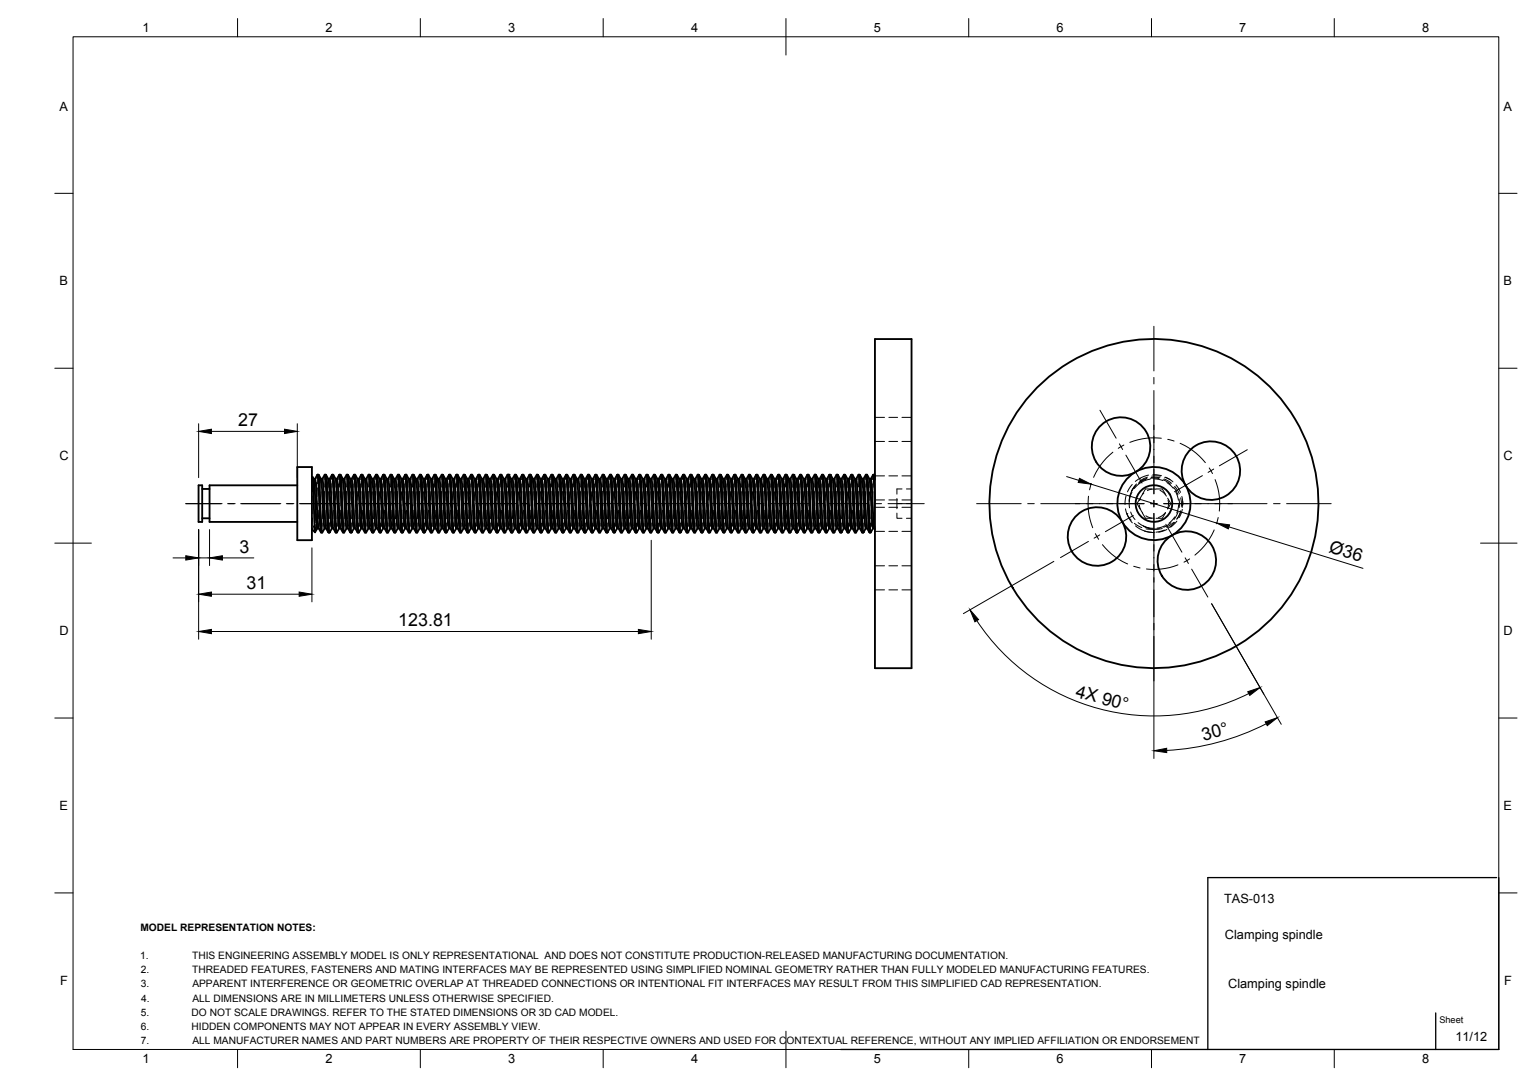
ISO-10303-21;
HEADER;
/* Generated by software containing ST-Developer
 * from STEP Tools, Inc. (www.steptools.com) 
 */

FILE_DESCRIPTION(
/* description */ (
'Independent guided parallel-jaw bracket clamp. Two12mm guide rods, re
placeable bronze sleeves, captured swiveling spindle, replaceable jaw 
pads and modeled M16x2 screw. Native slider/revolute joints linked2mm 
per revolution. Nominal opening0..122 with initial28mm. Base and two i
dentical supports welded. Standard fits, weld details and clamp load r
equire engineering selection.'),
/* implementation_level */ '2;1');

FILE_NAME(
/* name */ 'Clamping spindle.step',
/* time_stamp */ '2026-11-14T09:15:44-08:00',
/* author */ (''),
/* organization */ (''),
/* preprocessor_version */ 'ST-DEVELOPER v20.2',
/* originating_system */ 'Autodesk Translation Framework v15.17.0.0',
/* authorisation */ '');

FILE_SCHEMA (('AUTOMOTIVE_DESIGN { 1 0 10303 214 3 1 1 }'));
ENDSEC;

DATA;
#10=MECHANICAL_DESIGN_GEOMETRIC_PRESENTATION_REPRESENTATION('',(#918),#105806);
#95=B_SPLINE_SURFACE_WITH_KNOTS('',3,3,((#67139,#67140,#67141,#67142,#67143,
#67144,#67145,#67146,#67147,#67148,#67149,#67150,#67151,#67152,#67153,#67154,
#67155,#67156,#67157,#67158,#67159,#67160,#67161,#67162,#67163,#67164,#67165,
#67166,#67167,#67168,#67169,#67170,#67171,#67172,#67173,#67174,#67175,#67176,
#67177,#67178,#67179,#67180,#67181,#67182,#67183,#67184,#67185,#67186,#67187,
#67188,#67189,#67190,#67191,#67192,#67193,#67194,#67195,#67196,#67197,#67198,
#67199,#67200,#67201,#67202,#67203,#67204,#67205,#67206,#67207,#67208,#67209,
#67210,#67211,#67212,#67213,#67214,#67215,#67216,#67217,#67218,#67219,#67220,
#67221,#67222,#67223,#67224,#67225,#67226,#67227,#67228,#67229,#67230,#67231,
#67232,#67233,#67234,#67235,#67236,#67237,#67238,#67239,#67240,#67241,#67242,
#67243,#67244,#67245,#67246,#67247,#67248,#67249,#67250,#67251,#67252,#67253,
#67254,#67255,#67256,#67257,#67258,#67259,#67260,#67261,#67262,#67263,#67264,
#67265,#67266,#67267,#67268,#67269,#67270,#67271,#67272,#67273,#67274,#67275,
#67276,#67277,#67278,#67279,#67280,#67281,#67282,#67283,#67284,#67285,#67286,
#67287,#67288,#67289,#67290,#67291,#67292,#67293,#67294,#67295,#67296,#67297,
#67298,#67299,#67300,#67301,#67302,#67303,#67304,#67305,#67306,#67307,#67308,
#67309,#67310,#67311,#67312,#67313,#67314,#67315,#67316,#67317,#67318,#67319,
#67320,#67321,#67322,#67323,#67324,#67325,#67326,#67327,#67328,#67329,#67330,
#67331,#67332,#67333,#67334,#67335,#67336,#67337,#67338,#67339,#67340,#67341,
#67342,#67343,#67344,#67345,#67346,#67347,#67348,#67349,#67350,#67351,#67352,
#67353,#67354,#67355,#67356,#67357,#67358,#67359,#67360,#67361,#67362,#67363,
#67364,#67365,#67366,#67367,#67368,#67369,#67370,#67371,#67372,#67373,#67374,
#67375,#67376,#67377,#67378,#67379,#67380,#67381,#67382,#67383,#67384,#67385,
#67386,#67387,#67388,#67389,#67390,#67391,#67392,#67393,#67394,#67395,#67396,
#67397,#67398,#67399,#67400,#67401,#67402,#67403,#67404,#67405,#67406,#67407,
#67408,#67409,#67410,#67411,#67412,#67413,#67414,#67415,#67416,#67417,#67418,
#67419,#67420,#67421,#67422,#67423,#67424,#67425,#67426,#67427,#67428,#67429,
#67430,#67431,#67432,#67433,#67434,#67435,#67436,#67437,#67438,#67439,#67440,
#67441,#67442,#67443,#67444,#67445,#67446,#67447,#67448,#67449,#67450,#67451,
#67452,#67453,#67454,#67455,#67456,#67457,#67458,#67459,#67460,#67461,#67462,
#67463,#67464,#67465,#67466,#67467,#67468,#67469,#67470,#67471,#67472,#67473,
#67474,#67475,#67476,#67477,#67478,#67479,#67480,#67481,#67482,#67483,#67484,
#67485,#67486,#67487,#67488,#67489,#67490,#67491,#67492,#67493,#67494,#67495,
#67496,#67497,#67498,#67499,#67500,#67501,#67502,#67503,#67504,#67505,#67506,
#67507,#67508,#67509,#67510,#67511,#67512,#67513,#67514,#67515,#67516,#67517,
#67518,#67519,#67520,#67521,#67522,#67523,#67524,#67525,#67526,#67527,#67528,
#67529,#67530,#67531,#67532,#67533,#67534,#67535,#67536,#67537,#67538,#67539,
#67540,#67541,#67542,#67543,#67544,#67545,#67546,#67547,#67548,#67549,#67550,
#67551,#67552,#67553,#67554,#67555,#67556,#67557,#67558,#67559,#67560,#67561,
#67562,#67563,#67564,#67565,#67566,#67567,#67568,#67569,#67570,#67571,#67572,
#67573,#67574,#67575,#67576,#67577,#67578,#67579,#67580,#67581,#67582,#67583,
#67584,#67585,#67586,#67587,#67588,#67589,#67590,#67591,#67592,#67593,#67594,
#67595,#67596,#67597,#67598,#67599,#67600,#67601,#67602,#67603,#67604,#67605,
#67606,#67607,#67608,#67609,#67610,#67611,#67612,#67613,#67614,#67615,#67616,
#67617,#67618,#67619,#67620,#67621,#67622,#67623,#67624,#67625,#67626,#67627,
#67628,#67629,#67630,#67631,#67632,#67633,#67634,#67635,#67636,#67637,#67638,
#67639,#67640,#67641,#67642,#67643,#67644,#67645,#67646,#67647,#67648,#67649,
#67650,#67651,#67652,#67653,#67654,#67655,#67656,#67657,#67658,#67659,#67660,
#67661,#67662,#67663,#67664,#67665,#67666,#67667,#67668,#67669,#67670,#67671,
#67672,#67673,#67674,#67675,#67676,#67677,#67678,#67679,#67680,#67681,#67682,
#67683,#67684,#67685,#67686,#67687,#67688,#67689,#67690,#67691,#67692,#67693,
#67694,#67695,#67696),(#67697,#67698,#67699,#67700,#67701,#67702,#67703,
#67704,#67705,#67706,#67707,#67708,#67709,#67710,#67711,#67712,#67713,#67714,
#67715,#67716,#67717,#67718,#67719,#67720,#67721,#67722,#67723,#67724,#67725,
#67726,#67727,#67728,#67729,#67730,#67731,#67732,#67733,#67734,#67735,#67736,
#67737,#67738,#67739,#67740,#67741,#67742,#67743,#67744,#67745,#67746,#67747,
#67748,#67749,#67750,#67751,#67752,#67753,#67754,#67755,#67756,#67757,#67758,
#67759,#67760,#67761,#67762,#67763,#67764,#67765,#67766,#67767,#67768,#67769,
#67770,#67771,#67772,#67773,#67774,#67775,#67776,#67777,#67778,#67779,#67780,
#67781,#67782,#67783,#67784,#67785,#67786,#67787,#67788,#67789,#67790,#67791,
#67792,#67793,#67794,#67795,#67796,#67797,#67798,#67799,#67800,#67801,#67802,
#67803,#67804,#67805,#67806,#67807,#67808,#67809,#67810,#67811,#67812,#67813,
#67814,#67815,#67816,#67817,#67818,#67819,#67820,#67821,#67822,#67823,#67824,
#67825,#67826,#67827,#67828,#67829,#67830,#67831,#67832,#67833,#67834,#67835,
#67836,#67837,#67838,#67839,#67840,#67841,#67842,#67843,#67844,#67845,#67846,
#67847,#67848,#67849,#67850,#67851,#67852,#67853,#67854,#67855,#67856,#67857,
#67858,#67859,#67860,#67861,#67862,#67863,#67864,#67865,#67866,#67867,#67868,
#67869,#67870,#67871,#67872,#67873,#67874,#67875,#67876,#67877,#67878,#67879,
#67880,#67881,#67882,#67883,#67884,#67885,#67886,#67887,#67888,#67889,#67890,
#67891,#67892,#67893,#67894,#67895,#67896,#67897,#67898,#67899,#67900,#67901,
#67902,#67903,#67904,#67905,#67906,#67907,#67908,#67909,#67910,#67911,#67912,
#67913,#67914,#67915,#67916,#67917,#67918,#67919,#67920,#67921,#67922,#67923,
#67924,#67925,#67926,#67927,#67928,#67929,#67930,#67931,#67932,#67933,#67934,
#67935,#67936,#67937,#67938,#67939,#67940,#67941,#67942,#67943,#67944,#67945,
#67946,#67947,#67948,#67949,#67950,#67951,#67952,#67953,#67954,#67955,#67956,
#67957,#67958,#67959,#67960,#67961,#67962,#67963,#67964,#67965,#67966,#67967,
#67968,#67969,#67970,#67971,#67972,#67973,#67974,#67975,#67976,#67977,#67978,
#67979,#67980,#67981,#67982,#67983,#67984,#67985,#67986,#67987,#67988,#67989,
#67990,#67991,#67992,#67993,#67994,#67995,#67996,#67997,#67998,#67999,#68000,
#68001,#68002,#68003,#68004,#68005,#68006,#68007,#68008,#68009,#68010,#68011,
#68012,#68013,#68014,#68015,#68016,#68017,#68018,#68019,#68020,#68021,#68022,
#68023,#68024,#68025,#68026,#68027,#68028,#68029,#68030,#68031,#68032,#68033,
#68034,#68035,#68036,#68037,#68038,#68039,#68040,#68041,#68042,#68043,#68044,
#68045,#68046,#68047,#68048,#68049,#68050,#68051,#68052,#68053,#68054,#68055,
#68056,#68057,#68058,#68059,#68060,#68061,#68062,#68063,#68064,#68065,#68066,
#68067,#68068,#68069,#68070,#68071,#68072,#68073,#68074,#68075,#68076,#68077,
#68078,#68079,#68080,#68081,#68082,#68083,#68084,#68085,#68086,#68087,#68088,
#68089,#68090,#68091,#68092,#68093,#68094,#68095,#68096,#68097,#68098,#68099,
#68100,#68101,#68102,#68103,#68104,#68105,#68106,#68107,#68108,#68109,#68110,
#68111,#68112,#68113,#68114,#68115,#68116,#68117,#68118,#68119,#68120,#68121,
#68122,#68123,#68124,#68125,#68126,#68127,#68128,#68129,#68130,#68131,#68132,
#68133,#68134,#68135,#68136,#68137,#68138,#68139,#68140,#68141,#68142,#68143,
#68144,#68145,#68146,#68147,#68148,#68149,#68150,#68151,#68152,#68153,#68154,
#68155,#68156,#68157,#68158,#68159,#68160,#68161,#68162,#68163,#68164,#68165,
#68166,#68167,#68168,#68169,#68170,#68171,#68172,#68173,#68174,#68175,#68176,
#68177,#68178,#68179,#68180,#68181,#68182,#68183,#68184,#68185,#68186,#68187,
#68188,#68189,#68190,#68191,#68192,#68193,#68194,#68195,#68196,#68197,#68198,
#68199,#68200,#68201,#68202,#68203,#68204,#68205,#68206,#68207,#68208,#68209,
#68210,#68211,#68212,#68213,#68214,#68215,#68216,#68217,#68218,#68219,#68220,
#68221,#68222,#68223,#68224,#68225,#68226,#68227,#68228,#68229,#68230,#68231,
#68232,#68233,#68234,#68235,#68236,#68237,#68238,#68239,#68240,#68241,#68242,
#68243,#68244,#68245,#68246,#68247,#68248,#68249,#68250,#68251,#68252,#68253,
#68254),(#68255,#68256,#68257,#68258,#68259,#68260,#68261,#68262,#68263,
#68264,#68265,#68266,#68267,#68268,#68269,#68270,#68271,#68272,#68273,#68274,
#68275,#68276,#68277,#68278,#68279,#68280,#68281,#68282,#68283,#68284,#68285,
#68286,#68287,#68288,#68289,#68290,#68291,#68292,#68293,#68294,#68295,#68296,
#68297,#68298,#68299,#68300,#68301,#68302,#68303,#68304,#68305,#68306,#68307,
#68308,#68309,#68310,#68311,#68312,#68313,#68314,#68315,#68316,#68317,#68318,
#68319,#68320,#68321,#68322,#68323,#68324,#68325,#68326,#68327,#68328,#68329,
#68330,#68331,#68332,#68333,#68334,#68335,#68336,#68337,#68338,#68339,#68340,
#68341,#68342,#68343,#68344,#68345,#68346,#68347,#68348,#68349,#68350,#68351,
#68352,#68353,#68354,#68355,#68356,#68357,#68358,#68359,#68360,#68361,#68362,
#68363,#68364,#68365,#68366,#68367,#68368,#68369,#68370,#68371,#68372,#68373,
#68374,#68375,#68376,#68377,#68378,#68379,#68380,#68381,#68382,#68383,#68384,
#68385,#68386,#68387,#68388,#68389,#68390,#68391,#68392,#68393,#68394,#68395,
#68396,#68397,#68398,#68399,#68400,#68401,#68402,#68403,#68404,#68405,#68406,
#68407,#68408,#68409,#68410,#68411,#68412,#68413,#68414,#68415,#68416,#68417,
#68418,#68419,#68420,#68421,#68422,#68423,#68424,#68425,#68426,#68427,#68428,
#68429,#68430,#68431,#68432,#68433,#68434,#68435,#68436,#68437,#68438,#68439,
#68440,#68441,#68442,#68443,#68444,#68445,#68446,#68447,#68448,#68449,#68450,
#68451,#68452,#68453,#68454,#68455,#68456,#68457,#68458,#68459,#68460,#68461,
#68462,#68463,#68464,#68465,#68466,#68467,#68468,#68469,#68470,#68471,#68472,
#68473,#68474,#68475,#68476,#68477,#68478,#68479,#68480,#68481,#68482,#68483,
#68484,#68485,#68486,#68487,#68488,#68489,#68490,#68491,#68492,#68493,#68494,
#68495,#68496,#68497,#68498,#68499,#68500,#68501,#68502,#68503,#68504,#68505,
#68506,#68507,#68508,#68509,#68510,#68511,#68512,#68513,#68514,#68515,#68516,
#68517,#68518,#68519,#68520,#68521,#68522,#68523,#68524,#68525,#68526,#68527,
#68528,#68529,#68530,#68531,#68532,#68533,#68534,#68535,#68536,#68537,#68538,
#68539,#68540,#68541,#68542,#68543,#68544,#68545,#68546,#68547,#68548,#68549,
#68550,#68551,#68552,#68553,#68554,#68555,#68556,#68557,#68558,#68559,#68560,
#68561,#68562,#68563,#68564,#68565,#68566,#68567,#68568,#68569,#68570,#68571,
#68572,#68573,#68574,#68575,#68576,#68577,#68578,#68579,#68580,#68581,#68582,
#68583,#68584,#68585,#68586,#68587,#68588,#68589,#68590,#68591,#68592,#68593,
#68594,#68595,#68596,#68597,#68598,#68599,#68600,#68601,#68602,#68603,#68604,
#68605,#68606,#68607,#68608,#68609,#68610,#68611,#68612,#68613,#68614,#68615,
#68616,#68617,#68618,#68619,#68620,#68621,#68622,#68623,#68624,#68625,#68626,
#68627,#68628,#68629,#68630,#68631,#68632,#68633,#68634,#68635,#68636,#68637,
#68638,#68639,#68640,#68641,#68642,#68643,#68644,#68645,#68646,#68647,#68648,
#68649,#68650,#68651,#68652,#68653,#68654,#68655,#68656,#68657,#68658,#68659,
#68660,#68661,#68662,#68663,#68664,#68665,#68666,#68667,#68668,#68669,#68670,
#68671,#68672,#68673,#68674,#68675,#68676,#68677,#68678,#68679,#68680,#68681,
#68682,#68683,#68684,#68685,#68686,#68687,#68688,#68689,#68690,#68691,#68692,
#68693,#68694,#68695,#68696,#68697,#68698,#68699,#68700,#68701,#68702,#68703,
#68704,#68705,#68706,#68707,#68708,#68709,#68710,#68711,#68712,#68713,#68714,
#68715,#68716,#68717,#68718,#68719,#68720,#68721,#68722,#68723,#68724,#68725,
#68726,#68727,#68728,#68729,#68730,#68731,#68732,#68733,#68734,#68735,#68736,
#68737,#68738,#68739,#68740,#68741,#68742,#68743,#68744,#68745,#68746,#68747,
#68748,#68749,#68750,#68751,#68752,#68753,#68754,#68755,#68756,#68757,#68758,
#68759,#68760,#68761,#68762,#68763,#68764,#68765,#68766,#68767,#68768,#68769,
#68770,#68771,#68772,#68773,#68774,#68775,#68776,#68777,#68778,#68779,#68780,
#68781,#68782,#68783,#68784,#68785,#68786,#68787,#68788,#68789,#68790,#68791,
#68792,#68793,#68794,#68795,#68796,#68797,#68798,#68799,#68800,#68801,#68802,
#68803,#68804,#68805,#68806,#68807,#68808,#68809,#68810,#68811,#68812),
(#68813,#68814,#68815,#68816,#68817,#68818,#68819,#68820,#68821,#68822,
#68823,#68824,#68825,#68826,#68827,#68828,#68829,#68830,#68831,#68832,#68833,
#68834,#68835,#68836,#68837,#68838,#68839,#68840,#68841,#68842,#68843,#68844,
#68845,#68846,#68847,#68848,#68849,#68850,#68851,#68852,#68853,#68854,#68855,
#68856,#68857,#68858,#68859,#68860,#68861,#68862,#68863,#68864,#68865,#68866,
#68867,#68868,#68869,#68870,#68871,#68872,#68873,#68874,#68875,#68876,#68877,
#68878,#68879,#68880,#68881,#68882,#68883,#68884,#68885,#68886,#68887,#68888,
#68889,#68890,#68891,#68892,#68893,#68894,#68895,#68896,#68897,#68898,#68899,
#68900,#68901,#68902,#68903,#68904,#68905,#68906,#68907,#68908,#68909,#68910,
#68911,#68912,#68913,#68914,#68915,#68916,#68917,#68918,#68919,#68920,#68921,
#68922,#68923,#68924,#68925,#68926,#68927,#68928,#68929,#68930,#68931,#68932,
#68933,#68934,#68935,#68936,#68937,#68938,#68939,#68940,#68941,#68942,#68943,
#68944,#68945,#68946,#68947,#68948,#68949,#68950,#68951,#68952,#68953,#68954,
#68955,#68956,#68957,#68958,#68959,#68960,#68961,#68962,#68963,#68964,#68965,
#68966,#68967,#68968,#68969,#68970,#68971,#68972,#68973,#68974,#68975,#68976,
#68977,#68978,#68979,#68980,#68981,#68982,#68983,#68984,#68985,#68986,#68987,
#68988,#68989,#68990,#68991,#68992,#68993,#68994,#68995,#68996,#68997,#68998,
#68999,#69000,#69001,#69002,#69003,#69004,#69005,#69006,#69007,#69008,#69009,
#69010,#69011,#69012,#69013,#69014,#69015,#69016,#69017,#69018,#69019,#69020,
#69021,#69022,#69023,#69024,#69025,#69026,#69027,#69028,#69029,#69030,#69031,
#69032,#69033,#69034,#69035,#69036,#69037,#69038,#69039,#69040,#69041,#69042,
#69043,#69044,#69045,#69046,#69047,#69048,#69049,#69050,#69051,#69052,#69053,
#69054,#69055,#69056,#69057,#69058,#69059,#69060,#69061,#69062,#69063,#69064,
#69065,#69066,#69067,#69068,#69069,#69070,#69071,#69072,#69073,#69074,#69075,
#69076,#69077,#69078,#69079,#69080,#69081,#69082,#69083,#69084,#69085,#69086,
#69087,#69088,#69089,#69090,#69091,#69092,#69093,#69094,#69095,#69096,#69097,
#69098,#69099,#69100,#69101,#69102,#69103,#69104,#69105,#69106,#69107,#69108,
#69109,#69110,#69111,#69112,#69113,#69114,#69115,#69116,#69117,#69118,#69119,
#69120,#69121,#69122,#69123,#69124,#69125,#69126,#69127,#69128,#69129,#69130,
#69131,#69132,#69133,#69134,#69135,#69136,#69137,#69138,#69139,#69140,#69141,
#69142,#69143,#69144,#69145,#69146,#69147,#69148,#69149,#69150,#69151,#69152,
#69153,#69154,#69155,#69156,#69157,#69158,#69159,#69160,#69161,#69162,#69163,
#69164,#69165,#69166,#69167,#69168,#69169,#69170,#69171,#69172,#69173,#69174,
#69175,#69176,#69177,#69178,#69179,#69180,#69181,#69182,#69183,#69184,#69185,
#69186,#69187,#69188,#69189,#69190,#69191,#69192,#69193,#69194,#69195,#69196,
#69197,#69198,#69199,#69200,#69201,#69202,#69203,#69204,#69205,#69206,#69207,
#69208,#69209,#69210,#69211,#69212,#69213,#69214,#69215,#69216,#69217,#69218,
#69219,#69220,#69221,#69222,#69223,#69224,#69225,#69226,#69227,#69228,#69229,
#69230,#69231,#69232,#69233,#69234,#69235,#69236,#69237,#69238,#69239,#69240,
#69241,#69242,#69243,#69244,#69245,#69246,#69247,#69248,#69249,#69250,#69251,
#69252,#69253,#69254,#69255,#69256,#69257,#69258,#69259,#69260,#69261,#69262,
#69263,#69264,#69265,#69266,#69267,#69268,#69269,#69270,#69271,#69272,#69273,
#69274,#69275,#69276,#69277,#69278,#69279,#69280,#69281,#69282,#69283,#69284,
#69285,#69286,#69287,#69288,#69289,#69290,#69291,#69292,#69293,#69294,#69295,
#69296,#69297,#69298,#69299,#69300,#69301,#69302,#69303,#69304,#69305,#69306,
#69307,#69308,#69309,#69310,#69311,#69312,#69313,#69314,#69315,#69316,#69317,
#69318,#69319,#69320,#69321,#69322,#69323,#69324,#69325,#69326,#69327,#69328,
#69329,#69330,#69331,#69332,#69333,#69334,#69335,#69336,#69337,#69338,#69339,
#69340,#69341,#69342,#69343,#69344,#69345,#69346,#69347,#69348,#69349,#69350,
#69351,#69352,#69353,#69354,#69355,#69356,#69357,#69358,#69359,#69360,#69361,
#69362,#69363,#69364,#69365,#69366,#69367,#69368,#69369,#69370)),
 .UNSPECIFIED.,.F.,.F.,.F.,(4,4),(4,1,1,1,1,1,1,1,1,1,1,1,1,1,1,1,1,1,1,
1,1,1,1,1,1,1,1,1,1,1,1,1,1,1,1,1,1,1,1,1,1,1,1,1,1,1,1,1,1,1,1,1,1,1,1,
1,1,1,1,1,1,1,1,1,1,1,1,1,1,1,1,1,1,1,1,1,1,1,1,1,1,1,1,1,1,1,1,1,1,1,1,
1,1,1,1,1,1,1,1,1,1,1,1,1,1,1,1,1,1,1,1,1,1,1,1,1,1,1,1,1,1,1,1,1,1,1,1,
1,1,1,1,1,1,1,1,1,1,1,1,1,1,1,1,1,1,1,1,1,1,1,1,1,1,1,1,1,1,1,1,1,1,1,1,
1,1,1,1,1,1,1,1,1,1,1,1,1,1,1,1,1,1,1,1,1,1,1,1,1,1,1,1,1,1,1,1,1,1,1,1,
1,1,1,1,1,1,1,1,1,1,1,1,1,1,1,1,1,1,1,1,1,1,1,1,1,1,1,1,1,1,1,1,1,1,1,1,
1,1,1,1,1,1,1,1,1,1,1,1,1,1,1,1,1,1,1,1,1,1,1,1,1,1,1,1,1,1,1,1,1,1,1,1,
1,1,1,1,1,1,1,1,1,1,1,1,1,1,1,1,1,1,1,1,1,1,1,1,1,1,1,1,1,1,1,1,1,1,1,1,
1,1,1,1,1,1,1,1,1,1,1,1,1,1,1,1,1,1,1,1,1,1,1,1,1,1,1,1,1,1,1,1,1,1,1,1,
1,1,1,1,1,1,1,1,1,1,1,1,1,1,1,1,1,1,1,1,1,1,1,1,1,1,1,1,1,1,1,1,1,1,1,1,
1,1,1,1,1,1,1,1,1,1,1,1,1,1,1,1,1,1,1,1,1,1,1,1,1,1,1,1,1,1,1,1,1,1,1,1,
1,1,1,1,1,1,1,1,1,1,1,1,1,1,1,1,1,1,1,1,1,1,1,1,1,1,1,1,1,1,1,1,1,1,1,1,
1,1,1,1,1,1,1,1,1,1,1,1,1,1,1,1,1,1,1,1,1,1,1,1,1,1,1,1,1,1,1,1,1,1,1,1,
1,1,1,1,1,1,1,1,1,1,1,1,1,1,1,1,1,1,1,1,1,1,1,1,1,1,1,1,1,1,1,1,1,1,1,1,
1,1,1,1,1,1,1,1,1,1,1,1,1,1,1,1,1,1,1,1,1,1,1,1,1,1,1,1,1,1,1,1,4),(-0.00312009804042434,
0.132901482941916),(11.6144980695961,12.1142368518449,12.6134408558704,
13.6118488639213,14.6102568719722,15.6086648800232,16.6070728880741,17.605480896125,
18.1046849001504,18.6038889041759,19.6022969122268,20.6007049202777,21.5991129283287,
22.5975209363796,23.5959289444305,24.5943369524814,25.0935409565069,25.5927449605323,
26.5911529685832,27.5895609766342,28.5879689846851,29.586376992736,30.5847850007869,
31.5831930088378,32.0823970128633,32.5816010168887,33.5800090249397,34.5784170329906,
35.5768250410415,36.5752330490924,37.5736410571433,38.5720490651942,39.0712530692197,
39.5704570732452,40.5688650812961,41.567273089347,42.5656810973979,43.5640891054488,
44.5624971134997,45.5609051215507,46.0601091255761,46.5593131296016,47.5577211376525,
48.5561291457034,49.5545371537543,50.5529451618052,51.5513531698562,52.5497611779071,
53.0489651819325,53.548169185958,54.5465771940089,55.5449852020598,56.5433932101108,
57.5418012181617,58.5402092262126,59.5386172342635,60.037821238289,60.5370252423144,
61.5354332503653,62.5338412584163,63.5322492664672,64.5306572745181,65.529065282569,
66.5274732906199,67.0266772946454,67.5258812986708,68.5242893067218,69.5226973147727,
70.5211053228236,71.5195133308745,72.5179213389254,73.5163293469763,74.0155333510018,
74.5147373550273,75.5131453630782,76.5115533711291,77.50996137918,78.5083693872309,
79.5067773952818,80.5051854033328,81.0043894073582,81.5035934113837,82.5020014194346,
83.5004094274855,84.4988174355364,85.4972254435874,86.4956334516383,87.4940414596892,
87.9932454637146,88.4924494677401,89.490857475791,90.4892654838419,91.4876734918928,
92.4860814999438,93.4844895079947,94.4828975160456,94.9821015200711,95.4813055240965,
96.4797135321474,97.4781215401984,98.4765295482493,99.4749375563002,100.473345564351,
101.471753572402,101.970957576427,102.470161580453,103.468569588504,104.466977596555,
105.465385604606,106.463793612657,107.462201620708,108.460609628758,108.959813632784,
109.459017636809,110.45742564486,111.455833652911,112.454241660962,113.452649669013,
114.451057677064,115.449465685115,115.94866968914,116.447873693166,117.446281701217,
118.444689709268,119.443097717319,120.441505725369,121.43991373342,122.438321741471,
122.937525745497,123.436729749522,124.435137757573,125.433545765624,126.431953773675,
127.430361781726,128.428769789777,129.427177797828,129.926381801853,130.425585805879,
131.42399381393,132.42240182198,133.420809830031,134.419217838082,135.417625846133,
136.416033854184,136.91523785821,137.414441862235,138.412849870286,139.411257878337,
140.409665886388,141.408073894439,142.40648190249,143.404889910541,143.904093914566,
144.403297918591,145.401705926642,146.400113934693,147.398521942744,148.396929950795,
149.395337958846,150.393745966897,150.892949970922,151.392153974948,152.390561982999,
153.38896999105,154.387377999101,155.385786007152,156.384194015202,157.382602023253,
157.881806027279,158.381010031304,159.379418039355,160.377826047406,161.376234055457,
162.374642063508,163.373050071559,164.37145807961,164.870662083635,165.369866087661,
166.368274095712,167.366682103763,168.365090111813,169.363498119864,170.361906127915,
171.360314135966,171.859518139992,172.358722144017,173.357130152068,174.355538160119,
175.35394616817,176.352354176221,177.350762184272,178.349170192323,178.848374196348,
179.347578200374,180.345986208424,181.344394216475,182.342802224526,183.341210232577,
184.339618240628,185.338026248679,185.837230252705,186.33643425673,187.334842264781,
188.333250272832,189.331658280883,190.330066288934,191.328474296985,192.326882305035,
192.826086309061,193.325290313086,194.323698321137,195.322106329188,196.320514337239,
197.31892234529,198.317330353341,199.315738361392,199.814942365417,200.314146369443,
201.312554377494,202.310962385545,203.309370393596,204.307778401646,205.306186409697,
206.304594417748,206.803798421774,207.303002425799,208.30141043385,209.299818441901,
210.298226449952,211.296634458003,212.295042466054,213.293450474105,213.79265447813,
214.291858482156,215.290266490207,216.288674498257,217.287082506308,218.285490514359,
219.28389852241,220.282306530461,220.781510534487,221.280714538512,222.279122546563,
223.277530554614,224.275938562665,225.274346570716,226.272754578767,227.271162586818,
227.770366590843,228.269570594868,229.267978602919,230.26638661097,231.264794619021,
232.263202627072,233.261610635123,234.260018643174,234.759222647199,235.258426651225,
236.256834659276,237.255242667327,238.253650675378,239.252058683429,240.250466691479,
241.24887469953,241.748078703556,242.247282707581,243.245690715632,244.244098723683,
245.242506731734,246.240914739785,247.239322747836,248.237730755887,248.736934759912,
249.236138763938,250.234546771989,251.23295478004,252.23136278809,253.229770796141,
254.228178804192,255.226586812243,256.224994820294,257.223402828345,258.221810836396,
258.721014840421,259.220218844447,260.218626852498,261.217034860549,262.2154428686,
263.213850876651,264.212258884701,265.210666892752,265.709870896778,266.209074900803,
267.207482908854,268.205890916905,269.204298924956,270.202706933007,271.201114941058,
272.199522949109,272.698726953134,273.19793095716,274.196338965211,275.194746973262,
276.193154981312,277.191562989363,278.189970997414,279.188379005465,279.687583009491,
280.186787013516,281.185195021567,282.183603029618,283.182011037669,284.18041904572,
285.178827053771,286.177235061822,286.676439065847,287.175643069873,288.174051077923,
289.172459085974,290.170867094025,291.169275102076,292.167683110127,293.166091118178,
293.665295122204,294.164499126229,295.16290713428,296.161315142331,297.159723150382,
298.158131158433,299.156539166484,300.154947174534,300.65415117856,301.153355182585,
302.151763190636,303.150171198687,304.148579206738,305.146987214789,306.14539522284,
307.143803230891,307.643007234916,308.142211238942,309.140619246993,310.139027255044,
311.137435263095,312.135843271145,313.134251279196,314.132659287247,314.631863291273,
315.131067295298,316.129475303349,317.1278833114,318.126291319451,319.124699327502,
320.123107335553,321.121515343604,321.620719347629,322.119923351655,323.118331359706,
324.116739367757,325.115147375807,326.113555383858,327.111963391909,328.11037139996,
328.609575403986,329.108779408011,330.107187416062,331.105595424113,332.104003432164,
333.102411440215,334.100819448266,335.099227456317,335.598431460342,336.097635464367,
337.096043472418,338.094451480469,339.09285948852,340.091267496571,341.089675504622,
342.088083512673,342.587287516698,343.086491520724,344.084899528775,345.083307536826,
346.081715544877,347.080123552928,348.078531560978,349.076939569029,349.576143573055,
350.07534757708,351.073755585131,352.072163593182,353.070571601233,354.068979609284,
355.067387617335,356.065795625386,356.564999629411,357.064203633437,358.062611641488,
359.061019649539,360.059427657589,361.05783566564,362.056243673691,363.054651681742,
363.553855685768,364.053059689793,365.051467697844,366.049875705895,367.048283713946,
368.046691721997,369.045099730048,370.043507738099,370.542711742124,371.04191574615,
372.040323754201,373.038731762251,374.037139770302,375.035547778353,376.033955786404,
377.032363794455,377.531567798481,378.030771802506,379.029179810557,380.027587818608,
381.025995826659,382.02440383471,383.022811842761,384.021219850812,384.520423854837,
385.019627858862,386.018035866913,387.016443874964,388.014851883015,389.013259891066,
390.011667899117,391.010075907168,391.509279911193,392.008483915219,393.00689192327,
394.005299931321,395.003707939372,396.002115947423,397.000523955473,397.998931963524,
398.49813596755,398.997339971575,399.995747979626,400.994155987677,401.992563995728,
402.990972003779,403.98938001183,404.987788019881,405.486992023906,405.986196027932,
406.984604035983,407.983012044034,408.981420052084,409.979828060135,410.978236068186,
411.976644076237,412.475848080263,412.975052084288,413.973460092339,414.97186810039,
415.970276108441,416.968684116492,417.967092124543,418.965500132594,419.464704136619,
419.963908140644,420.962316148695,421.960724156746,422.959132164797,423.957540172848,
424.955948180899,425.95435618895,426.453560192975,426.952764197001,427.951172205052,
428.949580213103,429.947988221154,430.946396229205,431.944804237256,432.943212245306,
433.442416249332,433.941620253357,434.940028261408,435.938436269459,436.93684427751,
437.935252285561,438.933660293612,439.932068301663,440.431272305688,440.930476309714,
441.928884317765,442.927292325816,443.925700333867,444.924108341917,445.922516349968,
446.920924358019,447.420128362045,447.91933236607,448.917740374121,449.916148382172,
450.914556390223,451.912964398274,452.911372406325,453.909780414376,454.408984418401,
454.908188422427,455.906596430478,456.905004438528,457.903412446579,458.90182045463,
459.900228462681,460.898636470732,461.397840474758,461.897044478783,462.895452486834,
463.893860494885,464.892268502936,465.890676510987,466.889084519038,467.887492527089,
468.386696531114,468.885900535139,469.88430854319,470.882716551241,471.881124559292,
472.879532567343,473.877940575394,474.876348583445,475.37555258747,475.874756591496,
476.873164599547,477.871572607598,478.869980615649,479.8683886237,480.86679663175,
481.865204639801,482.364408643827,482.863612647852,483.862020655903,484.860428663954,
485.858836672005,486.857244680056,487.855652688107,488.854060696158,489.353264700183,
489.852468704209,490.85087671226,491.849284720311,492.847692728361,493.846100736412,
494.844508744463,495.343712748489,495.842949180242),.UNSPECIFIED.);
#96=B_SPLINE_SURFACE_WITH_KNOTS('',3,3,((#69480,#69481,#69482,#69483,#69484,
#69485,#69486,#69487,#69488,#69489,#69490,#69491,#69492,#69493,#69494,#69495,
#69496,#69497,#69498,#69499,#69500,#69501,#69502,#69503,#69504,#69505,#69506,
#69507,#69508,#69509,#69510,#69511,#69512,#69513,#69514,#69515,#69516,#69517,
#69518,#69519,#69520,#69521,#69522,#69523,#69524,#69525,#69526,#69527,#69528,
#69529,#69530,#69531,#69532,#69533,#69534,#69535,#69536,#69537,#69538,#69539,
#69540,#69541,#69542,#69543,#69544,#69545,#69546,#69547,#69548,#69549,#69550,
#69551,#69552,#69553,#69554,#69555,#69556,#69557,#69558,#69559,#69560,#69561,
#69562,#69563,#69564,#69565,#69566,#69567,#69568,#69569,#69570,#69571,#69572,
#69573,#69574,#69575,#69576,#69577,#69578,#69579,#69580,#69581,#69582,#69583,
#69584,#69585,#69586,#69587,#69588,#69589,#69590,#69591,#69592,#69593,#69594,
#69595,#69596,#69597,#69598,#69599,#69600,#69601,#69602,#69603,#69604,#69605,
#69606,#69607,#69608,#69609,#69610,#69611,#69612,#69613,#69614,#69615,#69616,
#69617,#69618,#69619,#69620,#69621,#69622,#69623,#69624,#69625,#69626,#69627,
#69628,#69629,#69630,#69631,#69632,#69633,#69634,#69635,#69636,#69637,#69638,
#69639,#69640,#69641,#69642,#69643,#69644,#69645,#69646,#69647,#69648,#69649,
#69650,#69651,#69652,#69653,#69654,#69655,#69656,#69657,#69658,#69659,#69660,
#69661,#69662,#69663,#69664,#69665,#69666,#69667,#69668,#69669,#69670,#69671,
#69672,#69673,#69674,#69675,#69676,#69677,#69678,#69679,#69680,#69681,#69682,
#69683,#69684,#69685,#69686,#69687,#69688,#69689,#69690,#69691,#69692,#69693,
#69694,#69695,#69696,#69697,#69698,#69699,#69700,#69701,#69702,#69703,#69704,
#69705,#69706,#69707,#69708,#69709,#69710,#69711,#69712,#69713,#69714,#69715,
#69716,#69717,#69718,#69719,#69720,#69721,#69722,#69723,#69724,#69725,#69726,
#69727,#69728,#69729,#69730,#69731,#69732,#69733,#69734,#69735,#69736,#69737,
#69738,#69739,#69740,#69741,#69742,#69743,#69744,#69745,#69746,#69747,#69748,
#69749,#69750,#69751,#69752,#69753,#69754,#69755,#69756,#69757,#69758,#69759,
#69760,#69761,#69762,#69763,#69764,#69765,#69766,#69767,#69768,#69769,#69770,
#69771,#69772,#69773,#69774,#69775,#69776,#69777,#69778,#69779,#69780,#69781,
#69782,#69783,#69784,#69785,#69786,#69787,#69788,#69789,#69790,#69791,#69792,
#69793,#69794,#69795,#69796,#69797,#69798,#69799,#69800,#69801,#69802,#69803,
#69804,#69805,#69806,#69807,#69808,#69809,#69810,#69811,#69812,#69813,#69814,
#69815,#69816,#69817,#69818,#69819,#69820,#69821,#69822,#69823,#69824,#69825,
#69826,#69827,#69828,#69829,#69830,#69831,#69832,#69833,#69834,#69835,#69836,
#69837,#69838,#69839,#69840,#69841,#69842,#69843,#69844,#69845,#69846,#69847,
#69848,#69849,#69850,#69851,#69852,#69853,#69854,#69855,#69856,#69857,#69858,
#69859,#69860,#69861,#69862,#69863,#69864,#69865,#69866,#69867,#69868,#69869,
#69870,#69871,#69872,#69873,#69874,#69875,#69876,#69877,#69878,#69879,#69880,
#69881,#69882,#69883,#69884,#69885,#69886,#69887,#69888,#69889,#69890,#69891,
#69892,#69893,#69894,#69895,#69896,#69897,#69898,#69899,#69900,#69901,#69902,
#69903,#69904,#69905,#69906,#69907,#69908,#69909,#69910,#69911,#69912,#69913,
#69914,#69915,#69916,#69917,#69918,#69919,#69920,#69921,#69922,#69923,#69924,
#69925,#69926,#69927,#69928,#69929,#69930,#69931,#69932,#69933,#69934,#69935,
#69936,#69937,#69938,#69939,#69940,#69941,#69942,#69943,#69944,#69945,#69946,
#69947,#69948,#69949,#69950,#69951,#69952,#69953,#69954,#69955,#69956,#69957,
#69958,#69959,#69960,#69961,#69962,#69963,#69964,#69965,#69966,#69967,#69968,
#69969,#69970,#69971,#69972,#69973,#69974,#69975,#69976,#69977,#69978,#69979,
#69980,#69981,#69982,#69983,#69984,#69985,#69986,#69987,#69988,#69989,#69990,
#69991,#69992,#69993,#69994,#69995,#69996,#69997,#69998,#69999,#70000,#70001,
#70002,#70003,#70004,#70005,#70006,#70007,#70008,#70009,#70010,#70011,#70012,
#70013,#70014,#70015,#70016,#70017,#70018,#70019,#70020,#70021,#70022,#70023,
#70024,#70025,#70026,#70027,#70028,#70029,#70030,#70031,#70032,#70033,#70034,
#70035,#70036,#70037,#70038),(#70039,#70040,#70041,#70042,#70043,#70044,
#70045,#70046,#70047,#70048,#70049,#70050,#70051,#70052,#70053,#70054,#70055,
#70056,#70057,#70058,#70059,#70060,#70061,#70062,#70063,#70064,#70065,#70066,
#70067,#70068,#70069,#70070,#70071,#70072,#70073,#70074,#70075,#70076,#70077,
#70078,#70079,#70080,#70081,#70082,#70083,#70084,#70085,#70086,#70087,#70088,
#70089,#70090,#70091,#70092,#70093,#70094,#70095,#70096,#70097,#70098,#70099,
#70100,#70101,#70102,#70103,#70104,#70105,#70106,#70107,#70108,#70109,#70110,
#70111,#70112,#70113,#70114,#70115,#70116,#70117,#70118,#70119,#70120,#70121,
#70122,#70123,#70124,#70125,#70126,#70127,#70128,#70129,#70130,#70131,#70132,
#70133,#70134,#70135,#70136,#70137,#70138,#70139,#70140,#70141,#70142,#70143,
#70144,#70145,#70146,#70147,#70148,#70149,#70150,#70151,#70152,#70153,#70154,
#70155,#70156,#70157,#70158,#70159,#70160,#70161,#70162,#70163,#70164,#70165,
#70166,#70167,#70168,#70169,#70170,#70171,#70172,#70173,#70174,#70175,#70176,
#70177,#70178,#70179,#70180,#70181,#70182,#70183,#70184,#70185,#70186,#70187,
#70188,#70189,#70190,#70191,#70192,#70193,#70194,#70195,#70196,#70197,#70198,
#70199,#70200,#70201,#70202,#70203,#70204,#70205,#70206,#70207,#70208,#70209,
#70210,#70211,#70212,#70213,#70214,#70215,#70216,#70217,#70218,#70219,#70220,
#70221,#70222,#70223,#70224,#70225,#70226,#70227,#70228,#70229,#70230,#70231,
#70232,#70233,#70234,#70235,#70236,#70237,#70238,#70239,#70240,#70241,#70242,
#70243,#70244,#70245,#70246,#70247,#70248,#70249,#70250,#70251,#70252,#70253,
#70254,#70255,#70256,#70257,#70258,#70259,#70260,#70261,#70262,#70263,#70264,
#70265,#70266,#70267,#70268,#70269,#70270,#70271,#70272,#70273,#70274,#70275,
#70276,#70277,#70278,#70279,#70280,#70281,#70282,#70283,#70284,#70285,#70286,
#70287,#70288,#70289,#70290,#70291,#70292,#70293,#70294,#70295,#70296,#70297,
#70298,#70299,#70300,#70301,#70302,#70303,#70304,#70305,#70306,#70307,#70308,
#70309,#70310,#70311,#70312,#70313,#70314,#70315,#70316,#70317,#70318,#70319,
#70320,#70321,#70322,#70323,#70324,#70325,#70326,#70327,#70328,#70329,#70330,
#70331,#70332,#70333,#70334,#70335,#70336,#70337,#70338,#70339,#70340,#70341,
#70342,#70343,#70344,#70345,#70346,#70347,#70348,#70349,#70350,#70351,#70352,
#70353,#70354,#70355,#70356,#70357,#70358,#70359,#70360,#70361,#70362,#70363,
#70364,#70365,#70366,#70367,#70368,#70369,#70370,#70371,#70372,#70373,#70374,
#70375,#70376,#70377,#70378,#70379,#70380,#70381,#70382,#70383,#70384,#70385,
#70386,#70387,#70388,#70389,#70390,#70391,#70392,#70393,#70394,#70395,#70396,
#70397,#70398,#70399,#70400,#70401,#70402,#70403,#70404,#70405,#70406,#70407,
#70408,#70409,#70410,#70411,#70412,#70413,#70414,#70415,#70416,#70417,#70418,
#70419,#70420,#70421,#70422,#70423,#70424,#70425,#70426,#70427,#70428,#70429,
#70430,#70431,#70432,#70433,#70434,#70435,#70436,#70437,#70438,#70439,#70440,
#70441,#70442,#70443,#70444,#70445,#70446,#70447,#70448,#70449,#70450,#70451,
#70452,#70453,#70454,#70455,#70456,#70457,#70458,#70459,#70460,#70461,#70462,
#70463,#70464,#70465,#70466,#70467,#70468,#70469,#70470,#70471,#70472,#70473,
#70474,#70475,#70476,#70477,#70478,#70479,#70480,#70481,#70482,#70483,#70484,
#70485,#70486,#70487,#70488,#70489,#70490,#70491,#70492,#70493,#70494,#70495,
#70496,#70497,#70498,#70499,#70500,#70501,#70502,#70503,#70504,#70505,#70506,
#70507,#70508,#70509,#70510,#70511,#70512,#70513,#70514,#70515,#70516,#70517,
#70518,#70519,#70520,#70521,#70522,#70523,#70524,#70525,#70526,#70527,#70528,
#70529,#70530,#70531,#70532,#70533,#70534,#70535,#70536,#70537,#70538,#70539,
#70540,#70541,#70542,#70543,#70544,#70545,#70546,#70547,#70548,#70549,#70550,
#70551,#70552,#70553,#70554,#70555,#70556,#70557,#70558,#70559,#70560,#70561,
#70562,#70563,#70564,#70565,#70566,#70567,#70568,#70569,#70570,#70571,#70572,
#70573,#70574,#70575,#70576,#70577,#70578,#70579,#70580,#70581,#70582,#70583,
#70584,#70585,#70586,#70587,#70588,#70589,#70590,#70591,#70592,#70593,#70594,
#70595,#70596,#70597),(#70598,#70599,#70600,#70601,#70602,#70603,#70604,
#70605,#70606,#70607,#70608,#70609,#70610,#70611,#70612,#70613,#70614,#70615,
#70616,#70617,#70618,#70619,#70620,#70621,#70622,#70623,#70624,#70625,#70626,
#70627,#70628,#70629,#70630,#70631,#70632,#70633,#70634,#70635,#70636,#70637,
#70638,#70639,#70640,#70641,#70642,#70643,#70644,#70645,#70646,#70647,#70648,
#70649,#70650,#70651,#70652,#70653,#70654,#70655,#70656,#70657,#70658,#70659,
#70660,#70661,#70662,#70663,#70664,#70665,#70666,#70667,#70668,#70669,#70670,
#70671,#70672,#70673,#70674,#70675,#70676,#70677,#70678,#70679,#70680,#70681,
#70682,#70683,#70684,#70685,#70686,#70687,#70688,#70689,#70690,#70691,#70692,
#70693,#70694,#70695,#70696,#70697,#70698,#70699,#70700,#70701,#70702,#70703,
#70704,#70705,#70706,#70707,#70708,#70709,#70710,#70711,#70712,#70713,#70714,
#70715,#70716,#70717,#70718,#70719,#70720,#70721,#70722,#70723,#70724,#70725,
#70726,#70727,#70728,#70729,#70730,#70731,#70732,#70733,#70734,#70735,#70736,
#70737,#70738,#70739,#70740,#70741,#70742,#70743,#70744,#70745,#70746,#70747,
#70748,#70749,#70750,#70751,#70752,#70753,#70754,#70755,#70756,#70757,#70758,
#70759,#70760,#70761,#70762,#70763,#70764,#70765,#70766,#70767,#70768,#70769,
#70770,#70771,#70772,#70773,#70774,#70775,#70776,#70777,#70778,#70779,#70780,
#70781,#70782,#70783,#70784,#70785,#70786,#70787,#70788,#70789,#70790,#70791,
#70792,#70793,#70794,#70795,#70796,#70797,#70798,#70799,#70800,#70801,#70802,
#70803,#70804,#70805,#70806,#70807,#70808,#70809,#70810,#70811,#70812,#70813,
#70814,#70815,#70816,#70817,#70818,#70819,#70820,#70821,#70822,#70823,#70824,
#70825,#70826,#70827,#70828,#70829,#70830,#70831,#70832,#70833,#70834,#70835,
#70836,#70837,#70838,#70839,#70840,#70841,#70842,#70843,#70844,#70845,#70846,
#70847,#70848,#70849,#70850,#70851,#70852,#70853,#70854,#70855,#70856,#70857,
#70858,#70859,#70860,#70861,#70862,#70863,#70864,#70865,#70866,#70867,#70868,
#70869,#70870,#70871,#70872,#70873,#70874,#70875,#70876,#70877,#70878,#70879,
#70880,#70881,#70882,#70883,#70884,#70885,#70886,#70887,#70888,#70889,#70890,
#70891,#70892,#70893,#70894,#70895,#70896,#70897,#70898,#70899,#70900,#70901,
#70902,#70903,#70904,#70905,#70906,#70907,#70908,#70909,#70910,#70911,#70912,
#70913,#70914,#70915,#70916,#70917,#70918,#70919,#70920,#70921,#70922,#70923,
#70924,#70925,#70926,#70927,#70928,#70929,#70930,#70931,#70932,#70933,#70934,
#70935,#70936,#70937,#70938,#70939,#70940,#70941,#70942,#70943,#70944,#70945,
#70946,#70947,#70948,#70949,#70950,#70951,#70952,#70953,#70954,#70955,#70956,
#70957,#70958,#70959,#70960,#70961,#70962,#70963,#70964,#70965,#70966,#70967,
#70968,#70969,#70970,#70971,#70972,#70973,#70974,#70975,#70976,#70977,#70978,
#70979,#70980,#70981,#70982,#70983,#70984,#70985,#70986,#70987,#70988,#70989,
#70990,#70991,#70992,#70993,#70994,#70995,#70996,#70997,#70998,#70999,#71000,
#71001,#71002,#71003,#71004,#71005,#71006,#71007,#71008,#71009,#71010,#71011,
#71012,#71013,#71014,#71015,#71016,#71017,#71018,#71019,#71020,#71021,#71022,
#71023,#71024,#71025,#71026,#71027,#71028,#71029,#71030,#71031,#71032,#71033,
#71034,#71035,#71036,#71037,#71038,#71039,#71040,#71041,#71042,#71043,#71044,
#71045,#71046,#71047,#71048,#71049,#71050,#71051,#71052,#71053,#71054,#71055,
#71056,#71057,#71058,#71059,#71060,#71061,#71062,#71063,#71064,#71065,#71066,
#71067,#71068,#71069,#71070,#71071,#71072,#71073,#71074,#71075,#71076,#71077,
#71078,#71079,#71080,#71081,#71082,#71083,#71084,#71085,#71086,#71087,#71088,
#71089,#71090,#71091,#71092,#71093,#71094,#71095,#71096,#71097,#71098,#71099,
#71100,#71101,#71102,#71103,#71104,#71105,#71106,#71107,#71108,#71109,#71110,
#71111,#71112,#71113,#71114,#71115,#71116,#71117,#71118,#71119,#71120,#71121,
#71122,#71123,#71124,#71125,#71126,#71127,#71128,#71129,#71130,#71131,#71132,
#71133,#71134,#71135,#71136,#71137,#71138,#71139,#71140,#71141,#71142,#71143,
#71144,#71145,#71146,#71147,#71148,#71149,#71150,#71151,#71152,#71153,#71154,
#71155,#71156),(#71157,#71158,#71159,#71160,#71161,#71162,#71163,#71164,
#71165,#71166,#71167,#71168,#71169,#71170,#71171,#71172,#71173,#71174,#71175,
#71176,#71177,#71178,#71179,#71180,#71181,#71182,#71183,#71184,#71185,#71186,
#71187,#71188,#71189,#71190,#71191,#71192,#71193,#71194,#71195,#71196,#71197,
#71198,#71199,#71200,#71201,#71202,#71203,#71204,#71205,#71206,#71207,#71208,
#71209,#71210,#71211,#71212,#71213,#71214,#71215,#71216,#71217,#71218,#71219,
#71220,#71221,#71222,#71223,#71224,#71225,#71226,#71227,#71228,#71229,#71230,
#71231,#71232,#71233,#71234,#71235,#71236,#71237,#71238,#71239,#71240,#71241,
#71242,#71243,#71244,#71245,#71246,#71247,#71248,#71249,#71250,#71251,#71252,
#71253,#71254,#71255,#71256,#71257,#71258,#71259,#71260,#71261,#71262,#71263,
#71264,#71265,#71266,#71267,#71268,#71269,#71270,#71271,#71272,#71273,#71274,
#71275,#71276,#71277,#71278,#71279,#71280,#71281,#71282,#71283,#71284,#71285,
#71286,#71287,#71288,#71289,#71290,#71291,#71292,#71293,#71294,#71295,#71296,
#71297,#71298,#71299,#71300,#71301,#71302,#71303,#71304,#71305,#71306,#71307,
#71308,#71309,#71310,#71311,#71312,#71313,#71314,#71315,#71316,#71317,#71318,
#71319,#71320,#71321,#71322,#71323,#71324,#71325,#71326,#71327,#71328,#71329,
#71330,#71331,#71332,#71333,#71334,#71335,#71336,#71337,#71338,#71339,#71340,
#71341,#71342,#71343,#71344,#71345,#71346,#71347,#71348,#71349,#71350,#71351,
#71352,#71353,#71354,#71355,#71356,#71357,#71358,#71359,#71360,#71361,#71362,
#71363,#71364,#71365,#71366,#71367,#71368,#71369,#71370,#71371,#71372,#71373,
#71374,#71375,#71376,#71377,#71378,#71379,#71380,#71381,#71382,#71383,#71384,
#71385,#71386,#71387,#71388,#71389,#71390,#71391,#71392,#71393,#71394,#71395,
#71396,#71397,#71398,#71399,#71400,#71401,#71402,#71403,#71404,#71405,#71406,
#71407,#71408,#71409,#71410,#71411,#71412,#71413,#71414,#71415,#71416,#71417,
#71418,#71419,#71420,#71421,#71422,#71423,#71424,#71425,#71426,#71427,#71428,
#71429,#71430,#71431,#71432,#71433,#71434,#71435,#71436,#71437,#71438,#71439,
#71440,#71441,#71442,#71443,#71444,#71445,#71446,#71447,#71448,#71449,#71450,
#71451,#71452,#71453,#71454,#71455,#71456,#71457,#71458,#71459,#71460,#71461,
#71462,#71463,#71464,#71465,#71466,#71467,#71468,#71469,#71470,#71471,#71472,
#71473,#71474,#71475,#71476,#71477,#71478,#71479,#71480,#71481,#71482,#71483,
#71484,#71485,#71486,#71487,#71488,#71489,#71490,#71491,#71492,#71493,#71494,
#71495,#71496,#71497,#71498,#71499,#71500,#71501,#71502,#71503,#71504,#71505,
#71506,#71507,#71508,#71509,#71510,#71511,#71512,#71513,#71514,#71515,#71516,
#71517,#71518,#71519,#71520,#71521,#71522,#71523,#71524,#71525,#71526,#71527,
#71528,#71529,#71530,#71531,#71532,#71533,#71534,#71535,#71536,#71537,#71538,
#71539,#71540,#71541,#71542,#71543,#71544,#71545,#71546,#71547,#71548,#71549,
#71550,#71551,#71552,#71553,#71554,#71555,#71556,#71557,#71558,#71559,#71560,
#71561,#71562,#71563,#71564,#71565,#71566,#71567,#71568,#71569,#71570,#71571,
#71572,#71573,#71574,#71575,#71576,#71577,#71578,#71579,#71580,#71581,#71582,
#71583,#71584,#71585,#71586,#71587,#71588,#71589,#71590,#71591,#71592,#71593,
#71594,#71595,#71596,#71597,#71598,#71599,#71600,#71601,#71602,#71603,#71604,
#71605,#71606,#71607,#71608,#71609,#71610,#71611,#71612,#71613,#71614,#71615,
#71616,#71617,#71618,#71619,#71620,#71621,#71622,#71623,#71624,#71625,#71626,
#71627,#71628,#71629,#71630,#71631,#71632,#71633,#71634,#71635,#71636,#71637,
#71638,#71639,#71640,#71641,#71642,#71643,#71644,#71645,#71646,#71647,#71648,
#71649,#71650,#71651,#71652,#71653,#71654,#71655,#71656,#71657,#71658,#71659,
#71660,#71661,#71662,#71663,#71664,#71665,#71666,#71667,#71668,#71669,#71670,
#71671,#71672,#71673,#71674,#71675,#71676,#71677,#71678,#71679,#71680,#71681,
#71682,#71683,#71684,#71685,#71686,#71687,#71688,#71689,#71690,#71691,#71692,
#71693,#71694,#71695,#71696,#71697,#71698,#71699,#71700,#71701,#71702,#71703,
#71704,#71705,#71706,#71707,#71708,#71709,#71710,#71711,#71712,#71713,#71714,
#71715)),.UNSPECIFIED.,.F.,.F.,.F.,(4,4),(4,1,1,1,1,1,1,1,1,1,1,1,1,1,1,
1,1,1,1,1,1,1,1,1,1,1,1,1,1,1,1,1,1,1,1,1,1,1,1,1,1,1,1,1,1,1,1,1,1,1,1,
1,1,1,1,1,1,1,1,1,1,1,1,1,1,1,1,1,1,1,1,1,1,1,1,1,1,1,1,1,1,1,1,1,1,1,1,
1,1,1,1,1,1,1,1,1,1,1,1,1,1,1,1,1,1,1,1,1,1,1,1,1,1,1,1,1,1,1,1,1,1,1,1,
1,1,1,1,1,1,1,1,1,1,1,1,1,1,1,1,1,1,1,1,1,1,1,1,1,1,1,1,1,1,1,1,1,1,1,1,
1,1,1,1,1,1,1,1,1,1,1,1,1,1,1,1,1,1,1,1,1,1,1,1,1,1,1,1,1,1,1,1,1,1,1,1,
1,1,1,1,1,1,1,1,1,1,1,1,1,1,1,1,1,1,1,1,1,1,1,1,1,1,1,1,1,1,1,1,1,1,1,1,
1,1,1,1,1,1,1,1,1,1,1,1,1,1,1,1,1,1,1,1,1,1,1,1,1,1,1,1,1,1,1,1,1,1,1,1,
1,1,1,1,1,1,1,1,1,1,1,1,1,1,1,1,1,1,1,1,1,1,1,1,1,1,1,1,1,1,1,1,1,1,1,1,
1,1,1,1,1,1,1,1,1,1,1,1,1,1,1,1,1,1,1,1,1,1,1,1,1,1,1,1,1,1,1,1,1,1,1,1,
1,1,1,1,1,1,1,1,1,1,1,1,1,1,1,1,1,1,1,1,1,1,1,1,1,1,1,1,1,1,1,1,1,1,1,1,
1,1,1,1,1,1,1,1,1,1,1,1,1,1,1,1,1,1,1,1,1,1,1,1,1,1,1,1,1,1,1,1,1,1,1,1,
1,1,1,1,1,1,1,1,1,1,1,1,1,1,1,1,1,1,1,1,1,1,1,1,1,1,1,1,1,1,1,1,1,1,1,1,
1,1,1,1,1,1,1,1,1,1,1,1,1,1,1,1,1,1,1,1,1,1,1,1,1,1,1,1,1,1,1,1,1,1,1,1,
1,1,1,1,1,1,1,1,1,1,1,1,1,1,1,1,1,1,1,1,1,1,1,1,1,1,1,1,1,1,1,1,1,1,1,1,
1,1,1,1,1,1,1,1,1,1,1,1,1,1,1,1,1,1,1,1,1,1,1,1,1,1,1,1,1,1,1,1,1,1,1,1,
1,4),(-0.00081013426626431,0.132758442671244),(8.30110427451238,8.80100606031193,
9.30088286599662,10.300636477366,11.3003900887353,12.3001437001047,13.2998973114741,
14.2996509228435,14.7995277285281,15.2994045342128,16.2991581455822,17.2989117569516,
18.2986653683209,19.2984189796903,20.2981725910597,21.297926202429,21.7978030081137,
22.2976798137984,23.2974334251678,24.2971870365371,25.2969406479065,26.2966942592759,
27.2964478706452,28.2962014820146,28.7960782876993,29.295955093384,30.2957087047533,
31.2954623161227,32.2952159274921,33.2949695388614,34.2947231502308,35.2944767616002,
35.7943535672848,36.2942303729695,37.2939839843389,38.2937375957083,39.2934912070776,
40.293244818447,41.2929984298164,42.2927520411857,42.7926288468704,43.2925056525551,
44.2922592639245,45.2920128752938,46.2917664866632,47.2915200980326,48.2912737094019,
49.2910273207713,49.790904126456,50.2907809321407,51.29053454351,52.2902881548794,
53.2900417662488,54.2897953776181,55.2895489889875,56.2893026003569,56.7891794060416,
57.2890562117262,58.2888098230956,59.288563434465,60.2883170458343,61.2880706572037,
62.2878242685731,63.2875778799424,63.7874546856271,64.2873314913118,65.2870851026812,
66.2868387140505,67.2865923254199,68.2863459367893,69.2860995481586,70.285853159528,
70.7857299652127,71.2856067708974,72.2853603822667,73.2851139936361,74.2848676050055,
75.2846212163748,76.2843748277442,77.2841284391136,77.7840052447983,78.2838820504829,
79.2836356618523,80.2833892732217,81.283142884591,82.2828964959604,83.2826501073298,
84.2824037186991,84.7822805243838,85.2821573300685,86.2819109414379,87.2816645528073,
88.2814181641766,89.281171775546,90.2809253869154,91.2806789982847,91.7805558039694,
92.2804326096541,93.2801862210235,94.2799398323928,95.2796934437622,96.2794470551316,
97.2792006665009,98.2789542778703,98.778831083555,99.2787078892397,100.278461500609,
101.278215111978,102.277968723348,103.277722334717,104.277475946086,105.277229557456,
105.777106363141,106.276983168825,107.276736780195,108.276490391564,109.276244002933,
110.275997614303,111.275751225672,112.275504837041,112.775381642726,113.275258448411,
114.27501205978,115.27476567115,116.274519282519,117.274272893888,118.274026505258,
119.273780116627,119.773656922312,120.273533727996,121.273287339366,122.273040950735,
123.272794562104,124.272548173474,125.272301784843,126.272055396213,126.771932201897,
127.271809007582,128.271562618951,129.271316230321,130.27106984169,131.270823453059,
132.270577064429,133.270330675798,133.770207481483,134.270084287167,135.269837898537,
136.269591509906,137.269345121276,138.269098732645,139.268852344014,140.268605955384,
140.768482761068,141.268359566753,142.268113178122,143.267866789492,144.267620400861,
145.267374012231,146.2671276236,147.266881234969,147.766758040654,148.266634846339,
149.266388457708,150.266142069077,151.265895680447,152.265649291816,153.265402903185,
154.265156514555,154.76503332024,155.264910125924,156.264663737294,157.264417348663,
158.264170960032,159.263924571402,160.263678182771,161.26343179414,161.763308599825,
162.26318540551,163.262939016879,164.262692628249,165.262446239618,166.262199850987,
167.261953462357,168.261707073726,168.761583879411,169.261460685095,170.261214296465,
171.260967907834,172.260721519203,173.260475130573,174.260228741942,175.259982353312,
175.759859158996,176.259735964681,177.25948957605,178.25924318742,179.258996798789,
180.258750410158,181.258504021528,182.258257632897,182.758134438582,183.258011244266,
184.257764855636,185.257518467005,186.257272078375,187.257025689744,188.256779301113,
189.256532912483,189.756409718167,190.256286523852,191.256040135221,192.255793746591,
193.25554735796,194.25530096933,195.255054580699,196.254808192068,196.754684997753,
197.254561803438,198.254315414807,199.254069026176,200.253822637546,201.253576248915,
202.253329860284,203.253083471654,203.752960277339,204.252837083023,205.252590694393,
206.252344305762,207.252097917131,208.251851528501,209.25160513987,210.251358751239,
210.751235556924,211.251112362609,212.250865973978,213.250619585347,214.250373196717,
215.250126808086,216.249880419456,217.249634030825,217.74951083651,218.249387642194,
219.249141253564,220.248894864933,221.248648476302,222.248402087672,223.248155699041,
224.247909310411,224.747786116095,225.24766292178,226.247416533149,227.247170144519,
228.246923755888,229.246677367257,230.246430978627,231.246184589996,231.746061395681,
232.245938201365,233.245691812735,234.245445424104,235.245199035474,236.244952646843,
237.244706258212,238.244459869582,238.744336675266,239.244213480951,240.24396709232,
241.24372070369,242.243474315059,243.243227926429,244.242981537798,245.242735149167,
245.742611954852,246.242488760537,247.242242371906,248.241995983275,249.241749594645,
250.241503206014,251.241256817383,252.241010428753,253.240764040122,254.240517651492,
255.240271262861,256.24002487423,256.739901679915,257.2397784856,258.239532096969,
259.239285708338,260.239039319708,261.238792931077,262.238546542446,263.238300153816,
263.7381769595,264.238053765185,265.237807376555,266.237560987924,267.237314599293,
268.237068210663,269.236821822032,270.236575433401,270.736452239086,271.236329044771,
272.23608265614,273.23583626751,274.235589878879,275.235343490248,276.235097101618,
277.234850712987,277.734727518672,278.234604324356,279.234357935726,280.234111547095,
281.233865158464,282.233618769834,283.233372381203,284.233125992573,284.733002798257,
285.232879603942,286.232633215311,287.232386826681,288.23214043805,289.231894049419,
290.231647660789,291.231401272158,291.731278077843,292.231154883527,293.230908494897,
294.230662106266,295.230415717636,296.230169329005,297.229922940374,298.229676551744,
298.729553357428,299.229430163113,300.229183774482,301.228937385852,302.228690997221,
303.228444608591,304.22819821996,305.227951831329,305.727828637014,306.227705442699,
307.227459054068,308.227212665437,309.226966276807,310.226719888176,311.226473499545,
312.226227110915,312.7261039166,313.225980722284,314.225734333654,315.225487945023,
316.225241556392,317.224995167762,318.224748779131,319.2245023905,319.724379196185,
320.22425600187,321.224009613239,322.223763224608,323.223516835978,324.223270447347,
325.223024058717,326.222777670086,326.722654475771,327.222531281455,328.222284892825,
329.222038504194,330.221792115563,331.221545726933,332.221299338302,333.221052949672,
333.720929755356,334.220806561041,335.22056017241,336.22031378378,337.220067395149,
338.219821006518,339.219574617888,340.219328229257,340.719205034942,341.219081840626,
342.218835451996,343.218589063365,344.218342674735,345.218096286104,346.217849897473,
347.217603508843,347.717480314527,348.217357120212,349.217110731581,350.216864342951,
351.21661795432,352.216371565689,353.216125177059,354.215878788428,354.715755594113,
355.215632399798,356.215386011167,357.215139622536,358.214893233906,359.214646845275,
360.214400456644,361.214154068014,361.714030873699,362.213907679383,363.213661290753,
364.213414902122,365.213168513491,366.212922124861,367.21267573623,368.212429347599,
368.712306153284,369.212182958969,370.211936570338,371.211690181707,372.211443793077,
373.211197404446,374.210951015816,375.210704627185,375.71058143287,376.210458238554,
377.210211849924,378.209965461293,379.209719072662,380.209472684032,381.209226295401,
382.208979906771,382.708856712455,383.20873351814,384.208487129509,385.208240740879,
386.207994352248,387.207747963617,388.207501574987,389.207255186356,389.707131992041,
390.207008797725,391.206762409095,392.206516020464,393.206269631834,394.206023243203,
395.205776854572,396.205530465942,396.705407271626,397.205284077311,398.20503768868,
399.20479130005,400.204544911419,401.204298522789,402.204052134158,403.203805745527,
403.703682551212,404.203559356897,405.203312968266,406.203066579635,407.202820191005,
408.202573802374,409.202327413743,410.202081025113,410.701957830797,411.201834636482,
412.201588247852,413.201341859221,414.20109547059,415.20084908196,416.200602693329,
417.200356304698,417.700233110383,418.200109916068,419.199863527437,420.199617138806,
421.199370750176,422.199124361545,423.198877972915,424.198631584284,424.698508389969,
425.198385195653,426.198138807023,427.197892418392,428.197646029761,429.197399641131,
430.1971532525,431.19690686387,431.696783669554,432.196660475239,433.196414086608,
434.196167697978,435.195921309347,436.195674920716,437.195428532086,438.195182143455,
438.69505894914,439.194935754824,440.194689366194,441.194442977563,442.194196588933,
443.193950200302,444.193703811671,445.193457423041,445.693334228725,446.19321103441,
447.192964645779,448.192718257149,449.192471868518,450.192225479887,451.191979091257,
452.191732702626,452.691609508311,453.191486313996,454.191239925365,455.190993536734,
456.190747148104,457.190500759473,458.190254370842,459.190007982212,459.689884787896,
460.189761593581,461.189515204951,462.18926881632,463.189022427689,464.188776039059,
465.188529650428,466.188283261797,466.688160067482,467.188036873167,468.187790484536,
469.187544095905,470.187297707275,471.187051318644,472.186804930014,473.186558541383,
473.686435347068,474.186312152752,475.186065764122,476.185819375491,477.18557298686,
478.18532659823,479.185080209599,480.184833820968,480.684710626653,481.184587432338,
482.184341043707,483.184094655077,484.183848266446,485.183601877815,486.183355489185,
487.183109100554,487.682985906239,488.182862711923,489.182616323293,490.182369934662,
491.182123546032,492.181877157401,493.18163076877,493.681507574455,494.18151432674),
 .UNSPECIFIED.);
#105=CONICAL_SURFACE('',#7514,7.5,0.785398163397451);
#107=ELLIPSE('',#7497,6.37218304159764,5.71843041940893);
#108=ELLIPSE('',#7498,6.23535398393752,5.62417080294212);
#109=B_SPLINE_CURVE_WITH_KNOTS('',3,(#8945,#8946,#8947,#8948,#8949,#8950,
#8951,#8952,#8953,#8954,#8955,#8956,#8957,#8958,#8959,#8960,#8961,#8962,
#8963,#8964,#8965,#8966,#8967,#8968,#8969,#8970,#8971,#8972,#8973,#8974,
#8975,#8976,#8977,#8978,#8979,#8980,#8981,#8982,#8983,#8984,#8985,#8986,
#8987,#8988,#8989,#8990,#8991,#8992,#8993,#8994,#8995,#8996,#8997,#8998,
#8999,#9000,#9001,#9002,#9003,#9004,#9005,#9006,#9007,#9008,#9009,#9010,
#9011,#9012,#9013,#9014,#9015,#9016,#9017,#9018,#9019,#9020,#9021,#9022,
#9023,#9024,#9025,#9026,#9027,#9028,#9029,#9030,#9031,#9032,#9033,#9034,
#9035,#9036,#9037,#9038,#9039,#9040,#9041,#9042,#9043,#9044,#9045,#9046,
#9047,#9048,#9049,#9050,#9051,#9052,#9053,#9054,#9055,#9056,#9057,#9058,
#9059,#9060,#9061,#9062,#9063,#9064,#9065,#9066,#9067,#9068,#9069,#9070,
#9071,#9072,#9073,#9074,#9075,#9076,#9077),.UNSPECIFIED.,.F.,.F.,(4,3,3,
3,3,3,3,3,3,3,3,3,3,3,3,3,3,3,3,3,3,3,3,3,3,3,3,3,3,3,3,3,3,3,3,3,3,3,3,
3,3,3,3,3,4),(10.3769047257236,10.4527816077004,10.5285705693428,10.6042884681534,
10.6799520845211,10.7575068350479,10.8331228590851,10.9087383619952,10.9843684364558,
11.0633738495257,11.1391179258011,11.2149124638109,11.2908054681926,11.3003900887353,
11.3780272612758,11.4555770973186,11.5330551296334,11.610476839924,11.6878576694966,
11.7652227836524,11.8425815660687,11.9199479598844,11.9973359098454,12.0748026220138,
12.152309867659,12.2299284461808,12.3001437001047,12.3771329899878,12.4540352583854,
12.5308666134793,12.6076431087672,12.6843807554362,12.761320324941,12.8380442272445,
12.9147794477103,12.9915404486635,13.0686296643661,13.1455244992986,13.2227109053863,
13.2998973114741,13.3773518589841,13.4546868229213,13.531953152234,13.6091519910909,
13.661913603788),.UNSPECIFIED.);
#110=B_SPLINE_CURVE_WITH_KNOTS('',3,(#9080,#9081,#9082,#9083,#9084,#9085,
#9086,#9087,#9088,#9089,#9090,#9091,#9092,#9093,#9094,#9095,#9096,#9097,
#9098,#9099,#9100,#9101,#9102,#9103,#9104,#9105,#9106,#9107,#9108,#9109,
#9110,#9111,#9112,#9113,#9114,#9115,#9116,#9117,#9118,#9119,#9120,#9121,
#9122,#9123,#9124,#9125,#9126,#9127,#9128,#9129,#9130,#9131,#9132,#9133,
#9134,#9135,#9136,#9137,#9138,#9139,#9140,#9141,#9142,#9143,#9144,#9145,
#9146,#9147,#9148,#9149,#9150,#9151,#9152,#9153,#9154,#9155),
 .UNSPECIFIED.,.F.,.F.,(4,3,3,3,3,3,3,3,3,3,3,3,3,3,3,3,3,3,3,3,3,3,3,3,
3,4),(11.6150328478195,11.6974944507364,11.7799553878079,11.8624156864323,
11.9448753740057,12.0273344779219,12.1097930255731,12.1922510443491,12.2747085616382,
12.3613793526067,12.4438461362102,12.5263112474637,12.6087747960201,12.6912368915109,
12.7736976435469,12.8561571617202,12.9386155556056,13.0210729347622,13.1035393166313,
13.1860025148144,13.2684629678307,13.3509211140436,13.4333867103942,13.515846583346,
13.598310680714,13.661441217134),.UNSPECIFIED.);
#111=B_SPLINE_CURVE_WITH_KNOTS('',3,(#9161,#9162,#9163,#9164,#9165,#9166,
#9167,#9168,#9169,#9170,#9171,#9172,#9173,#9174,#9175,#9176,#9177,#9178,
#9179,#9180,#9181,#9182,#9183,#9184,#9185,#9186,#9187,#9188,#9189,#9190,
#9191,#9192,#9193,#9194,#9195,#9196,#9197,#9198,#9199,#9200,#9201,#9202,
#9203,#9204,#9205,#9206,#9207,#9208,#9209,#9210,#9211,#9212,#9213,#9214,
#9215,#9216,#9217,#9218,#9219,#9220,#9221,#9222,#9223,#9224,#9225,#9226,
#9227,#9228,#9229,#9230,#9231,#9232,#9233,#9234,#9235,#9236,#9237,#9238,
#9239,#9240,#9241,#9242,#9243,#9244,#9245,#9246,#9247,#9248,#9249,#9250,
#9251,#9252,#9253,#9254,#9255,#9256,#9257,#9258,#9259,#9260,#9261,#9262,
#9263,#9264,#9265,#9266,#9267,#9268,#9269,#9270,#9271,#9272,#9273,#9274,
#9275,#9276,#9277,#9278,#9279,#9280,#9281,#9282,#9283,#9284,#9285,#9286,
#9287,#9288,#9289,#9290,#9291,#9292,#9293,#9294,#9295,#9296,#9297,#9298,
#9299,#9300,#9301,#9302,#9303,#9304,#9305,#9306,#9307,#9308,#9309,#9310,
#9311,#9312,#9313,#9314,#9315,#9316,#9317),.UNSPECIFIED.,.F.,.F.,(4,3,3,
3,3,3,3,3,3,3,3,3,3,3,3,3,3,3,3,3,3,3,3,3,3,3,3,3,3,3,3,3,3,3,3,3,3,3,3,
3,3,3,3,3,3,3,3,3,3,3,3,3,4),(15.7079632679501,15.7904254739863,15.8728873317261,
15.9553488480197,16.0378100297171,16.1202708836684,16.2027314167227,16.2851916357294,
16.3676515475373,16.450111158995,16.5325704769509,16.6150295082534,16.69748825975,
16.7799467382885,16.8624049507163,16.9448629038807,17.0273206046285,17.1097780598065,
17.1922352762608,17.2782475027625,17.361571847186,17.4440384526314,17.5265042138728,
17.6089691583254,17.6914333134013,17.7738967065101,17.8563593650587,17.9388213164515,
18.0212825880902,18.1037432073744,18.1862032017012,18.2686625984657,18.3511214250608,
18.4335797088775,18.516037477305,18.5984947577303,18.6826279931418,18.7650939912334,
18.8475583675889,18.9300212318511,19.0124826936418,19.0949428625629,19.1774018481984,
19.2598597601156,19.3454556056404,19.4279203422406,19.5103821142425,19.5928413600846,
19.6752985180616,19.7577610363429,19.8402187071978,19.9226774971486,19.9446265243138),
 .UNSPECIFIED.);
#112=B_SPLINE_CURVE_WITH_KNOTS('',3,(#9318,#9319,#9320,#9321,#9322,#9323,
#9324,#9325,#9326,#9327,#9328,#9329,#9330,#9331,#9332,#9333,#9334,#9335,
#9336,#9337,#9338,#9339,#9340,#9341,#9342,#9343,#9344,#9345,#9346,#9347,
#9348,#9349,#9350,#9351,#9352,#9353,#9354,#9355,#9356,#9357,#9358,#9359,
#9360,#9361,#9362,#9363,#9364,#9365,#9366,#9367,#9368,#9369,#9370,#9371,
#9372,#9373,#9374,#9375,#9376,#9377,#9378,#9379,#9380,#9381,#9382,#9383,
#9384,#9385,#9386,#9387,#9388,#9389,#9390,#9391,#9392,#9393,#9394,#9395,
#9396,#9397,#9398,#9399,#9400,#9401,#9402),.UNSPECIFIED.,.F.,.F.,(4,3,3,
3,3,3,3,3,3,3,3,3,3,3,3,3,3,3,3,3,3,3,3,3,3,3,3,3,4),(13.661913603788,13.74163076867,
13.8187547130951,13.8958776827639,13.9730138226308,14.0501772823724,14.1274181186823,
14.2047051682193,14.2820865197271,14.2996509228435,14.3812500628693,14.4627432830108,
14.5469393943902,14.6282018702999,14.7093852717979,14.79047384344,14.7995277285281,
14.8805147931035,14.9615778600741,15.0460345286088,15.1273201750453,15.2086838620509,
15.2901690288209,15.2994045342128,15.3835468826529,15.4674320024452,15.5511589990445,
15.634627823912,15.7079632679501),.UNSPECIFIED.);
#113=B_SPLINE_CURVE_WITH_KNOTS('',3,(#9404,#9405,#9406,#9407,#9408,#9409,
#9410,#9411,#9412,#9413,#9414,#9415,#9416,#9417,#9418,#9419,#9420,#9421,
#9422,#9423,#9424,#9425,#9426,#9427,#9428,#9429,#9430,#9431,#9432,#9433,
#9434,#9435,#9436,#9437,#9438,#9439,#9440,#9441,#9442,#9443,#9444,#9445,
#9446,#9447,#9448,#9449,#9450,#9451,#9452,#9453,#9454,#9455,#9456,#9457,
#9458,#9459,#9460,#9461,#9462,#9463,#9464,#9465,#9466,#9467,#9468,#9469,
#9470,#9471,#9472,#9473,#9474,#9475,#9476,#9477,#9478,#9479),
 .UNSPECIFIED.,.F.,.F.,(4,3,3,3,3,3,3,3,3,3,3,3,3,3,3,3,3,3,3,3,3,3,3,3,
3,4),(13.661441217134,13.7439028162622,13.8263637496976,13.9088240448388,
13.9912837290816,14.0737428298202,14.1562013744464,14.2386593903501,14.3211169049196,
14.4077589589255,14.4902257335027,14.5726908363028,14.6551543769792,14.7376164651628,
14.8200772104646,14.9025367224764,14.9849951107731,15.0674524849134,15.1499188490036,
15.2323820317,15.314842471521,15.3973006068293,15.4797661687128,15.5622260163633,
15.6446900491511,15.7073897690138),.UNSPECIFIED.);
#114=B_SPLINE_CURVE_WITH_KNOTS('',3,(#9480,#9481,#9482,#9483,#9484,#9485,
#9486,#9487,#9488,#9489,#9490,#9491,#9492,#9493,#9494,#9495,#9496,#9497,
#9498,#9499,#9500,#9501,#9502,#9503,#9504,#9505,#9506,#9507,#9508,#9509,
#9510,#9511,#9512,#9513,#9514,#9515,#9516,#9517,#9518,#9519,#9520,#9521,
#9522,#9523,#9524,#9525,#9526,#9527,#9528,#9529,#9530,#9531,#9532,#9533,
#9534,#9535,#9536,#9537,#9538,#9539,#9540,#9541,#9542,#9543,#9544,#9545,
#9546,#9547,#9548,#9549,#9550,#9551,#9552,#9553,#9554,#9555,#9556,#9557,
#9558,#9559,#9560,#9561,#9562,#9563,#9564,#9565,#9566,#9567,#9568,#9569,
#9570,#9571,#9572,#9573,#9574,#9575,#9576,#9577,#9578,#9579,#9580,#9581,
#9582,#9583,#9584,#9585,#9586,#9587,#9588,#9589,#9590,#9591,#9592,#9593,
#9594,#9595,#9596,#9597,#9598,#9599,#9600,#9601,#9602,#9603,#9604,#9605,
#9606,#9607,#9608,#9609,#9610,#9611,#9612,#9613,#9614,#9615,#9616,#9617,
#9618,#9619,#9620,#9621,#9622,#9623,#9624,#9625,#9626,#9627,#9628,#9629,
#9630,#9631,#9632,#9633,#9634,#9635,#9636,#9637,#9638,#9639,#9640,#9641,
#9642,#9643,#9644,#9645,#9646,#9647,#9648,#9649,#9650,#9651),
 .UNSPECIFIED.,.F.,.F.,(4,3,3,3,3,3,3,3,3,3,3,3,3,3,3,3,3,3,3,3,3,3,3,3,
3,3,3,3,3,3,3,3,3,3,3,3,3,3,3,3,3,3,3,3,3,3,3,3,3,3,3,3,3,3,3,3,3,4),(15.7079632952952,
15.7840025321932,15.8599648001924,15.9358667980574,16.011725164846,16.0875668207261,
16.1634020177953,16.2392457593701,16.3151130540793,16.3910644371312,16.4670598741112,
16.5431728456518,16.6070728880741,16.6845222139964,16.7618780204501,16.8391560772364,
16.9163720976792,16.9935417500323,17.0706879712162,17.1478232165181,17.2249616213568,
17.3021173203171,17.3793459856373,17.4566118378682,17.5339848547524,17.605480896125,
17.6870848273324,17.7685832167635,17.8526086376102,17.9338773603292,18.0192811302398,
18.1003738605163,18.1046849001504,18.1856750726475,18.2667409241249,18.3510279191377,
18.432315204022,18.5136802303654,18.5951660787181,18.6038889041759,18.6814065367343,
18.7588426168442,18.8362127393099,18.9135324517233,18.9908172650905,19.0680957040123,
19.1453735563204,19.2226648395218,19.2999835760365,19.3773904489576,19.4548430590586,
19.5324155966512,19.6022969122268,19.6791914072041,19.7559671805278,19.8326746431303,
19.9093157129169,19.9452932995404),.UNSPECIFIED.);
#115=B_SPLINE_CURVE_WITH_KNOTS('',3,(#9657,#9658,#9659,#9660,#9661,#9662,
#9663,#9664,#9665,#9666,#9667,#9668,#9669,#9670,#9671,#9672,#9673,#9674,
#9675,#9676,#9677,#9678,#9679,#9680,#9681,#9682,#9683,#9684,#9685,#9686,
#9687,#9688,#9689,#9690,#9691,#9692,#9693,#9694,#9695,#9696,#9697,#9698,
#9699,#9700,#9701,#9702,#9703,#9704,#9705,#9706,#9707,#9708,#9709,#9710,
#9711,#9712,#9713,#9714,#9715,#9716,#9717,#9718,#9719,#9720,#9721,#9722,
#9723,#9724,#9725,#9726,#9727,#9728,#9729,#9730,#9731,#9732,#9733,#9734,
#9735,#9736,#9737,#9738,#9739,#9740,#9741,#9742,#9743,#9744,#9745,#9746,
#9747,#9748,#9749,#9750,#9751,#9752,#9753,#9754,#9755,#9756,#9757,#9758,
#9759,#9760,#9761,#9762,#9763,#9764,#9765,#9766,#9767,#9768,#9769,#9770,
#9771,#9772,#9773,#9774,#9775,#9776,#9777,#9778,#9779,#9780,#9781,#9782,
#9783,#9784,#9785,#9786,#9787,#9788,#9789,#9790,#9791,#9792,#9793,#9794,
#9795,#9796,#9797,#9798,#9799,#9800,#9801,#9802,#9803,#9804,#9805,#9806,
#9807,#9808,#9809,#9810,#9811,#9812,#9813,#9814,#9815,#9816,#9817,#9818,
#9819,#9820,#9821,#9822),.UNSPECIFIED.,.F.,.F.,(4,3,3,3,3,3,3,3,3,3,3,3,
3,3,3,3,3,3,3,3,3,3,3,3,3,3,3,3,3,3,3,3,3,3,3,3,3,3,3,3,3,3,3,3,3,3,3,3,
3,3,3,3,3,3,3,4),(21.9911485751297,22.0810996357526,22.1714401170014,22.262210689136,
22.2976798137984,22.3751954065669,22.4526295180584,22.5299977443591,22.6073156343901,
22.6845987005346,22.7618755834062,22.8391519603175,22.9164418501864,22.9937592768941,
23.0711652742691,23.1486170734114,23.2261896715283,23.2974334251678,23.374282115361,
23.4510370293504,23.5277144368787,23.6043305452548,23.6809015129049,23.7579372033589,
23.8344796918291,23.9110280983708,23.9875969999661,24.0649945091089,24.1416856601052,
24.2194363483211,24.2971870365371,24.3747045940136,24.4521348195148,24.5294933687083,
24.6067958458031,24.6840578144639,24.7613050472459,24.838546565628,24.9157964232056,
24.9930686756278,25.0704216413305,25.1478160415037,25.2253243771904,25.2969406479065,
25.374461596459,25.4518944782164,25.5292549516708,25.6065586232433,25.6841896108983,
25.7614330861104,25.8386698613634,25.9159139891612,25.9938371229918,26.0711686401118,
26.1493875822976,26.2276065244835),.UNSPECIFIED.);
#116=B_SPLINE_CURVE_WITH_KNOTS('',3,(#9823,#9824,#9825,#9826,#9827,#9828,
#9829,#9830,#9831,#9832,#9833,#9834,#9835,#9836,#9837,#9838,#9839,#9840,
#9841,#9842,#9843,#9844,#9845,#9846,#9847,#9848,#9849,#9850,#9851,#9852,
#9853,#9854,#9855,#9856,#9857,#9858,#9859,#9860,#9861,#9862,#9863,#9864,
#9865,#9866,#9867,#9868,#9869,#9870,#9871,#9872,#9873,#9874,#9875,#9876,
#9877,#9878,#9879,#9880,#9881,#9882,#9883,#9884,#9885,#9886,#9887,#9888,
#9889,#9890,#9891,#9892,#9893,#9894,#9895,#9896,#9897,#9898),
 .UNSPECIFIED.,.F.,.F.,(4,3,3,3,3,3,3,3,3,3,3,3,3,3,3,3,3,3,3,3,3,3,3,3,
3,4),(19.9446265243138,20.0270881281676,20.1095490661382,20.1920093656239,
20.2744690540208,20.3569281587228,20.439386707122,20.5218447266083,20.6043022445699,
20.6909801402299,20.7734469260655,20.8559120394093,20.9383755899145,21.0208376872122,
21.1032984409136,21.1857579606107,21.2682163558785,21.3506737362757,21.4331401225421,
21.5156033245558,21.5980637808363,21.6805219297472,21.7629875346264,21.8454474138409,
21.9279115272047,21.9911485751297),.UNSPECIFIED.);
#117=B_SPLINE_CURVE_WITH_KNOTS('',3,(#9900,#9901,#9902,#9903,#9904,#9905,
#9906,#9907,#9908,#9909,#9910,#9911,#9912,#9913,#9914,#9915,#9916,#9917,
#9918,#9919,#9920,#9921,#9922,#9923,#9924,#9925,#9926,#9927,#9928,#9929,
#9930,#9931,#9932,#9933,#9934,#9935,#9936,#9937,#9938,#9939,#9940,#9941,
#9942,#9943,#9944,#9945,#9946,#9947,#9948,#9949,#9950,#9951,#9952,#9953,
#9954,#9955,#9956,#9957,#9958,#9959,#9960,#9961,#9962,#9963,#9964,#9965,
#9966,#9967,#9968,#9969,#9970,#9971,#9972,#9973,#9974,#9975,#9976,#9977,
#9978,#9979,#9980,#9981),.UNSPECIFIED.,.F.,.F.,(4,3,3,3,3,3,3,3,3,3,3,3,
3,3,3,3,3,3,3,3,3,3,3,3,3,3,3,4),(19.9452932995404,20.0218764286094,20.098449829705,
20.1750215389486,20.2516061131552,20.3282181146041,20.4049138676908,20.4816564455584,
20.5585073870191,20.6007049202777,20.6782317587392,20.7556714715145,20.8330397034221,
20.9103520480074,20.9876240584291,21.0648814996859,21.1421333592579,21.2193936816471,
21.2966765134702,21.3740398998633,21.4514448142151,21.5289629928235,21.5991129283287,
21.6853515317677,21.7712477478555,21.8569207098858,21.9422242479864,21.9911485750449),
 .UNSPECIFIED.);
#118=B_SPLINE_CURVE_WITH_KNOTS('',3,(#9982,#9983,#9984,#9985,#9986,#9987,
#9988,#9989,#9990,#9991,#9992,#9993,#9994,#9995,#9996,#9997,#9998,#9999,
#10000,#10001,#10002,#10003,#10004,#10005,#10006,#10007,#10008,#10009,#10010,
#10011,#10012,#10013,#10014,#10015,#10016,#10017,#10018,#10019,#10020,#10021,
#10022,#10023,#10024,#10025,#10026,#10027,#10028,#10029,#10030,#10031,#10032,
#10033,#10034,#10035,#10036,#10037,#10038,#10039,#10040,#10041,#10042,#10043,
#10044,#10045,#10046,#10047,#10048,#10049,#10050,#10051,#10052,#10053,#10054,
#10055,#10056,#10057,#10058,#10059,#10060,#10061,#10062,#10063,#10064,#10065,
#10066,#10067,#10068,#10069,#10070,#10071,#10072,#10073,#10074,#10075,#10076,
#10077,#10078,#10079,#10080,#10081,#10082,#10083,#10084,#10085,#10086,#10087,
#10088,#10089,#10090,#10091,#10092,#10093,#10094,#10095,#10096,#10097,#10098,
#10099,#10100,#10101,#10102,#10103,#10104,#10105,#10106,#10107,#10108,#10109,
#10110,#10111,#10112,#10113,#10114,#10115,#10116,#10117,#10118,#10119,#10120,
#10121,#10122,#10123,#10124,#10125,#10126,#10127,#10128,#10129,#10130,#10131,
#10132,#10133,#10134,#10135,#10136,#10137,#10138,#10139,#10140,#10141,#10142,
#10143,#10144,#10145,#10146,#10147,#10148,#10149,#10150,#10151,#10152,#10153),
 .UNSPECIFIED.,.F.,.F.,(4,3,3,3,3,3,3,3,3,3,3,3,3,3,3,3,3,3,3,3,3,3,3,3,
3,3,3,3,3,3,3,3,3,3,3,3,3,3,3,3,3,3,3,3,3,3,3,3,3,3,3,3,3,3,3,3,3,4),(21.9911485751295,
22.0695184733941,22.1479066212012,22.2263255018552,22.3047876151167,22.3833550279714,
22.46197914016,22.5407293214231,22.5975209363796,22.6743586591899,22.7511073831277,
22.8277833450473,22.90440272373,22.9809816530099,23.0578500644375,23.1344119450102,
23.2109840282971,23.2875808824072,23.364667897913,23.441396891209,23.5186629178197,
23.5959289444305,23.6735231120596,23.7510248731705,23.8284498505637,23.9058136120981,
23.98313168169,24.0604268738106,24.1377114056863,24.2149992848633,24.2923045181101,
24.3696820492007,24.4470966131919,24.5246167262537,24.5943369524814,24.6758223858517,
24.7572035843824,24.8412879274136,24.922444368254,25.0035242804619,25.0845134135558,
25.0935409565069,25.1745548343586,25.2556443278473,25.3399194860185,25.4212298041297,
25.5026175723088,25.5841255927926,25.5927449605323,25.672078121751,25.7495172508508,
25.8268944839681,25.9042238961777,25.9850204847038,26.0623029562465,26.1395795805683,
26.2168751299167,26.2274102502822),.UNSPECIFIED.);
#119=B_SPLINE_CURVE_WITH_KNOTS('',3,(#10159,#10160,#10161,#10162,#10163,
#10164,#10165,#10166,#10167,#10168,#10169,#10170,#10171,#10172,#10173,#10174,
#10175,#10176,#10177,#10178,#10179,#10180,#10181,#10182,#10183,#10184,#10185,
#10186,#10187,#10188,#10189,#10190,#10191,#10192,#10193,#10194,#10195,#10196,
#10197,#10198,#10199,#10200,#10201,#10202,#10203,#10204,#10205,#10206,#10207,
#10208,#10209,#10210,#10211,#10212,#10213,#10214,#10215,#10216,#10217,#10218,
#10219,#10220,#10221,#10222,#10223,#10224,#10225,#10226,#10227,#10228,#10229,
#10230,#10231,#10232,#10233,#10234,#10235,#10236,#10237,#10238,#10239,#10240,
#10241,#10242,#10243,#10244,#10245,#10246,#10247,#10248,#10249,#10250,#10251,
#10252,#10253,#10254,#10255,#10256,#10257,#10258,#10259,#10260,#10261,#10262,
#10263,#10264,#10265,#10266,#10267,#10268,#10269,#10270,#10271,#10272,#10273,
#10274,#10275,#10276,#10277,#10278,#10279,#10280,#10281,#10282,#10283,#10284,
#10285,#10286,#10287,#10288,#10289,#10290,#10291,#10292,#10293,#10294,#10295,
#10296,#10297,#10298,#10299,#10300,#10301,#10302,#10303,#10304,#10305,#10306,
#10307,#10308,#10309,#10310,#10311,#10312,#10313,#10314,#10315,#10316,#10317,
#10318,#10319,#10320,#10321,#10322,#10323,#10324,#10325,#10326,#10327,#10328,
#10329,#10330),.UNSPECIFIED.,.F.,.F.,(4,3,3,3,3,3,3,3,3,3,3,3,3,3,3,3,3,
3,3,3,3,3,3,3,3,3,3,3,3,3,3,3,3,3,3,3,3,3,3,3,3,3,3,3,3,3,3,3,3,3,3,3,3,
3,3,3,3,4),(28.2743338823092,28.2962014820146,28.3776854389874,28.4590647871843,
28.543318162313,28.6244716418665,28.7055483043996,28.7865337170947,28.7960782876993,
28.8770866933325,28.9581709601934,29.0426169934911,29.1239230857728,29.2053068862678,
29.286811558155,29.295955093384,29.3734708701903,29.4509051691213,29.5282735860479,
29.6055916696782,29.6828749321845,29.7601520149366,29.8374285938519,29.9147186876652,
29.9920363200754,30.0694425247984,30.146894532504,30.2244673392231,30.2957087047533,
30.3725573280629,30.4493121745814,30.5259895141068,30.6026055540021,30.6791764527465,
30.7562121856686,30.8327546044912,30.9093029411695,30.9858717727319,31.0632694085796,
31.1399604896431,31.2177114028829,31.2954623161227,31.3729798679754,31.4504100876332,
31.5277686307702,31.6050711016021,31.6823330637999,31.7595802898336,31.8368218012941,
31.9140716517821,31.9913438969519,32.0686968551811,32.1460912477492,32.2235995756764,
32.2952159274921,32.3727404680712,32.4501637622965,32.5116015420207),
 .UNSPECIFIED.);
#120=B_SPLINE_CURVE_WITH_KNOTS('',3,(#10331,#10332,#10333,#10334,#10335,
#10336,#10337,#10338,#10339,#10340,#10341,#10342,#10343,#10344,#10345,#10346,
#10347,#10348,#10349,#10350,#10351,#10352,#10353,#10354,#10355,#10356,#10357,
#10358,#10359,#10360,#10361,#10362,#10363,#10364,#10365,#10366,#10367,#10368,
#10369,#10370,#10371,#10372,#10373,#10374,#10375,#10376,#10377,#10378,#10379,
#10380,#10381,#10382,#10383,#10384,#10385,#10386,#10387,#10388,#10389,#10390,
#10391,#10392,#10393,#10394,#10395,#10396,#10397,#10398,#10399,#10400,#10401,
#10402,#10403,#10404,#10405,#10406,#10407,#10408,#10409,#10410,#10411,#10412),
 .UNSPECIFIED.,.F.,.F.,(4,3,3,3,3,3,3,3,3,3,3,3,3,3,3,3,3,3,3,3,3,3,3,3,
3,3,3,4),(26.2276065244835,26.2966942592759,26.3735154661939,26.4502474382501,
26.5269064263103,26.6035086227474,26.6800701746596,26.7571173866578,26.8336615714257,
26.9102158616206,26.9867948367697,27.0642080952385,27.1409195856865,27.2186837281658,
27.2964478706452,27.3737810706327,27.4510218443257,27.5281860713245,27.605289574782,
27.6823481331002,27.7593848991671,27.836412147927,27.9134441159848,27.9904950400087,
28.0676179573777,28.1447798002582,28.2220420502019,28.2743338821727),
 .UNSPECIFIED.);
#121=B_SPLINE_CURVE_WITH_KNOTS('',3,(#10414,#10415,#10416,#10417,#10418,
#10419,#10420,#10421,#10422,#10423,#10424,#10425,#10426,#10427,#10428,#10429,
#10430,#10431,#10432,#10433,#10434,#10435,#10436,#10437,#10438,#10439,#10440,
#10441,#10442,#10443,#10444,#10445,#10446,#10447,#10448,#10449,#10450,#10451,
#10452,#10453,#10454,#10455,#10456,#10457,#10458,#10459,#10460,#10461,#10462,
#10463,#10464,#10465,#10466,#10467,#10468,#10469,#10470,#10471,#10472,#10473,
#10474,#10475,#10476,#10477,#10478,#10479,#10480,#10481,#10482,#10483,#10484,
#10485,#10486,#10487,#10488,#10489,#10490,#10491,#10492,#10493,#10494,#10495),
 .UNSPECIFIED.,.F.,.F.,(4,3,3,3,3,3,3,3,3,3,3,3,3,3,3,3,3,3,3,3,3,3,3,3,
3,3,3,4),(26.2274102502822,26.3047485634863,26.3821761878827,26.4596522575986,
26.5372438213464,26.5911529685832,26.6680164211604,26.7447863214985,26.8214789265624,
26.8981104312959,26.9746969820839,27.0515549814027,27.1281133751358,27.2046777808017,
27.2812627650986,27.3583373179825,27.435044209929,27.5123025932816,27.5895609766342,
27.6669870549331,27.7442937112837,27.821530825017,27.8987126059822,27.975853229399,
28.0529751002743,28.130084055375,28.2072164237887,28.2743338823091),
 .UNSPECIFIED.);
#122=B_SPLINE_CURVE_WITH_KNOTS('',3,(#10496,#10497,#10498,#10499,#10500,
#10501,#10502,#10503,#10504,#10505,#10506,#10507,#10508,#10509,#10510,#10511,
#10512,#10513,#10514,#10515,#10516,#10517,#10518,#10519,#10520,#10521,#10522,
#10523,#10524,#10525,#10526,#10527,#10528,#10529,#10530,#10531,#10532,#10533,
#10534,#10535,#10536,#10537,#10538,#10539,#10540,#10541,#10542,#10543,#10544,
#10545,#10546,#10547,#10548,#10549,#10550,#10551,#10552,#10553,#10554,#10555,
#10556,#10557,#10558,#10559,#10560,#10561,#10562,#10563,#10564,#10565,#10566,
#10567,#10568,#10569,#10570,#10571,#10572,#10573,#10574,#10575,#10576,#10577,
#10578,#10579,#10580,#10581,#10582,#10583,#10584,#10585,#10586,#10587,#10588,
#10589,#10590,#10591,#10592,#10593,#10594,#10595,#10596,#10597,#10598,#10599,
#10600,#10601,#10602,#10603,#10604,#10605,#10606,#10607,#10608,#10609,#10610,
#10611,#10612,#10613,#10614,#10615,#10616,#10617,#10618,#10619,#10620,#10621,
#10622,#10623,#10624,#10625,#10626,#10627,#10628,#10629,#10630,#10631,#10632,
#10633,#10634,#10635,#10636,#10637,#10638,#10639,#10640,#10641,#10642,#10643,
#10644,#10645,#10646,#10647,#10648,#10649,#10650,#10651,#10652,#10653,#10654,
#10655,#10656,#10657,#10658,#10659,#10660,#10661,#10662,#10663,#10664),
 .UNSPECIFIED.,.F.,.F.,(4,3,3,3,3,3,3,3,3,3,3,3,3,3,3,3,3,3,3,3,3,3,3,3,
3,3,3,3,3,3,3,3,3,3,3,3,3,3,3,3,3,3,3,3,3,3,3,3,3,3,3,3,3,3,3,3,4),(28.2743338823925,
28.3653751030432,28.4569879802351,28.5492606248583,28.5879689846851,28.6654990819551,
28.7429420901964,28.8203136506885,28.8976293534778,28.9749047482534,29.0521656022372,
29.1294208913882,29.2066846571501,29.283970943089,29.3613377821852,29.4387461535387,
29.5162677639265,29.586376992736,29.6632130347834,29.7399600605163,29.8166343081586,
29.8932519578245,29.9698291446533,30.04669862667,30.1232587394907,30.1998290469636,
30.2764241183324,30.353514338946,30.4302415458469,30.5075132733169,30.5847850007869,
30.6623796722761,30.7398819404659,30.8173074276379,30.8946717011361,30.9719902843659,
31.0492859909964,31.126571037823,31.2038594319365,31.2811651796506,31.3585432218276,
31.4359582957656,31.5134789122165,31.5831930088378,31.6646793075531,31.7460613742313,
31.8301452838893,31.9113025873758,31.9923833559512,32.0733733331285,32.0823970128633,
32.1633981440914,32.2444746546452,32.3256813350582,32.4069598838733,32.4883571744755,
32.5108171892216),.UNSPECIFIED.);
#123=B_SPLINE_CURVE_WITH_KNOTS('',3,(#10670,#10671,#10672,#10673,#10674,
#10675,#10676,#10677,#10678,#10679,#10680,#10681,#10682,#10683,#10684,#10685,
#10686,#10687,#10688,#10689,#10690,#10691,#10692,#10693,#10694,#10695,#10696,
#10697,#10698,#10699,#10700,#10701,#10702,#10703,#10704,#10705,#10706,#10707,
#10708,#10709,#10710,#10711,#10712,#10713,#10714,#10715,#10716,#10717,#10718,
#10719,#10720,#10721,#10722,#10723,#10724,#10725,#10726,#10727,#10728,#10729,
#10730,#10731,#10732,#10733,#10734,#10735,#10736,#10737,#10738,#10739,#10740,
#10741,#10742,#10743,#10744,#10745,#10746,#10747,#10748,#10749,#10750,#10751,
#10752,#10753,#10754,#10755,#10756,#10757,#10758,#10759,#10760,#10761,#10762,
#10763,#10764,#10765,#10766,#10767,#10768,#10769,#10770,#10771,#10772,#10773,
#10774,#10775,#10776,#10777,#10778,#10779,#10780,#10781,#10782,#10783,#10784,
#10785,#10786,#10787,#10788,#10789,#10790,#10791,#10792,#10793,#10794,#10795,
#10796,#10797,#10798,#10799,#10800,#10801,#10802,#10803,#10804,#10805,#10806,
#10807,#10808,#10809,#10810,#10811,#10812,#10813,#10814,#10815,#10816,#10817,
#10818,#10819,#10820,#10821,#10822,#10823,#10824,#10825,#10826),
 .UNSPECIFIED.,.F.,.F.,(4,3,3,3,3,3,3,3,3,3,3,3,3,3,3,3,3,3,3,3,3,3,3,3,
3,3,3,3,3,3,3,3,3,3,3,3,3,3,3,3,3,3,3,3,3,3,3,3,3,3,3,3,4),(34.5575191894888,
34.639981395525,34.7224432532648,34.8049047695584,34.887365951256,34.9698268052072,
35.0522873382615,35.1347475572681,35.217207469076,35.2996670805337,35.3821263984897,
35.4645854297921,35.5470441812887,35.6295026598273,35.7119608722552,35.7944188254196,
35.8768765261672,35.959333981345,36.0417911977997,36.1278034243013,36.2111277687248,
36.2935943741702,36.3760601354117,36.4585250798642,36.5409892349401,36.623452628049,
36.7059152865976,36.7883772379904,36.870838509629,36.9532991289132,37.03575912324,
37.1182185200045,37.2006773465996,37.2831356304163,37.3655933988438,37.4480506792692,
37.5321839146807,37.6146499127723,37.6971142891278,37.77957715339,37.8620386151806,
37.9444987841018,38.0269577697373,38.1094156816546,38.1950115271793,38.2774762637794,
38.3599380357814,38.4423972816235,38.5248544396006,38.6073169578818,38.6897746287368,
38.7722334186875,38.7941824458525),.UNSPECIFIED.);
#124=B_SPLINE_CURVE_WITH_KNOTS('',3,(#10827,#10828,#10829,#10830,#10831,
#10832,#10833,#10834,#10835,#10836,#10837,#10838,#10839,#10840,#10841,#10842,
#10843,#10844,#10845,#10846,#10847,#10848,#10849,#10850,#10851,#10852,#10853,
#10854,#10855,#10856,#10857,#10858,#10859,#10860,#10861,#10862,#10863,#10864,
#10865,#10866,#10867,#10868,#10869,#10870,#10871,#10872,#10873,#10874,#10875,
#10876,#10877,#10878,#10879,#10880,#10881,#10882,#10883,#10884,#10885,#10886,
#10887,#10888,#10889,#10890,#10891,#10892,#10893,#10894,#10895,#10896,#10897,
#10898,#10899,#10900,#10901,#10902,#10903,#10904,#10905),.UNSPECIFIED.,
 .F.,.F.,(4,3,3,3,3,3,3,3,3,3,3,3,3,3,3,3,3,3,3,3,3,3,3,3,3,3,4),(32.5116015420207,
32.5889141847545,32.666183147843,32.7447814467203,32.8220229675921,32.8992702080937,
32.9765372229118,33.0561453018992,33.1335323916167,33.214250965239,33.2949695388614,
33.3717907360345,33.4485226982671,33.5251816764331,33.6017838629126,33.6783454048116,
33.755392622989,33.8319367976511,33.908491077714,33.9850700427109,34.0624833195909,
34.1391947999148,34.2169589750728,34.2947231502308,34.398883755279,34.5003194542774,
34.5575191894888),.UNSPECIFIED.);
#125=B_SPLINE_CURVE_WITH_KNOTS('',3,(#10907,#10908,#10909,#10910,#10911,
#10912,#10913,#10914,#10915,#10916,#10917,#10918,#10919,#10920,#10921,#10922,
#10923,#10924,#10925,#10926,#10927,#10928,#10929,#10930,#10931,#10932,#10933,
#10934,#10935,#10936,#10937,#10938,#10939,#10940,#10941,#10942,#10943,#10944,
#10945,#10946,#10947,#10948,#10949,#10950,#10951,#10952,#10953,#10954,#10955,
#10956,#10957,#10958,#10959,#10960,#10961,#10962,#10963,#10964,#10965,#10966,
#10967,#10968,#10969,#10970,#10971,#10972,#10973,#10974,#10975,#10976,#10977,
#10978,#10979,#10980,#10981,#10982,#10983,#10984,#10985,#10986,#10987,#10988),
 .UNSPECIFIED.,.F.,.F.,(4,3,3,3,3,3,3,3,3,3,3,3,3,3,3,3,3,3,3,3,3,3,3,3,
3,3,3,4),(32.5108171892216,32.5816010168887,32.6591291686339,32.7365760421083,
32.8139572193074,32.8912882352399,32.9685845885241,33.0458748872923,33.1231647934493,
33.2004683138543,33.2777994603781,33.3552189485883,33.4326843053928,33.5102696900783,
33.5800090249397,33.656604099681,33.7331059794936,33.8095311195445,33.8858959089002,
33.9622166853699,34.0385190780695,34.1148140336137,34.1911162890776,34.2674405842712,
34.3438449513389,34.4202916671493,34.4968502747876,34.5575191893733),
 .UNSPECIFIED.);
#126=B_SPLINE_CURVE_WITH_KNOTS('',3,(#10989,#10990,#10991,#10992,#10993,
#10994,#10995,#10996,#10997,#10998,#10999,#11000,#11001,#11002,#11003,#11004,
#11005,#11006,#11007,#11008,#11009,#11010,#11011,#11012,#11013,#11014,#11015,
#11016,#11017,#11018,#11019,#11020,#11021,#11022,#11023,#11024,#11025,#11026,
#11027,#11028,#11029,#11030,#11031,#11032,#11033,#11034,#11035,#11036,#11037,
#11038,#11039,#11040,#11041,#11042,#11043,#11044,#11045,#11046,#11047,#11048,
#11049,#11050,#11051,#11052,#11053,#11054,#11055,#11056,#11057,#11058,#11059,
#11060,#11061,#11062,#11063,#11064,#11065,#11066,#11067,#11068,#11069,#11070,
#11071,#11072,#11073,#11074,#11075,#11076,#11077,#11078,#11079,#11080,#11081,
#11082,#11083,#11084,#11085,#11086,#11087,#11088,#11089,#11090,#11091,#11092,
#11093,#11094,#11095,#11096,#11097,#11098,#11099,#11100,#11101,#11102,#11103,
#11104,#11105,#11106,#11107,#11108,#11109,#11110,#11111,#11112,#11113,#11114,
#11115,#11116,#11117,#11118,#11119,#11120,#11121,#11122,#11123,#11124,#11125,
#11126,#11127,#11128,#11129,#11130,#11131,#11132,#11133,#11134,#11135,#11136,
#11137,#11138,#11139,#11140,#11141,#11142,#11143,#11144,#11145,#11146,#11147,
#11148,#11149,#11150,#11151,#11152,#11153,#11154,#11155,#11156,#11157),
 .UNSPECIFIED.,.F.,.F.,(4,3,3,3,3,3,3,3,3,3,3,3,3,3,3,3,3,3,3,3,3,3,3,3,
3,3,3,3,3,3,3,3,3,3,3,3,3,3,3,3,3,3,3,3,3,3,3,3,3,3,3,3,3,3,3,3,4),(34.5575191894887,
34.5784170329906,34.6559472296781,34.7333903245148,34.810761958805,34.8880777226114,
34.9653531656302,35.0426140482937,35.1198693541842,35.1971331247264,35.2744194034607,
35.3517862165038,35.4291945514629,35.5067161082775,35.5768250410415,35.6543551589462,
35.7317981881018,35.8091697697655,35.886485493962,35.9637609103589,36.0410217862186,
36.1182770973981,36.1955408853225,36.2728271935386,36.3501940549771,36.4276024487411,
36.5051240814463,36.5752330490924,36.6520690812362,36.7288160969845,36.8054903345689,
36.8821079741115,36.9586851507596,37.0355546390576,37.112114741601,37.188685038769,
37.2652800998119,37.3423703391448,37.4190975357463,37.4963692964448,37.5736410571433,
37.6512357266259,37.7287379927851,37.806163477905,37.8835277493315,37.9608463304722,
38.0381420349939,38.1154270797002,38.1927154716837,38.2700212172599,38.3473992572976,
38.4248143290925,38.5023349434136,38.5720490651942,38.6535432663946,38.7349057059727,
38.7946740022541),.UNSPECIFIED.);
#127=B_SPLINE_CURVE_WITH_KNOTS('',3,(#11163,#11164,#11165,#11166,#11167,
#11168,#11169,#11170,#11171,#11172,#11173,#11174,#11175,#11176,#11177,#11178,
#11179,#11180,#11181,#11182,#11183,#11184,#11185,#11186,#11187,#11188,#11189,
#11190,#11191,#11192,#11193,#11194,#11195,#11196,#11197,#11198,#11199,#11200,
#11201,#11202,#11203,#11204,#11205,#11206,#11207,#11208,#11209,#11210,#11211,
#11212,#11213,#11214,#11215,#11216,#11217,#11218,#11219,#11220,#11221,#11222,
#11223,#11224,#11225,#11226,#11227,#11228,#11229,#11230,#11231,#11232,#11233,
#11234,#11235,#11236,#11237,#11238,#11239,#11240,#11241,#11242,#11243,#11244,
#11245,#11246,#11247,#11248,#11249,#11250,#11251,#11252,#11253,#11254,#11255,
#11256,#11257,#11258,#11259,#11260,#11261,#11262,#11263,#11264,#11265,#11266,
#11267,#11268,#11269,#11270,#11271,#11272,#11273,#11274,#11275,#11276,#11277,
#11278,#11279,#11280,#11281,#11282,#11283,#11284,#11285,#11286,#11287,#11288,
#11289,#11290,#11291,#11292,#11293,#11294,#11295,#11296,#11297,#11298,#11299,
#11300,#11301,#11302,#11303,#11304,#11305,#11306,#11307,#11308,#11309,#11310,
#11311,#11312,#11313,#11314,#11315,#11316,#11317,#11318,#11319,#11320,#11321,
#11322,#11323,#11324,#11325,#11326,#11327,#11328,#11329,#11330,#11331,#11332,
#11333,#11334),.UNSPECIFIED.,.F.,.F.,(4,3,3,3,3,3,3,3,3,3,3,3,3,3,3,3,3,
3,3,3,3,3,3,3,3,3,3,3,3,3,3,3,3,3,3,3,3,3,3,3,3,3,3,3,3,3,3,3,3,3,3,3,3,
3,3,3,3,4),(40.8407044966684,40.9226860206192,41.0048355818795,41.0872473425637,
41.169800636749,41.2525762919204,41.2929984298164,41.3705810534312,41.4480710356402,
41.5254840128659,41.6028355663674,41.680141233279,41.7574238263243,41.8346956132684,
41.9119706131257,41.9892628440641,42.0666275164294,42.1440291248622,42.2215369394709,
42.2927520411857,42.3742360141403,42.4556153782796,42.5398687454273,42.6210222405984,
42.7020989185568,42.7830843463464,42.7926288468704,42.8736372427747,42.9547214996063,
43.0391675378435,43.1204736195508,43.2018574093194,43.2833620703483,43.2925056525551,
43.3700214308182,43.4474557312288,43.5248241496561,43.6021422348063,43.6794254988508,
43.7567025831623,43.8339791636502,43.9112692590475,43.9885868930519,44.0659930993764,
44.1434451086899,44.2210179170119,44.2922592639245,44.3691208876133,44.4458862286764,
44.5247399268615,44.6013498667174,44.6779187437654,44.7544611603038,44.8309916999188,
44.9075431458621,44.9841078702885,45.0607207321892,45.0767158141578),
 .UNSPECIFIED.);
#128=B_SPLINE_CURVE_WITH_KNOTS('',3,(#11335,#11336,#11337,#11338,#11339,
#11340,#11341,#11342,#11343,#11344,#11345,#11346,#11347,#11348,#11349,#11350,
#11351,#11352,#11353,#11354,#11355,#11356,#11357,#11358,#11359,#11360,#11361,
#11362,#11363,#11364,#11365,#11366,#11367,#11368,#11369,#11370,#11371,#11372,
#11373,#11374,#11375,#11376,#11377,#11378,#11379,#11380,#11381,#11382,#11383,
#11384,#11385,#11386,#11387,#11388,#11389,#11390,#11391,#11392,#11393,#11394,
#11395,#11396,#11397,#11398,#11399,#11400,#11401,#11402,#11403,#11404,#11405,
#11406,#11407,#11408,#11409,#11410),.UNSPECIFIED.,.F.,.F.,(4,3,3,3,3,3,
3,3,3,3,3,3,3,3,3,3,3,3,3,3,3,3,3,3,3,4),(38.7941824458525,38.8766440497063,
38.9591049876769,39.0415652871625,39.1240249755595,39.2064840802615,39.2889426286607,
39.371400648147,39.4538581661086,39.5405360617686,39.6230028476043,39.7054679609481,
39.7879315114532,39.870393608751,39.9528543624523,40.0353138821495,40.1177722774172,
40.2002296578144,40.2826960440808,40.3651592460946,40.4476197023751,40.5300778512858,
40.6125434561651,40.6950033353796,40.7774674487435,40.8407044966684),
 .UNSPECIFIED.);
#129=B_SPLINE_CURVE_WITH_KNOTS('',3,(#11412,#11413,#11414,#11415,#11416,
#11417,#11418,#11419,#11420,#11421,#11422,#11423,#11424,#11425,#11426,#11427,
#11428,#11429,#11430,#11431,#11432,#11433,#11434,#11435,#11436,#11437,#11438,
#11439,#11440,#11441,#11442,#11443,#11444,#11445,#11446,#11447,#11448,#11449,
#11450,#11451,#11452,#11453,#11454,#11455,#11456,#11457,#11458,#11459,#11460,
#11461,#11462,#11463,#11464,#11465,#11466,#11467,#11468,#11469,#11470,#11471,
#11472,#11473,#11474,#11475,#11476,#11477,#11478,#11479,#11480,#11481,#11482,
#11483,#11484,#11485,#11486,#11487,#11488,#11489,#11490,#11491,#11492,#11493),
 .UNSPECIFIED.,.F.,.F.,(4,3,3,3,3,3,3,3,3,3,3,3,3,3,3,3,3,3,3,3,3,3,3,3,
3,3,3,4),(38.7946740022541,38.8758554047595,38.9569584929794,39.037964427007,
39.0712530692197,39.1522661755758,39.2333548699162,39.3176304207485,39.3989398872088,
39.4803267884912,39.5618339273282,39.5704570732452,39.6479852264478,39.7254321014026,
39.8028132801034,39.8801442975572,39.9574406523807,40.03473095271,40.1120208604414,
40.1893243824326,40.2666555305528,40.3440750203668,40.4215403787817,40.4991257650728,
40.5688650812961,40.6659056003397,40.7613323688028,40.8407044966683),
 .UNSPECIFIED.);
#130=B_SPLINE_CURVE_WITH_KNOTS('',3,(#11494,#11495,#11496,#11497,#11498,
#11499,#11500,#11501,#11502,#11503,#11504,#11505,#11506,#11507,#11508,#11509,
#11510,#11511,#11512,#11513,#11514,#11515,#11516,#11517,#11518,#11519,#11520,
#11521,#11522,#11523,#11524,#11525,#11526,#11527,#11528,#11529,#11530,#11531,
#11532,#11533,#11534,#11535,#11536,#11537,#11538,#11539,#11540,#11541,#11542,
#11543,#11544,#11545,#11546,#11547,#11548,#11549,#11550,#11551,#11552,#11553,
#11554,#11555,#11556,#11557,#11558,#11559,#11560,#11561,#11562,#11563,#11564,
#11565,#11566,#11567,#11568,#11569,#11570,#11571,#11572,#11573,#11574,#11575,
#11576,#11577,#11578,#11579,#11580,#11581,#11582,#11583,#11584,#11585,#11586,
#11587,#11588,#11589,#11590,#11591,#11592,#11593,#11594,#11595,#11596,#11597,
#11598,#11599,#11600,#11601,#11602,#11603,#11604,#11605,#11606,#11607,#11608,
#11609,#11610,#11611,#11612,#11613,#11614,#11615,#11616,#11617,#11618,#11619,
#11620,#11621,#11622,#11623,#11624,#11625,#11626,#11627,#11628,#11629,#11630,
#11631,#11632,#11633,#11634,#11635,#11636,#11637,#11638,#11639,#11640,#11641,
#11642,#11643,#11644,#11645,#11646,#11647,#11648,#11649,#11650),
 .UNSPECIFIED.,.F.,.F.,(4,3,3,3,3,3,3,3,3,3,3,3,3,3,3,3,3,3,3,3,3,3,3,3,
3,3,3,3,3,3,3,3,3,3,3,3,3,3,3,3,3,3,3,3,3,3,3,3,3,3,3,3,4),(40.8407044966683,
40.9231667027045,41.0056285604443,41.088090076738,41.1705512584355,41.2530121123868,
41.3354726454411,41.4179328644477,41.5003927762555,41.5828523877132,41.6653117056691,
41.7477707369714,41.830229488468,41.9126879670064,41.9951461794344,42.0776041325986,
42.1600618333463,42.242519288524,42.3249765049787,42.4109887314803,42.4943130759038,
42.5767796813492,42.6592454425907,42.7417103870432,42.8241745421191,42.906637935228,
42.9891005937767,43.0715625451694,43.1540238168081,43.2364844360922,43.318944430419,
43.4014038271835,43.4838626537786,43.5663209375953,43.6487787060228,43.7312359864481,
43.8153692218596,43.8978352199512,43.9802995963067,44.062762460569,44.1452239223596,
44.2276840912808,44.3101430769163,44.3926009888336,44.4781968343584,44.5606615709585,
44.6431233429604,44.7255825888025,44.8080397467795,44.8905022650607,44.9729599359157,
45.0554187258664,45.0773677530319),.UNSPECIFIED.);
#131=B_SPLINE_CURVE_WITH_KNOTS('',3,(#11656,#11657,#11658,#11659,#11660,
#11661,#11662,#11663,#11664,#11665,#11666,#11667,#11668,#11669,#11670,#11671,
#11672,#11673,#11674,#11675,#11676,#11677,#11678,#11679,#11680,#11681,#11682,
#11683,#11684,#11685,#11686,#11687,#11688,#11689,#11690,#11691,#11692,#11693,
#11694,#11695,#11696,#11697,#11698,#11699,#11700,#11701,#11702,#11703,#11704,
#11705,#11706,#11707,#11708,#11709,#11710,#11711,#11712,#11713,#11714,#11715,
#11716,#11717,#11718,#11719,#11720,#11721,#11722,#11723,#11724,#11725,#11726,
#11727,#11728,#11729,#11730,#11731,#11732,#11733,#11734,#11735,#11736,#11737,
#11738,#11739,#11740,#11741,#11742,#11743,#11744,#11745,#11746,#11747,#11748,
#11749,#11750,#11751,#11752,#11753,#11754,#11755,#11756,#11757,#11758,#11759,
#11760,#11761,#11762,#11763,#11764,#11765,#11766,#11767,#11768,#11769,#11770,
#11771,#11772,#11773,#11774,#11775,#11776,#11777,#11778,#11779,#11780,#11781,
#11782,#11783,#11784,#11785,#11786,#11787,#11788,#11789,#11790,#11791,#11792,
#11793,#11794,#11795,#11796,#11797,#11798,#11799,#11800,#11801,#11802,#11803,
#11804,#11805,#11806,#11807,#11808,#11809,#11810,#11811,#11812,#11813,#11814,
#11815,#11816,#11817,#11818,#11819,#11820,#11821,#11822,#11823,#11824),
 .UNSPECIFIED.,.F.,.F.,(4,3,3,3,3,3,3,3,3,3,3,3,3,3,3,3,3,3,3,3,3,3,3,3,
3,3,3,3,3,3,3,3,3,3,3,3,3,3,3,3,3,3,3,3,3,3,3,3,3,3,3,3,3,3,3,3,4),(47.123889803848,
47.2517194303792,47.2915200980326,47.3683412951874,47.4450732574017,47.5217322355495,
47.5983344220109,47.6748959638918,47.7519431820806,47.8284873567249,47.9050416367702,
47.9816206017498,48.0590338786628,48.1357453589698,48.2135095341858,48.2912737094019,
48.3688563330162,48.4463463152247,48.5237592924499,48.601110845951,48.6784165128622,
48.7556991059071,48.8329708928507,48.9102458927076,48.9875381236454,49.0649027960103,
49.1423044044427,49.2198122190509,49.2910273207713,49.3725112937265,49.4538906578663,
49.5381440250137,49.6192975201854,49.7003741981444,49.7813596259345,49.790904126456,
49.8719125223601,49.9529967791915,50.0374428174288,50.1187488991358,50.2001326889043,
50.2816373499328,50.2907809321407,50.3682967104038,50.4457310108144,50.5230994292416,
50.6004175143919,50.6777007784363,50.7549778627479,50.8322544432357,50.9095445386331,
50.9868621726374,51.0642683789619,51.1417203882753,51.2192931965973,51.29053454351,
51.3611629585881),.UNSPECIFIED.);
#132=B_SPLINE_CURVE_WITH_KNOTS('',3,(#11825,#11826,#11827,#11828,#11829,
#11830,#11831,#11832,#11833,#11834,#11835,#11836,#11837,#11838,#11839,#11840,
#11841,#11842,#11843,#11844,#11845,#11846,#11847,#11848,#11849,#11850,#11851,
#11852,#11853,#11854,#11855,#11856,#11857,#11858,#11859,#11860,#11861,#11862,
#11863,#11864,#11865,#11866,#11867,#11868,#11869,#11870,#11871,#11872,#11873,
#11874,#11875,#11876,#11877,#11878,#11879,#11880,#11881,#11882,#11883,#11884,
#11885,#11886,#11887,#11888,#11889,#11890,#11891,#11892,#11893,#11894,#11895,
#11896,#11897,#11898,#11899,#11900,#11901,#11902,#11903,#11904,#11905,#11906),
 .UNSPECIFIED.,.F.,.F.,(4,3,3,3,3,3,3,3,3,3,3,3,3,3,3,3,3,3,3,3,3,3,3,3,
3,3,3,4),(45.0767158141578,45.1534176377557,45.2302334351738,45.2920128752938,
45.3695304269119,45.4469606463314,45.5243191892268,45.6016216598141,45.6788836217642,
45.7561308475469,45.8333723587542,45.910622208987,45.9878944538999,46.0652474118709,
46.1426418041797,46.2201501318482,46.2917664866632,46.3680381413798,46.4442228719431,
46.5203373350376,46.5963945826144,46.6724205164471,46.7484300824388,46.8244382133086,
46.9004926659308,46.976569510054,47.0527320234986,47.1238898037382),
 .UNSPECIFIED.);
#133=B_SPLINE_CURVE_WITH_KNOTS('',3,(#11908,#11909,#11910,#11911,#11912,
#11913,#11914,#11915,#11916,#11917,#11918,#11919,#11920,#11921,#11922,#11923,
#11924,#11925,#11926,#11927,#11928,#11929,#11930,#11931,#11932,#11933,#11934,
#11935,#11936,#11937,#11938,#11939,#11940,#11941,#11942,#11943,#11944,#11945,
#11946,#11947,#11948,#11949,#11950,#11951,#11952,#11953,#11954,#11955,#11956,
#11957,#11958,#11959,#11960,#11961,#11962,#11963,#11964,#11965,#11966,#11967,
#11968,#11969,#11970,#11971,#11972,#11973,#11974,#11975,#11976,#11977,#11978,
#11979,#11980,#11981,#11982,#11983),.UNSPECIFIED.,.F.,.F.,(4,3,3,3,3,3,
3,3,3,3,3,3,3,3,3,3,3,3,3,3,3,3,3,3,3,4),(45.0773677530319,45.1598293568857,
45.2422902948563,45.3247505943419,45.4072102827389,45.4896693874409,45.5721279358401,
45.6545859553264,45.7370434732879,45.8237213689479,45.9061881547836,45.9886532681274,
46.0711168186325,46.1535789159302,46.2360396696316,46.3184991893287,46.4009575845963,
46.4834149649933,46.5658813512597,46.6483445532735,46.7308050095539,46.8132631584647,
46.895728763344,46.9781886425586,47.0606527559224,47.1238898038478),
 .UNSPECIFIED.);
#134=B_SPLINE_CURVE_WITH_KNOTS('',3,(#11984,#11985,#11986,#11987,#11988,
#11989,#11990,#11991,#11992,#11993,#11994,#11995,#11996,#11997,#11998,#11999,
#12000,#12001,#12002,#12003,#12004,#12005,#12006,#12007,#12008,#12009,#12010,
#12011,#12012,#12013,#12014,#12015,#12016,#12017,#12018,#12019,#12020,#12021,
#12022,#12023,#12024,#12025,#12026,#12027,#12028,#12029,#12030,#12031,#12032,
#12033,#12034,#12035,#12036,#12037,#12038,#12039,#12040,#12041,#12042,#12043,
#12044,#12045,#12046,#12047,#12048,#12049,#12050,#12051,#12052,#12053,#12054,
#12055,#12056,#12057,#12058,#12059,#12060,#12061,#12062,#12063,#12064,#12065,
#12066,#12067,#12068,#12069,#12070,#12071,#12072,#12073,#12074,#12075,#12076,
#12077,#12078,#12079,#12080,#12081,#12082,#12083,#12084,#12085,#12086,#12087,
#12088,#12089,#12090,#12091,#12092,#12093,#12094,#12095,#12096,#12097,#12098,
#12099,#12100,#12101,#12102,#12103,#12104,#12105,#12106,#12107,#12108,#12109,
#12110,#12111,#12112,#12113,#12114,#12115,#12116,#12117,#12118,#12119,#12120,
#12121,#12122,#12123,#12124,#12125,#12126,#12127,#12128,#12129,#12130,#12131,
#12132,#12133,#12134,#12135,#12136,#12137,#12138,#12139,#12140,#12141,#12142,
#12143,#12144,#12145,#12146,#12147,#12148,#12149),.UNSPECIFIED.,.F.,.F.,
(4,3,3,3,3,3,3,3,3,3,3,3,3,3,3,3,3,3,3,3,3,3,3,3,3,3,3,3,3,3,3,3,3,3,3,
3,3,3,3,3,3,3,3,3,3,3,3,3,3,3,3,3,3,3,3,4),(47.1238898038478,47.2087594582049,
47.2959998780668,47.3815228915232,47.4696220145879,47.5577211376525,47.6345845223047,
47.7113543541143,47.7880468901028,47.8646783252696,47.941264806053,48.0181228485093,
48.0946811714726,48.171245506145,48.2478304192723,48.32490510088,48.4016119217489,
48.4788705337262,48.5561291457034,48.6336593421632,48.7111024367686,48.7884740708243,
48.865789834393,48.9430652771715,49.0203261595911,49.0975814652355,49.1748452355298,
49.2521315140141,49.3294983268062,49.4069066615132,49.4844282180761,49.5545371537543,
49.6320672718176,49.7095103011336,49.7868818829591,49.8641976073189,49.9414730238803,
50.0187338999058,50.095989211252,50.1732529993437,50.2505393077278,50.327906169334,
50.4053145632661,50.482836196138,50.5529451618052,50.6297918919989,50.7065473799042,
50.7832278737467,50.8598420747927,50.9364195440692,51.0129748672405,51.0895226140708,
51.166100998141,51.2426961532365,51.3193532626057,51.3596845371041),
 .UNSPECIFIED.);
#135=B_SPLINE_CURVE_WITH_KNOTS('',3,(#12155,#12156,#12157,#12158,#12159,
#12160,#12161,#12162,#12163,#12164,#12165,#12166,#12167,#12168,#12169,#12170,
#12171,#12172,#12173,#12174,#12175,#12176,#12177,#12178,#12179,#12180,#12181,
#12182,#12183,#12184,#12185,#12186,#12187,#12188,#12189,#12190,#12191,#12192,
#12193,#12194,#12195,#12196,#12197,#12198,#12199,#12200,#12201,#12202,#12203,
#12204,#12205,#12206,#12207,#12208,#12209,#12210,#12211,#12212,#12213,#12214,
#12215,#12216,#12217,#12218,#12219,#12220,#12221,#12222,#12223,#12224,#12225,
#12226,#12227,#12228,#12229,#12230,#12231,#12232,#12233,#12234,#12235,#12236,
#12237,#12238,#12239,#12240,#12241,#12242,#12243,#12244,#12245,#12246,#12247,
#12248,#12249,#12250,#12251,#12252,#12253,#12254,#12255,#12256,#12257,#12258,
#12259,#12260,#12261,#12262,#12263,#12264,#12265,#12266,#12267,#12268,#12269,
#12270,#12271,#12272,#12273,#12274,#12275,#12276,#12277,#12278,#12279,#12280,
#12281,#12282,#12283,#12284,#12285,#12286,#12287,#12288,#12289,#12290,#12291,
#12292,#12293,#12294,#12295,#12296,#12297,#12298,#12299,#12300,#12301,#12302,
#12303,#12304,#12305,#12306,#12307,#12308,#12309,#12310,#12311,#12312,#12313,
#12314,#12315,#12316,#12317,#12318,#12319,#12320,#12321,#12322,#12323,#12324,
#12325,#12326),.UNSPECIFIED.,.F.,.F.,(4,3,3,3,3,3,3,3,3,3,3,3,3,3,3,3,3,
3,3,3,3,3,3,3,3,3,3,3,3,3,3,3,3,3,3,3,3,3,3,3,3,3,3,3,3,3,3,3,3,3,3,3,3,
3,3,3,3,4),(53.4070751111438,53.4835343669011,53.5599178969044,53.63624215006,
53.7125235237776,53.7887875517728,53.8650452206851,53.941311322949,54.0176006546155,
54.0939682612546,54.1703794615919,54.2468951712867,54.2897953776181,54.3666165747729,
54.4433485369872,54.5200075151348,54.5966097015961,54.6731712434767,54.7502184616656,
54.8267626363099,54.9033169163554,54.9798958813348,55.057309158248,55.134020638555,
55.2117848137712,55.2895489889875,55.3671316126018,55.4446215948104,55.5220345720357,
55.5993861255369,55.6766917924485,55.7539743854934,55.8312461724371,55.9085211722938,
55.9858134032314,56.0631780755963,56.1405796840288,56.2180874986371,56.2893026003569,
56.3707865733119,56.4521659374517,56.5364193045992,56.6175727997706,56.6986494777297,
56.7796349055199,56.7891794060416,56.8701878019459,56.9512720587777,57.0357180970148,
57.1170241787221,57.1984079684906,57.2799126295192,57.2890562117262,57.36658694434,
57.4440154159151,57.5213849283417,57.5987011855334,57.6440769298056),
 .UNSPECIFIED.);
#136=B_SPLINE_CURVE_WITH_KNOTS('',3,(#12327,#12328,#12329,#12330,#12331,
#12332,#12333,#12334,#12335,#12336,#12337,#12338,#12339,#12340,#12341,#12342,
#12343,#12344,#12345,#12346,#12347,#12348,#12349,#12350,#12351,#12352,#12353,
#12354,#12355,#12356,#12357,#12358,#12359,#12360,#12361,#12362,#12363,#12364,
#12365,#12366,#12367,#12368,#12369,#12370,#12371,#12372,#12373,#12374,#12375,
#12376,#12377,#12378,#12379,#12380,#12381,#12382,#12383,#12384,#12385,#12386,
#12387,#12388,#12389,#12390,#12391,#12392,#12393,#12394,#12395,#12396,#12397,
#12398,#12399,#12400,#12401,#12402,#12403,#12404,#12405),.UNSPECIFIED.,
 .F.,.F.,(4,3,3,3,3,3,3,3,3,3,3,3,3,3,3,3,3,3,3,3,3,3,3,3,3,3,4),(51.3611629585881,
51.437924793484,51.5146078062219,51.5912282087005,51.6678021628812,51.7456129118809,
51.8221554642554,51.8987029014922,51.9752698002357,52.0540243888966,52.1307129766142,
52.2105005657468,52.2902881548794,52.3678057064975,52.445235925917,52.5225944688125,
52.5998969393998,52.6771589013499,52.7544061271325,52.8316476383397,52.9088974885726,
52.9861697334856,53.0635226914566,53.1409170837653,53.2184254114338,53.2900417662488,
53.4070751110276),.UNSPECIFIED.);
#137=B_SPLINE_CURVE_WITH_KNOTS('',3,(#12407,#12408,#12409,#12410,#12411,
#12412,#12413,#12414,#12415,#12416,#12417,#12418,#12419,#12420,#12421,#12422,
#12423,#12424,#12425,#12426,#12427,#12428,#12429,#12430,#12431,#12432,#12433,
#12434,#12435,#12436,#12437,#12438,#12439,#12440,#12441,#12442,#12443,#12444,
#12445,#12446,#12447,#12448,#12449,#12450,#12451,#12452,#12453,#12454,#12455,
#12456,#12457,#12458,#12459,#12460,#12461,#12462,#12463,#12464,#12465,#12466,
#12467,#12468,#12469,#12470,#12471,#12472,#12473,#12474,#12475,#12476,#12477,
#12478,#12479,#12480,#12481,#12482,#12483,#12484,#12485,#12486,#12487,#12488,
#12489,#12490,#12491),.UNSPECIFIED.,.F.,.F.,(4,3,3,3,3,3,3,3,3,3,3,3,3,
3,3,3,3,3,3,3,3,3,3,3,3,3,3,3,4),(51.3596845371041,51.4364397650722,51.5133076851397,
51.5513531698562,51.6289478392903,51.7064501054006,51.7838755904712,51.8612398618481,
51.938558442939,52.0158541474106,52.0931391920665,52.1704275839996,52.2477333295252,
52.3251113695126,52.4025264412572,52.4800470555284,52.5497611779071,52.63124749234,
52.7126295746991,52.7967134765075,52.8778707953606,52.958951579115,53.0399415711485,
53.0489651819325,53.1255961689623,53.202287407139,53.2790111285547,53.3558252447557,
53.4065880026861),.UNSPECIFIED.);
#138=B_SPLINE_CURVE_WITH_KNOTS('',3,(#12492,#12493,#12494,#12495,#12496,
#12497,#12498,#12499,#12500,#12501,#12502,#12503,#12504,#12505,#12506,#12507,
#12508,#12509,#12510,#12511,#12512,#12513,#12514,#12515,#12516,#12517,#12518,
#12519,#12520,#12521,#12522,#12523,#12524,#12525,#12526,#12527,#12528,#12529,
#12530,#12531,#12532,#12533,#12534,#12535,#12536,#12537,#12538,#12539,#12540,
#12541,#12542,#12543,#12544,#12545,#12546,#12547,#12548,#12549,#12550,#12551,
#12552,#12553,#12554,#12555,#12556,#12557,#12558,#12559,#12560,#12561,#12562,
#12563,#12564,#12565,#12566,#12567,#12568,#12569,#12570,#12571,#12572,#12573,
#12574,#12575,#12576,#12577,#12578,#12579,#12580,#12581,#12582,#12583,#12584,
#12585,#12586,#12587,#12588,#12589,#12590,#12591,#12592,#12593,#12594,#12595,
#12596,#12597,#12598,#12599,#12600,#12601,#12602,#12603,#12604,#12605,#12606,
#12607,#12608,#12609,#12610,#12611,#12612,#12613,#12614,#12615,#12616,#12617,
#12618,#12619,#12620,#12621,#12622,#12623,#12624,#12625,#12626,#12627,#12628,
#12629,#12630,#12631,#12632,#12633,#12634,#12635,#12636,#12637,#12638,#12639,
#12640,#12641,#12642,#12643,#12644,#12645,#12646,#12647,#12648),
 .UNSPECIFIED.,.F.,.F.,(4,3,3,3,3,3,3,3,3,3,3,3,3,3,3,3,3,3,3,3,3,3,3,3,
3,3,3,3,3,3,3,3,3,3,3,3,3,3,3,3,3,3,3,3,3,3,3,3,3,3,3,3,4),(53.4070751110274,
53.4895373170636,53.5719991748034,53.6544606910971,53.7369218727946,53.8193827267458,
53.9018432598001,53.9843034788068,54.0667633906146,54.1492230020723,54.2316823200283,
54.3141413513307,54.3966001028272,54.4790585813658,54.5615167937936,54.6439747469578,
54.7264324477054,54.8088899028833,54.8913471193378,54.9773593458395,55.0606836902629,
55.1431502957084,55.2256160569498,55.3080810014024,55.3905451564784,55.4730085495872,
55.5554712081358,55.6379331595286,55.7203944311673,55.8028550504514,55.8853150447782,
55.9677744415428,56.0502332681379,56.1326915519547,56.215149320382,56.2976066008073,
56.3817398362188,56.4642058343104,56.5466702106659,56.6291330749281,56.7115945367188,
56.7940547056399,56.8765136912755,56.9589716031927,57.0445674487175,57.1270321853176,
57.2094939573196,57.2919532031617,57.3744103611388,57.45687287942,57.539330550275,
57.6217893402258,57.6437383673911),.UNSPECIFIED.);
#139=B_SPLINE_CURVE_WITH_KNOTS('',3,(#12654,#12655,#12656,#12657,#12658,
#12659,#12660,#12661,#12662,#12663,#12664,#12665,#12666,#12667,#12668,#12669,
#12670,#12671,#12672,#12673,#12674,#12675,#12676,#12677,#12678,#12679,#12680,
#12681,#12682,#12683,#12684,#12685,#12686,#12687,#12688,#12689,#12690,#12691,
#12692,#12693,#12694,#12695,#12696,#12697,#12698,#12699,#12700,#12701,#12702,
#12703,#12704,#12705,#12706,#12707,#12708,#12709,#12710,#12711,#12712,#12713,
#12714,#12715,#12716,#12717,#12718,#12719,#12720,#12721,#12722,#12723,#12724,
#12725,#12726,#12727,#12728,#12729,#12730,#12731,#12732,#12733,#12734,#12735,
#12736,#12737,#12738,#12739,#12740,#12741,#12742,#12743,#12744,#12745,#12746,
#12747,#12748,#12749,#12750,#12751,#12752,#12753,#12754,#12755,#12756,#12757,
#12758,#12759,#12760,#12761,#12762,#12763,#12764,#12765,#12766,#12767,#12768,
#12769,#12770,#12771,#12772,#12773,#12774,#12775,#12776,#12777,#12778,#12779,
#12780,#12781,#12782,#12783,#12784,#12785,#12786,#12787,#12788,#12789,#12790,
#12791,#12792,#12793,#12794,#12795,#12796,#12797,#12798,#12799,#12800,#12801,
#12802,#12803,#12804,#12805,#12806,#12807,#12808,#12809,#12810),
 .UNSPECIFIED.,.F.,.F.,(4,3,3,3,3,3,3,3,3,3,3,3,3,3,3,3,3,3,3,3,3,3,3,3,
3,3,3,3,3,3,3,3,3,3,3,3,3,3,3,3,3,3,3,3,3,3,3,3,3,3,3,3,4),(59.6902604182072,
59.7727226242434,59.8551844819832,59.9376459982768,60.0201071799743,60.1025680339255,
60.1850285669798,60.2674887859865,60.3499486977942,60.4324083092519,60.514867627208,
60.5973266585102,60.6797854100069,60.7622438885454,60.8447021009733,60.9271600541376,
61.0096177548854,61.0920752100632,61.1745324265176,61.2605446530193,61.3438689974428,
61.4263356028882,61.5088013641297,61.5912663085822,61.6737304636581,61.756193856767,
61.8386565153156,61.9211184667083,62.003579738347,62.0860403576312,62.168500351958,
62.2509597487226,62.3334185753177,62.4158768591345,62.4983346275619,62.5807919079872,
62.6649251433987,62.7473911414903,62.8298555178458,62.912318382108,62.9947798438987,
63.0772400128198,63.1596989984554,63.2421569103726,63.3277527558974,63.4102174924975,
63.4926792644995,63.5751385103415,63.6575956683186,63.7400581865999,63.822515857455,
63.9049746474057,63.9269236745709),.UNSPECIFIED.);
#140=B_SPLINE_CURVE_WITH_KNOTS('',3,(#12811,#12812,#12813,#12814,#12815,
#12816,#12817,#12818,#12819,#12820,#12821,#12822,#12823,#12824,#12825,#12826,
#12827,#12828,#12829,#12830,#12831,#12832,#12833,#12834,#12835,#12836,#12837,
#12838,#12839,#12840,#12841,#12842,#12843,#12844,#12845,#12846,#12847,#12848,
#12849,#12850,#12851,#12852,#12853,#12854,#12855,#12856,#12857,#12858,#12859,
#12860,#12861,#12862,#12863,#12864,#12865,#12866,#12867,#12868,#12869,#12870,
#12871,#12872,#12873,#12874,#12875,#12876,#12877,#12878,#12879,#12880,#12881,
#12882,#12883,#12884,#12885,#12886,#12887,#12888,#12889,#12890,#12891,#12892),
 .UNSPECIFIED.,.F.,.F.,(4,3,3,3,3,3,3,3,3,3,3,3,3,3,3,3,3,3,3,3,3,3,3,3,
3,3,3,4),(57.6440769298056,57.7246685414669,57.8019436746278,57.8792271368914,
57.9565329492142,58.0338751424344,58.1113087178789,58.1887960545296,58.2663905274488,
58.2888098230956,58.3656584462832,58.4424132926799,58.5190906320844,58.5957066718592,
58.6722775704842,58.7493133034818,58.8258557221875,58.90240405875,58.9789728901979,
59.0563705262647,59.1330616072173,59.2108125208412,59.288563434465,59.3753375230801,
59.4617551097612,59.5479378979409,59.6337172903819,59.6902604182072),
 .UNSPECIFIED.);
#141=B_SPLINE_CURVE_WITH_KNOTS('',3,(#12894,#12895,#12896,#12897,#12898,
#12899,#12900,#12901,#12902,#12903,#12904,#12905,#12906,#12907,#12908,#12909,
#12910,#12911,#12912,#12913,#12914,#12915,#12916,#12917,#12918,#12919,#12920,
#12921,#12922,#12923,#12924,#12925,#12926,#12927,#12928,#12929,#12930,#12931,
#12932,#12933,#12934,#12935,#12936,#12937,#12938,#12939,#12940,#12941,#12942,
#12943,#12944,#12945,#12946,#12947,#12948,#12949,#12950,#12951,#12952,#12953,
#12954,#12955,#12956,#12957,#12958,#12959,#12960,#12961,#12962,#12963,#12964,
#12965,#12966,#12967,#12968,#12969),.UNSPECIFIED.,.F.,.F.,(4,3,3,3,3,3,
3,3,3,3,3,3,3,3,3,3,3,3,3,3,3,3,3,3,3,4),(57.6437383673911,57.7261999712449,
57.8086609092155,57.8911212087012,57.973580897098,58.0560400018002,58.1384985501993,
58.2209565696855,58.3034140876471,58.3900919833071,58.4725587691428,58.5550238824865,
58.6374874329917,58.7199495302894,58.8024102839909,58.884869803688,58.9673281989556,
59.0497855793529,59.1322519656194,59.2147151676331,59.2971756239135,59.3796337728243,
59.4620993777036,59.5445592569181,59.627023370282,59.690260418207),
 .UNSPECIFIED.);
#142=B_SPLINE_CURVE_WITH_KNOTS('',3,(#12970,#12971,#12972,#12973,#12974,
#12975,#12976,#12977,#12978,#12979,#12980,#12981,#12982,#12983,#12984,#12985,
#12986,#12987,#12988,#12989,#12990,#12991,#12992,#12993,#12994,#12995,#12996,
#12997,#12998,#12999,#13000,#13001,#13002,#13003,#13004,#13005,#13006,#13007,
#13008,#13009,#13010,#13011,#13012,#13013,#13014,#13015,#13016,#13017,#13018,
#13019,#13020,#13021,#13022,#13023,#13024,#13025,#13026,#13027,#13028,#13029,
#13030,#13031,#13032,#13033,#13034,#13035,#13036,#13037,#13038,#13039,#13040,
#13041,#13042,#13043,#13044,#13045,#13046,#13047,#13048,#13049,#13050,#13051,
#13052,#13053,#13054,#13055,#13056,#13057,#13058,#13059,#13060,#13061,#13062,
#13063,#13064,#13065,#13066,#13067,#13068,#13069,#13070,#13071,#13072,#13073,
#13074,#13075,#13076,#13077,#13078,#13079,#13080,#13081,#13082,#13083,#13084,
#13085,#13086,#13087,#13088,#13089,#13090,#13091,#13092,#13093,#13094,#13095,
#13096,#13097,#13098,#13099,#13100,#13101,#13102,#13103,#13104,#13105,#13106,
#13107,#13108,#13109,#13110,#13111,#13112,#13113,#13114,#13115,#13116,#13117,
#13118,#13119,#13120,#13121,#13122,#13123,#13124,#13125,#13126,#13127,#13128,
#13129,#13130,#13131,#13132,#13133,#13134,#13135,#13136,#13137,#13138),
 .UNSPECIFIED.,.F.,.F.,(4,3,3,3,3,3,3,3,3,3,3,3,3,3,3,3,3,3,3,3,3,3,3,3,
3,3,3,3,3,3,3,3,3,3,3,3,3,3,3,3,3,3,3,3,3,3,3,3,3,3,3,3,3,3,3,3,4),(59.690777377404,
59.7673619185021,59.8438612447857,59.9203113702036,59.9967242576866,60.037821238289,
60.1188343445795,60.1999230388526,60.284198589718,60.3655080561077,60.4468949573183,
60.5284020960833,60.5370252423144,60.6145533955236,60.6920002704849,60.7693814491924,
60.8467124666531,60.9240088214836,61.0012991218198,61.0785890295582,61.1558925515562,
61.2332236996835,61.3106431895045,61.3881085479264,61.4656939342244,61.5354332503653,
61.6122966350176,61.6890664668272,61.7657590028159,61.8423904379825,61.918976918766,
61.9958349612223,62.0723932841857,62.1489576188581,62.2255425319854,62.3026172135931,
62.379324034462,62.4565826464392,62.5338412584163,62.6113714548761,62.6888145494816,
62.7661861835372,62.8435019471059,62.9207773898842,62.9980382723037,63.075293577948,
63.1525573482421,63.2298436267263,63.3072104395184,63.3846187742254,63.4621403307883,
63.5322492664672,63.6097908036147,63.6891614337623,63.7665285349367,63.8469009295709,
63.9272733242051),.UNSPECIFIED.);
#143=B_SPLINE_CURVE_WITH_KNOTS('',3,(#13144,#13145,#13146,#13147,#13148,
#13149,#13150,#13151,#13152,#13153,#13154,#13155,#13156,#13157,#13158,#13159,
#13160,#13161,#13162,#13163,#13164,#13165,#13166,#13167,#13168,#13169,#13170,
#13171,#13172,#13173,#13174,#13175,#13176,#13177,#13178,#13179,#13180,#13181,
#13182,#13183,#13184,#13185,#13186,#13187,#13188,#13189,#13190,#13191,#13192,
#13193,#13194,#13195,#13196,#13197,#13198,#13199,#13200,#13201,#13202,#13203,
#13204,#13205,#13206,#13207,#13208,#13209,#13210,#13211,#13212,#13213,#13214,
#13215,#13216,#13217,#13218,#13219,#13220,#13221,#13222,#13223,#13224,#13225,
#13226,#13227,#13228,#13229,#13230,#13231,#13232,#13233,#13234,#13235,#13236,
#13237,#13238,#13239,#13240,#13241,#13242,#13243,#13244,#13245,#13246,#13247,
#13248,#13249,#13250,#13251,#13252,#13253,#13254,#13255,#13256,#13257,#13258,
#13259,#13260,#13261,#13262,#13263,#13264,#13265,#13266,#13267,#13268,#13269,
#13270,#13271,#13272,#13273,#13274,#13275,#13276,#13277,#13278,#13279,#13280,
#13281,#13282,#13283,#13284,#13285,#13286,#13287,#13288,#13289,#13290,#13291,
#13292,#13293,#13294,#13295,#13296,#13297,#13298,#13299,#13300,#13301,#13302,
#13303,#13304,#13305,#13306,#13307,#13308,#13309),.UNSPECIFIED.,.F.,.F.,
(4,3,3,3,3,3,3,3,3,3,3,3,3,3,3,3,3,3,3,3,3,3,3,3,3,3,3,3,3,3,3,3,3,3,3,
3,3,3,3,3,3,3,3,3,3,3,3,3,3,3,3,3,3,3,3,4),(65.9734457253868,66.0640275444732,
66.1552001016788,66.2470822494204,66.2868387140505,66.3643562656686,66.4417864850882,
66.5191450279837,66.596447498571,66.6737094605213,66.750956686304,66.8281981975113,
66.905448047744,66.9827202926568,67.0600732506278,67.1374676429365,67.214975970605,
67.2865923254199,67.364109694616,67.4415397620673,67.518898183337,67.5962005625517,
67.6734624633146,67.7507096740056,67.8279511982241,67.9052010895703,67.9824734037138,
68.0598264749397,68.1372210046912,68.2147295096535,68.2863459367893,68.3631671339441,
68.4398990961584,68.5165580743062,68.5931602607676,68.6697218026485,68.7467690208373,
68.8233131954816,68.8998674755269,68.9764464405066,69.0538597174196,69.1305711977265,
69.2083353729425,69.2860995481586,69.3636865021404,69.4411799732403,69.518595601332,
69.5959489704174,69.6732543422776,69.7505336933602,69.8278010512468,69.9050704341445,
69.9823887172598,70.0597308627986,70.1371583399476,70.2096877536336),
 .UNSPECIFIED.);
#144=B_SPLINE_CURVE_WITH_KNOTS('',3,(#13310,#13311,#13312,#13313,#13314,
#13315,#13316,#13317,#13318,#13319,#13320,#13321,#13322,#13323,#13324,#13325,
#13326,#13327,#13328,#13329,#13330,#13331,#13332,#13333,#13334,#13335,#13336,
#13337,#13338,#13339,#13340,#13341,#13342,#13343,#13344,#13345,#13346,#13347,
#13348,#13349,#13350,#13351,#13352,#13353,#13354,#13355,#13356,#13357,#13358,
#13359,#13360,#13361,#13362,#13363,#13364,#13365,#13366,#13367,#13368,#13369,
#13370,#13371,#13372,#13373,#13374,#13375,#13376,#13377,#13378,#13379,#13380,
#13381,#13382,#13383,#13384,#13385),.UNSPECIFIED.,.F.,.F.,(4,3,3,3,3,3,
3,3,3,3,3,3,3,3,3,3,3,3,3,3,3,3,3,3,3,4),(63.9269236745709,64.0093852784247,
64.0918462163953,64.1743065158809,64.2567662042778,64.3392253089798,64.421683857379,
64.5041418768653,64.5865993948268,64.6732772904868,64.7557440763225,64.8382091896663,
64.9206727401714,65.0031348374692,65.0855955911706,65.1680551108677,65.2505135061353,
65.3329708865325,65.415437272799,65.4979004748128,65.5803609310932,65.6628190800038,
65.7452846848831,65.8277445640976,65.9102086774615,65.9734457253868),
 .UNSPECIFIED.);
#145=B_SPLINE_CURVE_WITH_KNOTS('',3,(#13387,#13388,#13389,#13390,#13391,
#13392,#13393,#13394,#13395,#13396,#13397,#13398,#13399,#13400,#13401,#13402,
#13403,#13404,#13405,#13406,#13407,#13408,#13409,#13410,#13411,#13412,#13413,
#13414,#13415,#13416,#13417,#13418,#13419,#13420,#13421,#13422,#13423,#13424,
#13425,#13426,#13427,#13428,#13429,#13430,#13431,#13432,#13433,#13434,#13435,
#13436,#13437,#13438,#13439,#13440,#13441,#13442,#13443,#13444,#13445,#13446,
#13447,#13448,#13449,#13450,#13451,#13452,#13453,#13454,#13455,#13456,#13457,
#13458,#13459,#13460,#13461,#13462,#13463,#13464,#13465,#13466,#13467,#13468),
 .UNSPECIFIED.,.F.,.F.,(4,3,3,3,3,3,3,3,3,3,3,3,3,3,3,3,3,3,3,3,3,3,3,3,
3,3,3,4),(63.9272733242051,64.0045329596442,64.0817885003611,64.1590539876398,
64.2363434656992,64.3137140801567,64.3911275495765,64.4686520662923,64.5306572745181,
64.6074933066408,64.6842403223678,64.7609145599314,64.8375321994535,64.9141093760802,
64.9909788643913,65.0675389669138,65.144109264061,65.2207043250835,65.2977945644549,
65.3745217610364,65.4517935218027,65.529065282569,65.6144079592789,65.6995528569604,
65.7843842943116,65.8690119703541,65.9533377016775,65.9734457253866),
 .UNSPECIFIED.);
#146=B_SPLINE_CURVE_WITH_KNOTS('',3,(#13469,#13470,#13471,#13472,#13473,
#13474,#13475,#13476,#13477,#13478,#13479,#13480,#13481,#13482,#13483,#13484,
#13485,#13486,#13487,#13488,#13489,#13490,#13491,#13492,#13493,#13494,#13495,
#13496,#13497,#13498,#13499,#13500,#13501,#13502,#13503,#13504,#13505,#13506,
#13507,#13508,#13509,#13510,#13511,#13512,#13513,#13514,#13515,#13516,#13517,
#13518,#13519,#13520,#13521,#13522,#13523,#13524,#13525,#13526,#13527,#13528,
#13529,#13530,#13531,#13532,#13533,#13534,#13535,#13536,#13537,#13538,#13539,
#13540,#13541,#13542,#13543,#13544,#13545,#13546,#13547,#13548,#13549,#13550,
#13551,#13552,#13553,#13554,#13555,#13556,#13557,#13558,#13559,#13560,#13561,
#13562,#13563,#13564,#13565,#13566,#13567,#13568,#13569,#13570,#13571,#13572,
#13573,#13574,#13575,#13576,#13577,#13578,#13579,#13580,#13581,#13582,#13583,
#13584,#13585,#13586,#13587,#13588,#13589,#13590,#13591,#13592,#13593,#13594,
#13595,#13596,#13597,#13598,#13599,#13600,#13601,#13602,#13603,#13604,#13605,
#13606,#13607,#13608,#13609,#13610,#13611,#13612,#13613,#13614,#13615,#13616,
#13617,#13618,#13619,#13620,#13621,#13622,#13623,#13624,#13625),
 .UNSPECIFIED.,.F.,.F.,(4,3,3,3,3,3,3,3,3,3,3,3,3,3,3,3,3,3,3,3,3,3,3,3,
3,3,3,3,3,3,3,3,3,3,3,3,3,3,3,3,3,3,3,3,3,3,3,3,3,3,3,3,4),(65.9734457253866,
66.0559079314229,66.1383697891626,66.2208313054562,66.3032924871537,66.3857533411049,
66.4682138741592,66.5506740931658,66.6331340049737,66.7155936164313,66.7980529343874,
66.8805119656898,66.9629707171864,67.0454291957249,67.1278874081526,67.2103453613168,
67.2928030620647,67.3752605172425,67.457717733697,67.5437299601987,67.6270543046221,
67.7095209100676,67.7919866713091,67.8744516157616,67.9569157708375,68.0393791639464,
68.121841822495,68.2043037738878,68.2867650455265,68.3692256648107,68.4516856591375,
68.534145055902,68.6166038824972,68.6990621663138,68.7815199347413,68.8639772151668,
68.9481104505782,69.0305764486698,69.1130408250253,69.1955036892875,69.2779651510782,
69.3604253199993,69.4428843056349,69.5253422175521,69.6109380630769,69.693402799677,
69.775864571679,69.8583238175211,69.9407809754981,70.0232434937793,70.1057011646343,
70.188159954585,70.2101089817503),.UNSPECIFIED.);
#147=B_SPLINE_CURVE_WITH_KNOTS('',3,(#13631,#13632,#13633,#13634,#13635,
#13636,#13637,#13638,#13639,#13640,#13641,#13642,#13643,#13644,#13645,#13646,
#13647,#13648,#13649,#13650,#13651,#13652,#13653,#13654,#13655,#13656,#13657,
#13658,#13659,#13660,#13661,#13662,#13663,#13664,#13665,#13666,#13667,#13668,
#13669,#13670,#13671,#13672,#13673,#13674,#13675,#13676,#13677,#13678,#13679,
#13680,#13681,#13682,#13683,#13684,#13685,#13686,#13687,#13688,#13689,#13690,
#13691,#13692,#13693,#13694,#13695,#13696,#13697,#13698,#13699,#13700,#13701,
#13702,#13703,#13704,#13705,#13706,#13707,#13708,#13709,#13710,#13711,#13712,
#13713,#13714,#13715,#13716,#13717,#13718,#13719,#13720,#13721,#13722,#13723,
#13724,#13725,#13726,#13727,#13728,#13729,#13730,#13731,#13732,#13733,#13734,
#13735,#13736,#13737,#13738,#13739,#13740,#13741,#13742,#13743,#13744,#13745,
#13746,#13747,#13748,#13749,#13750,#13751,#13752,#13753,#13754,#13755,#13756,
#13757,#13758,#13759,#13760,#13761,#13762,#13763,#13764,#13765,#13766,#13767,
#13768,#13769,#13770,#13771,#13772,#13773,#13774,#13775,#13776,#13777,#13778,
#13779,#13780,#13781,#13782,#13783,#13784,#13785,#13786,#13787,#13788,#13789,
#13790,#13791,#13792,#13793,#13794,#13795,#13796,#13797,#13798,#13799),
 .UNSPECIFIED.,.F.,.F.,(4,3,3,3,3,3,3,3,3,3,3,3,3,3,3,3,3,3,3,3,3,3,3,3,
3,3,3,3,3,3,3,3,3,3,3,3,3,3,3,3,3,3,3,3,3,3,3,3,3,3,3,3,3,3,3,3,4),(72.2566310325664,
72.2853603822667,72.3622090054542,72.4389638518509,72.5156411912554,72.5922572310304,
72.6688281296554,72.745863862653,72.8224062813587,72.8989546179213,72.975523449369,
73.0529210854358,73.1296121663885,73.2073630800123,73.2851139936361,73.3626315452542,
73.4400617646737,73.5174203075691,73.5947227781564,73.6719847401067,73.7492319658892,
73.8264734770964,73.9037233273291,73.9809955722419,74.0583485302129,74.1357429225217,
74.2132512501902,74.2848676050055,74.3623849742017,74.4398150416529,74.5171734629223,
74.594475842137,74.6717377429,74.7489849535909,74.8262264778095,74.9034763691557,
74.9807486832996,75.0581017545255,75.1354962842769,75.2130047892393,75.2846212163748,
75.3614424135295,75.4381743757438,75.5148333538919,75.5914355403534,75.6679970822344,
75.7450443004231,75.8215884750676,75.8981427551129,75.9747217200926,76.0521349970055,
76.1288464773124,76.2066106525283,76.2843748277442,76.3619669411825,76.4394513885415,
76.4938209771541),.UNSPECIFIED.);
#148=B_SPLINE_CURVE_WITH_KNOTS('',3,(#13800,#13801,#13802,#13803,#13804,
#13805,#13806,#13807,#13808,#13809,#13810,#13811,#13812,#13813,#13814,#13815,
#13816,#13817,#13818,#13819,#13820,#13821,#13822,#13823,#13824,#13825,#13826,
#13827,#13828,#13829,#13830,#13831,#13832,#13833,#13834,#13835,#13836,#13837,
#13838,#13839,#13840,#13841,#13842,#13843,#13844,#13845,#13846,#13847,#13848,
#13849,#13850,#13851,#13852,#13853,#13854,#13855,#13856,#13857,#13858,#13859,
#13860,#13861,#13862,#13863,#13864,#13865,#13866,#13867,#13868,#13869,#13870,
#13871,#13872,#13873,#13874,#13875,#13876,#13877,#13878,#13879,#13880,#13881,
#13882,#13883,#13884),.UNSPECIFIED.,.F.,.F.,(4,3,3,3,3,3,3,3,3,3,3,3,3,
3,3,3,3,3,3,3,3,3,3,3,3,3,3,3,4),(70.2096877536336,70.285853159528,70.3673371324832,
70.4487164966231,70.5329698637705,70.6141233589421,70.6952000369013,70.7761854646915,
70.7857299652127,70.8667383611168,70.9478226179482,71.0322686561855,71.1135747378926,
71.194958527661,71.2764631886896,71.2856067708974,71.3627095955525,71.43973077825,
71.5166863056749,71.5935921150844,71.6704641059723,71.7473312580087,71.8241995322672,
71.9010832966186,71.9779969254215,72.0549985610845,72.132048764585,72.209212210575,
72.2566310324216),.UNSPECIFIED.);
#149=B_SPLINE_CURVE_WITH_KNOTS('',3,(#13886,#13887,#13888,#13889,#13890,
#13891,#13892,#13893,#13894,#13895,#13896,#13897,#13898,#13899,#13900,#13901,
#13902,#13903,#13904,#13905,#13906,#13907,#13908,#13909,#13910,#13911,#13912,
#13913,#13914,#13915,#13916,#13917,#13918,#13919,#13920,#13921,#13922,#13923,
#13924,#13925,#13926,#13927,#13928,#13929,#13930,#13931,#13932,#13933,#13934,
#13935,#13936,#13937,#13938,#13939,#13940,#13941,#13942,#13943,#13944,#13945,
#13946,#13947,#13948,#13949,#13950,#13951,#13952,#13953,#13954,#13955,#13956,
#13957,#13958,#13959,#13960,#13961),.UNSPECIFIED.,.F.,.F.,(4,3,3,3,3,3,
3,3,3,3,3,3,3,3,3,3,3,3,3,3,3,3,3,3,3,4),(70.2101089817503,70.292570585604,
70.3750315235746,70.4574918230603,70.5399515114572,70.6224106161593,70.7048691645584,
70.7873271840447,70.8697847020062,70.9564625976662,71.0389293835019,71.1213944968457,
71.2038580473508,71.2863201446486,71.36878089835,71.4512404180471,71.5336988133147,
71.6161561937119,71.6986225799783,71.781085781992,71.8635462382725,71.9460043871834,
72.0284699920626,72.1109298712771,72.193393984641,72.2566310325662),
 .UNSPECIFIED.);
#150=B_SPLINE_CURVE_WITH_KNOTS('',3,(#13962,#13963,#13964,#13965,#13966,
#13967,#13968,#13969,#13970,#13971,#13972,#13973,#13974,#13975,#13976,#13977,
#13978,#13979,#13980,#13981,#13982,#13983,#13984,#13985,#13986,#13987,#13988,
#13989,#13990,#13991,#13992,#13993,#13994,#13995,#13996,#13997,#13998,#13999,
#14000,#14001,#14002,#14003,#14004,#14005,#14006,#14007,#14008,#14009,#14010,
#14011,#14012,#14013,#14014,#14015,#14016,#14017,#14018,#14019,#14020,#14021,
#14022,#14023,#14024,#14025,#14026,#14027,#14028,#14029,#14030,#14031,#14032,
#14033,#14034,#14035,#14036,#14037,#14038,#14039,#14040,#14041,#14042,#14043,
#14044,#14045,#14046,#14047,#14048,#14049,#14050,#14051,#14052,#14053,#14054,
#14055,#14056,#14057,#14058,#14059,#14060,#14061,#14062,#14063,#14064,#14065,
#14066,#14067,#14068,#14069,#14070,#14071,#14072,#14073,#14074,#14075,#14076,
#14077,#14078,#14079,#14080,#14081,#14082,#14083,#14084,#14085,#14086,#14087,
#14088,#14089,#14090,#14091,#14092,#14093,#14094,#14095,#14096,#14097,#14098,
#14099,#14100,#14101,#14102,#14103,#14104,#14105,#14106,#14107,#14108,#14109,
#14110,#14111,#14112,#14113,#14114,#14115,#14116,#14117,#14118,#14119,#14120,
#14121,#14122,#14123,#14124,#14125,#14126,#14127,#14128,#14129,#14130),
 .UNSPECIFIED.,.F.,.F.,(4,3,3,3,3,3,3,3,3,3,3,3,3,3,3,3,3,3,3,3,3,3,3,3,
3,3,3,3,3,3,3,3,3,3,3,3,3,3,3,3,3,3,3,3,3,3,3,3,3,3,3,3,3,3,3,3,4),(72.2566310325662,
72.3530747522459,72.4514122093326,72.5179213389254,72.5955160083595,72.6730182744698,
72.7504437595404,72.8278080309172,72.9051266120081,72.9824223164796,73.0597073611356,
73.1369957530686,73.2143014985944,73.2916795385818,73.3690946103264,73.4466152245976,
73.5163293469763,73.5978156614092,73.6791977437682,73.7632816455766,73.8444389644296,
73.925519748184,74.0065097402177,74.0155333510018,74.0965464572923,74.1776351515654,
74.2619107024309,74.3432201688204,74.4246070700312,74.5061142087961,74.5147373550273,
74.5922655082364,74.6697123831978,74.7470935619053,74.8244245793659,74.9017209341962,
74.9790112345324,75.0563011422706,75.1336046642688,75.2109358123959,75.2883553022169,
75.3658206606387,75.4434060469367,75.5131453630782,75.5900097845677,75.66678043819,
75.7434735819713,75.8201054116923,75.8966920743709,75.973257994182,76.0498150013944,
76.1263776610667,76.2029605393919,76.2796199398358,76.3563198459075,76.433127667564,
76.4930533832794),.UNSPECIFIED.);
#151=B_SPLINE_CURVE_WITH_KNOTS('',3,(#14136,#14137,#14138,#14139,#14140,
#14141,#14142,#14143,#14144,#14145,#14146,#14147,#14148,#14149,#14150,#14151,
#14152,#14153,#14154,#14155,#14156,#14157,#14158,#14159,#14160,#14161,#14162,
#14163,#14164,#14165,#14166,#14167,#14168,#14169,#14170,#14171,#14172,#14173,
#14174,#14175,#14176,#14177,#14178,#14179,#14180,#14181,#14182,#14183,#14184,
#14185,#14186,#14187,#14188,#14189,#14190,#14191,#14192,#14193,#14194,#14195,
#14196,#14197,#14198,#14199,#14200,#14201,#14202,#14203,#14204,#14205,#14206,
#14207,#14208,#14209,#14210,#14211,#14212,#14213,#14214,#14215,#14216,#14217,
#14218,#14219,#14220,#14221,#14222,#14223,#14224,#14225,#14226,#14227,#14228,
#14229,#14230,#14231,#14232,#14233,#14234,#14235,#14236,#14237,#14238,#14239,
#14240,#14241,#14242,#14243,#14244,#14245,#14246,#14247,#14248,#14249,#14250,
#14251,#14252,#14253,#14254,#14255,#14256,#14257,#14258,#14259,#14260,#14261,
#14262,#14263,#14264,#14265,#14266,#14267,#14268,#14269,#14270,#14271,#14272,
#14273,#14274,#14275,#14276,#14277,#14278,#14279,#14280,#14281,#14282,#14283,
#14284,#14285,#14286,#14287,#14288,#14289,#14290,#14291,#14292),
 .UNSPECIFIED.,.F.,.F.,(4,3,3,3,3,3,3,3,3,3,3,3,3,3,3,3,3,3,3,3,3,3,3,3,
3,3,3,3,3,3,3,3,3,3,3,3,3,3,3,3,3,3,3,3,3,3,3,3,3,3,3,3,4),(78.539816339746,
78.6222785457822,78.7047404035219,78.7872019198156,78.869663101513,78.9521239554642,
79.0345844885185,79.1170447075251,79.1995046193329,79.2819642307906,79.3644235487466,
79.4468825800489,79.5293413315456,79.6117998100843,79.6942580225122,79.7767159756763,
79.8591736764241,79.941631131602,80.0240883480567,80.1101005745584,80.1934249189818,
80.2758915244273,80.3583572856687,80.4408222301212,80.5232863851971,80.605749778306,
80.6882124368546,80.7706743882473,80.853135659886,80.9355962791702,81.0180562734971,
81.1005156702615,81.1829744968567,81.2654327806733,81.3478905491008,81.430347829526,
81.5144810649375,81.5969470630291,81.6794114393846,81.7618743036468,81.8443357654375,
81.9267959343587,82.0092549199942,82.0917128319114,82.1773086774362,82.2597734140363,
82.3422351860383,82.4246944318803,82.5071515898574,82.5896141081386,82.6720717789937,
82.7545305689444,82.7764795961097),.UNSPECIFIED.);
#152=B_SPLINE_CURVE_WITH_KNOTS('',3,(#14293,#14294,#14295,#14296,#14297,
#14298,#14299,#14300,#14301,#14302,#14303,#14304,#14305,#14306,#14307,#14308,
#14309,#14310,#14311,#14312,#14313,#14314,#14315,#14316,#14317,#14318,#14319,
#14320,#14321,#14322,#14323,#14324,#14325,#14326,#14327,#14328,#14329,#14330,
#14331,#14332,#14333,#14334,#14335,#14336,#14337,#14338,#14339,#14340,#14341,
#14342,#14343,#14344,#14345,#14346,#14347,#14348,#14349,#14350,#14351,#14352,
#14353,#14354,#14355,#14356,#14357,#14358,#14359,#14360,#14361,#14362,#14363,
#14364,#14365,#14366,#14367,#14368,#14369,#14370,#14371,#14372,#14373,#14374,
#14375,#14376,#14377),.UNSPECIFIED.,.F.,.F.,(4,3,3,3,3,3,3,3,3,3,3,3,3,
3,3,3,3,3,3,3,3,3,3,3,3,3,3,3,4),(76.4938209771541,76.5711891910363,76.6485068967613,
76.7279595895554,76.80523291,76.8825056629844,76.9597918661467,77.0408760093884,
77.1182683546864,77.1957074620667,77.2732383485027,77.2841284391136,77.3656124120689,
77.4469917762085,77.5312451433559,77.6123986385272,77.6934753164871,77.7744607442775,
77.7840052447983,77.8650136407026,77.9460978975344,78.0305439357715,78.1118500174784,
78.1932338072473,78.2747384682758,78.2838820504829,78.380327679951,78.4755543569099,
78.539816339746),.UNSPECIFIED.);
#153=B_SPLINE_CURVE_WITH_KNOTS('',3,(#14379,#14380,#14381,#14382,#14383,
#14384,#14385,#14386,#14387,#14388,#14389,#14390,#14391,#14392,#14393,#14394,
#14395,#14396,#14397,#14398,#14399,#14400,#14401,#14402,#14403,#14404,#14405,
#14406,#14407,#14408,#14409,#14410,#14411,#14412,#14413,#14414,#14415,#14416,
#14417,#14418,#14419,#14420,#14421,#14422,#14423,#14424,#14425,#14426,#14427,
#14428,#14429,#14430,#14431,#14432,#14433,#14434,#14435,#14436,#14437,#14438,
#14439,#14440,#14441,#14442,#14443,#14444,#14445,#14446,#14447,#14448,#14449,
#14450,#14451,#14452,#14453,#14454,#14455,#14456,#14457,#14458,#14459,#14460,
#14461,#14462,#14463),.UNSPECIFIED.,.F.,.F.,(4,3,3,3,3,3,3,3,3,3,3,3,3,
3,3,3,3,3,3,3,3,3,3,3,3,3,3,3,4),(76.4930533832794,76.5115533711291,76.5890835675889,
76.6665266621943,76.74389829625,76.8212140598187,76.8984895025971,76.9757503850166,
77.053005690661,77.1302694609553,77.2075557394397,77.2849225522317,77.3623308869388,
77.4398524435017,77.50996137918,77.5874914972433,77.6649345265592,77.7423061083848,
77.8196218327448,77.8968972493061,77.9741581253316,78.0514134366779,78.1286772247696,
78.2059635331534,78.2833303947596,78.3607387886916,78.4382604215636,78.5083693872309,
78.5398163397458),.UNSPECIFIED.);
#154=B_SPLINE_CURVE_WITH_KNOTS('',3,(#14464,#14465,#14466,#14467,#14468,
#14469,#14470,#14471,#14472,#14473,#14474,#14475,#14476,#14477,#14478,#14479,
#14480,#14481,#14482,#14483,#14484,#14485,#14486,#14487,#14488,#14489,#14490,
#14491,#14492,#14493,#14494,#14495,#14496,#14497,#14498,#14499,#14500,#14501,
#14502,#14503,#14504,#14505,#14506,#14507,#14508,#14509,#14510,#14511,#14512,
#14513,#14514,#14515,#14516,#14517,#14518,#14519,#14520,#14521,#14522,#14523,
#14524,#14525,#14526,#14527,#14528,#14529,#14530,#14531,#14532,#14533,#14534,
#14535,#14536,#14537,#14538,#14539,#14540,#14541,#14542,#14543,#14544,#14545,
#14546,#14547,#14548,#14549,#14550,#14551,#14552,#14553,#14554,#14555,#14556,
#14557,#14558,#14559,#14560,#14561,#14562,#14563,#14564,#14565,#14566,#14567,
#14568,#14569,#14570,#14571,#14572,#14573,#14574,#14575,#14576,#14577,#14578,
#14579,#14580,#14581,#14582,#14583,#14584,#14585,#14586,#14587,#14588,#14589,
#14590,#14591,#14592,#14593,#14594,#14595,#14596,#14597,#14598,#14599,#14600,
#14601,#14602,#14603,#14604,#14605,#14606,#14607,#14608,#14609,#14610,#14611,
#14612,#14613,#14614,#14615,#14616,#14617,#14618,#14619,#14620,#14621,#14622,
#14623,#14624,#14625,#14626,#14627,#14628,#14629,#14630,#14631,#14632,#14633,
#14634,#14635),.UNSPECIFIED.,.F.,.F.,(4,3,3,3,3,3,3,3,3,3,3,3,3,3,3,3,3,
3,3,3,3,3,3,3,3,3,3,3,3,3,3,3,3,3,3,3,3,3,3,3,3,3,3,3,3,3,3,3,3,3,3,3,3,
3,3,3,3,4),(78.5398163398252,78.6162568128587,78.6926100374869,78.7688925258994,
78.8451207276279,78.9213110445758,78.9974920317676,79.0736713944741,79.1498639412457,
79.2260844876471,79.302392510473,79.3787481973464,79.4552194143481,79.5067773952818,
79.5843720647159,79.6618743308263,79.7392998158967,79.8166640872737,79.8939826683645,
79.9712783728361,80.048563417492,80.125851809425,80.2031575549505,80.2805355949379,
80.3579506666826,80.4354712809538,80.5051854033328,80.5866717177657,80.6680538001247,
80.7521377019331,80.833295020786,80.9143758045396,80.9953657965727,81.0043894073582,
81.0854025136485,81.1664912079208,81.2507667587865,81.3320762251763,81.4134631263875,
81.4949702651519,81.5035934113837,81.5811215645928,81.6585684395543,81.7359496182619,
81.8132806357227,81.8905769905536,81.9678672908898,82.045157198628,82.1224607206263,
82.1997918687533,82.2772113585743,82.3546767169963,82.4322621032943,82.5020014194346,
82.578859309981,82.6556351312199,82.7323238361827,82.7772962578755),
 .UNSPECIFIED.);
#155=B_SPLINE_CURVE_WITH_KNOTS('',3,(#14641,#14642,#14643,#14644,#14645,
#14646,#14647,#14648,#14649,#14650,#14651,#14652,#14653,#14654,#14655,#14656,
#14657,#14658,#14659,#14660,#14661,#14662,#14663,#14664,#14665,#14666,#14667,
#14668,#14669,#14670,#14671,#14672,#14673,#14674,#14675,#14676,#14677,#14678,
#14679,#14680,#14681,#14682,#14683,#14684,#14685,#14686,#14687,#14688,#14689,
#14690,#14691,#14692,#14693,#14694,#14695,#14696,#14697,#14698,#14699,#14700,
#14701,#14702,#14703,#14704,#14705,#14706,#14707,#14708,#14709,#14710,#14711,
#14712,#14713,#14714,#14715,#14716,#14717,#14718,#14719,#14720,#14721,#14722,
#14723,#14724,#14725,#14726,#14727,#14728,#14729,#14730,#14731,#14732,#14733,
#14734,#14735,#14736,#14737,#14738,#14739,#14740,#14741,#14742,#14743,#14744,
#14745,#14746,#14747,#14748,#14749,#14750,#14751,#14752,#14753,#14754,#14755,
#14756,#14757,#14758,#14759,#14760,#14761,#14762,#14763,#14764,#14765,#14766,
#14767,#14768,#14769,#14770,#14771,#14772,#14773,#14774,#14775,#14776,#14777,
#14778,#14779,#14780,#14781,#14782,#14783,#14784,#14785,#14786,#14787,#14788,
#14789,#14790,#14791,#14792,#14793,#14794,#14795,#14796,#14797,#14798,#14799,
#14800,#14801,#14802,#14803,#14804,#14805,#14806),.UNSPECIFIED.,.F.,.F.,
(4,3,3,3,3,3,3,3,3,3,3,3,3,3,3,3,3,3,3,3,3,3,3,3,3,3,3,3,3,3,3,3,3,3,3,
3,3,3,3,3,3,3,3,3,3,3,3,3,3,3,3,3,3,3,3,4),(84.8230016469256,84.9051841266213,
84.9874806104735,85.0699595040246,85.1525329936525,85.2352616759044,85.2821573300685,
85.3596731083316,85.4371074087423,85.5144758271695,85.5917939123196,85.669077176364,
85.7463542606756,85.8236308411634,85.9009209365608,85.9782385705651,86.0556447768896,
86.133096786203,86.2106695945251,86.2819109414379,86.3587595646253,86.4355144110222,
86.5121917504266,86.5888077902016,86.6653786888265,86.7424144218241,86.8189568405298,
86.8955051770924,86.97207400854,87.0494716446069,87.1261627255596,87.2039136391834,
87.2816645528073,87.3591821044254,87.4366123238449,87.5139708667404,87.5912733373275,
87.6685352992777,87.7457825250603,87.8230240362676,87.9002738865004,87.9775461314133,
88.0548990893843,88.132293481693,88.2098018093615,88.2814181641766,88.3589477898889,
88.4363876561042,88.5142386608849,88.5915371477998,88.668798429308,88.7460365802883,
88.8243263588036,88.9015777359387,88.9803867151441,89.0591956943495),
 .UNSPECIFIED.);
#156=B_SPLINE_CURVE_WITH_KNOTS('',3,(#14807,#14808,#14809,#14810,#14811,
#14812,#14813,#14814,#14815,#14816,#14817,#14818,#14819,#14820,#14821,#14822,
#14823,#14824,#14825,#14826,#14827,#14828,#14829,#14830,#14831,#14832,#14833,
#14834,#14835,#14836,#14837,#14838,#14839,#14840,#14841,#14842,#14843,#14844,
#14845,#14846,#14847,#14848,#14849,#14850,#14851,#14852,#14853,#14854,#14855,
#14856,#14857,#14858,#14859,#14860,#14861,#14862,#14863,#14864,#14865,#14866,
#14867,#14868,#14869,#14870,#14871,#14872,#14873,#14874,#14875,#14876,#14877,
#14878,#14879,#14880,#14881,#14882),.UNSPECIFIED.,.F.,.F.,(4,3,3,3,3,3,
3,3,3,3,3,3,3,3,3,3,3,3,3,3,3,3,3,3,3,4),(82.7764795961097,82.8589411999635,
82.941402137934,83.0238624374197,83.1063221258167,83.1887812305187,83.271239778918,
83.3536977984043,83.4361553163657,83.5228332120257,83.6052999978614,83.6877651112052,
83.7702286617103,83.852690759008,83.9351515127094,84.0176110324066,84.1000694276743,
84.1825268080714,84.2649931943378,84.3474563963516,84.4299168526321,84.5123750015429,
84.5948406064222,84.6773004856367,84.7597645990006,84.8230016469256),
 .UNSPECIFIED.);
#157=B_SPLINE_CURVE_WITH_KNOTS('',3,(#14884,#14885,#14886,#14887,#14888,
#14889,#14890,#14891,#14892,#14893,#14894,#14895,#14896,#14897,#14898,#14899,
#14900,#14901,#14902,#14903,#14904,#14905,#14906,#14907,#14908,#14909,#14910,
#14911,#14912,#14913,#14914,#14915,#14916,#14917,#14918,#14919,#14920,#14921,
#14922,#14923,#14924,#14925,#14926,#14927,#14928,#14929,#14930,#14931,#14932,
#14933,#14934,#14935,#14936,#14937,#14938,#14939,#14940,#14941,#14942,#14943,
#14944,#14945,#14946,#14947,#14948,#14949,#14950,#14951,#14952,#14953,#14954,
#14955,#14956,#14957,#14958,#14959,#14960,#14961,#14962,#14963,#14964,#14965),
 .UNSPECIFIED.,.F.,.F.,(4,3,3,3,3,3,3,3,3,3,3,3,3,3,3,3,3,3,3,3,3,3,3,3,
3,3,3,4),(82.7772962578755,82.8538993615407,82.9304669669959,83.0070270870308,
83.0835871435194,83.1601617015671,83.2367653327514,83.3134533235216,83.3901896333783,
83.4670319898012,83.5004094274855,83.5779396239453,83.655382718551,83.732754352607,
83.8100701161757,83.8873455589542,83.9646064413739,84.0418617470183,84.1191255173126,
84.1964117957971,84.2737786085891,84.3511869432957,84.4287084998586,84.4988174355364,
84.5900064650122,84.6808065702415,84.770854205132,84.8230016468377),
 .UNSPECIFIED.);
#158=B_SPLINE_CURVE_WITH_KNOTS('',3,(#14966,#14967,#14968,#14969,#14970,
#14971,#14972,#14973,#14974,#14975,#14976,#14977,#14978,#14979,#14980,#14981,
#14982,#14983,#14984,#14985,#14986,#14987,#14988,#14989,#14990,#14991,#14992,
#14993,#14994,#14995,#14996,#14997,#14998,#14999,#15000,#15001,#15002,#15003,
#15004,#15005,#15006,#15007,#15008,#15009,#15010,#15011,#15012,#15013,#15014,
#15015,#15016,#15017,#15018,#15019,#15020,#15021,#15022,#15023,#15024,#15025,
#15026,#15027,#15028,#15029,#15030,#15031,#15032,#15033,#15034,#15035,#15036,
#15037,#15038,#15039,#15040,#15041,#15042,#15043,#15044,#15045,#15046,#15047,
#15048,#15049,#15050,#15051,#15052,#15053,#15054,#15055,#15056,#15057,#15058,
#15059,#15060,#15061,#15062,#15063,#15064,#15065,#15066,#15067,#15068,#15069,
#15070,#15071,#15072,#15073,#15074,#15075,#15076,#15077,#15078,#15079,#15080,
#15081,#15082,#15083,#15084,#15085,#15086,#15087,#15088,#15089,#15090,#15091,
#15092,#15093,#15094,#15095,#15096,#15097,#15098,#15099,#15100,#15101,#15102,
#15103,#15104,#15105,#15106,#15107,#15108,#15109,#15110,#15111,#15112,#15113,
#15114,#15115,#15116,#15117,#15118,#15119,#15120,#15121,#15122,#15123,#15124,
#15125,#15126,#15127,#15128,#15129,#15130,#15131,#15132,#15133,#15134,#15135,
#15136,#15137),.UNSPECIFIED.,.F.,.F.,(4,3,3,3,3,3,3,3,3,3,3,3,3,3,3,3,3,
3,3,3,3,3,3,3,3,3,3,3,3,3,3,3,3,3,3,3,3,3,3,3,3,3,3,3,3,3,3,3,3,3,3,3,3,
3,3,3,3,4),(84.8230016469254,84.900259979548,84.9775140309716,85.0547691519919,
85.1320393290555,85.2093385544003,85.2867251748822,85.3641589545451,85.4417070272323,
85.4972254435874,85.57406147571,85.6508084914372,85.7274827290005,85.8041003685221,
85.8806775451493,85.9575470334604,86.0341071359831,86.1106774331304,86.1872724941531,
86.2643627335244,86.3410899301058,86.4183616908721,86.4956334516383,86.5732281210723,
86.6507303871827,86.7281558722534,86.8055201436303,86.8828387247205,86.9601344291921,
87.0374194738481,87.1147078657812,87.1920136113069,87.2693916512942,87.3468067230389,
87.4243273373101,87.4940414596892,87.5755277741222,87.6569098564808,87.7409937582893,
87.8221510771424,87.9032318608979,87.9842218529317,87.9932454637146,88.074258570005,
88.1553472642779,88.2396228151435,88.3209322815331,88.4023191827436,88.4838263215085,
88.4924494677401,88.5699718073358,88.6474167446868,88.724798397842,88.8021308455058,
88.8794289255214,88.9567073170796,89.0339881810012,89.0594182937293),
 .UNSPECIFIED.);
#159=B_SPLINE_CURVE_WITH_KNOTS('',3,(#15143,#15144,#15145,#15146,#15147,
#15148,#15149,#15150,#15151,#15152,#15153,#15154,#15155,#15156,#15157,#15158,
#15159,#15160,#15161,#15162,#15163,#15164,#15165,#15166,#15167,#15168,#15169,
#15170,#15171,#15172,#15173,#15174,#15175,#15176,#15177,#15178,#15179,#15180,
#15181,#15182,#15183,#15184,#15185,#15186,#15187,#15188,#15189,#15190,#15191,
#15192,#15193,#15194,#15195,#15196,#15197,#15198,#15199,#15200,#15201,#15202,
#15203,#15204,#15205,#15206,#15207,#15208,#15209,#15210,#15211,#15212,#15213,
#15214,#15215,#15216,#15217,#15218,#15219,#15220,#15221,#15222,#15223,#15224,
#15225,#15226,#15227,#15228,#15229,#15230,#15231,#15232,#15233,#15234,#15235,
#15236,#15237,#15238,#15239,#15240,#15241,#15242,#15243,#15244,#15245,#15246,
#15247,#15248,#15249,#15250,#15251,#15252,#15253,#15254,#15255,#15256,#15257,
#15258,#15259,#15260,#15261,#15262,#15263,#15264,#15265,#15266,#15267,#15268,
#15269,#15270,#15271,#15272,#15273,#15274,#15275,#15276,#15277,#15278,#15279,
#15280,#15281,#15282,#15283,#15284,#15285,#15286,#15287,#15288,#15289,#15290,
#15291,#15292,#15293,#15294,#15295,#15296,#15297,#15298,#15299),
 .UNSPECIFIED.,.F.,.F.,(4,3,3,3,3,3,3,3,3,3,3,3,3,3,3,3,3,3,3,3,3,3,3,3,
3,3,3,3,3,3,3,3,3,3,3,3,3,3,3,3,3,3,3,3,3,3,3,3,3,3,3,3,4),(91.1061869541052,
91.1886491601415,91.2711110178812,91.3535725341748,91.4360337158723,91.5184945698235,
91.6009551028778,91.6834153218843,91.7658752336922,91.8483348451498,91.9307941631057,
92.0132531944081,92.0957119459048,92.1781704244433,92.2606286368711,92.3430865900354,
92.4255442907829,92.508001745961,92.5904589624156,92.6764711889173,92.7597955333408,
92.8422621387863,92.9247279000277,93.0071928444802,93.0896569995562,93.172120392665,
93.2545830512136,93.3370450026064,93.4195062742451,93.5019668935292,93.584426887856,
93.6668862846205,93.7493451112156,93.8318033950323,93.9142611634597,93.996718443885,
94.0808516792965,94.1633176773882,94.2457820537436,94.3282449180059,94.4107063797965,
94.4931665487176,94.5756255343531,94.6580834462704,94.7436792917952,94.8261440283953,
94.9086058003973,94.9910650462394,95.0735222042164,95.1559847224976,95.2384423933526,
95.3209011833033,95.3428502104689),.UNSPECIFIED.);
#160=B_SPLINE_CURVE_WITH_KNOTS('',3,(#15300,#15301,#15302,#15303,#15304,
#15305,#15306,#15307,#15308,#15309,#15310,#15311,#15312,#15313,#15314,#15315,
#15316,#15317,#15318,#15319,#15320,#15321,#15322,#15323,#15324,#15325,#15326,
#15327,#15328,#15329,#15330,#15331,#15332,#15333,#15334,#15335,#15336,#15337,
#15338,#15339,#15340,#15341,#15342,#15343,#15344,#15345,#15346,#15347,#15348,
#15349,#15350,#15351,#15352,#15353,#15354,#15355,#15356,#15357,#15358,#15359,
#15360,#15361,#15362,#15363,#15364,#15365,#15366,#15367,#15368,#15369,#15370,
#15371,#15372,#15373,#15374,#15375,#15376,#15377,#15378,#15379,#15380,#15381),
 .UNSPECIFIED.,.F.,.F.,(4,3,3,3,3,3,3,3,3,3,3,3,3,3,3,3,3,3,3,3,3,3,3,3,
3,3,3,4),(89.0591956943495,89.1365930519662,89.2141031437056,89.281171775546,
89.3579929727008,89.4347249349151,89.5113839130629,89.5879860995243,89.6645476414052,
89.741594859594,89.8181390342383,89.8946933142836,89.9712722792633,90.0486855561763,
90.1253970364832,90.2031612116993,90.2809253869154,90.3576414403888,90.4342648893733,
90.5108121340303,90.5872920412522,90.663734501548,90.7401542288347,90.8165659204488,
90.8930108655814,90.9694722519528,91.0460033091413,91.105416707111),
 .UNSPECIFIED.);
#161=B_SPLINE_CURVE_WITH_KNOTS('',3,(#15383,#15384,#15385,#15386,#15387,
#15388,#15389,#15390,#15391,#15392,#15393,#15394,#15395,#15396,#15397,#15398,
#15399,#15400,#15401,#15402,#15403,#15404,#15405,#15406,#15407,#15408,#15409,
#15410,#15411,#15412,#15413,#15414,#15415,#15416,#15417,#15418,#15419,#15420,
#15421,#15422,#15423,#15424,#15425,#15426,#15427,#15428,#15429,#15430,#15431,
#15432,#15433,#15434,#15435,#15436,#15437,#15438,#15439,#15440,#15441,#15442,
#15443,#15444,#15445,#15446,#15447,#15448,#15449,#15450,#15451,#15452,#15453,
#15454,#15455,#15456,#15457,#15458,#15459,#15460,#15461,#15462,#15463,#15464),
 .UNSPECIFIED.,.F.,.F.,(4,3,3,3,3,3,3,3,3,3,3,3,3,3,3,3,3,3,3,3,3,3,3,3,
3,3,3,4),(89.0594182937293,89.1367293492698,89.2140726386133,89.2915058024444,
89.3689889815936,89.4465849562361,89.490857475791,89.5677208604433,89.6444906922528,
89.7211832282412,89.7978146634082,89.8744011441913,89.9512591866476,90.027817509611,
90.1043818442834,90.1809667574108,90.2580414390186,90.3347482598874,90.4120068718647,
90.4892654838419,90.5677895481334,90.6462209244004,90.7245725981383,90.8028575049273,
90.8810803650547,90.9592661290473,91.0374327518346,91.106186954105),
 .UNSPECIFIED.);
#162=B_SPLINE_CURVE_WITH_KNOTS('',3,(#15465,#15466,#15467,#15468,#15469,
#15470,#15471,#15472,#15473,#15474,#15475,#15476,#15477,#15478,#15479,#15480,
#15481,#15482,#15483,#15484,#15485,#15486,#15487,#15488,#15489,#15490,#15491,
#15492,#15493,#15494,#15495,#15496,#15497,#15498,#15499,#15500,#15501,#15502,
#15503,#15504,#15505,#15506,#15507,#15508,#15509,#15510,#15511,#15512,#15513,
#15514,#15515,#15516,#15517,#15518,#15519,#15520,#15521,#15522,#15523,#15524,
#15525,#15526,#15527,#15528,#15529,#15530,#15531,#15532,#15533,#15534,#15535,
#15536,#15537,#15538,#15539,#15540,#15541,#15542,#15543,#15544,#15545,#15546,
#15547,#15548,#15549,#15550,#15551,#15552,#15553,#15554,#15555,#15556,#15557,
#15558,#15559,#15560,#15561,#15562,#15563,#15564,#15565,#15566,#15567,#15568,
#15569,#15570,#15571,#15572,#15573,#15574,#15575,#15576,#15577,#15578,#15579,
#15580,#15581,#15582,#15583,#15584,#15585,#15586,#15587,#15588,#15589,#15590,
#15591,#15592,#15593,#15594,#15595,#15596,#15597,#15598,#15599,#15600,#15601,
#15602,#15603,#15604,#15605,#15606,#15607,#15608,#15609,#15610,#15611,#15612,
#15613,#15614,#15615,#15616,#15617,#15618,#15619,#15620,#15621,#15622,#15623,
#15624,#15625,#15626,#15627,#15628,#15629,#15630,#15631,#15632,#15633),
 .UNSPECIFIED.,.F.,.F.,(4,3,3,3,3,3,3,3,3,3,3,3,3,3,3,3,3,3,3,3,3,3,3,3,
3,3,3,3,3,3,3,3,3,3,3,3,3,3,3,3,3,3,3,3,3,3,3,3,3,3,3,3,3,3,3,3,4),(91.106186954195,
91.1920170383312,91.2783242322604,91.3648739223735,91.4517397796147,91.4876734918928,
91.5652036099561,91.642646639272,91.7200182210975,91.7973339454571,91.8746093620186,
91.951870238044,92.0291255493902,92.1063893374818,92.1836756458659,92.2610425074721,
92.3384509014041,92.4159725342761,92.4860814999438,92.5629175320664,92.6396645477935,
92.7163387853568,92.7929564248784,92.8695336015055,92.9464030898166,93.0229631923393,
93.0995334894866,93.1761285505091,93.2532187898805,93.329945986462,93.4072177472283,
93.4844895079947,93.5620841774288,93.6395864435391,93.7170119286096,93.7943761999865,
93.8716947810774,93.9489904855489,94.0262755302049,94.1035639221379,94.1808696676636,
94.258247707651,94.3356627793956,94.4131833936668,94.4828975160456,94.5643838304785,
94.6457659128375,94.7298498146459,94.8110071334989,94.8920879172536,94.9730779092874,
94.9821015200711,95.0630915629816,95.1442058159851,95.2253866236002,95.3066844308499,
95.3424746944017),.UNSPECIFIED.);
#163=B_SPLINE_CURVE_WITH_KNOTS('',3,(#15639,#15640,#15641,#15642,#15643,
#15644,#15645,#15646,#15647,#15648,#15649,#15650,#15651,#15652,#15653,#15654,
#15655,#15656,#15657,#15658,#15659,#15660,#15661,#15662,#15663,#15664,#15665,
#15666,#15667,#15668,#15669,#15670,#15671,#15672,#15673,#15674,#15675,#15676,
#15677,#15678,#15679,#15680,#15681,#15682,#15683,#15684,#15685,#15686,#15687,
#15688,#15689,#15690,#15691,#15692,#15693,#15694,#15695,#15696,#15697,#15698,
#15699,#15700,#15701,#15702,#15703,#15704,#15705,#15706,#15707,#15708,#15709,
#15710,#15711,#15712,#15713,#15714,#15715,#15716,#15717,#15718,#15719,#15720,
#15721,#15722,#15723,#15724,#15725,#15726,#15727,#15728,#15729,#15730,#15731,
#15732,#15733,#15734,#15735,#15736,#15737,#15738,#15739,#15740,#15741,#15742,
#15743,#15744,#15745,#15746,#15747,#15748,#15749,#15750,#15751,#15752,#15753,
#15754,#15755,#15756,#15757,#15758,#15759,#15760,#15761,#15762,#15763,#15764,
#15765,#15766,#15767,#15768,#15769,#15770,#15771,#15772,#15773,#15774,#15775,
#15776,#15777,#15778,#15779,#15780,#15781,#15782,#15783,#15784,#15785,#15786,
#15787,#15788,#15789,#15790,#15791,#15792,#15793,#15794,#15795,#15796,#15797,
#15798,#15799,#15800,#15801,#15802,#15803,#15804,#15805,#15806,#15807,#15808,
#15809,#15810),.UNSPECIFIED.,.F.,.F.,(4,3,3,3,3,3,3,3,3,3,3,3,3,3,3,3,3,
3,3,3,3,3,3,3,3,3,3,3,3,3,3,3,3,3,3,3,3,3,3,3,3,3,3,3,3,3,3,3,3,3,3,3,3,
3,3,3,3,4),(97.3898726090998,97.4662065462312,97.5424567142456,97.6186396946541,
97.6947720072897,97.7708759140936,97.846966464458,97.9230585390012,97.9991670176848,
98.0753453720321,98.1515615244939,98.227877771978,98.2789542778703,98.3604382508255,
98.4418176149653,98.5260709821127,98.6072244772844,98.6883011552429,98.7692865830328,
98.778831083555,98.8598394794593,98.9409237362904,99.0253697745277,99.1066758562345,
99.1880596460033,99.2695643070317,99.2787078892397,99.3562236675028,99.4336579679133,
99.5110263863403,99.5883444714906,99.6656277355348,99.7429048198463,99.8201814003342,
99.8974714957315,99.9747891297362,100.052195336061,100.129647345374,100.207220153696,
100.278461500609,100.355310123796,100.432064970194,100.508742309598,100.585358349373,
100.661929247998,100.738964980996,100.815507399701,100.892055736264,100.968624567712,
101.046022203778,101.122713284731,101.200464198355,101.278215111978,101.355749929111,
101.433174288491,101.510534996438,101.587835153039,101.626359673358),
 .UNSPECIFIED.);
#164=B_SPLINE_CURVE_WITH_KNOTS('',3,(#15811,#15812,#15813,#15814,#15815,
#15816,#15817,#15818,#15819,#15820,#15821,#15822,#15823,#15824,#15825,#15826,
#15827,#15828,#15829,#15830,#15831,#15832,#15833,#15834,#15835,#15836,#15837,
#15838,#15839,#15840,#15841,#15842,#15843,#15844,#15845,#15846,#15847,#15848,
#15849,#15850,#15851,#15852,#15853,#15854,#15855,#15856,#15857,#15858,#15859,
#15860,#15861,#15862,#15863,#15864,#15865,#15866,#15867,#15868,#15869,#15870,
#15871,#15872,#15873,#15874,#15875,#15876,#15877,#15878,#15879,#15880,#15881,
#15882,#15883,#15884,#15885,#15886),.UNSPECIFIED.,.F.,.F.,(4,3,3,3,3,3,
3,3,3,3,3,3,3,3,3,3,3,3,3,3,3,3,3,3,3,4),(95.3428502104689,95.4253118143227,
95.5077727522932,95.5902330517789,95.6726927401757,95.7551518448778,95.837610393277,
95.9200684127633,96.0025259307248,96.0892038263848,96.1716706122204,96.2541357255642,
96.3365992760693,96.4190613733671,96.5015221270684,96.5839816467656,96.6664400420332,
96.7488974224304,96.8313638086968,96.9138270107106,96.9962874669912,97.0787456159018,
97.161211220781,97.2436710999955,97.3261352133594,97.3893722612848),
 .UNSPECIFIED.);
#165=B_SPLINE_CURVE_WITH_KNOTS('',3,(#15888,#15889,#15890,#15891,#15892,
#15893,#15894,#15895,#15896,#15897,#15898,#15899,#15900,#15901,#15902,#15903,
#15904,#15905,#15906,#15907,#15908,#15909,#15910,#15911,#15912,#15913,#15914,
#15915,#15916,#15917,#15918,#15919,#15920,#15921,#15922,#15923,#15924,#15925,
#15926,#15927,#15928,#15929,#15930,#15931,#15932,#15933,#15934,#15935,#15936,
#15937,#15938,#15939,#15940,#15941,#15942,#15943,#15944,#15945,#15946,#15947,
#15948,#15949,#15950,#15951,#15952,#15953,#15954,#15955,#15956,#15957,#15958,
#15959,#15960,#15961,#15962,#15963,#15964,#15965,#15966,#15967,#15968,#15969),
 .UNSPECIFIED.,.F.,.F.,(4,3,3,3,3,3,3,3,3,3,3,3,3,3,3,3,3,3,3,3,3,3,3,3,
3,3,3,4),(95.3424746944017,95.423953095677,95.4813055240965,95.5588336773056,
95.636280552267,95.7136617309745,95.7909927484351,95.8682891032655,95.9455794036017,
96.02286931134,96.1001728333381,96.1775039814651,96.2549234712861,96.3323888297079,
96.409974216006,96.4797135321474,96.5556971028836,96.6315883519272,96.7074041199809,
96.7831611674713,96.8588792362736,96.934577022471,97.0102695900154,97.0859719978792,
97.1617397381996,97.2375397227215,97.3134445270289,97.3887660913681),
 .UNSPECIFIED.);
#166=B_SPLINE_CURVE_WITH_KNOTS('',3,(#15970,#15971,#15972,#15973,#15974,
#15975,#15976,#15977,#15978,#15979,#15980,#15981,#15982,#15983,#15984,#15985,
#15986,#15987,#15988,#15989,#15990,#15991,#15992,#15993,#15994,#15995,#15996,
#15997,#15998,#15999,#16000,#16001,#16002,#16003,#16004,#16005,#16006,#16007,
#16008,#16009,#16010,#16011,#16012,#16013,#16014,#16015,#16016,#16017,#16018,
#16019,#16020,#16021,#16022,#16023,#16024,#16025,#16026,#16027,#16028,#16029,
#16030,#16031,#16032,#16033,#16034,#16035,#16036,#16037,#16038,#16039,#16040,
#16041,#16042,#16043,#16044,#16045,#16046,#16047,#16048,#16049,#16050,#16051,
#16052,#16053,#16054,#16055,#16056,#16057,#16058,#16059,#16060,#16061,#16062,
#16063,#16064,#16065,#16066,#16067,#16068,#16069,#16070,#16071,#16072,#16073,
#16074,#16075,#16076,#16077,#16078,#16079,#16080,#16081,#16082,#16083,#16084,
#16085,#16086,#16087,#16088,#16089,#16090,#16091,#16092,#16093,#16094,#16095,
#16096,#16097,#16098,#16099,#16100,#16101,#16102,#16103,#16104,#16105,#16106,
#16107,#16108,#16109,#16110,#16111,#16112,#16113,#16114,#16115,#16116,#16117,
#16118,#16119,#16120,#16121,#16122,#16123,#16124,#16125,#16126),
 .UNSPECIFIED.,.F.,.F.,(4,3,3,3,3,3,3,3,3,3,3,3,3,3,3,3,3,3,3,3,3,3,3,3,
3,3,3,3,3,3,3,3,3,3,3,3,3,3,3,3,3,3,3,3,3,3,3,3,3,3,3,3,4),(97.3893956674183,
97.4718578733547,97.5543197309966,97.6367812471942,97.7192424287977,97.8017032826569,
97.8841638156211,97.9666240345395,98.0490839462611,98.1315435576345,98.2140028755081,
98.29646190673,98.3789206581482,98.46137913661,98.5438373489633,98.6262953020549,
98.7087530027319,98.791210457841,98.8736676742287,98.9596791693356,99.0430028052203,
99.1254694104373,99.2079351714575,99.2904001156961,99.3728642705655,99.455327663475,
99.5377903218316,99.6202522730397,99.702713544501,99.785174163615,99.867634157779,
99.950093554388,100.032552380835,100.115010664511,100.197468432805,100.279925713104,
100.364057575888,100.446523573561,100.528987949525,100.611450813423,100.693912274877,
100.776372443489,100.858831428843,100.941289340506,101.026882612649,101.109347348554,
101.191809119956,101.274268365294,101.356725522863,101.439188039894,101.521645709882,
101.604104497894,101.626035517648),.UNSPECIFIED.);
#167=B_SPLINE_CURVE_WITH_KNOTS('',3,(#16132,#16133,#16134,#16135,#16136,
#16137,#16138,#16139,#16140,#16141,#16142,#16143,#16144,#16145,#16146,#16147,
#16148,#16149,#16150,#16151,#16152,#16153,#16154,#16155,#16156,#16157,#16158,
#16159,#16160,#16161,#16162,#16163,#16164,#16165,#16166,#16167,#16168,#16169,
#16170,#16171,#16172,#16173,#16174,#16175,#16176,#16177,#16178,#16179,#16180,
#16181,#16182,#16183,#16184,#16185,#16186,#16187,#16188,#16189,#16190,#16191,
#16192,#16193,#16194,#16195,#16196,#16197,#16198,#16199,#16200,#16201,#16202,
#16203,#16204,#16205,#16206,#16207,#16208,#16209,#16210,#16211,#16212,#16213,
#16214,#16215,#16216,#16217,#16218,#16219,#16220,#16221,#16222,#16223,#16224,
#16225,#16226,#16227,#16228,#16229,#16230,#16231,#16232,#16233,#16234,#16235,
#16236,#16237,#16238,#16239,#16240,#16241,#16242,#16243,#16244,#16245,#16246,
#16247,#16248,#16249,#16250,#16251,#16252,#16253,#16254,#16255,#16256,#16257,
#16258,#16259,#16260,#16261,#16262,#16263,#16264,#16265,#16266,#16267,#16268,
#16269,#16270,#16271,#16272,#16273,#16274,#16275,#16276,#16277,#16278,#16279,
#16280,#16281,#16282,#16283,#16284,#16285,#16286,#16287,#16288),
 .UNSPECIFIED.,.F.,.F.,(4,3,3,3,3,3,3,3,3,3,3,3,3,3,3,3,3,3,3,3,3,3,3,3,
3,3,3,3,3,3,3,3,3,3,3,3,3,3,3,3,3,3,3,3,3,3,3,3,3,3,3,3,4),(103.672557568464,
103.7550197745,103.83748163224,103.919943148534,104.002404330231,104.084865184182,
104.167325717237,104.249785936243,104.332245848051,104.414705459509,104.497164777465,
104.579623808767,104.662082560264,104.744541038802,104.82699925123,104.909457204394,
104.991914905142,105.07437236032,105.156829576775,105.242841803276,105.3261661477,
105.408632753145,105.491098514387,105.573563458839,105.656027613915,105.738491007024,
105.820953665572,105.903415616965,105.985876888604,106.068337507888,106.150797502215,
106.233256898979,106.315715725575,106.398174009391,106.480631777819,106.563089058244,
106.647222293656,106.729688291747,106.812152668103,106.894615532365,106.977076994156,
107.059537163077,107.141996148712,107.224454060629,107.310049906154,107.392514642754,
107.474976414756,107.557435660598,107.639892818576,107.722355336857,107.804813007712,
107.887271797662,107.909220824828),.UNSPECIFIED.);
#168=B_SPLINE_CURVE_WITH_KNOTS('',3,(#16289,#16290,#16291,#16292,#16293,
#16294,#16295,#16296,#16297,#16298,#16299,#16300,#16301,#16302,#16303,#16304,
#16305,#16306,#16307,#16308,#16309,#16310,#16311,#16312,#16313,#16314,#16315,
#16316,#16317,#16318,#16319,#16320,#16321,#16322,#16323,#16324,#16325,#16326,
#16327,#16328,#16329,#16330,#16331,#16332,#16333,#16334,#16335,#16336,#16337,
#16338,#16339,#16340,#16341,#16342,#16343,#16344,#16345,#16346,#16347,#16348,
#16349,#16350,#16351,#16352,#16353,#16354,#16355,#16356,#16357,#16358,#16359,
#16360,#16361,#16362,#16363,#16364,#16365,#16366,#16367,#16368,#16369,#16370),
 .UNSPECIFIED.,.F.,.F.,(4,3,3,3,3,3,3,3,3,3,3,3,3,3,3,3,3,3,3,3,3,3,3,3,
3,3,3,4),(101.626359673358,101.703607239662,101.780849858977,101.858093771854,
101.935353031952,102.012641698857,102.090013724377,102.167433491956,102.244956987448,
102.277968723348,102.355486092544,102.432916159996,102.510274581265,102.58757696048,
102.664838861243,102.742086071934,102.819327596153,102.896577487499,102.973849801642,
103.051202872868,103.12859740262,103.206105907582,103.277722334717,103.363331372225,
103.448584455864,103.533612860426,103.618273980915,103.672557568464),
 .UNSPECIFIED.);
#169=B_SPLINE_CURVE_WITH_KNOTS('',3,(#16372,#16373,#16374,#16375,#16376,
#16377,#16378,#16379,#16380,#16381,#16382,#16383,#16384,#16385,#16386,#16387,
#16388,#16389,#16390,#16391,#16392,#16393,#16394,#16395,#16396,#16397,#16398,
#16399,#16400,#16401,#16402,#16403,#16404,#16405,#16406,#16407,#16408,#16409,
#16410,#16411,#16412,#16413,#16414,#16415,#16416,#16417,#16418,#16419,#16420,
#16421,#16422,#16423,#16424,#16425,#16426,#16427,#16428,#16429,#16430,#16431,
#16432,#16433,#16434,#16435,#16436,#16437,#16438,#16439,#16440,#16441,#16442,
#16443,#16444,#16445,#16446,#16447),.UNSPECIFIED.,.F.,.F.,(4,3,3,3,3,3,
3,3,3,3,3,3,3,3,3,3,3,3,3,3,3,3,3,3,3,4),(101.626035517648,101.708497121502,
101.790958059472,101.873418358958,101.955878047355,102.038337152057,102.120795700456,
102.203253719943,102.285711237904,102.372389133564,102.4548559194,102.537321032744,
102.619784583249,102.702246680546,102.784707434248,102.867166953945,102.949625349213,
103.03208272961,103.114549115876,103.19701231789,103.279472774171,103.361930923081,
103.444396527961,103.526856407175,103.609320520539,103.672557568464),
 .UNSPECIFIED.);
#170=B_SPLINE_CURVE_WITH_KNOTS('',3,(#16448,#16449,#16450,#16451,#16452,
#16453,#16454,#16455,#16456,#16457,#16458,#16459,#16460,#16461,#16462,#16463,
#16464,#16465,#16466,#16467,#16468,#16469,#16470,#16471,#16472,#16473,#16474,
#16475,#16476,#16477,#16478,#16479,#16480,#16481,#16482,#16483,#16484,#16485,
#16486,#16487,#16488,#16489,#16490,#16491,#16492,#16493,#16494,#16495,#16496,
#16497,#16498,#16499,#16500,#16501,#16502,#16503,#16504,#16505,#16506,#16507,
#16508,#16509,#16510,#16511,#16512,#16513,#16514,#16515,#16516,#16517,#16518,
#16519,#16520,#16521,#16522,#16523,#16524,#16525,#16526,#16527,#16528,#16529,
#16530,#16531,#16532,#16533,#16534,#16535,#16536,#16537,#16538,#16539,#16540,
#16541,#16542,#16543,#16544,#16545,#16546,#16547,#16548,#16549,#16550,#16551,
#16552,#16553,#16554,#16555,#16556,#16557,#16558,#16559,#16560,#16561,#16562,
#16563,#16564,#16565,#16566,#16567,#16568,#16569,#16570,#16571,#16572,#16573,
#16574,#16575,#16576,#16577,#16578,#16579,#16580,#16581,#16582,#16583,#16584,
#16585,#16586,#16587,#16588,#16589,#16590,#16591,#16592,#16593,#16594,#16595,
#16596,#16597,#16598,#16599,#16600,#16601,#16602,#16603,#16604,#16605,#16606,
#16607,#16608,#16609,#16610,#16611,#16612,#16613,#16614,#16615,#16616),
 .UNSPECIFIED.,.F.,.F.,(4,3,3,3,3,3,3,3,3,3,3,3,3,3,3,3,3,3,3,3,3,3,3,3,
3,3,3,3,3,3,3,3,3,3,3,3,3,3,3,3,3,3,3,3,3,3,3,3,3,3,3,3,3,3,3,3,4),(103.673734240473,
103.74932672623,103.824858365227,103.900345978336,103.975815541418,104.051278467764,
104.126749916025,104.202245051749,104.277819299239,104.353438159594,104.429161669901,
104.466977596555,104.544507793015,104.62195088762,104.699322521676,104.776638285245,
104.853913728023,104.931174610443,105.008429916087,105.085693686381,105.162979964866,
105.240346777658,105.317755112365,105.395276668928,105.465385604606,105.542915722669,
105.620358751985,105.697730333811,105.77504605817,105.852321474732,105.929582350757,
106.006837662104,106.084101450195,106.161387758579,106.238754620185,106.316163014118,
106.39368464699,106.463793612657,106.54062964478,106.617376660507,106.69405089807,
106.770668537592,106.847245714218,106.92411520253,107.000675305052,107.0772456022,
107.153840663222,107.230930902593,107.307658099175,107.384929859941,107.462201620708,
107.539802243061,107.617313191671,107.694730000345,107.772092372968,107.849409710893,
107.909426078052),.UNSPECIFIED.);
#171=B_SPLINE_CURVE_WITH_KNOTS('',3,(#16622,#16623,#16624,#16625,#16626,
#16627,#16628,#16629,#16630,#16631,#16632,#16633,#16634,#16635,#16636,#16637,
#16638,#16639,#16640,#16641,#16642,#16643,#16644,#16645,#16646,#16647,#16648,
#16649,#16650,#16651,#16652,#16653,#16654,#16655,#16656,#16657,#16658,#16659,
#16660,#16661,#16662,#16663,#16664,#16665,#16666,#16667,#16668,#16669,#16670,
#16671,#16672,#16673,#16674,#16675,#16676,#16677,#16678,#16679,#16680,#16681,
#16682,#16683,#16684,#16685,#16686,#16687,#16688,#16689,#16690,#16691,#16692,
#16693,#16694,#16695,#16696,#16697,#16698,#16699,#16700,#16701,#16702,#16703,
#16704,#16705,#16706,#16707,#16708,#16709,#16710,#16711,#16712,#16713,#16714,
#16715,#16716,#16717,#16718,#16719,#16720,#16721,#16722,#16723,#16724,#16725,
#16726,#16727,#16728,#16729,#16730,#16731,#16732,#16733,#16734,#16735,#16736,
#16737,#16738,#16739,#16740,#16741,#16742,#16743,#16744,#16745,#16746,#16747,
#16748,#16749,#16750,#16751,#16752,#16753,#16754,#16755,#16756,#16757,#16758,
#16759,#16760,#16761,#16762,#16763,#16764,#16765,#16766,#16767,#16768,#16769,
#16770,#16771,#16772,#16773,#16774,#16775,#16776,#16777,#16778,#16779,#16780,
#16781,#16782,#16783,#16784,#16785,#16786,#16787,#16788,#16789,#16790),
 .UNSPECIFIED.,.F.,.F.,(4,3,3,3,3,3,3,3,3,3,3,3,3,3,3,3,3,3,3,3,3,3,3,3,
3,3,3,3,3,3,3,3,3,3,3,3,3,3,3,3,3,3,3,3,3,3,3,3,3,3,3,3,3,3,3,3,4),(109.955742875644,
110.04775906347,110.140427565771,110.233832795629,110.275997614303,110.352818811458,
110.429550773672,110.50620975182,110.582811938281,110.659373480162,110.736420698351,
110.812964872995,110.88951915304,110.96609811802,111.043511394933,111.12022287524,
111.197987050456,111.275751225672,111.353333849286,111.430823831495,111.50823680872,
111.585588362221,111.662894029132,111.740176622177,111.817448409121,111.894723408977,
111.972015639915,112.04938031228,112.126781920713,112.204289735321,112.275504837041,
112.356988809996,112.438368174136,112.522621541284,112.603775036455,112.684851714414,
112.765837142205,112.775381642726,112.85639003863,112.937474295461,113.021920333699,
113.103226415406,113.184610205174,113.266114866203,113.275258448411,113.352778156027,
113.430215472643,113.507585997295,113.584905281123,113.662193120441,113.739465144431,
113.816735373775,113.894017825487,113.971363883941,114.048742610616,114.126217904742,
114.192169701311),.UNSPECIFIED.);
#172=B_SPLINE_CURVE_WITH_KNOTS('',3,(#16791,#16792,#16793,#16794,#16795,
#16796,#16797,#16798,#16799,#16800,#16801,#16802,#16803,#16804,#16805,#16806,
#16807,#16808,#16809,#16810,#16811,#16812,#16813,#16814,#16815,#16816,#16817,
#16818,#16819,#16820,#16821,#16822,#16823,#16824,#16825,#16826,#16827,#16828,
#16829,#16830,#16831,#16832,#16833,#16834,#16835,#16836,#16837,#16838,#16839,
#16840,#16841,#16842,#16843,#16844,#16845,#16846,#16847,#16848,#16849,#16850,
#16851,#16852,#16853,#16854,#16855,#16856,#16857,#16858,#16859,#16860,#16861,
#16862,#16863,#16864,#16865,#16866),.UNSPECIFIED.,.F.,.F.,(4,3,3,3,3,3,
3,3,3,3,3,3,3,3,3,3,3,3,3,3,3,3,3,3,3,4),(107.909220824828,107.991682428682,
108.074143366652,108.156603666138,108.239063354535,108.321522459237,108.403981007636,
108.486439027122,108.568896545084,108.655574440744,108.73804122658,108.820506339923,
108.902969890429,108.985431987726,109.067892741428,109.150352261125,109.232810656392,
109.315268036789,109.397734423056,109.48019762507,109.56265808135,109.645116230261,
109.72758183514,109.810041714355,109.892505827719,109.955742875644),
 .UNSPECIFIED.);
#173=B_SPLINE_CURVE_WITH_KNOTS('',3,(#16868,#16869,#16870,#16871,#16872,
#16873,#16874,#16875,#16876,#16877,#16878,#16879,#16880,#16881,#16882,#16883,
#16884,#16885,#16886,#16887,#16888,#16889,#16890,#16891,#16892,#16893,#16894,
#16895,#16896,#16897,#16898,#16899,#16900,#16901,#16902,#16903,#16904,#16905,
#16906,#16907,#16908,#16909,#16910,#16911,#16912,#16913,#16914,#16915,#16916,
#16917,#16918,#16919,#16920,#16921,#16922,#16923,#16924,#16925,#16926,#16927,
#16928,#16929,#16930,#16931,#16932,#16933,#16934,#16935,#16936,#16937,#16938,
#16939,#16940,#16941,#16942,#16943,#16944,#16945,#16946,#16947,#16948,#16949,
#16950,#16951,#16952),.UNSPECIFIED.,.F.,.F.,(4,3,3,3,3,3,3,3,3,3,3,3,3,
3,3,3,3,3,3,3,3,3,3,3,3,3,3,3,4),(107.909426078052,107.986712289755,108.063998718063,
108.141299368798,108.221126933788,108.298533931578,108.379571780168,108.460609628758,
108.542095943191,108.623478025549,108.707561927358,108.788719246211,108.869800029965,
108.950790021998,108.959813632784,109.040826739075,109.121915433348,109.206190984213,
109.287500450603,109.368887351815,109.45039449058,109.459017636809,109.53951051673,
109.619892861137,109.703855364764,109.784009846555,109.864090723313,109.944088707341,
109.955742875644),.UNSPECIFIED.);
#174=B_SPLINE_CURVE_WITH_KNOTS('',3,(#16953,#16954,#16955,#16956,#16957,
#16958,#16959,#16960,#16961,#16962,#16963,#16964,#16965,#16966,#16967,#16968,
#16969,#16970,#16971,#16972,#16973,#16974,#16975,#16976,#16977,#16978,#16979,
#16980,#16981,#16982,#16983,#16984,#16985,#16986,#16987,#16988,#16989,#16990,
#16991,#16992,#16993,#16994,#16995,#16996,#16997,#16998,#16999,#17000,#17001,
#17002,#17003,#17004,#17005,#17006,#17007,#17008,#17009,#17010,#17011,#17012,
#17013,#17014,#17015,#17016,#17017,#17018,#17019,#17020,#17021,#17022,#17023,
#17024,#17025,#17026,#17027,#17028,#17029,#17030,#17031,#17032,#17033,#17034,
#17035,#17036,#17037,#17038,#17039,#17040,#17041,#17042,#17043,#17044,#17045,
#17046,#17047,#17048,#17049,#17050,#17051,#17052,#17053,#17054,#17055,#17056,
#17057,#17058,#17059,#17060,#17061,#17062,#17063,#17064,#17065,#17066,#17067,
#17068,#17069,#17070,#17071,#17072,#17073,#17074,#17075,#17076,#17077,#17078,
#17079,#17080,#17081,#17082,#17083,#17084,#17085,#17086,#17087,#17088,#17089,
#17090,#17091,#17092,#17093,#17094,#17095,#17096,#17097,#17098,#17099,#17100,
#17101,#17102,#17103,#17104,#17105,#17106,#17107,#17108,#17109,#17110,#17111,
#17112,#17113,#17114,#17115,#17116,#17117,#17118),.UNSPECIFIED.,.F.,.F.,
(4,3,3,3,3,3,3,3,3,3,3,3,3,3,3,3,3,3,3,3,3,3,3,3,3,3,3,3,3,3,3,3,3,3,3,
3,3,3,3,3,3,3,3,3,3,3,3,3,3,3,3,3,3,3,3,4),(109.955742875756,110.037633904134,
110.119660663075,110.204101908521,110.286477313102,110.371951478981,110.45742564486,
110.534289029512,110.611058861322,110.68775139731,110.764382832477,110.840969313261,
110.917827355717,110.99438567868,111.070950013353,111.14753492648,111.224609608088,
111.301316428957,111.378575040934,111.455833652911,111.533363849371,111.610806943976,
111.688178578032,111.765494341601,111.842769784379,111.920030666799,111.997285972443,
112.074549742738,112.151836021222,112.229202834014,112.306611168721,112.384132725284,
112.454241660962,112.531771779025,112.609214808341,112.686586390167,112.763902114527,
112.841177531088,112.918438407113,112.99569371846,113.072957506551,113.150243814935,
113.227610676542,113.305019070474,113.382540703346,113.452649669013,113.529500559795,
113.606259420334,113.682926572603,113.759541261625,113.836118100225,113.912671675508,
113.989233366542,114.065798318672,114.142407825684,114.191567845393),
 .UNSPECIFIED.);
#175=B_SPLINE_CURVE_WITH_KNOTS('',3,(#17124,#17125,#17126,#17127,#17128,
#17129,#17130,#17131,#17132,#17133,#17134,#17135,#17136,#17137,#17138,#17139,
#17140,#17141,#17142,#17143,#17144,#17145,#17146,#17147,#17148,#17149,#17150,
#17151,#17152,#17153,#17154,#17155,#17156,#17157,#17158,#17159,#17160,#17161,
#17162,#17163,#17164,#17165,#17166,#17167,#17168,#17169,#17170,#17171,#17172,
#17173,#17174,#17175,#17176,#17177,#17178,#17179,#17180,#17181,#17182,#17183,
#17184,#17185,#17186,#17187,#17188,#17189,#17190,#17191,#17192,#17193,#17194,
#17195,#17196,#17197,#17198,#17199,#17200,#17201,#17202,#17203,#17204,#17205,
#17206,#17207,#17208,#17209,#17210,#17211,#17212,#17213,#17214,#17215,#17216,
#17217,#17218,#17219,#17220,#17221,#17222,#17223,#17224,#17225,#17226,#17227,
#17228,#17229,#17230,#17231,#17232,#17233,#17234,#17235,#17236,#17237,#17238,
#17239,#17240,#17241,#17242,#17243,#17244,#17245,#17246,#17247,#17248,#17249,
#17250,#17251,#17252,#17253,#17254,#17255,#17256,#17257,#17258,#17259,#17260,
#17261,#17262,#17263,#17264,#17265,#17266,#17267,#17268,#17269,#17270,#17271,
#17272,#17273,#17274,#17275,#17276,#17277,#17278,#17279,#17280,#17281,#17282,
#17283,#17284,#17285,#17286,#17287,#17288,#17289,#17290,#17291,#17292,#17293,
#17294,#17295),.UNSPECIFIED.,.F.,.F.,(4,3,3,3,3,3,3,3,3,3,3,3,3,3,3,3,3,
3,3,3,3,3,3,3,3,3,3,3,3,3,3,3,3,3,3,3,3,3,3,3,3,3,3,3,3,3,3,3,3,3,3,3,3,
3,3,3,3,4),(116.238928182824,116.274519282519,116.352036651715,116.429466719167,
116.506825140436,116.584127519651,116.661389420414,116.738636631105,116.815878155324,
116.89312804667,116.970400360813,117.047753432039,117.125147961791,117.202656466753,
117.274272893888,117.351094091043,117.427826053257,117.504485031405,117.581087217866,
117.657648759747,117.734695977936,117.81124015258,117.887794432626,117.964373397605,
118.041786674519,118.118498154826,118.196262330042,118.274026505258,118.351609128872,
118.429099111081,118.506512088306,118.583863641807,118.661169308719,118.738451901764,
118.815723688708,118.892998688564,118.970290919503,119.047655591867,119.1250572003,
119.202565014908,119.273780116627,119.355264089582,119.436643453721,119.520896820869,
119.60205031604,119.683126993999,119.764112421789,119.773656922312,119.854665318216,
119.935749575048,120.020195613285,120.101501694992,120.182885484761,120.264390145789,
120.273533727996,120.351058891167,120.428490576211,120.47615534713),
 .UNSPECIFIED.);
#176=B_SPLINE_CURVE_WITH_KNOTS('',3,(#17296,#17297,#17298,#17299,#17300,
#17301,#17302,#17303,#17304,#17305,#17306,#17307,#17308,#17309,#17310,#17311,
#17312,#17313,#17314,#17315,#17316,#17317,#17318,#17319,#17320,#17321,#17322,
#17323,#17324,#17325,#17326,#17327,#17328,#17329,#17330,#17331,#17332,#17333,
#17334,#17335,#17336,#17337,#17338,#17339,#17340,#17341,#17342,#17343,#17344,
#17345,#17346,#17347,#17348,#17349,#17350,#17351,#17352,#17353,#17354,#17355,
#17356,#17357,#17358,#17359,#17360,#17361,#17362,#17363,#17364,#17365,#17366,
#17367,#17368,#17369,#17370,#17371,#17372,#17373,#17374,#17375,#17376,#17377,
#17378,#17379,#17380),.UNSPECIFIED.,.F.,.F.,(4,3,3,3,3,3,3,3,3,3,3,3,3,
3,3,3,3,3,3,3,3,3,3,3,3,3,3,3,4),(114.192169701311,114.269773263717,114.27501205978,
114.351860682967,114.428615529364,114.505292868769,114.581908908544,114.658479807169,
114.735515540166,114.812057958872,114.888606295434,114.965175126882,115.042572762949,
115.119263843902,115.197014757526,115.27476567115,115.351855019129,115.428857167646,
115.50578817035,115.582664026712,115.659500694152,115.736324251519,115.813143990561,
115.889974319783,115.966829651356,116.043764396594,116.120743639361,116.197826713264,
116.238928182687),.UNSPECIFIED.);
#177=B_SPLINE_CURVE_WITH_KNOTS('',3,(#17382,#17383,#17384,#17385,#17386,
#17387,#17388,#17389,#17390,#17391,#17392,#17393,#17394,#17395,#17396,#17397,
#17398,#17399,#17400,#17401,#17402,#17403,#17404,#17405,#17406,#17407,#17408,
#17409,#17410,#17411,#17412,#17413,#17414,#17415,#17416,#17417,#17418,#17419,
#17420,#17421,#17422,#17423,#17424,#17425,#17426,#17427,#17428,#17429,#17430,
#17431,#17432,#17433,#17434,#17435,#17436,#17437,#17438,#17439,#17440,#17441,
#17442,#17443,#17444,#17445,#17446,#17447,#17448,#17449,#17450,#17451,#17452,
#17453,#17454,#17455,#17456,#17457,#17458,#17459,#17460,#17461,#17462,#17463,
#17464,#17465,#17466),.UNSPECIFIED.,.F.,.F.,(4,3,3,3,3,3,3,3,3,3,3,3,3,
3,3,3,3,3,3,3,3,3,3,3,3,3,3,3,4),(114.191567845393,114.268277197137,114.345039195796,
114.42191142385,114.451057677064,114.528652346498,114.606154612608,114.683580097679,
114.760944369056,114.838262950147,114.915558654618,114.992843699274,115.070132091207,
115.147437836733,115.22481587672,115.302230948465,115.379751562736,115.449465685115,
115.530951999548,115.612334081907,115.696417983715,115.777575302568,115.858656086323,
115.939646078357,115.94866968914,116.024039768399,116.099422917702,116.174874532357,
116.238928182733),.UNSPECIFIED.);
#178=B_SPLINE_CURVE_WITH_KNOTS('',3,(#17467,#17468,#17469,#17470,#17471,
#17472,#17473,#17474,#17475,#17476,#17477,#17478,#17479,#17480,#17481,#17482,
#17483,#17484,#17485,#17486,#17487,#17488,#17489,#17490,#17491,#17492,#17493,
#17494,#17495,#17496,#17497,#17498,#17499,#17500,#17501,#17502,#17503,#17504,
#17505,#17506,#17507,#17508,#17509,#17510,#17511,#17512,#17513,#17514,#17515,
#17516,#17517,#17518,#17519,#17520,#17521,#17522,#17523,#17524,#17525,#17526,
#17527,#17528,#17529,#17530,#17531,#17532,#17533,#17534,#17535,#17536,#17537,
#17538,#17539,#17540,#17541,#17542,#17543,#17544,#17545,#17546,#17547,#17548,
#17549,#17550,#17551,#17552,#17553,#17554,#17555,#17556,#17557,#17558,#17559,
#17560,#17561,#17562,#17563,#17564,#17565,#17566,#17567,#17568,#17569,#17570,
#17571,#17572,#17573,#17574,#17575,#17576,#17577,#17578,#17579,#17580,#17581,
#17582,#17583,#17584,#17585,#17586,#17587,#17588,#17589,#17590,#17591,#17592,
#17593,#17594,#17595,#17596,#17597,#17598,#17599,#17600,#17601,#17602,#17603,
#17604,#17605,#17606,#17607,#17608,#17609,#17610,#17611,#17612,#17613,#17614,
#17615,#17616,#17617,#17618,#17619,#17620,#17621,#17622,#17623,#17624,#17625,
#17626,#17627,#17628,#17629,#17630,#17631,#17632),.UNSPECIFIED.,.F.,.F.,
(4,3,3,3,3,3,3,3,3,3,3,3,3,3,3,3,3,3,3,3,3,3,3,3,3,3,3,3,3,3,3,3,3,3,3,
3,3,3,3,3,3,3,3,3,3,3,3,3,3,3,3,3,3,3,3,4),(116.238928182823,116.343400937995,
116.447873693166,116.525401846375,116.602848721337,116.680229900044,116.757560917505,
116.834857272335,116.912147572671,116.98943748041,117.066741002408,117.144072150535,
117.221491640356,117.298956998778,117.376542385076,117.446281701217,117.523145085869,
117.599914917679,117.676607453668,117.753238888834,117.829825369618,117.906683412074,
117.983241735037,118.05980606971,118.136390982837,118.213465664445,118.290172485314,
118.367431097291,118.444689709268,118.522219905728,118.599663000333,118.677034634389,
118.754350397958,118.831625840736,118.908886723155,118.9861420288,119.063405799094,
119.140692077578,119.21805889037,119.295467225077,119.37298878164,119.443097717319,
119.520627835382,119.598070864698,119.675442446524,119.752758170883,119.830033587445,
119.90729446347,119.984549774816,120.061813562908,120.139099871292,120.216466732898,
120.29387512683,120.371396759702,120.441505725369,120.47591264955),
 .UNSPECIFIED.);
#179=B_SPLINE_CURVE_WITH_KNOTS('',3,(#17638,#17639,#17640,#17641,#17642,
#17643,#17644,#17645,#17646,#17647,#17648,#17649,#17650,#17651,#17652,#17653,
#17654,#17655,#17656,#17657,#17658,#17659,#17660,#17661,#17662,#17663,#17664,
#17665,#17666,#17667,#17668,#17669,#17670,#17671,#17672,#17673,#17674,#17675,
#17676,#17677,#17678,#17679,#17680,#17681,#17682,#17683,#17684,#17685,#17686,
#17687,#17688,#17689,#17690,#17691,#17692,#17693,#17694,#17695,#17696,#17697,
#17698,#17699,#17700,#17701,#17702,#17703,#17704,#17705,#17706,#17707,#17708,
#17709,#17710,#17711,#17712,#17713,#17714,#17715,#17716,#17717,#17718,#17719,
#17720,#17721,#17722,#17723,#17724,#17725,#17726,#17727,#17728,#17729,#17730,
#17731,#17732,#17733,#17734,#17735,#17736,#17737,#17738,#17739,#17740,#17741,
#17742,#17743,#17744,#17745,#17746,#17747,#17748,#17749,#17750,#17751,#17752,
#17753,#17754,#17755,#17756,#17757,#17758,#17759,#17760,#17761,#17762,#17763,
#17764,#17765,#17766,#17767,#17768,#17769,#17770,#17771,#17772,#17773,#17774,
#17775,#17776,#17777,#17778,#17779,#17780,#17781,#17782,#17783,#17784,#17785,
#17786,#17787,#17788,#17789,#17790,#17791,#17792,#17793,#17794),
 .UNSPECIFIED.,.F.,.F.,(4,3,3,3,3,3,3,3,3,3,3,3,3,3,3,3,3,3,3,3,3,3,3,3,
3,3,3,3,3,3,3,3,3,3,3,3,3,3,3,3,3,3,3,3,3,3,3,3,3,3,3,3,4),(122.522113490003,
122.604575696039,122.687037553779,122.769499070073,122.85196025177,122.934421105721,
123.016881638776,123.099341857782,123.18180176959,123.264261381048,123.346720699004,
123.429179730306,123.511638481803,123.594096960342,123.67655517277,123.759013125934,
123.841470826682,123.92392828186,124.006385498314,124.092397724816,124.175722069239,
124.258188674685,124.340654435926,124.423119380379,124.505583535455,124.588046928563,
124.670509587112,124.752971538505,124.835432810143,124.917893429428,125.000353423754,
125.082812820519,125.165271647114,125.247729930931,125.330187699358,125.412644979784,
125.496778215195,125.579244213287,125.661708589642,125.744171453904,125.826632915695,
125.909093084616,125.991552070252,126.074009982169,126.159605827694,126.242070564294,
126.324532336296,126.406991582138,126.489448740115,126.571911258396,126.654368929251,
126.736827719202,126.758776746367),.UNSPECIFIED.);
#180=B_SPLINE_CURVE_WITH_KNOTS('',3,(#17795,#17796,#17797,#17798,#17799,
#17800,#17801,#17802,#17803,#17804,#17805,#17806,#17807,#17808,#17809,#17810,
#17811,#17812,#17813,#17814,#17815,#17816,#17817,#17818,#17819,#17820,#17821,
#17822,#17823,#17824,#17825,#17826,#17827,#17828,#17829,#17830,#17831,#17832,
#17833,#17834,#17835,#17836,#17837,#17838,#17839,#17840,#17841,#17842,#17843,
#17844,#17845,#17846,#17847,#17848,#17849,#17850,#17851,#17852,#17853,#17854,
#17855,#17856,#17857,#17858,#17859,#17860,#17861,#17862,#17863,#17864,#17865,
#17866,#17867,#17868,#17869,#17870,#17871,#17872,#17873,#17874,#17875,#17876),
 .UNSPECIFIED.,.F.,.F.,(4,3,3,3,3,3,3,3,3,3,3,3,3,3,3,3,3,3,3,3,3,3,3,3,
3,3,3,4),(120.47615534713,120.553490920204,120.630785720323,120.711098422703,
120.788373593687,120.865657447954,120.942964006615,121.020307300857,121.097742078208,
121.175230936057,121.252826406552,121.273287339366,121.350135962554,121.42689080895,
121.503568148355,121.58018418813,121.656755086755,121.733790819752,121.810333238458,
121.886881575021,121.963450406469,122.040848042535,122.117539123488,122.195290037111,
122.273040950735,122.376675837801,122.477853026382,122.522113490003),
 .UNSPECIFIED.);
#181=B_SPLINE_CURVE_WITH_KNOTS('',3,(#17878,#17879,#17880,#17881,#17882,
#17883,#17884,#17885,#17886,#17887,#17888,#17889,#17890,#17891,#17892,#17893,
#17894,#17895,#17896,#17897,#17898,#17899,#17900,#17901,#17902,#17903,#17904,
#17905,#17906,#17907,#17908,#17909,#17910,#17911,#17912,#17913,#17914,#17915,
#17916,#17917,#17918,#17919,#17920,#17921,#17922,#17923,#17924,#17925,#17926,
#17927,#17928,#17929,#17930,#17931,#17932,#17933,#17934,#17935,#17936,#17937,
#17938,#17939,#17940,#17941,#17942,#17943,#17944,#17945,#17946,#17947,#17948,
#17949,#17950,#17951,#17952,#17953,#17954,#17955,#17956,#17957,#17958,#17959),
 .UNSPECIFIED.,.F.,.F.,(4,3,3,3,3,3,3,3,3,3,3,3,3,3,3,3,3,3,3,3,3,3,3,3,
3,3,3,4),(120.47591264955,120.55270682257,120.629419256148,120.706066160806,
120.782663694973,120.859227977659,120.935788714438,121.012351541726,121.088931025486,
121.165541739534,121.242242394116,121.318993148849,121.395858281635,121.43991373342,
121.517508402854,121.595010668965,121.672436154035,121.749800425412,121.827119006503,
121.904414710975,121.981699755631,122.058988147564,122.136293893089,122.213671933077,
122.291087004821,122.368607619093,122.438321741471,122.522113490003),
 .UNSPECIFIED.);
#182=B_SPLINE_CURVE_WITH_KNOTS('',3,(#17960,#17961,#17962,#17963,#17964,
#17965,#17966,#17967,#17968,#17969,#17970,#17971,#17972,#17973,#17974,#17975,
#17976,#17977,#17978,#17979,#17980,#17981,#17982,#17983,#17984,#17985,#17986,
#17987,#17988,#17989,#17990,#17991,#17992,#17993,#17994,#17995,#17996,#17997,
#17998,#17999,#18000,#18001,#18002,#18003,#18004,#18005,#18006,#18007,#18008,
#18009,#18010,#18011,#18012,#18013,#18014,#18015,#18016,#18017,#18018,#18019,
#18020,#18021,#18022,#18023,#18024,#18025,#18026,#18027,#18028,#18029,#18030,
#18031,#18032,#18033,#18034,#18035,#18036,#18037,#18038,#18039,#18040,#18041,
#18042,#18043,#18044,#18045,#18046,#18047,#18048,#18049,#18050,#18051,#18052,
#18053,#18054,#18055,#18056,#18057,#18058,#18059,#18060,#18061,#18062,#18063,
#18064,#18065,#18066,#18067,#18068,#18069,#18070,#18071,#18072,#18073,#18074,
#18075,#18076,#18077,#18078,#18079,#18080,#18081,#18082,#18083,#18084,#18085,
#18086,#18087,#18088,#18089,#18090,#18091,#18092,#18093,#18094,#18095,#18096,
#18097,#18098,#18099,#18100,#18101,#18102,#18103,#18104,#18105,#18106,#18107,
#18108,#18109,#18110,#18111,#18112,#18113,#18114,#18115,#18116,#18117,#18118,
#18119,#18120,#18121,#18122,#18123,#18124,#18125,#18126,#18127,#18128,#18129,
#18130,#18131),.UNSPECIFIED.,.F.,.F.,(4,3,3,3,3,3,3,3,3,3,3,3,3,3,3,3,3,
3,3,3,3,3,3,3,3,3,3,3,3,3,3,3,3,3,3,3,3,3,3,3,3,3,3,3,3,3,3,3,3,3,3,3,3,
3,3,3,3,4),(122.522113490138,122.600488126397,122.678775016274,122.756968288714,
122.835107118422,122.913196242504,122.937525745497,123.018538851787,123.099627546061,
123.183903096926,123.265212563315,123.346599464526,123.428106603291,123.436729749522,
123.514257902731,123.591704777692,123.6690859564,123.746416973861,123.823713328691,
123.901003629027,123.978293536765,124.055597058764,124.132928206891,124.210347696712,
124.287813055134,124.365398441432,124.435137757573,124.512001142225,124.588770974035,
124.665463510023,124.74209494519,124.818681425974,124.89553946843,124.972097791393,
125.048662126066,125.125247039194,125.202321720801,125.27902854167,125.356287153647,
125.433545765624,125.511075962084,125.588519056689,125.665890690745,125.743206454314,
125.820481897092,125.897742779511,125.974998085156,126.05226185545,126.129548133934,
126.206914946726,126.284323281433,126.361844837996,126.431953773675,126.509503675387,
126.586943713325,126.664320168059,126.741635992966,126.759271559359),
 .UNSPECIFIED.);
#183=B_SPLINE_CURVE_WITH_KNOTS('',3,(#18137,#18138,#18139,#18140,#18141,
#18142,#18143,#18144,#18145,#18146,#18147,#18148,#18149,#18150,#18151,#18152,
#18153,#18154,#18155,#18156,#18157,#18158,#18159,#18160,#18161,#18162,#18163,
#18164,#18165,#18166,#18167,#18168,#18169,#18170,#18171,#18172,#18173,#18174,
#18175,#18176,#18177,#18178,#18179,#18180,#18181,#18182,#18183,#18184,#18185,
#18186,#18187,#18188,#18189,#18190,#18191,#18192,#18193,#18194,#18195,#18196,
#18197,#18198,#18199,#18200,#18201,#18202,#18203,#18204,#18205,#18206,#18207,
#18208,#18209,#18210,#18211,#18212,#18213,#18214,#18215,#18216,#18217,#18218,
#18219,#18220,#18221,#18222,#18223,#18224,#18225,#18226,#18227,#18228,#18229,
#18230,#18231,#18232,#18233,#18234,#18235,#18236,#18237,#18238,#18239,#18240,
#18241,#18242,#18243,#18244,#18245,#18246,#18247,#18248,#18249,#18250,#18251,
#18252,#18253,#18254,#18255,#18256,#18257,#18258,#18259,#18260,#18261,#18262,
#18263,#18264,#18265,#18266,#18267,#18268,#18269,#18270,#18271,#18272,#18273,
#18274,#18275,#18276,#18277,#18278,#18279,#18280,#18281,#18282,#18283,#18284,
#18285,#18286,#18287,#18288,#18289,#18290,#18291,#18292,#18293,#18294,#18295,
#18296,#18297,#18298,#18299,#18300,#18301,#18302),.UNSPECIFIED.,.F.,.F.,
(4,3,3,3,3,3,3,3,3,3,3,3,3,3,3,3,3,3,3,3,3,3,3,3,3,3,3,3,3,3,3,3,3,3,3,
3,3,3,3,3,3,3,3,3,3,3,3,3,3,3,3,3,3,3,3,4),(128.805298797183,128.886590232838,
128.968013348574,129.049656555529,129.131416007228,129.213377057373,129.271316230321,
129.348833781939,129.426264001358,129.503622544254,129.580925014841,129.658186976791,
129.735434202574,129.812675713781,129.889925564013,129.967197808926,130.044550766897,
130.121945159206,130.199453486874,130.27106984169,130.348587210886,130.426017278337,
130.503375699607,130.580678078822,130.657939979585,130.735187190276,130.812428714494,
130.88967860584,130.966950919984,131.04430399121,131.121698520961,131.199207025924,
131.270823453059,131.347644650214,131.424376612428,131.501035590576,131.577637777037,
131.654199318918,131.731246537107,131.807790711751,131.884344991797,131.960923956776,
132.03833723369,132.115048713996,132.192812889213,132.270577064429,132.348173410429,
132.425674585281,132.503077670776,132.580424226377,132.657728326265,132.735004017898,
132.812281275791,132.889556293537,132.966874340892,133.041412044979),
 .UNSPECIFIED.);
#184=B_SPLINE_CURVE_WITH_KNOTS('',3,(#18303,#18304,#18305,#18306,#18307,
#18308,#18309,#18310,#18311,#18312,#18313,#18314,#18315,#18316,#18317,#18318,
#18319,#18320,#18321,#18322,#18323,#18324,#18325,#18326,#18327,#18328,#18329,
#18330,#18331,#18332,#18333,#18334,#18335,#18336,#18337,#18338,#18339,#18340,
#18341,#18342,#18343,#18344,#18345,#18346,#18347,#18348,#18349,#18350,#18351,
#18352,#18353,#18354,#18355,#18356,#18357,#18358,#18359,#18360,#18361,#18362,
#18363,#18364,#18365,#18366,#18367,#18368,#18369,#18370,#18371,#18372,#18373,
#18374,#18375,#18376,#18377,#18378),.UNSPECIFIED.,.F.,.F.,(4,3,3,3,3,3,
3,3,3,3,3,3,3,3,3,3,3,3,3,3,3,3,3,3,3,4),(126.758776746367,126.841238350221,
126.923699288191,127.006159587677,127.088619276074,127.171078380776,127.253536929175,
127.335994948661,127.418452466623,127.505130362283,127.587597148119,127.670062261462,
127.752525811968,127.834987909265,127.917448662967,127.999908182664,128.082366577931,
128.164823958328,128.247290344595,128.329753546609,128.412214002889,128.4946721518,
128.577137756679,128.659597635894,128.742061749258,128.805298797183),
 .UNSPECIFIED.);
#185=B_SPLINE_CURVE_WITH_KNOTS('',3,(#18380,#18381,#18382,#18383,#18384,
#18385,#18386,#18387,#18388,#18389,#18390,#18391,#18392,#18393,#18394,#18395,
#18396,#18397,#18398,#18399,#18400,#18401,#18402,#18403,#18404,#18405,#18406,
#18407,#18408,#18409,#18410,#18411,#18412,#18413,#18414,#18415,#18416,#18417,
#18418,#18419,#18420,#18421,#18422,#18423,#18424,#18425,#18426,#18427,#18428,
#18429,#18430,#18431,#18432,#18433,#18434,#18435,#18436,#18437,#18438,#18439,
#18440,#18441,#18442,#18443,#18444,#18445,#18446,#18447,#18448,#18449,#18450,
#18451,#18452,#18453,#18454,#18455,#18456,#18457,#18458,#18459,#18460,#18461),
 .UNSPECIFIED.,.F.,.F.,(4,3,3,3,3,3,3,3,3,3,3,3,3,3,3,3,3,3,3,3,3,3,3,3,
3,3,3,4),(126.759271559359,126.836539945911,126.913798313184,126.991054323545,
127.06832201822,127.145615442332,127.222990672096,127.300410320789,127.377938467087,
127.430361781726,127.507197813849,127.583944829576,127.660619067139,127.73723670666,
127.813813883287,127.890683371598,127.967243474121,128.043813771268,128.12040883229,
128.197499071661,128.274226268243,128.35149802901,128.428769789777,128.522902041628,
128.612256050619,128.701233126335,128.789600144613,128.805298797183),
 .UNSPECIFIED.);
#186=B_SPLINE_CURVE_WITH_KNOTS('',3,(#18462,#18463,#18464,#18465,#18466,
#18467,#18468,#18469,#18470,#18471,#18472,#18473,#18474,#18475,#18476,#18477,
#18478,#18479,#18480,#18481,#18482,#18483,#18484,#18485,#18486,#18487,#18488,
#18489,#18490,#18491,#18492,#18493,#18494,#18495,#18496,#18497,#18498,#18499,
#18500,#18501,#18502,#18503,#18504,#18505,#18506,#18507,#18508,#18509,#18510,
#18511,#18512,#18513,#18514,#18515,#18516,#18517,#18518,#18519,#18520,#18521,
#18522,#18523,#18524,#18525,#18526,#18527,#18528,#18529,#18530,#18531,#18532,
#18533,#18534,#18535,#18536,#18537,#18538,#18539,#18540,#18541,#18542,#18543,
#18544,#18545,#18546,#18547,#18548,#18549,#18550,#18551,#18552,#18553,#18554,
#18555,#18556,#18557,#18558,#18559,#18560,#18561,#18562,#18563,#18564,#18565,
#18566,#18567,#18568,#18569,#18570,#18571,#18572,#18573,#18574,#18575,#18576,
#18577,#18578,#18579,#18580,#18581,#18582,#18583,#18584,#18585,#18586,#18587,
#18588,#18589,#18590,#18591,#18592,#18593,#18594,#18595,#18596,#18597,#18598,
#18599,#18600,#18601,#18602,#18603,#18604,#18605,#18606,#18607,#18608,#18609,
#18610,#18611,#18612,#18613,#18614,#18615,#18616,#18617,#18618),
 .UNSPECIFIED.,.F.,.F.,(4,3,3,3,3,3,3,3,3,3,3,3,3,3,3,3,3,3,3,3,3,3,3,3,
3,3,3,3,3,3,3,3,3,3,3,3,3,3,3,3,3,3,3,3,3,3,3,3,3,3,3,3,4),(128.805298797183,
128.887761003219,128.970222860959,129.052684377253,129.13514555895,129.217606412901,
129.300066945956,129.382527164962,129.46498707677,129.547446688228,129.629906006184,
129.712365037486,129.794823788983,129.877282267521,129.959740479949,130.042198433113,
130.124656133861,130.207113589039,130.289570805493,130.375583031995,130.458907376419,
130.541373981864,130.623839743105,130.706304687558,130.788768842634,130.871232235743,
130.953694894291,131.036156845684,131.118618117323,131.201078736607,131.283538730934,
131.365998127698,131.448456954294,131.53091523811,131.613373006538,131.695830286963,
131.779963522374,131.862429520466,131.944893896822,132.027356761084,132.109818222874,
132.192278391796,132.274737377431,132.357195289348,132.442791134873,132.525255871473,
132.607717643475,132.690176889317,132.772634047294,132.855096565576,132.93755423643,
133.020013026381,133.041962053546),.UNSPECIFIED.);
#187=B_SPLINE_CURVE_WITH_KNOTS('',3,(#18624,#18625,#18626,#18627,#18628,
#18629,#18630,#18631,#18632,#18633,#18634,#18635,#18636,#18637,#18638,#18639,
#18640,#18641,#18642,#18643,#18644,#18645,#18646,#18647,#18648,#18649,#18650,
#18651,#18652,#18653,#18654,#18655,#18656,#18657,#18658,#18659,#18660,#18661,
#18662,#18663,#18664,#18665,#18666,#18667,#18668,#18669,#18670,#18671,#18672,
#18673,#18674,#18675,#18676,#18677,#18678,#18679,#18680,#18681,#18682,#18683,
#18684,#18685,#18686,#18687,#18688,#18689,#18690,#18691,#18692,#18693,#18694,
#18695,#18696,#18697,#18698,#18699,#18700,#18701,#18702,#18703,#18704,#18705,
#18706,#18707,#18708,#18709,#18710,#18711,#18712,#18713,#18714,#18715,#18716,
#18717,#18718,#18719,#18720,#18721,#18722,#18723,#18724,#18725,#18726,#18727,
#18728,#18729,#18730,#18731,#18732,#18733,#18734,#18735,#18736,#18737,#18738,
#18739,#18740,#18741,#18742,#18743,#18744,#18745,#18746,#18747,#18748,#18749,
#18750,#18751,#18752,#18753,#18754,#18755,#18756,#18757,#18758,#18759,#18760,
#18761,#18762,#18763,#18764,#18765,#18766,#18767,#18768,#18769,#18770,#18771,
#18772,#18773,#18774,#18775,#18776,#18777,#18778,#18779,#18780),
 .UNSPECIFIED.,.F.,.F.,(4,3,3,3,3,3,3,3,3,3,3,3,3,3,3,3,3,3,3,3,3,3,3,3,
3,3,3,3,3,3,3,3,3,3,3,3,3,3,3,3,3,3,3,3,3,3,3,3,3,3,3,3,4),(135.088484104362,
135.170946310398,135.253408168138,135.335869684432,135.418330866129,135.50079172008,
135.583252253135,135.665712472141,135.748172383949,135.830631995407,135.913091313363,
135.995550344665,136.078009096162,136.1604675747,136.242925787128,136.325383740292,
136.40784144104,136.490298896218,136.572756112673,136.658768339175,136.742092683598,
136.824559289043,136.907025050285,136.989489994737,137.071954149813,137.154417542922,
137.236880201471,137.319342152864,137.401803424502,137.484264043786,137.566724038113,
137.649183434878,137.731642261473,137.81410054529,137.896558313717,137.979015594142,
138.063148829554,138.145614827645,138.228079204001,138.310542068263,138.393003530054,
138.475463698975,138.557922684611,138.640380596528,138.725976442053,138.808441178653,
138.890902950655,138.973362196497,139.055819354474,139.138281872755,139.22073954361,
139.303198333561,139.325147360726),.UNSPECIFIED.);
#188=B_SPLINE_CURVE_WITH_KNOTS('',3,(#18781,#18782,#18783,#18784,#18785,
#18786,#18787,#18788,#18789,#18790,#18791,#18792,#18793,#18794,#18795,#18796,
#18797,#18798,#18799,#18800,#18801,#18802,#18803,#18804,#18805,#18806,#18807,
#18808,#18809,#18810,#18811,#18812,#18813,#18814,#18815,#18816,#18817,#18818,
#18819,#18820,#18821,#18822,#18823,#18824,#18825,#18826,#18827,#18828,#18829,
#18830,#18831,#18832,#18833,#18834,#18835,#18836,#18837,#18838,#18839,#18840,
#18841,#18842,#18843,#18844,#18845,#18846,#18847,#18848,#18849,#18850,#18851,
#18852,#18853,#18854,#18855,#18856,#18857,#18858,#18859,#18860,#18861,#18862,
#18863,#18864,#18865),.UNSPECIFIED.,.F.,.F.,(4,3,3,3,3,3,3,3,3,3,3,3,3,
3,3,3,3,3,3,3,3,3,3,3,3,3,3,3,4),(133.041412044979,133.118812100158,133.19631907369,
133.270330675798,133.351814648753,133.433194012892,133.51744738004,133.598600875211,
133.67967755317,133.76066298096,133.770207481483,133.851215877387,133.932300134219,
134.016746172456,134.098052254163,134.179436043931,134.26094070496,134.270084287167,
134.346164168423,134.42216215834,134.498094981456,134.573978218577,134.649834970144,
134.725680252268,134.801529071145,134.877429864499,134.953357532579,135.029372167759,
135.087670040789),.UNSPECIFIED.);
#189=B_SPLINE_CURVE_WITH_KNOTS('',3,(#18867,#18868,#18869,#18870,#18871,
#18872,#18873,#18874,#18875,#18876,#18877,#18878,#18879,#18880,#18881,#18882,
#18883,#18884,#18885,#18886,#18887,#18888,#18889,#18890,#18891,#18892,#18893,
#18894,#18895,#18896,#18897,#18898,#18899,#18900,#18901,#18902,#18903,#18904,
#18905,#18906,#18907,#18908,#18909,#18910,#18911,#18912,#18913,#18914,#18915,
#18916,#18917,#18918,#18919,#18920,#18921,#18922,#18923,#18924,#18925,#18926,
#18927,#18928,#18929,#18930,#18931,#18932,#18933,#18934,#18935,#18936,#18937,
#18938,#18939,#18940,#18941,#18942),.UNSPECIFIED.,.F.,.F.,(4,3,3,3,3,3,
3,3,3,3,3,3,3,3,3,3,3,3,3,3,3,3,3,3,3,4),(133.041962053546,133.1244236574,
133.206884595371,133.289344894856,133.371804583253,133.454263687955,133.536722236354,
133.619180255841,133.701637773802,133.788315669462,133.870782455298,133.953247568642,
134.035711119147,134.118173216444,134.200633970146,134.283093489843,134.365551885111,
134.448009265508,134.530475651774,134.612938853788,134.695399310068,134.777857458979,
134.860323063858,134.942782943073,135.025247056437,135.088484104362),
 .UNSPECIFIED.);
#190=B_SPLINE_CURVE_WITH_KNOTS('',3,(#18943,#18944,#18945,#18946,#18947,
#18948,#18949,#18950,#18951,#18952,#18953,#18954,#18955,#18956,#18957,#18958,
#18959,#18960,#18961,#18962,#18963,#18964,#18965,#18966,#18967,#18968,#18969,
#18970,#18971,#18972,#18973,#18974,#18975,#18976,#18977,#18978,#18979,#18980,
#18981,#18982,#18983,#18984,#18985,#18986,#18987,#18988,#18989,#18990,#18991,
#18992,#18993,#18994,#18995,#18996,#18997,#18998,#18999,#19000,#19001,#19002,
#19003,#19004,#19005,#19006,#19007,#19008,#19009,#19010,#19011,#19012,#19013,
#19014,#19015,#19016,#19017,#19018,#19019,#19020,#19021,#19022,#19023,#19024,
#19025,#19026,#19027,#19028,#19029,#19030,#19031,#19032,#19033,#19034,#19035,
#19036,#19037,#19038,#19039,#19040,#19041,#19042,#19043,#19044,#19045,#19046,
#19047,#19048,#19049,#19050,#19051,#19052,#19053,#19054,#19055,#19056,#19057,
#19058,#19059,#19060,#19061,#19062,#19063,#19064,#19065,#19066,#19067,#19068,
#19069,#19070,#19071,#19072,#19073,#19074,#19075,#19076,#19077,#19078,#19079,
#19080,#19081,#19082,#19083,#19084,#19085,#19086,#19087,#19088,#19089,#19090,
#19091,#19092,#19093,#19094,#19095,#19096,#19097,#19098,#19099,#19100,#19101,
#19102,#19103,#19104,#19105,#19106,#19107,#19108,#19109,#19110,#19111),
 .UNSPECIFIED.,.F.,.F.,(4,3,3,3,3,3,3,3,3,3,3,3,3,3,3,3,3,3,3,3,3,3,3,3,
3,3,3,3,3,3,3,3,3,3,3,3,3,3,3,3,3,3,3,3,3,3,3,3,3,3,3,3,3,3,3,3,4),(135.088484104362,
135.17791010341,135.267858742395,135.358486777205,135.417625846133,135.495220515567,
135.572722781677,135.650148266748,135.727512538125,135.804831119216,135.882126823688,
135.959411868344,136.036700260277,136.114006005803,136.19138404579,136.268799117535,
136.346319731806,136.416033854184,136.497520168617,136.578902250976,136.662986152784,
136.744143471637,136.825224255392,136.906214247426,136.91523785821,136.9962509645,
137.077339658773,137.161615209639,137.242924676028,137.324311577239,137.405818716004,
137.414441862235,137.491970015444,137.569416890405,137.646798069113,137.724129086573,
137.801425441404,137.87871574174,137.956005649478,138.033309171476,138.110640319603,
138.188059809424,138.265525167846,138.343110554144,138.412849870286,138.489718235985,
138.566492041822,138.643187549574,138.719820957949,138.796408239568,138.87297091787,
138.949523565454,139.026080746546,139.102691812507,139.179329837236,139.256058308962,
139.324627500385),.UNSPECIFIED.);
#191=B_SPLINE_CURVE_WITH_KNOTS('',3,(#19117,#19118,#19119,#19120,#19121,
#19122,#19123,#19124,#19125,#19126,#19127,#19128,#19129,#19130,#19131,#19132,
#19133,#19134,#19135,#19136,#19137,#19138,#19139,#19140,#19141,#19142,#19143,
#19144,#19145,#19146,#19147,#19148,#19149,#19150,#19151,#19152,#19153,#19154,
#19155,#19156,#19157,#19158,#19159,#19160,#19161,#19162,#19163,#19164,#19165,
#19166,#19167,#19168,#19169,#19170,#19171,#19172,#19173,#19174,#19175,#19176,
#19177,#19178,#19179,#19180,#19181,#19182,#19183,#19184,#19185,#19186,#19187,
#19188,#19189,#19190,#19191,#19192,#19193,#19194,#19195,#19196,#19197,#19198,
#19199,#19200,#19201,#19202,#19203,#19204,#19205,#19206,#19207,#19208,#19209,
#19210,#19211,#19212,#19213,#19214,#19215,#19216,#19217,#19218,#19219,#19220,
#19221,#19222,#19223,#19224,#19225,#19226,#19227,#19228,#19229,#19230,#19231,
#19232,#19233,#19234,#19235,#19236,#19237,#19238,#19239,#19240,#19241,#19242,
#19243,#19244,#19245,#19246,#19247,#19248,#19249,#19250,#19251,#19252,#19253,
#19254,#19255,#19256,#19257,#19258,#19259,#19260,#19261,#19262,#19263,#19264,
#19265,#19266,#19267,#19268,#19269,#19270,#19271,#19272,#19273,#19274,#19275,
#19276,#19277,#19278,#19279,#19280,#19281,#19282,#19283,#19284,#19285),
 .UNSPECIFIED.,.F.,.F.,(4,3,3,3,3,3,3,3,3,3,3,3,3,3,3,3,3,3,3,3,3,3,3,3,
3,3,3,3,3,3,3,3,3,3,3,3,3,3,3,3,3,3,3,3,3,3,3,3,3,3,3,3,3,3,3,3,4),(141.372263151081,
141.448917194025,141.525499836524,141.602027358791,141.6785159959,141.754993398329,
141.831467912504,141.907954196066,141.984466911852,142.061064659906,142.137708459711,
142.214465870369,142.268113178122,142.344961801309,142.421716647706,142.498393987111,
142.575010026885,142.65158092551,142.728616658508,142.805159077214,142.881707413776,
142.958276245224,143.035673881291,143.112364962244,143.190115875868,143.267866789492,
143.34538434111,143.42281456053,143.500173103425,143.577475574013,143.654737535963,
143.731984761746,143.809226272953,143.886476123186,143.963748368098,144.041101326069,
144.118495718378,144.196004046047,144.267620400861,144.345137770057,144.422567837509,
144.499926258778,144.577228637993,144.654490538756,144.731737749447,144.808979273666,
144.886229165012,144.963501479155,145.040854550381,145.118249080132,145.195757585095,
145.267374012231,145.344213795142,145.42094068026,145.497602569752,145.57420299272,
145.608744731738),.UNSPECIFIED.);
#192=B_SPLINE_CURVE_WITH_KNOTS('',3,(#19286,#19287,#19288,#19289,#19290,
#19291,#19292,#19293,#19294,#19295,#19296,#19297,#19298,#19299,#19300,#19301,
#19302,#19303,#19304,#19305,#19306,#19307,#19308,#19309,#19310,#19311,#19312,
#19313,#19314,#19315,#19316,#19317,#19318,#19319,#19320,#19321,#19322,#19323,
#19324,#19325,#19326,#19327,#19328,#19329,#19330,#19331,#19332,#19333,#19334,
#19335,#19336,#19337,#19338,#19339,#19340,#19341,#19342,#19343,#19344,#19345,
#19346,#19347,#19348,#19349,#19350,#19351,#19352,#19353,#19354,#19355,#19356,
#19357,#19358,#19359,#19360,#19361),.UNSPECIFIED.,.F.,.F.,(4,3,3,3,3,3,
3,3,3,3,3,3,3,3,3,3,3,3,3,3,3,3,3,3,3,4),(139.325147360726,139.40760896458,
139.49006990255,139.572530202036,139.654989890433,139.737448995135,139.819907543534,
139.90236556302,139.984823080982,140.071500976642,140.153967762478,140.236432875821,
140.318896426327,140.401358523624,140.483819277326,140.566278797023,140.64873719229,
140.731194572688,140.813660958954,140.896124160968,140.978584617248,141.061042766159,
141.143508371038,141.225968250253,141.308432363617,141.371669411542),
 .UNSPECIFIED.);
#193=B_SPLINE_CURVE_WITH_KNOTS('',3,(#19363,#19364,#19365,#19366,#19367,
#19368,#19369,#19370,#19371,#19372,#19373,#19374,#19375,#19376,#19377,#19378,
#19379,#19380,#19381,#19382,#19383,#19384,#19385,#19386,#19387,#19388,#19389,
#19390,#19391,#19392,#19393,#19394,#19395,#19396,#19397,#19398,#19399,#19400,
#19401,#19402,#19403,#19404,#19405,#19406,#19407,#19408,#19409,#19410,#19411,
#19412,#19413,#19414,#19415,#19416,#19417,#19418,#19419,#19420,#19421,#19422,
#19423,#19424,#19425,#19426,#19427,#19428,#19429,#19430,#19431,#19432,#19433,
#19434,#19435,#19436,#19437,#19438,#19439,#19440,#19441,#19442,#19443,#19444,
#19445,#19446,#19447),.UNSPECIFIED.,.F.,.F.,(4,3,3,3,3,3,3,3,3,3,3,3,3,
3,3,3,3,3,3,3,3,3,3,3,3,3,3,3,4),(139.324627500385,139.401481316582,139.411257878337,
139.488788074797,139.566231169402,139.643602803458,139.720918567027,139.798194009805,
139.875454892224,139.952710197869,140.029973968163,140.107260246647,140.18462705944,
140.262035394147,140.33955695071,140.409665886388,140.48672274472,140.563692688849,
140.640591798251,140.717436098154,140.794241571758,140.871034465617,140.947823924016,
141.024624379267,141.101450267632,141.178355915937,141.255306485282,141.332360681074,
141.371669411465),.UNSPECIFIED.);
#194=B_SPLINE_CURVE_WITH_KNOTS('',3,(#19448,#19449,#19450,#19451,#19452,
#19453,#19454,#19455,#19456,#19457,#19458,#19459,#19460,#19461,#19462,#19463,
#19464,#19465,#19466,#19467,#19468,#19469,#19470,#19471,#19472,#19473,#19474,
#19475,#19476,#19477,#19478,#19479,#19480,#19481,#19482,#19483,#19484,#19485,
#19486,#19487,#19488,#19489,#19490,#19491,#19492,#19493,#19494,#19495,#19496,
#19497,#19498,#19499,#19500,#19501,#19502,#19503,#19504,#19505,#19506,#19507,
#19508,#19509,#19510,#19511,#19512,#19513,#19514,#19515,#19516,#19517,#19518,
#19519,#19520,#19521,#19522,#19523,#19524,#19525,#19526,#19527,#19528,#19529,
#19530,#19531,#19532,#19533,#19534,#19535,#19536,#19537,#19538,#19539,#19540,
#19541,#19542,#19543,#19544,#19545,#19546,#19547,#19548,#19549,#19550,#19551,
#19552,#19553,#19554,#19555,#19556,#19557,#19558,#19559,#19560,#19561,#19562,
#19563,#19564,#19565,#19566,#19567,#19568,#19569,#19570,#19571,#19572,#19573,
#19574,#19575,#19576,#19577,#19578,#19579,#19580,#19581,#19582,#19583,#19584,
#19585,#19586,#19587,#19588,#19589,#19590,#19591,#19592,#19593,#19594,#19595,
#19596,#19597,#19598,#19599,#19600,#19601,#19602,#19603,#19604,#19605,#19606,
#19607,#19608,#19609,#19610,#19611,#19612,#19613,#19614,#19615,#19616,#19617,
#19618,#19619),.UNSPECIFIED.,.F.,.F.,(4,3,3,3,3,3,3,3,3,3,3,3,3,3,3,3,3,
3,3,3,3,3,3,3,3,3,3,3,3,3,3,3,3,3,3,3,3,3,3,3,3,3,3,3,3,3,3,3,3,3,3,3,3,
3,3,3,3,4),(141.371669411542,141.408073894439,141.484909926562,141.561656942289,
141.638331179852,141.714948819374,141.791525996001,141.868395484312,141.944955586835,
142.021525883982,142.098120945005,142.175211184376,142.251938380958,142.329210141724,
142.40648190249,142.484076571924,142.561578838034,142.639004323105,142.716368594482,
142.793687175573,142.870982880044,142.9482679247,143.025556316633,143.102862062159,
143.180240102146,143.257655173891,143.335175788162,143.404889910541,143.486376224974,
143.567758307333,143.651842209141,143.732999527994,143.814080311748,143.895070303782,
143.904093914566,143.985107020856,144.066195715129,144.150471265995,144.231780732384,
144.313167633595,144.39467477236,144.403297918591,144.4808260718,144.558272946762,
144.635654125469,144.71298514293,144.79028149776,144.867571798096,144.944861705834,
145.022165227832,145.09949637596,145.176915865781,145.254381224202,145.331966610501,
145.401705926642,145.478579288395,145.555343991007,145.609203979305),
 .UNSPECIFIED.);
#195=B_SPLINE_CURVE_WITH_KNOTS('',3,(#19625,#19626,#19627,#19628,#19629,
#19630,#19631,#19632,#19633,#19634,#19635,#19636,#19637,#19638,#19639,#19640,
#19641,#19642,#19643,#19644,#19645,#19646,#19647,#19648,#19649,#19650,#19651,
#19652,#19653,#19654,#19655,#19656,#19657,#19658,#19659,#19660,#19661,#19662,
#19663,#19664,#19665,#19666,#19667,#19668,#19669,#19670,#19671,#19672,#19673,
#19674,#19675,#19676,#19677,#19678,#19679,#19680,#19681,#19682,#19683,#19684,
#19685,#19686,#19687,#19688,#19689,#19690,#19691,#19692,#19693,#19694,#19695,
#19696,#19697,#19698,#19699,#19700,#19701,#19702,#19703,#19704,#19705,#19706,
#19707,#19708,#19709,#19710,#19711,#19712,#19713,#19714,#19715,#19716,#19717,
#19718,#19719,#19720,#19721,#19722,#19723,#19724,#19725,#19726,#19727,#19728,
#19729,#19730,#19731,#19732,#19733,#19734,#19735,#19736,#19737,#19738,#19739,
#19740,#19741,#19742,#19743,#19744,#19745,#19746,#19747,#19748,#19749,#19750,
#19751,#19752,#19753,#19754,#19755,#19756,#19757,#19758,#19759,#19760,#19761,
#19762,#19763,#19764,#19765,#19766,#19767,#19768,#19769,#19770,#19771,#19772,
#19773,#19774,#19775,#19776,#19777,#19778,#19779,#19780,#19781),
 .UNSPECIFIED.,.F.,.F.,(4,3,3,3,3,3,3,3,3,3,3,3,3,3,3,3,3,3,3,3,3,3,3,3,
3,3,3,3,3,3,3,3,3,3,3,3,3,3,3,3,3,3,3,3,3,3,3,3,3,3,3,3,4),(147.654854718721,
147.737316924757,147.819778782497,147.902240298791,147.984701480488,148.067162334439,
148.149622867494,148.2320830865,148.314542998308,148.397002609766,148.479461927722,
148.561920959024,148.644379710521,148.726838189059,148.809296401487,148.891754354652,
148.974212055399,149.056669510577,149.139126727032,149.225138953534,149.308463297957,
149.390929903402,149.473395664644,149.555860609096,149.638324764172,149.720788157281,
149.80325081583,149.885712767223,149.968174038861,150.050634658146,150.133094652472,
150.215554049237,150.298012875832,150.380471159649,150.462928928076,150.545386208501,
150.629519443913,150.711985442004,150.79444981836,150.876912682622,150.959374144413,
151.041834313334,151.124293298969,151.206751210887,151.292347056411,151.374811793012,
151.457273565014,151.539732810856,151.622189968833,151.704652487114,151.787110157969,
151.86956894792,151.891517975085),.UNSPECIFIED.);
#196=B_SPLINE_CURVE_WITH_KNOTS('',3,(#19782,#19783,#19784,#19785,#19786,
#19787,#19788,#19789,#19790,#19791,#19792,#19793,#19794,#19795,#19796,#19797,
#19798,#19799,#19800,#19801,#19802,#19803,#19804,#19805,#19806,#19807,#19808,
#19809,#19810,#19811,#19812,#19813,#19814,#19815,#19816,#19817,#19818,#19819,
#19820,#19821,#19822,#19823,#19824,#19825,#19826,#19827,#19828,#19829,#19830,
#19831,#19832,#19833,#19834,#19835,#19836,#19837,#19838,#19839,#19840,#19841,
#19842,#19843,#19844,#19845,#19846,#19847,#19848,#19849,#19850,#19851,#19852,
#19853,#19854,#19855,#19856,#19857,#19858,#19859,#19860,#19861,#19862,#19863),
 .UNSPECIFIED.,.F.,.F.,(4,3,3,3,3,3,3,3,3,3,3,3,3,3,3,3,3,3,3,3,3,3,3,3,
3,3,3,4),(145.608744731738,145.685293209367,145.761838066389,145.838384935465,
145.914948392851,145.99154302266,146.06822781809,146.144962671921,146.221812557441,
146.2671276236,146.344710247214,146.422200229423,146.499613206648,146.576964760148,
146.654270427059,146.731553020104,146.808824807048,146.886099806905,146.963392037843,
147.040756710208,147.11815831864,147.195666133248,147.266881234969,147.352578401241,
147.438023806837,147.523300561661,147.608298891338,147.654854718721),
 .UNSPECIFIED.);
#197=B_SPLINE_CURVE_WITH_KNOTS('',3,(#19865,#19866,#19867,#19868,#19869,
#19870,#19871,#19872,#19873,#19874,#19875,#19876,#19877,#19878,#19879,#19880,
#19881,#19882,#19883,#19884,#19885,#19886,#19887,#19888,#19889,#19890,#19891,
#19892,#19893,#19894,#19895,#19896,#19897,#19898,#19899,#19900,#19901,#19902,
#19903,#19904,#19905,#19906,#19907,#19908,#19909,#19910,#19911,#19912,#19913,
#19914,#19915,#19916,#19917,#19918,#19919,#19920,#19921,#19922,#19923,#19924,
#19925,#19926,#19927,#19928,#19929,#19930,#19931,#19932,#19933,#19934,#19935,
#19936,#19937,#19938,#19939,#19940,#19941,#19942,#19943,#19944,#19945,#19946),
 .UNSPECIFIED.,.F.,.F.,(4,3,3,3,3,3,3,3,3,3,3,3,3,3,3,3,3,3,3,3,3,3,3,3,
3,3,3,4),(145.609203979305,145.685851916934,145.762450096981,145.842158076695,
145.918717225157,145.995278590263,146.071856737559,146.148466240428,146.225160926237,
146.301905983306,146.378753985428,146.400113934693,146.477644131153,146.555087225758,
146.632458859814,146.709774623383,146.787050066161,146.864310948581,146.941566254225,
147.018830024519,147.096116303004,147.173483115796,147.250891450503,147.328413007066,
147.398521942744,147.497828613867,147.595438794475,147.654854718574),
 .UNSPECIFIED.);
#198=B_SPLINE_CURVE_WITH_KNOTS('',3,(#19947,#19948,#19949,#19950,#19951,
#19952,#19953,#19954,#19955,#19956,#19957,#19958,#19959,#19960,#19961,#19962,
#19963,#19964,#19965,#19966,#19967,#19968,#19969,#19970,#19971,#19972,#19973,
#19974,#19975,#19976,#19977,#19978,#19979,#19980,#19981,#19982,#19983,#19984,
#19985,#19986,#19987,#19988,#19989,#19990,#19991,#19992,#19993,#19994,#19995,
#19996,#19997,#19998,#19999,#20000,#20001,#20002,#20003,#20004,#20005,#20006,
#20007,#20008,#20009,#20010,#20011,#20012,#20013,#20014,#20015,#20016,#20017,
#20018,#20019,#20020,#20021,#20022,#20023,#20024,#20025,#20026,#20027,#20028,
#20029,#20030,#20031,#20032,#20033,#20034,#20035,#20036,#20037,#20038,#20039,
#20040,#20041,#20042,#20043,#20044,#20045,#20046,#20047,#20048,#20049,#20050,
#20051,#20052,#20053,#20054,#20055,#20056,#20057,#20058,#20059,#20060,#20061,
#20062,#20063,#20064,#20065,#20066,#20067,#20068,#20069,#20070,#20071,#20072,
#20073,#20074,#20075,#20076,#20077,#20078,#20079,#20080,#20081,#20082,#20083,
#20084,#20085,#20086,#20087,#20088,#20089,#20090,#20091,#20092,#20093,#20094,
#20095,#20096,#20097,#20098,#20099,#20100,#20101,#20102,#20103,#20104,#20105,
#20106,#20107,#20108,#20109,#20110,#20111,#20112,#20113,#20114,#20115,#20116,
#20117,#20118),.UNSPECIFIED.,.F.,.F.,(4,3,3,3,3,3,3,3,3,3,3,3,3,3,3,3,3,
3,3,3,3,3,3,3,3,3,3,3,3,3,3,3,3,3,3,3,3,3,3,3,3,3,3,3,3,3,3,3,3,3,3,3,3,
3,3,3,3,4),(147.654854718721,147.73146308114,147.808029341825,147.884579267218,
147.961123174402,148.037675664688,148.114251342376,148.190906657983,148.267605147702,
148.34441194142,148.396929950795,148.473765982918,148.550512998645,148.627187236208,
148.70380487573,148.780382052357,148.857251540668,148.933811643191,149.010381940338,
149.08697700136,149.164067240732,149.240794437313,149.31806619808,149.395337958846,
149.47293262828,149.55043489439,149.627860379461,149.705224650838,149.782543231928,
149.8598389364,149.937123981056,150.014412372988,150.091718118514,150.169096158502,
150.246511230246,150.324031844517,150.393745966897,150.47523228133,150.556614363689,
150.640698265497,150.72185558435,150.802936368105,150.883926360138,150.892949970922,
150.973963077213,151.055051771486,151.139327322352,151.220636788742,151.302023689953,
151.383530828717,151.392153974948,151.469682119129,151.547131796174,151.624517128286,
151.701846132548,151.779142456503,151.856423902883,151.891456894454),
 .UNSPECIFIED.);
#199=B_SPLINE_CURVE_WITH_KNOTS('',3,(#20124,#20125,#20126,#20127,#20128,
#20129,#20130,#20131,#20132,#20133,#20134,#20135,#20136,#20137,#20138,#20139,
#20140,#20141,#20142,#20143,#20144,#20145,#20146,#20147,#20148,#20149,#20150,
#20151,#20152,#20153,#20154,#20155,#20156,#20157,#20158,#20159,#20160,#20161,
#20162,#20163,#20164,#20165,#20166,#20167,#20168,#20169,#20170,#20171,#20172,
#20173,#20174,#20175,#20176,#20177,#20178,#20179,#20180,#20181,#20182,#20183,
#20184,#20185,#20186,#20187,#20188,#20189,#20190,#20191,#20192,#20193,#20194,
#20195,#20196,#20197,#20198,#20199,#20200,#20201,#20202,#20203,#20204,#20205,
#20206,#20207,#20208,#20209,#20210,#20211,#20212,#20213,#20214,#20215,#20216,
#20217,#20218,#20219,#20220,#20221,#20222,#20223,#20224,#20225,#20226,#20227,
#20228,#20229,#20230,#20231,#20232,#20233,#20234,#20235,#20236,#20237,#20238,
#20239,#20240,#20241,#20242,#20243,#20244,#20245,#20246,#20247,#20248,#20249,
#20250,#20251,#20252,#20253,#20254,#20255,#20256,#20257,#20258,#20259,#20260,
#20261,#20262,#20263,#20264,#20265,#20266,#20267,#20268,#20269,#20270,#20271,
#20272,#20273,#20274,#20275,#20276,#20277,#20278,#20279,#20280,#20281,#20282,
#20283,#20284,#20285,#20286,#20287,#20288,#20289,#20290,#20291,#20292),
 .UNSPECIFIED.,.F.,.F.,(4,3,3,3,3,3,3,3,3,3,3,3,3,3,3,3,3,3,3,3,3,3,3,3,
3,3,3,3,3,3,3,3,3,3,3,3,3,3,3,3,3,3,3,3,3,3,3,3,3,3,3,3,3,3,3,3,4),(153.938040025901,
154.026398361422,154.115124679214,154.204323905769,154.265156514555,154.34664048751,
154.428019851649,154.512273218797,154.593426713968,154.674503391927,154.755488819716,
154.76503332024,154.846041716144,154.927125972976,155.011572011213,155.09287809292,
155.174261882689,155.255766543717,155.264910125924,155.342425904187,155.419860204598,
155.497228623025,155.574546708175,155.65182997222,155.729107056531,155.806383637019,
155.883673732416,155.960991366421,156.038397572745,156.115849582059,156.193422390381,
156.264663737294,156.341512360481,156.418267206878,156.494944546283,156.571560586058,
156.648131484683,156.72516721768,156.801709636386,156.878257972948,156.954826804396,
157.032224440463,157.108915521415,157.186666435039,157.264417348663,157.341939624551,
157.419373573263,157.496734854269,157.574039074757,157.651302890406,157.728545527247,
157.805781044169,157.883023493393,157.960320239351,158.037645216973,158.115056529675,
158.174289778564),.UNSPECIFIED.);
#200=B_SPLINE_CURVE_WITH_KNOTS('',3,(#20293,#20294,#20295,#20296,#20297,
#20298,#20299,#20300,#20301,#20302,#20303,#20304,#20305,#20306,#20307,#20308,
#20309,#20310,#20311,#20312,#20313,#20314,#20315,#20316,#20317,#20318,#20319,
#20320,#20321,#20322,#20323,#20324,#20325,#20326,#20327,#20328,#20329,#20330,
#20331,#20332,#20333,#20334,#20335,#20336,#20337,#20338,#20339,#20340,#20341,
#20342,#20343,#20344,#20345,#20346,#20347,#20348,#20349,#20350,#20351,#20352,
#20353,#20354,#20355,#20356,#20357,#20358,#20359,#20360,#20361,#20362,#20363,
#20364,#20365,#20366,#20367,#20368),.UNSPECIFIED.,.F.,.F.,(4,3,3,3,3,3,
3,3,3,3,3,3,3,3,3,3,3,3,3,3,3,3,3,3,3,4),(151.891517975085,151.973979578939,
152.056440516909,152.138900816395,152.221360504792,152.303819609494,152.386278157893,
152.46873617738,152.551193695341,152.637871591001,152.720338376837,152.80280349018,
152.885267040686,152.967729137983,153.050189891685,153.132649411382,153.215107806649,
153.297565187046,153.380031573313,153.462494775327,153.544955231607,153.627413380518,
153.709878985397,153.792338864612,153.874802977975,153.938040025901),
 .UNSPECIFIED.);
#201=B_SPLINE_CURVE_WITH_KNOTS('',3,(#20370,#20371,#20372,#20373,#20374,
#20375,#20376,#20377,#20378,#20379,#20380,#20381,#20382,#20383,#20384,#20385,
#20386,#20387,#20388,#20389,#20390,#20391,#20392,#20393,#20394,#20395,#20396,
#20397,#20398,#20399,#20400,#20401,#20402,#20403,#20404,#20405,#20406,#20407,
#20408,#20409,#20410,#20411,#20412,#20413,#20414,#20415,#20416,#20417,#20418,
#20419,#20420,#20421,#20422,#20423,#20424,#20425,#20426,#20427,#20428,#20429,
#20430,#20431,#20432,#20433,#20434,#20435,#20436,#20437,#20438,#20439,#20440,
#20441,#20442,#20443,#20444,#20445,#20446,#20447,#20448,#20449,#20450,#20451),
 .UNSPECIFIED.,.F.,.F.,(4,3,3,3,3,3,3,3,3,3,3,3,3,3,3,3,3,3,3,3,3,3,3,3,
3,3,3,4),(151.891456894454,151.968751236879,152.046065543027,152.123413829604,
152.200852531408,152.27834282066,152.355943247076,152.390561982999,152.467425367651,
152.544195199461,152.620887735449,152.697519170616,152.774105651399,152.850963693856,
152.927522016819,153.004086351492,153.080671264619,153.157745946227,153.234452767096,
153.311711379073,153.38896999105,153.469176480459,153.549273741512,153.629271620513,
153.709148776534,153.788955061789,153.868679826393,153.938040025901),
 .UNSPECIFIED.);
#202=B_SPLINE_CURVE_WITH_KNOTS('',3,(#20452,#20453,#20454,#20455,#20456,
#20457,#20458,#20459,#20460,#20461,#20462,#20463,#20464,#20465,#20466,#20467,
#20468,#20469,#20470,#20471,#20472,#20473,#20474,#20475,#20476,#20477,#20478,
#20479,#20480,#20481,#20482,#20483,#20484,#20485,#20486,#20487,#20488,#20489,
#20490,#20491,#20492,#20493,#20494,#20495,#20496,#20497,#20498,#20499,#20500,
#20501,#20502,#20503,#20504,#20505,#20506,#20507,#20508,#20509,#20510,#20511,
#20512,#20513,#20514,#20515,#20516,#20517,#20518,#20519,#20520,#20521,#20522,
#20523,#20524,#20525,#20526,#20527,#20528,#20529,#20530,#20531,#20532,#20533,
#20534,#20535,#20536,#20537,#20538,#20539,#20540,#20541,#20542,#20543,#20544,
#20545,#20546,#20547,#20548,#20549,#20550,#20551,#20552,#20553,#20554,#20555,
#20556,#20557,#20558,#20559,#20560,#20561,#20562,#20563,#20564,#20565,#20566,
#20567,#20568,#20569,#20570,#20571,#20572,#20573,#20574,#20575,#20576,#20577,
#20578,#20579,#20580,#20581,#20582,#20583,#20584,#20585,#20586,#20587,#20588,
#20589,#20590,#20591,#20592,#20593,#20594,#20595,#20596,#20597,#20598,#20599,
#20600,#20601,#20602,#20603,#20604,#20605,#20606,#20607,#20608,#20609,#20610,
#20611,#20612,#20613,#20614,#20615,#20616,#20617,#20618,#20619,#20620),
 .UNSPECIFIED.,.F.,.F.,(4,3,3,3,3,3,3,3,3,3,3,3,3,3,3,3,3,3,3,3,3,3,3,3,
3,3,3,3,3,3,3,3,3,3,3,3,3,3,3,3,3,3,3,3,3,3,3,3,3,3,3,3,3,3,3,3,4),(153.93804002599,
154.020503748665,154.103125959518,154.185989566382,154.268982219652,154.352171395724,
154.387377999101,154.464908117164,154.54235114648,154.619722728306,154.697038452665,
154.774313869227,154.851574745252,154.928830056598,155.00609384469,155.083380153074,
155.16074701468,155.238155408612,155.315677041484,155.385786007152,155.462622039275,
155.539369055002,155.616043292565,155.692660932086,155.769238108713,155.846107597024,
155.922667699547,155.999237996694,156.075833057717,156.152923297088,156.229650493669,
156.306922254436,156.384194015202,156.461788684636,156.539290950746,156.616716435817,
156.694080707194,156.771399288285,156.848694992756,156.925980037412,157.003268429345,
157.080574174871,157.157952214858,157.235367286603,157.312887900874,157.382602023253,
157.464088337686,157.545470420045,157.629554321854,157.710711640707,157.791792424462,
157.872782416495,157.881806027279,157.962834259542,158.043923776839,158.12512824495,
158.174223456389),.UNSPECIFIED.);
#203=B_SPLINE_CURVE_WITH_KNOTS('',3,(#20626,#20627,#20628,#20629,#20630,
#20631,#20632,#20633,#20634,#20635,#20636,#20637,#20638,#20639,#20640,#20641,
#20642,#20643,#20644,#20645,#20646,#20647,#20648,#20649,#20650,#20651,#20652,
#20653,#20654,#20655,#20656,#20657,#20658,#20659,#20660,#20661,#20662,#20663,
#20664,#20665,#20666,#20667,#20668,#20669,#20670,#20671,#20672,#20673,#20674,
#20675,#20676,#20677,#20678,#20679,#20680,#20681,#20682,#20683,#20684,#20685,
#20686,#20687,#20688,#20689,#20690,#20691,#20692,#20693,#20694,#20695,#20696,
#20697,#20698,#20699,#20700,#20701,#20702,#20703,#20704,#20705,#20706,#20707,
#20708,#20709,#20710,#20711,#20712,#20713,#20714,#20715,#20716,#20717,#20718,
#20719,#20720,#20721,#20722,#20723,#20724,#20725,#20726,#20727,#20728,#20729,
#20730,#20731,#20732,#20733,#20734,#20735,#20736,#20737,#20738,#20739,#20740,
#20741,#20742,#20743,#20744,#20745,#20746,#20747,#20748,#20749,#20750,#20751,
#20752,#20753,#20754,#20755,#20756,#20757,#20758,#20759,#20760,#20761,#20762,
#20763,#20764,#20765,#20766,#20767,#20768,#20769,#20770,#20771,#20772,#20773,
#20774,#20775,#20776,#20777,#20778,#20779,#20780,#20781,#20782),
 .UNSPECIFIED.,.F.,.F.,(4,3,3,3,3,3,3,3,3,3,3,3,3,3,3,3,3,3,3,3,3,3,3,3,
3,3,3,3,3,3,3,3,3,3,3,3,3,3,3,3,3,3,3,3,3,3,3,3,3,3,3,3,4),(160.221293919461,
160.303756125205,160.386217982658,160.46867949867,160.551140680093,160.633601533774,
160.716062066564,160.798522285313,160.880982196868,160.963441808079,161.045901125793,
161.12836015686,161.210818908127,161.293277386441,161.37573559865,161.458193551602,
161.540651252142,161.623108707119,161.705565923378,161.791576006692,161.874898274903,
161.957364879679,162.039830640272,162.122295584098,162.204759738569,162.287223131093,
162.369685789079,162.452147739931,162.53460901105,162.617069629836,162.699529623685,
162.781989019994,162.864447846155,162.946906129559,163.029363897595,163.11182117765,
163.195950390887,163.278416387752,163.360880762961,163.443343626157,163.525805086962,
163.608265254977,163.690724239787,163.773182150959,163.85877045577,163.941235190332,
164.023696960577,164.106156204942,164.188613361723,164.271075876341,164.353533544655,
164.435992328928,164.457888589444),.UNSPECIFIED.);
#204=B_SPLINE_CURVE_WITH_KNOTS('',3,(#20783,#20784,#20785,#20786,#20787,
#20788,#20789,#20790,#20791,#20792,#20793,#20794,#20795,#20796,#20797,#20798,
#20799,#20800,#20801,#20802,#20803,#20804,#20805,#20806,#20807,#20808,#20809,
#20810,#20811,#20812,#20813,#20814,#20815,#20816,#20817,#20818,#20819,#20820,
#20821,#20822,#20823,#20824,#20825,#20826,#20827,#20828,#20829,#20830,#20831,
#20832,#20833,#20834,#20835,#20836,#20837,#20838,#20839,#20840,#20841,#20842,
#20843,#20844,#20845,#20846,#20847,#20848,#20849,#20850,#20851,#20852,#20853,
#20854,#20855,#20856,#20857,#20858,#20859,#20860,#20861,#20862,#20863,#20864,
#20865,#20866,#20867),.UNSPECIFIED.,.F.,.F.,(4,3,3,3,3,3,3,3,3,3,3,3,3,
3,3,3,3,3,3,3,3,3,3,3,3,3,3,3,4),(158.174289778564,158.25182298141,158.264170960032,
158.341688329228,158.419118396679,158.496476817949,158.573779197164,158.651041097927,
158.728288308618,158.805529832837,158.882779724183,158.960052038326,159.037405109552,
159.114799639304,159.192308144266,159.263924571402,159.340232490144,159.416451593538,
159.492598491568,159.568689727161,159.644741792255,159.720782406705,159.796820324337,
159.872870430293,159.948947616582,160.025109268506,160.101317979426,160.177636942526,
160.220785774833),.UNSPECIFIED.);
#205=B_SPLINE_CURVE_WITH_KNOTS('',3,(#20869,#20870,#20871,#20872,#20873,
#20874,#20875,#20876,#20877,#20878,#20879,#20880,#20881,#20882,#20883,#20884,
#20885,#20886,#20887,#20888,#20889,#20890,#20891,#20892,#20893,#20894,#20895,
#20896,#20897,#20898,#20899,#20900,#20901,#20902,#20903,#20904,#20905,#20906,
#20907,#20908,#20909,#20910,#20911,#20912,#20913,#20914,#20915,#20916,#20917,
#20918,#20919,#20920,#20921,#20922,#20923,#20924,#20925,#20926,#20927,#20928,
#20929,#20930,#20931,#20932,#20933,#20934,#20935,#20936,#20937,#20938,#20939,
#20940,#20941,#20942,#20943,#20944,#20945,#20946,#20947,#20948,#20949,#20950),
 .UNSPECIFIED.,.F.,.F.,(4,3,3,3,3,3,3,3,3,3,3,3,3,3,3,3,3,3,3,3,3,3,3,3,
3,3,3,4),(158.174223456389,158.255576040659,158.337061991695,158.381010031304,
158.458538184513,158.535985059474,158.613366238182,158.690697255642,158.767993610473,
158.845283910809,158.922573818547,158.999877340545,159.077208488672,159.154627978493,
159.232093336915,159.309678723213,159.379418039355,159.455165032216,159.530819705694,
159.606399033243,159.683142945243,159.758622758066,159.834082616388,159.909537686717,
159.987240847348,160.062760807305,160.141555568273,160.220350329241),
 .UNSPECIFIED.);
#206=B_SPLINE_CURVE_WITH_KNOTS('',3,(#20951,#20952,#20953,#20954,#20955,
#20956,#20957,#20958,#20959,#20960,#20961,#20962,#20963,#20964,#20965,#20966,
#20967,#20968,#20969,#20970,#20971,#20972,#20973,#20974,#20975,#20976,#20977,
#20978,#20979,#20980,#20981,#20982,#20983,#20984,#20985,#20986,#20987,#20988,
#20989,#20990,#20991,#20992,#20993,#20994,#20995,#20996,#20997,#20998,#20999,
#21000,#21001,#21002,#21003,#21004,#21005,#21006,#21007,#21008,#21009,#21010,
#21011,#21012,#21013,#21014,#21015,#21016,#21017,#21018,#21019,#21020,#21021,
#21022,#21023,#21024,#21025,#21026,#21027,#21028,#21029,#21030,#21031,#21032,
#21033,#21034,#21035,#21036,#21037,#21038,#21039,#21040,#21041,#21042,#21043,
#21044,#21045,#21046,#21047,#21048,#21049,#21050,#21051,#21052,#21053,#21054,
#21055,#21056,#21057,#21058,#21059,#21060,#21061,#21062,#21063,#21064,#21065,
#21066,#21067,#21068,#21069,#21070,#21071,#21072,#21073,#21074,#21075,#21076,
#21077,#21078,#21079,#21080,#21081,#21082,#21083,#21084,#21085,#21086,#21087,
#21088,#21089,#21090,#21091,#21092,#21093,#21094,#21095,#21096,#21097,#21098,
#21099,#21100,#21101,#21102,#21103,#21104,#21105,#21106,#21107),
 .UNSPECIFIED.,.F.,.F.,(4,3,3,3,3,3,3,3,3,3,3,3,3,3,3,3,3,3,3,3,3,3,3,3,
3,3,3,3,3,3,3,3,3,3,3,3,3,3,3,3,3,3,3,3,3,3,3,3,3,3,3,3,4),(160.22122533308,
160.303687539116,160.386149396856,160.46861091315,160.551072094847,160.633532948798,
160.715993481853,160.798453700859,160.880913612667,160.963373224125,161.045832542081,
161.128291573383,161.21075032488,161.293208803418,161.375667015846,161.45812496901,
161.540582669758,161.623040124936,161.70549734139,161.791509567892,161.874833912315,
161.957300517761,162.039766279002,162.122231223455,162.204695378531,162.28715877164,
162.369621430188,162.452083381581,162.53454465322,162.617005272504,162.699465266831,
162.781924663595,162.86438349019,162.946841774007,163.029299542434,163.11175682286,
163.195890058271,163.278356056363,163.360820432718,163.443283296981,163.525744758771,
163.608204927692,163.690663913328,163.773121825245,163.85871767077,163.94118240737,
164.023644179372,164.106103425214,164.188560583191,164.271023101472,164.353480772327,
164.435939562278,164.457888589444),.UNSPECIFIED.);
#207=B_SPLINE_CURVE_WITH_KNOTS('',3,(#21113,#21114,#21115,#21116,#21117,
#21118,#21119,#21120,#21121,#21122,#21123,#21124,#21125,#21126,#21127,#21128,
#21129,#21130,#21131,#21132,#21133,#21134,#21135,#21136,#21137,#21138,#21139,
#21140,#21141,#21142,#21143,#21144,#21145,#21146,#21147,#21148,#21149,#21150,
#21151,#21152,#21153,#21154,#21155,#21156,#21157,#21158,#21159,#21160,#21161,
#21162,#21163,#21164,#21165,#21166,#21167,#21168,#21169,#21170,#21171,#21172,
#21173,#21174,#21175,#21176,#21177,#21178,#21179,#21180,#21181,#21182,#21183,
#21184,#21185,#21186,#21187,#21188,#21189,#21190,#21191,#21192,#21193,#21194,
#21195,#21196,#21197,#21198,#21199,#21200,#21201,#21202,#21203,#21204,#21205,
#21206,#21207,#21208,#21209,#21210,#21211,#21212,#21213,#21214,#21215,#21216,
#21217,#21218,#21219,#21220,#21221,#21222,#21223,#21224,#21225,#21226,#21227,
#21228,#21229,#21230,#21231,#21232,#21233,#21234,#21235,#21236,#21237,#21238,
#21239,#21240,#21241,#21242,#21243,#21244,#21245,#21246,#21247,#21248,#21249,
#21250,#21251,#21252,#21253,#21254,#21255,#21256,#21257,#21258,#21259,#21260,
#21261,#21262,#21263,#21264,#21265,#21266,#21267,#21268,#21269),
 .UNSPECIFIED.,.F.,.F.,(4,3,3,3,3,3,3,3,3,3,3,3,3,3,3,3,3,3,3,3,3,3,3,3,
3,3,3,3,3,3,3,3,3,3,3,3,3,3,3,3,3,3,3,3,3,3,3,3,3,3,3,3,4),(166.50441064026,
166.586872846296,166.669334704036,166.75179622033,166.834257402027,166.916718255978,
166.999178789033,167.081639008039,167.164098919847,167.246558531305,167.329017849261,
167.411476880563,167.49393563206,167.576394110598,167.658852323026,167.741310276191,
167.823767976939,167.906225432117,167.988682648571,168.074694875073,168.158019219496,
168.240485824942,168.322951586183,168.405416530636,168.487880685712,168.570344078821,
168.652806737369,168.735268688762,168.817729960401,168.900190579685,168.982650574012,
169.065109970776,169.147568797371,169.230027081188,169.312484849615,169.394942130041,
169.479075365452,169.561541363544,169.644005739899,169.726468604162,169.808930065952,
169.891390234873,169.973849220509,170.056307132426,170.141902977951,170.224367714551,
170.306829486553,170.389288732395,170.471745890372,170.554208408653,170.636666079508,
170.719124869459,170.741073896624),.UNSPECIFIED.);
#208=B_SPLINE_CURVE_WITH_KNOTS('',3,(#21270,#21271,#21272,#21273,#21274,
#21275,#21276,#21277,#21278,#21279,#21280,#21281,#21282,#21283,#21284,#21285,
#21286,#21287,#21288,#21289,#21290,#21291,#21292,#21293,#21294,#21295,#21296,
#21297,#21298,#21299,#21300,#21301,#21302,#21303,#21304,#21305,#21306,#21307,
#21308,#21309,#21310,#21311,#21312,#21313,#21314,#21315,#21316,#21317,#21318,
#21319,#21320,#21321,#21322,#21323,#21324,#21325,#21326,#21327,#21328,#21329,
#21330,#21331,#21332,#21333,#21334,#21335,#21336,#21337,#21338,#21339,#21340,
#21341,#21342,#21343,#21344,#21345),.UNSPECIFIED.,.F.,.F.,(4,3,3,3,3,3,
3,3,3,3,3,3,3,3,3,3,3,3,3,3,3,3,3,3,3,4),(164.457888589444,164.540350193298,
164.622811131269,164.705271430754,164.787731119151,164.870190223853,164.952648772253,
165.035106791739,165.1175643097,165.204242205355,165.28670899119,165.369174104534,
165.451637655039,165.534099752337,165.616560506038,165.699020025736,165.781478421003,
165.8639358014,165.946402187667,166.028865389681,166.111325845961,166.193783994872,
166.276249599751,166.358709478965,166.441173592329,166.50441064017),
 .UNSPECIFIED.);
#209=B_SPLINE_CURVE_WITH_KNOTS('',3,(#21347,#21348,#21349,#21350,#21351,
#21352,#21353,#21354,#21355,#21356,#21357,#21358,#21359,#21360,#21361,#21362,
#21363,#21364,#21365,#21366,#21367,#21368,#21369,#21370,#21371,#21372,#21373,
#21374,#21375,#21376,#21377,#21378,#21379,#21380,#21381,#21382,#21383,#21384,
#21385,#21386,#21387,#21388,#21389,#21390,#21391,#21392,#21393,#21394,#21395,
#21396,#21397,#21398,#21399,#21400,#21401,#21402,#21403,#21404,#21405,#21406,
#21407,#21408,#21409,#21410,#21411,#21412,#21413,#21414,#21415,#21416,#21417,
#21418,#21419,#21420,#21421,#21422),.UNSPECIFIED.,.F.,.F.,(4,3,3,3,3,3,
3,3,3,3,3,3,3,3,3,3,3,3,3,3,3,3,3,3,3,4),(164.457888589444,164.540350193298,
164.622811131268,164.705271430754,164.787731119151,164.870190223853,164.952648772252,
165.035106791738,165.1175643097,165.20424220536,165.286708991196,165.369174104539,
165.451637655044,165.534099752342,165.616560506044,165.699020025741,165.781478421009,
165.863935801406,165.946402187672,166.028865389686,166.111325845966,166.193783994877,
166.276249599756,166.358709478971,166.441173592335,166.50441064026),
 .UNSPECIFIED.);
#210=B_SPLINE_CURVE_WITH_KNOTS('',3,(#21423,#21424,#21425,#21426,#21427,
#21428,#21429,#21430,#21431,#21432,#21433,#21434,#21435,#21436,#21437,#21438,
#21439,#21440,#21441,#21442,#21443,#21444,#21445,#21446,#21447,#21448,#21449,
#21450,#21451,#21452,#21453,#21454,#21455,#21456,#21457,#21458,#21459,#21460,
#21461,#21462,#21463,#21464,#21465,#21466,#21467,#21468,#21469,#21470,#21471,
#21472,#21473,#21474,#21475,#21476,#21477,#21478,#21479,#21480,#21481,#21482,
#21483,#21484,#21485,#21486,#21487,#21488,#21489,#21490,#21491,#21492,#21493,
#21494,#21495,#21496,#21497,#21498,#21499,#21500,#21501,#21502,#21503,#21504,
#21505,#21506,#21507,#21508,#21509,#21510,#21511,#21512,#21513,#21514,#21515,
#21516,#21517,#21518,#21519,#21520,#21521,#21522,#21523,#21524,#21525,#21526,
#21527,#21528,#21529,#21530,#21531,#21532,#21533,#21534,#21535,#21536,#21537,
#21538,#21539,#21540,#21541,#21542,#21543,#21544,#21545,#21546,#21547,#21548,
#21549,#21550,#21551,#21552,#21553,#21554,#21555,#21556,#21557,#21558,#21559,
#21560,#21561,#21562,#21563,#21564,#21565,#21566,#21567,#21568,#21569,#21570,
#21571,#21572,#21573,#21574,#21575,#21576,#21577,#21578,#21579,#21580,#21581,
#21582,#21583,#21584,#21585,#21586,#21587,#21588,#21589,#21590,#21591),
 .UNSPECIFIED.,.F.,.F.,(4,3,3,3,3,3,3,3,3,3,3,3,3,3,3,3,3,3,3,3,3,3,3,3,
3,3,3,3,3,3,3,3,3,3,3,3,3,3,3,3,3,3,3,3,3,3,3,3,3,3,3,3,3,3,3,3,4),(166.50541292827,
166.581074695536,166.656660402689,166.732186932408,166.811498828828,166.886966429492,
166.962429663997,167.037903691478,167.113403679882,167.188983704042,167.264610390849,
167.34033877611,167.366682103763,167.444212300223,167.521655394828,167.599027028884,
167.676342792453,167.753618235231,167.83087911765,167.908134423295,167.985398193589,
168.062684472073,168.140051284865,168.217459619572,168.294981176135,168.365090111813,
168.442620229876,168.520063259192,168.597434841018,168.674750565378,168.752025981939,
168.829286857964,168.90654216931,168.983805957402,169.061092265786,169.138459127392,
169.215867521324,169.293389154196,169.363498119864,169.440334151987,169.517081167714,
169.593755405277,169.670373044799,169.746950221425,169.823819709737,169.900379812259,
169.976950109407,170.053545170429,170.130635409801,170.207362606382,170.284634367149,
170.361906127915,170.439515156729,170.517006394961,170.594430128243,170.671788667788,
170.74144325617),.UNSPECIFIED.);
#211=B_SPLINE_CURVE_WITH_KNOTS('',3,(#21597,#21598,#21599,#21600,#21601,
#21602,#21603,#21604,#21605,#21606,#21607,#21608,#21609,#21610,#21611,#21612,
#21613,#21614,#21615,#21616,#21617,#21618,#21619,#21620,#21621,#21622,#21623,
#21624,#21625,#21626,#21627,#21628,#21629,#21630,#21631,#21632,#21633,#21634,
#21635,#21636,#21637,#21638,#21639,#21640,#21641,#21642,#21643,#21644,#21645,
#21646,#21647,#21648,#21649,#21650,#21651,#21652,#21653,#21654,#21655,#21656,
#21657,#21658,#21659,#21660,#21661,#21662,#21663,#21664,#21665,#21666,#21667,
#21668,#21669,#21670,#21671,#21672,#21673,#21674,#21675,#21676,#21677,#21678,
#21679,#21680,#21681,#21682,#21683,#21684,#21685,#21686,#21687,#21688,#21689,
#21690,#21691,#21692,#21693,#21694,#21695,#21696,#21697,#21698,#21699,#21700,
#21701,#21702,#21703,#21704,#21705,#21706,#21707,#21708,#21709,#21710,#21711,
#21712,#21713,#21714,#21715,#21716,#21717,#21718,#21719,#21720,#21721,#21722,
#21723,#21724,#21725,#21726,#21727,#21728,#21729,#21730,#21731,#21732,#21733,
#21734,#21735,#21736,#21737,#21738,#21739,#21740,#21741,#21742,#21743,#21744,
#21745,#21746,#21747,#21748,#21749,#21750,#21751,#21752,#21753,#21754,#21755,
#21756,#21757,#21758,#21759,#21760,#21761,#21762,#21763,#21764,#21765),
 .UNSPECIFIED.,.F.,.F.,(4,3,3,3,3,3,3,3,3,3,3,3,3,3,3,3,3,3,3,3,3,3,3,3,
3,3,3,3,3,3,3,3,3,3,3,3,3,3,3,3,3,3,3,3,3,3,3,3,3,3,3,3,3,3,3,3,4),(172.78759594744,
172.86986216778,172.952274762003,173.034920623703,173.117686797904,173.200653382848,
173.260475130573,173.337296327728,173.414028289942,173.49068726809,173.567289454552,
173.643850996432,173.720898214621,173.797442389266,173.873996669311,173.950575634291,
174.027988911204,174.104700391511,174.182464566726,174.260228741942,174.337811365556,
174.415301347765,174.49271432499,174.570065878491,174.647371545402,174.724654138447,
174.801925925391,174.879200925247,174.956493156185,175.03385782855,175.111259436983,
175.188767251591,175.259982353312,175.341466326267,175.422845690407,175.507099057554,
175.588252552726,175.669329230685,175.750314658476,175.759859158996,175.8408675549,
175.921951811731,176.006397849968,176.087703931675,176.169087721443,176.250592382472,
176.259735964681,176.337263655425,176.414707268943,176.492069608677,176.569385657828,
176.646669470485,176.723935079898,176.801217331499,176.87850613038,176.95584990749,
177.023722386416),.UNSPECIFIED.);
#212=B_SPLINE_CURVE_WITH_KNOTS('',3,(#21766,#21767,#21768,#21769,#21770,
#21771,#21772,#21773,#21774,#21775,#21776,#21777,#21778,#21779,#21780,#21781,
#21782,#21783,#21784,#21785,#21786,#21787,#21788,#21789,#21790,#21791,#21792,
#21793,#21794,#21795,#21796,#21797,#21798,#21799,#21800,#21801,#21802,#21803,
#21804,#21805,#21806,#21807,#21808,#21809,#21810,#21811,#21812,#21813,#21814,
#21815,#21816,#21817,#21818,#21819,#21820,#21821,#21822,#21823,#21824,#21825,
#21826,#21827,#21828,#21829,#21830,#21831,#21832,#21833,#21834,#21835,#21836,
#21837,#21838,#21839,#21840,#21841),.UNSPECIFIED.,.F.,.F.,(4,3,3,3,3,3,
3,3,3,3,3,3,3,3,3,3,3,3,3,3,3,3,3,3,3,4),(170.741073896624,170.823535500478,
170.905996438448,170.988456737934,171.070916426331,171.153375531033,171.235834079432,
171.318292098918,171.40074961688,171.48742751254,171.569894298376,171.652359411719,
171.734822962225,171.817285059522,171.899745813224,171.982205332921,172.064663728188,
172.147121108585,172.229587494852,172.312050696865,172.394511153146,172.476969302057,
172.559434906936,172.641894786151,172.724358899514,172.78759594744),
 .UNSPECIFIED.);
#213=B_SPLINE_CURVE_WITH_KNOTS('',3,(#21843,#21844,#21845,#21846,#21847,
#21848,#21849,#21850,#21851,#21852,#21853,#21854,#21855,#21856,#21857,#21858,
#21859,#21860,#21861,#21862,#21863,#21864,#21865,#21866,#21867,#21868,#21869,
#21870,#21871,#21872,#21873,#21874,#21875,#21876,#21877,#21878,#21879,#21880,
#21881,#21882,#21883,#21884,#21885,#21886,#21887,#21888,#21889,#21890,#21891,
#21892,#21893,#21894,#21895,#21896,#21897,#21898,#21899,#21900,#21901,#21902,
#21903,#21904,#21905,#21906,#21907,#21908,#21909,#21910,#21911,#21912,#21913,
#21914,#21915,#21916,#21917,#21918,#21919,#21920,#21921,#21922,#21923,#21924,
#21925,#21926,#21927),.UNSPECIFIED.,.F.,.F.,(4,3,3,3,3,3,3,3,3,3,3,3,3,
3,3,3,3,3,3,3,3,3,3,3,3,3,3,3,4),(170.74144325617,170.818802116145,170.896087588298,
170.973375029628,171.050678446185,171.12808736863,171.205498258243,171.283016619449,
171.360314135966,171.441800450399,171.523182532758,171.607266434566,171.688423753419,
171.769504537174,171.850494529207,171.859518139992,171.940531246283,172.021619940555,
172.105895491421,172.187204957811,172.268591859021,172.350098997786,172.358722144017,
172.44182853159,172.528270385522,172.61101135579,172.693618768605,172.776046178395,
172.787595947318),.UNSPECIFIED.);
#214=B_SPLINE_CURVE_WITH_KNOTS('',3,(#21928,#21929,#21930,#21931,#21932,
#21933,#21934,#21935,#21936,#21937,#21938,#21939,#21940,#21941,#21942,#21943,
#21944,#21945,#21946,#21947,#21948,#21949,#21950,#21951,#21952,#21953,#21954,
#21955,#21956,#21957,#21958,#21959,#21960,#21961,#21962,#21963,#21964,#21965,
#21966,#21967,#21968,#21969,#21970,#21971,#21972,#21973,#21974,#21975,#21976,
#21977,#21978,#21979,#21980,#21981,#21982,#21983,#21984,#21985,#21986,#21987,
#21988,#21989,#21990,#21991,#21992,#21993,#21994,#21995,#21996,#21997,#21998,
#21999,#22000,#22001,#22002,#22003,#22004,#22005,#22006,#22007,#22008,#22009,
#22010,#22011,#22012,#22013,#22014,#22015,#22016,#22017,#22018,#22019,#22020,
#22021,#22022,#22023,#22024,#22025,#22026,#22027,#22028,#22029,#22030,#22031,
#22032,#22033,#22034,#22035,#22036,#22037,#22038,#22039,#22040,#22041,#22042,
#22043,#22044,#22045,#22046,#22047,#22048,#22049,#22050,#22051,#22052,#22053,
#22054,#22055,#22056,#22057,#22058,#22059,#22060,#22061,#22062,#22063,#22064,
#22065,#22066,#22067,#22068,#22069,#22070,#22071,#22072,#22073,#22074,#22075,
#22076,#22077,#22078,#22079,#22080,#22081,#22082,#22083,#22084,#22085,#22086,
#22087,#22088,#22089,#22090,#22091,#22092,#22093),.UNSPECIFIED.,.F.,.F.,
(4,3,3,3,3,3,3,3,3,3,3,3,3,3,3,3,3,3,3,3,3,3,3,3,3,3,3,3,3,3,3,3,3,3,3,
3,3,3,3,3,3,3,3,3,3,3,3,3,3,3,3,3,3,3,3,4),(172.78759594744,172.867358168951,
172.947180515715,173.027072473787,173.109586893358,173.189701149854,173.273415650961,
173.357130152068,173.43399353672,173.51076336853,173.587455904518,173.664087339685,
173.740673820468,173.817531862925,173.894090185888,173.97065452056,174.047239433687,
174.124314115295,174.201020936164,174.278279548142,174.355538160119,174.433068356579,
174.510511451184,174.58788308524,174.665198848809,174.742474291587,174.819735174007,
174.896990479651,174.974254249945,175.05154052843,175.128907341222,175.206315675929,
175.283837232491,175.35394616817,175.431476286233,175.508919315549,175.586290897375,
175.663606621735,175.740882038296,175.818142914321,175.895398225668,175.972662013759,
176.049948322143,176.127315183749,176.204723577681,176.282245210553,176.352354176221,
176.42920941739,176.50594720523,176.582616756367,176.659232722429,176.735809718978,
176.812371831209,176.888923699021,176.965501877551,177.023545810813),
 .UNSPECIFIED.);
#215=B_SPLINE_CURVE_WITH_KNOTS('',3,(#22099,#22100,#22101,#22102,#22103,
#22104,#22105,#22106,#22107,#22108,#22109,#22110,#22111,#22112,#22113,#22114,
#22115,#22116,#22117,#22118,#22119,#22120,#22121,#22122,#22123,#22124,#22125,
#22126,#22127,#22128,#22129,#22130,#22131,#22132,#22133,#22134,#22135,#22136,
#22137,#22138,#22139,#22140,#22141,#22142,#22143,#22144,#22145,#22146,#22147,
#22148,#22149,#22150,#22151,#22152,#22153,#22154,#22155,#22156,#22157,#22158,
#22159,#22160,#22161,#22162,#22163,#22164,#22165,#22166,#22167,#22168,#22169,
#22170,#22171,#22172,#22173,#22174,#22175,#22176,#22177,#22178,#22179,#22180,
#22181,#22182,#22183,#22184,#22185,#22186,#22187,#22188,#22189,#22190,#22191,
#22192,#22193,#22194,#22195,#22196,#22197,#22198,#22199,#22200,#22201,#22202,
#22203,#22204,#22205,#22206,#22207,#22208,#22209,#22210,#22211,#22212,#22213,
#22214,#22215,#22216,#22217,#22218,#22219,#22220,#22221,#22222,#22223,#22224,
#22225,#22226,#22227,#22228,#22229,#22230,#22231,#22232,#22233,#22234,#22235,
#22236,#22237,#22238,#22239,#22240,#22241,#22242,#22243,#22244,#22245,#22246,
#22247,#22248,#22249,#22250,#22251,#22252,#22253,#22254,#22255,#22256,#22257,
#22258,#22259,#22260,#22261,#22262,#22263,#22264,#22265,#22266,#22267),
 .UNSPECIFIED.,.F.,.F.,(4,3,3,3,3,3,3,3,3,3,3,3,3,3,3,3,3,3,3,3,3,3,3,3,
3,3,3,3,3,3,3,3,3,3,3,3,3,3,3,3,3,3,3,3,3,3,3,3,3,3,3,3,3,3,3,3,4),(179.070781254619,
179.183730485173,179.258996798789,179.336514167985,179.413944235437,179.491302656706,
179.568605035921,179.645866936684,179.723114147375,179.800355671594,179.87760556294,
179.954877877083,180.032230948309,180.109625478061,180.187133983023,180.258750410158,
180.335571607313,180.412303569527,180.488962547675,180.565564734136,180.642126276017,
180.719173494206,180.79571766885,180.872271948896,180.948850913875,181.026264190788,
181.102975671095,181.180739846312,181.258504021528,181.336086645142,181.413576627351,
181.490989604576,181.568341158077,181.645646824989,181.722929418034,181.800201204978,
181.877476204834,181.954768435773,182.032133108138,182.10953471657,182.187042531178,
182.258257632897,182.339741605852,182.421120969991,182.505374337139,182.58652783231,
182.667604510269,182.748589938059,182.758134438582,182.839142834486,182.920227091318,
183.004673129555,183.085979211262,183.167363001031,183.24886766206,183.258011244266,
183.307783619138),.UNSPECIFIED.);
#216=B_SPLINE_CURVE_WITH_KNOTS('',3,(#22268,#22269,#22270,#22271,#22272,
#22273,#22274,#22275,#22276,#22277,#22278,#22279,#22280,#22281,#22282,#22283,
#22284,#22285,#22286,#22287,#22288,#22289,#22290,#22291,#22292,#22293,#22294,
#22295,#22296,#22297,#22298,#22299,#22300,#22301,#22302,#22303,#22304,#22305,
#22306,#22307,#22308,#22309,#22310,#22311,#22312,#22313,#22314,#22315,#22316,
#22317,#22318,#22319,#22320,#22321,#22322,#22323,#22324,#22325,#22326,#22327,
#22328,#22329,#22330,#22331,#22332,#22333,#22334,#22335,#22336,#22337,#22338,
#22339,#22340,#22341,#22342,#22343,#22344,#22345,#22346,#22347,#22348,#22349),
 .UNSPECIFIED.,.F.,.F.,(4,3,3,3,3,3,3,3,3,3,3,3,3,3,3,3,3,3,3,3,3,3,3,3,
3,3,3,4),(177.023722386416,177.101168095,177.180328835525,177.25948957605,
177.336338199237,177.413093045634,177.489770385039,177.566386424814,177.642957323439,
177.719993056436,177.796535475142,177.873083811704,177.949652643152,178.027050279219,
178.103741360172,178.181492273796,178.25924318742,178.335709385331,178.412087926232,
178.488395345374,178.564643301564,178.640858774118,178.717056604626,178.793251620891,
178.869486590712,178.945742773932,179.022071940622,179.070781254518),
 .UNSPECIFIED.);
#217=B_SPLINE_CURVE_WITH_KNOTS('',3,(#22351,#22352,#22353,#22354,#22355,
#22356,#22357,#22358,#22359,#22360,#22361,#22362,#22363,#22364,#22365,#22366,
#22367,#22368,#22369,#22370,#22371,#22372,#22373,#22374,#22375,#22376,#22377,
#22378,#22379,#22380,#22381,#22382,#22383,#22384,#22385,#22386,#22387,#22388,
#22389,#22390,#22391,#22392,#22393,#22394,#22395,#22396,#22397,#22398,#22399,
#22400,#22401,#22402,#22403,#22404,#22405,#22406,#22407,#22408,#22409,#22410,
#22411,#22412,#22413,#22414,#22415,#22416,#22417,#22418,#22419,#22420,#22421,
#22422,#22423,#22424,#22425,#22426,#22427,#22428,#22429,#22430,#22431,#22432,
#22433,#22434,#22435),.UNSPECIFIED.,.F.,.F.,(4,3,3,3,3,3,3,3,3,3,3,3,3,
3,3,3,3,3,3,3,3,3,3,3,3,3,3,3,4),(177.023545810813,177.100169179658,177.176883966167,
177.253652922408,177.330529681703,177.350762184272,177.428356853706,177.505859119816,
177.583284604887,177.660648876263,177.737967457355,177.815263161827,177.892548206483,
177.969836598416,178.047142343942,178.124520383929,178.201935455673,178.279456069945,
178.349170192323,178.430656506756,178.512038589115,178.596122490923,178.677279809776,
178.758360593529,178.839350585564,178.848374196348,178.922846731534,178.997365107791,
179.070781254619),.UNSPECIFIED.);
#218=B_SPLINE_CURVE_WITH_KNOTS('',3,(#22436,#22437,#22438,#22439,#22440,
#22441,#22442,#22443,#22444,#22445,#22446,#22447,#22448,#22449,#22450,#22451,
#22452,#22453,#22454,#22455,#22456,#22457,#22458,#22459,#22460,#22461,#22462,
#22463,#22464,#22465,#22466,#22467,#22468,#22469,#22470,#22471,#22472,#22473,
#22474,#22475,#22476,#22477,#22478,#22479,#22480,#22481,#22482,#22483,#22484,
#22485,#22486,#22487,#22488,#22489,#22490,#22491,#22492,#22493,#22494,#22495,
#22496,#22497,#22498,#22499,#22500,#22501,#22502,#22503,#22504,#22505,#22506,
#22507,#22508,#22509,#22510,#22511,#22512,#22513,#22514,#22515,#22516,#22517,
#22518,#22519,#22520,#22521,#22522,#22523,#22524,#22525,#22526,#22527,#22528,
#22529,#22530,#22531,#22532,#22533,#22534,#22535,#22536,#22537,#22538,#22539,
#22540,#22541,#22542,#22543,#22544,#22545,#22546,#22547,#22548,#22549,#22550,
#22551,#22552,#22553,#22554,#22555,#22556,#22557,#22558,#22559,#22560,#22561,
#22562,#22563,#22564,#22565,#22566,#22567,#22568,#22569,#22570,#22571,#22572,
#22573,#22574,#22575,#22576,#22577,#22578,#22579,#22580,#22581,#22582,#22583,
#22584,#22585,#22586,#22587,#22588,#22589,#22590,#22591,#22592,#22593,#22594,
#22595,#22596,#22597,#22598,#22599,#22600,#22601),.UNSPECIFIED.,.F.,.F.,
(4,3,3,3,3,3,3,3,3,3,3,3,3,3,3,3,3,3,3,3,3,3,3,3,3,3,3,3,3,3,3,3,3,3,3,
3,3,3,3,3,3,3,3,3,3,3,3,3,3,3,3,3,3,3,3,4),(179.070781254733,179.163109084924,
179.256222027202,179.347578200374,179.425106353583,179.502553228544,179.579934407252,
179.657265424712,179.734561779543,179.811852079879,179.889141987617,179.966445509615,
180.043776657743,180.121196147563,180.198661505985,180.276246892283,180.345986208424,
180.422849593076,180.499619424886,180.576311960874,180.652943396041,180.729529876824,
180.806387919281,180.882946242244,180.959510576916,181.036095490044,181.113170171652,
181.18987699252,181.267135604498,181.344394216475,181.421924412935,181.49936750754,
181.576739141596,181.654054905165,181.731330347943,181.808591230363,181.885846536007,
181.963110306301,182.040396584786,182.117763397578,182.195171732285,182.272693288848,
182.342802224526,182.420334076243,182.497778465331,182.575151034455,182.652467374736,
182.729743036649,182.807002031298,182.884254933068,182.961515782812,183.038798623121,
183.116154358625,183.193551410602,183.271044226858,183.307393789556),
 .UNSPECIFIED.);
#219=B_SPLINE_CURVE_WITH_KNOTS('',3,(#22607,#22608,#22609,#22610,#22611,
#22612,#22613,#22614,#22615,#22616,#22617,#22618,#22619,#22620,#22621,#22622,
#22623,#22624,#22625,#22626,#22627,#22628,#22629,#22630,#22631,#22632,#22633,
#22634,#22635,#22636,#22637,#22638,#22639,#22640,#22641,#22642,#22643,#22644,
#22645,#22646,#22647,#22648,#22649,#22650,#22651,#22652,#22653,#22654,#22655,
#22656,#22657,#22658,#22659,#22660,#22661,#22662,#22663,#22664,#22665,#22666,
#22667,#22668,#22669,#22670,#22671,#22672,#22673,#22674,#22675,#22676,#22677,
#22678,#22679,#22680,#22681,#22682,#22683,#22684,#22685,#22686,#22687,#22688,
#22689,#22690,#22691,#22692,#22693,#22694,#22695,#22696,#22697,#22698,#22699,
#22700,#22701,#22702,#22703,#22704,#22705,#22706,#22707,#22708,#22709,#22710,
#22711,#22712,#22713,#22714,#22715,#22716,#22717,#22718,#22719,#22720,#22721,
#22722,#22723,#22724,#22725,#22726,#22727,#22728,#22729,#22730,#22731,#22732,
#22733,#22734,#22735,#22736,#22737,#22738,#22739,#22740,#22741,#22742,#22743,
#22744,#22745,#22746,#22747,#22748,#22749,#22750,#22751,#22752,#22753,#22754,
#22755,#22756,#22757,#22758,#22759,#22760,#22761,#22762,#22763,#22764,#22765,
#22766,#22767,#22768,#22769,#22770,#22771,#22772),.UNSPECIFIED.,.F.,.F.,
(4,3,3,3,3,3,3,3,3,3,3,3,3,3,3,3,3,3,3,3,3,3,3,3,3,3,3,3,3,3,3,3,3,3,3,
3,3,3,3,3,3,3,3,3,3,3,3,3,3,3,3,3,3,3,3,4),(185.353966561943,185.430445028092,
185.506843351555,185.583177999209,185.659465382457,185.735729770735,185.811983844163,
185.888242397231,185.964520225521,186.040874639006,186.117269092864,186.193773470763,
186.257272078375,186.334789447571,186.412219515022,186.489577936292,186.566880315507,
186.64414221627,186.721389426961,186.798630951179,186.875880842525,186.953153156669,
187.030506227895,187.107900757646,187.185409262608,187.257025689744,187.333846886899,
187.410578849113,187.487237827261,187.563840013722,187.640401555603,187.717448773792,
187.793992948436,187.870547228482,187.947126193461,188.024539470374,188.101250950681,
188.179015125897,188.256779301113,188.334361924727,188.411851906936,188.489264884161,
188.566616437662,188.643922104574,188.721204697618,188.798476484562,188.875751484419,
188.953043715357,189.030408387722,189.107809996154,189.185317810762,189.256532912483,
189.340169471562,189.421534418449,189.506306783624,189.591079148798),
 .UNSPECIFIED.);
#220=B_SPLINE_CURVE_WITH_KNOTS('',3,(#22773,#22774,#22775,#22776,#22777,
#22778,#22779,#22780,#22781,#22782,#22783,#22784,#22785,#22786,#22787,#22788,
#22789,#22790,#22791,#22792,#22793,#22794,#22795,#22796,#22797,#22798,#22799,
#22800,#22801,#22802,#22803,#22804,#22805,#22806,#22807,#22808,#22809,#22810,
#22811,#22812,#22813,#22814,#22815,#22816,#22817,#22818,#22819,#22820,#22821,
#22822,#22823,#22824,#22825,#22826,#22827,#22828,#22829,#22830,#22831,#22832,
#22833,#22834,#22835,#22836,#22837,#22838,#22839,#22840,#22841,#22842,#22843,
#22844,#22845,#22846,#22847,#22848,#22849,#22850,#22851,#22852,#22853,#22854),
 .UNSPECIFIED.,.F.,.F.,(4,3,3,3,3,3,3,3,3,3,3,3,3,3,3,3,3,3,3,3,3,3,3,3,
3,3,3,4),(183.307783619138,183.385245296581,183.462635514118,183.539969836095,
183.617263786572,183.697326420205,183.774601632708,183.851885846054,183.929193081493,
184.006537370534,184.083973232362,184.161463460977,184.239059834349,184.257764855636,
184.334613478824,184.41136832522,184.488045664625,184.5646617044,184.641232603025,
184.718268336023,184.794810754728,184.871359091291,184.947927922739,185.025325558805,
185.102016639758,185.179767553382,185.257518467005,185.353966561799),
 .UNSPECIFIED.);
#221=B_SPLINE_CURVE_WITH_KNOTS('',3,(#22856,#22857,#22858,#22859,#22860,
#22861,#22862,#22863,#22864,#22865,#22866,#22867,#22868,#22869,#22870,#22871,
#22872,#22873,#22874,#22875,#22876,#22877,#22878,#22879,#22880,#22881,#22882,
#22883,#22884,#22885,#22886,#22887,#22888,#22889,#22890,#22891,#22892,#22893,
#22894,#22895,#22896,#22897,#22898,#22899,#22900,#22901,#22902,#22903,#22904,
#22905,#22906,#22907,#22908,#22909,#22910,#22911,#22912,#22913,#22914,#22915,
#22916,#22917,#22918,#22919,#22920,#22921,#22922,#22923,#22924,#22925,#22926,
#22927,#22928,#22929,#22930,#22931,#22932,#22933,#22934,#22935,#22936,#22937,
#22938,#22939,#22940),.UNSPECIFIED.,.F.,.F.,(4,3,3,3,3,3,3,3,3,3,3,3,3,
3,3,3,3,3,3,3,3,3,3,3,3,3,3,3,4),(183.307393789556,183.341210232577,183.4180462647,
183.494793280427,183.57146751799,183.648085157511,183.724662334139,183.80153182245,
183.878091924972,183.95466222212,184.031257283142,184.108347522514,184.185074719095,
184.262346479862,184.339618240628,184.417212910062,184.494715176172,184.572140661243,
184.64950493262,184.726823513711,184.804119218182,184.881404262838,184.958692654771,
185.035998400297,185.113376440285,185.190791512029,185.2683121263,185.338026248679,
185.353966561707),.UNSPECIFIED.);
#222=B_SPLINE_CURVE_WITH_KNOTS('',3,(#22941,#22942,#22943,#22944,#22945,
#22946,#22947,#22948,#22949,#22950,#22951,#22952,#22953,#22954,#22955,#22956,
#22957,#22958,#22959,#22960,#22961,#22962,#22963,#22964,#22965,#22966,#22967,
#22968,#22969,#22970,#22971,#22972,#22973,#22974,#22975,#22976,#22977,#22978,
#22979,#22980,#22981,#22982,#22983,#22984,#22985,#22986,#22987,#22988,#22989,
#22990,#22991,#22992,#22993,#22994,#22995,#22996,#22997,#22998,#22999,#23000,
#23001,#23002,#23003,#23004,#23005,#23006,#23007,#23008,#23009,#23010,#23011,
#23012,#23013,#23014,#23015,#23016,#23017,#23018,#23019,#23020,#23021,#23022,
#23023,#23024,#23025,#23026,#23027,#23028,#23029,#23030,#23031,#23032,#23033,
#23034,#23035,#23036,#23037,#23038,#23039,#23040,#23041,#23042,#23043,#23044,
#23045,#23046,#23047,#23048,#23049,#23050,#23051,#23052,#23053,#23054,#23055,
#23056,#23057,#23058,#23059,#23060,#23061,#23062,#23063,#23064,#23065,#23066,
#23067,#23068,#23069,#23070,#23071,#23072,#23073,#23074,#23075,#23076,#23077,
#23078,#23079,#23080,#23081,#23082,#23083,#23084,#23085,#23086,#23087,#23088,
#23089,#23090,#23091,#23092,#23093,#23094,#23095,#23096,#23097,#23098,#23099,
#23100,#23101,#23102,#23103,#23104,#23105,#23106,#23107,#23108,#23109),
 .UNSPECIFIED.,.F.,.F.,(4,3,3,3,3,3,3,3,3,3,3,3,3,3,3,3,3,3,3,3,3,3,3,3,
3,3,3,3,3,3,3,3,3,3,3,3,3,3,3,3,3,3,3,3,3,3,3,3,3,3,3,3,3,3,3,3,4),(185.353966561799,
185.434768406434,185.515467769198,185.596036962336,185.676529401149,185.756926595685,
185.837230252705,185.918243358995,185.999332053268,186.083607604134,186.164917070524,
186.246303971735,186.327811110499,186.33643425673,186.413962409939,186.491409284901,
186.568790463608,186.646121481069,186.723417835899,186.800708136235,186.877998043973,
186.955301565971,187.032632714098,187.110052203919,187.187517562341,187.265102948639,
187.334842264781,187.411705649433,187.488475481243,187.565168017232,187.641799452398,
187.718385933182,187.795243975638,187.871802298601,187.948366633274,188.024951546401,
188.102026228009,188.178733048878,188.255991660855,188.333250272832,188.410780469292,
188.488223563897,188.565595197953,188.642910961522,188.7201864043,188.79744728672,
188.874702592364,188.951966362658,189.029252641143,189.106619453935,189.184027788642,
189.261549345205,189.331658280883,189.409186417329,189.486637831798,189.564009604359,
189.59121340711),.UNSPECIFIED.);
#223=B_SPLINE_CURVE_WITH_KNOTS('',3,(#23115,#23116,#23117,#23118,#23119,
#23120,#23121,#23122,#23123,#23124,#23125,#23126,#23127,#23128,#23129,#23130,
#23131,#23132,#23133,#23134,#23135,#23136,#23137,#23138,#23139,#23140,#23141,
#23142,#23143,#23144,#23145,#23146,#23147,#23148,#23149,#23150,#23151,#23152,
#23153,#23154,#23155,#23156,#23157,#23158,#23159,#23160,#23161,#23162,#23163,
#23164,#23165,#23166,#23167,#23168,#23169,#23170,#23171,#23172,#23173,#23174,
#23175,#23176,#23177,#23178,#23179,#23180,#23181,#23182,#23183,#23184,#23185,
#23186,#23187,#23188,#23189,#23190,#23191,#23192,#23193,#23194,#23195,#23196,
#23197,#23198,#23199,#23200,#23201,#23202,#23203,#23204,#23205,#23206,#23207,
#23208,#23209,#23210,#23211,#23212,#23213,#23214,#23215,#23216,#23217,#23218,
#23219,#23220,#23221,#23222,#23223,#23224,#23225,#23226,#23227,#23228,#23229,
#23230,#23231,#23232,#23233,#23234,#23235,#23236,#23237,#23238,#23239,#23240,
#23241,#23242,#23243,#23244,#23245,#23246,#23247,#23248,#23249,#23250,#23251,
#23252,#23253,#23254,#23255,#23256,#23257,#23258,#23259,#23260,#23261,#23262,
#23263,#23264,#23265,#23266,#23267,#23268,#23269,#23270,#23271),
 .UNSPECIFIED.,.F.,.F.,(4,3,3,3,3,3,3,3,3,3,3,3,3,3,3,3,3,3,3,3,3,3,3,3,
3,3,3,3,3,3,3,3,3,3,3,3,3,3,3,3,3,3,3,3,3,3,3,3,3,3,3,3,4),(191.637151868978,
191.719614075014,191.802075932754,191.884537449048,191.966998630745,192.049459484696,
192.131920017751,192.214380236757,192.296840148565,192.379299760023,192.461759077979,
192.544218109281,192.626676860778,192.709135339316,192.791593551744,192.874051504908,
192.956509205656,193.038966660834,193.121423877288,193.20743610379,193.290760448213,
193.373227053659,193.4556928149,193.538157759353,193.620621914429,193.703085307538,
193.785547966086,193.868009917479,193.950471189118,194.032931808402,194.115391802729,
194.197851199493,194.280310026088,194.362768309905,194.445226078333,194.527683358758,
194.611816594169,194.694282592261,194.776746968617,194.859209832879,194.941671294669,
195.024131463591,195.106590449226,195.189048361143,195.274644206668,195.357108943268,
195.43957071527,195.522029961112,195.604487119089,195.686949637371,195.769407308226,
195.851866098176,195.873815125342),.UNSPECIFIED.);
#224=B_SPLINE_CURVE_WITH_KNOTS('',3,(#23272,#23273,#23274,#23275,#23276,
#23277,#23278,#23279,#23280,#23281,#23282,#23283,#23284,#23285,#23286,#23287,
#23288,#23289,#23290,#23291,#23292,#23293,#23294,#23295,#23296,#23297,#23298,
#23299,#23300,#23301,#23302,#23303,#23304,#23305,#23306,#23307,#23308,#23309,
#23310,#23311,#23312,#23313,#23314,#23315,#23316,#23317,#23318,#23319,#23320,
#23321,#23322,#23323,#23324,#23325,#23326,#23327,#23328,#23329,#23330,#23331,
#23332,#23333,#23334,#23335,#23336,#23337,#23338,#23339,#23340,#23341,#23342,
#23343,#23344,#23345,#23346,#23347,#23348,#23349,#23350,#23351,#23352,#23353),
 .UNSPECIFIED.,.F.,.F.,(4,3,3,3,3,3,3,3,3,3,3,3,3,3,3,3,3,3,3,3,3,3,3,3,
3,3,3,4),(189.591079148798,189.673744433483,189.756409718167,189.837418114071,
189.918502370903,190.00294840914,190.084254490847,190.165638280615,190.247142941643,
190.256286523852,190.333802302115,190.411236602526,190.488605020953,190.565923106103,
190.643206370148,190.72048345446,190.797760034947,190.875050130344,190.952367764349,
191.029773970673,191.107225979987,191.184798788309,191.256040135221,191.342802993755,
191.42913778928,191.51519425617,191.600806779982,191.637151868978),
 .UNSPECIFIED.);
#225=B_SPLINE_CURVE_WITH_KNOTS('',3,(#23355,#23356,#23357,#23358,#23359,
#23360,#23361,#23362,#23363,#23364,#23365,#23366,#23367,#23368,#23369,#23370,
#23371,#23372,#23373,#23374,#23375,#23376,#23377,#23378,#23379,#23380,#23381,
#23382,#23383,#23384,#23385,#23386,#23387,#23388,#23389,#23390,#23391,#23392,
#23393,#23394,#23395,#23396,#23397,#23398,#23399,#23400,#23401,#23402,#23403,
#23404,#23405,#23406,#23407,#23408,#23409,#23410,#23411,#23412,#23413,#23414,
#23415,#23416,#23417,#23418,#23419,#23420,#23421,#23422,#23423,#23424,#23425,
#23426,#23427,#23428,#23429,#23430,#23431,#23432,#23433,#23434,#23435,#23436),
 .UNSPECIFIED.,.F.,.F.,(4,3,3,3,3,3,3,3,3,3,3,3,3,3,3,3,3,3,3,3,3,3,3,3,
3,3,3,4),(189.59121340711,189.668513177153,189.745778103156,189.823035420156,
189.900292112866,189.977562222576,190.054859795428,190.132239819409,190.209665821967,
190.287197824615,190.330066288934,190.406902321057,190.483649336784,190.560323574347,
190.636941213869,190.713518390495,190.790387878807,190.866947981329,190.943518278477,
191.020113339499,191.097203578871,191.173930775452,191.251202536219,191.328474296985,
191.425080755061,191.52096575684,191.615472617705,191.637151868978),
 .UNSPECIFIED.);
#226=B_SPLINE_CURVE_WITH_KNOTS('',3,(#23437,#23438,#23439,#23440,#23441,
#23442,#23443,#23444,#23445,#23446,#23447,#23448,#23449,#23450,#23451,#23452,
#23453,#23454,#23455,#23456,#23457,#23458,#23459,#23460,#23461,#23462,#23463,
#23464,#23465,#23466,#23467,#23468,#23469,#23470,#23471,#23472,#23473,#23474,
#23475,#23476,#23477,#23478,#23479,#23480,#23481,#23482,#23483,#23484,#23485,
#23486,#23487,#23488,#23489,#23490,#23491,#23492,#23493,#23494,#23495,#23496,
#23497,#23498,#23499,#23500,#23501,#23502,#23503,#23504,#23505,#23506,#23507,
#23508,#23509,#23510,#23511,#23512,#23513,#23514,#23515,#23516,#23517,#23518,
#23519,#23520,#23521,#23522,#23523,#23524,#23525,#23526,#23527,#23528,#23529,
#23530,#23531,#23532,#23533,#23534,#23535,#23536,#23537,#23538,#23539,#23540,
#23541,#23542,#23543,#23544,#23545,#23546,#23547,#23548,#23549,#23550,#23551,
#23552,#23553,#23554,#23555,#23556,#23557,#23558,#23559,#23560,#23561,#23562,
#23563,#23564,#23565,#23566,#23567,#23568,#23569,#23570,#23571,#23572,#23573,
#23574,#23575,#23576,#23577,#23578,#23579,#23580,#23581,#23582,#23583,#23584,
#23585,#23586,#23587,#23588,#23589,#23590,#23591,#23592,#23593),
 .UNSPECIFIED.,.F.,.F.,(4,3,3,3,3,3,3,3,3,3,3,3,3,3,3,3,3,3,3,3,3,3,3,3,
3,3,3,3,3,3,3,3,3,3,3,3,3,3,3,3,3,3,3,3,3,3,3,3,3,3,3,3,4),(191.637151868978,
191.719614075014,191.802075932754,191.884537449048,191.966998630745,192.049459484696,
192.131920017751,192.214380236757,192.296840148565,192.379299760023,192.461759077979,
192.544218109281,192.626676860778,192.709135339316,192.791593551744,192.874051504908,
192.956509205656,193.038966660834,193.121423877288,193.20743610379,193.290760448214,
193.373227053659,193.4556928149,193.538157759353,193.620621914429,193.703085307538,
193.785547966086,193.868009917479,193.950471189118,194.032931808402,194.115391802729,
194.197851199493,194.280310026089,194.362768309905,194.445226078333,194.527683358758,
194.61181659417,194.694282592261,194.776746968617,194.859209832879,194.94167129467,
195.024131463591,195.106590449226,195.189048361143,195.274644206668,195.357108943268,
195.43957071527,195.522029961112,195.604487119089,195.686949637371,195.769407308226,
195.851866098176,195.873815125342),.UNSPECIFIED.);
#227=B_SPLINE_CURVE_WITH_KNOTS('',3,(#23599,#23600,#23601,#23602,#23603,
#23604,#23605,#23606,#23607,#23608,#23609,#23610,#23611,#23612,#23613,#23614,
#23615,#23616,#23617,#23618,#23619,#23620,#23621,#23622,#23623,#23624,#23625,
#23626,#23627,#23628,#23629,#23630,#23631,#23632,#23633,#23634,#23635,#23636,
#23637,#23638,#23639,#23640,#23641,#23642,#23643,#23644,#23645,#23646,#23647,
#23648,#23649,#23650,#23651,#23652,#23653,#23654,#23655,#23656,#23657,#23658,
#23659,#23660,#23661,#23662,#23663,#23664,#23665,#23666,#23667,#23668,#23669,
#23670,#23671,#23672,#23673,#23674,#23675,#23676,#23677,#23678,#23679,#23680,
#23681,#23682,#23683,#23684,#23685,#23686,#23687,#23688,#23689,#23690,#23691,
#23692,#23693,#23694,#23695,#23696,#23697,#23698,#23699,#23700,#23701,#23702,
#23703,#23704,#23705,#23706,#23707,#23708,#23709,#23710,#23711,#23712,#23713,
#23714,#23715,#23716,#23717,#23718,#23719,#23720,#23721,#23722,#23723,#23724,
#23725,#23726,#23727,#23728,#23729,#23730,#23731,#23732,#23733,#23734,#23735,
#23736,#23737,#23738,#23739,#23740,#23741,#23742,#23743,#23744,#23745,#23746,
#23747,#23748,#23749,#23750,#23751,#23752,#23753,#23754,#23755,#23756,#23757,
#23758,#23759,#23760,#23761,#23762,#23763,#23764),.UNSPECIFIED.,.F.,.F.,
(4,3,3,3,3,3,3,3,3,3,3,3,3,3,3,3,3,3,3,3,3,3,3,3,3,3,3,3,3,3,3,3,3,3,3,
3,3,3,3,3,3,3,3,3,3,3,3,3,3,3,3,3,3,3,3,4),(197.920337176158,198.012592287876,
198.105554173127,198.199343179307,198.254315414807,198.331164037994,198.407918884391,
198.484596223796,198.561212263571,198.637783162196,198.714818895193,198.791361313899,
198.867909650462,198.944478481909,199.021876117976,199.098567198929,199.176318112552,
199.254069026176,199.331586577794,199.409016797214,199.486375340109,199.563677810696,
199.640939772647,199.718186998429,199.795428509637,199.872678359869,199.949950604782,
200.027303562753,200.104697955062,200.182206282731,200.253822637546,200.331340006742,
200.408770074193,200.486128495463,200.563430874678,200.640692775441,200.717939986132,
200.79518151035,200.872431401696,200.94970371584,201.027056787066,201.104451316817,
201.181959821779,201.253576248915,201.330402679678,201.407138747595,201.483800708564,
201.560404758837,201.636968776588,201.713512055413,201.790049175251,201.866594709989,
201.943198542006,202.019832748578,202.096558624748,202.15629239339),
 .UNSPECIFIED.);
#228=B_SPLINE_CURVE_WITH_KNOTS('',3,(#23765,#23766,#23767,#23768,#23769,
#23770,#23771,#23772,#23773,#23774,#23775,#23776,#23777,#23778,#23779,#23780,
#23781,#23782,#23783,#23784,#23785,#23786,#23787,#23788,#23789,#23790,#23791,
#23792,#23793,#23794,#23795,#23796,#23797,#23798,#23799,#23800,#23801,#23802,
#23803,#23804,#23805,#23806,#23807,#23808,#23809,#23810,#23811,#23812,#23813,
#23814,#23815,#23816,#23817,#23818,#23819,#23820,#23821,#23822,#23823,#23824,
#23825,#23826,#23827,#23828,#23829,#23830,#23831,#23832,#23833,#23834,#23835,
#23836,#23837,#23838,#23839,#23840),.UNSPECIFIED.,.F.,.F.,(4,3,3,3,3,3,
3,3,3,3,3,3,3,3,3,3,3,3,3,3,3,3,3,3,3,4),(195.873815125342,195.956276729196,
196.038737667166,196.121197966652,196.203657655049,196.286116759751,196.36857530815,
196.451033327636,196.533490845598,196.620168741258,196.702635527094,196.785100640437,
196.867564190943,196.95002628824,197.032487041942,197.114946561639,197.197404956906,
197.279862337303,197.36232872357,197.444791925584,197.527252381864,197.609710530775,
197.692176135654,197.774636014869,197.857100128233,197.920337176158),
 .UNSPECIFIED.);
#229=B_SPLINE_CURVE_WITH_KNOTS('',3,(#23842,#23843,#23844,#23845,#23846,
#23847,#23848,#23849,#23850,#23851,#23852,#23853,#23854,#23855,#23856,#23857,
#23858,#23859,#23860,#23861,#23862,#23863,#23864,#23865,#23866,#23867,#23868,
#23869,#23870,#23871,#23872,#23873,#23874,#23875,#23876,#23877,#23878,#23879,
#23880,#23881,#23882,#23883,#23884,#23885,#23886,#23887,#23888,#23889,#23890,
#23891,#23892,#23893,#23894,#23895,#23896,#23897,#23898,#23899,#23900,#23901,
#23902,#23903,#23904,#23905,#23906,#23907,#23908,#23909,#23910,#23911,#23912,
#23913,#23914,#23915,#23916,#23917),.UNSPECIFIED.,.F.,.F.,(4,3,3,3,3,3,
3,3,3,3,3,3,3,3,3,3,3,3,3,3,3,3,3,3,3,4),(195.873815125342,195.956276729196,
196.038737667166,196.121197966652,196.203657655049,196.286116759751,196.36857530815,
196.451033327637,196.533490845598,196.620168741258,196.702635527094,196.785100640437,
196.867564190943,196.95002628824,197.032487041942,197.114946561639,197.197404956906,
197.279862337304,197.36232872357,197.444791925584,197.527252381865,197.609710530775,
197.692176135654,197.774636014869,197.857100128233,197.920337176158),
 .UNSPECIFIED.);
#230=B_SPLINE_CURVE_WITH_KNOTS('',3,(#23918,#23919,#23920,#23921,#23922,
#23923,#23924,#23925,#23926,#23927,#23928,#23929,#23930,#23931,#23932,#23933,
#23934,#23935,#23936,#23937,#23938,#23939,#23940,#23941,#23942,#23943,#23944,
#23945,#23946,#23947,#23948,#23949,#23950,#23951,#23952,#23953,#23954,#23955,
#23956,#23957,#23958,#23959,#23960,#23961,#23962,#23963,#23964,#23965,#23966,
#23967,#23968,#23969,#23970,#23971,#23972,#23973,#23974,#23975,#23976,#23977,
#23978,#23979,#23980,#23981,#23982,#23983,#23984,#23985,#23986,#23987,#23988,
#23989,#23990,#23991,#23992,#23993,#23994,#23995,#23996,#23997,#23998,#23999,
#24000,#24001,#24002,#24003,#24004,#24005,#24006,#24007,#24008,#24009,#24010,
#24011,#24012,#24013,#24014,#24015,#24016,#24017,#24018,#24019,#24020,#24021,
#24022,#24023,#24024,#24025,#24026,#24027,#24028,#24029,#24030,#24031,#24032,
#24033,#24034,#24035,#24036,#24037,#24038,#24039,#24040,#24041,#24042,#24043,
#24044,#24045,#24046,#24047,#24048,#24049,#24050,#24051,#24052,#24053,#24054,
#24055,#24056,#24057,#24058,#24059,#24060,#24061,#24062,#24063,#24064,#24065,
#24066,#24067,#24068,#24069,#24070,#24071,#24072,#24073,#24074,#24075,#24076,
#24077,#24078,#24079,#24080,#24081,#24082,#24083,#24084,#24085,#24086),
 .UNSPECIFIED.,.F.,.F.,(4,3,3,3,3,3,3,3,3,3,3,3,3,3,3,3,3,3,3,3,3,3,3,3,
3,3,3,3,3,3,3,3,3,3,3,3,3,3,3,3,3,3,3,3,3,3,3,3,3,3,3,3,3,3,3,3,4),(197.920337176158,
198.004940290032,198.089996506174,198.175284949322,198.260912878968,198.317330353341,
198.394925022775,198.472427288885,198.549852773956,198.627217045333,198.704535626423,
198.781831330895,198.859116375551,198.936404767484,199.013710513009,199.091088552997,
199.168503624741,199.246024239012,199.315738361392,199.397224675825,199.478606758184,
199.562690659992,199.643847978845,199.7249287626,199.805918754634,199.814942365417,
199.895955471707,199.97704416598,200.061319716846,200.142629183236,200.224016084447,
200.305523223211,200.314146369443,200.391674522652,200.469121397614,200.546502576321,
200.623833593782,200.701129948612,200.778420248948,200.855710156687,200.933013678685,
201.010344826812,201.087764316633,201.165229675055,201.242815061353,201.312554377494,
201.389426875665,201.466204023589,201.542902086867,201.619583820612,201.696169755043,
201.77272997862,201.849279064318,201.926048287445,202.002641694228,202.079498825528,
202.156355956828),.UNSPECIFIED.);
#231=B_SPLINE_CURVE_WITH_KNOTS('',3,(#24092,#24093,#24094,#24095,#24096,
#24097,#24098,#24099,#24100,#24101,#24102,#24103,#24104,#24105,#24106,#24107,
#24108,#24109,#24110,#24111,#24112,#24113,#24114,#24115,#24116,#24117,#24118,
#24119,#24120,#24121,#24122,#24123,#24124,#24125,#24126,#24127,#24128,#24129,
#24130,#24131,#24132,#24133,#24134,#24135,#24136,#24137,#24138,#24139,#24140,
#24141,#24142,#24143,#24144,#24145,#24146,#24147,#24148,#24149,#24150,#24151,
#24152,#24153,#24154,#24155,#24156,#24157,#24158,#24159,#24160,#24161,#24162,
#24163,#24164,#24165,#24166,#24167,#24168,#24169,#24170,#24171,#24172,#24173,
#24174,#24175,#24176,#24177,#24178,#24179,#24180,#24181,#24182,#24183,#24184,
#24185,#24186,#24187,#24188,#24189,#24190,#24191,#24192,#24193,#24194,#24195,
#24196,#24197,#24198,#24199,#24200,#24201,#24202,#24203,#24204,#24205,#24206,
#24207,#24208,#24209,#24210,#24211,#24212,#24213,#24214,#24215,#24216,#24217,
#24218,#24219,#24220,#24221,#24222,#24223,#24224,#24225,#24226,#24227,#24228,
#24229,#24230,#24231,#24232,#24233,#24234,#24235,#24236,#24237,#24238,#24239,
#24240,#24241,#24242,#24243,#24244,#24245,#24246,#24247,#24248,#24249,#24250,
#24251,#24252,#24253,#24254,#24255,#24256,#24257,#24258,#24259,#24260),
 .UNSPECIFIED.,.F.,.F.,(4,3,3,3,3,3,3,3,3,3,3,3,3,3,3,3,3,3,3,3,3,3,3,3,
3,3,3,3,3,3,3,3,3,3,3,3,3,3,3,3,3,3,3,3,3,3,3,3,3,3,3,3,3,3,3,3,4),(204.203522483338,
204.252837083023,204.330352861286,204.407787161697,204.485155580124,204.562473665274,
204.639756929319,204.71703401363,204.794310594118,204.871600689515,204.94891832352,
205.026324529844,205.103776539158,205.18134934748,205.252590694393,205.32943931758,
205.406194163977,205.482871503382,205.559487543157,205.636058441782,205.713094174779,
205.789636593485,205.866184930047,205.942753761495,206.020151397562,206.096842478515,
206.174593392138,206.252344305762,206.32986185738,206.4072920768,206.484650619695,
206.561953090282,206.639215052232,206.716462278015,206.793703789222,206.870953639455,
206.948225884368,207.025578842339,207.102973234648,207.180481562316,207.252097917131,
207.329615286327,207.407045353779,207.484403775048,207.561706154263,207.638968055026,
207.716215265717,207.793456789936,207.870706681282,207.947978995425,208.025332066651,
208.102726596403,208.180235101365,208.251851528501,208.328686636382,208.405419630659,
208.44084770076),.UNSPECIFIED.);
#232=B_SPLINE_CURVE_WITH_KNOTS('',3,(#24261,#24262,#24263,#24264,#24265,
#24266,#24267,#24268,#24269,#24270,#24271,#24272,#24273,#24274,#24275,#24276,
#24277,#24278,#24279,#24280,#24281,#24282,#24283,#24284,#24285,#24286,#24287,
#24288,#24289,#24290,#24291,#24292,#24293,#24294,#24295,#24296,#24297,#24298,
#24299,#24300,#24301,#24302,#24303,#24304,#24305,#24306,#24307,#24308,#24309,
#24310,#24311,#24312,#24313,#24314,#24315,#24316,#24317,#24318,#24319,#24320,
#24321,#24322,#24323,#24324,#24325,#24326,#24327,#24328,#24329,#24330,#24331,
#24332,#24333,#24334,#24335,#24336,#24337,#24338,#24339,#24340,#24341,#24342,
#24343,#24344,#24345),.UNSPECIFIED.,.F.,.F.,(4,3,3,3,3,3,3,3,3,3,3,3,3,
3,3,3,3,3,3,3,3,3,3,3,3,3,3,3,4),(202.15629239339,202.233154548504,202.253329860284,
202.330912483898,202.408402466107,202.485815443332,202.563166996833,202.640472663745,
202.717755256789,202.795027043733,202.87230204359,202.949594274528,203.026958946893,
203.104360555325,203.181868369934,203.253083471654,203.334567444609,203.415946808749,
203.500200175897,203.581353671069,203.662430349028,203.743415776818,203.752960277339,
203.832117663368,203.911324253774,203.990640924028,204.070016779426,204.149517729411,
204.203522483196),.UNSPECIFIED.);
#233=B_SPLINE_CURVE_WITH_KNOTS('',3,(#24347,#24348,#24349,#24350,#24351,
#24352,#24353,#24354,#24355,#24356,#24357,#24358,#24359,#24360,#24361,#24362,
#24363,#24364,#24365,#24366,#24367,#24368,#24369,#24370,#24371,#24372,#24373,
#24374,#24375,#24376,#24377,#24378,#24379,#24380,#24381,#24382,#24383,#24384,
#24385,#24386,#24387,#24388,#24389,#24390,#24391,#24392,#24393,#24394,#24395,
#24396,#24397,#24398,#24399,#24400,#24401,#24402,#24403,#24404,#24405,#24406,
#24407,#24408,#24409,#24410,#24411,#24412,#24413,#24414,#24415,#24416,#24417,
#24418,#24419,#24420,#24421,#24422,#24423,#24424,#24425,#24426,#24427,#24428),
 .UNSPECIFIED.,.F.,.F.,(4,3,3,3,3,3,3,3,3,3,3,3,3,3,3,3,3,3,3,3,3,3,3,3,
3,3,3,4),(202.156355956828,202.233659171187,202.310962385545,202.388492582005,
202.46593567661,202.543307310666,202.620623074235,202.697898517013,202.775159399432,
202.852414705077,202.929678475371,203.006964753856,203.084331566648,203.161739901355,
203.239261457917,203.309370393596,203.385852975525,203.462249014357,203.538575024898,
203.614847459918,203.691087020697,203.767310391095,203.843532386166,203.919767818159,
203.996069078579,204.072405451451,204.148839305911,204.203522483193),
 .UNSPECIFIED.);
#234=B_SPLINE_CURVE_WITH_KNOTS('',3,(#24429,#24430,#24431,#24432,#24433,
#24434,#24435,#24436,#24437,#24438,#24439,#24440,#24441,#24442,#24443,#24444,
#24445,#24446,#24447,#24448,#24449,#24450,#24451,#24452,#24453,#24454,#24455,
#24456,#24457,#24458,#24459,#24460,#24461,#24462,#24463,#24464,#24465,#24466,
#24467,#24468,#24469,#24470,#24471,#24472,#24473,#24474,#24475,#24476,#24477,
#24478,#24479,#24480,#24481,#24482,#24483,#24484,#24485,#24486,#24487,#24488,
#24489,#24490,#24491,#24492,#24493,#24494,#24495,#24496,#24497,#24498,#24499,
#24500,#24501,#24502,#24503,#24504,#24505,#24506,#24507,#24508,#24509,#24510,
#24511,#24512,#24513,#24514,#24515,#24516,#24517,#24518,#24519,#24520,#24521,
#24522,#24523,#24524,#24525,#24526,#24527,#24528,#24529,#24530,#24531,#24532,
#24533,#24534,#24535,#24536,#24537,#24538,#24539,#24540,#24541,#24542,#24543,
#24544,#24545,#24546,#24547,#24548,#24549,#24550,#24551,#24552,#24553,#24554,
#24555,#24556,#24557,#24558,#24559,#24560,#24561,#24562,#24563,#24564,#24565,
#24566,#24567,#24568,#24569,#24570,#24571,#24572,#24573,#24574,#24575,#24576,
#24577,#24578,#24579,#24580,#24581,#24582,#24583,#24584,#24585,#24586,#24587,
#24588,#24589,#24590,#24591,#24592,#24593,#24594,#24595,#24596,#24597),
 .UNSPECIFIED.,.F.,.F.,(4,3,3,3,3,3,3,3,3,3,3,3,3,3,3,3,3,3,3,3,3,3,3,3,
3,3,3,3,3,3,3,3,3,3,3,3,3,3,3,3,3,3,3,3,3,3,3,3,3,3,3,3,3,3,3,3,4),(204.203522483337,
204.307778401646,204.384614433769,204.461361449496,204.538035687059,204.614653326581,
204.691230503207,204.768099991519,204.844660094041,204.921230391189,204.997825452211,
205.074915691583,205.151642888164,205.228914648931,205.306186409697,205.383781079131,
205.461283345242,205.538708830312,205.616073101689,205.69339168278,205.770687387251,
205.847972431907,205.92526082384,206.002566569366,206.079944609354,206.157359681098,
206.234880295369,206.304594417748,206.386080732181,206.46746281454,206.551546716348,
206.632704035201,206.713784818956,206.79477481099,206.803798421774,206.884811528064,
206.965900222338,207.050175773203,207.131485239593,207.212872140803,207.294379279568,
207.303002425799,207.380530579008,207.457977453969,207.535358632677,207.612689650137,
207.689986004968,207.767276305304,207.844566213042,207.92186973504,207.999200883167,
208.076620372988,208.15408573141,208.231671117708,208.30141043385,208.378267534226,
208.440996940824),.UNSPECIFIED.);
#235=B_SPLINE_CURVE_WITH_KNOTS('',3,(#24603,#24604,#24605,#24606,#24607,
#24608,#24609,#24610,#24611,#24612,#24613,#24614,#24615,#24616,#24617,#24618,
#24619,#24620,#24621,#24622,#24623,#24624,#24625,#24626,#24627,#24628,#24629,
#24630,#24631,#24632,#24633,#24634,#24635,#24636,#24637,#24638,#24639,#24640,
#24641,#24642,#24643,#24644,#24645,#24646,#24647,#24648,#24649,#24650,#24651,
#24652,#24653,#24654,#24655,#24656,#24657,#24658,#24659,#24660,#24661,#24662,
#24663,#24664,#24665,#24666,#24667,#24668,#24669,#24670,#24671,#24672,#24673,
#24674,#24675,#24676,#24677,#24678,#24679,#24680,#24681,#24682,#24683,#24684,
#24685,#24686,#24687,#24688,#24689,#24690,#24691,#24692,#24693,#24694,#24695,
#24696,#24697,#24698,#24699,#24700,#24701,#24702,#24703,#24704,#24705,#24706,
#24707,#24708,#24709,#24710,#24711,#24712,#24713,#24714,#24715,#24716,#24717,
#24718,#24719,#24720,#24721,#24722,#24723,#24724,#24725,#24726,#24727,#24728,
#24729,#24730,#24731,#24732,#24733,#24734,#24735,#24736,#24737,#24738,#24739,
#24740,#24741,#24742,#24743,#24744,#24745,#24746,#24747,#24748,#24749,#24750,
#24751,#24752,#24753,#24754,#24755,#24756,#24757,#24758,#24759,#24760,#24761,
#24762,#24763,#24764,#24765,#24766,#24767,#24768,#24769,#24770,#24771),
 .UNSPECIFIED.,.F.,.F.,(4,3,3,3,3,3,3,3,3,3,3,3,3,3,3,3,3,3,3,3,3,3,3,3,
3,3,3,3,3,3,3,3,3,3,3,3,3,3,3,3,3,3,3,3,3,3,3,3,3,3,3,3,3,3,3,3,4),(210.486707790621,
210.561737282258,210.636722085166,210.711678368504,210.751235556924,210.832243952828,
210.91332820966,210.997774247897,211.079080329604,211.160464119372,211.2419687804,
211.251112362609,211.328628140872,211.406062441283,211.48343085971,211.56074894486,
211.638032208904,211.715309293216,211.792585873703,211.869875969101,211.947193603105,
212.02459980943,212.102051818743,212.179624627065,212.250865973978,212.327714597165,
212.404469443562,212.481146782966,212.557762822741,212.634333721366,212.711369454364,
212.787911873069,212.864460209632,212.94102904108,213.018426677146,213.095117758099,
213.172868671723,213.250619585347,213.328137136965,213.405567356384,213.48292589928,
213.560228369867,213.637490331817,213.7147375576,213.791979068807,213.86922891904,
213.946501163953,214.023854121924,214.101248514233,214.178756841901,214.250373196717,
214.327893335513,214.405328948147,214.48487533695,214.562173789417,214.642844146388,
214.723514503359),.UNSPECIFIED.);
#236=B_SPLINE_CURVE_WITH_KNOTS('',3,(#24772,#24773,#24774,#24775,#24776,
#24777,#24778,#24779,#24780,#24781,#24782,#24783,#24784,#24785,#24786,#24787,
#24788,#24789,#24790,#24791,#24792,#24793,#24794,#24795,#24796,#24797,#24798,
#24799,#24800,#24801,#24802,#24803,#24804,#24805,#24806,#24807,#24808,#24809,
#24810,#24811,#24812,#24813,#24814,#24815,#24816,#24817,#24818,#24819,#24820,
#24821,#24822,#24823,#24824,#24825,#24826,#24827,#24828,#24829,#24830,#24831,
#24832,#24833,#24834,#24835,#24836,#24837,#24838,#24839,#24840,#24841,#24842,
#24843,#24844,#24845,#24846,#24847,#24848,#24849,#24850,#24851,#24852,#24853),
 .UNSPECIFIED.,.F.,.F.,(4,3,3,3,3,3,3,3,3,3,3,3,3,3,3,3,3,3,3,3,3,3,3,3,
3,3,3,4),(208.44084770076,208.517478417994,208.594059812263,208.670608013932,
208.747152814121,208.823699785788,208.900263505226,208.976858556687,209.053543828347,
209.130279301935,209.207129569358,209.25160513987,209.329187763484,209.406677745693,
209.484090722918,209.561442276419,209.63874794333,209.716030536375,209.793302323319,
209.870577323175,209.947869554113,210.025234226478,210.102635834911,210.180143649519,
210.251358751239,210.349353062697,210.44622784609,210.486707790517),
 .UNSPECIFIED.);
#237=B_SPLINE_CURVE_WITH_KNOTS('',3,(#24855,#24856,#24857,#24858,#24859,
#24860,#24861,#24862,#24863,#24864,#24865,#24866,#24867,#24868,#24869,#24870,
#24871,#24872,#24873,#24874,#24875,#24876,#24877,#24878,#24879,#24880,#24881,
#24882,#24883,#24884,#24885,#24886,#24887,#24888,#24889,#24890,#24891,#24892,
#24893,#24894,#24895,#24896,#24897,#24898,#24899,#24900,#24901,#24902,#24903,
#24904,#24905,#24906,#24907,#24908,#24909,#24910,#24911,#24912,#24913,#24914,
#24915,#24916,#24917,#24918,#24919,#24920,#24921,#24922,#24923,#24924,#24925,
#24926,#24927,#24928,#24929,#24930,#24931,#24932,#24933,#24934,#24935,#24936),
 .UNSPECIFIED.,.F.,.F.,(4,3,3,3,3,3,3,3,3,3,3,3,3,3,3,3,3,3,3,3,3,3,3,3,
3,3,3,4),(208.440996940824,208.517702413484,208.594343824787,208.670937329106,
208.749547468205,208.826106181576,208.902668573492,208.979249209891,209.059391517893,
209.136092755801,209.212846284827,209.289699924151,209.299818441901,209.377348638361,
209.454791732966,209.532163367022,209.609479130591,209.686754573369,209.764015455789,
209.841270761433,209.918534531727,209.995820810212,210.073187623004,210.150595957711,
210.228117514274,210.298226449952,210.4108480197,210.486707790517),
 .UNSPECIFIED.);
#238=B_SPLINE_CURVE_WITH_KNOTS('',3,(#24937,#24938,#24939,#24940,#24941,
#24942,#24943,#24944,#24945,#24946,#24947,#24948,#24949,#24950,#24951,#24952,
#24953,#24954,#24955,#24956,#24957,#24958,#24959,#24960,#24961,#24962,#24963,
#24964,#24965,#24966,#24967,#24968,#24969,#24970,#24971,#24972,#24973,#24974,
#24975,#24976,#24977,#24978,#24979,#24980,#24981,#24982,#24983,#24984,#24985,
#24986,#24987,#24988,#24989,#24990,#24991,#24992,#24993,#24994,#24995,#24996,
#24997,#24998,#24999,#25000,#25001,#25002,#25003,#25004,#25005,#25006,#25007,
#25008,#25009,#25010,#25011,#25012,#25013,#25014,#25015,#25016,#25017,#25018,
#25019,#25020,#25021,#25022,#25023,#25024,#25025,#25026,#25027,#25028,#25029,
#25030,#25031,#25032,#25033,#25034,#25035,#25036,#25037,#25038,#25039,#25040,
#25041,#25042,#25043,#25044,#25045,#25046,#25047,#25048,#25049,#25050,#25051,
#25052,#25053,#25054,#25055,#25056,#25057,#25058,#25059,#25060,#25061,#25062,
#25063,#25064,#25065,#25066,#25067,#25068,#25069,#25070,#25071,#25072,#25073,
#25074,#25075,#25076,#25077,#25078,#25079,#25080,#25081,#25082,#25083,#25084,
#25085,#25086,#25087,#25088,#25089,#25090,#25091,#25092,#25093,#25094,#25095,
#25096,#25097,#25098,#25099,#25100,#25101,#25102,#25103,#25104,#25105,#25106,
#25107,#25108),.UNSPECIFIED.,.F.,.F.,(4,3,3,3,3,3,3,3,3,3,3,3,3,3,3,3,3,
3,3,3,3,3,3,3,3,3,3,3,3,3,3,3,3,3,3,3,3,3,3,3,3,3,3,3,3,3,3,3,3,3,3,3,3,
3,3,3,3,4),(210.486707790615,210.56305843767,210.639348328246,210.715593890765,
210.791820201114,210.868038882577,210.944264751554,211.020512627365,211.09683785511,
211.173205632822,211.249678514956,211.296634458003,211.373470490126,211.450217505853,
211.526891743416,211.603509382938,211.680086559565,211.756956047876,211.833516150399,
211.910086447546,211.986681508569,212.06377174794,212.140498944522,212.217770705288,
212.295042466054,212.372637135488,212.450139401598,212.527564886669,212.604929158045,
212.682247739136,212.759543443608,212.836828488264,212.914116880197,212.991422625723,
213.06880066571,213.146215737455,213.223736351726,213.293450474105,213.374936788538,
213.456318870897,213.540402772705,213.621560091558,213.702640875313,213.783630867346,
213.79265447813,213.873667584421,213.954756278693,214.039031829559,214.120341295949,
214.20172819716,214.283235335925,214.291858482156,214.369393170772,214.446848326865,
214.524224655243,214.601555290006,214.678852783169,214.723504023201),
 .UNSPECIFIED.);
#239=B_SPLINE_CURVE_WITH_KNOTS('',3,(#25114,#25115,#25116,#25117,#25118,
#25119,#25120,#25121,#25122,#25123,#25124,#25125,#25126,#25127,#25128,#25129,
#25130,#25131,#25132,#25133,#25134,#25135,#25136,#25137,#25138,#25139,#25140,
#25141,#25142,#25143,#25144,#25145,#25146,#25147,#25148,#25149,#25150,#25151,
#25152,#25153,#25154,#25155,#25156,#25157,#25158,#25159,#25160,#25161,#25162,
#25163,#25164,#25165,#25166,#25167,#25168,#25169,#25170,#25171,#25172,#25173,
#25174,#25175,#25176,#25177,#25178,#25179,#25180,#25181,#25182,#25183,#25184,
#25185,#25186,#25187,#25188,#25189,#25190,#25191,#25192,#25193,#25194,#25195,
#25196,#25197,#25198,#25199,#25200,#25201,#25202,#25203,#25204,#25205,#25206,
#25207,#25208,#25209,#25210,#25211,#25212,#25213,#25214,#25215,#25216,#25217,
#25218,#25219,#25220,#25221,#25222,#25223,#25224,#25225,#25226,#25227,#25228,
#25229,#25230,#25231,#25232,#25233,#25234,#25235,#25236,#25237,#25238,#25239,
#25240,#25241,#25242,#25243,#25244,#25245,#25246,#25247,#25248,#25249,#25250,
#25251,#25252,#25253,#25254,#25255,#25256,#25257,#25258,#25259,#25260,#25261,
#25262,#25263,#25264,#25265,#25266,#25267,#25268,#25269,#25270,#25271,#25272,
#25273,#25274,#25275,#25276,#25277,#25278,#25279,#25280,#25281,#25282),
 .UNSPECIFIED.,.F.,.F.,(4,3,3,3,3,3,3,3,3,3,3,3,3,3,3,3,3,3,3,3,3,3,3,3,
3,3,3,3,3,3,3,3,3,3,3,3,3,3,3,3,3,3,3,3,3,3,3,3,3,3,3,3,3,3,3,3,4),(216.769893157937,
216.850458882996,216.931110322007,217.011923257324,217.092818695108,217.173879256297,
217.249634030825,217.33111800378,217.412497367919,217.496750735067,217.577904230238,
217.658980908197,217.739966335986,217.74951083651,217.830519232414,217.911603489246,
217.996049527483,218.077355609191,218.158739398959,218.240244059988,218.249387642194,
218.326903420457,218.404337720868,218.481706139295,218.559024224445,218.636307488489,
218.713584572801,218.790861153289,218.868151248686,218.94546888269,219.022875089015,
219.100327098329,219.177899906651,219.249141253564,219.325989876751,219.402744723148,
219.479422062552,219.556038102327,219.632609000952,219.709644733949,219.786187152655,
219.862735489217,219.939304320665,220.016701956732,220.093393037685,220.171143951309,
220.248894864933,220.326425925142,220.403866965942,220.481217794065,220.558516873395,
220.635778303344,220.713016159321,220.790261594575,220.867509085248,220.944801936219,
221.00595800351),.UNSPECIFIED.);
#240=B_SPLINE_CURVE_WITH_KNOTS('',3,(#25283,#25284,#25285,#25286,#25287,
#25288,#25289,#25290,#25291,#25292,#25293,#25294,#25295,#25296,#25297,#25298,
#25299,#25300,#25301,#25302,#25303,#25304,#25305,#25306,#25307,#25308,#25309,
#25310,#25311,#25312,#25313,#25314,#25315,#25316,#25317,#25318,#25319,#25320,
#25321,#25322,#25323,#25324,#25325,#25326,#25327,#25328,#25329,#25330,#25331,
#25332,#25333,#25334,#25335,#25336,#25337,#25338,#25339,#25340,#25341,#25342,
#25343,#25344,#25345,#25346,#25347,#25348,#25349,#25350,#25351,#25352,#25353,
#25354,#25355,#25356,#25357,#25358,#25359,#25360,#25361,#25362,#25363,#25364),
 .UNSPECIFIED.,.F.,.F.,(4,3,3,3,3,3,3,3,3,3,3,3,3,3,3,3,3,3,3,3,3,3,3,3,
3,3,3,4),(214.723514503359,214.800756280101,214.878008065805,214.955283916887,
215.032641176327,215.110041371675,215.187553084504,215.250126808086,215.326948005241,
215.403679967455,215.480338945602,215.556941132064,215.633502673945,215.710549892134,
215.787094066779,215.863648346824,215.940227311803,216.017640588716,216.094352069023,
216.172116244239,216.249880419456,216.331821893514,216.413627368325,216.49530143724,
216.576798267279,216.658187206882,216.739434041545,216.769893097697),
 .UNSPECIFIED.);
#241=B_SPLINE_CURVE_WITH_KNOTS('',3,(#25366,#25367,#25368,#25369,#25370,
#25371,#25372,#25373,#25374,#25375,#25376,#25377,#25378,#25379,#25380,#25381,
#25382,#25383,#25384,#25385,#25386,#25387,#25388,#25389,#25390,#25391,#25392,
#25393,#25394,#25395,#25396,#25397,#25398,#25399,#25400,#25401,#25402,#25403,
#25404,#25405,#25406,#25407,#25408,#25409,#25410,#25411,#25412,#25413,#25414,
#25415,#25416,#25417,#25418,#25419,#25420,#25421,#25422,#25423,#25424,#25425,
#25426,#25427,#25428,#25429,#25430,#25431,#25432,#25433,#25434,#25435,#25436,
#25437,#25438,#25439,#25440,#25441,#25442,#25443,#25444,#25445,#25446,#25447),
 .UNSPECIFIED.,.F.,.F.,(4,3,3,3,3,3,3,3,3,3,3,3,3,3,3,3,3,3,3,3,3,3,3,3,
3,3,3,4),(214.723504023201,214.800792388271,214.878088454244,214.955406229928,
215.032759733642,215.110204171467,215.187701769873,215.265306891419,215.290266490207,
215.367129874859,215.443899706669,215.520592242657,215.597223677824,215.673810158607,
215.750668201063,215.827226524026,215.903790858699,215.980375771825,216.057450453433,
216.134157274302,216.21141588628,216.288674498257,216.371275620547,216.453735688925,
216.535990978226,216.618123682984,216.700074313751,216.769893097696),
 .UNSPECIFIED.);
#242=B_SPLINE_CURVE_WITH_KNOTS('',3,(#25448,#25449,#25450,#25451,#25452,
#25453,#25454,#25455,#25456,#25457,#25458,#25459,#25460,#25461,#25462,#25463,
#25464,#25465,#25466,#25467,#25468,#25469,#25470,#25471,#25472,#25473,#25474,
#25475,#25476,#25477,#25478,#25479,#25480,#25481,#25482,#25483,#25484,#25485,
#25486,#25487,#25488,#25489,#25490,#25491,#25492,#25493,#25494,#25495,#25496,
#25497,#25498,#25499,#25500,#25501,#25502,#25503,#25504,#25505,#25506,#25507,
#25508,#25509,#25510,#25511,#25512,#25513,#25514,#25515,#25516,#25517,#25518,
#25519,#25520,#25521,#25522,#25523,#25524,#25525,#25526,#25527,#25528,#25529,
#25530,#25531,#25532,#25533,#25534,#25535,#25536,#25537,#25538,#25539,#25540,
#25541,#25542,#25543,#25544,#25545,#25546,#25547,#25548,#25549,#25550,#25551,
#25552,#25553,#25554,#25555,#25556,#25557,#25558,#25559,#25560,#25561,#25562,
#25563,#25564,#25565,#25566,#25567,#25568,#25569,#25570,#25571,#25572,#25573,
#25574,#25575,#25576,#25577,#25578,#25579,#25580,#25581,#25582,#25583,#25584,
#25585,#25586,#25587,#25588,#25589,#25590,#25591,#25592,#25593,#25594,#25595,
#25596,#25597,#25598,#25599,#25600,#25601,#25602,#25603,#25604),
 .UNSPECIFIED.,.F.,.F.,(4,3,3,3,3,3,3,3,3,3,3,3,3,3,3,3,3,3,3,3,3,3,3,3,
3,3,3,3,3,3,3,3,3,3,3,3,3,3,3,3,3,3,3,3,3,3,3,3,3,3,3,3,4),(216.769893097696,
216.852355303732,216.934817161472,217.017278677766,217.099739859463,217.182200713414,
217.264661246469,217.347121465475,217.429581377283,217.512040988741,217.594500306697,
217.676959337999,217.759418089496,217.841876568034,217.924334780462,218.006792733627,
218.089250434374,218.171707889552,218.254165106007,218.340177332509,218.423501676932,
218.505968282378,218.588434043619,218.670898988072,218.753363143148,218.835826536257,
218.918289194805,219.000751146198,219.083212417837,219.165673037121,219.248133031448,
219.330592428212,219.413051254807,219.495509538624,219.577967307051,219.660424587477,
219.744557822888,219.82702382098,219.909488197335,219.991951061598,220.074412523388,
220.156872692309,220.239331677945,220.321789589862,220.407385435387,220.489850171987,
220.572311943989,220.654771189831,220.737228347808,220.819690866089,220.902148536944,
220.984607326895,221.00655635406),.UNSPECIFIED.);
#243=B_SPLINE_CURVE_WITH_KNOTS('',3,(#25610,#25611,#25612,#25613,#25614,
#25615,#25616,#25617,#25618,#25619,#25620,#25621,#25622,#25623,#25624,#25625,
#25626,#25627,#25628,#25629,#25630,#25631,#25632,#25633,#25634,#25635,#25636,
#25637,#25638,#25639,#25640,#25641,#25642,#25643,#25644,#25645,#25646,#25647,
#25648,#25649,#25650,#25651,#25652,#25653,#25654,#25655,#25656,#25657,#25658,
#25659,#25660,#25661,#25662,#25663,#25664,#25665,#25666,#25667,#25668,#25669,
#25670,#25671,#25672,#25673,#25674,#25675,#25676,#25677,#25678,#25679,#25680,
#25681,#25682,#25683,#25684,#25685,#25686,#25687,#25688,#25689,#25690,#25691,
#25692,#25693,#25694,#25695,#25696,#25697,#25698,#25699,#25700,#25701,#25702,
#25703,#25704,#25705,#25706,#25707,#25708,#25709,#25710,#25711,#25712,#25713,
#25714,#25715,#25716,#25717,#25718,#25719,#25720,#25721,#25722,#25723,#25724,
#25725,#25726,#25727,#25728,#25729,#25730,#25731,#25732,#25733,#25734,#25735,
#25736,#25737,#25738,#25739,#25740,#25741,#25742,#25743,#25744,#25745,#25746,
#25747,#25748,#25749,#25750,#25751,#25752,#25753,#25754,#25755,#25756,#25757,
#25758,#25759,#25760,#25761,#25762,#25763,#25764,#25765,#25766),
 .UNSPECIFIED.,.F.,.F.,(4,3,3,3,3,3,3,3,3,3,3,3,3,3,3,3,3,3,3,3,3,3,3,3,
3,3,3,3,3,3,3,3,3,3,3,3,3,3,3,3,3,3,3,3,3,3,3,3,3,3,3,3,4),(223.053078404876,
223.135540610912,223.218002468652,223.300463984946,223.382925166643,223.465386020594,
223.547846553649,223.630306772655,223.712766684463,223.795226295921,223.877685613877,
223.960144645179,224.042603396676,224.125061875214,224.207520087642,224.289978040806,
224.372435741554,224.454893196732,224.537350413187,224.623362639688,224.706686984112,
224.789153589557,224.871619350799,224.954084295251,225.036548450327,225.119011843436,
225.201474501985,225.283936453377,225.366397725016,225.4488583443,225.531318338627,
225.613777735392,225.696236561987,225.778694845803,225.861152614231,225.943609894656,
226.027743130068,226.110209128159,226.192673504515,226.275136368777,226.357597830568,
226.440057999489,226.522516985125,226.604974897042,226.690570742567,226.773035479167,
226.855497251169,226.937956497011,227.020413654988,227.102876173269,227.185333844124,
227.267792634075,227.28974166124),.UNSPECIFIED.);
#244=B_SPLINE_CURVE_WITH_KNOTS('',3,(#25767,#25768,#25769,#25770,#25771,
#25772,#25773,#25774,#25775,#25776,#25777,#25778,#25779,#25780,#25781,#25782,
#25783,#25784,#25785,#25786,#25787,#25788,#25789,#25790,#25791,#25792,#25793,
#25794,#25795,#25796,#25797,#25798,#25799,#25800,#25801,#25802,#25803,#25804,
#25805,#25806,#25807,#25808,#25809,#25810,#25811,#25812,#25813,#25814,#25815,
#25816,#25817,#25818,#25819,#25820,#25821,#25822,#25823,#25824,#25825,#25826,
#25827,#25828,#25829,#25830,#25831,#25832,#25833,#25834,#25835,#25836,#25837,
#25838,#25839,#25840,#25841,#25842,#25843,#25844,#25845,#25846,#25847,#25848,
#25849,#25850,#25851),.UNSPECIFIED.,.F.,.F.,(4,3,3,3,3,3,3,3,3,3,3,3,3,
3,3,3,3,3,3,3,3,3,3,3,3,3,3,3,4),(221.00595800351,221.083342689106,221.160778822706,
221.238313030152,221.248648476302,221.326165845499,221.403595912951,221.480954334221,
221.558256713437,221.6355186142,221.712765824892,221.790007349111,221.867257240458,
221.944529554602,222.021882625829,222.099277155581,222.176785660544,222.248402087672,
222.324092888759,222.39969460951,222.475224219875,222.550694126437,222.626131444521,
222.701551365929,222.776969066577,222.852428778147,222.927910739162,223.003468440949,
223.05190658296),.UNSPECIFIED.);
#245=B_SPLINE_CURVE_WITH_KNOTS('',3,(#25853,#25854,#25855,#25856,#25857,
#25858,#25859,#25860,#25861,#25862,#25863,#25864,#25865,#25866,#25867,#25868,
#25869,#25870,#25871,#25872,#25873,#25874,#25875,#25876,#25877,#25878,#25879,
#25880,#25881,#25882,#25883,#25884,#25885,#25886,#25887,#25888,#25889,#25890,
#25891,#25892,#25893,#25894,#25895,#25896,#25897,#25898,#25899,#25900,#25901,
#25902,#25903,#25904,#25905,#25906,#25907,#25908,#25909,#25910,#25911,#25912,
#25913,#25914,#25915,#25916,#25917,#25918,#25919,#25920,#25921,#25922,#25923,
#25924,#25925,#25926,#25927,#25928),.UNSPECIFIED.,.F.,.F.,(4,3,3,3,3,3,
3,3,3,3,3,3,3,3,3,3,3,3,3,3,3,3,3,3,3,4),(221.00655635406,221.089017957914,
221.171478895885,221.25393919537,221.336398883767,221.418857988469,221.501316536869,
221.583774556355,221.666232074316,221.75290996997,221.835376755805,221.917841869149,
222.000305419654,222.082767516952,222.165228270653,222.24768779035,222.330146185618,
222.412603566015,222.495069952282,222.577533154295,222.659993610576,222.742451759487,
222.824917364366,222.90737724358,222.989841356944,223.053078404766),
 .UNSPECIFIED.);
#246=B_SPLINE_CURVE_WITH_KNOTS('',3,(#25929,#25930,#25931,#25932,#25933,
#25934,#25935,#25936,#25937,#25938,#25939,#25940,#25941,#25942,#25943,#25944,
#25945,#25946,#25947,#25948,#25949,#25950,#25951,#25952,#25953,#25954,#25955,
#25956,#25957,#25958,#25959,#25960,#25961,#25962,#25963,#25964,#25965,#25966,
#25967,#25968,#25969,#25970,#25971,#25972,#25973,#25974,#25975,#25976,#25977,
#25978,#25979,#25980,#25981,#25982,#25983,#25984,#25985,#25986,#25987,#25988,
#25989,#25990,#25991,#25992,#25993,#25994,#25995,#25996,#25997,#25998,#25999,
#26000,#26001,#26002,#26003,#26004,#26005,#26006,#26007,#26008,#26009,#26010,
#26011,#26012,#26013,#26014,#26015,#26016,#26017,#26018,#26019,#26020,#26021,
#26022,#26023,#26024,#26025,#26026,#26027,#26028,#26029,#26030,#26031,#26032,
#26033,#26034,#26035,#26036,#26037,#26038,#26039,#26040,#26041,#26042,#26043,
#26044,#26045,#26046,#26047,#26048,#26049,#26050,#26051,#26052,#26053,#26054,
#26055,#26056,#26057,#26058,#26059,#26060,#26061,#26062,#26063,#26064,#26065,
#26066,#26067,#26068,#26069,#26070,#26071,#26072,#26073,#26074,#26075,#26076,
#26077,#26078,#26079,#26080,#26081,#26082,#26083,#26084,#26085),
 .UNSPECIFIED.,.F.,.F.,(4,3,3,3,3,3,3,3,3,3,3,3,3,3,3,3,3,3,3,3,3,3,3,3,
3,3,3,3,3,3,3,3,3,3,3,3,3,3,3,3,3,3,3,3,3,3,3,3,3,3,3,3,4),(223.053078404876,
223.135540610912,223.218002468652,223.300463984946,223.382925166643,223.465386020595,
223.547846553649,223.630306772655,223.712766684463,223.795226295921,223.877685613877,
223.960144645179,224.042603396676,224.125061875214,224.207520087642,224.289978040806,
224.372435741554,224.454893196732,224.537350413186,224.623362639688,224.706686984112,
224.789153589557,224.871619350799,224.954084295251,225.036548450327,225.119011843436,
225.201474501985,225.283936453377,225.366397725016,225.4488583443,225.531318338627,
225.613777735391,225.696236561987,225.778694845803,225.861152614231,225.943609894656,
226.027743130068,226.110209128159,226.192673504515,226.275136368777,226.357597830568,
226.440057999489,226.522516985124,226.604974897041,226.690570742566,226.773035479166,
226.855497251168,226.93795649701,227.020413654987,227.102876173269,227.185333844124,
227.267792634074,227.28974166124),.UNSPECIFIED.);
#247=B_SPLINE_CURVE_WITH_KNOTS('',3,(#26091,#26092,#26093,#26094,#26095,
#26096,#26097,#26098,#26099,#26100,#26101,#26102,#26103,#26104,#26105,#26106,
#26107,#26108,#26109,#26110,#26111,#26112,#26113,#26114,#26115,#26116,#26117,
#26118,#26119,#26120,#26121,#26122,#26123,#26124,#26125,#26126,#26127,#26128,
#26129,#26130,#26131,#26132,#26133,#26134,#26135,#26136,#26137,#26138,#26139,
#26140,#26141,#26142,#26143,#26144,#26145,#26146,#26147,#26148,#26149,#26150,
#26151,#26152,#26153,#26154,#26155,#26156,#26157,#26158,#26159,#26160,#26161,
#26162,#26163,#26164,#26165,#26166,#26167,#26168,#26169,#26170,#26171,#26172,
#26173,#26174,#26175,#26176,#26177,#26178,#26179,#26180,#26181,#26182,#26183,
#26184,#26185,#26186,#26187,#26188,#26189,#26190,#26191,#26192,#26193,#26194,
#26195,#26196,#26197,#26198,#26199,#26200,#26201,#26202,#26203,#26204,#26205,
#26206,#26207,#26208,#26209,#26210,#26211,#26212,#26213,#26214,#26215,#26216,
#26217,#26218,#26219,#26220,#26221,#26222,#26223,#26224,#26225,#26226,#26227,
#26228,#26229,#26230,#26231,#26232,#26233,#26234,#26235,#26236,#26237,#26238,
#26239,#26240,#26241,#26242,#26243,#26244,#26245,#26246,#26247,#26248,#26249,
#26250,#26251,#26252,#26253,#26254,#26255,#26256,#26257,#26258,#26259,#26260,
#26261,#26262),.UNSPECIFIED.,.F.,.F.,(4,3,3,3,3,3,3,3,3,3,3,3,3,3,3,3,3,
3,3,3,3,3,3,3,3,3,3,3,3,3,3,3,3,3,3,3,3,3,3,3,3,3,3,3,3,3,3,3,3,3,3,3,3,
3,3,3,3,4),(229.336901162253,229.412795891483,229.488610273219,229.56436110011,
229.640065098054,229.715860833126,229.791534894963,229.867214836791,229.942915732088,
230.018794543723,230.094620344256,230.170567362008,230.246430978627,230.324013601862,
230.401503583692,230.478916560538,230.55626811366,230.633573780193,230.710856372862,
230.788128159431,230.865403158915,230.942695389483,231.020060061483,231.097461669552,
231.174969483806,231.246184589996,231.327668566192,231.409047933538,231.493301299074,
231.57445479732,231.655531478291,231.736516908996,231.746061395681,231.827069786551,
231.908154038244,231.992600079024,232.073906155435,232.155289939871,232.236794595554,
232.245938201365,232.323453981237,232.400888283264,232.478256703313,232.55557479009,
232.632858055762,232.710135141701,232.787411723814,232.864701820835,232.942019456458,
233.019425664387,233.096877675298,233.174450485193,233.245691812735,233.322562143436,
233.399313507969,233.475996166199,233.552611946368,233.573644710383),
 .UNSPECIFIED.);
#248=B_SPLINE_CURVE_WITH_KNOTS('',3,(#26263,#26264,#26265,#26266,#26267,
#26268,#26269,#26270,#26271,#26272,#26273,#26274,#26275,#26276,#26277,#26278,
#26279,#26280,#26281,#26282,#26283,#26284,#26285,#26286,#26287,#26288,#26289,
#26290,#26291,#26292,#26293,#26294,#26295,#26296,#26297,#26298,#26299,#26300,
#26301,#26302,#26303,#26304,#26305,#26306,#26307,#26308,#26309,#26310,#26311,
#26312,#26313,#26314,#26315,#26316,#26317,#26318,#26319,#26320,#26321,#26322,
#26323,#26324,#26325,#26326,#26327,#26328,#26329,#26330,#26331,#26332,#26333,
#26334,#26335,#26336,#26337,#26338),.UNSPECIFIED.,.F.,.F.,(4,3,3,3,3,3,
3,3,3,3,3,3,3,3,3,3,3,3,3,3,3,3,3,3,3,4),(227.28974166124,227.372203265094,
227.454664203065,227.53712450255,227.619584190947,227.702043295649,227.784501844048,
227.866959863535,227.949417381496,228.036095277156,228.118562062992,228.201027176336,
228.283490726841,228.365952824138,228.44841357784,228.530873097537,228.613331492805,
228.695788873202,228.778255259468,228.860718461482,228.943178917763,229.025637066673,
229.108102671553,229.190562550767,229.273026664131,229.336263712056),
 .UNSPECIFIED.);
#249=B_SPLINE_CURVE_WITH_KNOTS('',3,(#26340,#26341,#26342,#26343,#26344,
#26345,#26346,#26347,#26348,#26349,#26350,#26351,#26352,#26353,#26354,#26355,
#26356,#26357,#26358,#26359,#26360,#26361,#26362,#26363,#26364,#26365,#26366,
#26367,#26368,#26369,#26370,#26371,#26372,#26373,#26374,#26375,#26376,#26377,
#26378,#26379,#26380,#26381,#26382,#26383,#26384,#26385,#26386,#26387,#26388,
#26389,#26390,#26391,#26392,#26393,#26394,#26395,#26396,#26397,#26398,#26399,
#26400,#26401,#26402,#26403,#26404,#26405,#26406,#26407,#26408,#26409,#26410,
#26411,#26412,#26413,#26414,#26415),.UNSPECIFIED.,.F.,.F.,(4,3,3,3,3,3,
3,3,3,3,3,3,3,3,3,3,3,3,3,3,3,3,3,3,3,4),(227.28974166124,227.372203265094,
227.454664203065,227.53712450255,227.619584190947,227.702043295649,227.784501844048,
227.866959863535,227.949417381496,228.036095277156,228.118562062992,228.201027176336,
228.283490726841,228.365952824139,228.44841357784,228.530873097537,228.613331492805,
228.695788873202,228.778255259468,228.860718461482,228.943178917763,229.025637066674,
229.108102671553,229.190562550767,229.273026664131,229.336263712056),
 .UNSPECIFIED.);
#250=B_SPLINE_CURVE_WITH_KNOTS('',3,(#26416,#26417,#26418,#26419,#26420,
#26421,#26422,#26423,#26424,#26425,#26426,#26427,#26428,#26429,#26430,#26431,
#26432,#26433,#26434,#26435,#26436,#26437,#26438,#26439,#26440,#26441,#26442,
#26443,#26444,#26445,#26446,#26447,#26448,#26449,#26450,#26451,#26452,#26453,
#26454,#26455,#26456,#26457,#26458,#26459,#26460,#26461,#26462,#26463,#26464,
#26465,#26466,#26467,#26468,#26469,#26470,#26471,#26472,#26473,#26474,#26475,
#26476,#26477,#26478,#26479,#26480,#26481,#26482,#26483,#26484,#26485,#26486,
#26487,#26488,#26489,#26490,#26491,#26492,#26493,#26494,#26495,#26496,#26497,
#26498,#26499,#26500,#26501,#26502,#26503,#26504,#26505,#26506,#26507,#26508,
#26509,#26510,#26511,#26512,#26513,#26514,#26515,#26516,#26517,#26518,#26519,
#26520,#26521,#26522,#26523,#26524,#26525,#26526,#26527,#26528,#26529,#26530,
#26531,#26532,#26533,#26534,#26535,#26536,#26537,#26538,#26539,#26540,#26541,
#26542,#26543,#26544,#26545,#26546,#26547,#26548,#26549,#26550,#26551,#26552,
#26553,#26554,#26555,#26556,#26557,#26558,#26559,#26560,#26561,#26562,#26563,
#26564,#26565,#26566,#26567,#26568,#26569,#26570,#26571,#26572,#26573,#26574,
#26575,#26576,#26577,#26578,#26579,#26580,#26581,#26582,#26583,#26584),
 .UNSPECIFIED.,.F.,.F.,(4,3,3,3,3,3,3,3,3,3,3,3,3,3,3,3,3,3,3,3,3,3,3,3,
3,3,3,3,3,3,3,3,3,3,3,3,3,3,3,3,3,3,3,3,3,3,3,3,3,3,3,3,3,3,3,3,4),(229.336929791429,
229.413011331548,229.489005470862,229.564928948207,229.640798431607,229.718996954027,
229.794819117296,229.870640824301,229.946477073216,230.022342871793,230.098291275127,
230.174289251926,230.250387401808,230.26638661097,230.343916807397,230.42135990197,
230.498731535993,230.57604729953,230.653322742275,230.730583624662,230.807838930274,
230.885102700535,230.962388978987,231.039755791747,231.117164126422,231.194685682953,
231.264794619021,231.34232473716,231.419767766552,231.497139348453,231.574455072888,
231.651730489525,231.728991365625,231.806246677046,231.883510465212,231.96079677367,
232.038163635349,232.115572029353,232.193093662296,232.263202627072,232.340038659166,
232.416785674865,232.4934599124,232.570077551894,232.646654728493,232.723524216822,
232.800084319319,232.876654616441,232.953249677439,233.03033991686,233.107067113419,
233.184338874271,233.261610635123,233.339561228579,233.417062450996,233.495237729972,
233.573413008948),.UNSPECIFIED.);
#251=B_SPLINE_CURVE_WITH_KNOTS('',3,(#26590,#26591,#26592,#26593,#26594,
#26595,#26596,#26597,#26598,#26599,#26600,#26601,#26602,#26603,#26604,#26605,
#26606,#26607,#26608,#26609,#26610,#26611,#26612,#26613,#26614,#26615,#26616,
#26617,#26618,#26619,#26620,#26621,#26622,#26623,#26624,#26625,#26626,#26627,
#26628,#26629,#26630,#26631,#26632,#26633,#26634,#26635,#26636,#26637,#26638,
#26639,#26640,#26641,#26642,#26643,#26644,#26645,#26646,#26647,#26648,#26649,
#26650,#26651,#26652,#26653,#26654,#26655,#26656,#26657,#26658,#26659,#26660,
#26661,#26662,#26663,#26664,#26665,#26666,#26667,#26668,#26669,#26670,#26671,
#26672,#26673,#26674,#26675,#26676,#26677,#26678,#26679,#26680,#26681,#26682,
#26683,#26684,#26685,#26686,#26687,#26688,#26689,#26690,#26691,#26692,#26693,
#26694,#26695,#26696,#26697,#26698,#26699,#26700,#26701,#26702,#26703,#26704,
#26705,#26706,#26707,#26708,#26709,#26710,#26711,#26712,#26713,#26714,#26715,
#26716,#26717,#26718,#26719,#26720,#26721,#26722,#26723,#26724,#26725,#26726,
#26727,#26728,#26729,#26730,#26731,#26732,#26733,#26734,#26735,#26736,#26737,
#26738,#26739,#26740,#26741,#26742,#26743,#26744,#26745,#26746,#26747,#26748,
#26749,#26750,#26751,#26752,#26753,#26754,#26755,#26756,#26757,#26758),
 .UNSPECIFIED.,.F.,.F.,(4,3,3,3,3,3,3,3,3,3,3,3,3,3,3,3,3,3,3,3,3,3,3,3,
3,3,3,3,3,3,3,3,3,3,3,3,3,3,3,3,3,3,3,3,3,3,3,3,3,3,3,3,3,3,3,3,4),(235.619449019235,
235.697636972686,235.775661087235,235.853706983637,235.931787708974,236.010078943441,
236.08830869253,236.166667592051,236.244952646843,236.321773856025,236.398505830341,
236.475164820654,236.551767019336,236.628328573482,236.705375784073,236.781919971036,
236.858474263409,236.935053240718,237.012466495091,237.089177987635,237.166942122923,
237.244706258212,237.322288813279,237.399778727044,237.477191635997,237.554543121465,
237.631848720652,237.709131246666,237.786402967016,237.863677900776,237.940970066177,
238.018334674233,238.095736218936,238.173243971391,238.244459869582,238.325944237156,
238.407323990691,238.491577161835,238.572731027894,238.653808068408,238.734793845643,
238.744336675266,238.825344565016,238.90642830662,238.990874600203,239.072180154111,
239.153563413515,239.235067544458,239.244213480951,239.321720046175,239.39914970984,
239.476516599848,239.553834805187,239.631122514021,239.708390676439,239.785671978346,
239.855757872884),.UNSPECIFIED.);
#252=B_SPLINE_CURVE_WITH_KNOTS('',3,(#26759,#26760,#26761,#26762,#26763,
#26764,#26765,#26766,#26767,#26768,#26769,#26770,#26771,#26772,#26773,#26774,
#26775,#26776,#26777,#26778,#26779,#26780,#26781,#26782,#26783,#26784,#26785,
#26786,#26787,#26788,#26789,#26790,#26791,#26792,#26793,#26794,#26795,#26796,
#26797,#26798,#26799,#26800,#26801,#26802,#26803,#26804,#26805,#26806,#26807,
#26808,#26809,#26810,#26811,#26812,#26813,#26814,#26815,#26816,#26817,#26818,
#26819,#26820,#26821,#26822,#26823,#26824,#26825,#26826,#26827,#26828,#26829,
#26830,#26831,#26832,#26833,#26834,#26835,#26836,#26837,#26838,#26839,#26840),
 .UNSPECIFIED.,.F.,.F.,(4,3,3,3,3,3,3,3,3,3,3,3,3,3,3,3,3,3,3,3,3,3,3,3,
3,3,3,4),(233.573644710383,233.650206026682,233.726753347748,233.803295926123,
233.879848336966,233.956425159158,234.033084777737,234.10978853501,234.186605455697,
234.245445424104,234.322962968516,234.400393180715,234.477751716383,234.555054179741,
234.63231613447,234.709563353064,234.786804857104,234.864054700197,234.941326938003,
235.018679888958,235.09607427429,235.173582595113,235.245199035474,235.332641113957,
235.419691044101,235.506472933431,235.592824860091,235.619449019142),
 .UNSPECIFIED.);
#253=B_SPLINE_CURVE_WITH_KNOTS('',3,(#26842,#26843,#26844,#26845,#26846,
#26847,#26848,#26849,#26850,#26851,#26852,#26853,#26854,#26855,#26856,#26857,
#26858,#26859,#26860,#26861,#26862,#26863,#26864,#26865,#26866,#26867,#26868,
#26869,#26870,#26871,#26872,#26873,#26874,#26875,#26876,#26877,#26878,#26879,
#26880,#26881,#26882,#26883,#26884,#26885,#26886,#26887,#26888,#26889,#26890,
#26891,#26892,#26893,#26894,#26895,#26896,#26897,#26898,#26899,#26900,#26901,
#26902,#26903,#26904,#26905,#26906,#26907,#26908,#26909,#26910,#26911,#26912,
#26913,#26914,#26915,#26916,#26917,#26918,#26919,#26920,#26921,#26922,#26923,
#26924,#26925,#26926),.UNSPECIFIED.,.F.,.F.,(4,3,3,3,3,3,3,3,3,3,3,3,3,
3,3,3,3,3,3,3,3,3,3,3,3,3,3,3,4),(233.573413008948,233.650730654674,233.728025925574,
233.805310883667,233.882599535934,233.959905888768,234.037284693043,234.114700841062,
234.19222204831,234.260018643174,234.341504960257,234.422887045237,234.506970945728,
234.588128267094,234.66920905331,234.750199047725,234.759222647199,234.840235749427,
234.921324439555,235.005599992472,235.086909454592,235.168296351503,235.249803485959,
235.258426651225,235.348682243228,235.435146195971,235.521372742441,235.607236547391,
235.619449019235),.UNSPECIFIED.);
#254=B_SPLINE_CURVE_WITH_KNOTS('',3,(#26927,#26928,#26929,#26930,#26931,
#26932,#26933,#26934,#26935,#26936,#26937,#26938,#26939,#26940,#26941,#26942,
#26943,#26944,#26945,#26946,#26947,#26948,#26949,#26950,#26951,#26952,#26953,
#26954,#26955,#26956,#26957,#26958,#26959,#26960,#26961,#26962,#26963,#26964,
#26965,#26966,#26967,#26968,#26969,#26970,#26971,#26972,#26973,#26974,#26975,
#26976,#26977,#26978,#26979,#26980,#26981,#26982,#26983,#26984,#26985,#26986,
#26987,#26988,#26989,#26990,#26991,#26992,#26993,#26994,#26995,#26996,#26997,
#26998,#26999,#27000,#27001,#27002,#27003,#27004,#27005,#27006,#27007,#27008,
#27009,#27010,#27011,#27012,#27013,#27014,#27015,#27016,#27017,#27018,#27019,
#27020,#27021,#27022,#27023,#27024,#27025,#27026,#27027,#27028,#27029,#27030,
#27031,#27032,#27033,#27034,#27035,#27036,#27037,#27038,#27039,#27040,#27041,
#27042,#27043,#27044,#27045,#27046,#27047,#27048,#27049,#27050,#27051,#27052,
#27053,#27054,#27055,#27056,#27057,#27058,#27059,#27060,#27061,#27062,#27063,
#27064,#27065,#27066,#27067,#27068,#27069,#27070,#27071,#27072,#27073,#27074,
#27075,#27076,#27077,#27078,#27079,#27080,#27081,#27082,#27083),
 .UNSPECIFIED.,.F.,.F.,(4,3,3,3,3,3,3,3,3,3,3,3,3,3,3,3,3,3,3,3,3,3,3,3,
3,3,3,3,3,3,3,3,3,3,3,3,3,3,3,3,3,3,3,3,3,3,3,3,3,3,3,3,4),(235.619449019235,
235.701911225271,235.784373083011,235.866834599305,235.949295781002,236.031756634953,
236.114217168008,236.196677387014,236.279137298822,236.36159691028,236.444056228236,
236.526515259538,236.608974011035,236.691432489573,236.773890702001,236.856348655165,
236.938806355913,237.021263811091,237.103721027545,237.189733254047,237.273057598471,
237.355524203916,237.437989965157,237.52045490961,237.602919064686,237.685382457795,
237.767845116343,237.850307067736,237.932768339375,238.015228958659,238.097688952986,
238.18014834975,238.262607176345,238.345065460162,238.42752322859,238.509980509015,
238.594113744427,238.676579742518,238.759044118874,238.841506983136,238.923968444927,
239.006428613848,239.088887599483,239.1713455114,239.256941356925,239.339406093525,
239.421867865527,239.50432711137,239.586784269347,239.669246787628,239.751704458483,
239.834163248434,239.856112275599),.UNSPECIFIED.);
#255=B_SPLINE_CURVE_WITH_KNOTS('',3,(#27089,#27090,#27091,#27092,#27093,
#27094,#27095,#27096,#27097,#27098,#27099,#27100,#27101,#27102,#27103,#27104,
#27105,#27106,#27107,#27108,#27109,#27110,#27111,#27112,#27113,#27114,#27115,
#27116,#27117,#27118,#27119,#27120,#27121,#27122,#27123,#27124,#27125,#27126,
#27127,#27128,#27129,#27130,#27131,#27132,#27133,#27134,#27135,#27136,#27137,
#27138,#27139,#27140,#27141,#27142,#27143,#27144,#27145,#27146,#27147,#27148,
#27149,#27150,#27151,#27152,#27153,#27154,#27155,#27156,#27157,#27158,#27159,
#27160,#27161,#27162,#27163,#27164,#27165,#27166,#27167,#27168,#27169,#27170,
#27171,#27172,#27173,#27174,#27175,#27176,#27177,#27178,#27179,#27180,#27181,
#27182,#27183,#27184,#27185,#27186,#27187,#27188,#27189,#27190,#27191,#27192,
#27193,#27194,#27195,#27196,#27197,#27198,#27199,#27200,#27201,#27202,#27203,
#27204,#27205,#27206,#27207,#27208,#27209,#27210,#27211,#27212,#27213,#27214,
#27215,#27216,#27217,#27218,#27219,#27220,#27221,#27222,#27223,#27224,#27225,
#27226,#27227,#27228,#27229,#27230,#27231,#27232,#27233,#27234,#27235,#27236,
#27237,#27238,#27239,#27240,#27241,#27242,#27243,#27244,#27245,#27246,#27247,
#27248,#27249,#27250,#27251,#27252,#27253,#27254),.UNSPECIFIED.,.F.,.F.,
(4,3,3,3,3,3,3,3,3,3,3,3,3,3,3,3,3,3,3,3,3,3,3,3,3,3,3,3,3,3,3,3,3,3,3,
3,3,3,3,3,3,3,3,3,3,3,3,3,3,3,3,3,3,3,3,4),(241.902634326508,241.991481549631,
242.08074815538,242.170566176986,242.243474315059,242.32099144496,242.398421266536,
242.47577943567,242.553081556801,242.630343193839,242.707590133178,242.784831381439,
242.862080992487,242.939353022252,243.016705804237,243.094100041666,243.171608251892,
243.243227926429,243.320052559492,243.396787962553,243.473450383891,243.550056013341,
243.626620995494,243.703666063282,243.780213655939,243.856771342673,243.933353700752,
244.010760660013,244.087475474036,244.165228505917,244.242981537798,244.320557095295,
244.398040041958,244.475446020934,244.552790620198,244.63008938361,244.707365173255,
244.784630219071,244.861898546201,244.93918417898,245.01654240536,245.093937641863,
245.171439269109,245.242735149167,245.324239347918,245.405638509028,245.489881870484,
245.571053821512,245.652148394617,245.733150864216,245.742611954852,245.823593928372,
245.904708754097,245.985890162213,246.067205728831,246.139010671909),
 .UNSPECIFIED.);
#256=B_SPLINE_CURVE_WITH_KNOTS('',3,(#27255,#27256,#27257,#27258,#27259,
#27260,#27261,#27262,#27263,#27264,#27265,#27266,#27267,#27268,#27269,#27270,
#27271,#27272,#27273,#27274,#27275,#27276,#27277,#27278,#27279,#27280,#27281,
#27282,#27283,#27284,#27285,#27286,#27287,#27288,#27289,#27290,#27291,#27292,
#27293,#27294,#27295,#27296,#27297,#27298,#27299,#27300,#27301,#27302,#27303,
#27304,#27305,#27306,#27307,#27308,#27309,#27310,#27311,#27312,#27313,#27314,
#27315,#27316,#27317,#27318,#27319,#27320,#27321,#27322,#27323,#27324,#27325,
#27326,#27327,#27328,#27329,#27330,#27331,#27332,#27333,#27334,#27335,#27336),
 .UNSPECIFIED.,.F.,.F.,(4,3,3,3,3,3,3,3,3,3,3,3,3,3,3,3,3,3,3,3,3,3,3,3,
3,3,3,4),(239.855757872884,239.93307233432,240.01079602382,240.088243427902,
240.166105260111,240.24396709232,240.320816209889,240.397571551698,240.474249387176,
240.550865923322,240.627437318259,240.704472741438,240.78101565417,240.857564483456,
240.934133806003,241.011530530425,241.088222094877,241.165971399284,241.24372070369,
241.3215239023,241.39920307501,241.476809248804,241.554356273541,241.631857962595,
241.709331190126,241.786787502144,241.864252488673,241.902634326415),
 .UNSPECIFIED.);
#257=B_SPLINE_CURVE_WITH_KNOTS('',3,(#27338,#27339,#27340,#27341,#27342,
#27343,#27344,#27345,#27346,#27347,#27348,#27349,#27350,#27351,#27352,#27353,
#27354,#27355,#27356,#27357,#27358,#27359,#27360,#27361,#27362,#27363,#27364,
#27365,#27366,#27367,#27368,#27369,#27370,#27371,#27372,#27373,#27374,#27375,
#27376,#27377,#27378,#27379,#27380,#27381,#27382,#27383,#27384,#27385,#27386,
#27387,#27388,#27389,#27390,#27391,#27392,#27393,#27394,#27395,#27396,#27397,
#27398,#27399,#27400,#27401,#27402,#27403,#27404,#27405,#27406,#27407,#27408,
#27409,#27410,#27411,#27412,#27413),.UNSPECIFIED.,.F.,.F.,(4,3,3,3,3,3,
3,3,3,3,3,3,3,3,3,3,3,3,3,3,3,3,3,3,3,4),(239.856112275599,239.938573879453,
240.021034817424,240.103495116909,240.185954805306,240.268413910008,240.350872458408,
240.433330477894,240.515787995855,240.602465891515,240.684932677351,240.767397790695,
240.8498613412,240.932323438498,241.014784192199,241.097243711896,241.179702107164,
241.262159487561,241.344625873827,241.427089075841,241.509549532122,241.592007681033,
241.674473285912,241.756933165126,241.83939727849,241.902634326415),
 .UNSPECIFIED.);
#258=B_SPLINE_CURVE_WITH_KNOTS('',3,(#27414,#27415,#27416,#27417,#27418,
#27419,#27420,#27421,#27422,#27423,#27424,#27425,#27426,#27427,#27428,#27429,
#27430,#27431,#27432,#27433,#27434,#27435,#27436,#27437,#27438,#27439,#27440,
#27441,#27442,#27443,#27444,#27445,#27446,#27447,#27448,#27449,#27450,#27451,
#27452,#27453,#27454,#27455,#27456,#27457,#27458,#27459,#27460,#27461,#27462,
#27463,#27464,#27465,#27466,#27467,#27468,#27469,#27470,#27471,#27472,#27473,
#27474,#27475,#27476,#27477,#27478,#27479,#27480,#27481,#27482,#27483,#27484,
#27485,#27486,#27487,#27488,#27489,#27490,#27491,#27492,#27493,#27494,#27495,
#27496,#27497,#27498,#27499,#27500,#27501,#27502,#27503,#27504,#27505,#27506,
#27507,#27508,#27509,#27510,#27511,#27512,#27513,#27514,#27515,#27516,#27517,
#27518,#27519,#27520,#27521,#27522,#27523,#27524,#27525,#27526,#27527,#27528,
#27529,#27530,#27531,#27532,#27533,#27534,#27535,#27536,#27537,#27538,#27539,
#27540,#27541,#27542,#27543,#27544,#27545,#27546,#27547,#27548,#27549,#27550,
#27551,#27552,#27553,#27554,#27555,#27556,#27557,#27558,#27559,#27560,#27561,
#27562,#27563,#27564,#27565,#27566,#27567,#27568,#27569,#27570,#27571,#27572,
#27573,#27574,#27575,#27576,#27577,#27578,#27579),.UNSPECIFIED.,.F.,.F.,
(4,3,3,3,3,3,3,3,3,3,3,3,3,3,3,3,3,3,3,3,3,3,3,3,3,3,3,3,3,3,3,3,3,3,3,
3,3,3,3,3,3,3,3,3,3,3,3,3,3,3,3,3,3,3,3,4),(241.902634326415,241.989992668194,
242.077614906619,242.165592798624,242.247282707581,242.324810843968,242.402257701764,
242.479638862983,242.556969862651,242.634266199403,242.711556481288,242.78884637035,
242.866149873463,242.943481002511,243.020900473052,243.098365812055,243.175951178883,
243.245690715632,243.322554508064,243.399324748456,243.476017693521,243.552649537958,
243.629236427911,243.706094214882,243.782652944994,243.859217685687,243.93580300344,
244.012876933501,244.089584152607,244.166841438145,244.244098723683,244.321628306997,
244.399070789021,244.476441811629,244.553756965454,244.63103180076,244.708292081124,
244.785546788089,244.862809963593,244.940095651694,245.017461884113,245.094869643067,
245.172390637053,245.242506731734,245.320041956006,245.397488959025,245.474863386662,
245.552180832619,245.629457522982,245.706713006305,245.78396132947,245.861216532633,
245.938523563794,246.015858858115,246.093274423267,246.138985228352),
 .UNSPECIFIED.);
#259=B_SPLINE_CURVE_WITH_KNOTS('',3,(#27585,#27586,#27587,#27588,#27589,
#27590,#27591,#27592,#27593,#27594,#27595,#27596,#27597,#27598,#27599,#27600,
#27601,#27602,#27603,#27604,#27605,#27606,#27607,#27608,#27609,#27610,#27611,
#27612,#27613,#27614,#27615,#27616,#27617,#27618,#27619,#27620,#27621,#27622,
#27623,#27624,#27625,#27626,#27627,#27628,#27629,#27630,#27631,#27632,#27633,
#27634,#27635,#27636,#27637,#27638,#27639,#27640,#27641,#27642,#27643,#27644,
#27645,#27646,#27647,#27648,#27649,#27650,#27651,#27652,#27653,#27654,#27655,
#27656,#27657,#27658,#27659,#27660,#27661,#27662,#27663,#27664,#27665,#27666,
#27667,#27668,#27669,#27670,#27671,#27672,#27673,#27674,#27675,#27676,#27677,
#27678,#27679,#27680,#27681,#27682,#27683,#27684,#27685,#27686,#27687,#27688,
#27689,#27690,#27691,#27692,#27693,#27694,#27695,#27696,#27697,#27698,#27699,
#27700,#27701,#27702,#27703,#27704,#27705,#27706,#27707,#27708,#27709,#27710,
#27711,#27712,#27713,#27714,#27715,#27716,#27717,#27718,#27719,#27720,#27721,
#27722,#27723,#27724,#27725,#27726,#27727,#27728,#27729,#27730,#27731,#27732,
#27733,#27734,#27735,#27736,#27737,#27738,#27739,#27740,#27741,#27742,#27743,
#27744,#27745,#27746,#27747,#27748,#27749,#27750,#27751,#27752,#27753),
 .UNSPECIFIED.,.F.,.F.,(4,3,3,3,3,3,3,3,3,3,3,3,3,3,3,3,3,3,3,3,3,3,3,3,
3,3,3,3,3,3,3,3,3,3,3,3,3,3,3,3,3,3,3,3,3,3,3,3,3,3,3,3,3,3,3,3,4),(248.185819633594,
248.241995983275,248.319487727223,248.396892528157,248.474226060436,248.551503947157,
248.628741771101,248.705965609896,248.783184193659,248.860411594013,248.937661884912,
249.014993781544,249.092367567984,249.16985625361,249.241749594645,249.3190756192,
249.396313467627,249.47347898075,249.550587946356,249.627656110613,249.704709720991,
249.781757743613,249.858814395049,249.935893894216,250.013055834642,250.090259859986,
250.167580736355,250.241503206014,250.318795771638,250.395999058236,250.473128942955,
250.550201248839,250.627231756401,250.704246300672,250.781254399568,250.858270298374,
250.935308244274,251.012427570257,251.089588337495,251.166865255886,251.241256817383,
251.318543779487,251.395742395434,251.472868538853,251.54993802998,251.626966647179,
251.703980715081,251.780989198166,251.858006341696,251.935046393322,252.012169177978,
252.089334144646,252.16661649259,252.241010428753,252.318356969681,252.395602472991,
252.423061447523),.UNSPECIFIED.);
#260=B_SPLINE_CURVE_WITH_KNOTS('',3,(#27754,#27755,#27756,#27757,#27758,
#27759,#27760,#27761,#27762,#27763,#27764,#27765,#27766,#27767,#27768,#27769,
#27770,#27771,#27772,#27773,#27774,#27775,#27776,#27777,#27778,#27779,#27780,
#27781,#27782,#27783,#27784,#27785,#27786,#27787,#27788,#27789,#27790,#27791,
#27792,#27793,#27794,#27795,#27796,#27797,#27798,#27799,#27800,#27801,#27802,
#27803,#27804,#27805,#27806,#27807,#27808,#27809,#27810,#27811,#27812,#27813,
#27814,#27815,#27816,#27817,#27818,#27819,#27820,#27821,#27822,#27823,#27824,
#27825,#27826,#27827,#27828,#27829,#27830,#27831,#27832,#27833,#27834,#27835,
#27836,#27837,#27838),.UNSPECIFIED.,.F.,.F.,(4,3,3,3,3,3,3,3,3,3,3,3,3,
3,3,3,3,3,3,3,3,3,3,3,3,3,3,3,4),(246.139010671909,246.22049939025,246.242488760537,
246.319972614284,246.39737478087,246.47471088857,246.55199651825,246.629247214064,
246.706491667892,246.783735582781,246.860993005942,246.938277989561,247.015651755802,
247.093071389889,247.17061224538,247.242242371906,247.318525712687,247.394716184162,
247.470830452629,247.54688511173,247.626751926949,247.702745016196,247.778732529846,
247.854729383306,247.930750496942,248.006848406085,248.082991117387,248.159232220467,
248.185819633476),.UNSPECIFIED.);
#261=B_SPLINE_CURVE_WITH_KNOTS('',3,(#27840,#27841,#27842,#27843,#27844,
#27845,#27846,#27847,#27848,#27849,#27850,#27851,#27852,#27853,#27854,#27855,
#27856,#27857,#27858,#27859,#27860,#27861,#27862,#27863,#27864,#27865,#27866,
#27867,#27868,#27869,#27870,#27871,#27872,#27873,#27874,#27875,#27876,#27877,
#27878,#27879,#27880,#27881,#27882,#27883,#27884,#27885,#27886,#27887,#27888,
#27889,#27890,#27891,#27892,#27893,#27894,#27895,#27896,#27897,#27898,#27899,
#27900,#27901,#27902,#27903,#27904,#27905,#27906,#27907,#27908,#27909,#27910,
#27911,#27912,#27913,#27914,#27915,#27916,#27917,#27918,#27919,#27920,#27921,
#27922,#27923,#27924),.UNSPECIFIED.,.F.,.F.,(4,3,3,3,3,3,3,3,3,3,3,3,3,
3,3,3,3,3,3,3,3,3,3,3,3,3,3,3,4),(246.138985228352,246.216525059607,246.240914739785,
246.317753603474,246.394503454466,246.471180528847,246.547801004633,246.624381014889,
246.701248731507,246.777811648328,246.854384750045,246.930982604032,247.008067639983,
247.084797579722,247.162060163779,247.239322747836,247.316388332712,247.393362019337,
247.47025992237,247.547098097972,247.626938289913,247.703711618014,247.780477476615,
247.857250311506,247.934044570009,248.010908994861,248.087815045339,248.164811091715,
248.185819633502),.UNSPECIFIED.);
#262=B_SPLINE_CURVE_WITH_KNOTS('',3,(#27925,#27926,#27927,#27928,#27929,
#27930,#27931,#27932,#27933,#27934,#27935,#27936,#27937,#27938,#27939,#27940,
#27941,#27942,#27943,#27944,#27945,#27946,#27947,#27948,#27949,#27950,#27951,
#27952,#27953,#27954,#27955,#27956,#27957,#27958,#27959,#27960,#27961,#27962,
#27963,#27964,#27965,#27966,#27967,#27968,#27969,#27970,#27971,#27972,#27973,
#27974,#27975,#27976,#27977,#27978,#27979,#27980,#27981,#27982,#27983,#27984,
#27985,#27986,#27987,#27988,#27989,#27990,#27991,#27992,#27993,#27994,#27995,
#27996,#27997,#27998,#27999,#28000,#28001,#28002,#28003,#28004,#28005,#28006,
#28007,#28008,#28009,#28010,#28011,#28012,#28013,#28014,#28015,#28016,#28017,
#28018,#28019,#28020,#28021,#28022,#28023,#28024,#28025,#28026,#28027,#28028,
#28029,#28030,#28031,#28032,#28033,#28034,#28035,#28036,#28037,#28038,#28039,
#28040,#28041,#28042,#28043,#28044,#28045,#28046,#28047,#28048,#28049,#28050,
#28051,#28052,#28053,#28054,#28055,#28056,#28057,#28058,#28059,#28060,#28061,
#28062,#28063,#28064,#28065,#28066,#28067,#28068,#28069,#28070,#28071,#28072,
#28073,#28074,#28075,#28076,#28077,#28078,#28079,#28080,#28081,#28082,#28083,
#28084,#28085,#28086,#28087,#28088,#28089,#28090,#28091,#28092,#28093,#28094,
#28095,#28096),.UNSPECIFIED.,.F.,.F.,(4,3,3,3,3,3,3,3,3,3,3,3,3,3,3,3,3,
3,3,3,3,3,3,3,3,3,3,3,3,3,3,3,3,3,3,3,3,3,3,3,3,3,3,3,3,3,3,3,3,3,3,3,3,
3,3,3,3,4),(248.185819633594,248.237730755887,248.319231491894,248.400627669662,
248.484704442224,248.565874851764,248.646968309605,248.727970345441,248.736934759912,
248.817943698033,248.899028371482,248.983305969596,249.064611849977,249.145995327554,
249.227499291205,249.236138763938,249.313639927106,249.39105963649,249.468413501639,
249.545717084913,249.622985912136,249.700248635407,249.777510938544,249.854786852635,
249.932090413791,250.009482497813,250.08692050769,250.164478904197,250.234546771989,
250.311465957294,250.388291594326,250.465039899041,250.541727026095,250.618369082065,
250.695192294312,250.771805665824,250.848424800283,250.925064228465,251.002036866359,
251.078797104637,251.155875942338,251.23295478004,251.310468016654,251.387894476587,
251.465249812563,251.542549626252,251.619809479155,251.697055364972,251.774296037089,
251.851545548233,251.928817953463,252.006171569364,252.083567057275,252.161076476131,
252.23136278809,252.308745271866,252.386027282496,252.423069114013),
 .UNSPECIFIED.);
#263=B_SPLINE_CURVE_WITH_KNOTS('',3,(#28102,#28103,#28104,#28105,#28106,
#28107,#28108,#28109,#28110,#28111,#28112,#28113,#28114,#28115,#28116,#28117,
#28118,#28119,#28120,#28121,#28122,#28123,#28124,#28125,#28126,#28127,#28128,
#28129,#28130,#28131,#28132,#28133,#28134,#28135,#28136,#28137,#28138,#28139,
#28140,#28141,#28142,#28143,#28144,#28145,#28146,#28147,#28148,#28149,#28150,
#28151,#28152,#28153,#28154,#28155,#28156,#28157,#28158,#28159,#28160,#28161,
#28162,#28163,#28164,#28165,#28166,#28167,#28168,#28169,#28170,#28171,#28172,
#28173,#28174,#28175,#28176,#28177,#28178,#28179,#28180,#28181,#28182,#28183,
#28184,#28185,#28186,#28187,#28188,#28189,#28190,#28191,#28192,#28193,#28194,
#28195,#28196,#28197,#28198,#28199,#28200,#28201,#28202,#28203,#28204,#28205,
#28206,#28207,#28208,#28209,#28210,#28211,#28212,#28213,#28214,#28215,#28216,
#28217,#28218,#28219,#28220,#28221,#28222,#28223,#28224,#28225,#28226,#28227,
#28228,#28229,#28230,#28231,#28232,#28233,#28234,#28235,#28236,#28237,#28238,
#28239,#28240,#28241,#28242,#28243,#28244,#28245,#28246,#28247,#28248,#28249,
#28250,#28251,#28252,#28253,#28254,#28255,#28256,#28257,#28258),
 .UNSPECIFIED.,.F.,.F.,(4,3,3,3,3,3,3,3,3,3,3,3,3,3,3,3,3,3,3,3,3,3,3,3,
3,3,3,3,3,3,3,3,3,3,3,3,3,3,3,3,3,3,3,3,3,3,3,3,3,3,3,3,4),(254.469004940774,
254.55146714681,254.63392900455,254.716390520844,254.798851702541,254.881312556492,
254.963773089547,255.046233308553,255.128693220361,255.211152831819,255.293612149775,
255.376071181077,255.458529932574,255.540988411113,255.623446623541,255.705904576705,
255.788362277453,255.87081973263,255.953276949085,256.039289175586,256.12261352001,
256.205080125455,256.287545886697,256.370010831149,256.452474986225,256.534938379334,
256.617401037883,256.699862989275,256.782324260914,256.864784880198,256.947244874525,
257.02970427129,257.112163097885,257.194621381701,257.277079150129,257.359536430554,
257.443669665966,257.526135664057,257.608600040413,257.691062904675,257.773524366466,
257.855984535387,257.938443521023,258.02090143294,258.106497278465,258.188962015065,
258.271423787067,258.353883032909,258.436340190886,258.518802709167,258.601260380022,
258.683719169973,258.705668197138),.UNSPECIFIED.);
#264=B_SPLINE_CURVE_WITH_KNOTS('',3,(#28259,#28260,#28261,#28262,#28263,
#28264,#28265,#28266,#28267,#28268,#28269,#28270,#28271,#28272,#28273,#28274,
#28275,#28276,#28277,#28278,#28279,#28280,#28281,#28282,#28283,#28284,#28285,
#28286,#28287,#28288,#28289,#28290,#28291,#28292,#28293,#28294,#28295,#28296,
#28297,#28298,#28299,#28300,#28301,#28302,#28303,#28304,#28305,#28306,#28307,
#28308,#28309,#28310,#28311,#28312,#28313,#28314,#28315,#28316,#28317,#28318,
#28319,#28320,#28321,#28322,#28323,#28324,#28325,#28326,#28327,#28328,#28329,
#28330,#28331,#28332,#28333,#28334,#28335,#28336,#28337,#28338,#28339,#28340),
 .UNSPECIFIED.,.F.,.F.,(4,3,3,3,3,3,3,3,3,3,3,3,3,3,3,3,3,3,3,3,3,3,3,3,
3,3,3,4),(252.423061447523,252.500207989694,252.577302788264,252.654361578884,
252.731411716478,252.808460577922,252.885522379586,252.962611342577,253.039783546726,
253.117001743405,253.194328265335,253.240764040122,253.318261963832,253.395671913165,
253.47300956625,253.550290549208,253.62753044714,253.704754798586,253.781972943272,
253.859198952847,253.936446900755,254.013774962946,254.0911440958,254.168626777181,
254.240517651492,254.344578896921,254.445902077886,254.469004940774),
 .UNSPECIFIED.);
#265=B_SPLINE_CURVE_WITH_KNOTS('',3,(#28342,#28343,#28344,#28345,#28346,
#28347,#28348,#28349,#28350,#28351,#28352,#28353,#28354,#28355,#28356,#28357,
#28358,#28359,#28360,#28361,#28362,#28363,#28364,#28365,#28366,#28367,#28368,
#28369,#28370,#28371,#28372,#28373,#28374,#28375,#28376,#28377,#28378,#28379,
#28380,#28381,#28382,#28383,#28384,#28385,#28386,#28387,#28388,#28389,#28390,
#28391,#28392,#28393,#28394,#28395,#28396,#28397,#28398,#28399,#28400,#28401,
#28402,#28403,#28404,#28405,#28406,#28407,#28408,#28409,#28410,#28411,#28412,
#28413,#28414,#28415,#28416,#28417,#28418,#28419,#28420,#28421,#28422,#28423),
 .UNSPECIFIED.,.F.,.F.,(4,3,3,3,3,3,3,3,3,3,3,3,3,3,3,3,3,3,3,3,3,3,3,3,
3,3,3,4),(252.423069114013,252.500249935134,252.57738204784,252.654481140577,
252.731575367837,252.808670952456,252.885782074225,252.962922919092,253.040148347162,
253.117421991369,253.1948013524,253.229770796141,253.306987152008,253.384114373385,
253.46116840088,253.538165120588,253.615120375872,253.69206034023,253.768994302006,
253.845936563417,253.922901428936,253.999948640481,254.077037871748,254.154244171017,
254.228178804192,254.331935348037,254.433147614106,254.469004940774),
 .UNSPECIFIED.);
#266=B_SPLINE_CURVE_WITH_KNOTS('',3,(#28424,#28425,#28426,#28427,#28428,
#28429,#28430,#28431,#28432,#28433,#28434,#28435,#28436,#28437,#28438,#28439,
#28440,#28441,#28442,#28443,#28444,#28445,#28446,#28447,#28448,#28449,#28450,
#28451,#28452,#28453,#28454,#28455,#28456,#28457,#28458,#28459,#28460,#28461,
#28462,#28463,#28464,#28465,#28466,#28467,#28468,#28469,#28470,#28471,#28472,
#28473,#28474,#28475,#28476,#28477,#28478,#28479,#28480,#28481,#28482,#28483,
#28484,#28485,#28486,#28487,#28488,#28489,#28490,#28491,#28492,#28493,#28494,
#28495,#28496,#28497,#28498,#28499,#28500,#28501,#28502,#28503,#28504,#28505,
#28506,#28507,#28508,#28509,#28510,#28511,#28512,#28513,#28514,#28515,#28516,
#28517,#28518,#28519,#28520,#28521,#28522,#28523,#28524,#28525,#28526,#28527,
#28528,#28529,#28530,#28531,#28532,#28533,#28534,#28535,#28536,#28537,#28538,
#28539,#28540,#28541,#28542,#28543,#28544,#28545,#28546,#28547,#28548,#28549,
#28550,#28551,#28552,#28553,#28554,#28555,#28556,#28557,#28558,#28559,#28560,
#28561,#28562,#28563,#28564,#28565,#28566,#28567,#28568,#28569,#28570,#28571,
#28572,#28573,#28574,#28575,#28576,#28577,#28578,#28579,#28580),
 .UNSPECIFIED.,.F.,.F.,(4,3,3,3,3,3,3,3,3,3,3,3,3,3,3,3,3,3,3,3,3,3,3,3,
3,3,3,3,3,3,3,3,3,3,3,3,3,3,3,3,3,3,3,3,3,3,3,3,3,3,3,3,4),(254.469004940774,
254.55146714681,254.63392900455,254.716390520844,254.798851702541,254.881312556492,
254.963773089547,255.046233308553,255.128693220361,255.211152831819,255.293612149775,
255.376071181077,255.458529932574,255.540988411112,255.62344662354,255.705904576704,
255.788362277452,255.87081973263,255.953276949084,256.039289175586,256.122613520009,
256.205080125455,256.287545886696,256.370010831148,256.452474986224,256.534938379333,
256.617401037882,256.699862989275,256.782324260913,256.864784880198,256.947244874524,
257.029704271289,257.112163097884,257.194621381701,257.277079150128,257.359536430553,
257.443669665965,257.526135664057,257.608600040412,257.691062904674,257.773524366465,
257.855984535386,257.938443521022,258.020901432939,258.106497278464,258.188962015064,
258.271423787066,258.353883032908,258.436340190885,258.518802709166,258.601260380021,
258.683719169972,258.705668197138),.UNSPECIFIED.);
#267=B_SPLINE_CURVE_WITH_KNOTS('',3,(#28586,#28587,#28588,#28589,#28590,
#28591,#28592,#28593,#28594,#28595,#28596,#28597,#28598,#28599,#28600,#28601,
#28602,#28603,#28604,#28605,#28606,#28607,#28608,#28609,#28610,#28611,#28612,
#28613,#28614,#28615,#28616,#28617,#28618,#28619,#28620,#28621,#28622,#28623,
#28624,#28625,#28626,#28627,#28628,#28629,#28630,#28631,#28632,#28633,#28634,
#28635,#28636,#28637,#28638,#28639,#28640,#28641,#28642,#28643,#28644,#28645,
#28646,#28647,#28648,#28649,#28650,#28651,#28652,#28653,#28654,#28655,#28656,
#28657,#28658,#28659,#28660,#28661,#28662,#28663,#28664,#28665,#28666,#28667,
#28668,#28669,#28670,#28671,#28672,#28673,#28674,#28675,#28676,#28677,#28678,
#28679,#28680,#28681,#28682,#28683,#28684,#28685,#28686,#28687,#28688,#28689,
#28690,#28691,#28692,#28693,#28694,#28695,#28696,#28697,#28698,#28699,#28700,
#28701,#28702,#28703,#28704,#28705,#28706,#28707,#28708,#28709,#28710,#28711,
#28712,#28713,#28714,#28715,#28716,#28717,#28718,#28719,#28720,#28721,#28722,
#28723,#28724,#28725,#28726,#28727,#28728,#28729,#28730,#28731,#28732,#28733,
#28734,#28735,#28736,#28737,#28738,#28739,#28740,#28741,#28742,#28743,#28744,
#28745,#28746,#28747,#28748,#28749,#28750,#28751,#28752,#28753,#28754),
 .UNSPECIFIED.,.F.,.F.,(4,3,3,3,3,3,3,3,3,3,3,3,3,3,3,3,3,3,3,3,3,3,3,3,
3,3,3,3,3,3,3,3,3,3,3,3,3,3,3,3,3,3,3,3,3,3,3,3,3,3,3,3,3,3,3,3,4),(260.752190247954,
260.833924659858,260.915784801191,260.997857630573,261.080038110251,261.162414601535,
261.238792931077,261.315614602842,261.392347043997,261.469006505033,261.54560917796,
261.622171209519,261.699218126134,261.775762796189,261.852317573389,261.928897036949,
262.006309413323,262.083021391968,262.160783967207,262.238546542446,262.316129158385,
262.393619133169,262.471032103223,262.548383649812,262.625689310076,262.702971896898,
262.780243677878,262.857518672036,262.934810897546,263.012175564937,263.089577168637,
263.167084978965,263.238300153816,263.319783597925,263.401162433877,263.485416065282,
263.566569041431,263.64764520618,263.728630130979,263.7381769595,263.819185708317,
263.900270329473,263.984716188401,264.066022655456,264.147406836517,264.228911894201,
264.238053765185,264.315582157019,264.393026319221,264.470388847433,264.547704869653,
264.624988440364,264.702253593051,264.779533264968,264.856819399072,264.934155284713,
264.988317180418),.UNSPECIFIED.);
#268=B_SPLINE_CURVE_WITH_KNOTS('',3,(#28755,#28756,#28757,#28758,#28759,
#28760,#28761,#28762,#28763,#28764,#28765,#28766,#28767,#28768,#28769,#28770,
#28771,#28772,#28773,#28774,#28775,#28776,#28777,#28778,#28779,#28780,#28781,
#28782,#28783,#28784,#28785,#28786,#28787,#28788,#28789,#28790,#28791,#28792,
#28793,#28794,#28795,#28796,#28797,#28798,#28799,#28800,#28801,#28802,#28803,
#28804,#28805,#28806,#28807,#28808,#28809,#28810,#28811,#28812,#28813,#28814,
#28815,#28816,#28817,#28818,#28819,#28820,#28821,#28822,#28823,#28824,#28825,
#28826,#28827,#28828,#28829,#28830),.UNSPECIFIED.,.F.,.F.,(4,3,3,3,3,3,
3,3,3,3,3,3,3,3,3,3,3,3,3,3,3,3,3,3,3,4),(258.705668197138,258.788129800992,
258.870590738963,258.953051038448,259.035510726845,259.117969831547,259.200428379947,
259.282886399433,259.365343917394,259.452021813054,259.53448859889,259.616953712234,
259.699417262739,259.781879360037,259.864340113738,259.946799633435,260.029258028703,
260.1117154091,260.194181795366,260.27664499738,260.359105453661,260.441563602571,
260.524029207451,260.606489086665,260.688953200029,260.752190247954),
 .UNSPECIFIED.);
#269=B_SPLINE_CURVE_WITH_KNOTS('',3,(#28832,#28833,#28834,#28835,#28836,
#28837,#28838,#28839,#28840,#28841,#28842,#28843,#28844,#28845,#28846,#28847,
#28848,#28849,#28850,#28851,#28852,#28853,#28854,#28855,#28856,#28857,#28858,
#28859,#28860,#28861,#28862,#28863,#28864,#28865,#28866,#28867,#28868,#28869,
#28870,#28871,#28872,#28873,#28874,#28875,#28876,#28877,#28878,#28879,#28880,
#28881,#28882,#28883,#28884,#28885,#28886,#28887,#28888,#28889,#28890,#28891,
#28892,#28893,#28894,#28895,#28896,#28897,#28898,#28899,#28900,#28901,#28902,
#28903,#28904,#28905,#28906,#28907),.UNSPECIFIED.,.F.,.F.,(4,3,3,3,3,3,
3,3,3,3,3,3,3,3,3,3,3,3,3,3,3,3,3,3,3,4),(258.705668197138,258.788129800991,
258.870590738962,258.953051038448,259.035510726845,259.117969831547,259.200428379946,
259.282886399432,259.365343917394,259.452021813054,259.534488598889,259.616953712233,
259.699417262738,259.781879360036,259.864340113737,259.946799633435,260.029258028702,
260.111715409099,260.194181795366,260.276644997379,260.35910545366,260.441563602571,
260.52402920745,260.606489086665,260.688953200028,260.752190247953),
 .UNSPECIFIED.);
#270=B_SPLINE_CURVE_WITH_KNOTS('',3,(#28908,#28909,#28910,#28911,#28912,
#28913,#28914,#28915,#28916,#28917,#28918,#28919,#28920,#28921,#28922,#28923,
#28924,#28925,#28926,#28927,#28928,#28929,#28930,#28931,#28932,#28933,#28934,
#28935,#28936,#28937,#28938,#28939,#28940,#28941,#28942,#28943,#28944,#28945,
#28946,#28947,#28948,#28949,#28950,#28951,#28952,#28953,#28954,#28955,#28956,
#28957,#28958,#28959,#28960,#28961,#28962,#28963,#28964,#28965,#28966,#28967,
#28968,#28969,#28970,#28971,#28972,#28973,#28974,#28975,#28976,#28977,#28978,
#28979,#28980,#28981,#28982,#28983,#28984,#28985,#28986,#28987,#28988,#28989,
#28990,#28991,#28992,#28993,#28994,#28995,#28996,#28997,#28998,#28999,#29000,
#29001,#29002,#29003,#29004,#29005,#29006,#29007,#29008,#29009,#29010,#29011,
#29012,#29013,#29014,#29015,#29016,#29017,#29018,#29019,#29020,#29021,#29022,
#29023,#29024,#29025,#29026,#29027,#29028,#29029,#29030,#29031,#29032,#29033,
#29034,#29035,#29036,#29037,#29038,#29039,#29040,#29041,#29042,#29043,#29044,
#29045,#29046,#29047,#29048,#29049,#29050,#29051,#29052,#29053,#29054,#29055,
#29056,#29057,#29058,#29059,#29060,#29061,#29062,#29063,#29064,#29065,#29066,
#29067,#29068,#29069,#29070,#29071,#29072,#29073),.UNSPECIFIED.,.F.,.F.,
(4,3,3,3,3,3,3,3,3,3,3,3,3,3,3,3,3,3,3,3,3,3,3,3,3,3,3,3,3,3,3,3,3,3,3,
3,3,3,3,3,3,3,3,3,3,3,3,3,3,3,3,3,3,3,3,4),(260.752190247953,260.833508676024,
260.914959009631,260.996629128698,261.07841550255,261.160402427617,261.217034860549,
261.294564756422,261.372007551726,261.449378888063,261.526694355795,261.603969504918,
261.681230098028,261.758485117062,261.835748603716,261.913034601805,261.990401140851,
262.067809205046,262.145330499162,262.2154428686,262.29297242758,262.370414889339,
262.447785895736,262.525101037391,262.60237586456,262.679636142938,262.756890851673,
262.834154032701,262.911439730082,262.988805977652,263.066213754988,263.14373477266,
263.213850876651,263.290687299622,263.367434709828,263.444109345184,263.520727385502,
263.59730496563,263.674174205513,263.750734716384,263.827305423362,263.903900895436,
263.980990392753,264.057718000293,264.134988442497,264.212258884701,264.289866799726,
264.367379857018,264.444995213602,264.522354264186,264.599671172362,264.676959973276,
264.754795657381,264.832085034435,264.910193872066,264.988302709697),
 .UNSPECIFIED.);
#271=B_SPLINE_CURVE_WITH_KNOTS('',3,(#29079,#29080,#29081,#29082,#29083,
#29084,#29085,#29086,#29087,#29088,#29089,#29090,#29091,#29092,#29093,#29094,
#29095,#29096,#29097,#29098,#29099,#29100,#29101,#29102,#29103,#29104,#29105,
#29106,#29107,#29108,#29109,#29110,#29111,#29112,#29113,#29114,#29115,#29116,
#29117,#29118,#29119,#29120,#29121,#29122,#29123,#29124,#29125,#29126,#29127,
#29128,#29129,#29130,#29131,#29132,#29133,#29134,#29135,#29136,#29137,#29138,
#29139,#29140,#29141,#29142,#29143,#29144,#29145,#29146,#29147,#29148,#29149,
#29150,#29151,#29152,#29153,#29154,#29155,#29156,#29157,#29158,#29159,#29160,
#29161,#29162,#29163,#29164,#29165,#29166,#29167,#29168,#29169,#29170,#29171,
#29172,#29173,#29174,#29175,#29176,#29177,#29178,#29179,#29180,#29181,#29182,
#29183,#29184,#29185,#29186,#29187,#29188,#29189,#29190,#29191,#29192,#29193,
#29194,#29195,#29196,#29197,#29198,#29199,#29200,#29201,#29202,#29203,#29204,
#29205,#29206,#29207,#29208,#29209,#29210,#29211,#29212,#29213,#29214,#29215,
#29216,#29217,#29218,#29219,#29220,#29221,#29222,#29223,#29224,#29225,#29226,
#29227,#29228,#29229,#29230,#29231,#29232,#29233,#29234,#29235,#29236,#29237,
#29238,#29239,#29240,#29241,#29242,#29243,#29244,#29245,#29246,#29247),
 .UNSPECIFIED.,.F.,.F.,(4,3,3,3,3,3,3,3,3,3,3,3,3,3,3,3,3,3,3,3,3,3,3,3,
3,3,3,3,3,3,3,3,3,3,3,3,3,3,3,3,3,3,3,3,3,3,3,3,3,3,3,3,3,3,3,3,4),(267.035375555133,
267.144452834569,267.237314599293,267.314831961683,267.392262022246,267.469620436555,
267.546922808741,267.624184702416,267.701431905952,267.778673422974,267.855923307091,
267.933195613976,268.010548677938,268.087943200411,268.16545169814,268.237068210663,
268.313889409591,268.390621373587,268.467280353525,268.543882541783,268.620444085465,
268.697491302536,268.774035478986,268.850589760838,268.927168727623,269.004582001225,
269.081293483321,269.159057652676,269.236821822032,269.31440444721,269.391894430998,
269.469307409814,269.546658964918,269.623964633442,269.701247228109,269.77851901668,
269.855794018169,269.933086250741,270.010450924736,270.087852534799,270.165360351022,
270.236575433401,270.318059401026,270.399438759856,270.483692129663,270.564845619648,
270.64592229249,270.726907715281,270.736452239086,270.817460637931,270.89854489779,
270.982990934535,271.064297019422,271.145680812412,271.227185476696,271.236329044771,
271.272326787262),.UNSPECIFIED.);
#272=B_SPLINE_CURVE_WITH_KNOTS('',3,(#29248,#29249,#29250,#29251,#29252,
#29253,#29254,#29255,#29256,#29257,#29258,#29259,#29260,#29261,#29262,#29263,
#29264,#29265,#29266,#29267,#29268,#29269,#29270,#29271,#29272,#29273,#29274,
#29275,#29276,#29277,#29278,#29279,#29280,#29281,#29282,#29283,#29284,#29285,
#29286,#29287,#29288,#29289,#29290,#29291,#29292,#29293,#29294,#29295,#29296,
#29297,#29298,#29299,#29300,#29301,#29302,#29303,#29304,#29305,#29306,#29307,
#29308,#29309,#29310,#29311,#29312,#29313,#29314,#29315,#29316,#29317,#29318,
#29319,#29320,#29321,#29322,#29323,#29324,#29325,#29326,#29327,#29328,#29329,
#29330,#29331,#29332),.UNSPECIFIED.,.F.,.F.,(4,3,3,3,3,3,3,3,3,3,3,3,3,
3,3,3,3,3,3,3,3,3,3,3,3,3,3,3,4),(264.988317180418,265.065754055233,265.143245580455,
265.220842788067,265.237807376555,265.31465601182,265.391410870359,265.468088221961,
265.544704273979,265.621275184883,265.698310910263,265.774853341281,265.851401690157,
265.92797053391,266.005368147414,266.082059240563,266.159810114243,266.237560987924,
266.314064343492,266.390479740073,266.46682368928,266.543107292491,266.619357978181,
266.695590567042,266.771819865679,266.848086066066,266.924373142649,267.000726718474,
267.035375555007),.UNSPECIFIED.);
#273=B_SPLINE_CURVE_WITH_KNOTS('',3,(#29334,#29335,#29336,#29337,#29338,
#29339,#29340,#29341,#29342,#29343,#29344,#29345,#29346,#29347,#29348,#29349,
#29350,#29351,#29352,#29353,#29354,#29355,#29356,#29357,#29358,#29359,#29360,
#29361,#29362,#29363,#29364,#29365,#29366,#29367,#29368,#29369,#29370,#29371,
#29372,#29373,#29374,#29375,#29376,#29377,#29378,#29379,#29380,#29381,#29382,
#29383,#29384,#29385,#29386,#29387,#29388,#29389,#29390,#29391,#29392,#29393,
#29394,#29395,#29396,#29397,#29398,#29399,#29400,#29401,#29402,#29403,#29404,
#29405,#29406,#29407,#29408,#29409,#29410,#29411,#29412,#29413,#29414,#29415,
#29416,#29417,#29418),.UNSPECIFIED.,.F.,.F.,(4,3,3,3,3,3,3,3,3,3,3,3,3,
3,3,3,3,3,3,3,3,3,3,3,3,3,3,3,4),(264.988302709697,265.065719049362,265.143240355639,
265.210666892752,265.292152799803,265.373534475164,265.457618580567,265.53877549918,
265.619855887071,265.700845490964,265.709870896778,265.790884280144,265.871973260509,
265.956248670583,266.037558439693,266.118945648338,266.200453098809,266.209074900803,
266.285179233415,266.361201935431,266.437159715668,266.513068483997,266.588951011644,
266.664822302395,266.740697350382,266.816626102046,266.892581841232,266.968628479594,
267.034597505135),.UNSPECIFIED.);
#274=B_SPLINE_CURVE_WITH_KNOTS('',3,(#29419,#29420,#29421,#29422,#29423,
#29424,#29425,#29426,#29427,#29428,#29429,#29430,#29431,#29432,#29433,#29434,
#29435,#29436,#29437,#29438,#29439,#29440,#29441,#29442,#29443,#29444,#29445,
#29446,#29447,#29448,#29449,#29450,#29451,#29452,#29453,#29454,#29455,#29456,
#29457,#29458,#29459,#29460,#29461,#29462,#29463,#29464,#29465,#29466,#29467,
#29468,#29469,#29470,#29471,#29472,#29473,#29474,#29475,#29476,#29477,#29478,
#29479,#29480,#29481,#29482,#29483,#29484,#29485,#29486,#29487,#29488,#29489,
#29490,#29491,#29492,#29493,#29494,#29495,#29496,#29497,#29498,#29499,#29500,
#29501,#29502,#29503,#29504,#29505,#29506,#29507,#29508,#29509,#29510,#29511,
#29512,#29513,#29514,#29515,#29516,#29517,#29518,#29519,#29520,#29521,#29522,
#29523,#29524,#29525,#29526,#29527,#29528,#29529,#29530,#29531,#29532,#29533,
#29534,#29535,#29536,#29537,#29538,#29539,#29540,#29541,#29542,#29543,#29544,
#29545,#29546,#29547,#29548,#29549,#29550,#29551,#29552,#29553,#29554,#29555,
#29556,#29557,#29558,#29559,#29560,#29561,#29562,#29563,#29564,#29565,#29566,
#29567,#29568,#29569,#29570,#29571,#29572,#29573,#29574,#29575),
 .UNSPECIFIED.,.F.,.F.,(4,3,3,3,3,3,3,3,3,3,3,3,3,3,3,3,3,3,3,3,3,3,3,3,
3,3,3,3,3,3,3,3,3,3,3,3,3,3,3,3,3,3,3,3,3,3,3,3,3,3,3,3,4),(267.035375555133,
267.117837761169,267.200299618909,267.282761135203,267.3652223169,267.447683170851,
267.530143703906,267.612603922912,267.69506383472,267.777523446178,267.859982764134,
267.942441795436,268.024900546933,268.107359025471,268.189817237899,268.272275191063,
268.354732891811,268.437190346989,268.519647563443,268.605659789945,268.688984134369,
268.771450739814,268.853916501055,268.936381445508,269.018845600584,269.101308993693,
269.183771652241,269.266233603634,269.348694875273,269.431155494557,269.513615488884,
269.596074885648,269.678533712244,269.76099199606,269.843449764488,269.925907044913,
270.010040280324,270.092506278416,270.174970654772,270.257433519034,270.339894980824,
270.422355149746,270.504814135381,270.587272047298,270.672867892823,270.755332629423,
270.837794401425,270.920253647267,271.002710805245,271.085173323526,271.167630994381,
271.250089784331,271.272038811497),.UNSPECIFIED.);
#275=B_SPLINE_CURVE_WITH_KNOTS('',3,(#29581,#29582,#29583,#29584,#29585,
#29586,#29587,#29588,#29589,#29590,#29591,#29592,#29593,#29594,#29595,#29596,
#29597,#29598,#29599,#29600,#29601,#29602,#29603,#29604,#29605,#29606,#29607,
#29608,#29609,#29610,#29611,#29612,#29613,#29614,#29615,#29616,#29617,#29618,
#29619,#29620,#29621,#29622,#29623,#29624,#29625,#29626,#29627,#29628,#29629,
#29630,#29631,#29632,#29633,#29634,#29635,#29636,#29637,#29638,#29639,#29640,
#29641,#29642,#29643,#29644,#29645,#29646,#29647,#29648,#29649,#29650,#29651,
#29652,#29653,#29654,#29655,#29656,#29657,#29658,#29659,#29660,#29661,#29662,
#29663,#29664,#29665,#29666,#29667,#29668,#29669,#29670,#29671,#29672,#29673,
#29674,#29675,#29676,#29677,#29678,#29679,#29680,#29681,#29682,#29683,#29684,
#29685,#29686,#29687,#29688,#29689,#29690,#29691,#29692,#29693,#29694,#29695,
#29696,#29697,#29698,#29699,#29700,#29701,#29702,#29703,#29704,#29705,#29706,
#29707,#29708,#29709,#29710,#29711,#29712,#29713,#29714,#29715,#29716,#29717,
#29718,#29719,#29720,#29721,#29722,#29723,#29724,#29725,#29726,#29727,#29728,
#29729,#29730,#29731,#29732,#29733,#29734,#29735,#29736,#29737,#29738,#29739,
#29740,#29741,#29742,#29743,#29744,#29745,#29746),.UNSPECIFIED.,.F.,.F.,
(4,3,3,3,3,3,3,3,3,3,3,3,3,3,3,3,3,3,3,3,3,3,3,3,3,3,3,3,3,3,3,3,3,3,3,
3,3,3,3,3,3,3,3,3,3,3,3,3,3,3,3,3,3,3,3,4),(273.318560862452,273.395142880457,
273.471642911441,273.548077363806,273.624462590287,273.700853501361,273.777200930976,
273.853550909225,273.929918174114,274.006361413199,274.082842797132,274.15943777032,
274.235589878879,274.313107248038,274.390537315452,274.467895736685,274.545198115862,
274.622460016587,274.69970722724,274.77694875142,274.854198642728,274.931470956833,
275.008824028021,275.086218557734,275.163727062659,275.235343490248,275.312164687398,
275.388896649607,275.465555627749,275.542157814205,275.61871935608,275.695766574272,
275.77231074891,275.84886502895,275.925443993923,276.002857270847,276.079568751148,
276.157332926383,276.235097101618,276.31267972525,276.390169707476,276.467582684719,
276.544934238238,276.622239905168,276.699522498231,276.776794285192,276.854069285067,
276.931361516023,277.008726188406,277.086127796857,277.163635611483,277.234850712987,
277.316315177658,277.397686217241,277.478930272538,277.55569081987),
 .UNSPECIFIED.);
#276=B_SPLINE_CURVE_WITH_KNOTS('',3,(#29747,#29748,#29749,#29750,#29751,
#29752,#29753,#29754,#29755,#29756,#29757,#29758,#29759,#29760,#29761,#29762,
#29763,#29764,#29765,#29766,#29767,#29768,#29769,#29770,#29771,#29772,#29773,
#29774,#29775,#29776,#29777,#29778,#29779,#29780,#29781,#29782,#29783,#29784,
#29785,#29786,#29787,#29788,#29789,#29790,#29791,#29792,#29793,#29794,#29795,
#29796,#29797,#29798,#29799,#29800,#29801,#29802,#29803,#29804,#29805,#29806,
#29807,#29808,#29809,#29810,#29811,#29812,#29813,#29814,#29815,#29816,#29817,
#29818,#29819,#29820,#29821,#29822,#29823,#29824,#29825,#29826,#29827,#29828),
 .UNSPECIFIED.,.F.,.F.,(4,3,3,3,3,3,3,3,3,3,3,3,3,3,3,3,3,3,3,3,3,3,3,3,
3,3,3,4),(271.272326787262,271.349802796202,271.427204574214,271.504547693917,
271.581847685763,271.659120048451,271.736395155182,271.813676265128,271.890977398363,
271.968312583541,272.045738465872,272.123216012992,272.200804181388,272.23608265614,
272.31293127929,272.389686125647,272.466363465012,272.542979504746,272.619550403329,
272.696586136352,272.773128555014,272.849676891532,272.926245722935,273.003643359079,
273.080334439985,273.158085353747,273.23583626751,273.318560862313),
 .UNSPECIFIED.);
#277=B_SPLINE_CURVE_WITH_KNOTS('',3,(#29830,#29831,#29832,#29833,#29834,
#29835,#29836,#29837,#29838,#29839,#29840,#29841,#29842,#29843,#29844,#29845,
#29846,#29847,#29848,#29849,#29850,#29851,#29852,#29853,#29854,#29855,#29856,
#29857,#29858,#29859,#29860,#29861,#29862,#29863,#29864,#29865,#29866,#29867,
#29868,#29869,#29870,#29871,#29872,#29873,#29874,#29875,#29876,#29877,#29878,
#29879,#29880,#29881,#29882,#29883,#29884,#29885,#29886,#29887,#29888,#29889,
#29890,#29891,#29892,#29893,#29894,#29895,#29896,#29897,#29898,#29899,#29900,
#29901,#29902,#29903,#29904,#29905),.UNSPECIFIED.,.F.,.F.,(4,3,3,3,3,3,
3,3,3,3,3,3,3,3,3,3,3,3,3,3,3,3,3,3,3,4),(271.272038811497,271.354500415351,
271.436961353322,271.519421652807,271.601881341204,271.684340445906,271.766798994306,
271.849257013792,271.931714531753,272.018392427413,272.100859213249,272.183324326593,
272.265787877098,272.348249974396,272.430710728097,272.513170247794,272.595628643062,
272.678086023459,272.760552409725,272.843015611739,272.92547606802,273.007934216931,
273.09039982181,273.172859701024,273.255323814388,273.318560862313),
 .UNSPECIFIED.);
#278=B_SPLINE_CURVE_WITH_KNOTS('',3,(#29906,#29907,#29908,#29909,#29910,
#29911,#29912,#29913,#29914,#29915,#29916,#29917,#29918,#29919,#29920,#29921,
#29922,#29923,#29924,#29925,#29926,#29927,#29928,#29929,#29930,#29931,#29932,
#29933,#29934,#29935,#29936,#29937,#29938,#29939,#29940,#29941,#29942,#29943,
#29944,#29945,#29946,#29947,#29948,#29949,#29950,#29951,#29952,#29953,#29954,
#29955,#29956,#29957,#29958,#29959,#29960,#29961,#29962,#29963,#29964,#29965,
#29966,#29967,#29968,#29969,#29970,#29971,#29972,#29973,#29974,#29975,#29976,
#29977,#29978,#29979,#29980,#29981,#29982,#29983,#29984,#29985,#29986,#29987,
#29988,#29989,#29990,#29991,#29992,#29993,#29994,#29995,#29996,#29997,#29998,
#29999,#30000,#30001,#30002,#30003,#30004,#30005,#30006,#30007,#30008,#30009,
#30010,#30011,#30012,#30013,#30014,#30015,#30016,#30017,#30018,#30019,#30020,
#30021,#30022,#30023,#30024,#30025,#30026,#30027,#30028,#30029,#30030,#30031,
#30032,#30033,#30034,#30035,#30036,#30037,#30038,#30039,#30040,#30041,#30042,
#30043,#30044,#30045,#30046,#30047,#30048,#30049,#30050,#30051,#30052,#30053,
#30054,#30055,#30056,#30057,#30058,#30059,#30060,#30061,#30062,#30063,#30064,
#30065,#30066,#30067,#30068,#30069,#30070,#30071,#30072,#30073,#30074),
 .UNSPECIFIED.,.F.,.F.,(4,3,3,3,3,3,3,3,3,3,3,3,3,3,3,3,3,3,3,3,3,3,3,3,
3,3,3,3,3,3,3,3,3,3,3,3,3,3,3,3,3,3,3,3,3,3,3,3,3,3,3,3,3,3,3,3,4),(273.319207559223,
273.395811164144,273.472346602566,273.548830171782,273.62527812616,273.701718887028,
273.778159754071,273.854615409225,273.931100541588,274.007671395534,274.084291096307,
274.161018943372,274.196338965211,274.273202349841,274.349972181628,274.426664717593,
274.503296152736,274.579882633495,274.656740675966,274.733298998903,274.809863333548,
274.886448246649,274.963522928302,275.040229749143,275.117488361202,275.194746973262,
275.272277169792,275.349720264468,275.427091898596,275.504407662237,275.581683105089,
275.658943987583,275.736199293302,275.813463063672,275.890749342232,275.9681161551,
276.045524489883,276.123046046522,276.193154981312,276.270685099344,276.348128128628,
276.425499710421,276.502815434749,276.580090851278,276.657351727271,276.734607038584,
276.811870826643,276.889157134995,276.966523996568,277.043932390467,277.121454023307,
277.191562989363,277.268414568166,277.345153547054,277.421827869475,277.498442284338,
277.555563663649),.UNSPECIFIED.);
#279=B_SPLINE_CURVE_WITH_KNOTS('',3,(#30080,#30081,#30082,#30083,#30084,
#30085,#30086,#30087,#30088,#30089,#30090,#30091,#30092,#30093,#30094,#30095,
#30096,#30097,#30098,#30099,#30100,#30101,#30102,#30103,#30104,#30105,#30106,
#30107,#30108,#30109,#30110,#30111,#30112,#30113,#30114,#30115,#30116,#30117,
#30118,#30119,#30120,#30121,#30122,#30123,#30124,#30125,#30126,#30127,#30128,
#30129,#30130,#30131,#30132,#30133,#30134,#30135,#30136,#30137,#30138,#30139,
#30140,#30141,#30142,#30143,#30144,#30145,#30146,#30147,#30148,#30149,#30150,
#30151,#30152,#30153,#30154,#30155,#30156,#30157,#30158,#30159,#30160,#30161,
#30162,#30163,#30164,#30165,#30166,#30167,#30168,#30169,#30170,#30171,#30172,
#30173,#30174,#30175,#30176,#30177,#30178,#30179,#30180,#30181,#30182,#30183,
#30184,#30185,#30186,#30187,#30188,#30189,#30190,#30191,#30192,#30193,#30194,
#30195,#30196,#30197,#30198,#30199,#30200,#30201,#30202,#30203,#30204,#30205,
#30206,#30207,#30208,#30209,#30210,#30211,#30212,#30213,#30214,#30215,#30216,
#30217,#30218,#30219,#30220,#30221,#30222,#30223,#30224,#30225,#30226,#30227,
#30228,#30229,#30230,#30231,#30232,#30233,#30234,#30235,#30236),
 .UNSPECIFIED.,.F.,.F.,(4,3,3,3,3,3,3,3,3,3,3,3,3,3,3,3,3,3,3,3,3,3,3,3,
3,3,3,3,3,3,3,3,3,3,3,3,3,3,3,3,3,3,3,3,3,3,3,3,3,3,3,3,4),(279.601746169492,
279.684208375528,279.766670233268,279.849131749562,279.931592931259,280.01405378521,
280.096514318265,280.178974537271,280.261434449079,280.343894060537,280.426353378493,
280.508812409795,280.591271161292,280.67372963983,280.756187852258,280.838645805422,
280.92110350617,281.003560961348,281.086018177803,281.172030404304,281.255354748728,
281.337821354173,281.420287115415,281.502752059867,281.585216214943,281.667679608052,
281.750142266601,281.832604217993,281.915065489632,281.997526108916,282.079986103243,
282.162445500008,282.244904326603,282.32736261042,282.409820378847,282.492277659272,
282.576410894684,282.658876892776,282.741341269131,282.823804133393,282.906265595184,
282.988725764105,283.071184749741,283.153642661658,283.239238507183,283.321703243783,
283.404165015785,283.486624261627,283.569081419604,283.651543937885,283.73400160874,
283.816460398691,283.838409425857),.UNSPECIFIED.);
#280=B_SPLINE_CURVE_WITH_KNOTS('',3,(#30237,#30238,#30239,#30240,#30241,
#30242,#30243,#30244,#30245,#30246,#30247,#30248,#30249,#30250,#30251,#30252,
#30253,#30254,#30255,#30256,#30257,#30258,#30259,#30260,#30261,#30262,#30263,
#30264,#30265,#30266,#30267,#30268,#30269,#30270,#30271,#30272,#30273,#30274,
#30275,#30276,#30277,#30278,#30279,#30280,#30281,#30282,#30283,#30284,#30285,
#30286,#30287,#30288,#30289,#30290,#30291,#30292,#30293,#30294,#30295,#30296,
#30297,#30298,#30299,#30300,#30301,#30302,#30303,#30304,#30305,#30306,#30307,
#30308,#30309,#30310,#30311,#30312,#30313,#30314,#30315,#30316,#30317,#30318,
#30319,#30320,#30321),.UNSPECIFIED.,.F.,.F.,(4,3,3,3,3,3,3,3,3,3,3,3,3,
3,3,3,3,3,3,3,3,3,3,3,3,3,3,3,4),(277.55569081987,277.636774286884,277.717764514931,
277.734727518672,277.81573591459,277.896820171437,277.981266209667,278.062572291388,
278.143956081171,278.225460742215,278.234604324356,278.312120102618,278.389554403028,
278.466922821455,278.544240906604,278.621524170649,278.69880125496,278.776077835447,
278.853367930843,278.930685564847,279.008091771171,279.085543780483,279.163116588805,
279.234357935726,279.326204994167,279.413442625825,279.500358458254,279.586782436634,
279.601746169492),.UNSPECIFIED.);
#281=B_SPLINE_CURVE_WITH_KNOTS('',3,(#30323,#30324,#30325,#30326,#30327,
#30328,#30329,#30330,#30331,#30332,#30333,#30334,#30335,#30336,#30337,#30338,
#30339,#30340,#30341,#30342,#30343,#30344,#30345,#30346,#30347,#30348,#30349,
#30350,#30351,#30352,#30353,#30354,#30355,#30356,#30357,#30358,#30359,#30360,
#30361,#30362,#30363,#30364,#30365,#30366,#30367,#30368,#30369,#30370,#30371,
#30372,#30373,#30374,#30375,#30376,#30377,#30378,#30379,#30380,#30381,#30382,
#30383,#30384,#30385,#30386,#30387,#30388,#30389,#30390,#30391,#30392,#30393,
#30394,#30395,#30396,#30397,#30398,#30399,#30400,#30401,#30402,#30403,#30404),
 .UNSPECIFIED.,.F.,.F.,(4,3,3,3,3,3,3,3,3,3,3,3,3,3,3,3,3,3,3,3,3,3,3,3,
3,3,3,4),(277.555563663649,277.63486458037,277.711424395415,277.787991167071,
277.864579462952,277.941203861465,278.017919785118,278.094690191056,278.171567907073,
278.189970997414,278.267565666862,278.345067932986,278.422493418071,278.499857689461,
278.577176270567,278.654471975053,278.731757019723,278.80904541167,278.88635115721,
278.963729197212,279.041144268971,279.118664883257,279.188379005465,279.272860664689,
279.357122338694,279.441244749164,279.525133664988,279.601746169492),
 .UNSPECIFIED.);
#282=B_SPLINE_CURVE_WITH_KNOTS('',3,(#30405,#30406,#30407,#30408,#30409,
#30410,#30411,#30412,#30413,#30414,#30415,#30416,#30417,#30418,#30419,#30420,
#30421,#30422,#30423,#30424,#30425,#30426,#30427,#30428,#30429,#30430,#30431,
#30432,#30433,#30434,#30435,#30436,#30437,#30438,#30439,#30440,#30441,#30442,
#30443,#30444,#30445,#30446,#30447,#30448,#30449,#30450,#30451,#30452,#30453,
#30454,#30455,#30456,#30457,#30458,#30459,#30460,#30461,#30462,#30463,#30464,
#30465,#30466,#30467,#30468,#30469,#30470,#30471,#30472,#30473,#30474,#30475,
#30476,#30477,#30478,#30479,#30480,#30481,#30482,#30483,#30484,#30485,#30486,
#30487,#30488,#30489,#30490,#30491,#30492,#30493,#30494,#30495,#30496,#30497,
#30498,#30499,#30500,#30501,#30502,#30503,#30504,#30505,#30506,#30507,#30508,
#30509,#30510,#30511,#30512,#30513,#30514,#30515,#30516,#30517,#30518,#30519,
#30520,#30521,#30522,#30523,#30524,#30525,#30526,#30527,#30528,#30529,#30530,
#30531,#30532,#30533,#30534,#30535,#30536,#30537,#30538,#30539,#30540,#30541,
#30542,#30543,#30544,#30545,#30546,#30547,#30548,#30549,#30550,#30551,#30552,
#30553,#30554,#30555,#30556,#30557,#30558,#30559,#30560,#30561),
 .UNSPECIFIED.,.F.,.F.,(4,3,3,3,3,3,3,3,3,3,3,3,3,3,3,3,3,3,3,3,3,3,3,3,
3,3,3,3,3,3,3,3,3,3,3,3,3,3,3,3,3,3,3,3,3,3,3,3,3,3,3,3,4),(279.601746169492,
279.684208375528,279.766670233268,279.849131749562,279.931592931259,280.01405378521,
280.096514318265,280.178974537271,280.261434449079,280.343894060537,280.426353378493,
280.508812409795,280.591271161292,280.67372963983,280.756187852258,280.838645805422,
280.92110350617,281.003560961348,281.086018177803,281.172030404304,281.255354748728,
281.337821354173,281.420287115415,281.502752059867,281.585216214943,281.667679608052,
281.750142266601,281.832604217993,281.915065489632,281.997526108916,282.079986103243,
282.162445500008,282.244904326603,282.32736261042,282.409820378847,282.492277659272,
282.576410894684,282.658876892775,282.741341269131,282.823804133393,282.906265595184,
282.988725764105,283.071184749741,283.153642661658,283.239238507183,283.321703243783,
283.404165015785,283.486624261627,283.569081419604,283.651543937885,283.73400160874,
283.816460398691,283.838409425856),.UNSPECIFIED.);
#283=B_SPLINE_CURVE_WITH_KNOTS('',3,(#30567,#30568,#30569,#30570,#30571,
#30572,#30573,#30574,#30575,#30576,#30577,#30578,#30579,#30580,#30581,#30582,
#30583,#30584,#30585,#30586,#30587,#30588,#30589,#30590,#30591,#30592,#30593,
#30594,#30595,#30596,#30597,#30598,#30599,#30600,#30601,#30602,#30603,#30604,
#30605,#30606,#30607,#30608,#30609,#30610,#30611,#30612,#30613,#30614,#30615,
#30616,#30617,#30618,#30619,#30620,#30621,#30622,#30623,#30624,#30625,#30626,
#30627,#30628,#30629,#30630,#30631,#30632,#30633,#30634,#30635,#30636,#30637,
#30638,#30639,#30640,#30641,#30642,#30643,#30644,#30645,#30646,#30647,#30648,
#30649,#30650,#30651,#30652,#30653,#30654,#30655,#30656,#30657,#30658,#30659,
#30660,#30661,#30662,#30663,#30664,#30665,#30666,#30667,#30668,#30669,#30670,
#30671,#30672,#30673,#30674,#30675,#30676,#30677,#30678,#30679,#30680,#30681,
#30682,#30683,#30684,#30685,#30686,#30687,#30688,#30689,#30690,#30691,#30692,
#30693,#30694,#30695,#30696,#30697,#30698,#30699,#30700,#30701,#30702,#30703,
#30704,#30705,#30706,#30707,#30708,#30709,#30710,#30711,#30712,#30713,#30714,
#30715,#30716,#30717,#30718,#30719,#30720,#30721,#30722,#30723,#30724,#30725,
#30726,#30727,#30728,#30729,#30730,#30731,#30732),.UNSPECIFIED.,.F.,.F.,
(4,3,3,3,3,3,3,3,3,3,3,3,3,3,3,3,3,3,3,3,3,3,3,3,3,3,3,3,3,3,3,3,3,3,3,
3,3,3,3,3,3,3,3,3,3,3,3,3,3,3,3,3,3,3,3,4),(285.884931476672,285.975939179837,
286.067542544567,286.159888532299,286.232633215311,286.309481838498,286.386236684895,
286.462914024299,286.539530064074,286.616100962699,286.693136695697,286.769679114403,
286.846227450965,286.922796282413,287.00019391848,287.076884999432,287.154635913057,
287.232386826681,287.309904378299,287.387334597719,287.464693140614,287.541995611201,
287.619257573152,287.696504798934,287.773746310141,287.850996160374,287.928268405287,
288.005621363258,288.083015755567,288.160524083235,288.23214043805,288.309657807246,
288.387087874697,288.464446295967,288.541748675182,288.619010575945,288.696257786636,
288.773499310854,288.8507492022,288.928021516344,289.00537458757,289.082769117321,
289.160277622283,289.231894049419,289.308721255141,289.385457937991,289.462120354592,
289.538724701759,289.615288304219,289.691830941501,289.768367193544,289.844911634042,
289.92151149413,289.998141634467,290.074856761555,290.120845093709),
 .UNSPECIFIED.);
#284=B_SPLINE_CURVE_WITH_KNOTS('',3,(#30733,#30734,#30735,#30736,#30737,
#30738,#30739,#30740,#30741,#30742,#30743,#30744,#30745,#30746,#30747,#30748,
#30749,#30750,#30751,#30752,#30753,#30754,#30755,#30756,#30757,#30758,#30759,
#30760,#30761,#30762,#30763,#30764,#30765,#30766,#30767,#30768,#30769,#30770,
#30771,#30772,#30773,#30774,#30775,#30776,#30777,#30778,#30779,#30780,#30781,
#30782,#30783,#30784,#30785,#30786,#30787,#30788,#30789,#30790,#30791,#30792,
#30793,#30794,#30795,#30796,#30797,#30798,#30799,#30800,#30801,#30802,#30803,
#30804,#30805,#30806,#30807,#30808),.UNSPECIFIED.,.F.,.F.,(4,3,3,3,3,3,
3,3,3,3,3,3,3,3,3,3,3,3,3,3,3,3,3,3,3,4),(283.838409425857,283.92087102971,
284.003331967681,284.085792267167,284.168251955563,284.250711060266,284.333169608665,
284.415627628151,284.498085146113,284.584763041773,284.667229827608,284.749694940952,
284.832158491457,284.914620588755,284.997081342456,285.079540862153,285.161999257421,
285.244456637818,285.326923024085,285.409386226098,285.491846682379,285.57430483129,
285.656770436169,285.739230315383,285.821694428747,285.884931476672),
 .UNSPECIFIED.);
#285=B_SPLINE_CURVE_WITH_KNOTS('',3,(#30810,#30811,#30812,#30813,#30814,
#30815,#30816,#30817,#30818,#30819,#30820,#30821,#30822,#30823,#30824,#30825,
#30826,#30827,#30828,#30829,#30830,#30831,#30832,#30833,#30834,#30835,#30836,
#30837,#30838,#30839,#30840,#30841,#30842,#30843,#30844,#30845,#30846,#30847,
#30848,#30849,#30850,#30851,#30852,#30853,#30854,#30855,#30856,#30857,#30858,
#30859,#30860,#30861,#30862,#30863,#30864,#30865,#30866,#30867,#30868,#30869,
#30870,#30871,#30872,#30873,#30874,#30875,#30876,#30877,#30878,#30879,#30880,
#30881,#30882,#30883,#30884,#30885),.UNSPECIFIED.,.F.,.F.,(4,3,3,3,3,3,
3,3,3,3,3,3,3,3,3,3,3,3,3,3,3,3,3,3,3,4),(283.838409425856,283.92087102971,
284.003331967681,284.085792267167,284.168251955563,284.250711060265,284.333169608665,
284.415627628151,284.498085146112,284.584763041772,284.667229827608,284.749694940952,
284.832158491457,284.914620588755,284.997081342456,285.079540862153,285.161999257421,
285.244456637818,285.326923024085,285.409386226098,285.491846682379,285.574304831289,
285.656770436169,285.739230315383,285.821694428747,285.884931476672),
 .UNSPECIFIED.);
#286=B_SPLINE_CURVE_WITH_KNOTS('',3,(#30886,#30887,#30888,#30889,#30890,
#30891,#30892,#30893,#30894),.UNSPECIFIED.,.F.,.F.,(4,1,1,1,1,1,4),(285.884931476672,
286.177235061822,286.676439065847,287.175643069873,288.174051077923,289.172459085974,
290.121294042707),.UNSPECIFIED.);
#287=B_SPLINE_CURVE_WITH_KNOTS('',3,(#30900,#30901,#30902,#30903,#30904,
#30905,#30906,#30907,#30908,#30909,#30910,#30911,#30912,#30913,#30914,#30915,
#30916,#30917,#30918,#30919,#30920,#30921,#30922,#30923,#30924,#30925,#30926,
#30927,#30928,#30929,#30930,#30931,#30932,#30933,#30934,#30935,#30936,#30937,
#30938,#30939,#30940,#30941,#30942,#30943,#30944,#30945,#30946,#30947,#30948,
#30949,#30950,#30951,#30952,#30953,#30954,#30955,#30956,#30957,#30958,#30959,
#30960,#30961,#30962,#30963,#30964,#30965,#30966,#30967,#30968,#30969,#30970,
#30971,#30972,#30973,#30974,#30975,#30976,#30977,#30978,#30979,#30980,#30981,
#30982,#30983,#30984,#30985,#30986,#30987,#30988,#30989,#30990,#30991,#30992,
#30993,#30994,#30995,#30996,#30997,#30998,#30999,#31000,#31001,#31002,#31003,
#31004,#31005,#31006,#31007,#31008,#31009,#31010,#31011,#31012,#31013,#31014,
#31015,#31016,#31017,#31018,#31019,#31020,#31021,#31022,#31023,#31024,#31025,
#31026,#31027,#31028,#31029,#31030,#31031,#31032,#31033,#31034,#31035,#31036,
#31037,#31038,#31039,#31040,#31041,#31042,#31043,#31044,#31045,#31046,#31047,
#31048,#31049,#31050,#31051,#31052,#31053,#31054,#31055,#31056,#31057,#31058,
#31059,#31060,#31061,#31062,#31063,#31064,#31065,#31066,#31067,#31068),
 .UNSPECIFIED.,.F.,.F.,(4,3,3,3,3,3,3,3,3,3,3,3,3,3,3,3,3,3,3,3,3,3,3,3,
3,3,3,3,3,3,3,3,3,3,3,3,3,3,3,3,3,3,3,3,3,3,3,3,3,3,3,3,3,3,3,3,4),(292.168116783851,
292.231154883527,292.30867066179,292.386104962201,292.463473380628,292.540791465778,
292.618074729823,292.695351814134,292.772628394622,292.849918490019,292.927236124024,
293.004642330348,293.082094339661,293.159667147983,293.230908494897,293.307757118085,
293.384511964481,293.461189303886,293.537805343661,293.614376242286,293.691411975283,
293.767954393989,293.844502730552,293.921071561999,293.998469198066,294.075160279019,
294.152911192642,294.230662106266,294.308179657884,294.385609877304,294.462968420199,
294.540270890786,294.617532852736,294.694780078519,294.772021589726,294.849271439959,
294.926543684872,295.003896642843,295.081291035152,295.15879936282,295.230415717636,
295.307933086832,295.385363154283,295.462721575553,295.540023954768,295.617285855531,
295.694533066222,295.77177459044,295.849024481786,295.92629679593,296.003649867156,
296.081044396907,296.158552901869,296.230169329005,296.307007919613,296.383745713197,
296.405440486054),.UNSPECIFIED.);
#288=B_SPLINE_CURVE_WITH_KNOTS('',3,(#31069,#31070,#31071,#31072,#31073,
#31074,#31075,#31076,#31077,#31078,#31079,#31080,#31081,#31082,#31083,#31084,
#31085,#31086,#31087,#31088,#31089,#31090,#31091,#31092,#31093,#31094,#31095,
#31096,#31097,#31098,#31099,#31100,#31101,#31102,#31103,#31104,#31105,#31106,
#31107,#31108,#31109,#31110,#31111,#31112,#31113,#31114,#31115,#31116,#31117,
#31118,#31119,#31120,#31121,#31122,#31123,#31124,#31125,#31126,#31127,#31128,
#31129,#31130,#31131,#31132,#31133,#31134,#31135,#31136,#31137,#31138,#31139,
#31140,#31141,#31142,#31143,#31144,#31145,#31146,#31147,#31148,#31149,#31150,
#31151,#31152,#31153),.UNSPECIFIED.,.F.,.F.,(4,3,3,3,3,3,3,3,3,3,3,3,3,
3,3,3,3,3,3,3,3,3,3,3,3,3,3,3,4),(290.120845093709,290.197700313849,290.231647660789,
290.309230284403,290.386720266612,290.464133243837,290.541484797339,290.61879046425,
290.696073057295,290.773344844239,290.850619844096,290.927912075034,291.005276747399,
291.082678355831,291.160186170439,291.231401272158,291.312885245113,291.394264609253,
291.4785179764,291.559671471572,291.640748149531,291.721733577321,291.731278077843,
291.809987718527,291.888741433474,291.967597102425,292.046509246341,292.125538329813,
292.16811678375),.UNSPECIFIED.);
#289=B_SPLINE_CURVE_WITH_KNOTS('',3,(#31155,#31156,#31157,#31158,#31159,
#31160),.UNSPECIFIED.,.F.,.F.,(4,1,1,4),(290.121294042707,290.170867094025,
291.169275102076,292.168116783851),.UNSPECIFIED.);
#290=B_SPLINE_CURVE_WITH_KNOTS('',3,(#31161,#31162,#31163,#31164,#31165,
#31166,#31167,#31168,#31169,#31170,#31171,#31172,#31173,#31174,#31175,#31176,
#31177,#31178,#31179,#31180,#31181,#31182,#31183,#31184,#31185,#31186,#31187,
#31188,#31189,#31190,#31191,#31192,#31193,#31194,#31195,#31196,#31197,#31198,
#31199,#31200,#31201,#31202,#31203,#31204,#31205,#31206,#31207,#31208,#31209,
#31210,#31211,#31212,#31213,#31214,#31215,#31216,#31217,#31218,#31219,#31220,
#31221,#31222,#31223,#31224,#31225,#31226,#31227,#31228,#31229,#31230,#31231,
#31232,#31233,#31234,#31235,#31236,#31237,#31238,#31239,#31240,#31241,#31242,
#31243,#31244,#31245,#31246,#31247,#31248,#31249,#31250,#31251,#31252,#31253,
#31254,#31255,#31256,#31257,#31258,#31259,#31260,#31261,#31262,#31263,#31264,
#31265,#31266,#31267,#31268,#31269,#31270,#31271,#31272,#31273,#31274,#31275,
#31276,#31277,#31278,#31279,#31280,#31281,#31282,#31283,#31284,#31285,#31286,
#31287,#31288,#31289,#31290,#31291,#31292,#31293,#31294,#31295,#31296,#31297,
#31298,#31299,#31300,#31301,#31302,#31303,#31304,#31305,#31306,#31307,#31308,
#31309,#31310,#31311,#31312,#31313,#31314,#31315,#31316,#31317,#31318,#31319,
#31320,#31321,#31322,#31323,#31324,#31325,#31326,#31327,#31328,#31329,#31330,
#31331,#31332),.UNSPECIFIED.,.F.,.F.,(4,3,3,3,3,3,3,3,3,3,3,3,3,3,3,3,3,
3,3,3,3,3,3,3,3,3,3,3,3,3,3,3,3,3,3,3,3,3,3,3,3,3,3,3,3,3,3,3,3,3,3,3,3,
3,3,3,3,4),(292.168116807891,292.245704681638,292.32320014403,292.40061882437,
292.477976296989,292.555288092261,292.632577034805,292.709855342602,292.787137029005,
292.864436106611,292.941807486204,293.019215943154,293.09672985486,293.166091118178,
293.247577432611,293.32895951497,293.413043416778,293.494200735631,293.575281519386,
293.65627151142,293.665295122204,293.746308228494,293.827396922767,293.911672473633,
293.992981940022,294.074368841233,294.155875979998,294.164499126229,294.242027279438,
294.319474154399,294.396855333107,294.474186350567,294.551482705398,294.628773005734,
294.706062913472,294.78336643547,294.860697583597,294.938117073418,295.01558243184,
295.093167818138,295.16290713428,295.239770518932,295.316540350742,295.39323288673,
295.469864321897,295.546450802681,295.623308845137,295.6998671681,295.776431502773,
295.8530164159,295.930091097508,296.006797918377,296.084056530354,296.161315142331,
296.238846498326,296.316301020837,296.393676769827,296.405239013614),
 .UNSPECIFIED.);
#291=B_SPLINE_CURVE_WITH_KNOTS('',3,(#31338,#31339,#31340,#31341,#31342,
#31343,#31344,#31345,#31346,#31347,#31348,#31349,#31350,#31351,#31352,#31353,
#31354,#31355,#31356,#31357,#31358,#31359,#31360,#31361,#31362,#31363,#31364,
#31365,#31366,#31367,#31368,#31369,#31370,#31371,#31372,#31373,#31374,#31375,
#31376,#31377,#31378,#31379,#31380,#31381,#31382,#31383,#31384,#31385,#31386,
#31387,#31388,#31389,#31390,#31391,#31392,#31393,#31394,#31395,#31396,#31397,
#31398,#31399,#31400,#31401,#31402,#31403,#31404,#31405,#31406,#31407,#31408,
#31409,#31410,#31411,#31412,#31413,#31414,#31415,#31416,#31417,#31418,#31419,
#31420,#31421,#31422,#31423,#31424,#31425,#31426,#31427,#31428,#31429,#31430,
#31431,#31432,#31433,#31434,#31435,#31436,#31437,#31438,#31439,#31440,#31441,
#31442,#31443,#31444,#31445,#31446,#31447,#31448,#31449,#31450,#31451,#31452,
#31453,#31454,#31455,#31456,#31457,#31458,#31459,#31460,#31461,#31462,#31463,
#31464,#31465,#31466,#31467,#31468,#31469,#31470,#31471,#31472,#31473,#31474,
#31475,#31476,#31477,#31478,#31479,#31480,#31481,#31482,#31483,#31484,#31485,
#31486,#31487,#31488,#31489,#31490,#31491,#31492,#31493,#31494,#31495,#31496,
#31497,#31498,#31499,#31500,#31501,#31502,#31503,#31504,#31505,#31506),
 .UNSPECIFIED.,.F.,.F.,(4,3,3,3,3,3,3,3,3,3,3,3,3,3,3,3,3,3,3,3,3,3,3,3,
3,3,3,3,3,3,3,3,3,3,3,3,3,3,3,3,3,3,3,3,3,3,3,3,3,3,3,3,3,3,3,3,4),(298.451302091176,
298.526537089347,298.601724537959,298.676880845604,298.729553357428,298.810561753332,
298.891646010163,298.976092048401,299.057398130108,299.138781919876,299.220286580905,
299.229430163113,299.306945941376,299.384380241787,299.461748660214,299.539066745364,
299.616350009409,299.693627093721,299.770903674209,299.848193769606,299.925511403611,
300.002917609935,300.080369619249,300.157942427571,300.229183774482,300.306032397669,
300.382787244066,300.459464583471,300.536080623246,300.612651521871,300.689687254868,
300.766229673574,300.842778010136,300.919346841584,300.996744477651,301.073435558604,
301.151186472228,301.228937385852,301.30645493747,301.38388515689,301.461243699785,
301.538546170373,301.615808132323,301.693055358106,301.770296869313,301.847546719545,
301.924818964458,302.002171922429,302.079566314738,302.157074642406,302.228690997221,
302.306212598582,302.383649456979,302.460999992763,302.538300277288,302.615564024868,
302.688147330401),.UNSPECIFIED.);
#292=B_SPLINE_CURVE_WITH_KNOTS('',3,(#31507,#31508,#31509,#31510,#31511,
#31512,#31513,#31514,#31515,#31516,#31517,#31518,#31519,#31520,#31521,#31522,
#31523,#31524,#31525,#31526,#31527,#31528,#31529,#31530,#31531,#31532,#31533,
#31534,#31535,#31536,#31537,#31538,#31539,#31540,#31541,#31542,#31543,#31544,
#31545,#31546,#31547,#31548,#31549,#31550,#31551,#31552,#31553,#31554,#31555,
#31556,#31557,#31558,#31559,#31560,#31561,#31562,#31563,#31564,#31565,#31566,
#31567,#31568,#31569,#31570,#31571,#31572,#31573,#31574,#31575,#31576,#31577,
#31578,#31579,#31580,#31581,#31582,#31583,#31584,#31585,#31586,#31587,#31588),
 .UNSPECIFIED.,.F.,.F.,(4,3,3,3,3,3,3,3,3,3,3,3,3,3,3,3,3,3,3,3,3,3,3,3,
3,3,3,4),(296.405440486054,296.482081738333,296.558670776144,296.635223736031,
296.711769685511,296.788315197546,296.864874847928,296.941463218834,297.018140894284,
297.094866423305,297.171710683336,297.229922940374,297.307505563988,297.384995546197,
297.462408523422,297.539760076923,297.617065743835,297.694348336879,297.771620123823,
297.84889512368,297.926187354618,298.003552026983,298.080953635415,298.158461450023,
298.229676551744,298.329594899379,298.428201754546,298.451302091031),
 .UNSPECIFIED.);
#293=B_SPLINE_CURVE_WITH_KNOTS('',3,(#31590,#31591,#31592,#31593,#31594,
#31595,#31596,#31597,#31598,#31599,#31600,#31601,#31602,#31603,#31604,#31605,
#31606,#31607,#31608,#31609,#31610,#31611,#31612,#31613,#31614,#31615,#31616,
#31617,#31618,#31619,#31620,#31621,#31622,#31623,#31624,#31625,#31626,#31627,
#31628,#31629,#31630,#31631,#31632,#31633,#31634,#31635,#31636,#31637,#31638,
#31639,#31640,#31641,#31642,#31643,#31644,#31645,#31646,#31647,#31648,#31649,
#31650,#31651,#31652,#31653,#31654,#31655,#31656,#31657,#31658,#31659,#31660,
#31661,#31662,#31663,#31664,#31665,#31666,#31667,#31668,#31669,#31670,#31671),
 .UNSPECIFIED.,.F.,.F.,(4,3,3,3,3,3,3,3,3,3,3,3,3,3,3,3,3,3,3,3,3,3,3,3,
3,3,3,4),(296.405239013614,296.4825477514,296.559818493679,296.637077647407,
296.714333326596,296.791599572495,296.868890429628,296.946262650532,297.023678284972,
297.101204017291,297.159723150382,297.237253268445,297.314696297761,297.392067879587,
297.469383603947,297.546659020508,297.623919896534,297.70117520788,297.778438995972,
297.855725304356,297.933092165962,298.010500559894,298.088022192766,298.158131158433,
298.252011547859,298.345286298481,298.437505102726,298.451302091031),
 .UNSPECIFIED.);
#294=B_SPLINE_CURVE_WITH_KNOTS('',3,(#31672,#31673,#31674,#31675,#31676,
#31677,#31678,#31679,#31680,#31681,#31682,#31683,#31684,#31685,#31686,#31687,
#31688,#31689,#31690,#31691,#31692,#31693,#31694,#31695,#31696,#31697,#31698,
#31699,#31700,#31701,#31702,#31703,#31704,#31705,#31706,#31707,#31708,#31709,
#31710,#31711,#31712,#31713,#31714,#31715,#31716,#31717,#31718,#31719,#31720,
#31721,#31722,#31723,#31724,#31725,#31726,#31727,#31728,#31729,#31730,#31731,
#31732,#31733,#31734,#31735,#31736,#31737,#31738,#31739,#31740,#31741,#31742,
#31743,#31744,#31745,#31746,#31747,#31748,#31749,#31750,#31751,#31752,#31753,
#31754,#31755,#31756,#31757,#31758,#31759,#31760,#31761,#31762,#31763,#31764,
#31765,#31766,#31767,#31768,#31769,#31770,#31771,#31772,#31773,#31774,#31775,
#31776,#31777,#31778,#31779,#31780,#31781,#31782,#31783,#31784,#31785,#31786,
#31787,#31788,#31789,#31790,#31791,#31792,#31793,#31794,#31795,#31796,#31797,
#31798,#31799,#31800,#31801,#31802,#31803,#31804,#31805,#31806,#31807,#31808,
#31809,#31810,#31811,#31812,#31813,#31814,#31815,#31816,#31817,#31818,#31819,
#31820,#31821,#31822,#31823,#31824,#31825,#31826,#31827,#31828),
 .UNSPECIFIED.,.F.,.F.,(4,3,3,3,3,3,3,3,3,3,3,3,3,3,3,3,3,3,3,3,3,3,3,3,
3,3,3,3,3,3,3,3,3,3,3,3,3,3,3,3,3,3,3,3,3,3,3,3,3,3,3,3,4),(298.451302091031,
298.533764297067,298.616226154807,298.698687671101,298.781148852798,298.86360970675,
298.946070239804,299.02853045881,299.110990370618,299.193449982076,299.275909300032,
299.358368331334,299.440827082831,299.52328556137,299.605743773797,299.688201726962,
299.770659427709,299.853116882887,299.935574099342,300.021586325843,300.104910670267,
300.187377275712,300.269843036954,300.352307981406,300.434772136482,300.517235529591,
300.59969818814,300.682160139532,300.764621411171,300.847082030455,300.929542024782,
301.012001421547,301.094460248142,301.176918531959,301.259376300386,301.341833580811,
301.425966816223,301.508432814314,301.59089719067,301.673360054932,301.755821516723,
301.838281685644,301.920740671279,302.003198583197,302.088794428721,302.171259165321,
302.253720937323,302.336180183165,302.418637341143,302.501099859424,302.583557530279,
302.66601632023,302.687965347395),.UNSPECIFIED.);
#295=B_SPLINE_CURVE_WITH_KNOTS('',3,(#31834,#31835,#31836,#31837,#31838,
#31839,#31840,#31841,#31842,#31843,#31844,#31845,#31846,#31847,#31848,#31849,
#31850,#31851,#31852,#31853,#31854,#31855,#31856,#31857,#31858,#31859,#31860,
#31861,#31862,#31863,#31864,#31865,#31866,#31867,#31868,#31869,#31870,#31871,
#31872,#31873,#31874,#31875,#31876,#31877,#31878,#31879,#31880,#31881,#31882,
#31883,#31884,#31885,#31886,#31887,#31888,#31889,#31890,#31891,#31892,#31893,
#31894,#31895,#31896,#31897,#31898,#31899,#31900,#31901,#31902,#31903,#31904,
#31905,#31906,#31907,#31908,#31909,#31910,#31911,#31912,#31913,#31914,#31915,
#31916,#31917,#31918,#31919,#31920,#31921,#31922,#31923,#31924,#31925,#31926,
#31927,#31928,#31929,#31930,#31931,#31932,#31933,#31934,#31935,#31936,#31937,
#31938,#31939,#31940,#31941,#31942,#31943,#31944,#31945,#31946,#31947,#31948,
#31949,#31950,#31951,#31952,#31953,#31954,#31955,#31956,#31957,#31958,#31959,
#31960,#31961,#31962,#31963,#31964,#31965,#31966,#31967,#31968,#31969,#31970,
#31971,#31972,#31973,#31974,#31975,#31976,#31977,#31978,#31979,#31980,#31981,
#31982,#31983,#31984,#31985,#31986,#31987,#31988,#31989,#31990,#31991,#31992,
#31993,#31994,#31995,#31996,#31997,#31998,#31999,#32000,#32001,#32002),
 .UNSPECIFIED.,.F.,.F.,(4,3,3,3,3,3,3,3,3,3,3,3,3,3,3,3,3,3,3,3,3,3,3,3,
3,3,3,3,3,3,3,3,3,3,3,3,3,3,3,3,3,3,3,3,3,3,3,3,3,3,3,3,3,3,3,3,4),(304.734487420068,
304.814617174688,304.894819206556,304.978102362749,305.058528818975,305.143240325152,
305.227951831329,305.309435804284,305.390815168424,305.475068535572,305.556222030744,
305.637298708704,305.718284136494,305.727828637014,305.808837032918,305.889921289749,
305.974367327987,306.055673409694,306.137057199462,306.218561860491,306.227705442699,
306.305221220962,306.382655521373,306.4600239398,306.53734202495,306.614625288994,
306.691902373306,306.769178953793,306.84646904919,306.923786683195,307.001192889519,
307.078644898833,307.156217707154,307.227459054068,307.304307677255,307.381062523652,
307.457739863057,307.534355902832,307.610926801457,307.687962534454,307.76450495316,
307.841053289722,307.91762212117,307.995019757237,308.07171083819,308.149461751813,
308.227212665437,308.3047445604,308.382186284033,308.459537513191,308.536836778233,
308.614098178985,308.691335791111,308.768579033392,308.845824246208,308.923110025222,
308.970560612253),.UNSPECIFIED.);
#296=B_SPLINE_CURVE_WITH_KNOTS('',3,(#32003,#32004,#32005,#32006,#32007,
#32008,#32009,#32010,#32011,#32012,#32013,#32014,#32015,#32016,#32017,#32018,
#32019,#32020,#32021,#32022,#32023,#32024,#32025,#32026,#32027,#32028,#32029,
#32030,#32031,#32032,#32033,#32034,#32035,#32036,#32037,#32038,#32039,#32040,
#32041,#32042,#32043,#32044,#32045,#32046,#32047,#32048,#32049,#32050,#32051,
#32052,#32053,#32054,#32055,#32056,#32057,#32058,#32059,#32060,#32061,#32062,
#32063,#32064,#32065,#32066,#32067,#32068,#32069,#32070,#32071,#32072,#32073,
#32074,#32075,#32076,#32077,#32078,#32079,#32080,#32081,#32082,#32083,#32084),
 .UNSPECIFIED.,.F.,.F.,(4,3,3,3,3,3,3,3,3,3,3,3,3,3,3,3,3,3,3,3,3,3,3,3,
3,3,3,4),(302.688147330401,302.765388799308,302.842637787327,302.919908349782,
302.997259325273,303.074650996299,303.152157927652,303.228444608591,303.305265805746,
303.38199776796,303.458656746108,303.53525893257,303.611820474451,303.68886769264,
303.765411867284,303.841966147329,303.918545112309,303.995958389222,304.072669869529,
304.150434044744,304.22819821996,304.310669468899,304.392996678695,304.478369358574,
304.560356137155,304.642222416059,304.723932153712,304.73448739821),
 .UNSPECIFIED.);
#297=B_SPLINE_CURVE_WITH_KNOTS('',3,(#32086,#32087,#32088,#32089,#32090,
#32091,#32092,#32093,#32094,#32095,#32096,#32097,#32098,#32099,#32100,#32101,
#32102,#32103,#32104,#32105,#32106,#32107,#32108,#32109,#32110,#32111,#32112,
#32113,#32114,#32115,#32116,#32117,#32118,#32119,#32120,#32121,#32122,#32123,
#32124,#32125,#32126,#32127,#32128,#32129,#32130,#32131,#32132,#32133,#32134,
#32135,#32136,#32137,#32138,#32139,#32140,#32141,#32142,#32143,#32144,#32145,
#32146,#32147,#32148,#32149,#32150,#32151,#32152,#32153,#32154,#32155,#32156,
#32157,#32158,#32159,#32160,#32161),.UNSPECIFIED.,.F.,.F.,(4,3,3,3,3,3,
3,3,3,3,3,3,3,3,3,3,3,3,3,3,3,3,3,3,3,4),(302.687965347395,302.770426951249,
302.852887889219,302.935348188705,303.017807877102,303.100266981804,303.182725530203,
303.265183549689,303.347641067651,303.434318963311,303.516785749146,303.59925086249,
303.681714412995,303.764176510293,303.846637263994,303.929096783691,304.011555178959,
304.094012559356,304.176478945622,304.258942147636,304.341402603916,304.423860752827,
304.506326357706,304.588786236921,304.671250350285,304.73448739821),
 .UNSPECIFIED.);
#298=B_SPLINE_CURVE_WITH_KNOTS('',3,(#32162,#32163,#32164,#32165,#32166,
#32167,#32168,#32169,#32170,#32171,#32172,#32173,#32174,#32175,#32176,#32177,
#32178,#32179,#32180,#32181,#32182,#32183,#32184,#32185,#32186,#32187,#32188,
#32189,#32190,#32191,#32192,#32193,#32194,#32195,#32196,#32197,#32198,#32199,
#32200,#32201,#32202,#32203,#32204,#32205,#32206,#32207,#32208,#32209,#32210,
#32211,#32212,#32213,#32214,#32215,#32216,#32217,#32218,#32219,#32220,#32221,
#32222,#32223,#32224,#32225,#32226,#32227,#32228,#32229,#32230,#32231,#32232,
#32233,#32234,#32235,#32236,#32237,#32238,#32239,#32240,#32241,#32242,#32243,
#32244,#32245,#32246,#32247,#32248,#32249,#32250,#32251,#32252,#32253,#32254,
#32255,#32256,#32257,#32258,#32259,#32260,#32261,#32262,#32263,#32264,#32265,
#32266,#32267,#32268,#32269,#32270,#32271,#32272,#32273,#32274,#32275,#32276,
#32277,#32278,#32279,#32280,#32281,#32282,#32283,#32284,#32285,#32286,#32287,
#32288,#32289,#32290,#32291,#32292,#32293,#32294,#32295,#32296,#32297,#32298,
#32299,#32300,#32301,#32302,#32303,#32304,#32305,#32306,#32307,#32308,#32309,
#32310,#32311,#32312,#32313,#32314,#32315,#32316,#32317,#32318,#32319,#32320,
#32321,#32322,#32323,#32324,#32325,#32326,#32327,#32328,#32329,#32330),
 .UNSPECIFIED.,.F.,.F.,(4,3,3,3,3,3,3,3,3,3,3,3,3,3,3,3,3,3,3,3,3,3,3,3,
3,3,3,3,3,3,3,3,3,3,3,3,3,3,3,3,3,3,3,3,3,3,3,3,3,3,3,3,3,3,3,3,4),(304.73448739821,
304.819534618296,304.905005814465,304.990685396803,305.076670221159,305.146987214789,
305.223823246912,305.300570262639,305.377244500202,305.453862139724,305.530439316351,
305.607308804662,305.683868907185,305.760439204332,305.837034265354,305.914124504726,
305.990851701307,306.068123462074,306.14539522284,306.222989892274,306.300492158384,
306.377917643455,306.455281914832,306.532600495923,306.609896200394,306.68718124505,
306.764469636983,306.841775382509,306.919153422496,306.996568494241,307.074089108512,
307.143803230891,307.225289545324,307.306671627683,307.390755529491,307.471912848344,
307.552993632099,307.633983624133,307.643007234916,307.724020341206,307.80510903548,
307.889384586345,307.970694052735,308.052080953946,308.13358809271,308.142211238942,
308.219747731918,308.297201075221,308.37458685742,308.451916100716,308.529214275392,
308.606495402004,308.683773488848,308.761089684787,308.838425502775,308.915831968875,
308.970671977892),.UNSPECIFIED.);
#299=B_SPLINE_CURVE_WITH_KNOTS('',3,(#32336,#32337,#32338,#32339,#32340,
#32341,#32342,#32343,#32344,#32345,#32346,#32347,#32348,#32349,#32350,#32351,
#32352,#32353,#32354,#32355,#32356,#32357,#32358,#32359,#32360,#32361,#32362,
#32363,#32364,#32365,#32366,#32367,#32368,#32369,#32370,#32371,#32372,#32373,
#32374,#32375,#32376,#32377,#32378,#32379,#32380,#32381,#32382,#32383,#32384,
#32385,#32386,#32387,#32388,#32389,#32390,#32391,#32392,#32393,#32394,#32395,
#32396,#32397,#32398,#32399,#32400,#32401,#32402,#32403,#32404,#32405,#32406,
#32407,#32408,#32409,#32410,#32411,#32412,#32413,#32414,#32415,#32416,#32417,
#32418,#32419,#32420,#32421,#32422,#32423,#32424,#32425,#32426,#32427,#32428,
#32429,#32430,#32431,#32432,#32433,#32434,#32435,#32436,#32437,#32438,#32439,
#32440,#32441,#32442,#32443,#32444,#32445,#32446,#32447,#32448,#32449,#32450,
#32451,#32452,#32453,#32454,#32455,#32456,#32457,#32458,#32459,#32460,#32461,
#32462,#32463,#32464,#32465,#32466,#32467,#32468,#32469,#32470,#32471,#32472,
#32473,#32474,#32475,#32476,#32477,#32478,#32479,#32480,#32481,#32482,#32483,
#32484,#32485,#32486,#32487,#32488,#32489,#32490,#32491,#32492),
 .UNSPECIFIED.,.F.,.F.,(4,3,3,3,3,3,3,3,3,3,3,3,3,3,3,3,3,3,3,3,3,3,3,3,
3,3,3,3,3,3,3,3,3,3,3,3,3,3,3,3,3,3,3,3,3,3,3,3,3,3,3,3,4),(311.01767270539,
311.100134911426,311.182596769166,311.26505828546,311.347519467157,311.429980321108,
311.512440854162,311.594901073169,311.677360984977,311.759820596435,311.842279914391,
311.924738945693,312.007197697189,312.089656175728,312.172114388156,312.25457234132,
312.337030042068,312.419487497245,312.5019447137,312.587956940202,312.671281284625,
312.753747890071,312.836213651312,312.918678595765,313.001142750841,313.08360614395,
313.166068802498,313.248530753891,313.33099202553,313.413452644814,313.495912639141,
313.578372035905,313.6608308625,313.743289146317,313.825746914745,313.90820419517,
313.992337430581,314.074803428673,314.157267805029,314.239730669291,314.322192131081,
314.404652300003,314.487111285638,314.569569197555,314.65516504308,314.73762977968,
314.820091551682,314.902550797524,314.985007955501,315.067470473783,315.149928144638,
315.232386934588,315.254335961755),.UNSPECIFIED.);
#300=B_SPLINE_CURVE_WITH_KNOTS('',3,(#32493,#32494,#32495,#32496,#32497,
#32498,#32499,#32500,#32501,#32502,#32503,#32504,#32505,#32506,#32507,#32508,
#32509,#32510,#32511,#32512,#32513,#32514,#32515,#32516,#32517,#32518,#32519,
#32520,#32521,#32522,#32523,#32524,#32525,#32526,#32527,#32528,#32529,#32530,
#32531,#32532,#32533,#32534,#32535,#32536,#32537,#32538,#32539,#32540,#32541,
#32542,#32543,#32544,#32545,#32546,#32547,#32548,#32549,#32550,#32551,#32552,
#32553,#32554,#32555,#32556,#32557,#32558,#32559,#32560,#32561,#32562,#32563,
#32564,#32565,#32566,#32567,#32568,#32569,#32570,#32571,#32572,#32573,#32574,
#32575,#32576,#32577),.UNSPECIFIED.,.F.,.F.,(4,3,3,3,3,3,3,3,3,3,3,3,3,
3,3,3,3,3,3,3,3,3,3,3,3,3,3,3,4),(308.970560612253,309.047937498109,309.125363586437,
309.20289114427,309.226966276807,309.304483646003,309.381913713454,309.459272134724,
309.536574513939,309.613836414702,309.691083625393,309.768325149612,309.845575040958,
309.922847355101,310.000200426327,310.077594956079,310.155103461041,310.226719888176,
310.302445972709,310.37808266474,310.453646918017,310.529150574392,310.604621220853,
310.680074035677,310.755524180882,310.831013238727,310.906524250404,310.982104336895,
311.016482328777),.UNSPECIFIED.);
#301=B_SPLINE_CURVE_WITH_KNOTS('',3,(#32579,#32580,#32581,#32582,#32583,
#32584,#32585,#32586,#32587,#32588,#32589,#32590,#32591,#32592,#32593,#32594,
#32595,#32596,#32597,#32598,#32599,#32600,#32601,#32602,#32603,#32604,#32605,
#32606,#32607,#32608,#32609,#32610,#32611,#32612,#32613,#32614,#32615,#32616,
#32617,#32618,#32619,#32620,#32621,#32622,#32623,#32624,#32625,#32626,#32627,
#32628,#32629,#32630,#32631,#32632,#32633,#32634,#32635,#32636,#32637,#32638,
#32639,#32640,#32641,#32642,#32643,#32644,#32645,#32646,#32647,#32648,#32649,
#32650,#32651,#32652,#32653,#32654,#32655,#32656,#32657,#32658,#32659,#32660,
#32661,#32662,#32663),.UNSPECIFIED.,.F.,.F.,(4,3,3,3,3,3,3,3,3,3,3,3,3,
3,3,3,3,3,3,3,3,3,3,3,3,3,3,3,4),(308.970671977892,309.048177449884,309.125787753225,
309.140619246993,309.217482631645,309.294252463455,309.370944999443,309.44757643461,
309.524162915393,309.60102095785,309.677579280813,309.754143615486,309.830728528613,
309.90780321022,309.984510031089,310.061768643067,310.139027255044,310.215551403013,
310.29198879418,310.368355917333,310.444669199715,310.520948512192,310.597211241812,
310.673472180531,310.749746117098,310.826082051884,310.902452802341,310.978912686717,
311.017672705276),.UNSPECIFIED.);
#302=B_SPLINE_CURVE_WITH_KNOTS('',3,(#32664,#32665,#32666,#32667,#32668,
#32669,#32670,#32671,#32672,#32673,#32674,#32675,#32676,#32677,#32678,#32679,
#32680,#32681,#32682,#32683,#32684,#32685,#32686,#32687,#32688,#32689,#32690,
#32691,#32692,#32693,#32694,#32695,#32696,#32697,#32698,#32699,#32700,#32701,
#32702,#32703,#32704,#32705,#32706,#32707,#32708,#32709,#32710,#32711,#32712,
#32713,#32714,#32715,#32716,#32717,#32718,#32719,#32720,#32721,#32722,#32723,
#32724,#32725,#32726,#32727,#32728,#32729,#32730,#32731,#32732,#32733,#32734,
#32735,#32736,#32737,#32738,#32739,#32740,#32741,#32742,#32743,#32744,#32745,
#32746,#32747,#32748,#32749,#32750,#32751,#32752,#32753,#32754,#32755,#32756,
#32757,#32758,#32759,#32760,#32761,#32762,#32763,#32764,#32765,#32766,#32767,
#32768,#32769,#32770,#32771,#32772,#32773,#32774,#32775,#32776,#32777,#32778,
#32779,#32780,#32781,#32782,#32783,#32784,#32785,#32786,#32787,#32788,#32789,
#32790,#32791,#32792,#32793,#32794,#32795,#32796,#32797,#32798,#32799,#32800,
#32801,#32802,#32803,#32804,#32805,#32806,#32807,#32808,#32809,#32810,#32811,
#32812,#32813,#32814,#32815,#32816,#32817,#32818,#32819,#32820,#32821,#32822,
#32823,#32824,#32825,#32826,#32827,#32828,#32829,#32830,#32831,#32832),
 .UNSPECIFIED.,.F.,.F.,(4,3,3,3,3,3,3,3,3,3,3,3,3,3,3,3,3,3,3,3,3,3,3,3,
3,3,3,3,3,3,3,3,3,3,3,3,3,3,3,3,3,3,3,3,3,3,3,3,3,3,3,3,3,3,3,3,4),(311.01767270539,
311.137435263095,311.214965381158,311.292408410474,311.3697799923,311.44709571666,
311.524371133221,311.601632009246,311.678887320593,311.756151108684,311.833437417069,
311.910804278675,311.988212672607,312.065734305479,312.135843271145,312.212679303268,
312.289426318995,312.366100556558,312.442718196079,312.519295372706,312.596164861018,
312.67272496354,312.749295260688,312.82589032171,312.902980561082,312.979707757663,
313.056979518429,313.134251279196,313.21184594863,313.289348214741,313.366773699811,
313.444137971188,313.521456552279,313.598752256751,313.676037301407,313.75332569334,
313.830631438866,313.908009478853,313.985424550598,314.062945164869,314.132659287247,
314.21414560168,314.295527684039,314.379611585847,314.460768904701,314.541849688455,
314.622839680489,314.631863291273,314.712876397564,314.793965091837,314.878240642702,
314.959550109092,315.040937010302,315.122444149067,315.131067295298,315.20859582047,
315.254853130802),.UNSPECIFIED.);
#303=B_SPLINE_CURVE_WITH_KNOTS('',3,(#32838,#32839,#32840,#32841,#32842,
#32843,#32844,#32845,#32846,#32847,#32848,#32849,#32850,#32851,#32852,#32853,
#32854,#32855,#32856,#32857,#32858,#32859,#32860,#32861,#32862,#32863,#32864,
#32865,#32866,#32867,#32868,#32869,#32870,#32871,#32872,#32873,#32874,#32875,
#32876,#32877,#32878,#32879,#32880,#32881,#32882,#32883,#32884,#32885,#32886,
#32887,#32888,#32889,#32890,#32891,#32892,#32893,#32894,#32895,#32896,#32897,
#32898,#32899,#32900,#32901,#32902,#32903,#32904,#32905,#32906,#32907,#32908,
#32909,#32910,#32911,#32912,#32913,#32914,#32915,#32916,#32917,#32918,#32919,
#32920,#32921,#32922,#32923,#32924,#32925,#32926,#32927,#32928,#32929,#32930,
#32931,#32932,#32933,#32934,#32935,#32936,#32937,#32938,#32939,#32940,#32941,
#32942,#32943,#32944,#32945,#32946,#32947,#32948,#32949,#32950,#32951,#32952,
#32953,#32954,#32955,#32956,#32957,#32958,#32959,#32960,#32961,#32962,#32963,
#32964,#32965,#32966,#32967,#32968,#32969,#32970,#32971,#32972,#32973,#32974,
#32975,#32976,#32977,#32978,#32979,#32980,#32981,#32982,#32983,#32984,#32985,
#32986,#32987,#32988,#32989,#32990,#32991,#32992,#32993,#32994,#32995,#32996,
#32997,#32998,#32999,#33000,#33001,#33002,#33003,#33004,#33005,#33006,#33007,
#33008,#33009),.UNSPECIFIED.,.F.,.F.,(4,3,3,3,3,3,3,3,3,3,3,3,3,3,3,3,3,
3,3,3,3,3,3,3,3,3,3,3,3,3,3,3,3,3,3,3,3,3,3,3,3,3,3,3,3,3,3,3,3,3,3,3,3,
3,3,3,3,4),(317.301428870433,317.377425349235,317.453339462372,317.52918796026,
317.604987526603,317.682457683169,317.758222508873,317.833991512175,317.909779722749,
317.988521986845,318.064434773949,318.140401796158,318.216471684351,318.224748779131,
318.302331402745,318.379821384954,318.457234362179,318.53458591568,318.611891582591,
318.689174175636,318.76644596258,318.843720962437,318.921013193375,318.998377865739,
319.075779474172,319.15328728878,319.2245023905,319.305986363455,319.387365727595,
319.471619094743,319.552772589915,319.633849267873,319.714834695664,319.724379196185,
319.805387592089,319.886471848921,319.970917887158,320.052223968865,320.133607758634,
320.215112419662,320.22425600187,320.301771780133,320.379206080543,320.456574498971,
320.533892584121,320.611175848165,320.688452932477,320.765729512964,320.843019608362,
320.920337242366,320.99774344869,321.075195458004,321.152768266326,321.224009613239,
321.302574934875,321.379326931844,321.458798915814,321.538270899783),
 .UNSPECIFIED.);
#304=B_SPLINE_CURVE_WITH_KNOTS('',3,(#33010,#33011,#33012,#33013,#33014,
#33015,#33016,#33017,#33018,#33019,#33020,#33021,#33022,#33023,#33024,#33025,
#33026,#33027,#33028,#33029,#33030,#33031,#33032,#33033,#33034,#33035,#33036,
#33037,#33038,#33039,#33040,#33041,#33042,#33043,#33044,#33045,#33046,#33047,
#33048,#33049,#33050,#33051,#33052,#33053,#33054,#33055,#33056,#33057,#33058,
#33059,#33060,#33061,#33062,#33063,#33064,#33065,#33066,#33067,#33068,#33069,
#33070,#33071,#33072,#33073,#33074,#33075,#33076,#33077,#33078,#33079,#33080,
#33081,#33082,#33083,#33084,#33085),.UNSPECIFIED.,.F.,.F.,(4,3,3,3,3,3,
3,3,3,3,3,3,3,3,3,3,3,3,3,3,3,3,3,3,3,4),(315.254335961755,315.336797565608,
315.419258503579,315.501718803065,315.584178491462,315.666637596164,315.749096144563,
315.831554164049,315.914011682011,316.000689577671,316.083156363506,316.16562147685,
316.248085027355,316.330547124653,316.413007878354,316.495467398051,316.577925793319,
316.660383173716,316.742849559983,316.825312761996,316.907773218277,316.990231367188,
317.072696972067,317.155156851281,317.237620964645,317.30085801257),
 .UNSPECIFIED.);
#305=B_SPLINE_CURVE_WITH_KNOTS('',3,(#33087,#33088,#33089,#33090,#33091,
#33092,#33093,#33094,#33095,#33096,#33097,#33098,#33099,#33100,#33101,#33102,
#33103,#33104,#33105,#33106,#33107,#33108,#33109,#33110,#33111,#33112,#33113,
#33114,#33115,#33116,#33117,#33118,#33119,#33120,#33121,#33122,#33123,#33124,
#33125,#33126,#33127,#33128,#33129,#33130,#33131,#33132,#33133,#33134,#33135,
#33136,#33137,#33138,#33139,#33140,#33141,#33142,#33143,#33144,#33145,#33146,
#33147,#33148,#33149,#33150,#33151,#33152,#33153,#33154,#33155,#33156,#33157,
#33158,#33159,#33160,#33161,#33162,#33163,#33164,#33165,#33166,#33167,#33168),
 .UNSPECIFIED.,.F.,.F.,(4,3,3,3,3,3,3,3,3,3,3,3,3,3,3,3,3,3,3,3,3,3,3,3,
3,3,3,4),(315.254853130802,315.332258903035,315.409608261007,315.486916716749,
315.567236540074,315.644524969973,315.721821920583,315.799141401053,315.876497430504,
315.953944630171,316.031445729455,316.109053139725,316.129475303349,316.206338688001,
316.283108519811,316.3598010558,316.436432490966,316.51301897175,316.589877014206,
316.66643533717,316.742999671842,316.819584584969,316.896659266577,316.973366087446,
317.050624699423,317.1278833114,317.252579983701,317.300858012569),
 .UNSPECIFIED.);
#306=B_SPLINE_CURVE_WITH_KNOTS('',3,(#33169,#33170,#33171,#33172,#33173,
#33174,#33175,#33176,#33177,#33178,#33179,#33180,#33181,#33182,#33183,#33184,
#33185,#33186,#33187,#33188,#33189,#33190,#33191,#33192,#33193,#33194,#33195,
#33196,#33197,#33198,#33199,#33200,#33201,#33202,#33203,#33204,#33205,#33206,
#33207,#33208,#33209,#33210,#33211,#33212,#33213,#33214,#33215,#33216,#33217,
#33218,#33219,#33220,#33221,#33222,#33223,#33224,#33225,#33226,#33227,#33228,
#33229,#33230,#33231,#33232,#33233,#33234,#33235,#33236,#33237,#33238,#33239,
#33240,#33241,#33242,#33243,#33244,#33245,#33246,#33247,#33248,#33249,#33250,
#33251,#33252,#33253,#33254,#33255,#33256,#33257,#33258,#33259,#33260,#33261,
#33262,#33263,#33264,#33265,#33266,#33267,#33268,#33269,#33270,#33271,#33272,
#33273,#33274,#33275,#33276,#33277,#33278,#33279,#33280,#33281,#33282,#33283,
#33284,#33285,#33286,#33287,#33288,#33289,#33290,#33291,#33292,#33293,#33294,
#33295,#33296,#33297,#33298,#33299,#33300,#33301,#33302,#33303,#33304,#33305,
#33306,#33307,#33308,#33309,#33310,#33311,#33312,#33313,#33314,#33315,#33316,
#33317,#33318,#33319,#33320,#33321,#33322,#33323,#33324,#33325,#33326,#33327,
#33328,#33329,#33330,#33331,#33332,#33333,#33334),.UNSPECIFIED.,.F.,.F.,
(4,3,3,3,3,3,3,3,3,3,3,3,3,3,3,3,3,3,3,3,3,3,3,3,3,3,3,3,3,3,3,3,3,3,3,
3,3,3,3,3,3,3,3,3,3,3,3,3,3,3,3,3,3,3,3,4),(317.300858012671,317.377039648526,
317.453155161215,317.529221117743,317.605261090874,317.681288920083,317.757319530207,
317.833367846566,317.909490964028,317.985652971468,318.06192404716,318.126291319451,
318.203821437514,318.281264466831,318.358636048656,318.435951773016,318.513227189577,
318.590488065603,318.667743376949,318.745007165041,318.822293473425,318.899660335031,
318.977068728963,319.054590361835,319.124699327502,319.201535359625,319.278282375352,
319.354956612915,319.431574252437,319.508151429064,319.585020917376,319.661581019898,
319.738151317046,319.814746378068,319.891836617439,319.968563814021,320.045835574787,
320.123107335553,320.200702004987,320.278204271098,320.355629756168,320.432994027545,
320.510312608635,320.587608313107,320.664893357763,320.742181749696,320.819487495222,
320.896865535209,320.974280606954,321.051801221225,321.121515343604,321.203013892014,
321.28671011981,321.367969374234,321.452884088717,321.537798803201),
 .UNSPECIFIED.);
#307=B_SPLINE_CURVE_WITH_KNOTS('',3,(#33340,#33341,#33342,#33343,#33344,
#33345,#33346,#33347,#33348,#33349,#33350,#33351,#33352,#33353,#33354,#33355,
#33356,#33357,#33358,#33359,#33360,#33361,#33362,#33363,#33364,#33365,#33366,
#33367,#33368,#33369,#33370,#33371,#33372,#33373,#33374,#33375,#33376,#33377,
#33378,#33379,#33380,#33381,#33382,#33383,#33384,#33385,#33386,#33387,#33388,
#33389,#33390,#33391,#33392,#33393,#33394,#33395,#33396,#33397,#33398,#33399,
#33400,#33401,#33402,#33403,#33404,#33405,#33406,#33407,#33408,#33409,#33410,
#33411,#33412,#33413,#33414,#33415,#33416,#33417,#33418,#33419,#33420,#33421,
#33422,#33423,#33424,#33425,#33426,#33427,#33428,#33429,#33430,#33431,#33432,
#33433,#33434,#33435,#33436,#33437,#33438,#33439,#33440,#33441,#33442,#33443,
#33444,#33445,#33446,#33447,#33448,#33449,#33450,#33451,#33452,#33453,#33454,
#33455,#33456,#33457,#33458,#33459,#33460,#33461,#33462,#33463,#33464,#33465,
#33466,#33467,#33468,#33469,#33470,#33471,#33472,#33473,#33474,#33475,#33476,
#33477,#33478,#33479,#33480,#33481,#33482,#33483,#33484,#33485,#33486,#33487,
#33488,#33489,#33490,#33491,#33492,#33493,#33494,#33495,#33496,#33497,#33498,
#33499,#33500,#33501,#33502,#33503,#33504,#33505,#33506,#33507,#33508,#33509,
#33510,#33511),.UNSPECIFIED.,.F.,.F.,(4,3,3,3,3,3,3,3,3,3,3,3,3,3,3,3,3,
3,3,3,3,3,3,3,3,3,3,3,3,3,3,3,3,3,3,3,3,3,3,3,3,3,3,3,3,3,3,3,3,3,3,3,3,
3,3,3,3,4),(323.584043319749,323.663946710699,323.741728431509,323.819526019224,
323.897352847792,323.978832247681,324.056801261427,324.134828908685,324.212963354016,
324.223270447347,324.300091644502,324.376823606716,324.453482584864,324.530084771325,
324.606646313206,324.683693531395,324.76023770604,324.836791986085,324.913370951065,
324.990784227978,325.067495708285,325.145259883501,325.223024058717,325.300606682331,
325.37809666454,325.455509641765,325.532861195267,325.610166862178,325.687449455223,
325.764721242167,325.841996242024,325.919288472962,325.996653145327,326.074054753759,
326.151562568367,326.222777670086,326.304261643041,326.385641007181,326.469894374328,
326.5510478695,326.632124547458,326.713109975248,326.722654475771,326.803662871675,
326.884747128507,326.969193166744,327.050499248452,327.13188303822,327.213387699248,
327.222531281455,327.300038871417,327.377469344525,327.454836829461,327.532155415822,
327.609442145055,327.686709244247,327.763985749949,327.820383538779),
 .UNSPECIFIED.);
#308=B_SPLINE_CURVE_WITH_KNOTS('',3,(#33512,#33513,#33514,#33515,#33516,
#33517,#33518,#33519,#33520,#33521,#33522,#33523,#33524,#33525,#33526,#33527,
#33528,#33529,#33530,#33531,#33532,#33533,#33534,#33535,#33536,#33537,#33538,
#33539,#33540,#33541,#33542,#33543,#33544,#33545,#33546,#33547,#33548,#33549,
#33550,#33551,#33552,#33553,#33554,#33555,#33556,#33557,#33558,#33559,#33560,
#33561,#33562,#33563,#33564,#33565,#33566,#33567,#33568,#33569,#33570,#33571,
#33572,#33573,#33574,#33575,#33576,#33577,#33578,#33579,#33580,#33581,#33582,
#33583,#33584,#33585,#33586,#33587,#33588,#33589,#33590),.UNSPECIFIED.,
 .F.,.F.,(4,3,3,3,3,3,3,3,3,3,3,3,3,3,3,3,3,3,3,3,3,3,3,3,3,3,4),(321.538270899783,
321.614838307952,321.691388010917,321.767930365409,321.844479946831,321.921051332763,
321.997704444672,322.074399352265,322.151211241319,322.223763224608,322.301280776226,
322.378710995646,322.456069538541,322.533372009128,322.610633971078,322.68788119686,
322.765122708068,322.8423725583,322.919644803214,322.996997761185,323.074392153494,
323.151900481162,323.223516835978,323.313648456897,323.401631282329,323.492837300992,
323.584043319654),.UNSPECIFIED.);
#309=B_SPLINE_CURVE_WITH_KNOTS('',3,(#33592,#33593,#33594,#33595,#33596,
#33597,#33598,#33599,#33600,#33601,#33602,#33603,#33604,#33605,#33606,#33607,
#33608,#33609,#33610,#33611,#33612,#33613,#33614,#33615,#33616,#33617,#33618,
#33619,#33620,#33621,#33622,#33623,#33624,#33625,#33626,#33627,#33628,#33629,
#33630,#33631,#33632,#33633,#33634,#33635,#33636,#33637,#33638,#33639,#33640,
#33641,#33642,#33643,#33644,#33645,#33646,#33647,#33648,#33649,#33650,#33651,
#33652,#33653,#33654,#33655,#33656,#33657,#33658,#33659,#33660,#33661,#33662,
#33663,#33664,#33665,#33666,#33667,#33668,#33669,#33670,#33671,#33672,#33673),
 .UNSPECIFIED.,.F.,.F.,(4,3,3,3,3,3,3,3,3,3,3,3,3,3,3,3,3,3,3,3,3,3,3,3,
3,3,3,4),(321.537798803201,321.620719347629,321.701732453919,321.782821148193,
321.867096699058,321.948406165448,322.029793066659,322.111300205424,322.119923351655,
322.197451504864,322.274898379826,322.352279558533,322.429610575994,322.506906930824,
322.584197231161,322.661487138899,322.738790660897,322.816121809025,322.893541298846,
322.971006657268,323.048592043566,323.118331359706,323.200496339367,323.28250033732,
323.364275949166,323.44591614499,323.527362179731,323.584043319749),
 .UNSPECIFIED.);
#310=B_SPLINE_CURVE_WITH_KNOTS('',3,(#33674,#33675,#33676,#33677,#33678,
#33679,#33680,#33681,#33682,#33683,#33684,#33685,#33686,#33687,#33688,#33689,
#33690,#33691,#33692,#33693,#33694,#33695,#33696,#33697,#33698,#33699,#33700,
#33701,#33702,#33703,#33704,#33705,#33706,#33707,#33708,#33709,#33710,#33711,
#33712,#33713,#33714,#33715,#33716,#33717,#33718,#33719,#33720,#33721,#33722,
#33723,#33724,#33725,#33726,#33727,#33728,#33729,#33730,#33731,#33732,#33733,
#33734,#33735,#33736,#33737,#33738,#33739,#33740,#33741,#33742,#33743,#33744,
#33745,#33746,#33747,#33748,#33749,#33750,#33751,#33752,#33753,#33754,#33755,
#33756,#33757,#33758,#33759,#33760,#33761,#33762,#33763,#33764,#33765,#33766,
#33767,#33768,#33769,#33770,#33771,#33772,#33773,#33774,#33775,#33776,#33777,
#33778,#33779,#33780,#33781,#33782,#33783,#33784,#33785,#33786,#33787,#33788,
#33789,#33790,#33791,#33792,#33793,#33794,#33795,#33796,#33797,#33798,#33799,
#33800,#33801,#33802,#33803,#33804,#33805,#33806,#33807,#33808,#33809,#33810,
#33811,#33812,#33813,#33814,#33815,#33816,#33817,#33818,#33819,#33820,#33821,
#33822,#33823,#33824,#33825,#33826,#33827,#33828,#33829,#33830),
 .UNSPECIFIED.,.F.,.F.,(4,3,3,3,3,3,3,3,3,3,3,3,3,3,3,3,3,3,3,3,3,3,3,3,
3,3,3,3,3,3,3,3,3,3,3,3,3,3,3,3,3,3,3,3,3,3,3,3,3,3,3,3,4),(323.584043319749,
323.666505525785,323.748967383525,323.831428899819,323.913890081516,323.996350935467,
324.078811468522,324.161271687528,324.243731599336,324.326191210794,324.40865052875,
324.491109560052,324.573568311549,324.656026790088,324.738485002515,324.82094295568,
324.903400656427,324.985858111605,325.06831532806,325.154327554562,325.237651898985,
325.320118504431,325.402584265672,325.485049210125,325.567513365201,325.649976758309,
325.732439416858,325.814901368251,325.89736263989,325.979823259174,326.062283253501,
326.144742650265,326.22720147686,326.309659760677,326.392117529104,326.47457480953,
326.558708044941,326.641174043033,326.723638419388,326.80610128365,326.888562745441,
326.971022914362,327.053481899998,327.135939811915,327.22153565744,327.30400039404,
327.386462166042,327.468921411884,327.551378569861,327.633841088142,327.716298758997,
327.798757548948,327.820706576114),.UNSPECIFIED.);
#311=B_SPLINE_CURVE_WITH_KNOTS('',3,(#33836,#33837,#33838,#33839,#33840,
#33841,#33842,#33843,#33844,#33845,#33846,#33847,#33848,#33849,#33850,#33851,
#33852,#33853,#33854,#33855,#33856,#33857,#33858,#33859,#33860,#33861,#33862,
#33863,#33864,#33865,#33866,#33867,#33868,#33869,#33870,#33871,#33872,#33873,
#33874,#33875,#33876,#33877,#33878,#33879,#33880,#33881,#33882,#33883,#33884,
#33885,#33886,#33887,#33888,#33889,#33890,#33891,#33892,#33893,#33894,#33895,
#33896,#33897,#33898,#33899,#33900,#33901,#33902,#33903,#33904,#33905,#33906,
#33907,#33908,#33909,#33910,#33911,#33912,#33913,#33914,#33915,#33916,#33917,
#33918,#33919,#33920,#33921,#33922,#33923,#33924,#33925,#33926,#33927,#33928,
#33929,#33930,#33931,#33932,#33933,#33934,#33935,#33936,#33937,#33938,#33939,
#33940,#33941,#33942,#33943,#33944,#33945,#33946,#33947,#33948,#33949,#33950,
#33951,#33952,#33953,#33954,#33955,#33956,#33957,#33958,#33959,#33960,#33961,
#33962,#33963,#33964,#33965,#33966,#33967,#33968,#33969,#33970,#33971,#33972,
#33973,#33974,#33975,#33976,#33977,#33978,#33979,#33980,#33981,#33982,#33983,
#33984,#33985,#33986,#33987,#33988,#33989,#33990,#33991,#33992,#33993,#33994,
#33995,#33996,#33997,#33998,#33999,#34000,#34001),.UNSPECIFIED.,.F.,.F.,
(4,3,3,3,3,3,3,3,3,3,3,3,3,3,3,3,3,3,3,3,3,3,3,3,3,3,3,3,3,3,3,3,3,3,3,
3,3,3,3,3,3,3,3,3,3,3,3,3,3,3,3,3,3,3,3,4),(329.867228627023,329.955869499158,
330.044072983203,330.132932549383,330.221792115563,330.299309484759,330.37673955221,
330.45409797348,330.531400352695,330.608662253457,330.685909464148,330.763150988367,
330.840400879713,330.917673193857,330.995026265082,331.072420794834,331.149929299796,
331.221545726933,331.298366924088,331.375098886302,331.45175786445,331.528360050912,
331.604921592793,331.681968810981,331.758512985626,331.835067265671,331.911646230651,
331.989059507564,332.065770987871,332.143535163086,332.221299338302,332.298881961916,
332.376371944125,332.45378492135,332.531136474851,332.608442141762,332.685724734807,
332.762996521751,332.840271521607,332.917563752545,332.99492842491,333.072330033342,
333.149837847951,333.221052949672,333.302536922627,333.383916286767,333.468169653915,
333.549323149086,333.630399827046,333.711385254836,333.720929755356,333.801918491159,
333.883036778197,333.964221658522,334.045533951161,334.10356649952),
 .UNSPECIFIED.);
#312=B_SPLINE_CURVE_WITH_KNOTS('',3,(#34002,#34003,#34004,#34005,#34006,
#34007,#34008,#34009,#34010,#34011,#34012,#34013,#34014,#34015,#34016,#34017,
#34018,#34019,#34020,#34021,#34022,#34023,#34024,#34025,#34026,#34027,#34028,
#34029,#34030,#34031,#34032,#34033,#34034,#34035,#34036,#34037,#34038,#34039,
#34040,#34041,#34042,#34043,#34044,#34045,#34046,#34047,#34048,#34049,#34050,
#34051,#34052,#34053,#34054,#34055,#34056,#34057,#34058,#34059,#34060,#34061,
#34062,#34063,#34064,#34065,#34066,#34067,#34068,#34069,#34070,#34071,#34072,
#34073,#34074,#34075,#34076,#34077,#34078,#34079,#34080,#34081,#34082,#34083,
#34084,#34085,#34086),.UNSPECIFIED.,.F.,.F.,(4,3,3,3,3,3,3,3,3,3,3,3,3,
3,3,3,3,3,3,3,3,3,3,3,3,3,3,3,4),(327.820383538779,327.897692338465,327.978840477055,
328.056281233109,328.13377762746,328.211378106877,328.222284892825,328.299133516012,
328.375888362409,328.452565701814,328.529181741589,328.605752640213,328.682788373211,
328.759330791917,328.835879128479,328.912447959927,328.989845595994,329.066536676947,
329.14428759057,329.222038504194,329.302687269536,329.380591352408,329.458420870289,
329.536189422896,329.613910572277,329.691598450072,329.769267328952,329.846937730223,
329.867228626929),.UNSPECIFIED.);
#313=B_SPLINE_CURVE_WITH_KNOTS('',3,(#34088,#34089,#34090,#34091,#34092,
#34093,#34094,#34095,#34096,#34097,#34098,#34099,#34100,#34101,#34102,#34103,
#34104,#34105,#34106,#34107,#34108,#34109,#34110,#34111,#34112,#34113,#34114,
#34115,#34116,#34117,#34118,#34119,#34120,#34121,#34122,#34123,#34124,#34125,
#34126,#34127,#34128,#34129,#34130,#34131,#34132,#34133,#34134,#34135,#34136,
#34137,#34138,#34139,#34140,#34141,#34142,#34143,#34144,#34145,#34146,#34147,
#34148,#34149,#34150,#34151,#34152,#34153,#34154,#34155,#34156,#34157,#34158,
#34159,#34160,#34161,#34162,#34163),.UNSPECIFIED.,.F.,.F.,(4,3,3,3,3,3,
3,3,3,3,3,3,3,3,3,3,3,3,3,3,3,3,3,3,3,4),(327.820706576114,327.903168179967,
327.985629117938,328.068089417424,328.15054910582,328.233008210523,328.315466758922,
328.397924778408,328.48038229637,328.56706019203,328.649526977865,328.731992091209,
328.814455641714,328.896917739012,328.979378492713,329.06183801241,329.144296407678,
329.226753788075,329.309220174342,329.391683376355,329.474143832636,329.556601981547,
329.639067586426,329.72152746564,329.803991579004,329.867228626929),
 .UNSPECIFIED.);
#314=B_SPLINE_CURVE_WITH_KNOTS('',3,(#34164,#34165,#34166,#34167,#34168,
#34169,#34170,#34171,#34172,#34173,#34174,#34175,#34176,#34177,#34178,#34179,
#34180,#34181,#34182,#34183,#34184,#34185,#34186,#34187,#34188,#34189,#34190,
#34191,#34192,#34193,#34194,#34195,#34196,#34197,#34198,#34199,#34200,#34201,
#34202,#34203,#34204,#34205,#34206,#34207,#34208,#34209,#34210,#34211,#34212,
#34213,#34214,#34215,#34216,#34217,#34218,#34219,#34220,#34221,#34222,#34223,
#34224,#34225,#34226,#34227,#34228,#34229,#34230,#34231,#34232,#34233,#34234,
#34235,#34236,#34237,#34238,#34239,#34240,#34241,#34242,#34243,#34244,#34245,
#34246,#34247,#34248,#34249,#34250,#34251,#34252,#34253,#34254,#34255,#34256,
#34257,#34258,#34259,#34260,#34261,#34262,#34263,#34264,#34265,#34266,#34267,
#34268,#34269,#34270,#34271,#34272,#34273,#34274,#34275,#34276,#34277,#34278,
#34279,#34280,#34281,#34282,#34283,#34284,#34285,#34286,#34287,#34288,#34289,
#34290,#34291,#34292,#34293,#34294,#34295,#34296,#34297,#34298,#34299,#34300,
#34301,#34302,#34303,#34304,#34305,#34306,#34307,#34308,#34309,#34310,#34311,
#34312,#34313,#34314,#34315,#34316,#34317,#34318,#34319,#34320,#34321,#34322,
#34323,#34324,#34325,#34326,#34327,#34328,#34329,#34330,#34331,#34332),
 .UNSPECIFIED.,.F.,.F.,(4,3,3,3,3,3,3,3,3,3,3,3,3,3,3,3,3,3,3,3,3,3,3,3,
3,3,3,3,3,3,3,3,3,3,3,3,3,3,3,3,3,3,3,3,3,3,3,3,3,3,3,3,3,3,3,3,4),(329.867228626929,
329.972215293944,330.081178832984,330.107187416062,330.184050800714,330.260820632524,
330.337513168512,330.414144603679,330.490731084463,330.567589126919,330.644147449882,
330.720711784555,330.797296697682,330.87437137929,330.951078200159,331.028336812136,
331.105595424113,331.183125620573,331.260568715178,331.337940349234,331.415256112803,
331.492531555581,331.569792438001,331.647047743645,331.724311513939,331.801597792424,
331.878964605216,331.956372939923,332.033894496486,332.104003432164,332.181533550227,
332.258976579543,332.336348161369,332.413663885729,332.49093930229,332.568200178315,
332.645455489662,332.722719277753,332.800005586137,332.877372447744,332.954780841676,
333.032302474548,333.102411440215,333.179247472338,333.255994488065,333.332668725628,
333.40928636515,333.485863541777,333.562733030088,333.639293132611,333.715863429758,
333.79245849078,333.869548730152,333.946275926733,334.0235476875,334.100819448266,
334.103694651294),.UNSPECIFIED.);
#315=B_SPLINE_CURVE_WITH_KNOTS('',3,(#34338,#34339,#34340,#34341,#34342,
#34343,#34344,#34345,#34346,#34347,#34348,#34349,#34350,#34351,#34352,#34353,
#34354,#34355,#34356,#34357,#34358,#34359,#34360,#34361,#34362,#34363,#34364,
#34365,#34366,#34367,#34368,#34369,#34370,#34371,#34372,#34373,#34374,#34375,
#34376,#34377,#34378,#34379,#34380,#34381,#34382,#34383,#34384,#34385,#34386,
#34387,#34388,#34389,#34390,#34391,#34392,#34393,#34394,#34395,#34396,#34397,
#34398,#34399,#34400,#34401,#34402,#34403,#34404,#34405,#34406,#34407,#34408,
#34409,#34410,#34411,#34412,#34413,#34414,#34415,#34416,#34417,#34418,#34419,
#34420,#34421,#34422,#34423,#34424,#34425,#34426,#34427,#34428,#34429,#34430,
#34431,#34432,#34433,#34434,#34435,#34436,#34437,#34438,#34439,#34440,#34441,
#34442,#34443,#34444,#34445,#34446,#34447,#34448,#34449,#34450,#34451,#34452,
#34453,#34454,#34455,#34456,#34457,#34458,#34459,#34460,#34461,#34462,#34463,
#34464,#34465,#34466,#34467,#34468,#34469,#34470,#34471,#34472,#34473,#34474,
#34475,#34476,#34477,#34478,#34479,#34480,#34481,#34482,#34483,#34484,#34485,
#34486,#34487,#34488,#34489,#34490,#34491,#34492,#34493,#34494),
 .UNSPECIFIED.,.F.,.F.,(4,3,3,3,3,3,3,3,3,3,3,3,3,3,3,3,3,3,3,3,3,3,3,3,
3,3,3,3,3,3,3,3,3,3,3,3,3,3,3,3,3,3,3,3,3,3,3,3,3,3,3,3,4),(336.150413934108,
336.232876140144,336.315337997884,336.397799514178,336.480260695875,336.562721549826,
336.645182082881,336.727642301887,336.810102213695,336.892561825153,336.975021143109,
337.057480174411,337.139938925907,337.222397404446,337.304855616874,337.387313570038,
337.469771270786,337.552228725964,337.634685942418,337.72069816892,337.804022513344,
337.886489118789,337.96895488003,338.051419824483,338.133883979559,338.216347372668,
338.298810031216,338.381271982609,338.463733254248,338.546193873532,338.628653867859,
338.711113264623,338.793572091218,338.876030375035,338.958488143463,339.040945423888,
339.125078659299,339.207544657391,339.290009033747,339.372471898009,339.454933359799,
339.537393528721,339.619852514356,339.702310426273,339.787906271798,339.870371008398,
339.9528327804,340.035292026242,340.11774918422,340.200211702501,340.282669373356,
340.365128163307,340.387077190473),.UNSPECIFIED.);
#316=B_SPLINE_CURVE_WITH_KNOTS('',3,(#34495,#34496,#34497,#34498,#34499,
#34500,#34501,#34502,#34503,#34504,#34505,#34506,#34507,#34508,#34509,#34510,
#34511,#34512,#34513,#34514,#34515,#34516,#34517,#34518,#34519,#34520,#34521,
#34522,#34523,#34524,#34525,#34526,#34527,#34528,#34529,#34530,#34531,#34532,
#34533,#34534,#34535,#34536,#34537,#34538,#34539,#34540,#34541,#34542,#34543,
#34544,#34545,#34546,#34547,#34548,#34549,#34550,#34551,#34552,#34553,#34554,
#34555,#34556,#34557,#34558,#34559,#34560,#34561,#34562,#34563,#34564,#34565,
#34566,#34567,#34568,#34569,#34570,#34571,#34572,#34573,#34574,#34575,#34576,
#34577,#34578,#34579),.UNSPECIFIED.,.F.,.F.,(4,3,3,3,3,3,3,3,3,3,3,3,3,
3,3,3,3,3,3,3,3,3,3,3,3,3,3,3,4),(334.10356649952,334.185054976864,334.220806561041,
334.298322339304,334.375756639715,334.453125058142,334.530443143292,334.607726407336,
334.685003491648,334.762280072136,334.839570167533,334.916887801538,334.994294007862,
335.071746017176,335.149318825498,335.22056017241,335.29665931971,335.372665757179,
335.44859625978,335.5244675252,335.602643271341,335.678454145347,335.754259719948,
335.830074999942,335.90591499605,335.981830549012,336.057791521109,336.133846841639,
336.149873494327),.UNSPECIFIED.);
#317=B_SPLINE_CURVE_WITH_KNOTS('',3,(#34581,#34582,#34583,#34584,#34585,
#34586,#34587,#34588,#34589,#34590,#34591,#34592,#34593,#34594,#34595,#34596,
#34597,#34598,#34599,#34600,#34601,#34602,#34603,#34604,#34605,#34606,#34607,
#34608,#34609,#34610,#34611,#34612,#34613,#34614,#34615,#34616,#34617,#34618,
#34619,#34620,#34621,#34622,#34623,#34624,#34625,#34626,#34627,#34628,#34629,
#34630,#34631,#34632,#34633,#34634,#34635,#34636,#34637,#34638,#34639,#34640,
#34641,#34642,#34643,#34644,#34645,#34646,#34647,#34648,#34649,#34650,#34651,
#34652,#34653,#34654,#34655,#34656,#34657,#34658,#34659,#34660,#34661,#34662,
#34663,#34664,#34665),.UNSPECIFIED.,.F.,.F.,(4,3,3,3,3,3,3,3,3,3,3,3,3,
3,3,3,3,3,3,3,3,3,3,3,3,3,3,3,4),(334.103694651294,334.181285619702,334.258784764403,
334.33620770544,334.413570008341,334.490887195091,334.568182255047,334.645467173949,
334.722755958722,334.800062615803,334.87744180169,334.954858485744,335.032379990469,
335.099227456317,335.18071377075,335.262095853109,335.346179754917,335.42733707377,
335.508417857525,335.589407849559,335.598431460342,335.679444566632,335.760533260905,
335.84480881177,335.92611827816,336.00750517937,336.089012318135,336.097635464367,
336.150413934108),.UNSPECIFIED.);
#318=B_SPLINE_CURVE_WITH_KNOTS('',3,(#34666,#34667,#34668,#34669,#34670,
#34671,#34672,#34673,#34674,#34675,#34676,#34677,#34678,#34679,#34680,#34681,
#34682,#34683,#34684,#34685,#34686,#34687,#34688,#34689,#34690,#34691,#34692,
#34693,#34694,#34695,#34696,#34697,#34698,#34699,#34700,#34701,#34702,#34703,
#34704,#34705,#34706,#34707,#34708,#34709,#34710,#34711,#34712,#34713,#34714,
#34715,#34716,#34717,#34718,#34719,#34720,#34721,#34722,#34723,#34724,#34725,
#34726,#34727,#34728,#34729,#34730,#34731,#34732,#34733,#34734,#34735,#34736,
#34737,#34738,#34739,#34740,#34741,#34742,#34743,#34744,#34745,#34746,#34747,
#34748,#34749,#34750,#34751,#34752,#34753,#34754,#34755,#34756,#34757,#34758,
#34759,#34760,#34761,#34762,#34763,#34764,#34765,#34766,#34767,#34768,#34769,
#34770,#34771,#34772,#34773,#34774,#34775,#34776,#34777,#34778,#34779,#34780,
#34781,#34782,#34783,#34784,#34785,#34786,#34787,#34788,#34789,#34790,#34791,
#34792,#34793,#34794,#34795,#34796,#34797,#34798,#34799,#34800,#34801,#34802,
#34803,#34804,#34805,#34806,#34807,#34808,#34809,#34810,#34811,#34812,#34813,
#34814,#34815,#34816,#34817,#34818,#34819,#34820,#34821,#34822,#34823,#34824,
#34825,#34826,#34827,#34828,#34829,#34830,#34831,#34832,#34833,#34834),
 .UNSPECIFIED.,.F.,.F.,(4,3,3,3,3,3,3,3,3,3,3,3,3,3,3,3,3,3,3,3,3,3,3,3,
3,3,3,3,3,3,3,3,3,3,3,3,3,3,3,3,3,3,3,3,3,3,3,3,3,3,3,3,3,3,3,3,4),(336.150413934201,
336.227400235554,336.304308354968,336.381154357483,336.457954260505,336.537715411994,
336.61448474228,336.69125925539,336.768053400328,336.844881635197,336.921798512557,
336.998767926114,337.075842526394,337.096043472418,337.17290685707,337.24967668888,
337.326369224869,337.403000660035,337.479587140819,337.556445183275,337.633003506238,
337.709567840911,337.786152754038,337.863227435646,337.939934256515,338.017192868492,
338.094451480469,338.171981676929,338.249424771534,338.32679640559,338.404112169159,
338.481387611937,338.558648494356,338.635903800001,338.713167570295,338.790453848779,
338.867820661571,338.945228996279,339.022750552842,339.09285948852,339.170389606583,
339.247832635899,339.325204217725,339.402519942085,339.479795358647,339.557056234672,
339.634311546018,339.71157533411,339.788861642495,339.866228504101,339.943636898033,
340.021158530905,340.091267496571,340.168094604426,340.244843419813,340.321511037319,
340.387601338952),.UNSPECIFIED.);
#319=B_SPLINE_CURVE_WITH_KNOTS('',3,(#34840,#34841,#34842,#34843,#34844,
#34845,#34846,#34847,#34848,#34849,#34850,#34851,#34852,#34853,#34854,#34855,
#34856,#34857,#34858,#34859,#34860,#34861,#34862,#34863,#34864,#34865,#34866,
#34867,#34868,#34869,#34870,#34871,#34872,#34873,#34874,#34875,#34876,#34877,
#34878,#34879,#34880,#34881,#34882,#34883,#34884,#34885,#34886,#34887,#34888,
#34889,#34890,#34891,#34892,#34893,#34894,#34895,#34896,#34897,#34898,#34899,
#34900,#34901,#34902,#34903,#34904,#34905,#34906,#34907,#34908,#34909,#34910,
#34911,#34912,#34913,#34914,#34915,#34916,#34917,#34918,#34919,#34920,#34921,
#34922,#34923,#34924,#34925,#34926,#34927,#34928,#34929,#34930,#34931,#34932,
#34933,#34934,#34935,#34936,#34937,#34938,#34939,#34940,#34941,#34942,#34943,
#34944,#34945,#34946,#34947,#34948,#34949,#34950,#34951,#34952,#34953,#34954,
#34955,#34956,#34957,#34958,#34959,#34960,#34961,#34962,#34963,#34964,#34965,
#34966,#34967,#34968,#34969,#34970,#34971,#34972,#34973,#34974,#34975,#34976,
#34977,#34978,#34979,#34980,#34981,#34982,#34983,#34984,#34985,#34986,#34987,
#34988,#34989,#34990,#34991,#34992,#34993,#34994,#34995,#34996,#34997,#34998,
#34999,#35000,#35001,#35002,#35003,#35004,#35005,#35006,#35007,#35008),
 .UNSPECIFIED.,.F.,.F.,(4,3,3,3,3,3,3,3,3,3,3,3,3,3,3,3,3,3,3,3,3,3,3,3,
3,3,3,3,3,3,3,3,3,3,3,3,3,3,3,3,3,3,3,3,3,3,3,3,3,3,3,3,3,3,3,3,4),(342.434795335461,
342.510391140104,342.585928653286,342.665011204546,342.740491920252,342.815969007295,
342.891457617893,342.966972913604,343.042568927301,343.118212230254,343.193957241268,
343.218589063365,343.296106614983,343.373536834403,343.450895377298,343.528197847885,
343.605459809836,343.682707035618,343.759948546825,343.837198397058,343.914470641971,
343.991823599942,344.069217992251,344.146726319919,344.218342674735,344.295860043931,
344.373290111383,344.450648532652,344.527950911867,344.60521281263,344.682460023321,
344.75970154754,344.836951438886,344.914223753029,344.991576824255,345.068971354007,
345.146479858969,345.218096286104,345.294917483259,345.371649445473,345.448308423621,
345.524910610082,345.601472151963,345.678519370152,345.755063544796,345.831617824842,
345.908196789821,345.985610066734,346.062321547041,346.140085722257,346.217849897473,
346.295437931297,346.372936137223,346.450339998853,346.527689274207,346.604993913737,
346.67045654415),.UNSPECIFIED.);
#320=B_SPLINE_CURVE_WITH_KNOTS('',3,(#35009,#35010,#35011,#35012,#35013,
#35014,#35015,#35016,#35017,#35018,#35019,#35020,#35021,#35022,#35023,#35024,
#35025,#35026,#35027,#35028,#35029,#35030,#35031,#35032,#35033,#35034,#35035,
#35036,#35037,#35038,#35039,#35040,#35041,#35042,#35043,#35044,#35045,#35046,
#35047,#35048,#35049,#35050,#35051,#35052,#35053,#35054,#35055,#35056,#35057,
#35058,#35059,#35060,#35061,#35062,#35063,#35064,#35065,#35066,#35067,#35068,
#35069,#35070,#35071,#35072,#35073,#35074,#35075,#35076,#35077,#35078,#35079,
#35080,#35081,#35082,#35083,#35084),.UNSPECIFIED.,.F.,.F.,(4,3,3,3,3,3,
3,3,3,3,3,3,3,3,3,3,3,3,3,3,3,3,3,3,3,4),(340.387077190473,340.469538794326,
340.551999732297,340.634460031783,340.71691972018,340.799378824882,340.881837373281,
340.964295392767,341.046752910729,341.133430806389,341.215897592224,341.298362705568,
341.380826256073,341.463288353371,341.545749107072,341.628208626769,341.710667022037,
341.793124402434,341.8755907887,341.958053990714,342.040514446995,342.122972595905,
342.205438200785,342.287898079999,342.370362193363,342.433599241288),
 .UNSPECIFIED.);
#321=B_SPLINE_CURVE_WITH_KNOTS('',3,(#35086,#35087,#35088,#35089,#35090,
#35091,#35092,#35093,#35094,#35095,#35096,#35097,#35098,#35099,#35100,#35101,
#35102,#35103,#35104,#35105,#35106,#35107,#35108,#35109,#35110,#35111,#35112,
#35113,#35114,#35115,#35116,#35117,#35118,#35119,#35120,#35121,#35122,#35123,
#35124,#35125,#35126,#35127,#35128,#35129,#35130,#35131,#35132,#35133,#35134,
#35135,#35136,#35137,#35138,#35139,#35140,#35141,#35142,#35143,#35144,#35145,
#35146,#35147,#35148,#35149,#35150,#35151,#35152,#35153,#35154,#35155,#35156,
#35157,#35158,#35159,#35160,#35161,#35162,#35163,#35164),.UNSPECIFIED.,
 .F.,.F.,(4,3,3,3,3,3,3,3,3,3,3,3,3,3,3,3,3,3,3,3,3,3,3,3,3,3,4),(340.387601338952,
340.464183127824,340.542369674924,340.618929532378,340.69549783046,340.77208913748,
340.851485729266,340.92820838647,341.008941945546,341.089675504622,341.167270174056,
341.244772440167,341.322197925238,341.399562196615,341.476880777705,341.554176482177,
341.631461526833,341.708749918765,341.786055664291,341.863433704278,341.940848776023,
342.018369390294,342.088083512673,342.176003795807,342.263719859844,342.351021027598,
342.433599241288),.UNSPECIFIED.);
#322=B_SPLINE_CURVE_WITH_KNOTS('',3,(#35165,#35166,#35167,#35168,#35169,
#35170,#35171,#35172,#35173,#35174,#35175,#35176,#35177,#35178,#35179,#35180,
#35181,#35182,#35183,#35184,#35185,#35186,#35187,#35188,#35189,#35190,#35191,
#35192,#35193,#35194,#35195,#35196,#35197,#35198,#35199,#35200,#35201,#35202,
#35203,#35204,#35205,#35206,#35207,#35208,#35209,#35210,#35211,#35212,#35213,
#35214,#35215,#35216,#35217,#35218,#35219,#35220,#35221,#35222,#35223,#35224,
#35225,#35226,#35227,#35228,#35229,#35230,#35231,#35232,#35233,#35234,#35235,
#35236,#35237,#35238,#35239,#35240,#35241,#35242,#35243,#35244,#35245,#35246,
#35247,#35248,#35249,#35250,#35251,#35252,#35253,#35254,#35255,#35256,#35257,
#35258,#35259,#35260,#35261,#35262,#35263,#35264,#35265,#35266,#35267,#35268,
#35269,#35270,#35271,#35272,#35273,#35274,#35275,#35276,#35277,#35278,#35279,
#35280,#35281,#35282,#35283,#35284,#35285,#35286,#35287,#35288,#35289,#35290,
#35291,#35292,#35293,#35294,#35295,#35296,#35297,#35298,#35299,#35300,#35301,
#35302,#35303,#35304,#35305,#35306,#35307,#35308,#35309,#35310,#35311,#35312,
#35313,#35314,#35315,#35316,#35317,#35318,#35319,#35320,#35321),
 .UNSPECIFIED.,.F.,.F.,(4,3,3,3,3,3,3,3,3,3,3,3,3,3,3,3,3,3,3,3,3,3,3,3,
3,3,3,3,3,3,3,3,3,3,3,3,3,3,3,3,3,3,3,3,3,3,3,3,3,3,3,3,4),(342.433599241288,
342.516061447324,342.598523305064,342.680984821358,342.763446003055,342.845906857006,
342.928367390061,343.010827609067,343.093287520875,343.175747132333,343.258206450289,
343.340665481591,343.423124233088,343.505582711626,343.588040924054,343.670498877219,
343.752956577966,343.835414033144,343.917871249599,344.0038834761,344.087207820524,
344.169674425969,344.252140187211,344.334605131663,344.417069286739,344.499532679848,
344.581995338397,344.664457289789,344.746918561428,344.829379180712,344.911839175039,
344.994298571804,345.076757398399,345.159215682215,345.241673450643,345.324130731068,
345.40826396648,345.490729964571,345.573194340927,345.655657205189,345.73811866698,
345.820578835901,345.903037821536,345.985495733454,346.071091578978,346.153556315578,
346.23601808758,346.318477333422,346.4009344914,346.483397009681,346.565854680536,
346.648313470487,346.670262497652),.UNSPECIFIED.);
#323=B_SPLINE_CURVE_WITH_KNOTS('',3,(#35327,#35328,#35329,#35330,#35331,
#35332,#35333,#35334,#35335,#35336,#35337,#35338,#35339,#35340,#35341,#35342,
#35343,#35344,#35345,#35346,#35347,#35348,#35349,#35350,#35351,#35352,#35353,
#35354,#35355,#35356,#35357,#35358,#35359,#35360,#35361,#35362,#35363,#35364,
#35365,#35366,#35367,#35368,#35369,#35370,#35371,#35372,#35373,#35374,#35375,
#35376,#35377,#35378,#35379,#35380,#35381,#35382,#35383,#35384,#35385,#35386,
#35387,#35388,#35389,#35390,#35391,#35392,#35393,#35394,#35395,#35396,#35397,
#35398,#35399,#35400,#35401,#35402,#35403,#35404,#35405,#35406,#35407,#35408,
#35409,#35410,#35411,#35412,#35413,#35414,#35415,#35416,#35417,#35418,#35419,
#35420,#35421,#35422,#35423,#35424,#35425,#35426,#35427,#35428,#35429,#35430,
#35431,#35432,#35433,#35434,#35435,#35436,#35437,#35438,#35439,#35440,#35441,
#35442,#35443,#35444,#35445,#35446,#35447,#35448,#35449,#35450,#35451,#35452,
#35453,#35454,#35455,#35456,#35457,#35458,#35459,#35460,#35461,#35462,#35463,
#35464,#35465,#35466,#35467,#35468,#35469,#35470,#35471,#35472,#35473,#35474,
#35475,#35476,#35477,#35478,#35479,#35480,#35481,#35482,#35483,#35484,#35485,
#35486,#35487,#35488,#35489,#35490,#35491,#35492),.UNSPECIFIED.,.F.,.F.,
(4,3,3,3,3,3,3,3,3,3,3,3,3,3,3,3,3,3,3,3,3,3,3,3,3,3,3,3,3,3,3,3,3,3,3,
3,3,3,3,3,3,3,3,3,3,3,3,3,3,3,3,3,3,3,3,4),(348.71678454858,348.798749648545,
348.880854154498,348.964918298769,349.047377608491,349.132244170036,349.217110731581,
349.293959354768,349.370714201165,349.44739154057,349.524007580345,349.60057847897,
349.677614211967,349.754156630673,349.830704967236,349.907273798684,349.98467143475,
350.061362515703,350.139113429327,350.216864342951,350.294381894569,350.371812113989,
350.449170656884,350.526473127471,350.603735089421,350.680982315204,350.758223826411,
350.835473676644,350.912745921557,350.990098879528,351.067493271836,351.145001599505,
351.21661795432,351.294135323516,351.371565390967,351.448923812237,351.526226191452,
351.603488092215,351.680735302906,351.757976827124,351.83522671847,351.912499032614,
351.98985210384,352.067246633591,352.144755138553,352.216371565689,352.293207911534,
352.369951958647,352.446603917339,352.523203174201,352.599764352909,352.676302051195,
352.752847255585,352.829395570524,352.905987356481,352.952608162855),
 .UNSPECIFIED.);
#324=B_SPLINE_CURVE_WITH_KNOTS('',3,(#35493,#35494,#35495,#35496,#35497,
#35498,#35499,#35500,#35501,#35502,#35503,#35504,#35505,#35506,#35507,#35508,
#35509,#35510,#35511,#35512,#35513,#35514,#35515,#35516,#35517,#35518,#35519,
#35520,#35521,#35522,#35523,#35524,#35525,#35526,#35527,#35528,#35529,#35530,
#35531,#35532,#35533,#35534,#35535,#35536,#35537,#35538,#35539,#35540,#35541,
#35542,#35543,#35544,#35545,#35546,#35547,#35548,#35549,#35550,#35551,#35552,
#35553,#35554,#35555,#35556,#35557,#35558,#35559,#35560,#35561,#35562,#35563,
#35564,#35565,#35566,#35567,#35568,#35569,#35570,#35571,#35572,#35573,#35574,
#35575,#35576,#35577),.UNSPECIFIED.,.F.,.F.,(4,3,3,3,3,3,3,3,3,3,3,3,3,
3,3,3,3,3,3,3,3,3,3,3,3,3,3,3,4),(346.67045654415,346.747729075593,346.825002676091,
346.902291363443,346.981119399793,347.058515331763,347.138059420303,347.217603508843,
347.299087481798,347.380466845939,347.464720213086,347.545873708258,347.626950386218,
347.707935814007,347.717480314527,347.798488710431,347.879572967262,347.964019005499,
348.045325087206,348.126708876974,348.208213538003,348.217357120212,348.297778607236,
348.378089974019,348.458300350398,348.538389101135,348.618404721531,348.698337586771,
348.716784548467),.UNSPECIFIED.);
#325=B_SPLINE_CURVE_WITH_KNOTS('',3,(#35579,#35580,#35581,#35582,#35583,
#35584,#35585,#35586,#35587,#35588,#35589,#35590,#35591,#35592,#35593,#35594,
#35595,#35596,#35597,#35598,#35599,#35600,#35601,#35602,#35603,#35604,#35605,
#35606,#35607,#35608,#35609,#35610,#35611,#35612,#35613,#35614,#35615,#35616,
#35617,#35618,#35619,#35620,#35621,#35622,#35623,#35624,#35625,#35626,#35627,
#35628,#35629,#35630,#35631,#35632,#35633,#35634,#35635,#35636,#35637,#35638,
#35639,#35640,#35641,#35642,#35643,#35644,#35645,#35646,#35647,#35648,#35649,
#35650,#35651,#35652,#35653,#35654),.UNSPECIFIED.,.F.,.F.,(4,3,3,3,3,3,
3,3,3,3,3,3,3,3,3,3,3,3,3,3,3,3,3,3,3,4),(346.670262497652,346.752724101506,
346.835185039476,346.917645338962,347.000105027359,347.082564132061,347.16502268046,
347.247480699946,347.329938217908,347.416616113568,347.499082899404,347.581548012747,
347.664011563253,347.74647366055,347.828934414252,347.911393933949,347.993852329216,
348.076309709614,348.15877609588,348.241239297894,348.323699754174,348.406157903085,
348.488623507964,348.571083387179,348.653547500543,348.716784548467),
 .UNSPECIFIED.);
#326=B_SPLINE_CURVE_WITH_KNOTS('',3,(#35655,#35656,#35657,#35658,#35659,
#35660,#35661,#35662,#35663,#35664,#35665,#35666,#35667,#35668,#35669,#35670,
#35671,#35672,#35673,#35674,#35675,#35676,#35677,#35678,#35679,#35680,#35681,
#35682,#35683,#35684,#35685,#35686,#35687,#35688,#35689,#35690,#35691,#35692,
#35693,#35694,#35695,#35696,#35697,#35698,#35699,#35700,#35701,#35702,#35703,
#35704,#35705,#35706,#35707,#35708,#35709,#35710,#35711,#35712,#35713,#35714,
#35715,#35716,#35717,#35718,#35719,#35720,#35721,#35722,#35723,#35724,#35725,
#35726,#35727,#35728,#35729,#35730,#35731,#35732,#35733,#35734,#35735,#35736,
#35737,#35738,#35739,#35740,#35741,#35742,#35743,#35744,#35745,#35746,#35747,
#35748,#35749,#35750,#35751,#35752,#35753,#35754,#35755,#35756,#35757,#35758,
#35759,#35760,#35761,#35762,#35763,#35764,#35765,#35766,#35767,#35768,#35769,
#35770,#35771,#35772,#35773,#35774,#35775,#35776,#35777,#35778,#35779,#35780,
#35781,#35782,#35783,#35784,#35785,#35786,#35787,#35788,#35789,#35790,#35791,
#35792,#35793,#35794,#35795,#35796,#35797,#35798,#35799,#35800,#35801,#35802,
#35803,#35804,#35805,#35806,#35807,#35808,#35809,#35810,#35811,#35812,#35813,
#35814,#35815,#35816,#35817,#35818,#35819,#35820,#35821,#35822,#35823,#35824,
#35825,#35826),.UNSPECIFIED.,.F.,.F.,(4,3,3,3,3,3,3,3,3,3,3,3,3,3,3,3,3,
3,3,3,3,3,3,3,3,3,3,3,3,3,3,3,3,3,3,3,3,3,3,3,3,3,3,3,3,3,3,3,3,3,3,3,3,
3,3,3,3,4),(348.716784548467,348.806823303607,348.893179792152,348.979765980959,
349.06662943043,349.076939569029,349.158425883462,349.239807965821,349.323891867629,
349.405049186482,349.486129970237,349.56711996227,349.576143573055,349.657156679345,
349.738245373618,349.822520924484,349.903830390873,349.985217292084,350.066724430849,
350.07534757708,350.152875730289,350.23032260525,350.307703783958,350.385034801418,
350.462331156249,350.539621456585,350.616911364323,350.694214886321,350.771546034448,
350.848965524269,350.926430882691,351.004016268989,351.073755585131,351.150618969783,
351.227388801593,351.304081337581,351.380712772748,351.457299253532,351.534157295988,
351.610715618951,351.687279953624,351.763864866751,351.840939548359,351.917646369228,
351.994904981205,352.072163593182,352.149700020288,352.227148045033,352.304523313686,
352.385577908728,352.462853150381,352.540107610983,352.617355336625,352.694610366867,
352.771914614152,352.84924762751,352.92665352286,352.952960074025),
 .UNSPECIFIED.);
#327=B_SPLINE_CURVE_WITH_KNOTS('',3,(#35832,#35833,#35834,#35835,#35836,
#35837,#35838,#35839,#35840,#35841,#35842,#35843,#35844,#35845,#35846,#35847,
#35848,#35849,#35850,#35851,#35852,#35853,#35854,#35855,#35856,#35857,#35858,
#35859,#35860,#35861,#35862,#35863,#35864,#35865,#35866,#35867,#35868,#35869,
#35870,#35871,#35872,#35873,#35874,#35875,#35876,#35877,#35878,#35879,#35880,
#35881,#35882,#35883,#35884,#35885,#35886,#35887,#35888,#35889,#35890,#35891,
#35892,#35893,#35894,#35895,#35896,#35897,#35898,#35899,#35900,#35901,#35902,
#35903,#35904,#35905,#35906,#35907,#35908,#35909,#35910,#35911,#35912,#35913,
#35914,#35915,#35916,#35917,#35918,#35919,#35920,#35921,#35922,#35923,#35924,
#35925,#35926,#35927,#35928,#35929,#35930,#35931,#35932,#35933,#35934,#35935,
#35936,#35937,#35938,#35939,#35940,#35941,#35942,#35943,#35944,#35945,#35946,
#35947,#35948,#35949,#35950,#35951,#35952,#35953,#35954,#35955,#35956,#35957,
#35958,#35959,#35960,#35961,#35962,#35963,#35964,#35965,#35966,#35967,#35968,
#35969,#35970,#35971,#35972,#35973,#35974,#35975,#35976,#35977,#35978,#35979,
#35980,#35981,#35982,#35983,#35984,#35985,#35986,#35987,#35988,#35989,#35990,
#35991,#35992,#35993,#35994,#35995,#35996,#35997,#35998,#35999,#36000),
 .UNSPECIFIED.,.F.,.F.,(4,3,3,3,3,3,3,3,3,3,3,3,3,3,3,3,3,3,3,3,3,3,3,3,
3,3,3,3,3,3,3,3,3,3,3,3,3,3,3,3,3,3,3,3,3,3,3,3,3,3,3,3,3,3,3,3,4),(354.999969855647,
355.099329048981,355.20011625081,355.215632399798,355.293148178061,355.370582478472,
355.447950896899,355.525268982049,355.602552246093,355.679829330405,355.757105910892,
355.83439600629,355.911713640294,355.989119846618,356.066571855932,356.144144664254,
356.215386011167,356.292234634354,356.368989480751,356.445666820156,356.522282859931,
356.598853758556,356.675889491553,356.752431910259,356.828980246821,356.905549078269,
356.982946714336,357.059637795289,357.137388708912,357.215139622536,357.292657174154,
357.370087393574,357.447445936469,357.524748407056,357.602010369007,357.679257594789,
357.756499105997,357.833748956229,357.911021201142,357.988374159113,358.065768551422,
358.143276879091,358.214893233906,358.292410603102,358.369840670553,358.447199091823,
358.524501471038,358.601763371801,358.679010582492,358.75625210671,358.833501998056,
358.9107743122,358.988127383426,359.065521913177,359.14303041814,359.214646845275,
359.236895376301),.UNSPECIFIED.);
#328=B_SPLINE_CURVE_WITH_KNOTS('',3,(#36001,#36002,#36003,#36004,#36005,
#36006,#36007,#36008,#36009,#36010,#36011,#36012,#36013,#36014,#36015,#36016,
#36017,#36018,#36019,#36020,#36021,#36022,#36023,#36024,#36025,#36026,#36027,
#36028,#36029,#36030,#36031,#36032,#36033,#36034,#36035,#36036,#36037,#36038,
#36039,#36040,#36041,#36042,#36043,#36044,#36045,#36046,#36047,#36048,#36049,
#36050,#36051,#36052,#36053,#36054,#36055,#36056,#36057,#36058,#36059,#36060,
#36061,#36062,#36063,#36064,#36065,#36066,#36067,#36068,#36069,#36070,#36071,
#36072,#36073,#36074,#36075,#36076,#36077,#36078,#36079,#36080,#36081,#36082,
#36083,#36084,#36085),.UNSPECIFIED.,.F.,.F.,(4,3,3,3,3,3,3,3,3,3,3,3,3,
3,3,3,3,3,3,3,3,3,3,3,3,3,3,3,4),(352.952608162855,353.029299967087,353.106043896697,
353.182899467382,353.216125177059,353.293707800673,353.371197782882,353.448610760107,
353.525962313608,353.60326798052,353.680550573564,353.757822360508,353.835097360365,
353.912389591303,353.989754263668,354.0671558721,354.144663686709,354.215878788428,
354.297362761383,354.378742125522,354.46299549267,354.544148987842,354.6252256658,
354.70621109359,354.715755594113,354.791007671957,354.866272417376,354.941602667642,
354.999969855565),.UNSPECIFIED.);
#329=B_SPLINE_CURVE_WITH_KNOTS('',3,(#36087,#36088,#36089,#36090,#36091,
#36092,#36093,#36094,#36095,#36096,#36097,#36098,#36099,#36100,#36101,#36102,
#36103,#36104,#36105,#36106,#36107,#36108,#36109,#36110,#36111,#36112,#36113,
#36114,#36115,#36116,#36117,#36118,#36119,#36120,#36121,#36122,#36123,#36124,
#36125,#36126,#36127,#36128,#36129,#36130,#36131,#36132,#36133,#36134,#36135,
#36136,#36137,#36138,#36139,#36140,#36141,#36142,#36143,#36144,#36145,#36146,
#36147,#36148,#36149,#36150,#36151,#36152,#36153,#36154,#36155,#36156,#36157,
#36158,#36159,#36160,#36161,#36162,#36163,#36164,#36165,#36166,#36167,#36168,
#36169,#36170,#36171),.UNSPECIFIED.,.F.,.F.,(4,3,3,3,3,3,3,3,3,3,3,3,3,
3,3,3,3,3,3,3,3,3,3,3,3,3,3,3,4),(352.952960074025,353.03049316836,353.070571601233,
353.148101719296,353.225544748612,353.302916330438,353.380232054798,353.457507471359,
353.534768347385,353.612023658731,353.689287446823,353.766573755207,353.843940616813,
353.921349010745,353.998870643617,354.068979609284,354.145073751402,354.2210795021,
354.297013600867,354.372892715455,354.451194742664,354.52702406611,354.602852026218,
354.678693617442,354.754563843074,354.830515470671,354.906515871729,354.982615653516,
354.999308933125),.UNSPECIFIED.);
#330=B_SPLINE_CURVE_WITH_KNOTS('',3,(#36172,#36173,#36174,#36175,#36176,
#36177,#36178,#36179,#36180,#36181,#36182,#36183,#36184,#36185,#36186,#36187,
#36188,#36189,#36190,#36191,#36192,#36193,#36194,#36195,#36196,#36197,#36198,
#36199,#36200,#36201,#36202,#36203,#36204,#36205,#36206,#36207,#36208,#36209,
#36210,#36211,#36212,#36213,#36214,#36215,#36216,#36217,#36218,#36219,#36220,
#36221,#36222,#36223,#36224,#36225,#36226,#36227,#36228,#36229,#36230,#36231,
#36232,#36233,#36234,#36235,#36236,#36237,#36238,#36239,#36240,#36241,#36242,
#36243,#36244,#36245,#36246,#36247,#36248,#36249,#36250,#36251,#36252,#36253,
#36254,#36255,#36256,#36257,#36258,#36259,#36260,#36261,#36262,#36263,#36264,
#36265,#36266,#36267,#36268,#36269,#36270,#36271,#36272,#36273,#36274,#36275,
#36276,#36277,#36278,#36279,#36280,#36281,#36282,#36283,#36284,#36285,#36286,
#36287,#36288,#36289,#36290,#36291,#36292,#36293,#36294,#36295,#36296,#36297,
#36298,#36299,#36300,#36301,#36302,#36303,#36304,#36305,#36306,#36307,#36308,
#36309,#36310,#36311,#36312,#36313,#36314,#36315,#36316,#36317,#36318,#36319,
#36320,#36321,#36322,#36323,#36324,#36325,#36326,#36327,#36328),
 .UNSPECIFIED.,.F.,.F.,(4,3,3,3,3,3,3,3,3,3,3,3,3,3,3,3,3,3,3,3,3,3,3,3,
3,3,3,3,3,3,3,3,3,3,3,3,3,3,3,3,3,3,3,3,3,3,3,3,3,3,3,3,4),(354.999969855647,
355.082432061683,355.164893919423,355.247355435717,355.329816617414,355.412277471365,
355.49473800442,355.577198223426,355.659658135234,355.742117746692,355.824577064648,
355.90703609595,355.989494847447,356.071953325985,356.154411538413,356.236869491577,
356.319327192325,356.401784647503,356.484241863957,356.570254090459,356.653578434882,
356.736045040328,356.818510801569,356.900975746022,356.983439901098,357.065903294207,
357.148365952755,357.230827904148,357.313289175787,357.395749795071,357.478209789398,
357.560669186162,357.643128012757,357.725586296574,357.808044065001,357.890501345427,
357.974634580838,358.05710057893,358.139564955285,358.222027819548,358.304489281338,
358.386949450259,358.469408435895,358.551866347812,358.637462193337,358.719926929937,
358.802388701939,358.884847947781,358.967305105758,359.049767624039,359.132225294894,
359.214684084845,359.236633112011),.UNSPECIFIED.);
#331=B_SPLINE_CURVE_WITH_KNOTS('',3,(#36334,#36335,#36336,#36337,#36338,
#36339,#36340,#36341,#36342,#36343,#36344,#36345,#36346,#36347,#36348,#36349,
#36350,#36351,#36352,#36353,#36354,#36355,#36356,#36357,#36358,#36359,#36360,
#36361,#36362,#36363,#36364,#36365,#36366,#36367,#36368,#36369,#36370,#36371,
#36372,#36373,#36374,#36375,#36376,#36377,#36378,#36379,#36380,#36381,#36382,
#36383,#36384,#36385,#36386,#36387,#36388,#36389,#36390,#36391,#36392,#36393,
#36394,#36395,#36396,#36397,#36398,#36399,#36400,#36401,#36402,#36403,#36404,
#36405,#36406,#36407,#36408,#36409,#36410,#36411,#36412,#36413,#36414,#36415,
#36416,#36417,#36418,#36419,#36420,#36421,#36422,#36423,#36424,#36425,#36426,
#36427,#36428,#36429,#36430,#36431,#36432,#36433,#36434,#36435,#36436,#36437,
#36438,#36439,#36440,#36441,#36442,#36443,#36444,#36445,#36446,#36447,#36448,
#36449,#36450,#36451,#36452,#36453,#36454,#36455,#36456,#36457,#36458,#36459,
#36460,#36461,#36462,#36463,#36464,#36465,#36466,#36467,#36468,#36469,#36470,
#36471,#36472,#36473,#36474,#36475,#36476,#36477,#36478,#36479,#36480,#36481,
#36482,#36483,#36484,#36485,#36486,#36487,#36488,#36489,#36490,#36491,#36492,
#36493,#36494,#36495,#36496,#36497,#36498,#36499,#36500,#36501,#36502),
 .UNSPECIFIED.,.F.,.F.,(4,3,3,3,3,3,3,3,3,3,3,3,3,3,3,3,3,3,3,3,3,3,3,3,
3,3,3,3,3,3,3,3,3,3,3,3,3,3,3,3,3,3,3,3,3,3,3,3,3,3,3,3,3,3,3,3,4),(361.283155162939,
361.361992357148,361.440737819558,361.519381858553,361.597966756718,361.676494051824,
361.714030873699,361.795039269603,361.876123526435,361.960569564672,362.041875646379,
362.123259436148,362.204764097177,362.213907679383,362.291423457646,362.368857758057,
362.446226176484,362.523544261634,362.600827525678,362.678104609989,362.755381190477,
362.832671285875,362.909988919879,362.987395126203,363.064847135517,363.142419943839,
363.213661290753,363.29050991394,363.367264760337,363.443942099742,363.520558139517,
363.597129038141,363.674164771139,363.750707189845,363.827255526407,363.903824357855,
363.981221993922,364.057913074875,364.135663988498,364.213414902122,364.29093245374,
364.36836267316,364.445721216055,364.523023686642,364.600285648592,364.677532874375,
364.754774385583,364.832024235815,364.909296480728,364.986649438699,365.064043831008,
365.141552158676,365.213168513491,365.290675335511,365.368105554801,365.445456107835,
365.520350523813),.UNSPECIFIED.);
#332=B_SPLINE_CURVE_WITH_KNOTS('',3,(#36503,#36504,#36505,#36506,#36507,
#36508,#36509,#36510,#36511,#36512,#36513,#36514,#36515,#36516,#36517,#36518,
#36519,#36520,#36521,#36522,#36523,#36524,#36525,#36526,#36527,#36528,#36529,
#36530,#36531,#36532,#36533,#36534,#36535,#36536,#36537,#36538,#36539,#36540,
#36541,#36542,#36543,#36544,#36545,#36546,#36547,#36548,#36549,#36550,#36551,
#36552,#36553,#36554,#36555,#36556,#36557,#36558,#36559,#36560,#36561,#36562,
#36563,#36564,#36565,#36566,#36567,#36568,#36569,#36570,#36571,#36572,#36573,
#36574,#36575,#36576,#36577,#36578,#36579,#36580,#36581,#36582,#36583,#36584),
 .UNSPECIFIED.,.F.,.F.,(4,3,3,3,3,3,3,3,3,3,3,3,3,3,3,3,3,3,3,3,3,3,3,3,
3,3,3,4),(359.236895376301,359.313689066245,359.390398232431,359.467039107372,
359.543627869032,359.620180653732,359.696726555118,359.773272110338,359.849831895196,
359.926420491938,360.003098426069,360.079824295919,360.156668757418,360.214400456644,
360.291983080258,360.369473062467,360.446886039692,360.524237593193,360.601543260104,
360.678825853149,360.756097640093,360.83337263995,360.910664870888,360.988029543253,
361.065431151685,361.142938966293,361.214154068014,361.283155162827),
 .UNSPECIFIED.);
#333=B_SPLINE_CURVE_WITH_KNOTS('',3,(#36586,#36587,#36588,#36589,#36590,
#36591,#36592,#36593,#36594,#36595,#36596,#36597,#36598,#36599,#36600,#36601,
#36602,#36603,#36604,#36605,#36606,#36607,#36608,#36609,#36610,#36611,#36612,
#36613,#36614,#36615,#36616,#36617,#36618,#36619,#36620,#36621,#36622,#36623,
#36624,#36625,#36626,#36627,#36628,#36629,#36630,#36631,#36632,#36633,#36634,
#36635,#36636,#36637,#36638,#36639,#36640,#36641,#36642,#36643,#36644,#36645,
#36646,#36647,#36648,#36649,#36650,#36651,#36652,#36653,#36654,#36655,#36656,
#36657,#36658,#36659,#36660,#36661),.UNSPECIFIED.,.F.,.F.,(4,3,3,3,3,3,
3,3,3,3,3,3,3,3,3,3,3,3,3,3,3,3,3,3,3,4),(359.236633112011,359.319094715865,
359.401555653835,359.484015953321,359.566475641718,359.64893474642,359.731393294819,
359.813851314306,359.896308832267,359.982986727927,360.065453513763,360.147918627107,
360.230382177612,360.31284427491,360.395305028611,360.477764548308,360.560222943576,
360.642680323973,360.725146710239,360.807609912253,360.890070368533,360.972528517444,
361.054994122323,361.137454001538,361.219918114902,361.283155162826),
 .UNSPECIFIED.);
#334=B_SPLINE_CURVE_WITH_KNOTS('',3,(#36662,#36663,#36664,#36665,#36666,
#36667,#36668,#36669,#36670,#36671,#36672,#36673,#36674,#36675,#36676,#36677,
#36678,#36679,#36680,#36681,#36682,#36683,#36684,#36685,#36686,#36687,#36688,
#36689,#36690,#36691,#36692,#36693,#36694,#36695,#36696,#36697,#36698,#36699,
#36700,#36701,#36702,#36703,#36704,#36705,#36706,#36707,#36708,#36709,#36710,
#36711,#36712,#36713,#36714,#36715,#36716,#36717,#36718,#36719,#36720,#36721,
#36722,#36723,#36724,#36725,#36726,#36727,#36728,#36729,#36730,#36731,#36732,
#36733,#36734,#36735,#36736,#36737,#36738,#36739,#36740,#36741,#36742,#36743,
#36744,#36745,#36746,#36747,#36748,#36749,#36750,#36751,#36752,#36753,#36754,
#36755,#36756,#36757,#36758,#36759,#36760,#36761,#36762,#36763,#36764,#36765,
#36766,#36767,#36768,#36769,#36770,#36771,#36772,#36773,#36774,#36775,#36776,
#36777,#36778,#36779,#36780,#36781,#36782,#36783,#36784,#36785,#36786,#36787,
#36788,#36789,#36790,#36791,#36792,#36793,#36794,#36795,#36796,#36797,#36798,
#36799,#36800,#36801,#36802,#36803,#36804,#36805,#36806,#36807,#36808,#36809,
#36810,#36811,#36812,#36813,#36814,#36815,#36816,#36817,#36818),
 .UNSPECIFIED.,.F.,.F.,(4,3,3,3,3,3,3,3,3,3,3,3,3,3,3,3,3,3,3,3,3,3,3,3,
3,3,3,3,3,3,3,3,3,3,3,3,3,3,3,3,3,3,3,3,3,3,3,3,3,3,3,3,4),(361.283155162924,
361.365617368961,361.4480792267,361.530540742994,361.613001924692,361.695462778643,
361.777923311697,361.860383530704,361.942843442512,362.025303053969,362.107762371925,
362.190221403228,362.272680154724,362.355138633263,362.437596845691,362.520054798855,
362.602512499603,362.68496995478,362.767427171235,362.853439397734,362.936763742154,
363.0192303476,363.101696108841,363.184161053294,363.266625208369,363.349088601478,
363.431551260027,363.51401321142,363.596474483059,363.678935102343,363.76139509667,
363.843854493434,363.926313320029,364.008771603846,364.091229372273,364.173686652699,
364.257819888105,364.340285886196,364.422750262552,364.505213126814,364.587674588605,
364.670134757526,364.752593743161,364.835051655079,364.920647500593,365.003112237193,
365.085574009195,365.168033255037,365.250490413014,365.332952931295,365.41541060215,
365.497869392101,365.519818419191),.UNSPECIFIED.);
#335=B_SPLINE_CURVE_WITH_KNOTS('',3,(#36824,#36825,#36826,#36827,#36828,
#36829,#36830,#36831,#36832,#36833,#36834,#36835,#36836,#36837,#36838,#36839,
#36840,#36841,#36842,#36843,#36844,#36845,#36846,#36847,#36848,#36849,#36850,
#36851,#36852,#36853,#36854,#36855,#36856,#36857,#36858,#36859,#36860,#36861,
#36862,#36863,#36864,#36865,#36866,#36867,#36868,#36869,#36870,#36871,#36872,
#36873,#36874,#36875,#36876,#36877,#36878,#36879,#36880,#36881,#36882,#36883,
#36884,#36885,#36886,#36887,#36888,#36889,#36890,#36891,#36892,#36893,#36894,
#36895,#36896,#36897,#36898,#36899,#36900,#36901,#36902,#36903,#36904,#36905,
#36906,#36907,#36908,#36909,#36910,#36911,#36912,#36913,#36914,#36915,#36916,
#36917,#36918,#36919,#36920,#36921,#36922,#36923,#36924,#36925,#36926,#36927,
#36928,#36929,#36930,#36931,#36932,#36933,#36934,#36935,#36936,#36937,#36938,
#36939,#36940,#36941,#36942,#36943,#36944,#36945,#36946,#36947,#36948,#36949,
#36950,#36951,#36952,#36953,#36954,#36955,#36956,#36957,#36958,#36959,#36960,
#36961,#36962,#36963,#36964,#36965,#36966,#36967,#36968,#36969,#36970,#36971,
#36972,#36973,#36974,#36975,#36976,#36977,#36978,#36979,#36980),
 .UNSPECIFIED.,.F.,.F.,(4,3,3,3,3,3,3,3,3,3,3,3,3,3,3,3,3,3,3,3,3,3,3,3,
3,3,3,3,3,3,3,3,3,3,3,3,3,3,3,3,3,3,3,3,3,3,3,3,3,3,3,3,4),(367.566340470006,
367.648802676042,367.731264533782,367.813726050076,367.896187231773,367.978648085724,
368.061108618779,368.143568837785,368.226028749593,368.308488361051,368.390947679007,
368.473406710309,368.555865461806,368.638323940344,368.720782152772,368.803240105936,
368.885697806684,368.968155261862,369.050612478316,369.136624704818,369.219949049241,
369.302415654687,369.384881415928,369.467346360381,369.549810515457,369.632273908566,
369.714736567114,369.797198518507,369.879659790146,369.96212040943,370.044580403757,
370.127039800521,370.209498627116,370.291956910933,370.37441467936,370.456871959786,
370.541005195197,370.623471193289,370.705935569645,370.788398433907,370.870859895697,
370.953320064619,371.035779050254,371.118236962171,371.203832807696,371.286297544296,
371.368759316298,371.451218562141,371.533675720118,371.616138238399,371.698595909254,
371.781054699205,371.803003726371),.UNSPECIFIED.);
#336=B_SPLINE_CURVE_WITH_KNOTS('',3,(#36981,#36982,#36983,#36984,#36985,
#36986,#36987,#36988,#36989,#36990,#36991,#36992,#36993,#36994,#36995,#36996,
#36997,#36998,#36999,#37000,#37001,#37002,#37003,#37004,#37005,#37006,#37007,
#37008,#37009,#37010,#37011,#37012,#37013,#37014,#37015,#37016,#37017,#37018,
#37019,#37020,#37021,#37022,#37023,#37024,#37025,#37026,#37027,#37028,#37029,
#37030,#37031,#37032,#37033,#37034,#37035,#37036,#37037,#37038,#37039,#37040,
#37041,#37042,#37043,#37044,#37045,#37046,#37047,#37048,#37049,#37050,#37051,
#37052,#37053,#37054,#37055,#37056,#37057,#37058,#37059),.UNSPECIFIED.,
 .F.,.F.,(4,3,3,3,3,3,3,3,3,3,3,3,3,3,3,3,3,3,3,3,3,3,3,3,3,3,4),(365.520350523813,
365.59761345909,365.674861075843,365.752102564901,365.829351979924,365.9066233764,
365.983975351626,366.061368388441,366.138876067688,366.212922124861,366.289743322016,
366.36647528423,366.443134262378,366.519736448839,366.59629799072,366.673345208909,
366.749889383553,366.826443663599,366.903022628578,366.980435905491,367.057147385798,
367.134911561014,367.21267573623,367.304424888357,367.395763544426,367.486235917466,
367.566340470006),.UNSPECIFIED.);
#337=B_SPLINE_CURVE_WITH_KNOTS('',3,(#37061,#37062,#37063,#37064,#37065,
#37066,#37067,#37068,#37069,#37070,#37071,#37072,#37073,#37074,#37075,#37076,
#37077,#37078,#37079,#37080,#37081,#37082,#37083,#37084,#37085,#37086,#37087,
#37088,#37089,#37090,#37091,#37092,#37093,#37094,#37095,#37096,#37097,#37098,
#37099,#37100,#37101,#37102,#37103,#37104,#37105,#37106,#37107,#37108,#37109,
#37110,#37111,#37112,#37113,#37114,#37115,#37116,#37117,#37118,#37119,#37120,
#37121,#37122,#37123,#37124,#37125,#37126,#37127,#37128,#37129,#37130,#37131,
#37132,#37133,#37134,#37135,#37136),.UNSPECIFIED.,.F.,.F.,(4,3,3,3,3,3,
3,3,3,3,3,3,3,3,3,3,3,3,3,3,3,3,3,3,3,4),(365.519818419191,365.602280023045,
365.684740961015,365.767201260501,365.849660948898,365.9321200536,366.014578601999,
366.097036621485,366.179494139447,366.266172035107,366.348638820942,366.431103934286,
366.513567484791,366.596029582089,366.67849033579,366.760949855487,366.843408250755,
366.925865631152,367.008332017419,367.090795219433,367.173255675713,367.255713824624,
367.338179429503,367.420639308717,367.503103422081,367.566340470006),
 .UNSPECIFIED.);
#338=B_SPLINE_CURVE_WITH_KNOTS('',3,(#37137,#37138,#37139,#37140,#37141,
#37142,#37143,#37144,#37145,#37146,#37147,#37148,#37149,#37150,#37151,#37152,
#37153,#37154,#37155,#37156,#37157,#37158,#37159,#37160,#37161,#37162,#37163,
#37164,#37165,#37166,#37167,#37168,#37169,#37170,#37171,#37172,#37173,#37174,
#37175,#37176,#37177,#37178,#37179,#37180,#37181,#37182,#37183,#37184,#37185,
#37186,#37187,#37188,#37189,#37190,#37191,#37192,#37193,#37194,#37195,#37196,
#37197,#37198,#37199,#37200,#37201,#37202,#37203,#37204,#37205,#37206,#37207,
#37208,#37209,#37210,#37211,#37212,#37213,#37214,#37215,#37216,#37217,#37218,
#37219,#37220,#37221,#37222,#37223,#37224,#37225,#37226,#37227,#37228,#37229,
#37230,#37231,#37232,#37233,#37234,#37235,#37236,#37237,#37238,#37239,#37240,
#37241,#37242,#37243,#37244,#37245,#37246,#37247,#37248,#37249,#37250,#37251,
#37252,#37253,#37254,#37255,#37256,#37257,#37258,#37259,#37260,#37261,#37262,
#37263,#37264,#37265,#37266,#37267,#37268,#37269,#37270,#37271,#37272,#37273,
#37274,#37275,#37276,#37277,#37278,#37279,#37280,#37281,#37282,#37283,#37284,
#37285,#37286,#37287,#37288,#37289,#37290,#37291,#37292,#37293,#37294,#37295,
#37296,#37297,#37298,#37299,#37300,#37301,#37302,#37303,#37304,#37305),
 .UNSPECIFIED.,.F.,.F.,(4,3,3,3,3,3,3,3,3,3,3,3,3,3,3,3,3,3,3,3,3,3,3,3,
3,3,3,3,3,3,3,3,3,3,3,3,3,3,3,3,3,3,3,3,3,3,3,3,3,3,3,3,3,3,3,3,4),(367.566340470006,
367.648290370595,367.73037350154,367.812676296979,367.895091244229,367.977702695954,
368.046691721997,368.12352775412,368.200274769847,368.27694900741,368.353566646932,
368.430143823559,368.50701331187,368.583573414393,368.66014371154,368.736738772563,
368.813829011934,368.890556208516,368.967827969282,369.045099730048,369.122694399482,
369.200196665592,369.277622150663,369.35498642204,369.432305003131,369.509600707602,
369.586885752258,369.664174144191,369.741479889717,369.818857929704,369.896273001449,
369.97379361572,370.043507738099,370.124994052532,370.206376134891,370.290460036699,
370.371617355552,370.452698139307,370.533688131341,370.542711742124,370.623724848415,
370.704813542688,370.789089093553,370.870398559943,370.951785461154,371.033292599919,
371.04191574615,371.11945589795,371.196912152052,371.274287332535,371.351616341408,
371.428913220703,371.506191991676,371.583487044263,371.660788730736,371.738144147497,
371.802470582125),.UNSPECIFIED.);
#339=B_SPLINE_CURVE_WITH_KNOTS('',3,(#37311,#37312,#37313,#37314,#37315,
#37316,#37317,#37318,#37319,#37320,#37321,#37322,#37323,#37324,#37325,#37326,
#37327,#37328,#37329,#37330,#37331,#37332,#37333,#37334,#37335,#37336,#37337,
#37338,#37339,#37340,#37341,#37342,#37343,#37344,#37345,#37346,#37347,#37348,
#37349,#37350,#37351,#37352,#37353,#37354,#37355,#37356,#37357,#37358,#37359,
#37360,#37361,#37362,#37363,#37364,#37365,#37366,#37367,#37368,#37369,#37370,
#37371,#37372,#37373,#37374,#37375,#37376,#37377,#37378,#37379,#37380,#37381,
#37382,#37383,#37384,#37385,#37386,#37387,#37388,#37389,#37390,#37391,#37392,
#37393,#37394,#37395,#37396,#37397,#37398,#37399,#37400,#37401,#37402,#37403,
#37404,#37405,#37406,#37407,#37408,#37409,#37410,#37411,#37412,#37413,#37414,
#37415,#37416,#37417,#37418,#37419,#37420,#37421,#37422,#37423,#37424,#37425,
#37426,#37427,#37428,#37429,#37430,#37431,#37432,#37433,#37434,#37435,#37436,
#37437,#37438,#37439,#37440,#37441,#37442,#37443,#37444,#37445,#37446,#37447,
#37448,#37449,#37450,#37451,#37452,#37453,#37454,#37455,#37456,#37457,#37458,
#37459,#37460,#37461,#37462,#37463,#37464,#37465,#37466,#37467,#37468,#37469,
#37470,#37471,#37472,#37473,#37474,#37475,#37476,#37477,#37478,#37479),
 .UNSPECIFIED.,.F.,.F.,(4,3,3,3,3,3,3,3,3,3,3,3,3,3,3,3,3,3,3,3,3,3,3,3,
3,3,3,3,3,3,3,3,3,3,3,3,3,3,3,3,3,3,3,3,3,3,3,3,3,3,3,3,3,3,3,3,4),(373.849525777186,
373.939882086844,374.027315055066,374.119133035441,374.210951015816,374.28853363943,
374.366023621639,374.443436598864,374.520788152365,374.598093819277,374.675376412322,
374.752648199266,374.829923199122,374.907215430061,374.984580102425,375.061981710858,
375.139489525466,375.210704627185,375.29218860014,375.373567964279,375.457821331427,
375.538974826598,375.620051504557,375.701036932347,375.71058143287,375.791589828774,
375.872674085606,375.957120123843,376.03842620555,376.119809995319,376.201314656348,
376.210458238554,376.287974016817,376.365408317228,376.442776735655,376.520094820805,
376.59737808485,376.674655169161,376.751931749649,376.829221845046,376.906539479051,
376.983945685375,377.061397694688,377.13897050301,377.210211849924,377.287067742821,
377.363828411422,377.440510132449,377.521143703061,377.597712851444,377.674257387839,
377.750791894756,377.827330946169,377.903916893023,377.980530118534,378.057216121923,
378.085578697343),.UNSPECIFIED.);
#340=B_SPLINE_CURVE_WITH_KNOTS('',3,(#37480,#37481,#37482,#37483,#37484,
#37485,#37486,#37487,#37488,#37489,#37490,#37491,#37492,#37493,#37494,#37495,
#37496,#37497,#37498,#37499,#37500,#37501,#37502,#37503,#37504,#37505,#37506,
#37507,#37508,#37509,#37510,#37511,#37512,#37513,#37514,#37515,#37516,#37517,
#37518,#37519,#37520,#37521,#37522,#37523,#37524,#37525,#37526,#37527,#37528,
#37529,#37530,#37531,#37532,#37533,#37534,#37535,#37536,#37537,#37538,#37539,
#37540,#37541,#37542,#37543,#37544,#37545,#37546,#37547,#37548,#37549,#37550,
#37551,#37552,#37553,#37554,#37555),.UNSPECIFIED.,.F.,.F.,(4,3,3,3,3,3,
3,3,3,3,3,3,3,3,3,3,3,3,3,3,3,3,3,3,3,4),(371.803003726371,371.885465330225,
371.967926268195,372.050386567681,372.132846256078,372.21530536078,372.297763909179,
372.380221928665,372.462679446627,372.549357342287,372.631824128122,372.714289241466,
372.796752791971,372.879214889269,372.96167564297,373.044135162667,373.126593557935,
373.209050938332,373.291517324598,373.373980526612,373.456440982893,373.538899131804,
373.621364736683,373.703824615897,373.786288729261,373.849525777186),
 .UNSPECIFIED.);
#341=B_SPLINE_CURVE_WITH_KNOTS('',3,(#37557,#37558,#37559,#37560,#37561,
#37562,#37563,#37564,#37565,#37566,#37567,#37568,#37569,#37570,#37571,#37572,
#37573,#37574,#37575,#37576,#37577,#37578,#37579,#37580,#37581,#37582,#37583,
#37584,#37585,#37586,#37587,#37588,#37589,#37590,#37591,#37592,#37593,#37594,
#37595,#37596,#37597,#37598,#37599,#37600,#37601,#37602,#37603,#37604,#37605,
#37606,#37607,#37608,#37609,#37610,#37611,#37612,#37613,#37614,#37615,#37616,
#37617,#37618,#37619,#37620,#37621,#37622,#37623,#37624,#37625,#37626,#37627,
#37628,#37629,#37630,#37631,#37632,#37633,#37634,#37635,#37636,#37637,#37638),
 .UNSPECIFIED.,.F.,.F.,(4,3,3,3,3,3,3,3,3,3,3,3,3,3,3,3,3,3,3,3,3,3,3,3,
3,3,3,4),(371.802470582125,371.879927317619,371.96012553591,372.040323754201,
372.117187138853,372.193956970663,372.270649506651,372.347280941818,372.423867422602,
372.500725465058,372.577283788021,372.653848122693,372.730433035821,372.807507717428,
372.884214538297,372.961473150274,373.038731762251,373.115212093748,373.191604985852,
373.267926963156,373.344189739056,373.420420198739,373.496633175304,373.572843488199,
373.649093809448,373.725365467059,373.801709882622,373.849525777084),
 .UNSPECIFIED.);
#342=B_SPLINE_CURVE_WITH_KNOTS('',3,(#37639,#37640,#37641,#37642,#37643,
#37644,#37645,#37646,#37647,#37648,#37649,#37650,#37651,#37652,#37653,#37654,
#37655,#37656,#37657,#37658,#37659,#37660,#37661,#37662,#37663,#37664,#37665,
#37666,#37667,#37668,#37669,#37670,#37671,#37672,#37673,#37674,#37675,#37676,
#37677,#37678,#37679,#37680,#37681,#37682,#37683,#37684,#37685,#37686,#37687,
#37688,#37689,#37690,#37691,#37692,#37693,#37694,#37695,#37696,#37697,#37698,
#37699,#37700,#37701,#37702,#37703,#37704,#37705,#37706,#37707,#37708,#37709,
#37710,#37711,#37712,#37713,#37714,#37715,#37716,#37717,#37718,#37719,#37720,
#37721,#37722,#37723,#37724,#37725,#37726,#37727,#37728,#37729,#37730,#37731,
#37732,#37733,#37734,#37735,#37736,#37737,#37738,#37739,#37740,#37741,#37742,
#37743,#37744,#37745,#37746,#37747,#37748,#37749,#37750,#37751,#37752,#37753,
#37754,#37755,#37756,#37757,#37758,#37759,#37760,#37761,#37762,#37763,#37764,
#37765,#37766,#37767,#37768,#37769,#37770,#37771,#37772,#37773,#37774,#37775,
#37776,#37777,#37778,#37779,#37780,#37781,#37782,#37783,#37784,#37785,#37786,
#37787,#37788,#37789,#37790,#37791,#37792,#37793,#37794,#37795,#37796,#37797,
#37798,#37799,#37800,#37801,#37802,#37803,#37804,#37805,#37806,#37807),
 .UNSPECIFIED.,.F.,.F.,(4,3,3,3,3,3,3,3,3,3,3,3,3,3,3,3,3,3,3,3,3,3,3,3,
3,3,3,3,3,3,3,3,3,3,3,3,3,3,3,3,3,3,3,3,3,3,3,3,3,3,3,3,3,3,3,3,4),(373.849525777185,
373.962412552688,374.037139770302,374.114669888365,374.192112917681,374.269484499507,
374.346800223867,374.424075640428,374.501336516453,374.5785918278,374.655855615891,
374.733141924275,374.810508785882,374.887917179814,374.965438812686,375.035547778353,
375.112383810476,375.189130826203,375.265805063766,375.342422703287,375.418999879914,
375.495869368226,375.572429470748,375.648999767896,375.725594828918,375.80268506829,
375.879412264871,375.956684025638,376.033955786404,376.111550455838,376.189052721949,
376.266478207019,376.343842478396,376.421161059487,376.498456763959,376.575741808615,
376.653030200548,376.730335946073,376.807713986061,376.885129057805,376.962649672077,
377.032363794455,377.113850108888,377.195232191247,377.279316093056,377.360473411909,
377.441554195663,377.522544187697,377.531567798481,377.612580904771,377.693669599045,
377.77794514991,377.8592546163,377.94064151751,378.022148656275,378.030771802506,
378.086546493803),.UNSPECIFIED.);
#343=B_SPLINE_CURVE_WITH_KNOTS('',3,(#37813,#37814,#37815,#37816,#37817,
#37818,#37819,#37820,#37821,#37822,#37823,#37824,#37825,#37826,#37827,#37828,
#37829,#37830,#37831,#37832,#37833,#37834,#37835,#37836,#37837,#37838,#37839,
#37840,#37841,#37842,#37843,#37844,#37845,#37846,#37847,#37848,#37849,#37850,
#37851,#37852,#37853,#37854,#37855,#37856,#37857,#37858,#37859,#37860,#37861,
#37862,#37863,#37864,#37865,#37866,#37867,#37868,#37869,#37870,#37871,#37872,
#37873,#37874,#37875,#37876,#37877,#37878,#37879,#37880,#37881,#37882,#37883,
#37884,#37885,#37886,#37887,#37888,#37889,#37890,#37891,#37892,#37893,#37894,
#37895,#37896,#37897,#37898,#37899,#37900,#37901,#37902,#37903,#37904,#37905,
#37906,#37907,#37908,#37909,#37910,#37911,#37912,#37913,#37914,#37915,#37916,
#37917,#37918,#37919,#37920,#37921,#37922,#37923,#37924,#37925,#37926,#37927,
#37928,#37929,#37930,#37931,#37932,#37933,#37934,#37935,#37936,#37937,#37938,
#37939,#37940,#37941,#37942,#37943,#37944,#37945,#37946,#37947,#37948,#37949,
#37950,#37951,#37952,#37953,#37954,#37955,#37956,#37957,#37958,#37959,#37960,
#37961,#37962,#37963,#37964,#37965,#37966,#37967,#37968,#37969,#37970,#37971,
#37972,#37973,#37974,#37975,#37976,#37977,#37978,#37979,#37980,#37981,#37982,
#37983,#37984),.UNSPECIFIED.,.F.,.F.,(4,3,3,3,3,3,3,3,3,3,3,3,3,3,3,3,3,
3,3,3,3,3,3,3,3,3,3,3,3,3,3,3,3,3,3,3,3,3,3,3,3,3,3,3,3,3,3,3,3,3,3,3,3,
3,3,3,3,4),(380.132711084365,380.209472684032,380.286293881187,380.363025843401,
380.439684821549,380.516287008011,380.592848549892,380.66989576808,380.746439942725,
380.82299422277,380.89957318775,380.976986464663,381.05369794497,381.131462120185,
381.209226295401,381.286808919015,381.364298901224,381.441711878449,381.51906343195,
381.596369098861,381.673651691906,381.750923478849,381.828198478706,381.905490709644,
381.982855382009,382.060256990441,382.137764805049,382.208979906771,382.290463879726,
382.371843243866,382.456096611013,382.537250106185,382.618326784144,382.699312211935,
382.708856712455,382.789865108359,382.87094936519,382.955395403427,383.036701485134,
383.118085274902,383.199589935931,383.20873351814,383.286249296403,383.363683596814,
383.441052015241,383.518370100391,383.595653364436,383.672930448747,383.750207029235,
383.827497124633,383.904814758637,383.982220964962,384.059672974275,384.137245782597,
384.208487129509,384.289356128012,384.366119952296,384.370225126515),
 .UNSPECIFIED.);
#344=B_SPLINE_CURVE_WITH_KNOTS('',3,(#37985,#37986,#37987,#37988,#37989,
#37990,#37991,#37992,#37993,#37994,#37995,#37996,#37997,#37998,#37999,#38000,
#38001,#38002,#38003,#38004,#38005,#38006,#38007,#38008,#38009,#38010,#38011,
#38012,#38013,#38014,#38015,#38016,#38017,#38018,#38019,#38020,#38021,#38022,
#38023,#38024,#38025,#38026,#38027,#38028,#38029,#38030,#38031,#38032,#38033,
#38034,#38035,#38036,#38037,#38038,#38039,#38040,#38041,#38042,#38043,#38044,
#38045,#38046,#38047,#38048,#38049,#38050,#38051,#38052,#38053,#38054,#38055,
#38056,#38057,#38058,#38059,#38060,#38061,#38062,#38063,#38064,#38065,#38066),
 .UNSPECIFIED.,.F.,.F.,(4,3,3,3,3,3,3,3,3,3,3,3,3,3,3,3,3,3,3,3,3,3,3,3,
3,3,3,4),(378.085578697343,378.162400136614,378.209965461293,378.287483012911,
378.364913232331,378.442271775226,378.519574245813,378.596836207763,378.674083433546,
378.751324944753,378.828574794986,378.905847039899,378.98319999787,379.060594390178,
379.138102717847,379.209719072662,379.286373742231,379.362941556512,379.43943891038,
379.515882139391,379.592985757496,379.669379149644,379.745770602541,379.822174824489,
379.899808889424,379.976317652966,380.054514368598,380.132711084231),
 .UNSPECIFIED.);
#345=B_SPLINE_CURVE_WITH_KNOTS('',3,(#38068,#38069,#38070,#38071,#38072,
#38073,#38074,#38075,#38076,#38077,#38078,#38079,#38080,#38081,#38082,#38083,
#38084,#38085,#38086,#38087,#38088,#38089,#38090,#38091,#38092,#38093,#38094,
#38095,#38096,#38097,#38098,#38099,#38100,#38101,#38102,#38103,#38104,#38105,
#38106,#38107,#38108,#38109,#38110,#38111,#38112,#38113,#38114,#38115,#38116,
#38117,#38118,#38119,#38120,#38121,#38122,#38123,#38124,#38125,#38126,#38127,
#38128,#38129,#38130,#38131,#38132,#38133,#38134,#38135,#38136,#38137,#38138,
#38139,#38140,#38141,#38142,#38143,#38144,#38145,#38146,#38147,#38148,#38149),
 .UNSPECIFIED.,.F.,.F.,(4,3,3,3,3,3,3,3,3,3,3,3,3,3,3,3,3,3,3,3,3,3,3,3,
3,3,3,4),(378.086546493803,378.164014608403,378.241412658057,378.318756189873,
378.396060711637,378.475200599002,378.552489271051,378.629787960677,378.707110677723,
378.787627960932,378.865082320076,378.942592443613,379.020205864669,379.029179810557,
379.106043195209,379.182813027019,379.259505563008,379.336136998175,379.412723478958,
379.489581521414,379.566139844378,379.64270417905,379.719289092178,379.796363773785,
379.873070594654,379.950329206631,380.027587818608,380.132711084365),
 .UNSPECIFIED.);
#346=B_SPLINE_CURVE_WITH_KNOTS('',3,(#38150,#38151,#38152,#38153,#38154,
#38155,#38156,#38157,#38158,#38159,#38160,#38161,#38162,#38163,#38164,#38165,
#38166,#38167,#38168,#38169,#38170,#38171,#38172,#38173,#38174,#38175,#38176,
#38177,#38178,#38179,#38180,#38181,#38182,#38183,#38184,#38185,#38186,#38187,
#38188,#38189,#38190,#38191,#38192,#38193,#38194,#38195,#38196,#38197,#38198,
#38199,#38200,#38201,#38202,#38203,#38204,#38205,#38206,#38207,#38208,#38209,
#38210,#38211,#38212,#38213,#38214,#38215,#38216,#38217,#38218,#38219,#38220,
#38221,#38222,#38223,#38224,#38225,#38226,#38227,#38228,#38229,#38230,#38231,
#38232,#38233,#38234,#38235,#38236,#38237,#38238,#38239,#38240,#38241,#38242,
#38243,#38244,#38245,#38246,#38247,#38248,#38249,#38250,#38251,#38252,#38253,
#38254,#38255,#38256,#38257,#38258,#38259,#38260,#38261,#38262,#38263,#38264,
#38265,#38266,#38267,#38268,#38269,#38270,#38271,#38272,#38273,#38274,#38275,
#38276,#38277,#38278,#38279,#38280,#38281,#38282,#38283,#38284,#38285,#38286,
#38287,#38288,#38289,#38290,#38291,#38292,#38293,#38294,#38295,#38296,#38297,
#38298,#38299,#38300,#38301,#38302,#38303,#38304,#38305,#38306,#38307,#38308,
#38309,#38310,#38311,#38312,#38313,#38314,#38315,#38316,#38317,#38318),
 .UNSPECIFIED.,.F.,.F.,(4,3,3,3,3,3,3,3,3,3,3,3,3,3,3,3,3,3,3,3,3,3,3,3,
3,3,3,3,3,3,3,3,3,3,3,3,3,3,3,3,3,3,3,3,3,3,3,3,3,3,3,3,3,3,3,3,4),(380.132711084509,
380.209146011696,380.285502285353,380.361796391818,380.438044762713,380.51427208158,
380.590490501068,380.666714837056,380.74295990752,380.819281847043,380.895645188911,
380.972115510485,381.025995826659,381.103525944722,381.180968974038,381.258340555864,
381.335656280224,381.412931696785,381.49019257281,381.567447884157,381.644711672248,
381.721997980632,381.799364842238,381.87677323617,381.954294869042,382.02440383471,
382.101239866833,382.17798688256,382.254661120123,382.331278759644,382.407855936271,
382.484725424582,382.561285527105,382.637855824252,382.714450885275,382.791541124646,
382.868268321228,382.945540081994,383.022811842761,383.100406512195,383.177908778305,
383.255334263376,383.332698534753,383.410017115843,383.487312820315,383.564597864971,
383.641886256904,383.71919200243,383.796570042417,383.873985114162,383.951505728433,
384.021219850812,384.102728867264,384.184095183531,384.265374191124,384.346544891823,
384.369798917099),.UNSPECIFIED.);
#347=B_SPLINE_CURVE_WITH_KNOTS('',3,(#38324,#38325,#38326,#38327,#38328,
#38329,#38330,#38331,#38332,#38333,#38334,#38335,#38336,#38337,#38338,#38339,
#38340,#38341,#38342,#38343,#38344,#38345,#38346,#38347,#38348,#38349,#38350,
#38351,#38352,#38353,#38354,#38355,#38356,#38357,#38358,#38359,#38360,#38361,
#38362,#38363,#38364,#38365,#38366,#38367,#38368,#38369,#38370,#38371,#38372,
#38373,#38374,#38375,#38376,#38377,#38378,#38379,#38380,#38381,#38382,#38383,
#38384,#38385,#38386,#38387,#38388,#38389,#38390,#38391,#38392,#38393,#38394,
#38395,#38396,#38397,#38398,#38399,#38400,#38401,#38402,#38403,#38404,#38405,
#38406,#38407,#38408,#38409,#38410,#38411,#38412,#38413,#38414,#38415,#38416,
#38417,#38418,#38419,#38420,#38421,#38422,#38423,#38424,#38425,#38426,#38427,
#38428,#38429,#38430,#38431,#38432,#38433,#38434,#38435,#38436,#38437,#38438,
#38439,#38440,#38441,#38442,#38443,#38444,#38445,#38446,#38447,#38448,#38449,
#38450,#38451,#38452,#38453,#38454,#38455,#38456,#38457,#38458,#38459,#38460,
#38461,#38462,#38463,#38464,#38465,#38466,#38467,#38468,#38469,#38470,#38471,
#38472,#38473,#38474,#38475,#38476,#38477,#38478,#38479,#38480,#38481,#38482,
#38483,#38484,#38485,#38486,#38487,#38488,#38489,#38490,#38491,#38492,#38493,
#38494,#38495),.UNSPECIFIED.,.F.,.F.,(4,3,3,3,3,3,3,3,3,3,3,3,3,3,3,3,3,
3,3,3,3,3,3,3,3,3,3,3,3,3,3,3,3,3,3,3,3,3,3,3,3,3,3,3,3,3,3,3,3,3,3,3,3,
3,3,3,3,4),(386.415896391638,386.492266579159,386.568580662424,386.648476575073,
386.724737129527,386.800994886678,386.877264638518,386.953561182954,387.029937546182,
387.106360703212,387.182883946858,387.207747963617,387.284569160772,387.361301122986,
387.437960101134,387.514562287595,387.591123829476,387.668171047665,387.744715222309,
387.821269502354,387.897848467334,387.975261744247,388.051973224554,388.129737399771,
388.207501574987,388.285084198601,388.36257418081,388.439987158035,388.517338711537,
388.594644378448,388.671926971493,388.749198758437,388.826473758294,388.903765989233,
388.981130661597,389.05853227003,389.136040084638,389.207255186356,389.288739159311,
389.370118523451,389.454371890598,389.53552538577,389.616602063728,389.697587491518,
389.707131992041,389.788140387945,389.869224644777,389.953670683014,390.034976764721,
390.116360554489,390.197865215518,390.207008797725,390.284529776728,390.361971240382,
390.439334128285,390.516651255725,390.593936971202,390.65265496374),
 .UNSPECIFIED.);
#348=B_SPLINE_CURVE_WITH_KNOTS('',3,(#38496,#38497,#38498,#38499,#38500,
#38501,#38502,#38503,#38504,#38505,#38506,#38507,#38508,#38509,#38510,#38511,
#38512,#38513,#38514,#38515,#38516,#38517,#38518,#38519,#38520,#38521,#38522,
#38523,#38524,#38525,#38526,#38527,#38528,#38529,#38530,#38531,#38532,#38533,
#38534,#38535,#38536,#38537,#38538,#38539,#38540,#38541,#38542,#38543,#38544,
#38545,#38546,#38547,#38548,#38549,#38550,#38551,#38552,#38553,#38554,#38555,
#38556,#38557,#38558,#38559,#38560,#38561,#38562,#38563,#38564,#38565,#38566,
#38567,#38568,#38569,#38570,#38571,#38572,#38573,#38574),.UNSPECIFIED.,
 .F.,.F.,(4,3,3,3,3,3,3,3,3,3,3,3,3,3,3,3,3,3,3,3,3,3,3,3,3,3,4),(384.370225126515,
384.446895198235,384.52350568592,384.600072743613,384.676622302571,384.753164657178,
384.829714382817,384.906286057132,384.982939517875,385.059634903868,385.13644705767,
385.208240740879,385.285758292497,385.363188511917,385.440547054812,385.5178495254,
385.59511148735,385.672358713133,385.74960022434,385.826850074573,385.904122319486,
385.981475277457,386.058869669766,386.136377997434,386.207994352248,386.315585392158,
386.415896391545),.UNSPECIFIED.);
#349=B_SPLINE_CURVE_WITH_KNOTS('',3,(#38576,#38577,#38578,#38579,#38580,
#38581,#38582,#38583,#38584,#38585,#38586,#38587,#38588,#38589,#38590,#38591,
#38592,#38593,#38594,#38595,#38596,#38597,#38598,#38599,#38600,#38601,#38602,
#38603,#38604,#38605,#38606,#38607,#38608,#38609,#38610,#38611,#38612,#38613,
#38614,#38615,#38616,#38617,#38618,#38619,#38620,#38621,#38622,#38623,#38624,
#38625,#38626,#38627,#38628,#38629,#38630,#38631,#38632,#38633,#38634,#38635,
#38636,#38637,#38638,#38639,#38640,#38641,#38642,#38643,#38644,#38645,#38646,
#38647,#38648,#38649,#38650,#38651,#38652,#38653,#38654,#38655,#38656,#38657),
 .UNSPECIFIED.,.F.,.F.,(4,3,3,3,3,3,3,3,3,3,3,3,3,3,3,3,3,3,3,3,3,3,3,3,
3,3,3,4),(384.369798917099,384.450830355207,384.520423854837,384.601436961128,
384.6825256554,384.766801206265,384.848110672655,384.929497573866,385.011004712631,
385.019627858862,385.097156012071,385.174602887032,385.251984065739,385.3293150832,
385.40661143803,385.483901738366,385.561191646104,385.638495168102,385.71582631623,
385.793245806051,385.870711164473,385.948296550771,386.018035866913,386.103676425215,
386.188941402707,386.273971573959,386.358616605109,386.415896391545),
 .UNSPECIFIED.);
#350=B_SPLINE_CURVE_WITH_KNOTS('',3,(#38658,#38659,#38660,#38661,#38662,
#38663,#38664,#38665,#38666,#38667,#38668,#38669,#38670,#38671,#38672,#38673,
#38674,#38675,#38676,#38677,#38678,#38679,#38680,#38681,#38682,#38683,#38684,
#38685,#38686,#38687,#38688,#38689,#38690,#38691,#38692,#38693,#38694,#38695,
#38696,#38697,#38698,#38699,#38700,#38701,#38702,#38703,#38704,#38705,#38706,
#38707,#38708,#38709,#38710,#38711,#38712,#38713,#38714,#38715,#38716,#38717,
#38718,#38719,#38720,#38721,#38722,#38723,#38724,#38725,#38726,#38727,#38728,
#38729,#38730,#38731,#38732,#38733,#38734,#38735,#38736,#38737,#38738,#38739,
#38740,#38741,#38742,#38743,#38744,#38745,#38746,#38747,#38748,#38749,#38750,
#38751,#38752,#38753,#38754,#38755,#38756,#38757,#38758,#38759,#38760,#38761,
#38762,#38763,#38764,#38765,#38766,#38767,#38768,#38769,#38770,#38771,#38772,
#38773,#38774,#38775,#38776,#38777,#38778,#38779,#38780,#38781,#38782,#38783,
#38784,#38785,#38786,#38787,#38788,#38789,#38790,#38791,#38792,#38793,#38794,
#38795,#38796,#38797,#38798,#38799,#38800,#38801,#38802,#38803,#38804,#38805,
#38806,#38807,#38808,#38809,#38810,#38811,#38812,#38813,#38814),
 .UNSPECIFIED.,.F.,.F.,(4,3,3,3,3,3,3,3,3,3,3,3,3,3,3,3,3,3,3,3,3,3,3,3,
3,3,3,3,3,3,3,3,3,3,3,3,3,3,3,3,3,3,3,3,3,3,3,3,3,3,3,3,4),(386.415896391545,
386.498358597581,386.580820455321,386.663281971615,386.745743153312,386.828204007263,
386.910664540318,386.993124759324,387.075584671132,387.15804428259,387.240503600546,
387.322962631848,387.405421383345,387.487879861883,387.570338074311,387.652796027475,
387.735253728223,387.817711183401,387.900168399856,387.986180626357,388.069504970781,
388.151971576226,388.234437337468,388.31690228192,388.399366436996,388.481829830105,
388.564292488654,388.646754440046,388.729215711685,388.811676330969,388.894136325296,
388.976595722061,389.059054548656,389.141512832472,389.2239706009,389.306427881325,
389.390561116737,389.473027114828,389.555491491184,389.637954355446,389.720415817236,
389.802875986158,389.885334971793,389.96779288371,390.053388729235,390.135853465835,
390.218315237837,390.300774483679,390.383231641656,390.465694159938,390.548151830793,
390.630610620743,390.652559647909),.UNSPECIFIED.);
#351=B_SPLINE_CURVE_WITH_KNOTS('',3,(#38820,#38821,#38822,#38823,#38824,
#38825,#38826,#38827,#38828,#38829,#38830,#38831,#38832,#38833,#38834,#38835,
#38836,#38837,#38838,#38839,#38840,#38841,#38842,#38843,#38844,#38845,#38846,
#38847,#38848,#38849,#38850,#38851,#38852,#38853,#38854,#38855,#38856,#38857,
#38858,#38859,#38860,#38861,#38862,#38863,#38864,#38865,#38866,#38867,#38868,
#38869,#38870,#38871,#38872,#38873,#38874,#38875,#38876,#38877,#38878,#38879,
#38880,#38881,#38882,#38883,#38884,#38885,#38886,#38887,#38888,#38889,#38890,
#38891,#38892,#38893,#38894,#38895,#38896,#38897,#38898,#38899,#38900,#38901,
#38902,#38903,#38904,#38905,#38906,#38907,#38908,#38909,#38910,#38911,#38912,
#38913,#38914,#38915,#38916,#38917,#38918,#38919,#38920,#38921,#38922,#38923,
#38924,#38925,#38926,#38927,#38928,#38929,#38930,#38931,#38932,#38933,#38934,
#38935,#38936,#38937,#38938,#38939,#38940,#38941,#38942,#38943,#38944,#38945,
#38946,#38947,#38948,#38949,#38950,#38951,#38952,#38953,#38954,#38955,#38956,
#38957,#38958,#38959,#38960,#38961,#38962,#38963,#38964,#38965,#38966,#38967,
#38968,#38969,#38970,#38971,#38972,#38973,#38974,#38975,#38976),
 .UNSPECIFIED.,.F.,.F.,(4,3,3,3,3,3,3,3,3,3,3,3,3,3,3,3,3,3,3,3,3,3,3,3,
3,3,3,3,3,3,3,3,3,3,3,3,3,3,3,3,3,3,3,3,3,3,3,3,3,3,3,3,4),(392.699081698725,
392.781543904761,392.864005762501,392.946467278795,393.028928460492,393.111389314443,
393.193849847498,393.276310066504,393.358769978312,393.44122958977,393.523688907726,
393.606147939028,393.688606690525,393.771065169063,393.853523381491,393.935981334655,
394.018439035403,394.100896490581,394.183353707035,394.269365933537,394.35269027796,
394.435156883406,394.517622644647,394.6000875891,394.682551744176,394.765015137285,
394.847477795833,394.929939747226,395.012401018865,395.094861638149,395.177321632476,
395.25978102924,395.342239855835,395.424698139652,395.507155908079,395.589613188505,
395.673746423916,395.756212422008,395.838676798363,395.921139662626,396.003601124416,
396.086061293337,396.168520278973,396.25097819089,396.336574036415,396.419038773015,
396.501500545017,396.583959790859,396.666416948836,396.748879467117,396.831337137972,
396.913795927923,396.935744955089),.UNSPECIFIED.);
#352=B_SPLINE_CURVE_WITH_KNOTS('',3,(#38977,#38978,#38979,#38980,#38981,
#38982,#38983,#38984,#38985,#38986,#38987,#38988,#38989,#38990,#38991,#38992,
#38993,#38994,#38995,#38996,#38997,#38998,#38999,#39000,#39001,#39002,#39003,
#39004,#39005,#39006,#39007,#39008,#39009,#39010,#39011,#39012,#39013,#39014,
#39015,#39016,#39017,#39018,#39019,#39020,#39021,#39022,#39023,#39024,#39025,
#39026,#39027,#39028,#39029,#39030,#39031,#39032,#39033,#39034,#39035,#39036,
#39037,#39038,#39039,#39040,#39041,#39042,#39043,#39044,#39045,#39046,#39047,
#39048,#39049,#39050,#39051,#39052,#39053,#39054,#39055,#39056,#39057,#39058),
 .UNSPECIFIED.,.F.,.F.,(4,3,3,3,3,3,3,3,3,3,3,3,3,3,3,3,3,3,3,3,3,3,3,3,
3,3,3,4),(390.65265496374,390.729930386465,390.807215958564,390.884525701835,
390.96508487865,391.042526763526,391.120024575373,391.197626008844,391.206762409095,
391.283611032282,391.360365878679,391.437043218083,391.513659257858,391.590230156482,
391.66726588948,391.743808308186,391.820356644748,391.896925476196,391.974323112263,
392.051014193216,392.12876510684,392.206516020464,392.288683850341,392.370716624168,
392.452807892807,392.534533417735,392.61680755823,392.699081698725),
 .UNSPECIFIED.);
#353=B_SPLINE_CURVE_WITH_KNOTS('',3,(#39060,#39061,#39062,#39063,#39064,
#39065,#39066,#39067,#39068,#39069,#39070,#39071,#39072,#39073,#39074,#39075,
#39076,#39077,#39078,#39079,#39080,#39081,#39082,#39083,#39084,#39085,#39086,
#39087,#39088,#39089,#39090,#39091,#39092,#39093,#39094,#39095,#39096,#39097,
#39098,#39099,#39100,#39101,#39102,#39103,#39104,#39105,#39106,#39107,#39108,
#39109,#39110,#39111,#39112,#39113,#39114,#39115,#39116,#39117,#39118,#39119,
#39120,#39121,#39122,#39123,#39124,#39125,#39126,#39127,#39128,#39129,#39130,
#39131,#39132,#39133,#39134,#39135),.UNSPECIFIED.,.F.,.F.,(4,3,3,3,3,3,
3,3,3,3,3,3,3,3,3,3,3,3,3,3,3,3,3,3,3,4),(390.652559647909,390.735021251763,
390.817482189734,390.899942489219,390.982402177616,391.064861282318,391.147319830717,
391.229777850204,391.312235368165,391.398913263825,391.481380049661,391.563845163004,
391.64630871351,391.728770810807,391.811231564509,391.893691084206,391.976149479473,
392.058606859871,392.141073246137,392.223536448151,392.305996904431,392.388455053342,
392.470920658221,392.553380537436,392.6358446508,392.699081698724),
 .UNSPECIFIED.);
#354=B_SPLINE_CURVE_WITH_KNOTS('',3,(#39136,#39137,#39138,#39139,#39140,
#39141,#39142,#39143,#39144,#39145,#39146,#39147,#39148,#39149,#39150,#39151,
#39152,#39153,#39154,#39155,#39156,#39157,#39158,#39159,#39160,#39161,#39162,
#39163,#39164,#39165,#39166,#39167,#39168,#39169,#39170,#39171,#39172,#39173,
#39174,#39175,#39176,#39177,#39178,#39179,#39180,#39181,#39182,#39183,#39184,
#39185,#39186,#39187,#39188,#39189,#39190,#39191,#39192,#39193,#39194,#39195,
#39196,#39197,#39198,#39199,#39200,#39201,#39202,#39203,#39204,#39205,#39206,
#39207,#39208,#39209,#39210,#39211,#39212,#39213,#39214,#39215,#39216,#39217,
#39218,#39219,#39220,#39221,#39222,#39223,#39224,#39225,#39226,#39227,#39228,
#39229,#39230,#39231,#39232,#39233,#39234,#39235,#39236,#39237,#39238,#39239,
#39240,#39241,#39242,#39243,#39244,#39245,#39246,#39247,#39248,#39249,#39250,
#39251,#39252,#39253,#39254,#39255,#39256,#39257,#39258,#39259,#39260,#39261,
#39262,#39263,#39264,#39265,#39266,#39267,#39268,#39269,#39270,#39271,#39272,
#39273,#39274,#39275,#39276,#39277,#39278,#39279,#39280,#39281,#39282,#39283,
#39284,#39285,#39286,#39287,#39288,#39289,#39290,#39291,#39292,#39293,#39294,
#39295,#39296,#39297,#39298,#39299,#39300,#39301,#39302,#39303,#39304),
 .UNSPECIFIED.,.F.,.F.,(4,3,3,3,3,3,3,3,3,3,3,3,3,3,3,3,3,3,3,3,3,3,3,3,
3,3,3,3,3,3,3,3,3,3,3,3,3,3,3,3,3,3,3,3,3,3,3,3,3,3,3,3,3,3,3,3,4),(392.699081698724,
392.793961387981,392.889826204111,392.986708190667,393.00689192327,393.083755307922,
393.160525139732,393.237217675721,393.313849110887,393.390435591671,393.467293634127,
393.54385195709,393.620416291763,393.69700120489,393.774075886498,393.850782707367,
393.928041319344,394.005299931321,394.082830127781,394.160273222386,394.237644856442,
394.314960620011,394.392236062789,394.469496945209,394.546752250853,394.624016021147,
394.701302299632,394.778669112424,394.856077447131,394.933599003694,395.003707939372,
395.081238057435,395.158681086751,395.236052668577,395.313368392936,395.390643809498,
395.467904685523,395.545159996869,395.622423784961,395.699710093345,395.777076954951,
395.854485348883,395.932006981755,396.002115947423,396.078955451781,396.155705180829,
396.232381376134,396.30900022039,396.387270367678,396.463830766461,396.540385985712,
396.616950589475,396.69650329178,396.773165637115,396.849872557563,396.926668187919,
396.935161398696),.UNSPECIFIED.);
#355=B_SPLINE_CURVE_WITH_KNOTS('',3,(#39310,#39311,#39312,#39313,#39314,
#39315,#39316,#39317,#39318,#39319,#39320,#39321,#39322,#39323,#39324,#39325,
#39326,#39327,#39328,#39329,#39330,#39331,#39332,#39333,#39334,#39335,#39336,
#39337,#39338,#39339,#39340,#39341,#39342,#39343,#39344,#39345,#39346,#39347,
#39348,#39349,#39350,#39351,#39352,#39353,#39354,#39355,#39356,#39357,#39358,
#39359,#39360,#39361,#39362,#39363,#39364,#39365,#39366,#39367,#39368,#39369,
#39370,#39371,#39372,#39373,#39374,#39375,#39376,#39377,#39378,#39379,#39380,
#39381,#39382,#39383,#39384,#39385,#39386,#39387,#39388,#39389,#39390,#39391,
#39392,#39393,#39394,#39395,#39396,#39397,#39398,#39399,#39400,#39401,#39402,
#39403,#39404,#39405,#39406,#39407,#39408,#39409,#39410,#39411,#39412,#39413,
#39414,#39415,#39416,#39417,#39418,#39419,#39420,#39421,#39422,#39423,#39424,
#39425,#39426,#39427,#39428,#39429,#39430,#39431,#39432,#39433,#39434,#39435,
#39436,#39437,#39438,#39439,#39440,#39441,#39442,#39443,#39444,#39445,#39446,
#39447,#39448,#39449,#39450,#39451,#39452,#39453,#39454,#39455,#39456,#39457,
#39458,#39459,#39460,#39461,#39462,#39463,#39464,#39465,#39466),
 .UNSPECIFIED.,.F.,.F.,(4,3,3,3,3,3,3,3,3,3,3,3,3,3,3,3,3,3,3,3,3,3,3,3,
3,3,3,3,3,3,3,3,3,3,3,3,3,3,3,3,3,3,3,3,3,3,3,3,3,3,3,3,4),(398.982267005904,
399.06472921194,399.14719106968,399.229652585974,399.312113767671,399.394574621622,
399.477035154677,399.559495373683,399.641955285491,399.724414896949,399.806874214905,
399.889333246207,399.971791997704,400.054250476242,400.13670868867,400.219166641834,
400.301624342582,400.38408179776,400.466539014214,400.552551240716,400.63587558514,
400.718342190585,400.800807951827,400.883272896279,400.965737051355,401.048200444464,
401.130663103012,401.213125054405,401.295586326044,401.378046945328,401.460506939655,
401.542966336419,401.625425163015,401.707883446831,401.790341215259,401.872798495684,
401.956931731096,402.039397729187,402.121862105543,402.204324969805,402.286786431596,
402.369246600517,402.451705586152,402.53416349807,402.619759343595,402.702224080195,
402.784685852197,402.867145098039,402.949602256016,403.032064774297,403.114522445152,
403.196981235103,403.218930262269),.UNSPECIFIED.);
#356=B_SPLINE_CURVE_WITH_KNOTS('',3,(#39467,#39468,#39469,#39470,#39471,
#39472,#39473,#39474,#39475,#39476,#39477,#39478,#39479,#39480,#39481,#39482,
#39483,#39484,#39485,#39486,#39487,#39488,#39489,#39490,#39491,#39492,#39493,
#39494,#39495,#39496,#39497,#39498,#39499,#39500,#39501,#39502,#39503,#39504,
#39505,#39506,#39507,#39508,#39509,#39510,#39511,#39512,#39513,#39514,#39515,
#39516,#39517,#39518,#39519,#39520,#39521,#39522,#39523,#39524,#39525,#39526,
#39527,#39528,#39529,#39530,#39531,#39532,#39533,#39534,#39535,#39536,#39537,
#39538,#39539,#39540,#39541,#39542),.UNSPECIFIED.,.F.,.F.,(4,3,3,3,3,3,
3,3,3,3,3,3,3,3,3,3,3,3,3,3,3,3,3,3,3,4),(396.935744955089,397.018206558943,
397.100667496913,397.183127796399,397.265587484796,397.348046589498,397.430505137897,
397.512963157383,397.595420675345,397.682098570996,397.764565356832,397.847030470175,
397.929494020681,398.011956117978,398.09441687168,398.176876391377,398.259334786644,
398.341792167041,398.424258553308,398.506721755322,398.589182211602,398.671640360513,
398.754105965392,398.836565844606,398.91902995797,398.982267005763),
 .UNSPECIFIED.);
#357=B_SPLINE_CURVE_WITH_KNOTS('',3,(#39544,#39545,#39546,#39547,#39548,
#39549,#39550,#39551,#39552,#39553,#39554,#39555,#39556,#39557,#39558,#39559,
#39560,#39561,#39562,#39563,#39564,#39565,#39566,#39567,#39568,#39569,#39570,
#39571,#39572,#39573,#39574,#39575,#39576,#39577,#39578,#39579,#39580,#39581,
#39582,#39583,#39584,#39585,#39586,#39587,#39588,#39589,#39590,#39591,#39592,
#39593,#39594,#39595,#39596,#39597,#39598,#39599,#39600,#39601,#39602,#39603,
#39604,#39605,#39606,#39607,#39608,#39609,#39610,#39611,#39612,#39613,#39614,
#39615,#39616,#39617,#39618,#39619,#39620,#39621,#39622,#39623,#39624,#39625),
 .UNSPECIFIED.,.F.,.F.,(4,3,3,3,3,3,3,3,3,3,3,3,3,3,3,3,3,3,3,3,3,3,3,3,
3,3,3,4),(396.935161398696,397.000523955473,397.078118624907,397.155620891017,
397.233046376088,397.310410647465,397.387729228556,397.465024933027,397.542309977683,
397.619598369616,397.696904115142,397.774282155129,397.851697226874,397.929217841145,
397.998931963524,398.080418277957,398.161800360316,398.245884262125,398.327041580978,
398.408122364732,398.489112356766,398.49813596755,398.57854070701,398.659011250048,
398.739825189012,398.820496803775,398.901381904839,398.982267005904),
 .UNSPECIFIED.);
#358=B_SPLINE_CURVE_WITH_KNOTS('',3,(#39626,#39627,#39628,#39629,#39630,
#39631,#39632,#39633,#39634,#39635,#39636,#39637,#39638,#39639,#39640,#39641,
#39642,#39643,#39644,#39645,#39646,#39647,#39648,#39649,#39650,#39651,#39652,
#39653,#39654,#39655,#39656,#39657,#39658,#39659,#39660,#39661,#39662,#39663,
#39664,#39665,#39666,#39667,#39668,#39669,#39670,#39671,#39672,#39673,#39674,
#39675,#39676,#39677,#39678,#39679,#39680,#39681,#39682,#39683,#39684,#39685,
#39686,#39687,#39688,#39689,#39690,#39691,#39692,#39693,#39694,#39695,#39696,
#39697,#39698,#39699,#39700,#39701,#39702,#39703,#39704,#39705,#39706,#39707,
#39708,#39709,#39710,#39711,#39712,#39713,#39714,#39715,#39716,#39717,#39718,
#39719,#39720,#39721,#39722,#39723,#39724,#39725,#39726,#39727,#39728,#39729,
#39730,#39731,#39732,#39733,#39734,#39735,#39736,#39737,#39738,#39739,#39740,
#39741,#39742,#39743,#39744,#39745,#39746,#39747,#39748,#39749,#39750,#39751,
#39752,#39753,#39754,#39755,#39756,#39757,#39758,#39759,#39760,#39761,#39762,
#39763,#39764,#39765,#39766,#39767,#39768,#39769,#39770,#39771,#39772,#39773,
#39774,#39775,#39776,#39777,#39778,#39779,#39780,#39781,#39782,#39783,#39784,
#39785,#39786,#39787,#39788,#39789,#39790,#39791,#39792,#39793,#39794),
 .UNSPECIFIED.,.F.,.F.,(4,3,3,3,3,3,3,3,3,3,3,3,3,3,3,3,3,3,3,3,3,3,3,3,
3,3,3,3,3,3,3,3,3,3,3,3,3,3,3,3,3,3,3,3,3,3,3,3,3,3,3,3,3,3,3,3,4),(398.982267006007,
398.997339971575,399.074868124784,399.152314999745,399.229696178453,399.307027195914,
399.384323550744,399.46161385108,399.538903758818,399.616207280817,399.693538428944,
399.770957918765,399.848423277186,399.926008663485,399.995747979626,400.072611364278,
400.149381196088,400.226073732077,400.302705167243,400.379291648027,400.456149690483,
400.532708013447,400.609272348119,400.685857261246,400.762931942854,400.839638763723,
400.9168973757,400.994155987677,401.071686184137,401.149129278742,401.226500912798,
401.303816676367,401.381092119145,401.458353001565,401.535608307209,401.612872077503,
401.690158355987,401.767525168779,401.844933503486,401.922455060049,401.992563995728,
402.070094113791,402.147537143107,402.224908724933,402.302224449293,402.379499865854,
402.45676074188,402.534016053226,402.611279841318,402.688566149701,402.765933011308,
402.84334140524,402.920863038112,402.990972003779,403.067812533307,403.144549620671,
403.219566237065),.UNSPECIFIED.);
#359=B_SPLINE_CURVE_WITH_KNOTS('',3,(#39800,#39801,#39802,#39803,#39804,
#39805,#39806,#39807,#39808,#39809,#39810,#39811,#39812,#39813,#39814,#39815,
#39816,#39817,#39818,#39819,#39820,#39821,#39822,#39823,#39824,#39825,#39826,
#39827,#39828,#39829,#39830,#39831,#39832,#39833,#39834,#39835,#39836,#39837,
#39838,#39839,#39840,#39841,#39842,#39843,#39844,#39845,#39846,#39847,#39848,
#39849,#39850,#39851,#39852,#39853,#39854,#39855,#39856,#39857,#39858,#39859,
#39860,#39861,#39862,#39863,#39864,#39865,#39866,#39867,#39868,#39869,#39870,
#39871,#39872,#39873,#39874,#39875,#39876,#39877,#39878,#39879,#39880,#39881,
#39882,#39883,#39884,#39885,#39886,#39887,#39888,#39889,#39890,#39891,#39892,
#39893,#39894,#39895,#39896,#39897,#39898,#39899,#39900,#39901,#39902,#39903,
#39904,#39905,#39906,#39907,#39908,#39909,#39910,#39911,#39912,#39913,#39914,
#39915,#39916,#39917,#39918,#39919,#39920,#39921,#39922,#39923,#39924,#39925,
#39926,#39927,#39928,#39929,#39930,#39931,#39932,#39933,#39934,#39935,#39936,
#39937,#39938,#39939,#39940,#39941,#39942,#39943,#39944,#39945,#39946,#39947,
#39948,#39949,#39950,#39951,#39952,#39953,#39954,#39955,#39956,#39957,#39958,
#39959,#39960,#39961,#39962,#39963,#39964,#39965,#39966,#39967,#39968),
 .UNSPECIFIED.,.F.,.F.,(4,3,3,3,3,3,3,3,3,3,3,3,3,3,3,3,3,3,3,3,3,3,3,3,
3,3,3,3,3,3,3,3,3,3,3,3,3,3,3,3,3,3,3,3,3,3,3,3,3,3,3,3,3,3,3,3,4),(405.266047532152,
405.342168931996,405.418201910201,405.494163189336,405.570069420944,405.649194065781,
405.72505049336,405.800905647069,405.876774507432,405.952672063747,406.028652258912,
406.104681216099,406.180812293953,406.203066579635,406.280584131253,406.358014350673,
406.435372893568,406.512675364155,406.589937326106,406.667184551888,406.744426063095,
406.821675913328,406.898948158241,406.976301116212,407.053695508521,407.131203836189,
407.202820191005,407.280337560201,407.357767627653,407.435126048922,407.512428428137,
407.5896903289,407.666937539591,407.744179063809,407.821428955156,407.898701269299,
407.976054340525,408.053448870277,408.130957375239,408.202573802374,408.279394999529,
408.356126961743,408.432785939891,408.509388126352,408.585949668233,408.662996886422,
408.739541061066,408.816095341111,408.892674306091,408.970087583004,409.046799063311,
409.124563238527,409.202327413743,409.279899717308,409.357391118293,409.434795562625,
409.502619229227),.UNSPECIFIED.);
#360=B_SPLINE_CURVE_WITH_KNOTS('',3,(#39969,#39970,#39971,#39972,#39973,
#39974,#39975,#39976,#39977,#39978,#39979,#39980,#39981,#39982,#39983,#39984,
#39985,#39986,#39987,#39988,#39989,#39990,#39991,#39992,#39993,#39994,#39995,
#39996,#39997,#39998,#39999,#40000,#40001,#40002,#40003,#40004,#40005,#40006,
#40007,#40008,#40009,#40010,#40011,#40012,#40013,#40014,#40015,#40016,#40017,
#40018,#40019,#40020,#40021,#40022,#40023,#40024,#40025,#40026,#40027,#40028,
#40029,#40030,#40031,#40032,#40033,#40034,#40035,#40036,#40037,#40038,#40039,
#40040,#40041,#40042,#40043,#40044),.UNSPECIFIED.,.F.,.F.,(4,3,3,3,3,3,
3,3,3,3,3,3,3,3,3,3,3,3,3,3,3,3,3,3,3,4),(403.218930262269,403.301391865812,
403.383852803484,403.466313102684,403.548772790808,403.631231895249,403.7136904434,
403.796148462651,403.878605980389,403.965281519416,404.047748304511,404.130213417161,
404.21267696702,404.295139063719,404.377599816867,404.460059336059,404.542517730868,
404.624975110854,404.707441495662,404.789904696405,404.872365151602,404.954823299618,
405.037288901668,405.119748778805,405.202212886862,405.26541460481),
 .UNSPECIFIED.);
#361=B_SPLINE_CURVE_WITH_KNOTS('',3,(#40046,#40047,#40048,#40049,#40050,
#40051,#40052,#40053,#40054,#40055,#40056,#40057,#40058,#40059,#40060,#40061,
#40062,#40063,#40064,#40065,#40066,#40067,#40068,#40069,#40070,#40071,#40072,
#40073,#40074,#40075,#40076,#40077,#40078,#40079,#40080,#40081,#40082,#40083,
#40084,#40085,#40086,#40087,#40088,#40089,#40090,#40091,#40092,#40093,#40094,
#40095,#40096,#40097,#40098,#40099,#40100,#40101,#40102,#40103,#40104,#40105,
#40106,#40107,#40108,#40109,#40110,#40111,#40112,#40113,#40114,#40115,#40116,
#40117,#40118,#40119,#40120,#40121,#40122,#40123,#40124),.UNSPECIFIED.,
 .F.,.F.,(4,3,3,3,3,3,3,3,3,3,3,3,3,3,3,3,3,3,3,3,3,3,3,3,3,3,4),(403.219566237065,
403.29618493328,403.372762816884,403.449839966252,403.526400016109,403.602969984034,
403.67956443912,403.757018332297,403.833744806059,403.911562408944,403.98938001183,
404.066974681264,404.144476947374,404.221902432444,404.299266703822,404.376585284913,
404.453880989385,404.531166034041,404.608454425974,404.6857601715,404.763138211487,
404.840553283232,404.918073897503,404.987788019881,405.080944670191,405.173367791108,
405.265452312954),.UNSPECIFIED.);
#362=B_SPLINE_CURVE_WITH_KNOTS('',3,(#40125,#40126,#40127,#40128,#40129,
#40130,#40131,#40132,#40133,#40134,#40135,#40136,#40137,#40138,#40139,#40140,
#40141,#40142,#40143,#40144,#40145,#40146,#40147,#40148,#40149,#40150,#40151,
#40152,#40153,#40154,#40155,#40156,#40157,#40158,#40159,#40160,#40161,#40162,
#40163,#40164,#40165,#40166,#40167,#40168,#40169,#40170,#40171,#40172,#40173,
#40174,#40175,#40176,#40177,#40178,#40179,#40180,#40181,#40182,#40183,#40184,
#40185,#40186,#40187,#40188,#40189,#40190,#40191,#40192,#40193,#40194,#40195,
#40196,#40197,#40198,#40199,#40200,#40201,#40202,#40203,#40204,#40205,#40206,
#40207,#40208,#40209,#40210,#40211,#40212,#40213,#40214,#40215,#40216,#40217,
#40218,#40219,#40220,#40221,#40222,#40223,#40224,#40225,#40226,#40227,#40228,
#40229,#40230,#40231,#40232,#40233,#40234,#40235,#40236,#40237,#40238,#40239,
#40240,#40241,#40242,#40243,#40244,#40245,#40246,#40247,#40248,#40249,#40250,
#40251,#40252,#40253,#40254,#40255,#40256,#40257,#40258,#40259,#40260,#40261,
#40262,#40263,#40264,#40265,#40266,#40267,#40268,#40269,#40270,#40271,#40272,
#40273,#40274,#40275,#40276,#40277,#40278,#40279,#40280,#40281,#40282,#40283,
#40284,#40285,#40286,#40287,#40288,#40289,#40290,#40291,#40292,#40293),
 .UNSPECIFIED.,.F.,.F.,(4,3,3,3,3,3,3,3,3,3,3,3,3,3,3,3,3,3,3,3,3,3,3,3,
3,3,3,3,3,3,3,3,3,3,3,3,3,3,3,3,3,3,3,3,3,3,3,3,3,3,3,3,3,3,3,3,4),(405.265452313083,
405.339961026927,405.414439462604,405.486992023906,405.568005130196,405.649093824469,
405.733369375335,405.814678841724,405.896065742935,405.977572881699,405.986196027932,
406.063724181141,406.141171056103,406.21855223481,406.295883252271,406.373179607101,
406.450469907437,406.527759815175,406.605063337174,406.682394485301,406.759813975122,
406.837279333544,406.914864719842,406.984604035983,407.061467420635,407.138237252445,
407.214929788433,407.2915612236,407.368147704383,407.44500574684,407.521564069803,
407.598128404475,407.674713317602,407.75178799921,407.828494820079,407.905753432056,
407.983012044034,408.060542240494,408.137985335099,408.215356969155,408.292672732723,
408.369948175502,408.447209057922,408.524464363566,408.60172813386,408.679014412345,
408.756381225137,408.833789559843,408.911311116406,408.981420052084,409.058948032863,
409.136392455252,409.21376749302,409.291079443884,409.368354321232,409.445611213136,
409.50212192641),.UNSPECIFIED.);
#363=B_SPLINE_CURVE_WITH_KNOTS('',3,(#40299,#40300,#40301,#40302,#40303,
#40304,#40305,#40306,#40307,#40308,#40309,#40310,#40311,#40312,#40313,#40314,
#40315,#40316,#40317,#40318,#40319,#40320,#40321,#40322,#40323,#40324,#40325,
#40326,#40327,#40328,#40329,#40330,#40331,#40332,#40333,#40334,#40335,#40336,
#40337,#40338,#40339,#40340,#40341,#40342,#40343,#40344,#40345,#40346,#40347,
#40348,#40349,#40350,#40351,#40352,#40353,#40354,#40355,#40356,#40357,#40358,
#40359,#40360,#40361,#40362,#40363,#40364,#40365,#40366,#40367,#40368,#40369,
#40370,#40371,#40372,#40373,#40374,#40375,#40376,#40377,#40378,#40379,#40380,
#40381,#40382,#40383,#40384,#40385,#40386,#40387,#40388,#40389,#40390,#40391,
#40392,#40393,#40394,#40395,#40396,#40397,#40398,#40399,#40400,#40401,#40402,
#40403,#40404,#40405,#40406,#40407,#40408,#40409,#40410,#40411,#40412,#40413,
#40414,#40415,#40416,#40417,#40418,#40419,#40420,#40421,#40422,#40423,#40424,
#40425,#40426,#40427,#40428,#40429,#40430,#40431,#40432,#40433,#40434,#40435,
#40436,#40437,#40438,#40439,#40440,#40441,#40442,#40443,#40444,#40445,#40446,
#40447,#40448,#40449,#40450,#40451,#40452,#40453,#40454,#40455),
 .UNSPECIFIED.,.F.,.F.,(4,3,3,3,3,3,3,3,3,3,3,3,3,3,3,3,3,3,3,3,3,3,3,3,
3,3,3,3,3,3,3,3,3,3,3,3,3,3,3,3,3,3,3,3,3,3,3,3,3,3,3,3,4),(411.548637620263,
411.631099826299,411.713561684039,411.796023200333,411.87848438203,411.960945235981,
412.043405769036,412.125865988042,412.20832589985,412.290785511308,412.373244829264,
412.455703860566,412.538162612063,412.620621090601,412.703079303029,412.785537256194,
412.867994956942,412.950452412119,413.032909628574,413.118921855076,413.202246199499,
413.284712804945,413.367178566186,413.449643510639,413.532107665714,413.614571058823,
413.697033717372,413.779495668765,413.861956940403,413.944417559688,414.026877554014,
414.109336950779,414.191795777374,414.274254061191,414.356711829618,414.439169110044,
414.523302345455,414.605768343547,414.688232719902,414.770695584164,414.853157045955,
414.935617214876,415.018076200512,415.100534112429,415.186129957954,415.268594694554,
415.351056466556,415.433515712398,415.515972870375,415.598435388656,415.680893059511,
415.763351849462,415.785300876628),.UNSPECIFIED.);
#364=B_SPLINE_CURVE_WITH_KNOTS('',3,(#40456,#40457,#40458,#40459,#40460,
#40461,#40462,#40463,#40464,#40465,#40466,#40467,#40468,#40469,#40470,#40471,
#40472,#40473,#40474,#40475,#40476,#40477,#40478,#40479,#40480,#40481,#40482,
#40483,#40484,#40485,#40486,#40487,#40488,#40489,#40490,#40491,#40492,#40493,
#40494,#40495,#40496,#40497,#40498,#40499,#40500,#40501,#40502,#40503,#40504,
#40505,#40506,#40507,#40508,#40509,#40510,#40511,#40512,#40513,#40514,#40515,
#40516,#40517,#40518,#40519,#40520,#40521,#40522,#40523,#40524,#40525,#40526,
#40527,#40528,#40529,#40530,#40531,#40532,#40533,#40534,#40535,#40536,#40537),
 .UNSPECIFIED.,.F.,.F.,(4,3,3,3,3,3,3,3,3,3,3,3,3,3,3,3,3,3,3,3,3,3,3,3,
3,3,3,4),(409.502619229227,409.579929720954,409.657698633974,409.734970961888,
409.812244860335,409.889534347183,409.967671016666,410.045068067043,410.123574546078,
410.202081025113,410.283564998068,410.364944362208,410.449197729356,410.530351224527,
410.611427902487,410.692413330278,410.701957830797,410.782966226701,410.864050483532,
410.948496521769,411.029802603476,411.111186393244,411.192691054272,411.201834636482,
411.289530195866,411.376982381924,411.463959432209,411.548637620263),
 .UNSPECIFIED.);
#365=B_SPLINE_CURVE_WITH_KNOTS('',3,(#40539,#40540,#40541,#40542,#40543,
#40544,#40545,#40546,#40547,#40548,#40549,#40550,#40551,#40552,#40553,#40554,
#40555,#40556,#40557,#40558,#40559,#40560,#40561,#40562,#40563,#40564,#40565,
#40566,#40567,#40568,#40569,#40570,#40571,#40572,#40573,#40574,#40575,#40576,
#40577,#40578,#40579,#40580,#40581,#40582,#40583,#40584,#40585,#40586,#40587,
#40588,#40589,#40590,#40591,#40592,#40593,#40594,#40595,#40596,#40597,#40598,
#40599,#40600,#40601,#40602,#40603,#40604,#40605,#40606,#40607,#40608,#40609,
#40610,#40611,#40612,#40613,#40614,#40615,#40616,#40617,#40618,#40619,#40620),
 .UNSPECIFIED.,.F.,.F.,(4,3,3,3,3,3,3,3,3,3,3,3,3,3,3,3,3,3,3,3,3,3,3,3,
3,3,3,4),(409.50212192641,409.579382058547,409.656660938385,409.737452718823,
409.814850708878,409.89230004659,409.969847131038,409.979828060135,410.056664092258,
410.133411107985,410.210085345548,410.28670298507,410.363280161696,410.440149650008,
410.51670975253,410.593280049678,410.6698751107,410.746965350071,410.823692546653,
410.900964307419,410.978236068186,411.058503823145,411.13865788409,411.218708071292,
411.301190458535,411.381034500472,411.464836060367,411.548637620263),
 .UNSPECIFIED.);
#366=B_SPLINE_CURVE_WITH_KNOTS('',3,(#40621,#40622,#40623,#40624,#40625,
#40626,#40627,#40628,#40629,#40630,#40631,#40632,#40633,#40634,#40635,#40636,
#40637,#40638,#40639,#40640,#40641,#40642,#40643,#40644,#40645,#40646,#40647,
#40648,#40649,#40650,#40651,#40652,#40653,#40654,#40655,#40656,#40657,#40658,
#40659,#40660,#40661,#40662,#40663,#40664,#40665,#40666,#40667,#40668,#40669,
#40670,#40671,#40672,#40673,#40674,#40675,#40676,#40677,#40678,#40679,#40680,
#40681,#40682,#40683,#40684,#40685,#40686,#40687,#40688,#40689,#40690,#40691,
#40692,#40693,#40694,#40695,#40696,#40697,#40698,#40699,#40700,#40701,#40702,
#40703,#40704,#40705,#40706,#40707,#40708,#40709,#40710,#40711,#40712,#40713,
#40714,#40715,#40716,#40717,#40718,#40719,#40720,#40721,#40722,#40723,#40724,
#40725,#40726,#40727,#40728,#40729,#40730,#40731,#40732,#40733,#40734,#40735,
#40736,#40737,#40738,#40739,#40740,#40741,#40742,#40743,#40744,#40745,#40746,
#40747,#40748,#40749,#40750,#40751,#40752,#40753,#40754,#40755,#40756,#40757,
#40758,#40759,#40760,#40761,#40762,#40763,#40764,#40765,#40766,#40767,#40768,
#40769,#40770,#40771,#40772,#40773,#40774,#40775,#40776,#40777,#40778,#40779,
#40780,#40781,#40782,#40783,#40784,#40785,#40786,#40787,#40788,#40789,#40790,
#40791,#40792),.UNSPECIFIED.,.F.,.F.,(4,3,3,3,3,3,3,3,3,3,3,3,3,3,3,3,3,
3,3,3,3,3,3,3,3,3,3,3,3,3,3,3,3,3,3,3,3,3,3,3,3,3,3,3,3,3,3,3,3,3,3,3,3,
3,3,3,3,4),(411.548637620392,411.631116923562,411.717498711731,411.800360156989,
411.883345085508,411.966503474013,411.976644076237,412.05813039067,412.139512473029,
412.223596374837,412.30475369369,412.385834477445,412.466824469478,412.475848080263,
412.556861186553,412.637949880827,412.722225431692,412.803534898082,412.884921799293,
412.966428938058,412.975052084288,413.052580237497,413.130027112458,413.207408291166,
413.284739308626,413.362035663457,413.439325963793,413.516615871531,413.593919393529,
413.671250541656,413.748670031477,413.826135389899,413.903720776197,413.973460092339,
414.050323476991,414.127093308801,414.203785844789,414.280417279956,414.35700376074,
414.433861803196,414.510420126159,414.586984460832,414.663569373959,414.740644055567,
414.817350876436,414.894609488413,414.97186810039,415.04940838302,415.126859511665,
415.20423713556,415.281549096136,415.358824470978,415.436077322192,415.513321696487,
415.590593756579,415.667880944835,415.745225934373,415.784711144052),
 .UNSPECIFIED.);
#367=B_SPLINE_CURVE_WITH_KNOTS('',3,(#40798,#40799,#40800,#40801,#40802,
#40803,#40804,#40805,#40806,#40807,#40808,#40809,#40810,#40811,#40812,#40813,
#40814,#40815,#40816,#40817,#40818,#40819,#40820,#40821,#40822,#40823,#40824,
#40825,#40826,#40827,#40828,#40829,#40830,#40831,#40832,#40833,#40834,#40835,
#40836,#40837,#40838,#40839,#40840,#40841,#40842,#40843,#40844,#40845,#40846,
#40847,#40848,#40849,#40850,#40851,#40852,#40853,#40854,#40855,#40856,#40857,
#40858,#40859,#40860,#40861,#40862,#40863,#40864,#40865,#40866,#40867,#40868,
#40869,#40870,#40871,#40872,#40873,#40874,#40875,#40876,#40877,#40878,#40879,
#40880,#40881,#40882,#40883,#40884,#40885,#40886,#40887,#40888,#40889,#40890,
#40891,#40892,#40893,#40894,#40895,#40896,#40897,#40898,#40899,#40900,#40901,
#40902,#40903,#40904,#40905,#40906,#40907,#40908,#40909,#40910,#40911,#40912,
#40913,#40914,#40915,#40916,#40917,#40918,#40919,#40920,#40921,#40922,#40923,
#40924,#40925,#40926,#40927,#40928,#40929,#40930,#40931,#40932,#40933,#40934,
#40935,#40936,#40937,#40938,#40939,#40940,#40941,#40942,#40943,#40944,#40945,
#40946,#40947,#40948,#40949,#40950,#40951,#40952,#40953,#40954,#40955,#40956,
#40957,#40958,#40959,#40960,#40961,#40962,#40963,#40964,#40965,#40966),
 .UNSPECIFIED.,.F.,.F.,(4,3,3,3,3,3,3,3,3,3,3,3,3,3,3,3,3,3,3,3,3,3,3,3,
3,3,3,3,3,3,3,3,3,3,3,3,3,3,3,3,3,3,3,3,3,3,3,3,3,3,3,3,3,3,3,3,4),(417.831822927443,
417.917729261325,418.004018421998,418.090499078249,418.17721376897,418.200109916068,
418.277625694331,418.355059994742,418.432428413169,418.509746498319,418.587029762363,
418.664306846675,418.741583427162,418.81887352256,418.896191156564,418.973597362888,
419.051049372202,419.128622180524,419.199863527437,419.276712150624,419.353466997021,
419.430144336426,419.506760376201,419.583331274826,419.660367007823,419.736909426529,
419.813457763091,419.890026594539,419.967424230606,420.044115311559,420.121866225182,
420.199617138806,420.277134690424,420.354564909844,420.431923452739,420.509225923326,
420.586487885276,420.663735111059,420.740976622266,420.818226472499,420.895498717412,
420.972851675383,421.050246067692,421.12775439536,421.199370750176,421.276895112083,
421.354330721744,421.431693240297,421.511244244508,421.58850615986,421.665746689699,
421.742979892556,421.824260237913,421.901548057031,421.978864899425,422.05624938853,
422.068101273987),.UNSPECIFIED.);
#368=B_SPLINE_CURVE_WITH_KNOTS('',3,(#40967,#40968,#40969,#40970,#40971,
#40972,#40973,#40974,#40975,#40976,#40977,#40978,#40979,#40980,#40981,#40982,
#40983,#40984,#40985,#40986,#40987,#40988,#40989,#40990,#40991,#40992,#40993,
#40994,#40995,#40996,#40997,#40998,#40999,#41000,#41001,#41002,#41003,#41004,
#41005,#41006,#41007,#41008,#41009,#41010,#41011,#41012,#41013,#41014,#41015,
#41016,#41017,#41018,#41019,#41020,#41021,#41022,#41023,#41024,#41025,#41026,
#41027,#41028,#41029,#41030,#41031,#41032,#41033,#41034,#41035,#41036,#41037,
#41038,#41039,#41040,#41041,#41042),.UNSPECIFIED.,.F.,.F.,(4,3,3,3,3,3,
3,3,3,3,3,3,3,3,3,3,3,3,3,3,3,3,3,3,3,4),(415.785300876628,415.867762480482,
415.950223418452,416.032683717938,416.115143406335,416.197602511037,416.280061059436,
416.362519078922,416.444976596884,416.531654492544,416.614121278379,416.696586391723,
416.779049942228,416.861512039526,416.943972793228,417.026432312925,417.108890708192,
417.191348088589,417.273814474856,417.35627767687,417.43873813315,417.521196282061,
417.60366188694,417.686121766155,417.768585879518,417.831822927443),
 .UNSPECIFIED.);
#369=B_SPLINE_CURVE_WITH_KNOTS('',3,(#41044,#41045,#41046,#41047,#41048,
#41049,#41050,#41051,#41052,#41053,#41054,#41055,#41056,#41057,#41058,#41059,
#41060,#41061,#41062,#41063,#41064,#41065,#41066,#41067,#41068,#41069,#41070,
#41071,#41072,#41073,#41074,#41075,#41076,#41077,#41078,#41079,#41080,#41081,
#41082,#41083,#41084,#41085,#41086,#41087,#41088,#41089,#41090,#41091,#41092,
#41093,#41094,#41095,#41096,#41097,#41098,#41099,#41100,#41101,#41102,#41103,
#41104,#41105,#41106,#41107,#41108,#41109,#41110,#41111,#41112,#41113,#41114,
#41115,#41116,#41117,#41118,#41119,#41120,#41121,#41122,#41123,#41124,#41125,
#41126,#41127,#41128),.UNSPECIFIED.,.F.,.F.,(4,3,3,3,3,3,3,3,3,3,3,3,3,
3,3,3,3,3,3,3,3,3,3,3,3,3,3,3,4),(415.784711144052,415.862145526228,415.939682750499,
415.970276108441,416.047806226504,416.12524925582,416.202620837646,416.279936562006,
416.357211978567,416.434472854593,416.511728165939,416.588991954031,416.666278262415,
416.743645124021,416.821053517953,416.898575150825,416.968684116492,417.044412302149,
417.120052278303,417.19562098838,417.275021363452,417.350500604425,417.425964305112,
417.501427624748,417.576905721553,417.652447414651,417.728026121681,417.803692848326,
417.830823988957),.UNSPECIFIED.);
#370=B_SPLINE_CURVE_WITH_KNOTS('',3,(#41129,#41130,#41131,#41132,#41133,
#41134,#41135,#41136,#41137,#41138,#41139,#41140,#41141,#41142,#41143,#41144,
#41145,#41146,#41147,#41148,#41149,#41150,#41151,#41152,#41153,#41154,#41155,
#41156,#41157,#41158,#41159,#41160,#41161,#41162,#41163,#41164,#41165,#41166,
#41167,#41168,#41169,#41170,#41171,#41172,#41173,#41174,#41175,#41176,#41177,
#41178,#41179,#41180,#41181,#41182,#41183,#41184,#41185,#41186,#41187,#41188,
#41189,#41190,#41191,#41192,#41193,#41194,#41195,#41196,#41197,#41198,#41199,
#41200,#41201,#41202,#41203,#41204,#41205,#41206,#41207,#41208,#41209,#41210,
#41211,#41212,#41213,#41214,#41215,#41216,#41217,#41218,#41219,#41220,#41221,
#41222,#41223,#41224,#41225,#41226,#41227,#41228,#41229,#41230,#41231,#41232,
#41233,#41234,#41235,#41236,#41237,#41238,#41239,#41240,#41241,#41242,#41243,
#41244,#41245,#41246,#41247,#41248,#41249,#41250,#41251,#41252,#41253,#41254,
#41255,#41256,#41257,#41258,#41259,#41260,#41261,#41262,#41263,#41264,#41265,
#41266,#41267,#41268,#41269,#41270,#41271,#41272,#41273,#41274,#41275,#41276,
#41277,#41278,#41279,#41280,#41281,#41282,#41283,#41284,#41285),
 .UNSPECIFIED.,.F.,.F.,(4,3,3,3,3,3,3,3,3,3,3,3,3,3,3,3,3,3,3,3,3,3,3,3,
3,3,3,3,3,3,3,3,3,3,3,3,3,3,3,3,3,3,3,3,3,3,3,3,3,3,3,3,4),(417.831822927443,
417.914285133479,417.996746991219,418.079208507513,418.16166968921,418.244130543161,
418.326591076216,418.409051295222,418.49151120703,418.573970818488,418.656430136444,
418.738889167746,418.821347919243,418.903806397781,418.986264610209,419.068722563373,
419.151180264121,419.233637719299,419.316094935754,419.402107162255,419.485431506679,
419.567898112124,419.650363873366,419.732828817818,419.815292972894,419.897756366003,
419.980219024552,420.062680975944,420.145142247583,420.227602866867,420.310062861194,
420.392522257958,420.474981084554,420.55743936837,420.639897136798,420.722354417223,
420.806487652635,420.888953650726,420.971418027082,421.053880891344,421.136342353135,
421.218802522056,421.301261507691,421.383719419608,421.469315265133,421.551780001734,
421.634241773735,421.716701019578,421.799158177554,421.881620695836,421.964078366691,
422.046537156641,422.068486183807),.UNSPECIFIED.);
#371=B_SPLINE_CURVE_WITH_KNOTS('',3,(#41291,#41292,#41293,#41294,#41295,
#41296,#41297,#41298,#41299,#41300,#41301,#41302,#41303,#41304,#41305,#41306,
#41307,#41308,#41309,#41310,#41311,#41312,#41313,#41314,#41315,#41316,#41317,
#41318,#41319,#41320,#41321,#41322,#41323,#41324,#41325,#41326,#41327,#41328,
#41329,#41330,#41331,#41332,#41333,#41334,#41335,#41336,#41337,#41338,#41339,
#41340,#41341,#41342,#41343,#41344,#41345,#41346,#41347,#41348,#41349,#41350,
#41351,#41352,#41353,#41354,#41355,#41356,#41357,#41358,#41359,#41360,#41361,
#41362,#41363,#41364,#41365,#41366,#41367,#41368,#41369,#41370,#41371,#41372,
#41373,#41374,#41375,#41376,#41377,#41378,#41379,#41380,#41381,#41382,#41383,
#41384,#41385,#41386,#41387,#41388,#41389,#41390,#41391,#41392,#41393,#41394,
#41395,#41396,#41397,#41398,#41399,#41400,#41401,#41402,#41403,#41404,#41405,
#41406,#41407,#41408,#41409,#41410,#41411,#41412,#41413,#41414,#41415,#41416,
#41417,#41418,#41419,#41420,#41421,#41422,#41423,#41424,#41425,#41426,#41427,
#41428,#41429,#41430,#41431,#41432,#41433,#41434,#41435,#41436,#41437,#41438,
#41439,#41440,#41441,#41442,#41443,#41444,#41445,#41446,#41447),
 .UNSPECIFIED.,.F.,.F.,(4,3,3,3,3,3,3,3,3,3,3,3,3,3,3,3,3,3,3,3,3,3,3,3,
3,3,3,3,3,3,3,3,3,3,3,3,3,3,3,3,3,3,3,3,3,3,3,3,3,3,3,3,4),(424.115008234622,
424.197470440658,424.279932298398,424.362393814692,424.444854996389,424.52731585034,
424.609776383395,424.692236602401,424.774696514209,424.857156125667,424.939615443623,
425.022074474925,425.104533226422,425.18699170496,425.269449917388,425.351907870552,
425.4343655713,425.516823026478,425.599280242933,425.685292469434,425.768616813858,
425.851083419303,425.933549180545,426.016014124997,426.098478280073,426.180941673182,
426.263404331731,426.345866283123,426.428327554762,426.510788174046,426.593248168373,
426.675707565138,426.758166391733,426.840624675549,426.923082443977,427.005539724402,
427.089672959814,427.172138957905,427.254603334261,427.337066198523,427.419527660314,
427.501987829235,427.584446814871,427.666904726788,427.752500572313,427.834965308913,
427.917427080915,427.999886326757,428.082343484734,428.164806003015,428.24726367387,
428.329722463821,428.351671490987),.UNSPECIFIED.);
#372=B_SPLINE_CURVE_WITH_KNOTS('',3,(#41448,#41449,#41450,#41451,#41452,
#41453,#41454,#41455,#41456,#41457,#41458,#41459,#41460,#41461,#41462,#41463,
#41464,#41465,#41466,#41467,#41468,#41469,#41470,#41471,#41472,#41473,#41474,
#41475,#41476,#41477,#41478,#41479,#41480,#41481,#41482,#41483,#41484,#41485,
#41486,#41487,#41488,#41489,#41490,#41491,#41492,#41493,#41494,#41495,#41496,
#41497,#41498,#41499,#41500,#41501,#41502,#41503,#41504,#41505,#41506,#41507,
#41508,#41509,#41510,#41511,#41512,#41513,#41514,#41515,#41516,#41517,#41518,
#41519,#41520,#41521,#41522,#41523,#41524,#41525,#41526,#41527,#41528,#41529),
 .UNSPECIFIED.,.F.,.F.,(4,3,3,3,3,3,3,3,3,3,3,3,3,3,3,3,3,3,3,3,3,3,3,3,
3,3,3,4),(422.068101273987,422.145616415958,422.199124361545,422.2759455587,
422.352677520914,422.429336499062,422.505938685523,422.582500227404,422.659547445593,
422.736091620237,422.812645900282,422.889224865262,422.966638142175,423.043349622482,
423.121113797699,423.198877972915,423.275729950139,423.352489963892,423.429174304041,
423.505799199108,423.582382255955,423.658943276863,423.735496866981,423.812057624682,
423.888677214912,423.965326054594,424.042071142312,424.114488541238),
 .UNSPECIFIED.);
#373=B_SPLINE_CURVE_WITH_KNOTS('',3,(#41531,#41532,#41533,#41534,#41535,
#41536,#41537,#41538,#41539,#41540,#41541,#41542,#41543,#41544,#41545,#41546,
#41547,#41548,#41549,#41550,#41551,#41552,#41553,#41554,#41555,#41556,#41557,
#41558,#41559,#41560,#41561,#41562,#41563,#41564,#41565,#41566,#41567,#41568,
#41569,#41570,#41571,#41572,#41573,#41574,#41575,#41576,#41577,#41578,#41579,
#41580,#41581,#41582,#41583,#41584,#41585,#41586,#41587,#41588,#41589,#41590,
#41591,#41592,#41593,#41594,#41595,#41596,#41597,#41598,#41599,#41600,#41601,
#41602,#41603,#41604,#41605,#41606),.UNSPECIFIED.,.F.,.F.,(4,3,3,3,3,3,
3,3,3,3,3,3,3,3,3,3,3,3,3,3,3,3,3,3,3,4),(422.068486183807,422.150947787661,
422.233408725631,422.315869025117,422.398328713514,422.480787818216,422.563246366615,
422.645704386102,422.728161904063,422.814839799723,422.897306585559,422.979771698902,
423.062235249407,423.144697346705,423.227158100407,423.309617620104,423.392076015371,
423.474533395768,423.556999782035,423.639462984048,423.721923440329,423.80438158924,
423.886847194119,423.969307073333,424.051771186697,424.115008234622),
 .UNSPECIFIED.);
#374=B_SPLINE_CURVE_WITH_KNOTS('',3,(#41607,#41608,#41609,#41610,#41611,
#41612,#41613,#41614,#41615,#41616,#41617,#41618,#41619,#41620,#41621,#41622,
#41623,#41624,#41625,#41626,#41627,#41628,#41629,#41630,#41631,#41632,#41633,
#41634,#41635,#41636,#41637,#41638,#41639,#41640,#41641,#41642,#41643,#41644,
#41645,#41646,#41647,#41648,#41649,#41650,#41651,#41652,#41653,#41654,#41655,
#41656,#41657,#41658,#41659,#41660,#41661,#41662,#41663,#41664,#41665,#41666,
#41667,#41668,#41669,#41670,#41671,#41672,#41673,#41674,#41675,#41676,#41677,
#41678,#41679,#41680,#41681,#41682,#41683,#41684,#41685,#41686,#41687,#41688,
#41689,#41690,#41691,#41692,#41693,#41694,#41695,#41696,#41697,#41698,#41699,
#41700,#41701,#41702,#41703,#41704,#41705,#41706,#41707,#41708,#41709,#41710,
#41711,#41712,#41713,#41714,#41715,#41716,#41717,#41718,#41719,#41720,#41721,
#41722,#41723,#41724,#41725,#41726,#41727,#41728,#41729,#41730,#41731,#41732,
#41733,#41734,#41735,#41736,#41737,#41738,#41739,#41740,#41741,#41742,#41743,
#41744,#41745,#41746,#41747,#41748,#41749,#41750,#41751,#41752,#41753,#41754,
#41755,#41756,#41757,#41758,#41759,#41760,#41761,#41762,#41763,#41764,#41765,
#41766,#41767,#41768,#41769,#41770,#41771,#41772,#41773,#41774,#41775,#41776,
#41777,#41778),.UNSPECIFIED.,.F.,.F.,(4,3,3,3,3,3,3,3,3,3,3,3,3,3,3,3,3,
3,3,3,3,3,3,3,3,3,3,3,3,3,3,3,3,3,3,3,3,3,3,3,3,3,3,3,3,3,3,3,3,3,3,3,3,
3,3,3,3,4),(424.115885367393,424.191504095843,424.267055281936,424.342555776663,
424.419229827192,424.494691854454,424.570156747353,424.64563967224,424.723216799404,
424.798820852266,424.877384516583,424.955948180899,425.033542850333,425.111045116443,
425.188470601514,425.265834872891,425.343153453981,425.420449158453,425.497734203109,
425.575022595042,425.652328340568,425.729706380555,425.8071214523,425.884642066571,
425.95435618895,426.035842503383,426.117224585742,426.20130848755,426.282465806403,
426.363546590159,426.444536582192,426.453560192975,426.534573299266,426.615661993539,
426.699937544405,426.781247010794,426.862633912005,426.94414105077,426.952764197001,
427.03029235021,427.107739225172,427.185120403879,427.26245142134,427.339747776171,
427.417038076507,427.494327984246,427.571631506244,427.648962654371,427.726382144192,
427.803847502614,427.881432888912,427.951172205052,428.028047342388,428.104830802628,
428.181519055578,428.258152428406,428.334738399456,428.352171190823),
 .UNSPECIFIED.);
#375=B_SPLINE_CURVE_WITH_KNOTS('',3,(#41784,#41785,#41786,#41787,#41788,
#41789,#41790,#41791,#41792,#41793,#41794,#41795,#41796,#41797,#41798,#41799,
#41800,#41801,#41802,#41803,#41804,#41805,#41806,#41807,#41808,#41809,#41810,
#41811,#41812,#41813,#41814,#41815,#41816,#41817,#41818,#41819,#41820,#41821,
#41822,#41823,#41824,#41825,#41826,#41827,#41828,#41829,#41830,#41831,#41832,
#41833,#41834,#41835,#41836,#41837,#41838,#41839,#41840,#41841,#41842,#41843,
#41844,#41845,#41846,#41847,#41848,#41849,#41850,#41851,#41852,#41853,#41854,
#41855,#41856,#41857,#41858,#41859,#41860,#41861,#41862,#41863,#41864,#41865,
#41866,#41867,#41868,#41869,#41870,#41871,#41872,#41873,#41874,#41875,#41876,
#41877,#41878,#41879,#41880,#41881,#41882,#41883,#41884,#41885,#41886,#41887,
#41888,#41889,#41890,#41891,#41892,#41893,#41894,#41895,#41896,#41897,#41898,
#41899,#41900,#41901,#41902,#41903,#41904,#41905,#41906,#41907,#41908,#41909,
#41910,#41911,#41912,#41913,#41914,#41915,#41916,#41917,#41918,#41919,#41920,
#41921,#41922,#41923,#41924,#41925,#41926,#41927,#41928,#41929,#41930,#41931,
#41932,#41933,#41934,#41935,#41936,#41937,#41938,#41939,#41940,#41941,#41942,
#41943,#41944,#41945,#41946,#41947,#41948,#41949,#41950,#41951,#41952,#41953,
#41954,#41955),.UNSPECIFIED.,.F.,.F.,(4,3,3,3,3,3,3,3,3,3,3,3,3,3,3,3,3,
3,3,3,3,3,3,3,3,3,3,3,3,3,3,3,3,3,3,3,3,3,3,3,3,3,3,3,3,3,3,3,3,3,3,3,3,
3,3,3,3,4),(430.399063857647,430.47506981317,430.551009478196,430.626899514323,
430.702762601598,430.778613508728,430.854467241634,430.930338807012,431.006280296983,
431.082261107464,431.158338427554,431.19690686387,431.278390836825,431.359770200965,
431.444023568112,431.525177063284,431.606253741244,431.687239169034,431.696783669554,
431.777792065458,431.858876322289,431.943322360527,432.024628442234,432.106012232002,
432.18751689303,432.196660475239,432.274176253502,432.351610553913,432.42897897234,
432.50629705749,432.583580321534,432.660857405846,432.738133986334,432.815424081731,
432.892741715736,432.97014792206,433.047599931373,433.125172739696,433.196414086608,
433.273262709795,433.350017556192,433.426694895597,433.503310935372,433.579881833997,
433.656917566995,433.7334599857,433.810008322263,433.886577153711,433.963974789777,
434.04066587073,434.118416784354,434.196167697978,434.273691750868,434.351130704965,
434.428482608017,434.5057841065,434.583046149192,434.634961198303),
 .UNSPECIFIED.);
#376=B_SPLINE_CURVE_WITH_KNOTS('',3,(#41956,#41957,#41958,#41959,#41960,
#41961,#41962,#41963,#41964,#41965,#41966,#41967,#41968,#41969,#41970,#41971,
#41972,#41973,#41974,#41975,#41976,#41977,#41978,#41979,#41980,#41981,#41982,
#41983,#41984,#41985,#41986,#41987,#41988,#41989,#41990,#41991,#41992,#41993,
#41994,#41995,#41996,#41997,#41998,#41999,#42000,#42001,#42002,#42003,#42004,
#42005,#42006,#42007,#42008,#42009,#42010,#42011,#42012,#42013,#42014,#42015,
#42016,#42017,#42018,#42019,#42020,#42021,#42022,#42023,#42024,#42025,#42026,
#42027,#42028,#42029,#42030,#42031),.UNSPECIFIED.,.F.,.F.,(4,3,3,3,3,3,
3,3,3,3,3,3,3,3,3,3,3,3,3,3,3,3,3,3,3,4),(428.351671490987,428.434133094841,
428.516594032811,428.599054332297,428.681514020694,428.763973125396,428.846431673795,
428.928889693281,429.011347211243,429.098025106903,429.180491892739,429.262957006082,
429.345420556587,429.427882653885,429.510343407587,429.592802927284,429.675261322551,
429.757718702948,429.840185089215,429.922648291229,430.005108747509,430.08756689642,
430.170032501299,430.252492380514,430.334956493877,430.398193541802),
 .UNSPECIFIED.);
#377=B_SPLINE_CURVE_WITH_KNOTS('',3,(#42033,#42034,#42035,#42036,#42037,
#42038,#42039,#42040,#42041,#42042,#42043,#42044,#42045,#42046,#42047,#42048,
#42049,#42050,#42051,#42052,#42053,#42054,#42055,#42056,#42057,#42058,#42059,
#42060,#42061,#42062,#42063,#42064,#42065,#42066,#42067,#42068,#42069,#42070,
#42071,#42072,#42073,#42074,#42075,#42076,#42077,#42078,#42079,#42080,#42081,
#42082,#42083,#42084,#42085,#42086,#42087,#42088,#42089,#42090,#42091,#42092,
#42093,#42094,#42095,#42096,#42097,#42098,#42099,#42100,#42101,#42102,#42103,
#42104,#42105,#42106,#42107,#42108,#42109,#42110,#42111,#42112,#42113,#42114),
 .UNSPECIFIED.,.F.,.F.,(4,3,3,3,3,3,3,3,3,3,3,3,3,3,3,3,3,3,3,3,3,3,3,3,
3,3,3,4),(428.352171190823,428.428734883338,428.505293287412,428.581860967938,
428.658452493169,428.735126353376,428.811843832614,428.888674740058,428.949580213103,
429.027110409563,429.104553504168,429.181925138224,429.259240901792,429.336516344571,
429.41377722699,429.491032532635,429.568296302929,429.645582581413,429.722949394205,
429.800357728912,429.877879285475,429.947988221154,430.031143785834,430.114144129527,
430.196918607618,430.27955349429,430.361988636971,430.398193541718),
 .UNSPECIFIED.);
#378=B_SPLINE_CURVE_WITH_KNOTS('',3,(#42115,#42116,#42117,#42118,#42119,
#42120,#42121,#42122,#42123,#42124,#42125,#42126,#42127,#42128,#42129,#42130,
#42131,#42132,#42133,#42134,#42135,#42136,#42137,#42138,#42139,#42140,#42141,
#42142,#42143,#42144,#42145,#42146,#42147,#42148,#42149,#42150,#42151,#42152,
#42153,#42154,#42155,#42156,#42157,#42158,#42159,#42160,#42161,#42162,#42163,
#42164,#42165,#42166,#42167,#42168,#42169,#42170,#42171,#42172,#42173,#42174,
#42175,#42176,#42177,#42178,#42179,#42180,#42181,#42182,#42183,#42184,#42185,
#42186,#42187,#42188,#42189,#42190,#42191,#42192,#42193,#42194,#42195,#42196,
#42197,#42198,#42199,#42200,#42201,#42202,#42203,#42204,#42205,#42206,#42207,
#42208,#42209,#42210,#42211,#42212,#42213,#42214,#42215,#42216,#42217,#42218,
#42219,#42220,#42221,#42222,#42223,#42224,#42225,#42226,#42227,#42228,#42229,
#42230,#42231,#42232,#42233,#42234,#42235,#42236,#42237,#42238,#42239,#42240,
#42241,#42242,#42243,#42244,#42245,#42246,#42247,#42248,#42249,#42250,#42251,
#42252,#42253,#42254,#42255,#42256,#42257,#42258,#42259,#42260,#42261,#42262,
#42263,#42264,#42265,#42266,#42267,#42268,#42269,#42270,#42271,#42272,#42273,
#42274,#42275,#42276,#42277,#42278,#42279,#42280,#42281,#42282,#42283),
 .UNSPECIFIED.,.F.,.F.,(4,3,3,3,3,3,3,3,3,3,3,3,3,3,3,3,3,3,3,3,3,3,3,3,
3,3,3,3,3,3,3,3,3,3,3,3,3,3,3,3,3,3,3,3,3,3,3,3,3,3,3,3,3,3,3,3,4),(430.398193541802,
430.477934676748,430.557733637174,430.637599956251,430.717603913083,430.797679697289,
430.877905131397,430.946396229205,431.023232261328,431.099979277055,431.176653514618,
431.253271154139,431.329848330766,431.406717819077,431.4832779216,431.559848218747,
431.636443279769,431.713533519141,431.790260715722,431.867532476489,431.944804237256,
432.02239890669,432.0999011728,432.177326657871,432.254690929248,432.332009510339,
432.40930521481,432.486590259466,432.563878651399,432.641184396925,432.718562436912,
432.795977508657,432.873498122928,432.943212245306,433.024698559739,433.106080642097,
433.190164543906,433.271321862759,433.352402646513,433.433392638546,433.442416249332,
433.523429355622,433.604518049896,433.688793600761,433.770103067151,433.851489968362,
433.932997107127,433.941620253357,434.019164244903,434.096602312649,434.17397907238,
434.251308597381,434.328604931425,434.405895237983,434.483179196186,434.560499114131,
434.634363295085),.UNSPECIFIED.);
#379=B_SPLINE_CURVE_WITH_KNOTS('',3,(#42289,#42290,#42291,#42292,#42293,
#42294,#42295,#42296,#42297,#42298,#42299,#42300,#42301,#42302,#42303,#42304,
#42305,#42306,#42307,#42308,#42309,#42310,#42311,#42312,#42313,#42314,#42315,
#42316,#42317,#42318,#42319,#42320,#42321,#42322,#42323,#42324,#42325,#42326,
#42327,#42328,#42329,#42330,#42331,#42332,#42333,#42334,#42335,#42336,#42337,
#42338,#42339,#42340,#42341,#42342,#42343,#42344,#42345,#42346,#42347,#42348,
#42349,#42350,#42351,#42352,#42353,#42354,#42355,#42356,#42357,#42358,#42359,
#42360,#42361,#42362,#42363,#42364,#42365,#42366,#42367,#42368,#42369,#42370,
#42371,#42372,#42373,#42374,#42375,#42376,#42377,#42378,#42379,#42380,#42381,
#42382,#42383,#42384,#42385,#42386,#42387,#42388,#42389,#42390,#42391,#42392,
#42393,#42394,#42395,#42396,#42397,#42398,#42399,#42400,#42401,#42402,#42403,
#42404,#42405,#42406,#42407,#42408,#42409,#42410,#42411,#42412,#42413,#42414,
#42415,#42416,#42417,#42418,#42419,#42420,#42421,#42422,#42423,#42424,#42425,
#42426,#42427,#42428,#42429,#42430,#42431,#42432,#42433,#42434,#42435,#42436,
#42437,#42438,#42439,#42440,#42441,#42442,#42443,#42444,#42445),
 .UNSPECIFIED.,.F.,.F.,(4,3,3,3,3,3,3,3,3,3,3,3,3,3,3,3,3,3,3,3,3,3,3,3,
3,3,3,3,3,3,3,3,3,3,3,3,3,3,3,3,3,3,3,3,3,3,3,3,3,3,3,3,4),(436.681385966666,
436.763848172672,436.846310030382,436.928771546646,437.011232728315,437.093693582238,
437.176154115265,437.258614334245,437.341074246026,437.423533857458,437.50599317539,
437.588452206667,437.67091095814,437.753369436655,437.835827649061,437.918285602203,
438.000743302929,438.083200758086,438.16565797452,438.251669978609,438.334994107569,
438.417460712945,438.499926474119,438.582391418507,438.66485557352,438.747318966568,
438.829781625058,438.912243576395,438.99470484798,439.077165467212,439.159625461489,
439.242084858207,439.324543684757,439.407001968531,439.489459736917,439.571917017304,
439.656049835307,439.738515833271,439.820980209508,439.903443073659,439.985904535348,
440.068364704175,440.150823689725,440.233281601565,440.318876664537,440.401341400926,
440.483803172746,440.566262418435,440.648719576287,440.731182094189,440.81363976478,
440.896098554141,440.918042105346),.UNSPECIFIED.);
#380=B_SPLINE_CURVE_WITH_KNOTS('',3,(#42446,#42447,#42448,#42449,#42450,
#42451,#42452,#42453,#42454,#42455,#42456,#42457,#42458,#42459,#42460,#42461,
#42462,#42463,#42464,#42465,#42466,#42467,#42468,#42469,#42470,#42471,#42472,
#42473,#42474,#42475,#42476,#42477,#42478,#42479,#42480,#42481,#42482,#42483,
#42484,#42485,#42486,#42487,#42488,#42489,#42490,#42491,#42492,#42493,#42494,
#42495,#42496,#42497,#42498,#42499,#42500,#42501,#42502,#42503,#42504,#42505,
#42506,#42507,#42508,#42509,#42510,#42511,#42512,#42513,#42514,#42515,#42516,
#42517,#42518,#42519,#42520,#42521,#42522,#42523,#42524,#42525,#42526,#42527),
 .UNSPECIFIED.,.F.,.F.,(4,3,3,3,3,3,3,3,3,3,3,3,3,3,3,3,3,3,3,3,3,3,3,3,
3,3,3,4),(434.634961198303,434.71220303447,434.789448602289,434.866711955887,
434.944007156678,435.021386553096,435.098815887312,435.176345568828,435.195921309347,
435.273438678543,435.350868745995,435.428227167264,435.505529546479,435.582791447241,
435.660038657932,435.737280182151,435.814530073497,435.89180238764,435.969155458866,
436.046549988618,436.12405849358,436.195674920716,436.276868002695,436.357923541258,
436.438790770997,436.519548903297,436.600434123478,436.681319343659),
 .UNSPECIFIED.);
#381=B_SPLINE_CURVE_WITH_KNOTS('',3,(#42529,#42530,#42531,#42532,#42533,
#42534,#42535,#42536,#42537,#42538,#42539,#42540,#42541,#42542,#42543,#42544,
#42545,#42546,#42547,#42548,#42549,#42550,#42551,#42552,#42553,#42554,#42555,
#42556,#42557,#42558,#42559,#42560,#42561,#42562,#42563,#42564,#42565,#42566,
#42567,#42568,#42569,#42570,#42571,#42572,#42573,#42574,#42575,#42576,#42577,
#42578,#42579,#42580,#42581,#42582,#42583,#42584,#42585,#42586,#42587,#42588,
#42589,#42590,#42591,#42592,#42593,#42594,#42595,#42596,#42597,#42598,#42599,
#42600,#42601,#42602,#42603,#42604,#42605,#42606,#42607,#42608,#42609,#42610),
 .UNSPECIFIED.,.F.,.F.,(4,3,3,3,3,3,3,3,3,3,3,3,3,3,3,3,3,3,3,3,3,3,3,3,
3,3,3,4),(434.634363295085,434.711781031404,434.789244072866,434.866828149655,
434.940028261408,435.01689164606,435.09366147787,435.170354013859,435.246985449026,
435.32357192981,435.400429972266,435.476988295229,435.553552629902,435.630137543029,
435.707212224636,435.783919045505,435.861177657482,435.938436269459,436.015252140749,
436.091978335191,436.168616513899,436.245204529027,436.321757030141,436.398288642394,
436.474832648956,436.551381985816,436.627980740001,436.681378848981),
 .UNSPECIFIED.);
#382=B_SPLINE_CURVE_WITH_KNOTS('',3,(#42611,#42612,#42613,#42614,#42615,
#42616,#42617,#42618,#42619,#42620,#42621,#42622,#42623,#42624,#42625,#42626,
#42627,#42628,#42629,#42630,#42631,#42632,#42633,#42634,#42635,#42636,#42637,
#42638,#42639,#42640,#42641,#42642,#42643,#42644,#42645,#42646,#42647,#42648,
#42649,#42650,#42651,#42652,#42653,#42654,#42655,#42656,#42657,#42658,#42659,
#42660,#42661,#42662,#42663,#42664,#42665,#42666,#42667,#42668,#42669,#42670,
#42671,#42672,#42673,#42674,#42675,#42676,#42677,#42678,#42679,#42680,#42681,
#42682,#42683,#42684,#42685,#42686,#42687,#42688,#42689,#42690,#42691,#42692,
#42693,#42694,#42695,#42696,#42697,#42698,#42699,#42700,#42701,#42702,#42703,
#42704,#42705,#42706,#42707,#42708,#42709,#42710,#42711,#42712,#42713,#42714,
#42715,#42716,#42717,#42718,#42719,#42720,#42721,#42722,#42723,#42724,#42725,
#42726,#42727,#42728,#42729,#42730,#42731,#42732,#42733,#42734,#42735,#42736,
#42737,#42738,#42739,#42740,#42741,#42742,#42743,#42744,#42745,#42746,#42747,
#42748,#42749,#42750,#42751,#42752,#42753,#42754,#42755,#42756,#42757,#42758,
#42759,#42760,#42761,#42762,#42763,#42764,#42765,#42766,#42767,#42768,#42769,
#42770,#42771,#42772,#42773,#42774,#42775,#42776),.UNSPECIFIED.,.F.,.F.,
(4,3,3,3,3,3,3,3,3,3,3,3,3,3,3,3,3,3,3,3,3,3,3,3,3,3,3,3,3,3,3,3,3,3,3,
3,3,3,3,3,3,3,3,3,3,3,3,3,3,3,3,3,3,3,3,4),(436.681378849124,436.778854694112,
436.87810332322,436.93684427751,437.014374395573,437.091817424889,437.169189006715,
437.246504731075,437.323780147636,437.401041023662,437.478296335008,437.5555601231,
437.632846431484,437.71021329309,437.787621687022,437.865143319894,437.935252285561,
438.012088317684,438.088835333411,438.165509570974,438.242127210496,438.318704387123,
438.395573875434,438.472133977957,438.548704275104,438.625299336126,438.702389575498,
438.779116772079,438.856388532846,438.933660293612,439.011254963046,439.088757229156,
439.166182714227,439.243546985604,439.320865566695,439.398161271166,439.475446315822,
439.552734707755,439.630040453281,439.707418493268,439.784833565012,439.862354179284,
439.932068301663,440.013554616096,440.094936698455,440.179020600263,440.260177919116,
440.341258702871,440.422248694905,440.431272305688,440.512283283703,440.593369813142,
440.674600105717,440.755901737176,440.837349893263,440.918106228972),
 .UNSPECIFIED.);
#383=B_SPLINE_CURVE_WITH_KNOTS('',3,(#42782,#42783,#42784,#42785,#42786,
#42787,#42788,#42789,#42790,#42791,#42792,#42793,#42794,#42795,#42796,#42797,
#42798,#42799,#42800,#42801,#42802,#42803,#42804,#42805,#42806,#42807,#42808,
#42809,#42810,#42811,#42812,#42813,#42814,#42815,#42816,#42817,#42818,#42819,
#42820,#42821,#42822,#42823,#42824,#42825,#42826,#42827,#42828,#42829,#42830,
#42831,#42832,#42833,#42834,#42835,#42836,#42837,#42838,#42839,#42840,#42841,
#42842,#42843,#42844,#42845,#42846,#42847,#42848,#42849,#42850,#42851,#42852,
#42853,#42854,#42855,#42856,#42857,#42858,#42859,#42860,#42861,#42862,#42863,
#42864,#42865,#42866,#42867,#42868,#42869,#42870,#42871,#42872,#42873,#42874,
#42875,#42876,#42877,#42878,#42879,#42880,#42881,#42882,#42883,#42884,#42885,
#42886,#42887,#42888,#42889,#42890,#42891,#42892,#42893,#42894,#42895,#42896,
#42897,#42898,#42899,#42900,#42901,#42902,#42903,#42904,#42905,#42906,#42907,
#42908,#42909,#42910,#42911,#42912,#42913,#42914,#42915,#42916,#42917,#42918,
#42919,#42920,#42921,#42922,#42923,#42924,#42925,#42926,#42927,#42928,#42929,
#42930,#42931,#42932,#42933,#42934,#42935,#42936,#42937,#42938,#42939,#42940,
#42941,#42942,#42943,#42944,#42945,#42946,#42947,#42948,#42949,#42950,#42951,
#42952,#42953),.UNSPECIFIED.,.F.,.F.,(4,3,3,3,3,3,3,3,3,3,3,3,3,3,3,3,3,
3,3,3,3,3,3,3,3,3,3,3,3,3,3,3,3,3,3,3,3,3,3,3,3,3,3,3,3,3,3,3,3,3,3,3,3,
3,3,3,3,4),(442.964564156161,443.069008632475,443.176903439814,443.193950200302,
443.270771397457,443.347503359671,443.424162337819,443.500764524281,443.577326066162,
443.65437328435,443.730917458995,443.80747173904,443.88405070402,443.961463980933,
444.03817546124,444.115939636455,444.193703811671,444.271286435285,444.348776417494,
444.426189394719,444.50354094822,444.580846615131,444.658129208176,444.73540099512,
444.812675994976,444.889968225914,444.967332898279,445.044734506712,445.12224232132,
445.193457423041,445.274941395996,445.356320760136,445.440574127284,445.521727622455,
445.602804300415,445.683789728205,445.693334228725,445.774342624629,445.85542688146,
445.939872919697,446.021179001404,446.102562791172,446.184067452201,446.19321103441,
446.270726812673,446.348161113084,446.425529531511,446.502847616661,446.580130880706,
446.657407965018,446.734684545506,446.811974640903,446.889292274908,446.966698481232,
447.044150490546,447.121723298868,447.192964645779,447.201503895611),
 .UNSPECIFIED.);
#384=B_SPLINE_CURVE_WITH_KNOTS('',3,(#42954,#42955,#42956,#42957,#42958,
#42959,#42960,#42961,#42962,#42963,#42964,#42965,#42966,#42967,#42968,#42969,
#42970,#42971,#42972,#42973,#42974,#42975,#42976,#42977,#42978,#42979,#42980,
#42981,#42982,#42983,#42984,#42985,#42986,#42987,#42988,#42989,#42990,#42991,
#42992,#42993,#42994,#42995,#42996,#42997,#42998,#42999,#43000,#43001,#43002,
#43003,#43004,#43005,#43006,#43007,#43008,#43009,#43010,#43011,#43012,#43013,
#43014,#43015,#43016,#43017,#43018,#43019,#43020,#43021,#43022,#43023,#43024,
#43025,#43026,#43027,#43028,#43029),.UNSPECIFIED.,.F.,.F.,(4,3,3,3,3,3,
3,3,3,3,3,3,3,3,3,3,3,3,3,3,3,3,3,3,3,4),(440.918042105346,441.0005037092,
441.08296464717,441.165424946656,441.247884635053,441.330343739755,441.412802288154,
441.49526030764,441.577717825602,441.664395721262,441.746862507097,441.829327620441,
441.911791170946,441.994253268244,442.076714021946,442.159173541643,442.24163193691,
442.324089317308,442.406555703574,442.489018905588,442.571479361868,442.653937510779,
442.736403115658,442.818862994873,442.901327108237,442.964564156161),
 .UNSPECIFIED.);
#385=B_SPLINE_CURVE_WITH_KNOTS('',3,(#43031,#43032,#43033,#43034,#43035,
#43036,#43037,#43038,#43039,#43040,#43041,#43042,#43043,#43044,#43045,#43046,
#43047,#43048,#43049,#43050,#43051,#43052,#43053,#43054,#43055,#43056,#43057,
#43058,#43059,#43060,#43061,#43062,#43063,#43064,#43065,#43066,#43067,#43068,
#43069,#43070,#43071,#43072,#43073,#43074,#43075,#43076,#43077,#43078,#43079,
#43080,#43081,#43082,#43083,#43084,#43085,#43086,#43087,#43088,#43089,#43090,
#43091,#43092,#43093,#43094,#43095,#43096,#43097,#43098,#43099,#43100,#43101,
#43102,#43103,#43104,#43105,#43106,#43107,#43108,#43109,#43110,#43111,#43112,
#43113,#43114,#43115),.UNSPECIFIED.,.F.,.F.,(4,3,3,3,3,3,3,3,3,3,3,3,3,
3,3,3,3,3,3,3,3,3,3,3,3,3,3,3,4),(440.918106228972,440.930476309714,441.008004462923,
441.085451337885,441.162832516592,441.240163534053,441.317459888883,441.394750189219,
441.472040096958,441.549343618956,441.626674767083,441.704094256904,441.781559615326,
441.859145001624,441.928884317765,442.005747702417,442.082517534227,442.159210070215,
442.235841505382,442.312427986166,442.389286028622,442.465844351585,442.542408686258,
442.618993599385,442.696068280993,442.772775101861,442.850033713839,442.927292325816,
442.964564156161),.UNSPECIFIED.);
#386=B_SPLINE_CURVE_WITH_KNOTS('',3,(#43116,#43117,#43118,#43119,#43120,
#43121,#43122,#43123,#43124,#43125,#43126,#43127,#43128,#43129,#43130,#43131,
#43132,#43133,#43134,#43135,#43136,#43137,#43138,#43139,#43140,#43141,#43142,
#43143,#43144,#43145,#43146,#43147,#43148,#43149,#43150,#43151,#43152,#43153,
#43154,#43155,#43156,#43157,#43158,#43159,#43160,#43161,#43162,#43163,#43164,
#43165,#43166,#43167,#43168,#43169,#43170,#43171,#43172,#43173,#43174,#43175,
#43176,#43177,#43178,#43179,#43180,#43181,#43182,#43183,#43184,#43185,#43186,
#43187,#43188,#43189,#43190,#43191,#43192,#43193,#43194,#43195,#43196,#43197,
#43198,#43199,#43200,#43201,#43202,#43203,#43204,#43205,#43206,#43207,#43208,
#43209,#43210,#43211,#43212,#43213,#43214,#43215,#43216,#43217,#43218,#43219,
#43220,#43221,#43222,#43223,#43224,#43225,#43226,#43227,#43228,#43229,#43230,
#43231,#43232,#43233,#43234,#43235,#43236,#43237,#43238,#43239,#43240,#43241,
#43242,#43243,#43244,#43245,#43246,#43247,#43248,#43249,#43250,#43251,#43252,
#43253,#43254,#43255,#43256,#43257,#43258,#43259,#43260,#43261,#43262,#43263,
#43264,#43265,#43266,#43267,#43268,#43269,#43270,#43271,#43272,#43273,#43274,
#43275,#43276,#43277,#43278,#43279,#43280,#43281,#43282,#43283,#43284),
 .UNSPECIFIED.,.F.,.F.,(4,3,3,3,3,3,3,3,3,3,3,3,3,3,3,3,3,3,3,3,3,3,3,3,
3,3,3,3,3,3,3,3,3,3,3,3,3,3,3,3,3,3,3,3,3,3,3,3,3,3,3,3,3,3,3,3,4),(442.964564156239,
443.041606665765,443.118563047945,443.195449387586,443.272281715771,443.349076022084,
443.425858940481,443.50263918525,443.579431196097,443.656249417148,443.733148432809,
443.810093056011,443.887141978737,443.925700333867,444.00323045193,444.080673481246,
444.158045063072,444.235360787431,444.312636203992,444.389897080018,444.467152391364,
444.544416179456,444.62170248784,444.699069349446,444.776477743378,444.85399937625,
444.924108341917,445.00094437404,445.077691389767,445.15436562733,445.230983266851,
445.307560443478,445.384429931789,445.460990034312,445.537560331459,445.614155392481,
445.691245631853,445.767972828434,445.845244589201,445.922516349968,446.000111019402,
446.077613285513,446.155038770583,446.23240304196,446.309721623051,446.387017327523,
446.464302372179,446.541590764112,446.618896509638,446.696274549625,446.77368962137,
446.851210235641,446.920924358019,447.002401893102,447.083786687234,447.16505270286,
447.201722713917),.UNSPECIFIED.);
#387=B_SPLINE_CURVE_WITH_KNOTS('',3,(#43290,#43291,#43292,#43293,#43294,
#43295,#43296,#43297,#43298,#43299,#43300,#43301,#43302,#43303,#43304,#43305,
#43306,#43307,#43308,#43309,#43310,#43311,#43312,#43313,#43314,#43315,#43316,
#43317,#43318,#43319,#43320,#43321,#43322,#43323,#43324,#43325,#43326,#43327,
#43328,#43329,#43330,#43331,#43332,#43333,#43334,#43335,#43336,#43337,#43338,
#43339,#43340,#43341,#43342,#43343,#43344,#43345,#43346,#43347,#43348,#43349,
#43350,#43351,#43352,#43353,#43354,#43355,#43356,#43357,#43358,#43359,#43360,
#43361,#43362,#43363,#43364,#43365,#43366,#43367,#43368,#43369,#43370,#43371,
#43372,#43373,#43374,#43375,#43376,#43377,#43378,#43379,#43380,#43381,#43382,
#43383,#43384,#43385,#43386,#43387,#43388,#43389,#43390,#43391,#43392,#43393,
#43394,#43395,#43396,#43397,#43398,#43399,#43400,#43401,#43402,#43403,#43404,
#43405,#43406,#43407,#43408,#43409,#43410,#43411,#43412,#43413,#43414,#43415,
#43416,#43417,#43418,#43419,#43420,#43421,#43422,#43423,#43424,#43425,#43426,
#43427,#43428,#43429,#43430,#43431,#43432,#43433,#43434,#43435,#43436,#43437,
#43438,#43439,#43440,#43441,#43442,#43443,#43444,#43445,#43446,#43447,#43448,
#43449,#43450,#43451,#43452,#43453,#43454,#43455,#43456,#43457,#43458,#43459,
#43460,#43461),.UNSPECIFIED.,.F.,.F.,(4,3,3,3,3,3,3,3,3,3,3,3,3,3,3,3,3,
3,3,3,3,3,3,3,3,3,3,3,3,3,3,3,3,3,3,3,3,3,3,3,3,3,3,3,3,3,3,3,3,3,3,3,3,
3,3,3,3,4),(449.247749463436,449.324633812506,449.401433890599,449.478165896341,
449.554845974575,449.634518412739,449.711153848794,449.787789394436,449.864439596091,
449.941119006604,450.017880231656,450.09468995308,450.171599527214,450.192225479887,
450.269046677042,450.345778639256,450.422437617404,450.499039803865,450.575601345746,
450.652648563934,450.729192738579,450.805747018624,450.882325983604,450.959739260517,
451.036450740824,451.11421491604,451.191979091257,451.269561714871,451.34705169708,
451.424464674305,451.501816227806,451.579121894718,451.656404487763,451.733676274706,
451.810951274563,451.888243505501,451.965608177866,452.043009786299,452.120517600907,
452.191732702626,452.273216675581,452.354596039721,452.438849406868,452.52000290204,
452.601079579999,452.682065007789,452.691609508311,452.772617904215,452.853702161046,
452.938148199284,453.019454280991,453.100838070759,453.182342731788,453.191486313996,
453.268994750771,453.346431169528,453.423794734071,453.484880270082),
 .UNSPECIFIED.);
#388=B_SPLINE_CURVE_WITH_KNOTS('',3,(#43462,#43463,#43464,#43465,#43466,
#43467,#43468,#43469,#43470,#43471,#43472,#43473,#43474,#43475,#43476,#43477,
#43478,#43479,#43480,#43481,#43482,#43483,#43484,#43485,#43486,#43487,#43488,
#43489,#43490,#43491,#43492,#43493,#43494,#43495,#43496,#43497,#43498,#43499,
#43500,#43501,#43502,#43503,#43504,#43505,#43506,#43507,#43508,#43509,#43510,
#43511,#43512,#43513,#43514,#43515,#43516,#43517,#43518,#43519,#43520,#43521,
#43522,#43523,#43524,#43525,#43526,#43527,#43528,#43529,#43530,#43531,#43532,
#43533,#43534,#43535,#43536,#43537,#43538,#43539,#43540,#43541,#43542,#43543),
 .UNSPECIFIED.,.F.,.F.,(4,3,3,3,3,3,3,3,3,3,3,3,3,3,3,3,3,3,3,3,3,3,3,3,
3,3,3,4),(447.201503895611,447.278341299462,447.355086736831,447.431756469874,
447.508366699878,447.584933580683,447.661483067255,447.738025422464,447.814575221681,
447.891147042584,447.967800680472,448.044496309227,448.121308597704,448.192718257149,
448.270235808767,448.347666028187,448.425024571082,448.502327041669,448.579589003619,
448.656836229402,448.734077740609,448.811327590842,448.888599835755,448.965952793727,
449.043347186035,449.120855513704,449.192471868518,449.247749463341),
 .UNSPECIFIED.);
#389=B_SPLINE_CURVE_WITH_KNOTS('',3,(#43545,#43546,#43547,#43548,#43549,
#43550,#43551,#43552,#43553,#43554,#43555,#43556,#43557,#43558,#43559,#43560,
#43561,#43562,#43563,#43564,#43565,#43566,#43567,#43568,#43569,#43570,#43571,
#43572,#43573,#43574,#43575,#43576,#43577,#43578,#43579,#43580,#43581,#43582,
#43583,#43584,#43585,#43586,#43587,#43588,#43589,#43590,#43591,#43592,#43593,
#43594,#43595,#43596,#43597,#43598,#43599,#43600,#43601,#43602,#43603,#43604,
#43605,#43606,#43607,#43608,#43609,#43610,#43611,#43612,#43613,#43614,#43615,
#43616,#43617,#43618,#43619,#43620,#43621,#43622,#43623,#43624,#43625,#43626),
 .UNSPECIFIED.,.F.,.F.,(4,3,3,3,3,3,3,3,3,3,3,3,3,3,3,3,3,3,3,3,3,3,3,3,
3,3,3,4),(447.201722713917,447.282847402085,447.363869242774,447.420128362045,
447.501141468335,447.582230162609,447.666505713474,447.747815179864,447.829202081075,
447.91070921984,447.91933236607,447.996860519279,448.07430739424,448.151688572948,
448.229019590409,448.306315945239,448.383606245575,448.460896153313,448.538199675311,
448.615530823439,448.69295031326,448.770415671682,448.84800105798,448.917740374121,
449.008245292473,449.098328326512,449.187621314979,449.24774946334),
 .UNSPECIFIED.);
#390=B_SPLINE_CURVE_WITH_KNOTS('',3,(#43627,#43628,#43629,#43630,#43631,
#43632,#43633,#43634,#43635,#43636,#43637,#43638,#43639,#43640,#43641,#43642,
#43643,#43644,#43645,#43646,#43647,#43648,#43649,#43650,#43651,#43652,#43653,
#43654,#43655,#43656,#43657,#43658,#43659,#43660,#43661,#43662,#43663,#43664,
#43665,#43666,#43667,#43668,#43669,#43670,#43671,#43672,#43673,#43674,#43675,
#43676,#43677,#43678,#43679,#43680,#43681,#43682,#43683,#43684,#43685,#43686,
#43687,#43688,#43689,#43690,#43691,#43692,#43693,#43694,#43695,#43696,#43697,
#43698,#43699,#43700,#43701,#43702,#43703,#43704,#43705,#43706,#43707,#43708,
#43709,#43710,#43711,#43712,#43713,#43714,#43715,#43716,#43717,#43718,#43719,
#43720,#43721,#43722,#43723,#43724,#43725,#43726,#43727,#43728,#43729,#43730,
#43731,#43732,#43733,#43734,#43735,#43736,#43737,#43738,#43739,#43740,#43741,
#43742,#43743,#43744,#43745,#43746,#43747,#43748,#43749,#43750,#43751,#43752,
#43753,#43754,#43755,#43756,#43757,#43758,#43759,#43760,#43761,#43762,#43763,
#43764,#43765,#43766,#43767,#43768,#43769,#43770,#43771,#43772,#43773,#43774,
#43775,#43776,#43777,#43778,#43779,#43780,#43781,#43782,#43783),
 .UNSPECIFIED.,.F.,.F.,(4,3,3,3,3,3,3,3,3,3,3,3,3,3,3,3,3,3,3,3,3,3,3,3,
3,3,3,3,3,3,3,3,3,3,3,3,3,3,3,3,3,3,3,3,3,3,3,3,3,3,3,3,4),(449.24774946334,
449.330211669376,449.412673527116,449.49513504341,449.577596225107,449.660057079059,
449.742517612113,449.824977831119,449.907437742927,449.989897354385,450.072356672341,
450.154815703643,450.23727445514,450.319732933678,450.402191146106,450.484649099271,
450.567106800018,450.649564255196,450.732021471651,450.818033698152,450.901358042576,
450.983824648021,451.066290409263,451.148755353715,451.231219508791,451.3136829019,
451.396145560449,451.478607511841,451.56106878348,451.643529402764,451.725989397091,
451.808448793856,451.890907620451,451.973365904268,452.055823672695,452.13828095312,
452.222414188532,452.304880186624,452.387344562979,452.469807427241,452.552268889032,
452.634729057953,452.717188043589,452.799645955506,452.885241801031,452.967706537631,
453.050168309633,453.132627555475,453.215084713452,453.297547231733,453.380004902588,
453.462463692539,453.484412719705),.UNSPECIFIED.);
#391=B_SPLINE_CURVE_WITH_KNOTS('',3,(#43789,#43790,#43791,#43792,#43793,
#43794,#43795,#43796,#43797,#43798,#43799,#43800,#43801,#43802,#43803,#43804,
#43805,#43806,#43807,#43808,#43809,#43810,#43811,#43812,#43813,#43814,#43815,
#43816,#43817,#43818,#43819,#43820,#43821,#43822,#43823,#43824,#43825,#43826,
#43827,#43828,#43829,#43830,#43831,#43832,#43833,#43834,#43835,#43836,#43837,
#43838,#43839,#43840,#43841,#43842,#43843,#43844,#43845,#43846,#43847,#43848,
#43849,#43850,#43851,#43852,#43853,#43854,#43855,#43856,#43857,#43858,#43859,
#43860,#43861,#43862,#43863,#43864,#43865,#43866,#43867,#43868,#43869,#43870,
#43871,#43872,#43873,#43874,#43875,#43876,#43877,#43878,#43879,#43880,#43881,
#43882,#43883,#43884,#43885,#43886,#43887,#43888,#43889,#43890,#43891,#43892,
#43893,#43894,#43895,#43896,#43897,#43898,#43899,#43900,#43901,#43902,#43903,
#43904,#43905,#43906,#43907,#43908,#43909,#43910,#43911,#43912,#43913,#43914,
#43915,#43916,#43917,#43918,#43919,#43920,#43921,#43922,#43923,#43924,#43925,
#43926,#43927,#43928,#43929,#43930,#43931,#43932,#43933,#43934,#43935,#43936,
#43937,#43938,#43939,#43940,#43941,#43942,#43943,#43944,#43945),
 .UNSPECIFIED.,.F.,.F.,(4,3,3,3,3,3,3,3,3,3,3,3,3,3,3,3,3,3,3,3,3,3,3,3,
3,3,3,3,3,3,3,3,3,3,3,3,3,3,3,3,3,3,3,3,3,3,3,3,3,3,3,3,4),(455.53093477052,
455.613396976556,455.695858834296,455.77832035059,455.860781532287,455.943242386238,
456.025702919293,456.108163138299,456.190623050107,456.273082661565,456.355541979521,
456.438001010823,456.52045976232,456.602918240858,456.685376453286,456.767834406451,
456.850292107198,456.932749562376,457.015206778831,457.101219005332,457.184543349756,
457.267009955201,457.349475716443,457.431940660895,457.514404815971,457.59686820908,
457.679330867629,457.761792819021,457.84425409066,457.926714709944,458.009174704271,
458.091634101036,458.174092927631,458.256551211448,458.339008979875,458.4214662603,
458.505599495712,458.588065493804,458.670529870159,458.752992734421,458.835454196212,
458.917914365133,459.000373350769,459.082831262686,459.168427108211,459.250891844811,
459.333353616813,459.415812862655,459.498270020632,459.580732538913,459.663190209768,
459.745648999719,459.767598026885),.UNSPECIFIED.);
#392=B_SPLINE_CURVE_WITH_KNOTS('',3,(#43946,#43947,#43948,#43949,#43950,
#43951,#43952,#43953,#43954,#43955,#43956,#43957,#43958,#43959,#43960,#43961,
#43962,#43963,#43964,#43965,#43966,#43967,#43968,#43969,#43970,#43971,#43972,
#43973,#43974,#43975,#43976,#43977,#43978,#43979,#43980,#43981,#43982,#43983,
#43984,#43985,#43986,#43987,#43988,#43989,#43990,#43991,#43992,#43993,#43994,
#43995,#43996,#43997,#43998,#43999,#44000,#44001,#44002,#44003,#44004,#44005,
#44006,#44007,#44008,#44009,#44010,#44011,#44012,#44013,#44014,#44015,#44016,
#44017,#44018,#44019,#44020,#44021,#44022,#44023,#44024),.UNSPECIFIED.,
 .F.,.F.,(4,3,3,3,3,3,3,3,3,3,3,3,3,3,3,3,3,3,3,3,3,3,3,3,3,3,4),(453.484880270082,
453.5621695649,453.640803359958,453.718078947669,453.795365350718,453.872676591241,
453.952317424772,454.029761082876,454.110500504121,454.191239925365,454.268088548552,
454.344843394949,454.421520734353,454.498136774128,454.574707672753,454.65174340575,
454.728285824456,454.804834161018,454.881402992466,454.958800628533,455.035491709486,
455.11324262311,455.190993536734,455.282364191347,455.373352208432,455.463557419382,
455.53093477052),.UNSPECIFIED.);
#393=B_SPLINE_CURVE_WITH_KNOTS('',3,(#44026,#44027,#44028,#44029,#44030,
#44031,#44032,#44033,#44034,#44035,#44036,#44037,#44038,#44039,#44040,#44041,
#44042,#44043,#44044,#44045,#44046,#44047,#44048,#44049,#44050,#44051,#44052,
#44053,#44054,#44055,#44056,#44057,#44058,#44059,#44060,#44061,#44062,#44063,
#44064,#44065,#44066,#44067,#44068,#44069,#44070,#44071,#44072,#44073,#44074,
#44075,#44076,#44077,#44078,#44079,#44080,#44081,#44082,#44083,#44084,#44085,
#44086,#44087,#44088,#44089,#44090,#44091,#44092,#44093,#44094,#44095,#44096,
#44097,#44098,#44099,#44100,#44101),.UNSPECIFIED.,.F.,.F.,(4,3,3,3,3,3,
3,3,3,3,3,3,3,3,3,3,3,3,3,3,3,3,3,3,3,4),(453.484412719705,453.566874323559,
453.649335261529,453.731795561015,453.814255249412,453.896714354114,453.979172902513,
454.061630921999,454.144088439961,454.230766335621,454.313233121457,454.3956982348,
454.478161785305,454.560623882603,454.643084636305,454.725544156002,454.808002551269,
454.890459931666,454.972926317933,455.055389519947,455.137849976227,455.220308125138,
455.302773730017,455.385233609232,455.467697722596,455.53093477052),
 .UNSPECIFIED.);
#394=B_SPLINE_CURVE_WITH_KNOTS('',3,(#44102,#44103,#44104,#44105,#44106,
#44107,#44108,#44109,#44110,#44111,#44112,#44113,#44114,#44115,#44116,#44117,
#44118,#44119,#44120,#44121,#44122,#44123,#44124,#44125,#44126,#44127,#44128,
#44129,#44130,#44131,#44132,#44133,#44134,#44135,#44136,#44137,#44138,#44139,
#44140,#44141,#44142,#44143,#44144,#44145,#44146,#44147,#44148,#44149,#44150,
#44151,#44152,#44153,#44154,#44155,#44156,#44157,#44158,#44159,#44160,#44161,
#44162,#44163,#44164,#44165,#44166,#44167,#44168,#44169,#44170,#44171,#44172,
#44173,#44174,#44175,#44176,#44177,#44178,#44179,#44180,#44181,#44182,#44183,
#44184,#44185,#44186,#44187,#44188,#44189,#44190,#44191,#44192,#44193,#44194,
#44195,#44196,#44197,#44198,#44199,#44200,#44201,#44202,#44203,#44204,#44205,
#44206,#44207,#44208,#44209,#44210,#44211,#44212,#44213,#44214,#44215,#44216,
#44217,#44218,#44219,#44220,#44221,#44222,#44223,#44224,#44225,#44226,#44227,
#44228,#44229,#44230,#44231,#44232,#44233,#44234,#44235,#44236,#44237,#44238,
#44239,#44240,#44241,#44242,#44243,#44244,#44245,#44246,#44247,#44248,#44249,
#44250,#44251,#44252,#44253,#44254,#44255,#44256,#44257,#44258,#44259,#44260,
#44261,#44262,#44263,#44264,#44265,#44266,#44267,#44268,#44269,#44270),
 .UNSPECIFIED.,.F.,.F.,(4,3,3,3,3,3,3,3,3,3,3,3,3,3,3,3,3,3,3,3,3,3,3,3,
3,3,3,3,3,3,3,3,3,3,3,3,3,3,3,3,3,3,3,3,3,3,3,3,3,3,3,3,3,3,3,3,4),(455.53093477052,
455.619328038375,455.708463066107,455.797969399037,455.887897298536,455.906596430478,
455.98345981513,456.06022964694,456.136922182928,456.213553618095,456.290140098879,
456.366998141335,456.443556464298,456.520120798971,456.596705712098,456.673780393705,
456.750487214574,456.827745826551,456.905004438528,456.982534634988,457.059977729593,
457.137349363649,457.214665127217,457.291940569996,457.369201452415,457.44645675806,
457.523720528354,457.601006806838,457.67837361963,457.755781954337,457.8333035109,
457.903412446579,457.980942564642,458.058385593958,458.135757175784,458.213072900144,
458.290348316705,458.367609192731,458.444864504077,458.522128292169,458.599414600553,
458.676781462159,458.754189856091,458.831711488963,458.90182045463,458.978663768531,
459.055416516633,459.132094944059,459.211432932134,459.288010571749,459.364567540298,
459.441118406981,459.517677734815,459.594288165648,459.670929289699,459.747644296304,
459.766798848659),.UNSPECIFIED.);
#395=B_SPLINE_CURVE_WITH_KNOTS('',3,(#44276,#44277,#44278,#44279,#44280,
#44281,#44282,#44283,#44284,#44285,#44286,#44287,#44288,#44289,#44290,#44291,
#44292,#44293,#44294,#44295,#44296,#44297,#44298,#44299,#44300,#44301,#44302,
#44303,#44304,#44305,#44306,#44307,#44308,#44309,#44310,#44311,#44312,#44313,
#44314,#44315,#44316,#44317,#44318,#44319,#44320,#44321,#44322,#44323,#44324,
#44325,#44326,#44327,#44328,#44329,#44330,#44331,#44332,#44333,#44334,#44335,
#44336,#44337,#44338,#44339,#44340,#44341,#44342,#44343,#44344,#44345,#44346,
#44347,#44348,#44349,#44350,#44351,#44352,#44353,#44354,#44355,#44356,#44357,
#44358,#44359,#44360,#44361,#44362,#44363,#44364,#44365,#44366,#44367,#44368,
#44369,#44370,#44371,#44372,#44373,#44374,#44375,#44376,#44377,#44378,#44379,
#44380,#44381,#44382,#44383,#44384,#44385,#44386,#44387,#44388,#44389,#44390,
#44391,#44392,#44393,#44394,#44395,#44396,#44397,#44398,#44399,#44400,#44401,
#44402,#44403,#44404,#44405,#44406,#44407,#44408,#44409,#44410,#44411,#44412,
#44413,#44414,#44415,#44416,#44417,#44418,#44419,#44420,#44421,#44422,#44423,
#44424,#44425,#44426,#44427,#44428,#44429,#44430,#44431,#44432,#44433,#44434,
#44435,#44436,#44437,#44438,#44439,#44440,#44441),.UNSPECIFIED.,.F.,.F.,
(4,3,3,3,3,3,3,3,3,3,3,3,3,3,3,3,3,3,3,3,3,3,3,3,3,3,3,3,3,3,3,3,3,3,3,
3,3,3,3,3,3,3,3,3,3,3,3,3,3,3,3,3,3,3,3,4),(461.8141200777,461.899839896198,
461.986073399186,462.072573444055,462.159420638358,462.18926881632,462.266786367938,
462.344216587357,462.421575130251,462.498877600838,462.576139562788,462.65338678857,
462.730628299776,462.807878150009,462.885150394921,462.962503352891,463.0398977452,
463.117406072867,463.189022427689,463.266539796888,463.343969864341,463.421328285613,
463.498630664831,463.575892565596,463.653139776289,463.73038130051,463.807631191859,
463.884903506005,463.962256577233,464.039651106987,464.117159611951,464.188776039059,
464.265597236211,464.342329198423,464.418988176569,464.495590363028,464.572151904906,
464.649199123096,464.725743297738,464.802297577781,464.878876542759,464.956289819676,
465.033001299981,465.110765475204,465.188529650428,465.266120294956,465.343616772867,
465.421034726906,465.499685965902,465.576989793296,465.654266870418,465.731531224882,
465.81120957838,465.888513538795,465.969379088835,466.050244638876),
 .UNSPECIFIED.);
#396=B_SPLINE_CURVE_WITH_KNOTS('',3,(#44442,#44443,#44444,#44445,#44446,
#44447,#44448,#44449,#44450,#44451,#44452,#44453,#44454,#44455,#44456,#44457,
#44458,#44459,#44460,#44461,#44462,#44463,#44464,#44465,#44466,#44467,#44468,
#44469,#44470,#44471,#44472,#44473,#44474,#44475,#44476,#44477,#44478,#44479,
#44480,#44481,#44482,#44483,#44484,#44485,#44486,#44487,#44488,#44489,#44490,
#44491,#44492,#44493,#44494,#44495,#44496,#44497,#44498,#44499,#44500,#44501,
#44502,#44503,#44504,#44505,#44506,#44507,#44508,#44509,#44510,#44511,#44512,
#44513,#44514,#44515,#44516,#44517),.UNSPECIFIED.,.F.,.F.,(4,3,3,3,3,3,
3,3,3,3,3,3,3,3,3,3,3,3,3,3,3,3,3,3,3,4),(459.767598026885,459.850059630739,
459.932520568709,460.014980868195,460.097440556592,460.179899661294,460.262358209693,
460.34481622918,460.427273747141,460.513951642801,460.596418428637,460.67888354198,
460.761347092486,460.843809189783,460.926269943485,461.008729463182,461.09118785845,
461.173645238847,461.256111625113,461.338574827127,461.421035283408,461.503493432319,
461.585959037198,461.668418916412,461.750883029776,461.8141200777),
 .UNSPECIFIED.);
#397=B_SPLINE_CURVE_WITH_KNOTS('',3,(#44519,#44520,#44521,#44522,#44523,
#44524,#44525,#44526,#44527,#44528,#44529,#44530,#44531,#44532,#44533,#44534,
#44535,#44536,#44537,#44538,#44539,#44540,#44541,#44542,#44543,#44544,#44545,
#44546,#44547,#44548,#44549,#44550,#44551,#44552,#44553,#44554,#44555,#44556,
#44557,#44558,#44559,#44560,#44561,#44562,#44563,#44564,#44565,#44566,#44567,
#44568,#44569,#44570,#44571,#44572,#44573,#44574,#44575,#44576,#44577,#44578,
#44579,#44580,#44581,#44582,#44583,#44584,#44585,#44586,#44587,#44588,#44589,
#44590,#44591,#44592,#44593,#44594,#44595,#44596,#44597,#44598,#44599,#44600,
#44601,#44602,#44603),.UNSPECIFIED.,.F.,.F.,(4,3,3,3,3,3,3,3,3,3,3,3,3,
3,3,3,3,3,3,3,3,3,3,3,3,3,3,3,4),(459.766798848659,459.843658493391,459.900228462681,
459.977823132115,460.055325398226,460.132750883296,460.210115154673,460.287433735764,
460.364729440236,460.442014484892,460.519302876825,460.596608622351,460.673986662338,
460.751401734083,460.828922348354,460.898636470732,460.980122785165,461.061504867524,
461.145588769333,461.226746088186,461.307826871941,461.388816863975,461.397840474758,
461.475955296957,461.554107861435,461.632351562766,461.710648170262,461.789049728251,
461.814120077565),.UNSPECIFIED.);
#398=B_SPLINE_CURVE_WITH_KNOTS('',3,(#44604,#44605,#44606,#44607,#44608,
#44609,#44610,#44611,#44612,#44613,#44614,#44615,#44616,#44617,#44618,#44619,
#44620,#44621,#44622,#44623,#44624,#44625,#44626,#44627,#44628,#44629,#44630,
#44631,#44632,#44633,#44634,#44635,#44636,#44637,#44638,#44639,#44640,#44641,
#44642,#44643,#44644,#44645,#44646,#44647,#44648,#44649,#44650,#44651,#44652,
#44653,#44654,#44655,#44656,#44657,#44658,#44659,#44660,#44661,#44662,#44663,
#44664,#44665,#44666,#44667,#44668,#44669,#44670,#44671,#44672,#44673,#44674,
#44675,#44676,#44677,#44678,#44679,#44680,#44681,#44682,#44683,#44684,#44685,
#44686,#44687,#44688,#44689,#44690,#44691,#44692,#44693,#44694,#44695,#44696,
#44697,#44698,#44699,#44700,#44701,#44702,#44703,#44704,#44705,#44706,#44707,
#44708,#44709,#44710,#44711,#44712,#44713,#44714,#44715,#44716,#44717,#44718,
#44719,#44720,#44721,#44722,#44723,#44724,#44725,#44726,#44727,#44728,#44729,
#44730,#44731,#44732,#44733,#44734,#44735,#44736,#44737,#44738,#44739,#44740,
#44741,#44742,#44743,#44744,#44745,#44746,#44747,#44748,#44749,#44750,#44751,
#44752,#44753,#44754,#44755,#44756,#44757,#44758,#44759,#44760,#44761,#44762,
#44763,#44764,#44765,#44766,#44767,#44768,#44769),.UNSPECIFIED.,.F.,.F.,
(4,3,3,3,3,3,3,3,3,3,3,3,3,3,3,3,3,3,3,3,3,3,3,3,3,3,3,3,3,3,3,3,3,3,3,
3,3,3,3,3,3,3,3,3,3,3,3,3,3,3,3,3,3,3,3,4),(461.814120077699,461.897044478783,
461.974572631993,462.052019506954,462.129400685662,462.206731703123,462.284028057954,
462.361318358291,462.438608266029,462.515911788028,462.593242936156,462.670662425977,
462.748127784399,462.825713170698,462.895452486834,462.972315871486,463.049085703295,
463.125778239283,463.20240967445,463.278996155233,463.35585419769,463.432412520653,
463.508976855325,463.585561768452,463.66263645006,463.739343270929,463.816601882907,
463.893860494885,463.971390691344,464.048833785949,464.126205420004,464.203521183572,
464.28079662635,464.358057508769,464.435312814412,464.512576584706,464.58986286319,
464.667229675981,464.744638010688,464.82215956725,464.892268502936,464.969798621002,
465.04724165032,465.124613232148,465.20192895651,465.279204373074,465.356465249102,
465.43372056045,465.510984348545,465.588270656931,465.665637518539,465.743045912474,
465.820567545348,465.890676510987,465.97105445669,466.051432402393),
 .UNSPECIFIED.);
#399=B_SPLINE_CURVE_WITH_KNOTS('',3,(#44775,#44776,#44777,#44778,#44779,
#44780,#44781,#44782,#44783,#44784,#44785,#44786,#44787,#44788,#44789,#44790,
#44791,#44792,#44793,#44794,#44795,#44796,#44797,#44798,#44799,#44800,#44801,
#44802,#44803,#44804,#44805,#44806,#44807,#44808,#44809,#44810,#44811,#44812,
#44813,#44814,#44815,#44816,#44817,#44818,#44819,#44820,#44821,#44822,#44823,
#44824,#44825,#44826,#44827,#44828,#44829,#44830,#44831,#44832,#44833,#44834,
#44835,#44836,#44837,#44838,#44839,#44840,#44841,#44842,#44843,#44844,#44845,
#44846,#44847,#44848,#44849,#44850,#44851,#44852,#44853,#44854,#44855,#44856,
#44857,#44858,#44859,#44860,#44861,#44862,#44863,#44864,#44865,#44866,#44867,
#44868,#44869,#44870,#44871,#44872,#44873,#44874,#44875,#44876,#44877,#44878,
#44879,#44880,#44881,#44882,#44883,#44884,#44885,#44886,#44887,#44888,#44889,
#44890,#44891,#44892,#44893,#44894,#44895,#44896,#44897,#44898,#44899,#44900,
#44901,#44902,#44903,#44904,#44905,#44906,#44907,#44908,#44909,#44910,#44911,
#44912,#44913,#44914,#44915,#44916,#44917,#44918,#44919,#44920,#44921,#44922,
#44923,#44924,#44925,#44926,#44927,#44928,#44929,#44930,#44931),
 .UNSPECIFIED.,.F.,.F.,(4,3,3,3,3,3,3,3,3,3,3,3,3,3,3,3,3,3,3,3,3,3,3,3,
3,3,3,3,3,3,3,3,3,3,3,3,3,3,3,3,3,3,3,3,3,3,3,3,3,3,3,3,4),(468.097305384879,
468.179767590915,468.262229448655,468.344690964949,468.427152146646,468.509613000597,
468.592073533652,468.674533752658,468.756993664466,468.839453275924,468.92191259388,
469.004371625182,469.086830376679,469.169288855217,469.251747067645,469.33420502081,
469.416662721557,469.499120176735,469.58157739319,469.667589619691,469.750913964115,
469.83338056956,469.915846330802,469.998311275254,470.08077543033,470.163238823439,
470.245701481988,470.328163433381,470.410624705019,470.493085324303,470.57554531863,
470.658004715395,470.74046354199,470.822921825806,470.905379594234,470.987836874659,
471.071970110071,471.154436108162,471.236900484518,471.31936334878,471.401824810571,
471.484284979492,471.566743965127,471.649201877045,471.73479772257,471.81726245917,
471.899724231172,471.982183477014,472.064640634991,472.147103153272,472.229560824127,
472.312019614078,472.333968641244),.UNSPECIFIED.);
#400=B_SPLINE_CURVE_WITH_KNOTS('',3,(#44932,#44933,#44934,#44935,#44936,
#44937,#44938,#44939,#44940,#44941,#44942,#44943,#44944,#44945,#44946,#44947,
#44948,#44949,#44950,#44951,#44952,#44953,#44954,#44955,#44956,#44957,#44958,
#44959,#44960,#44961,#44962,#44963,#44964,#44965,#44966,#44967,#44968,#44969,
#44970,#44971,#44972,#44973,#44974,#44975,#44976,#44977,#44978,#44979,#44980,
#44981,#44982,#44983,#44984,#44985,#44986,#44987,#44988,#44989,#44990,#44991,
#44992,#44993,#44994,#44995,#44996,#44997,#44998,#44999,#45000,#45001,#45002,
#45003,#45004,#45005,#45006,#45007,#45008,#45009,#45010,#45011,#45012,#45013,
#45014,#45015,#45016),.UNSPECIFIED.,.F.,.F.,(4,3,3,3,3,3,3,3,3,3,3,3,3,
3,3,3,3,3,3,3,3,3,3,3,3,3,3,3,4),(466.050244638876,466.127755854532,466.188283261797,
466.269767234823,466.351146599033,466.435399966145,466.516553461384,466.59763013941,
466.678615567264,466.688160067482,466.769168463268,466.850252719979,466.934698758276,
467.016004839858,467.0973886295,467.178893290403,467.188036873167,467.264497215168,
467.340875943928,467.417189540611,467.493454429304,467.569694421594,467.645922807574,
467.722154389377,467.798403969437,467.874729422595,467.951093785583,468.027569488965,
468.096918372593),.UNSPECIFIED.);
#401=B_SPLINE_CURVE_WITH_KNOTS('',3,(#45018,#45019,#45020,#45021,#45022,
#45023,#45024,#45025,#45026,#45027,#45028,#45029,#45030,#45031,#45032,#45033,
#45034,#45035,#45036,#45037,#45038,#45039,#45040,#45041,#45042,#45043,#45044,
#45045,#45046,#45047,#45048,#45049,#45050,#45051,#45052,#45053,#45054,#45055,
#45056,#45057,#45058,#45059,#45060,#45061,#45062,#45063,#45064,#45065,#45066,
#45067,#45068,#45069,#45070,#45071,#45072,#45073,#45074,#45075,#45076,#45077,
#45078,#45079,#45080,#45081,#45082,#45083,#45084,#45085,#45086,#45087,#45088,
#45089,#45090,#45091,#45092,#45093,#45094,#45095,#45096),.UNSPECIFIED.,
 .F.,.F.,(4,3,3,3,3,3,3,3,3,3,3,3,3,3,3,3,3,3,3,3,3,3,3,3,3,3,4),(466.051432402393,
466.128100662332,466.204713834782,466.281288051319,466.357851539603,466.434411961159,
466.510983881253,466.587581869918,466.664267937965,466.740999464938,466.817853223278,
466.889084519038,466.966679188465,467.044181454569,467.121606939632,467.198971211002,
467.276289792086,467.353585496551,467.4308705412,467.508158933126,467.585464678645,
467.662842718626,467.740257790364,467.817778404628,467.887492527089,467.992398955984,
468.097305384879),.UNSPECIFIED.);
#402=B_SPLINE_CURVE_WITH_KNOTS('',3,(#45097,#45098,#45099,#45100,#45101,
#45102,#45103,#45104,#45105,#45106,#45107,#45108,#45109,#45110,#45111,#45112,
#45113,#45114,#45115,#45116,#45117,#45118,#45119,#45120,#45121,#45122,#45123,
#45124,#45125,#45126,#45127,#45128,#45129,#45130,#45131,#45132,#45133,#45134,
#45135,#45136,#45137,#45138,#45139,#45140,#45141,#45142,#45143,#45144,#45145,
#45146,#45147,#45148,#45149,#45150,#45151,#45152,#45153,#45154,#45155,#45156,
#45157,#45158,#45159,#45160,#45161,#45162,#45163,#45164,#45165,#45166,#45167,
#45168,#45169,#45170,#45171,#45172,#45173,#45174,#45175,#45176,#45177,#45178,
#45179,#45180,#45181,#45182,#45183,#45184,#45185,#45186,#45187,#45188,#45189,
#45190,#45191,#45192,#45193,#45194,#45195,#45196,#45197,#45198,#45199,#45200,
#45201,#45202,#45203,#45204,#45205,#45206,#45207,#45208,#45209,#45210,#45211,
#45212,#45213,#45214,#45215,#45216,#45217,#45218,#45219,#45220,#45221,#45222,
#45223,#45224,#45225,#45226,#45227,#45228,#45229,#45230,#45231,#45232,#45233,
#45234,#45235,#45236,#45237,#45238,#45239,#45240,#45241,#45242,#45243,#45244,
#45245,#45246,#45247,#45248,#45249,#45250,#45251,#45252,#45253,#45254,#45255,
#45256,#45257,#45258,#45259,#45260,#45261,#45262,#45263,#45264,#45265),
 .UNSPECIFIED.,.F.,.F.,(4,3,3,3,3,3,3,3,3,3,3,3,3,3,3,3,3,3,3,3,3,3,3,3,
3,3,3,3,3,3,3,3,3,3,3,3,3,3,3,3,3,3,3,3,3,3,3,3,3,3,3,3,3,3,3,3,4),(468.097305384968,
468.172742017472,468.248128780957,468.323482174757,468.386696531114,468.467709637285,
468.548798331437,468.633073882363,468.714383348627,468.795770249711,468.877277388349,
468.885900535139,468.963428688398,469.040875563409,469.118256742166,469.195587759677,
469.272884114558,469.350174414944,469.427464322733,469.504767844781,469.582098992958,
469.659518482829,469.7369838413,469.814569227647,469.88430854319,469.961171927862,
470.037941759691,470.1146342957,470.191265730887,470.267852211691,470.344710254135,
470.421268577119,470.497832911812,470.574417824961,470.651492506531,470.728199327421,
470.805457939331,470.882716551241,470.960246747535,471.037689841973,471.115061475862,
471.192377239264,471.269652681875,471.346913564128,471.424168869606,471.501432639735,
471.578718918054,471.656085730683,471.733494065228,471.811015621632,471.881124559292,
471.958659520324,472.036109852615,472.113473924364,472.19078786829,472.268064511653,
472.334165849073),.UNSPECIFIED.);
#403=B_SPLINE_CURVE_WITH_KNOTS('',3,(#45271,#45272,#45273,#45274,#45275,
#45276,#45277,#45278,#45279,#45280,#45281,#45282,#45283,#45284,#45285,#45286,
#45287,#45288,#45289,#45290,#45291,#45292,#45293,#45294,#45295,#45296,#45297,
#45298,#45299,#45300,#45301,#45302,#45303,#45304,#45305,#45306,#45307,#45308,
#45309,#45310,#45311,#45312,#45313,#45314,#45315,#45316,#45317,#45318,#45319,
#45320,#45321,#45322,#45323,#45324,#45325,#45326,#45327,#45328,#45329,#45330,
#45331,#45332,#45333,#45334,#45335,#45336,#45337,#45338,#45339,#45340,#45341,
#45342,#45343,#45344,#45345,#45346,#45347,#45348,#45349,#45350,#45351,#45352,
#45353,#45354,#45355,#45356,#45357,#45358,#45359,#45360,#45361,#45362,#45363,
#45364,#45365,#45366,#45367,#45368,#45369,#45370,#45371,#45372,#45373,#45374,
#45375,#45376,#45377,#45378,#45379,#45380,#45381,#45382,#45383,#45384,#45385,
#45386,#45387,#45388,#45389,#45390,#45391,#45392,#45393,#45394,#45395,#45396,
#45397,#45398,#45399,#45400,#45401,#45402,#45403,#45404,#45405,#45406,#45407,
#45408,#45409,#45410,#45411,#45412,#45413,#45414,#45415,#45416,#45417,#45418,
#45419,#45420,#45421,#45422,#45423,#45424,#45425,#45426,#45427,#45428,#45429,
#45430,#45431,#45432,#45433,#45434,#45435,#45436,#45437,#45438,#45439),
 .UNSPECIFIED.,.F.,.F.,(4,3,3,3,3,3,3,3,3,3,3,3,3,3,3,3,3,3,3,3,3,3,3,3,
3,3,3,3,3,3,3,3,3,3,3,3,3,3,3,3,3,3,3,3,3,3,3,3,3,3,3,3,3,3,3,3,4),(474.381281477029,
474.45785620268,474.534379006077,474.610866110696,474.687346011724,474.763825899523,
474.840320428267,474.91684425907,474.993454306524,475.070112975877,475.146881411406,
475.186065764122,475.262914397353,475.339669253825,475.416346603329,475.49296265322,
475.569533561969,475.646569288659,475.723111717468,475.799660064117,475.876228905626,
475.953626523092,476.030317613975,476.108068494733,476.185819375491,476.263336904457,
476.34076710121,476.418125621448,476.495428069405,476.572690008776,476.64993721213,
476.727178701002,476.804428529013,476.881700751837,476.959053688043,477.036448058732,
477.113956365229,477.18557298686,477.263090364072,477.340520439403,477.417878868409,
477.495181255212,477.57244316341,477.649690381279,477.726931912518,477.804181810723,
477.881454131557,477.958807209175,478.036201745166,478.113710256049,478.18532659823,
478.26215530598,478.338896867184,478.415549744414,478.492151381125,478.568713263294,
478.61726357937),.UNSPECIFIED.);
#404=B_SPLINE_CURVE_WITH_KNOTS('',3,(#45440,#45441,#45442,#45443,#45444,
#45445,#45446,#45447,#45448,#45449,#45450,#45451,#45452,#45453,#45454,#45455,
#45456,#45457,#45458,#45459,#45460,#45461,#45462,#45463,#45464,#45465,#45466,
#45467,#45468,#45469,#45470,#45471,#45472,#45473,#45474,#45475,#45476,#45477,
#45478,#45479,#45480,#45481,#45482,#45483,#45484,#45485,#45486,#45487,#45488,
#45489,#45490,#45491,#45492,#45493,#45494,#45495,#45496,#45497,#45498,#45499,
#45500,#45501,#45502,#45503,#45504,#45505,#45506,#45507,#45508,#45509,#45510,
#45511,#45512,#45513,#45514,#45515),.UNSPECIFIED.,.F.,.F.,(4,3,3,3,3,3,
3,3,3,3,3,3,3,3,3,3,3,3,3,3,3,3,3,3,3,4),(472.333968641244,472.416430245098,
472.498891183068,472.581351482554,472.663811170951,472.746270275653,472.828728824052,
472.911186843538,472.9936443615,473.080322256826,473.162789042661,473.245254156005,
473.32771770651,473.410179803808,473.492640557509,473.575100077206,473.657558472473,
473.74001585287,473.822482239137,473.90494544115,473.987405897431,474.069864046341,
474.15232965122,474.234789530434,474.317253643797,474.380490686714),
 .UNSPECIFIED.);
#405=B_SPLINE_CURVE_WITH_KNOTS('',3,(#45517,#45518,#45519,#45520,#45521,
#45522,#45523,#45524,#45525,#45526,#45527,#45528,#45529,#45530,#45531,#45532,
#45533,#45534,#45535,#45536,#45537,#45538,#45539,#45540,#45541,#45542,#45543,
#45544,#45545,#45546,#45547,#45548,#45549,#45550,#45551,#45552,#45553,#45554,
#45555,#45556,#45557,#45558,#45559,#45560,#45561,#45562,#45563,#45564,#45565,
#45566,#45567,#45568,#45569,#45570,#45571,#45572,#45573,#45574,#45575,#45576,
#45577,#45578,#45579,#45580,#45581,#45582,#45583,#45584,#45585,#45586,#45587,
#45588,#45589,#45590,#45591,#45592,#45593,#45594,#45595),.UNSPECIFIED.,
 .F.,.F.,(4,3,3,3,3,3,3,3,3,3,3,3,3,3,3,3,3,3,3,3,3,3,3,3,3,3,4),(472.334165849073,
472.411421096754,472.488682793709,472.565964982701,472.644356878861,472.721759112864,
472.800645840103,472.879532567343,472.956368599592,473.033115615447,473.10978985314,
473.186407492793,473.262984669552,473.339854157782,473.416414260441,473.492984557726,
473.569579618888,473.646669858014,473.723397054735,473.800668815065,473.877940575394,
473.960532450875,474.042978969928,474.127356900436,474.209459716935,474.294975204449,
474.380490691962),.UNSPECIFIED.);
#406=B_SPLINE_CURVE_WITH_KNOTS('',3,(#45596,#45597,#45598,#45599,#45600,
#45601,#45602,#45603,#45604,#45605,#45606,#45607,#45608,#45609,#45610,#45611,
#45612,#45613,#45614,#45615,#45616,#45617,#45618,#45619,#45620,#45621,#45622,
#45623,#45624,#45625,#45626,#45627,#45628,#45629,#45630,#45631,#45632,#45633,
#45634,#45635,#45636,#45637,#45638,#45639,#45640,#45641,#45642,#45643,#45644,
#45645,#45646,#45647,#45648,#45649,#45650,#45651,#45652,#45653,#45654,#45655,
#45656,#45657,#45658,#45659,#45660,#45661,#45662,#45663,#45664,#45665,#45666,
#45667,#45668,#45669,#45670,#45671,#45672,#45673,#45674,#45675,#45676,#45677,
#45678,#45679,#45680,#45681,#45682,#45683,#45684,#45685,#45686,#45687,#45688,
#45689,#45690,#45691,#45692,#45693,#45694,#45695,#45696,#45697,#45698,#45699,
#45700,#45701,#45702,#45703,#45704,#45705,#45706,#45707,#45708,#45709,#45710,
#45711,#45712,#45713,#45714,#45715,#45716,#45717,#45718,#45719,#45720,#45721,
#45722,#45723,#45724,#45725,#45726,#45727,#45728,#45729,#45730,#45731,#45732,
#45733,#45734,#45735,#45736,#45737,#45738,#45739,#45740,#45741,#45742,#45743,
#45744,#45745,#45746,#45747,#45748,#45749,#45750,#45751,#45752,#45753,#45754,
#45755,#45756,#45757,#45758,#45759,#45760,#45761,#45762,#45763,#45764,#45765,
#45766,#45767),.UNSPECIFIED.,.F.,.F.,(4,3,3,3,3,3,3,3,3,3,3,3,3,3,3,3,3,
3,3,3,3,3,3,3,3,3,3,3,3,3,3,3,3,3,3,3,3,3,3,3,3,3,3,3,3,3,3,3,3,3,3,3,3,
3,3,3,3,4),(474.380490692059,474.460535231213,474.540649030064,474.624573918409,
474.704907259135,474.785320660555,474.865863059083,474.876348583445,474.957834908585,
475.03921700152,475.123300898008,475.204458226965,475.285539020607,475.366529022188,
475.37555258747,475.456565678807,475.53765435784,475.621929916254,475.703239366989,
475.784626252454,475.866133375462,475.874756591496,475.952284746877,476.029731624016,
476.107112804903,476.184443824544,476.261740181554,476.33903048406,476.416320393962,
476.493623918116,476.570955068389,476.648374560329,476.725839920858,476.803425309224,
476.873164599547,476.950027994422,477.026797836485,477.10349038275,477.18012182821,
477.256708319294,477.333566355332,477.410124688572,477.486689033502,477.563273956862,
477.640348619546,477.71705545051,477.794314029054,477.871572607598,477.949116904188,
478.02657129614,478.103935562688,478.181248091713,478.258522970496,478.335774262294,
478.413031632214,478.49029111365,478.567591847394,478.616565862282),
 .UNSPECIFIED.);
#407=B_SPLINE_CURVE_WITH_KNOTS('',3,(#45773,#45774,#45775,#45776,#45777,
#45778,#45779,#45780,#45781,#45782,#45783,#45784,#45785,#45786,#45787,#45788,
#45789,#45790,#45791,#45792,#45793,#45794,#45795,#45796,#45797,#45798,#45799,
#45800,#45801,#45802,#45803,#45804,#45805,#45806,#45807,#45808,#45809,#45810,
#45811,#45812,#45813,#45814,#45815,#45816,#45817,#45818,#45819,#45820,#45821,
#45822,#45823,#45824,#45825,#45826,#45827,#45828,#45829,#45830,#45831,#45832,
#45833,#45834,#45835,#45836,#45837,#45838,#45839,#45840,#45841,#45842,#45843,
#45844,#45845,#45846,#45847,#45848,#45849,#45850,#45851,#45852,#45853,#45854,
#45855,#45856,#45857,#45858,#45859,#45860,#45861,#45862,#45863,#45864,#45865,
#45866,#45867,#45868,#45869,#45870,#45871,#45872,#45873,#45874,#45875,#45876,
#45877,#45878,#45879,#45880,#45881,#45882,#45883,#45884,#45885,#45886,#45887,
#45888,#45889,#45890,#45891,#45892,#45893,#45894,#45895,#45896,#45897,#45898,
#45899,#45900,#45901,#45902,#45903,#45904,#45905,#45906,#45907,#45908,#45909,
#45910,#45911,#45912,#45913,#45914,#45915,#45916,#45917,#45918,#45919,#45920,
#45921,#45922,#45923,#45924,#45925,#45926,#45927,#45928,#45929,#45930,#45931,
#45932,#45933,#45934,#45935,#45936,#45937,#45938,#45939,#45940,#45941,#45942,
#45943,#45944),.UNSPECIFIED.,.F.,.F.,(4,3,3,3,3,3,3,3,3,3,3,3,3,3,3,3,3,
3,3,3,3,3,3,3,3,3,3,3,3,3,3,3,3,3,3,3,3,3,3,3,3,3,3,3,3,3,3,3,3,3,3,3,3,
3,3,3,3,4),(480.663675999238,480.684710626653,480.765718118816,480.846801459616,
480.931247952797,481.012553105523,481.09393596496,481.175439700502,481.184587432338,
481.262102728308,481.339536542789,481.416904472146,481.494222065579,481.571504835749,
481.648781424568,481.726057508624,481.803347107084,481.880664244083,481.958069955971,
482.035521471495,482.11309379188,482.184341043707,482.261191456613,482.33794809446,
482.414627225727,482.491245056489,482.567817743952,482.644852357843,482.721396552421,
482.797946658388,482.874517251629,482.951911602491,483.028604413594,483.106349534335,
483.184094655077,483.261610631392,483.339039282175,483.416396264486,483.493697183922,
483.57095760554,483.648203312351,483.725443317765,483.802691676646,483.879962445922,
483.957313960686,484.03470692534,484.112213865109,484.183848266446,484.261378360035,
484.341194605466,484.418541443881,484.495836336518,484.573093386162,484.650326671363,
484.727562409331,484.8048003573,484.882070368431,484.899908323481),
 .UNSPECIFIED.);
#408=B_SPLINE_CURVE_WITH_KNOTS('',3,(#45945,#45946,#45947,#45948,#45949,
#45950,#45951,#45952,#45953,#45954,#45955,#45956,#45957,#45958,#45959,#45960,
#45961,#45962,#45963,#45964,#45965,#45966,#45967,#45968,#45969,#45970,#45971,
#45972,#45973,#45974,#45975,#45976,#45977,#45978,#45979,#45980,#45981,#45982,
#45983,#45984,#45985,#45986,#45987,#45988,#45989,#45990,#45991,#45992,#45993,
#45994,#45995,#45996,#45997,#45998,#45999,#46000,#46001,#46002,#46003,#46004,
#46005,#46006,#46007,#46008,#46009,#46010,#46011,#46012,#46013,#46014,#46015,
#46016,#46017,#46018,#46019,#46020,#46021,#46022,#46023,#46024,#46025,#46026),
 .UNSPECIFIED.,.F.,.F.,(4,3,3,3,3,3,3,3,3,3,3,3,3,3,3,3,3,3,3,3,3,3,3,3,
3,3,3,4),(478.61726357937,478.693807784374,478.770356670326,478.846924814219,
478.923526802521,479.000219846047,479.07696535096,479.153821951485,479.185080209599,
479.262662623704,479.340152397017,479.417565166163,479.494916512606,479.572221973682,
479.64950436344,479.726775948689,479.804050748628,479.881342781611,479.958707260156,
480.036108676756,480.113616304678,480.184833820968,480.266932938396,480.348920644616,
480.430754232682,480.512494601567,480.594104446945,480.663675999104),
 .UNSPECIFIED.);
#409=B_SPLINE_CURVE_WITH_KNOTS('',3,(#46028,#46029,#46030,#46031,#46032,
#46033,#46034,#46035,#46036,#46037,#46038,#46039,#46040,#46041,#46042,#46043,
#46044,#46045,#46046,#46047,#46048,#46049,#46050,#46051,#46052,#46053,#46054,
#46055,#46056,#46057,#46058,#46059,#46060,#46061,#46062,#46063,#46064,#46065,
#46066,#46067,#46068,#46069,#46070,#46071,#46072,#46073,#46074,#46075,#46076,
#46077,#46078,#46079,#46080,#46081,#46082,#46083,#46084,#46085,#46086,#46087,
#46088,#46089,#46090,#46091,#46092,#46093,#46094,#46095,#46096,#46097,#46098,
#46099,#46100,#46101,#46102,#46103,#46104,#46105,#46106,#46107,#46108,#46109,
#46110,#46111,#46112),.UNSPECIFIED.,.F.,.F.,(4,3,3,3,3,3,3,3,3,3,3,3,3,
3,3,3,3,3,3,3,3,3,3,3,3,3,3,3,4),(478.616565862282,478.693957480818,478.771398631114,
478.848940229736,478.869980615649,478.947510740726,479.024953776917,479.102325365474,
479.179641096418,479.256916519409,479.334177401614,479.411432718986,479.488696512945,
479.565982827034,479.643349694059,479.720758093262,479.798279731107,479.8683886237,
479.944116203083,480.019754722875,480.095321134249,480.170827543791,480.246301274037,
480.321757502312,480.397211390023,480.472705398315,480.548221608717,480.623809108532,
480.662500463276),.UNSPECIFIED.);
#410=B_SPLINE_CURVE_WITH_KNOTS('',3,(#46113,#46114,#46115,#46116,#46117,
#46118,#46119,#46120,#46121,#46122,#46123,#46124,#46125,#46126,#46127,#46128,
#46129,#46130,#46131,#46132,#46133,#46134,#46135,#46136,#46137,#46138,#46139,
#46140,#46141,#46142,#46143,#46144,#46145,#46146,#46147,#46148,#46149,#46150,
#46151,#46152,#46153,#46154,#46155,#46156,#46157,#46158,#46159,#46160,#46161,
#46162,#46163,#46164,#46165,#46166,#46167,#46168,#46169,#46170,#46171,#46172,
#46173,#46174,#46175,#46176,#46177,#46178,#46179,#46180,#46181,#46182,#46183,
#46184,#46185,#46186,#46187,#46188,#46189,#46190,#46191,#46192,#46193,#46194,
#46195,#46196,#46197,#46198,#46199,#46200,#46201,#46202,#46203,#46204,#46205,
#46206,#46207,#46208,#46209,#46210,#46211,#46212,#46213,#46214,#46215,#46216,
#46217,#46218,#46219,#46220,#46221,#46222,#46223,#46224,#46225,#46226,#46227,
#46228,#46229,#46230,#46231,#46232,#46233,#46234,#46235,#46236,#46237,#46238,
#46239,#46240,#46241,#46242,#46243,#46244,#46245,#46246,#46247,#46248,#46249,
#46250,#46251,#46252,#46253,#46254,#46255,#46256,#46257,#46258,#46259,#46260,
#46261,#46262,#46263,#46264,#46265,#46266,#46267,#46268,#46269),
 .UNSPECIFIED.,.F.,.F.,(4,3,3,3,3,3,3,3,3,3,3,3,3,3,3,3,3,3,3,3,3,3,3,3,
3,3,3,3,3,3,3,3,3,3,3,3,3,3,3,3,3,3,3,3,3,3,3,3,3,3,3,3,4),(480.663675999238,
480.746138205274,480.828600063014,480.911061579308,480.993522761005,481.075983614956,
481.158444148011,481.240904367017,481.323364278825,481.405823890283,481.488283208239,
481.570742239541,481.653200991038,481.735659469576,481.818117682004,481.900575635168,
481.983033335916,482.065490791094,482.147948007548,482.23396023405,482.317284578474,
482.399751183919,482.482216945161,482.564681889613,482.647146044689,482.729609437798,
482.812072096347,482.894534047739,482.976995319378,483.059455938662,483.141915932989,
483.224375329753,483.306834156349,483.389292440165,483.471750208593,483.554207489018,
483.63834072443,483.720806722521,483.803271098877,483.885733963139,483.96819542493,
484.050655593851,484.133114579486,484.215572491404,484.301168336929,484.383633073529,
484.466094845531,484.548554091373,484.63101124935,484.713473767631,484.795931438486,
484.878390228437,484.900339255603),.UNSPECIFIED.);
#411=B_SPLINE_CURVE_WITH_KNOTS('',3,(#46275,#46276,#46277,#46278,#46279,
#46280,#46281,#46282,#46283,#46284,#46285,#46286,#46287,#46288,#46289,#46290,
#46291,#46292,#46293,#46294,#46295,#46296,#46297,#46298,#46299,#46300,#46301,
#46302,#46303,#46304,#46305,#46306,#46307,#46308,#46309,#46310,#46311,#46312,
#46313,#46314,#46315,#46316,#46317,#46318,#46319,#46320,#46321,#46322,#46323,
#46324,#46325,#46326,#46327,#46328,#46329,#46330,#46331,#46332,#46333,#46334,
#46335,#46336,#46337,#46338,#46339,#46340,#46341,#46342,#46343,#46344,#46345,
#46346,#46347,#46348,#46349,#46350,#46351,#46352,#46353,#46354,#46355,#46356,
#46357,#46358,#46359,#46360,#46361,#46362,#46363,#46364,#46365,#46366,#46367,
#46368,#46369,#46370,#46371,#46372,#46373,#46374,#46375,#46376,#46377,#46378,
#46379,#46380,#46381,#46382,#46383,#46384,#46385,#46386,#46387,#46388,#46389,
#46390,#46391,#46392,#46393,#46394,#46395,#46396,#46397,#46398,#46399,#46400,
#46401,#46402,#46403,#46404,#46405,#46406,#46407,#46408,#46409,#46410,#46411,
#46412,#46413,#46414,#46415,#46416,#46417,#46418,#46419,#46420,#46421,#46422,
#46423,#46424,#46425,#46426,#46427,#46428,#46429,#46430,#46431,#46432,#46433,
#46434,#46435,#46436,#46437,#46438,#46439,#46440,#46441,#46442,#46443,#46444,
#46445,#46446),.UNSPECIFIED.,.F.,.F.,(4,3,3,3,3,3,3,3,3,3,3,3,3,3,3,3,3,
3,3,3,3,3,3,3,3,3,3,3,3,3,3,3,3,3,3,3,3,3,3,3,3,3,3,3,3,3,3,3,3,3,3,3,3,
3,3,3,3,4),(486.946861306558,487.044487898057,487.143729854774,487.183109100554,
487.264573506176,487.345932819536,487.430196091212,487.511328644414,487.59238417966,
487.673348279245,487.682985906239,487.764098416933,487.845289914188,487.929683113621,
488.011102046416,488.092600239478,488.174220613748,488.182862711923,488.26023174493,
488.337518441393,488.414738542001,488.491907739137,488.569041687839,488.646169300824,
488.723296324374,488.800436904579,488.877605192613,488.954863121079,489.032167203152,
489.109594111933,489.182616323293,489.259647825886,489.336585302471,489.413444889173,
489.490242661691,489.566994648111,489.64391655893,489.720637692983,489.797363683864,
489.874108990205,489.951174226319,490.028037590024,490.105203762343,490.182369934662,
490.259996871395,490.337538182827,490.415009395564,490.492425986359,490.569803392715,
490.64716767186,490.724527198585,490.801895915988,490.879287769664,490.956760855184,
491.034275833432,491.111904375155,491.182123546032,491.183619892445),
 .UNSPECIFIED.);
#412=B_SPLINE_CURVE_WITH_KNOTS('',3,(#46447,#46448,#46449,#46450,#46451,
#46452,#46453,#46454,#46455,#46456,#46457,#46458,#46459,#46460,#46461,#46462,
#46463,#46464,#46465,#46466,#46467,#46468,#46469,#46470,#46471,#46472,#46473,
#46474,#46475,#46476,#46477,#46478,#46479,#46480,#46481,#46482,#46483,#46484,
#46485,#46486,#46487,#46488,#46489,#46490,#46491,#46492,#46493,#46494,#46495,
#46496,#46497,#46498,#46499,#46500,#46501,#46502,#46503,#46504,#46505,#46506,
#46507,#46508,#46509,#46510,#46511,#46512,#46513,#46514,#46515,#46516,#46517,
#46518,#46519,#46520,#46521,#46522,#46523,#46524,#46525,#46526,#46527,#46528),
 .UNSPECIFIED.,.F.,.F.,(4,3,3,3,3,3,3,3,3,3,3,3,3,3,3,3,3,3,3,3,3,3,3,3,
3,3,3,4),(484.899908323481,484.977267642619,485.054671733857,485.132184395316,
485.183601877815,485.260435582513,485.337180053993,485.41385153389,485.490466205502,
485.567040206957,485.644079617235,485.720636132414,485.797202697583,485.873793884144,
485.951184285404,486.027907737698,486.105631613442,486.183355489185,486.26034438458,
486.337238710065,486.414037400464,486.490781268223,486.567484870917,486.644162739328,
486.720847671068,486.797533478452,486.874268418715,486.946861306418),
 .UNSPECIFIED.);
#413=B_SPLINE_CURVE_WITH_KNOTS('',3,(#46530,#46531,#46532,#46533,#46534,
#46535,#46536,#46537,#46538,#46539,#46540,#46541,#46542,#46543,#46544,#46545,
#46546,#46547,#46548,#46549,#46550,#46551,#46552,#46553,#46554,#46555,#46556,
#46557,#46558,#46559,#46560,#46561,#46562,#46563,#46564,#46565,#46566,#46567,
#46568,#46569,#46570,#46571,#46572,#46573,#46574,#46575,#46576,#46577,#46578,
#46579,#46580,#46581,#46582,#46583,#46584,#46585,#46586,#46587,#46588,#46589,
#46590,#46591,#46592,#46593,#46594,#46595,#46596,#46597,#46598,#46599,#46600,
#46601,#46602,#46603,#46604,#46605),.UNSPECIFIED.,.F.,.F.,(4,3,3,3,3,3,
3,3,3,3,3,3,3,3,3,3,3,3,3,3,3,3,3,3,3,4),(484.900339255603,484.982800859457,
485.065261797427,485.147722096913,485.23018178531,485.312640890012,485.395099438411,
485.477557457898,485.560014975859,485.646692871519,485.729159657355,485.811624770699,
485.894088321204,485.976550418501,486.059011172203,486.1414706919,486.223929087168,
486.306386467565,486.388852853831,486.471316055845,486.553776512125,486.636234661036,
486.718700265915,486.80116014513,486.883624258494,486.946861306418),
 .UNSPECIFIED.);
#414=B_SPLINE_CURVE_WITH_KNOTS('',3,(#46606,#46607,#46608,#46609,#46610,
#46611,#46612,#46613,#46614,#46615,#46616,#46617,#46618,#46619,#46620,#46621,
#46622,#46623,#46624,#46625,#46626,#46627,#46628,#46629,#46630,#46631,#46632,
#46633,#46634,#46635,#46636,#46637,#46638,#46639,#46640,#46641,#46642,#46643,
#46644,#46645,#46646,#46647,#46648,#46649,#46650,#46651,#46652,#46653,#46654,
#46655,#46656,#46657,#46658,#46659,#46660,#46661,#46662,#46663,#46664,#46665,
#46666,#46667,#46668,#46669,#46670,#46671,#46672,#46673,#46674,#46675,#46676,
#46677,#46678,#46679,#46680,#46681,#46682,#46683,#46684,#46685,#46686,#46687,
#46688,#46689,#46690,#46691,#46692,#46693,#46694,#46695,#46696,#46697,#46698,
#46699,#46700,#46701,#46702,#46703,#46704,#46705,#46706,#46707,#46708,#46709,
#46710,#46711,#46712,#46713,#46714,#46715,#46716,#46717,#46718,#46719,#46720,
#46721,#46722,#46723,#46724,#46725,#46726,#46727,#46728,#46729,#46730,#46731,
#46732,#46733,#46734,#46735,#46736,#46737,#46738,#46739,#46740,#46741,#46742,
#46743,#46744,#46745,#46746,#46747,#46748,#46749,#46750,#46751,#46752,#46753,
#46754,#46755,#46756,#46757,#46758,#46759,#46760,#46761,#46762,#46763,#46764,
#46765,#46766,#46767,#46768,#46769,#46770,#46771,#46772,#46773,#46774),
 .UNSPECIFIED.,.F.,.F.,(4,3,3,3,3,3,3,3,3,3,3,3,3,3,3,3,3,3,3,3,3,3,3,3,
3,3,3,3,3,3,3,3,3,3,3,3,3,3,3,3,3,3,3,3,3,3,3,3,3,3,3,3,3,3,3,3,4),(486.947493603795,
487.023416751433,487.099259735571,487.175039333094,487.25077225503,487.326484557484,
487.402187752868,487.477896898353,487.553627054983,487.629439912187,487.705294636798,
487.781269679046,487.855652688107,487.933234538829,488.010724097938,488.088136999181,
488.1654888214,488.242795099555,488.320078763446,488.39735192979,488.474628616324,
488.551922840107,488.629289707096,488.70669378104,488.784203794078,488.854060696158,
488.935525654771,489.016885920646,489.10098061553,489.182115309453,489.263173304526,
489.344140380854,489.353264700183,489.434384302318,489.51558265585,489.599804167939,
489.681228944152,489.76684882418,489.852468704209,489.929849868594,490.00714889331,
490.084381506189,490.161563386952,490.238710178132,490.315850761355,490.392990868986,
490.470144636184,490.547326203241,490.624597185865,490.701914393361,490.779353655883,
490.85087671226,490.927942593232,491.004889365967,491.08176741454,491.158578222174,
491.184226656328),.UNSPECIFIED.);
#415=B_SPLINE_CURVE_WITH_KNOTS('',3,(#46777,#46778,#46779,#46780,#46781,
#46782,#46783,#46784,#46785,#46786,#46787,#46788,#46789,#46790,#46791,#46792,
#46793,#46794,#46795,#46796,#46797,#46798,#46799,#46800,#46801,#46802,#46803,
#46804,#46805,#46806,#46807,#46808,#46809,#46810,#46811,#46812,#46813,#46814,
#46815,#46816,#46817,#46818,#46819,#46820,#46821,#46822,#46823,#46824,#46825,
#46826,#46827,#46828,#46829,#46830,#46831,#46832,#46833,#46834,#46835,#46836,
#46837,#46838,#46839,#46840,#46841,#46842,#46843,#46844,#46845,#46846,#46847,
#46848,#46849,#46850,#46851,#46852,#46853,#46854,#46855,#46856,#46857,#46858),
 .UNSPECIFIED.,.F.,.F.,(4,3,3,3,3,3,3,3,3,3,3,3,3,3,3,3,3,3,3,3,3,3,3,3,
3,3,3,4),(491.184226656328,491.260981276608,491.337721764863,491.414457587017,
491.491203190154,491.567973024665,491.644823201061,491.721717208307,491.798719032839,
491.849284720311,491.926926082042,492.004482049841,492.081968133548,492.159399793344,
492.236792450328,492.314172138313,492.391547200536,492.468931565718,492.546339165133,
492.623827783714,492.701358365424,492.779001757603,492.847692728361,492.93409170758,
493.020099915774,493.10585418754,493.191201426576,493.230046613597),
 .UNSPECIFIED.);
#416=B_SPLINE_CURVE_WITH_KNOTS('',3,(#46860,#46861,#46862,#46863,#46864,
#46865,#46866,#46867,#46868,#46869,#46870,#46871,#46872,#46873,#46874,#46875,
#46876,#46877,#46878,#46879,#46880,#46881,#46882,#46883,#46884,#46885,#46886,
#46887,#46888,#46889,#46890,#46891,#46892,#46893,#46894,#46895,#46896,#46897,
#46898,#46899,#46900,#46901,#46902,#46903,#46904,#46905,#46906,#46907,#46908,
#46909,#46910,#46911,#46912,#46913,#46914,#46915,#46916,#46917,#46918,#46919,
#46920,#46921,#46922,#46923,#46924,#46925,#46926,#46927,#46928,#46929,#46930,
#46931,#46932,#46933,#46934,#46935,#46936,#46937,#46938,#46939,#46940,#46941),
 .UNSPECIFIED.,.F.,.F.,(4,3,3,3,3,3,3,3,3,3,3,3,3,3,3,3,3,3,3,3,3,3,3,3,
3,3,3,4),(493.230046613597,493.312509443594,493.394971559946,493.477432990057,
493.559893761326,493.64235390115,493.724813436927,493.807272396048,493.889730805905,
493.972188693888,494.054646087385,494.139999550714,494.222465923618,494.304930650447,
494.38739384085,494.469855604453,494.552316050861,494.634775289664,494.717233430432,
494.799690582719,494.882156161897,494.964618662462,495.047078522896,495.129536181529,
495.212000247102,495.294459009407,495.376920343153,495.420301500648),
 .UNSPECIFIED.);
#417=B_SPLINE_CURVE_WITH_KNOTS('',3,(#46945,#46946,#46947,#46948,#46949,
#46950,#46951,#46952,#46953,#46954,#46955,#46956,#46957,#46958,#46959,#46960,
#46961,#46962,#46963,#46964,#46965,#46966,#46967,#46968,#46969,#46970,#46971,
#46972,#46973,#46974,#46975,#46976,#46977,#46978,#46979,#46980,#46981),
 .UNSPECIFIED.,.F.,.F.,(4,3,3,3,3,3,3,3,3,3,3,3,4),(493.230046613687,493.306330725309,
493.382561304179,493.458756735131,493.534929937347,493.611114993347,493.681507574455,
493.771594988047,493.861949931434,493.952493420372,494.043038074755,494.133417017897,
494.18138438014),.UNSPECIFIED.);
#418=B_SPLINE_CURVE_WITH_KNOTS('',3,(#46982,#46983,#46984,#46985,#46986,
#46987,#46988,#46989,#46990,#46991,#46992,#46993,#46994,#46995,#46996,#46997,
#46998,#46999,#47000,#47001,#47002,#47003,#47004,#47005,#47006,#47007,#47008,
#47009,#47010,#47011,#47012,#47013,#47014,#47015,#47016,#47017,#47018,#47019,
#47020,#47021,#47022,#47023,#47024,#47025,#47026,#47027,#47028,#47029,#47030,
#47031,#47032,#47033,#47034,#47035,#47036,#47037,#47038,#47039,#47040,#47041,
#47042,#47043,#47044,#47045,#47046,#47047,#47048,#47049,#47050,#47051,#47052,
#47053,#47054,#47055,#47056,#47057,#47058,#47059,#47060,#47061,#47062,#47063),
 .UNSPECIFIED.,.F.,.F.,(4,3,3,3,3,3,3,3,3,3,3,3,3,3,3,3,3,3,3,3,3,3,3,3,
3,3,3,4),(491.183619892445,491.260274943168,491.336841384986,491.413335588533,
491.489773864164,491.566172475915,491.6431355611,491.719519875166,491.795915578857,
491.872337359501,491.949722308976,492.026280748062,492.104078952732,492.181877157401,
492.260273681847,492.338574297521,492.41679371464,492.494946586276,492.573047518285,
492.65111327471,492.729160503911,492.80720237782,492.885252062782,492.963355326503,
493.0414860081,493.119700448305,493.18163076877,493.230046613597),
 .UNSPECIFIED.);
#419=B_SPLINE_CURVE_WITH_KNOTS('',3,(#47067,#47068,#47069,#47070,#47071,
#47072,#47073,#47074),.UNSPECIFIED.,.F.,.F.,(4,2,2,4),(-4.092356615175,
-3.25801350823578,-2.42309659634093,-2.07498647268394),.UNSPECIFIED.);
#420=B_SPLINE_CURVE_WITH_KNOTS('',3,(#47078,#47079,#47080,#47081,#47082,
#47083,#47084,#47085,#47086,#47087,#47088,#47089,#47090,#47091,#47092,#47093,
#47094,#47095,#47096,#47097,#47098,#47099,#47100,#47101,#47102,#47103,#47104,
#47105,#47106,#47107,#47108,#47109,#47110,#47111,#47112,#47113,#47114,#47115,
#47116,#47117,#47118,#47119,#47120),.UNSPECIFIED.,.F.,.F.,(4,3,3,3,3,3,
3,3,3,3,3,3,3,3,4),(1.45814303507282E-15,0.0869025370684598,0.173949593837137,
0.261014425040484,0.347993527889018,0.434679052537863,0.499876805684693,
0.574356627358125,0.64882817249345,0.723303820461166,0.797823564118164,
0.87236646746495,0.946980958560742,0.999753611369385,1.12364870614456),
 .UNSPECIFIED.);
#421=B_SPLINE_CURVE_WITH_KNOTS('',3,(#47122,#47123,#47124,#47125,#47126,
#47127,#47128,#47129,#47130,#47131,#47132,#47133,#47134,#47135,#47136,#47137,
#47138,#47139,#47140,#47141,#47142,#47143,#47144,#47145,#47146,#47147,#47148,
#47149,#47150,#47151,#47152,#47153,#47154,#47155,#47156,#47157,#47158,#47159,
#47160,#47161,#47162,#47163,#47164,#47165,#47166,#47167,#47168,#47169,#47170,
#47171,#47172,#47173,#47174,#47175,#47176,#47177,#47178,#47179,#47180,#47181,
#47182,#47183,#47184,#47185,#47186,#47187,#47188,#47189,#47190,#47191,#47192,
#47193,#47194,#47195,#47196,#47197,#47198,#47199,#47200,#47201,#47202,#47203,
#47204,#47205,#47206,#47207,#47208,#47209,#47210,#47211,#47212,#47213,#47214,
#47215,#47216,#47217,#47218,#47219,#47220,#47221,#47222,#47223,#47224,#47225,
#47226,#47227,#47228,#47229,#47230,#47231,#47232,#47233,#47234,#47235,#47236,
#47237,#47238,#47239,#47240,#47241,#47242,#47243,#47244,#47245,#47246,#47247,
#47248,#47249,#47250,#47251,#47252,#47253,#47254,#47255,#47256,#47257,#47258,
#47259,#47260,#47261,#47262,#47263,#47264,#47265,#47266,#47267,#47268,#47269,
#47270,#47271,#47272,#47273,#47274,#47275,#47276,#47277,#47278,#47279,#47280,
#47281,#47282,#47283,#47284,#47285,#47286,#47287,#47288,#47289,#47290,#47291,
#47292,#47293,#47294,#47295,#47296,#47297,#47298,#47299,#47300,#47301,#47302,
#47303,#47304,#47305,#47306,#47307,#47308,#47309,#47310,#47311,#47312,#47313,
#47314,#47315,#47316,#47317,#47318,#47319,#47320,#47321,#47322,#47323,#47324,
#47325,#47326,#47327,#47328,#47329,#47330,#47331,#47332,#47333,#47334,#47335,
#47336,#47337,#47338,#47339,#47340,#47341,#47342,#47343,#47344,#47345,#47346,
#47347,#47348,#47349,#47350,#47351,#47352,#47353,#47354,#47355,#47356,#47357,
#47358,#47359,#47360,#47361,#47362,#47363,#47364,#47365,#47366,#47367,#47368,
#47369,#47370,#47371,#47372,#47373,#47374,#47375,#47376,#47377,#47378,#47379,
#47380,#47381,#47382,#47383),.UNSPECIFIED.,.F.,.F.,(4,3,3,3,3,3,3,3,3,3,
3,3,3,3,3,3,3,3,3,3,3,3,3,3,3,3,3,3,3,3,3,3,3,3,3,3,3,3,3,3,3,3,3,3,3,3,
3,3,3,3,3,3,3,3,3,3,3,3,3,3,3,3,3,3,3,3,3,3,3,3,3,3,3,3,3,3,3,3,3,3,3,3,
3,3,3,3,3,4),(1.12364870625865,1.19799676400753,1.27229201830982,1.3465483781602,
1.42077972594984,1.49501440487335,1.5692543466832,1.64351211019356,1.71780026139656,
1.7921745179453,1.86659479891783,1.94112608036292,1.99950722273875,2.07326886306519,
2.14694154485294,2.22053985865856,2.29407833719155,2.36757146738224,2.44103370143537,
2.51449117423725,2.5879495180571,2.6614217918124,2.73492106084282,2.80849966885792,
2.88212232271905,2.9558467552384,2.99926083410811,3.07392477490812,3.1485076667527,
3.22302332634866,3.29748552634202,3.37190800412445,3.44630447027535,3.52070089524939,
3.59510114765806,3.66951762969037,3.74396274972424,3.81848536363884,3.89305240626076,
3.96771417016438,3.99901444547747,4.07305531525637,4.14701541720727,4.22090907995211,
4.2947505848787,4.36855417637488,4.44233407140981,4.51611917832578,4.5899113847781,
4.66372355262109,4.73756855269211,4.81150023318393,4.8854806822806,4.95956736916572,
4.99876805684683,5.07323997833421,5.14762491351672,5.22193690173382,5.29618993338574,
5.37039795939829,5.44457490016529,5.51874487792235,5.59291439456977,5.66709603139468,
5.7413023738179,5.81558137441948,5.88990170993551,5.96431394950146,5.99852166821619,
6.07699584702591,6.1553719672994,6.23365495938674,6.31181720086211,6.38990543199449,
6.46790051375185,6.49839847390087,6.57628401760595,6.65423975186325,6.73227087791391,
6.81043242117976,6.88866516313746,6.96701851048475,6.99827527958555,7.07919527083627,
7.16110495645824,7.24163505948288,7.32423453640351,7.40683401332414),
 .UNSPECIFIED.);
#422=B_SPLINE_CURVE_WITH_KNOTS('',3,(#47385,#47386,#47387,#47388,#47389,
#47390,#47391,#47392,#47393,#47394,#47395,#47396,#47397,#47398,#47399,#47400,
#47401,#47402),.UNSPECIFIED.,.F.,.F.,(4,2,2,2,2,2,2,2,4),(7.40683401332414,
8.241750925219,9.07666783711385,9.91158474900871,10.7465016609036,11.5814185727984,
12.4163354846933,13.2512523965881,13.6900193205037),.UNSPECIFIED.);
#423=B_SPLINE_CURVE_WITH_KNOTS('',3,(#47404,#47405,#47406,#47407,#47408,
#47409,#47410,#47411,#47412,#47413,#47414,#47415,#47416,#47417,#47418,#47419,
#47420,#47421,#47422,#47423,#47424,#47425,#47426,#47427,#47428,#47429,#47430,
#47431,#47432,#47433,#47434,#47435,#47436,#47437,#47438,#47439,#47440,#47441,
#47442,#47443,#47444,#47445,#47446,#47447,#47448,#47449,#47450,#47451,#47452,
#47453,#47454,#47455,#47456,#47457,#47458,#47459,#47460,#47461,#47462,#47463,
#47464,#47465,#47466,#47467,#47468,#47469,#47470,#47471,#47472,#47473,#47474,
#47475,#47476,#47477,#47478,#47479,#47480,#47481,#47482,#47483,#47484,#47485,
#47486,#47487,#47488,#47489,#47490,#47491,#47492,#47493,#47494,#47495,#47496,
#47497,#47498,#47499,#47500,#47501,#47502,#47503,#47504,#47505,#47506,#47507,
#47508,#47509,#47510,#47511,#47512,#47513,#47514,#47515,#47516,#47517,#47518,
#47519,#47520,#47521,#47522,#47523,#47524,#47525,#47526,#47527,#47528,#47529,
#47530,#47531,#47532,#47533,#47534,#47535,#47536,#47537,#47538,#47539,#47540,
#47541,#47542,#47543,#47544,#47545,#47546,#47547,#47548,#47549,#47550,#47551,
#47552,#47553,#47554,#47555,#47556,#47557,#47558,#47559,#47560,#47561,#47562,
#47563,#47564,#47565,#47566,#47567,#47568,#47569,#47570,#47571,#47572,#47573,
#47574,#47575,#47576,#47577,#47578,#47579,#47580,#47581,#47582,#47583,#47584,
#47585,#47586,#47587,#47588,#47589,#47590,#47591,#47592,#47593,#47594,#47595,
#47596,#47597,#47598,#47599,#47600,#47601,#47602,#47603,#47604,#47605,#47606,
#47607,#47608,#47609,#47610,#47611,#47612,#47613,#47614,#47615,#47616,#47617,
#47618,#47619,#47620,#47621,#47622,#47623,#47624,#47625,#47626,#47627,#47628,
#47629,#47630,#47631,#47632,#47633,#47634,#47635,#47636,#47637,#47638,#47639,
#47640,#47641,#47642,#47643,#47644,#47645,#47646,#47647,#47648,#47649,#47650,
#47651,#47652,#47653,#47654,#47655,#47656,#47657,#47658,#47659,#47660,#47661,
#47662,#47663,#47664,#47665,#47666,#47667,#47668),.UNSPECIFIED.,.F.,.F.,
(4,3,3,3,3,3,3,3,3,3,3,3,3,3,3,3,3,3,3,3,3,3,3,3,3,3,3,3,3,3,3,3,3,3,3,
3,3,3,3,3,3,3,3,3,3,3,3,3,3,3,3,3,3,3,3,3,3,3,3,3,3,3,3,3,3,3,3,3,3,3,3,
3,3,3,3,3,3,3,3,3,3,3,3,3,3,3,3,3,4),(13.6900193205037,13.7765255706091,
13.8633932766764,13.9506752568707,13.9965505591712,14.0710975762786,14.1455689584512,
14.2199785786351,14.2943402690552,14.3686678299873,14.4429750381826,14.5172909187391,
14.591616066856,14.6659629543546,14.7403440621851,14.8148113990801,14.8893280793008,
14.963947418968,14.9963041705405,15.0702098251051,15.1440284619494,15.2177745535932,
15.291462518635,15.3651067329712,15.4387215401563,15.5123334218691,15.5859473338826,
15.6595762406573,15.7332331132438,15.8069700911002,15.880751806945,15.9546350665569,
15.9960577819099,16.0706066884839,16.1450745481074,16.2194752868081,16.2938227862065,
16.3681308925289,16.4424134252073,16.5166969310457,16.5909849118941,16.6652898684778,
16.739624308151,16.8140380543639,16.8884971160856,16.9630531267513,16.9958113932792,
17.070360098545,17.144827784559,17.2192283772757,17.293575758261,17.3678837737038,
17.442166243016,17.516449726734,17.5907377111628,17.6650426970596,17.7393771918239,
17.8137910318318,17.8882502095728,17.9628063694821,17.9955650046486,18.0694442284512,
18.1432406348715,18.2169686795501,18.2906427675944,18.3642772645184,18.4378865063978,
18.5114990681443,18.5851175300349,18.658754858199,18.7324240275983,18.8061791702291,
18.8799823888292,18.9538922452339,18.9953186160179,19.0696902346647,19.143976089157,
19.2181903048216,19.2923469582718,19.3664600870775,19.4422813918206,19.516359529082,
19.5904390461399,19.6645326051933,19.7416570851506,19.8158504501171,19.8900876218651,
19.9644090480309,19.9730305250225),.UNSPECIFIED.);
#424=B_SPLINE_CURVE_WITH_KNOTS('',3,(#47670,#47671,#47672,#47673,#47674,
#47675,#47676,#47677,#47678,#47679,#47680,#47681,#47682,#47683,#47684,#47685,
#47686,#47687),.UNSPECIFIED.,.F.,.F.,(4,2,2,2,2,2,2,2,4),(19.973267472803,
20.8081215395782,21.643038451473,22.4779553633679,23.3128722752627,24.1477891871576,
24.9827060990525,25.8176230109473,26.2563899348629),.UNSPECIFIED.);
#425=B_SPLINE_CURVE_WITH_KNOTS('',3,(#47689,#47690,#47691,#47692,#47693,
#47694,#47695,#47696,#47697,#47698,#47699,#47700,#47701,#47702,#47703,#47704,
#47705,#47706),.UNSPECIFIED.,.F.,.F.,(4,2,2,2,2,2,2,2,4),(26.2563899348629,
27.0913068467578,27.9262237586526,28.7611406705475,29.5960575824423,30.4309744943372,
31.265891406232,32.1008083181269,32.5395752420425),.UNSPECIFIED.);
#426=B_SPLINE_CURVE_WITH_KNOTS('',3,(#47708,#47709,#47710,#47711,#47712,
#47713,#47714,#47715,#47716,#47717,#47718),.UNSPECIFIED.,.F.,.F.,(4,1,1,
1,1,1,1,1,4),(32.5395752420425,32.9918691751891,33.9916227865585,34.4914995922432,
34.9913763979279,35.9911300092972,36.9908836206666,37.990637232036,38.8223131615157),
 .UNSPECIFIED.);
#427=B_SPLINE_CURVE_WITH_KNOTS('',3,(#47720,#47721,#47722,#47723,#47724,
#47725,#47726,#47727,#47728,#47729,#47730,#47731,#47732,#47733,#47734,#47735,
#47736,#47737),.UNSPECIFIED.,.F.,.F.,(4,2,2,2,2,2,2,2,4),(38.8230221691357,
39.6576774611169,40.4925943730118,41.3275112849067,42.1624281968015,42.9973451086964,
43.8322620205912,44.6671789324861,45.105699052741),.UNSPECIFIED.);
#428=B_SPLINE_CURVE_WITH_KNOTS('',3,(#47739,#47740,#47741,#47742,#47743,
#47744,#47745,#47746,#47747,#47748,#47749),.UNSPECIFIED.,.F.,.F.,(4,1,1,
1,1,1,1,1,4),(45.1063437169403,45.9886661229909,46.9884197343603,47.9881733457296,
48.4880501514143,48.987926957099,49.9876805684683,50.9874341798377,51.3891311635813),
 .UNSPECIFIED.);
#429=B_SPLINE_CURVE_WITH_KNOTS('',3,(#47751,#47752,#47753,#47754,#47755,
#47756,#47757,#47758,#47759,#47760,#47761,#47762,#47763,#47764,#47765,#47766,
#47767,#47768),.UNSPECIFIED.,.F.,.F.,(4,2,2,2,2,2,2,2,4),(51.3891311635813,
52.2240480754761,53.058964987371,53.8938818992658,54.7287988111607,55.5637157230555,
56.3986326349504,57.2335495468452,57.6723164707609),.UNSPECIFIED.);
#430=B_SPLINE_CURVE_WITH_KNOTS('',3,(#47770,#47771,#47772,#47773,#47774,
#47775,#47776,#47777,#47778,#47779,#47780,#47781,#47782,#47783,#47784,#47785,
#47786,#47787),.UNSPECIFIED.,.F.,.F.,(4,2,2,2,2,2,2,2,4),(57.6723164707609,
58.5072333826557,59.3421502945506,60.1770672064454,61.0119841183403,61.8469010302351,
62.68181794213,63.5167348540249,63.9555017779405),.UNSPECIFIED.);
#431=B_SPLINE_CURVE_WITH_KNOTS('',3,(#47789,#47790,#47791,#47792,#47793,
#47794,#47795,#47796,#47797,#47798,#47799,#47800,#47801,#47802,#47803,#47804,
#47805,#47806),.UNSPECIFIED.,.F.,.F.,(4,2,2,2,2,2,2,2,4),(63.9555017779405,
64.7904186898353,65.6253356017302,66.4602525136251,67.29516942552,68.1300863374149,
68.9650032493097,69.7999201612046,70.23868708512),.UNSPECIFIED.);
#432=B_SPLINE_CURVE_WITH_KNOTS('',3,(#47808,#47809,#47810,#47811,#47812,
#47813,#47814,#47815,#47816,#47817,#47818,#47819,#47820,#47821,#47822,#47823,
#47824,#47825),.UNSPECIFIED.,.F.,.F.,(4,2,2,2,2,2,2,2,4),(70.23868708512,
71.0736039970149,71.9085209089098,72.7434378208046,73.5783547326995,74.4132716445944,
75.2481885564892,76.0831054683841,76.5218723922996),.UNSPECIFIED.);
#433=B_SPLINE_CURVE_WITH_KNOTS('',3,(#47827,#47828,#47829,#47830,#47831,
#47832,#47833,#47834,#47835,#47836),.UNSPECIFIED.,.F.,.F.,(4,1,1,1,1,1,
1,4),(76.5218723922996,76.9810280754412,77.9807816868106,78.98053529818,
79.9802889095494,80.9800425209187,81.9797961322881,82.8044636853364),
 .UNSPECIFIED.);
#434=B_SPLINE_CURVE_WITH_KNOTS('',3,(#47838,#47839,#47840,#47841,#47842,
#47843,#47844,#47845,#47846,#47847,#47848,#47849,#47850,#47851,#47852,#47853,
#47854,#47855),.UNSPECIFIED.,.F.,.F.,(4,2,2,2,2,2,2,2,4),(82.8052344214521,
83.6399746113741,84.474891523269,85.3098084351638,86.1447253470587,86.9796422589535,
87.8145591708484,88.6494760827433,89.088071555534),.UNSPECIFIED.);
#435=B_SPLINE_CURVE_WITH_KNOTS('',3,(#47857,#47858,#47859,#47860,#47861,
#47862,#47863,#47864,#47865,#47866,#47867,#47868,#47869,#47870,#47871,#47872,
#47873,#47874,#47875,#47876,#47877,#47878,#47879,#47880,#47881,#47882,#47883,
#47884,#47885,#47886,#47887,#47888,#47889,#47890,#47891,#47892,#47893,#47894,
#47895,#47896,#47897,#47898,#47899,#47900,#47901,#47902,#47903,#47904,#47905,
#47906,#47907,#47908,#47909,#47910,#47911,#47912,#47913,#47914,#47915,#47916,
#47917,#47918,#47919,#47920,#47921,#47922,#47923,#47924,#47925,#47926,#47927,
#47928,#47929,#47930,#47931,#47932,#47933,#47934,#47935,#47936,#47937,#47938,
#47939,#47940,#47941,#47942,#47943,#47944,#47945,#47946,#47947,#47948,#47949,
#47950,#47951,#47952,#47953,#47954,#47955,#47956,#47957,#47958,#47959,#47960,
#47961,#47962,#47963,#47964,#47965,#47966,#47967,#47968,#47969,#47970,#47971,
#47972,#47973,#47974,#47975,#47976,#47977,#47978,#47979,#47980,#47981,#47982,
#47983,#47984,#47985,#47986,#47987,#47988,#47989,#47990,#47991,#47992,#47993,
#47994,#47995,#47996,#47997,#47998,#47999,#48000,#48001,#48002,#48003,#48004,
#48005,#48006,#48007,#48008,#48009,#48010,#48011,#48012,#48013,#48014,#48015,
#48016,#48017,#48018,#48019,#48020,#48021,#48022,#48023,#48024,#48025,#48026,
#48027,#48028,#48029,#48030,#48031,#48032,#48033,#48034,#48035,#48036,#48037,
#48038,#48039,#48040,#48041,#48042,#48043,#48044,#48045,#48046,#48047,#48048,
#48049,#48050,#48051,#48052,#48053,#48054,#48055,#48056,#48057,#48058,#48059,
#48060,#48061,#48062,#48063,#48064,#48065,#48066,#48067,#48068,#48069,#48070,
#48071,#48072,#48073,#48074,#48075,#48076,#48077,#48078,#48079,#48080,#48081,
#48082,#48083,#48084,#48085,#48086,#48087,#48088,#48089,#48090,#48091,#48092,
#48093,#48094,#48095,#48096,#48097,#48098,#48099,#48100,#48101,#48102,#48103,
#48104,#48105,#48106,#48107,#48108,#48109,#48110,#48111,#48112,#48113,#48114,
#48115,#48116,#48117,#48118),.UNSPECIFIED.,.F.,.F.,(4,3,3,3,3,3,3,3,3,3,
3,3,3,3,3,3,3,3,3,3,3,3,3,3,3,3,3,3,3,3,3,3,3,3,3,3,3,3,3,3,3,3,3,3,3,3,
3,3,3,3,3,3,3,3,3,3,3,3,3,3,3,3,3,3,3,3,3,3,3,3,3,3,3,3,3,3,3,3,3,3,3,3,
3,3,3,3,3,4),(89.0885712435139,89.1619820578451,89.2353150691934,89.3085850276093,
89.3818066297448,89.456308928932,89.5294867054481,89.6026631980976,89.6758516412752,
89.7513449867672,89.8246300636465,89.9012275434448,89.977825023243,90.0561884454774,
90.1344550144504,90.2126300235391,90.2906873249174,90.3686726422253,90.4465682640788,
90.4777018289277,90.5556078870461,90.63358400619,90.7116353212181,90.7898165900036,
90.8680687618362,90.9464409348866,90.9775786346124,91.0521258301107,91.1265973938455,
91.2010071985689,91.2753690763153,91.3496968271721,91.4240042277022,91.4983203035823,
91.5726456488703,91.6469927352241,91.7213740434306,91.7958415820151,91.8703584649683,
91.9449780072942,91.9773322459818,92.0512378361067,92.1250564079675,92.1988024341337,
92.2724903332518,92.3461344812655,92.4197492217753,92.4933610364573,92.5669748812107,
92.6406037205372,92.7142605255286,92.7879974358707,92.8617790841371,92.93566227663,
92.9770858573511,93.0516347582909,93.1261026120739,93.2005033447333,93.2748508378962,
93.3491589377945,93.4234414638657,93.4977249628424,93.5720129366706,93.6463178860809,
93.7206523184315,93.7950660571295,93.8695251112157,93.9440811141211,93.9768394687205,
94.0513881942245,94.1258559007383,94.2002565141958,94.2746039161441,94.3489119527517,
94.4231944434118,94.4974779486874,94.5717659548025,94.6460709624977,94.7204054791555,
94.7948193410972,94.8692785408261,94.9438347226313,94.9765930800899,95.0589235913551,
95.1409198345418,95.2227089608825,95.3041468250003,95.3714283138384),
 .UNSPECIFIED.);
#436=B_SPLINE_CURVE_WITH_KNOTS('',3,(#48120,#48121,#48122,#48123,#48124,
#48125,#48126,#48127,#48128,#48129,#48130,#48131,#48132,#48133,#48134,#48135,
#48136,#48137),.UNSPECIFIED.,.F.,.F.,(4,2,2,2,2,2,2,2,4),(95.3714283138384,
96.2063452257333,97.0412621376282,97.876179049523,98.7110959614179,99.5460128733127,
100.380929785208,101.215846697102,101.654613621018),.UNSPECIFIED.);
#437=B_SPLINE_CURVE_WITH_KNOTS('',3,(#48139,#48140,#48141,#48142,#48143,
#48144,#48145,#48146,#48147,#48148,#48149,#48150,#48151,#48152,#48153,#48154,
#48155,#48156,#48157,#48158,#48159,#48160,#48161,#48162,#48163,#48164,#48165,
#48166,#48167,#48168,#48169,#48170,#48171,#48172,#48173,#48174,#48175,#48176,
#48177,#48178,#48179,#48180,#48181,#48182,#48183,#48184,#48185,#48186,#48187,
#48188,#48189,#48190,#48191,#48192,#48193,#48194,#48195,#48196,#48197,#48198,
#48199,#48200,#48201,#48202,#48203,#48204,#48205,#48206,#48207,#48208,#48209,
#48210,#48211,#48212,#48213,#48214,#48215,#48216,#48217,#48218,#48219,#48220,
#48221,#48222,#48223,#48224,#48225,#48226,#48227,#48228,#48229,#48230,#48231,
#48232,#48233,#48234,#48235,#48236,#48237,#48238,#48239,#48240,#48241,#48242,
#48243,#48244,#48245,#48246,#48247,#48248,#48249,#48250,#48251,#48252,#48253,
#48254,#48255,#48256,#48257,#48258,#48259,#48260,#48261,#48262,#48263,#48264,
#48265,#48266,#48267,#48268,#48269,#48270,#48271,#48272,#48273,#48274,#48275,
#48276,#48277,#48278,#48279,#48280,#48281,#48282,#48283,#48284,#48285,#48286,
#48287,#48288,#48289,#48290,#48291,#48292,#48293,#48294,#48295,#48296,#48297,
#48298,#48299,#48300,#48301,#48302,#48303,#48304,#48305,#48306,#48307,#48308,
#48309,#48310,#48311,#48312,#48313,#48314,#48315,#48316,#48317,#48318,#48319,
#48320,#48321,#48322,#48323,#48324,#48325,#48326,#48327,#48328,#48329,#48330,
#48331,#48332,#48333,#48334,#48335,#48336,#48337,#48338,#48339,#48340,#48341,
#48342,#48343,#48344,#48345,#48346,#48347,#48348,#48349,#48350,#48351,#48352,
#48353,#48354,#48355,#48356,#48357,#48358,#48359,#48360,#48361,#48362,#48363,
#48364,#48365,#48366,#48367,#48368,#48369,#48370,#48371,#48372,#48373,#48374,
#48375,#48376,#48377,#48378,#48379,#48380,#48381,#48382,#48383,#48384,#48385,
#48386,#48387,#48388,#48389,#48390,#48391,#48392,#48393,#48394,#48395,#48396,
#48397,#48398,#48399,#48400),.UNSPECIFIED.,.F.,.F.,(4,3,3,3,3,3,3,3,3,3,
3,3,3,3,3,3,3,3,3,3,3,3,3,3,3,3,3,3,3,3,3,3,3,3,3,3,3,3,3,3,3,3,3,3,3,3,
3,3,3,3,3,3,3,3,3,3,3,3,3,3,3,3,3,3,3,3,3,3,3,3,3,3,3,3,3,3,3,3,3,3,3,3,
3,3,3,3,3,4),(101.654613621018,101.743105911189,101.832203522192,101.922010479699,
101.974868359675,102.048747574089,102.122543971047,102.196272006199,102.269946084656,
102.343580571941,102.417189804136,102.490802356154,102.564420808288,102.638058126672,
102.711727286275,102.785482419128,102.859285627944,102.933195474639,102.974621971045,
103.049233451952,103.123758975888,103.198212451839,103.272607741207,103.346958666929,
103.42127902215,103.495592766087,103.569906252374,103.644231949046,103.718582328249,
103.793004671757,103.867468148569,103.942022108588,103.974375582414,104.052739004648,
104.131005573621,104.209180582708,104.287237884086,104.365223201394,104.443118823247,
104.474252388099,104.552158446218,104.630134565364,104.708185880393,104.786367149179,
104.864619321013,104.942991494064,104.974129193784,105.048676389282,105.123147953016,
105.19755775774,105.271919635486,105.346247386342,105.420554786872,105.494870862752,
105.56919620804,105.643543294394,105.7179246026,105.792392141185,105.866909024138,
105.941528566463,105.973882805153,106.047788395278,106.121606967139,106.195352993305,
106.269040892423,106.342685040436,106.416299780946,106.489911595628,106.563525440381,
106.637154279708,106.710811084699,106.784547995041,106.858329643307,106.9322128358,
106.973636416522,107.047773512522,107.121829677063,107.195819190245,107.269756285376,
107.343655159005,107.417923130154,107.491800560376,107.565684533812,107.639587867914,
107.714140632985,107.788154539542,107.86297673387,107.937798928198),
 .UNSPECIFIED.);
#438=B_SPLINE_CURVE_WITH_KNOTS('',3,(#48402,#48403,#48404,#48405,#48406,
#48407,#48408,#48409,#48410,#48411,#48412,#48413,#48414),.UNSPECIFIED.,
 .F.,.F.,(4,2,1,1,1,1,1,1,1,4),(107.937798928198,107.973390027892,108.973143639261,
109.97289725063,110.972650862,111.472527667684,111.972404473369,112.972158084738,
113.971911696108,114.220984235377),.UNSPECIFIED.);
#439=B_SPLINE_CURVE_WITH_KNOTS('',3,(#48416,#48417,#48418,#48419,#48420,
#48421,#48422,#48423,#48424,#48425,#48426,#48427,#48428,#48429,#48430,#48431,
#48432,#48433),.UNSPECIFIED.,.F.,.F.,(4,2,2,2,2,2,2,2,4),(114.220984235377,
115.055901147272,115.890818059167,116.725734971062,117.560651882957,118.395568794852,
119.230485706746,120.065402618641,120.504169542557),.UNSPECIFIED.);
#440=B_SPLINE_CURVE_WITH_KNOTS('',3,(#48435,#48436,#48437,#48438,#48439,
#48440,#48441,#48442,#48443,#48444,#48445,#48446,#48447,#48448,#48449,#48450,
#48451,#48452),.UNSPECIFIED.,.F.,.F.,(4,2,2,2,2,2,2,2,4),(120.504169542557,
121.339086454452,122.174003366346,123.008920278241,123.843837190136,124.678754102031,
125.513671013926,126.348587925821,126.787354849736),.UNSPECIFIED.);
#441=B_SPLINE_CURVE_WITH_KNOTS('',3,(#48454,#48455,#48456,#48457,#48458,
#48459,#48460,#48461,#48462,#48463,#48464,#48465,#48466,#48467,#48468,#48469,
#48470,#48471),.UNSPECIFIED.,.F.,.F.,(4,2,2,2,2,2,2,2,4),(126.787354849736,
127.622271761631,128.457188673526,129.292105585421,130.127022497316,130.961939409211,
131.796856321106,132.631773233001,133.070254297904),.UNSPECIFIED.);
#442=B_SPLINE_CURVE_WITH_KNOTS('',3,(#48473,#48474,#48475,#48476,#48477,
#48478,#48479,#48480,#48481,#48482,#48483,#48484,#48485,#48486,#48487,#48488,
#48489,#48490,#48491,#48492,#48493,#48494,#48495,#48496,#48497,#48498,#48499,
#48500,#48501,#48502,#48503,#48504,#48505,#48506,#48507,#48508,#48509,#48510,
#48511,#48512,#48513,#48514,#48515,#48516,#48517,#48518,#48519,#48520,#48521,
#48522,#48523,#48524,#48525,#48526,#48527,#48528,#48529,#48530,#48531,#48532,
#48533,#48534,#48535,#48536,#48537,#48538,#48539,#48540,#48541,#48542,#48543,
#48544,#48545,#48546,#48547,#48548,#48549,#48550,#48551,#48552,#48553,#48554,
#48555,#48556,#48557,#48558,#48559,#48560,#48561,#48562,#48563,#48564,#48565,
#48566,#48567,#48568,#48569,#48570,#48571,#48572,#48573,#48574,#48575,#48576,
#48577,#48578,#48579,#48580,#48581,#48582,#48583,#48584,#48585,#48586,#48587,
#48588,#48589,#48590,#48591,#48592,#48593,#48594,#48595,#48596,#48597,#48598,
#48599,#48600,#48601,#48602,#48603,#48604,#48605,#48606,#48607,#48608,#48609,
#48610,#48611,#48612,#48613,#48614,#48615,#48616,#48617,#48618,#48619,#48620,
#48621,#48622,#48623,#48624,#48625,#48626,#48627,#48628,#48629,#48630,#48631,
#48632,#48633,#48634,#48635,#48636,#48637,#48638,#48639,#48640,#48641,#48642,
#48643,#48644,#48645,#48646,#48647,#48648,#48649,#48650,#48651,#48652,#48653,
#48654,#48655,#48656,#48657,#48658,#48659,#48660,#48661,#48662,#48663,#48664,
#48665,#48666,#48667,#48668,#48669,#48670,#48671,#48672,#48673,#48674,#48675,
#48676,#48677,#48678,#48679,#48680,#48681,#48682,#48683,#48684,#48685,#48686,
#48687,#48688,#48689,#48690,#48691,#48692,#48693,#48694,#48695,#48696,#48697,
#48698,#48699,#48700,#48701,#48702,#48703,#48704,#48705,#48706,#48707,#48708,
#48709,#48710,#48711,#48712,#48713,#48714,#48715,#48716,#48717,#48718,#48719,
#48720,#48721,#48722,#48723,#48724,#48725,#48726,#48727,#48728,#48729,#48730,
#48731,#48732,#48733,#48734,#48735,#48736,#48737),.UNSPECIFIED.,.F.,.F.,
(4,3,3,3,3,3,3,3,3,3,3,3,3,3,3,3,3,3,3,3,3,3,3,3,3,3,3,3,3,3,3,3,3,3,3,
3,3,3,3,3,3,3,3,3,3,3,3,3,3,3,3,3,3,3,3,3,3,3,3,3,3,3,3,3,3,3,3,3,3,3,3,
3,3,3,3,3,3,3,3,3,3,3,3,3,3,3,3,3,4),(133.070847371309,133.144566118881,
133.218218486221,133.291818954969,133.365381967648,133.440582212129,133.51412749122,
133.587681041332,133.661255902816,133.737687907986,133.811382350179,133.885127816936,
133.958967914573,133.966983923495,134.04088951362,134.114708085481,134.188454111648,
134.262142010766,134.33578615878,134.40940089929,134.483012713973,134.556626558726,
134.630255398053,134.703912203045,134.777649113387,134.851430761653,134.925313954147,
134.966737534865,135.041286435805,135.115754289588,135.190155022248,135.264502515411,
135.338810615309,135.413093141381,135.487376640357,135.561664614186,135.635969563595,
135.710303995946,135.784717734645,135.859176788731,135.933732791636,135.966491146234,
136.041039871738,136.115507578251,136.189908191709,136.264255593657,136.338563630264,
136.412846120925,136.4871296262,136.561417632315,136.63572264001,136.710057156668,
136.784471018609,136.858930218338,136.933486400143,136.966244757603,137.040123972016,
137.113920368974,137.187648404125,137.261322482583,137.334956969868,137.408566202062,
137.48217875408,137.555797206213,137.629434524597,137.703103684199,137.776858817052,
137.850662025868,137.924571872562,137.965998368973,138.04060984988,138.115135373816,
138.189588849767,138.263984139136,138.338335064857,138.412655420078,138.486969164016,
138.561282650302,138.635608346975,138.709958726178,138.784381069686,138.858844546498,
138.933398506517,138.965751980342,139.048167245346,139.130346340956,139.212370217371,
139.294128390232,139.353725464096),.UNSPECIFIED.);
#443=B_SPLINE_CURVE_WITH_KNOTS('',3,(#48739,#48740,#48741,#48742,#48743,
#48744,#48745,#48746,#48747,#48748,#48749,#48750,#48751,#48752,#48753,#48754,
#48755,#48756),.UNSPECIFIED.,.F.,.F.,(4,2,2,2,2,2,2,2,4),(139.353725464096,
140.18864237599,141.023559287885,141.85847619978,142.693393111675,143.52831002357,
144.363226935464,145.198143847359,145.636910771275),.UNSPECIFIED.);
#444=B_SPLINE_CURVE_WITH_KNOTS('',3,(#48758,#48759,#48760,#48761,#48762,
#48763,#48764,#48765,#48766,#48767,#48768),.UNSPECIFIED.,.F.,.F.,(4,1,1,
1,1,1,1,1,4),(145.636910771275,145.964027259928,146.463904065612,146.963780871297,
147.963534482666,148.963288094036,149.963041705405,150.962795316774,151.919720738554),
 .UNSPECIFIED.);
#445=B_SPLINE_CURVE_WITH_KNOTS('',3,(#48770,#48771,#48772,#48773,#48774,
#48775,#48776,#48777,#48778,#48779,#48780,#48781,#48782,#48783,#48784,#48785,
#48786,#48787),.UNSPECIFIED.,.F.,.F.,(4,2,2,2,2,2,2,2,4),(151.920234954538,
152.75501299035,153.589929902244,154.424846814139,155.259763726034,156.094680637929,
156.929597549824,157.764514461719,158.203281385634),.UNSPECIFIED.);
#446=B_SPLINE_CURVE_WITH_KNOTS('',3,(#48789,#48790,#48791,#48792,#48793,
#48794,#48795,#48796,#48797,#48798,#48799,#48800,#48801,#48802,#48803,#48804,
#48805,#48806),.UNSPECIFIED.,.F.,.F.,(4,2,2,2,2,2,2,2,4),(158.203281385634,
159.038198297529,159.873115209424,160.708032121319,161.542949033214,162.377865945108,
163.212782857003,164.047699768898,164.486466692814),.UNSPECIFIED.);
#447=B_SPLINE_CURVE_WITH_KNOTS('',3,(#48808,#48809,#48810,#48811,#48812,
#48813,#48814,#48815,#48816,#48817,#48818),.UNSPECIFIED.,.F.,.F.,(4,1,1,
1,1,1,1,1,4),(164.486466692814,164.959345875946,165.959099487315,166.958853098684,
167.458729904369,167.958606710054,168.958360321423,169.958113932792,170.769651999993),
 .UNSPECIFIED.);
#448=B_SPLINE_CURVE_WITH_KNOTS('',3,(#48820,#48821,#48822,#48823,#48824,
#48825,#48826,#48827,#48828,#48829,#48830,#48831),.UNSPECIFIED.,.F.,.F.,
(4,1,1,1,1,1,1,1,1,4),(170.769651999993,170.957867544162,171.957621155531,
172.957374766901,173.95712837827,174.457005183955,174.956881989639,175.956635601009,
176.956389212378,177.052837307173),.UNSPECIFIED.);
#449=B_SPLINE_CURVE_WITH_KNOTS('',3,(#48833,#48834,#48835,#48836,#48837,
#48838,#48839,#48840,#48841,#48842,#48843,#48844,#48845,#48846,#48847,#48848,
#48849,#48850,#48851,#48852,#48853,#48854,#48855,#48856,#48857,#48858,#48859,
#48860,#48861,#48862,#48863,#48864,#48865,#48866,#48867,#48868,#48869,#48870,
#48871,#48872,#48873,#48874,#48875,#48876,#48877,#48878,#48879,#48880,#48881,
#48882,#48883,#48884,#48885,#48886,#48887,#48888,#48889,#48890,#48891,#48892,
#48893,#48894,#48895,#48896,#48897,#48898,#48899,#48900,#48901,#48902,#48903,
#48904,#48905,#48906,#48907,#48908,#48909,#48910,#48911,#48912,#48913,#48914,
#48915,#48916,#48917,#48918,#48919,#48920,#48921,#48922,#48923,#48924,#48925,
#48926,#48927,#48928,#48929,#48930,#48931,#48932,#48933,#48934,#48935,#48936,
#48937,#48938,#48939,#48940,#48941,#48942,#48943,#48944,#48945,#48946,#48947,
#48948,#48949,#48950,#48951,#48952,#48953,#48954,#48955,#48956,#48957,#48958,
#48959,#48960,#48961,#48962,#48963,#48964,#48965,#48966,#48967,#48968,#48969,
#48970,#48971,#48972,#48973,#48974,#48975,#48976,#48977,#48978,#48979,#48980,
#48981,#48982,#48983,#48984,#48985,#48986,#48987,#48988,#48989,#48990,#48991,
#48992,#48993,#48994,#48995,#48996,#48997,#48998,#48999,#49000,#49001,#49002,
#49003,#49004,#49005,#49006,#49007,#49008,#49009,#49010,#49011,#49012,#49013,
#49014,#49015,#49016,#49017,#49018,#49019,#49020,#49021,#49022,#49023,#49024,
#49025,#49026,#49027,#49028,#49029,#49030,#49031,#49032,#49033,#49034,#49035,
#49036,#49037,#49038,#49039,#49040,#49041,#49042,#49043,#49044,#49045,#49046,
#49047,#49048,#49049,#49050,#49051,#49052,#49053,#49054,#49055,#49056,#49057,
#49058,#49059,#49060,#49061,#49062,#49063,#49064,#49065,#49066,#49067,#49068,
#49069,#49070,#49071,#49072,#49073,#49074,#49075,#49076,#49077,#49078,#49079,
#49080,#49081,#49082,#49083,#49084,#49085,#49086,#49087,#49088,#49089,#49090,
#49091,#49092,#49093,#49094,#49095,#49096,#49097),.UNSPECIFIED.,.F.,.F.,
(4,3,3,3,3,3,3,3,3,3,3,3,3,3,3,3,3,3,3,3,3,3,3,3,3,3,3,3,3,3,3,3,3,3,3,
3,3,3,3,3,3,3,3,3,3,3,3,3,3,3,3,3,3,3,3,3,3,3,3,3,3,3,3,3,3,3,3,3,3,3,3,
3,3,3,3,3,3,3,3,3,3,3,3,3,3,3,3,3,4),(177.052837307173,177.126386915977,
177.199862112356,177.273277544079,177.346647810911,177.422834687515,177.496169099228,
177.569505281043,177.642856392112,177.716235599099,177.789691194626,177.863192111524,
177.936785246187,177.956142823747,178.030691549251,178.105159255765,178.179559869223,
178.253907271172,178.32821530778,178.40249779844,178.476781303716,178.551069309832,
178.625374317527,178.699708834184,178.774122696126,178.848581895855,178.923138077661,
178.955896435117,179.02977564953,179.103572046488,179.177300081639,179.250974160096,
179.324608647381,179.398217879575,179.471830431593,179.545448883726,179.61908620211,
179.692755361712,179.766510494565,179.840313703381,179.914223550075,179.955650046486,
180.030261527392,180.104787051329,180.17924052728,180.253635816648,180.32798674237,
180.402307097591,180.476620841528,180.550934327815,180.625260024487,180.699610403689,
180.774032747197,180.848496224009,180.923050184028,180.955403657855,181.03376708009,
181.112033649062,181.190208658151,181.268265959529,181.346251276837,181.424146898691,
181.45528046354,181.533186521659,181.611162640805,181.689213955835,181.767395224621,
181.845647396454,181.924019569505,181.955157269225,182.029704464723,182.104176028457,
182.17858583318,182.252947710927,182.327275461783,182.401582862314,182.475898938194,
182.550224283482,182.624571369835,182.698952678042,182.773420216626,182.847937099579,
182.922556641905,182.954910880594,183.038351025582,183.121389391934,183.204171436094,
183.286528896845,183.336022614352),.UNSPECIFIED.);
#450=B_SPLINE_CURVE_WITH_KNOTS('',3,(#49099,#49100,#49101,#49102,#49103,
#49104,#49105,#49106,#49107,#49108,#49109,#49110,#49111,#49112,#49113,#49114,
#49115,#49116),.UNSPECIFIED.,.F.,.F.,(4,2,2,2,2,2,2,2,4),(183.336022614352,
184.170939526247,185.005856438142,185.840773350037,186.675690261932,187.510607173827,
188.345524085721,189.180440997616,189.619207921532),.UNSPECIFIED.);
#451=B_SPLINE_CURVE_WITH_KNOTS('',3,(#49118,#49119,#49120,#49121,#49122,
#49123,#49124,#49125,#49126,#49127,#49128,#49129,#49130,#49131,#49132,#49133,
#49134,#49135,#49136,#49137,#49138,#49139,#49140,#49141,#49142,#49143,#49144,
#49145,#49146,#49147,#49148,#49149,#49150,#49151,#49152,#49153,#49154,#49155,
#49156,#49157,#49158,#49159,#49160,#49161,#49162,#49163,#49164,#49165,#49166,
#49167,#49168,#49169,#49170,#49171,#49172,#49173,#49174,#49175,#49176,#49177,
#49178,#49179,#49180,#49181,#49182,#49183,#49184,#49185,#49186,#49187,#49188,
#49189,#49190,#49191,#49192,#49193,#49194,#49195,#49196,#49197,#49198,#49199,
#49200,#49201,#49202,#49203,#49204,#49205,#49206,#49207,#49208,#49209,#49210,
#49211,#49212,#49213,#49214,#49215,#49216,#49217,#49218,#49219,#49220,#49221,
#49222,#49223,#49224,#49225,#49226,#49227,#49228,#49229,#49230,#49231,#49232,
#49233,#49234,#49235,#49236,#49237,#49238,#49239,#49240,#49241,#49242,#49243,
#49244,#49245,#49246,#49247,#49248,#49249,#49250,#49251,#49252,#49253,#49254,
#49255,#49256,#49257,#49258,#49259,#49260,#49261,#49262,#49263,#49264,#49265,
#49266,#49267,#49268,#49269,#49270,#49271,#49272,#49273,#49274,#49275,#49276,
#49277,#49278,#49279,#49280,#49281,#49282,#49283,#49284,#49285,#49286,#49287,
#49288,#49289,#49290,#49291,#49292,#49293,#49294,#49295,#49296,#49297,#49298,
#49299,#49300,#49301,#49302,#49303,#49304,#49305,#49306,#49307,#49308,#49309,
#49310,#49311,#49312,#49313,#49314,#49315,#49316,#49317,#49318,#49319,#49320,
#49321,#49322,#49323,#49324,#49325,#49326,#49327,#49328,#49329,#49330,#49331,
#49332,#49333,#49334,#49335,#49336,#49337,#49338,#49339,#49340,#49341,#49342,
#49343,#49344,#49345,#49346,#49347,#49348,#49349,#49350,#49351,#49352,#49353,
#49354,#49355,#49356,#49357,#49358,#49359,#49360,#49361,#49362,#49363,#49364,
#49365,#49366,#49367,#49368,#49369,#49370,#49371,#49372,#49373,#49374,#49375,
#49376,#49377,#49378,#49379),.UNSPECIFIED.,.F.,.F.,(4,3,3,3,3,3,3,3,3,3,
3,3,3,3,3,3,3,3,3,3,3,3,3,3,3,3,3,3,3,3,3,3,3,3,3,3,3,3,3,3,3,3,3,3,3,3,
3,3,3,3,3,3,3,3,3,3,3,3,3,3,3,3,3,3,3,3,3,3,3,3,3,3,3,3,3,3,3,3,3,3,3,3,
3,3,3,3,3,4),(189.619207921532,189.707929985649,189.797307795922,189.887481770886,
189.95318616018,190.027091750305,190.100910322165,190.174656348331,190.248344247449,
190.321988395462,190.395603135972,190.469214950654,190.542828795407,190.616457634733,
190.690114439724,190.763851350066,190.837632998332,190.911516190825,190.952939771549,
191.027488672489,191.101956526272,191.176357258931,191.250704752094,191.325012851992,
191.399295378063,191.47357887704,191.547866850868,191.622171800277,191.696506232628,
191.770919971326,191.845379025412,191.919935028318,191.952693382918,192.027242108422,
192.101709814936,192.176110428394,192.250457830343,192.324765866951,192.399048357611,
192.473331862887,192.547619869003,192.621924876698,192.696259393356,192.770673255297,
192.845132455027,192.919688636832,192.952446994288,193.026326208701,193.100122605659,
193.17385064081,193.247524719267,193.321159206551,193.394768438745,193.468380990763,
193.541999442896,193.61563676128,193.689305920882,193.763061053734,193.83686426255,
193.910774109244,193.952200605657,194.026812086564,194.1013376105,194.175791086452,
194.25018637582,194.324537301542,194.398857656763,194.473171400701,194.547484886987,
194.62181058366,194.696160962863,194.770583306371,194.845046783183,194.919600743203,
194.951954217027,195.030317639261,195.108584208233,195.186759217321,195.264816518699,
195.342801836007,195.42069745786,195.451831022711,195.527956948324,195.604128185549,
195.680403324837,195.756732301348,195.833183010997,195.902314075429),
 .UNSPECIFIED.);
#452=B_SPLINE_CURVE_WITH_KNOTS('',3,(#49381,#49382,#49383,#49384,#49385,
#49386,#49387,#49388,#49389,#49390,#49391,#49392,#49393,#49394,#49395,#49396,
#49397,#49398),.UNSPECIFIED.,.F.,.F.,(4,2,2,2,2,2,2,2,4),(195.902435354633,
196.737310140606,197.572227052501,198.407143964396,199.242060876291,200.076977788186,
200.911894700081,201.746811611976,202.185578535891),.UNSPECIFIED.);
#453=B_SPLINE_CURVE_WITH_KNOTS('',3,(#49400,#49401,#49402,#49403,#49404,
#49405,#49406,#49407,#49408,#49409,#49410,#49411,#49412,#49413,#49414,#49415,
#49416,#49417),.UNSPECIFIED.,.F.,.F.,(4,2,2,2,2,2,2,2,4),(202.185578535891,
203.020495447786,203.855412359681,204.690329271576,205.525246183471,206.360163095366,
207.19508000726,208.029996919155,208.468725328098),.UNSPECIFIED.);
#454=B_SPLINE_CURVE_WITH_KNOTS('',3,(#49419,#49420,#49421,#49422,#49423,
#49424,#49425,#49426,#49427,#49428,#49429,#49430,#49431,#49432,#49433,#49434,
#49435,#49436,#49437,#49438,#49439,#49440,#49441,#49442,#49443,#49444,#49445,
#49446,#49447,#49448,#49449,#49450,#49451,#49452,#49453,#49454,#49455,#49456,
#49457,#49458,#49459,#49460,#49461,#49462,#49463,#49464,#49465,#49466,#49467,
#49468,#49469,#49470,#49471,#49472,#49473,#49474,#49475,#49476,#49477,#49478,
#49479,#49480,#49481,#49482,#49483,#49484,#49485,#49486,#49487,#49488,#49489,
#49490,#49491,#49492,#49493,#49494,#49495,#49496,#49497,#49498,#49499,#49500,
#49501,#49502,#49503,#49504,#49505,#49506,#49507,#49508,#49509,#49510,#49511,
#49512,#49513,#49514,#49515,#49516,#49517,#49518,#49519,#49520,#49521,#49522,
#49523,#49524,#49525,#49526,#49527,#49528,#49529,#49530,#49531,#49532,#49533,
#49534,#49535,#49536,#49537,#49538,#49539,#49540,#49541,#49542,#49543,#49544,
#49545,#49546,#49547,#49548,#49549,#49550,#49551,#49552,#49553,#49554,#49555,
#49556,#49557,#49558,#49559,#49560,#49561,#49562,#49563,#49564,#49565,#49566,
#49567,#49568,#49569,#49570,#49571,#49572,#49573,#49574,#49575,#49576,#49577,
#49578,#49579,#49580,#49581,#49582,#49583,#49584,#49585,#49586,#49587,#49588,
#49589,#49590,#49591,#49592,#49593,#49594,#49595,#49596,#49597,#49598,#49599,
#49600,#49601,#49602,#49603,#49604,#49605,#49606,#49607,#49608,#49609,#49610,
#49611,#49612,#49613,#49614,#49615,#49616,#49617,#49618,#49619,#49620,#49621,
#49622,#49623,#49624,#49625,#49626,#49627,#49628,#49629,#49630,#49631,#49632,
#49633,#49634,#49635,#49636,#49637,#49638,#49639,#49640,#49641,#49642,#49643,
#49644,#49645,#49646,#49647,#49648,#49649,#49650,#49651,#49652,#49653,#49654,
#49655,#49656,#49657,#49658,#49659,#49660,#49661,#49662,#49663,#49664,#49665,
#49666,#49667,#49668,#49669,#49670,#49671,#49672,#49673,#49674,#49675,#49676,
#49677,#49678,#49679,#49680,#49681,#49682,#49683),.UNSPECIFIED.,.F.,.F.,
(4,3,3,3,3,3,3,3,3,3,3,3,3,3,3,3,3,3,3,3,3,3,3,3,3,3,3,3,3,3,3,3,3,3,3,
3,3,3,3,3,3,3,3,3,3,3,3,3,3,3,3,3,3,3,3,3,3,3,3,3,3,3,3,3,3,3,3,3,3,3,3,
3,3,3,3,3,3,3,3,3,3,3,3,3,3,3,3,3,4),(208.468825252627,208.546305652904,
208.623865211108,208.70502510238,208.78281664577,208.860690344446,208.938691508124,
208.948504776198,209.026868198431,209.105134767403,209.18330977649,209.261367077867,
209.339352395175,209.417248017027,209.448381581882,209.526287640001,209.604263759147,
209.682315074175,209.760496342961,209.838748514795,209.917120687846,209.948258387567,
210.022805583065,210.0972771468,210.171686951523,210.246048829269,210.320376580125,
210.394683980656,210.469000056536,210.543325401824,210.617672488177,210.692053796385,
210.766521334969,210.841038217922,210.915657760248,210.948011998936,211.021917589061,
211.095736160922,211.169482187088,211.243170086206,211.316814234219,211.390428974729,
211.464040789411,211.537654634165,211.611283473491,211.684940278482,211.758677188824,
211.83245883709,211.906342029583,211.947765610306,212.022314511246,212.096782365029,
212.171183097688,212.245530590852,212.31983869075,212.39412121682,212.468404715797,
212.542692689625,212.616997639035,212.691332071385,212.765745810084,212.84020486417,
212.914760867076,212.947519221675,213.02206794718,213.096535653694,213.170936267153,
213.245283669102,213.319591705711,213.393874196372,213.468157701649,213.542445707765,
213.61675071546,213.691085232118,213.76549909406,213.83995829379,213.914514475596,
213.947272833045,214.020064922963,214.092774329337,214.165416148347,214.238628258955,
214.311180237154,214.383713826874,214.45624252789,214.52996015422,214.602544126439,
214.676828579826,214.751113033212),.UNSPECIFIED.);
#455=B_SPLINE_CURVE_WITH_KNOTS('',3,(#49685,#49686,#49687,#49688,#49689,
#49690,#49691,#49692,#49693,#49694,#49695,#49696,#49697,#49698,#49699,#49700,
#49701,#49702),.UNSPECIFIED.,.F.,.F.,(4,2,2,2,2,2,2,2,4),(214.752284980915,
215.586866062145,216.42178297404,217.256699885935,218.091616797829,218.926533709724,
219.761450621619,220.596367533514,221.03492900151),.UNSPECIFIED.);
#456=B_SPLINE_CURVE_WITH_KNOTS('',3,(#49704,#49705,#49706,#49707,#49708,
#49709,#49710,#49711,#49712,#49713,#49714),.UNSPECIFIED.,.F.,.F.,(4,1,1,
1,1,1,1,1,4),(221.035575607579,221.945301723999,222.945055335369,223.444932141054,
223.944808946738,224.944562558108,225.944316169477,226.944069780846,227.31831244083),
 .UNSPECIFIED.);
#457=B_SPLINE_CURVE_WITH_KNOTS('',3,(#49716,#49717,#49718,#49719,#49720,
#49721,#49722,#49723,#49724,#49725,#49726,#49727,#49728,#49729,#49730,#49731,
#49732,#49733,#49734,#49735,#49736,#49737,#49738,#49739,#49740,#49741,#49742,
#49743,#49744,#49745,#49746,#49747,#49748,#49749,#49750,#49751,#49752,#49753,
#49754,#49755,#49756,#49757,#49758,#49759,#49760,#49761,#49762,#49763,#49764,
#49765,#49766,#49767,#49768,#49769,#49770,#49771,#49772,#49773,#49774,#49775,
#49776,#49777,#49778,#49779,#49780,#49781,#49782,#49783,#49784,#49785,#49786,
#49787,#49788,#49789,#49790,#49791,#49792,#49793,#49794,#49795,#49796,#49797,
#49798,#49799,#49800,#49801,#49802,#49803,#49804,#49805,#49806,#49807,#49808,
#49809,#49810,#49811,#49812,#49813,#49814,#49815,#49816,#49817,#49818,#49819,
#49820,#49821,#49822,#49823,#49824,#49825,#49826,#49827,#49828,#49829,#49830,
#49831,#49832,#49833,#49834,#49835,#49836,#49837,#49838,#49839,#49840,#49841,
#49842,#49843,#49844,#49845,#49846,#49847,#49848,#49849,#49850,#49851,#49852,
#49853,#49854,#49855,#49856,#49857,#49858,#49859,#49860,#49861,#49862,#49863,
#49864,#49865,#49866,#49867,#49868,#49869,#49870,#49871,#49872,#49873,#49874,
#49875,#49876,#49877,#49878,#49879,#49880,#49881,#49882,#49883,#49884,#49885,
#49886,#49887,#49888,#49889,#49890,#49891,#49892,#49893,#49894,#49895,#49896,
#49897,#49898,#49899,#49900,#49901,#49902,#49903,#49904,#49905,#49906,#49907,
#49908,#49909,#49910,#49911,#49912,#49913,#49914,#49915,#49916,#49917,#49918,
#49919,#49920,#49921,#49922,#49923,#49924,#49925,#49926,#49927,#49928,#49929,
#49930,#49931,#49932,#49933,#49934,#49935,#49936,#49937,#49938,#49939,#49940,
#49941,#49942,#49943,#49944,#49945,#49946,#49947,#49948,#49949,#49950,#49951,
#49952,#49953,#49954,#49955,#49956,#49957,#49958,#49959,#49960,#49961,#49962,
#49963,#49964,#49965,#49966,#49967,#49968,#49969,#49970,#49971,#49972,#49973,
#49974,#49975,#49976,#49977,#49978,#49979,#49980),.UNSPECIFIED.,.F.,.F.,
(4,3,3,3,3,3,3,3,3,3,3,3,3,3,3,3,3,3,3,3,3,3,3,3,3,3,3,3,3,3,3,3,3,3,3,
3,3,3,3,3,3,3,3,3,3,3,3,3,3,3,3,3,3,3,3,3,3,3,3,3,3,3,3,3,3,3,3,3,3,3,3,
3,3,3,3,3,3,3,3,3,3,3,3,3,3,3,3,3,4),(227.318319764609,227.39650771806,
227.471543782346,227.546599761227,227.621687259185,227.696817895653,227.77204346651,
227.847324610728,227.922710233808,227.943823392216,228.017702618196,228.091499026789,
228.165227073635,228.238901163838,228.312535662911,228.386144906928,228.459757470789,
228.533375934779,228.607013265027,228.680682436492,228.754437581151,228.828240801762,
228.902150660132,228.943577003585,229.018188418569,229.092713876678,229.167167286956,
229.241562510868,229.315913371408,229.390233661785,229.464547341577,229.538860764164,
229.613186397638,229.687536714199,229.761958996198,229.836422412068,229.91097631249,
229.943330614954,230.021694416695,230.099961360367,230.178136738113,230.256194396734,
230.334180063789,230.412076022717,230.443207420639,230.521112991988,230.599088615937,
230.677139428993,230.755320190006,230.833571851398,230.911943514346,230.943084226324,
231.017631417776,231.09210297716,231.166512777232,231.240874650033,231.315202395656,
231.389509790671,231.463825860633,231.538151199751,231.612498279687,231.686879581235,
231.761347112827,231.835863988587,231.91048352347,231.942837837693,232.016743903266,
232.090562951536,232.164309454742,232.237997831207,232.311642456557,232.385257674078,
232.45886996407,232.532484283145,232.606113595521,232.679770872006,232.753508249349,
232.827290362845,232.90117401393,232.942591449063,233.017415057715,233.09212234723,
233.166761385776,233.24134449427,233.315883961881,233.390394708471,233.464887403442,
233.539388711099,233.601505071789),.UNSPECIFIED.);
#458=B_SPLINE_CURVE_WITH_KNOTS('',3,(#49982,#49983,#49984,#49985,#49986,
#49987,#49988,#49989,#49990,#49991,#49992),.UNSPECIFIED.,.F.,.F.,(4,1,1,
1,1,1,1,1,4),(233.60151247774,233.942345060432,234.942098671801,235.941852283171,
236.94160589454,237.441482700225,237.941359505909,238.941113117279,239.884394119578),
 .UNSPECIFIED.);
#459=B_SPLINE_CURVE_WITH_KNOTS('',3,(#49994,#49995,#49996,#49997,#49998,
#49999,#50000,#50001,#50002,#50003,#50004,#50005,#50006,#50007,#50008,#50009,
#50010,#50011),.UNSPECIFIED.,.F.,.F.,(4,2,2,2,2,2,2,2,4),(239.884829668747,
240.719607290863,241.554524202758,242.389441114653,243.224358026548,244.059274938443,
244.894191850337,245.729108762232,246.167875686148),.UNSPECIFIED.);
#460=B_SPLINE_CURVE_WITH_KNOTS('',3,(#50013,#50014,#50015,#50016,#50017,
#50018,#50019,#50020,#50021,#50022,#50023,#50024,#50025,#50026,#50027,#50028,
#50029,#50030),.UNSPECIFIED.,.F.,.F.,(4,2,2,2,2,2,2,2,4),(246.167875686148,
247.002792598043,247.837709509938,248.672626421833,249.507543333728,250.342460245622,
251.177377157517,252.012294069412,252.451060993328),.UNSPECIFIED.);
#461=B_SPLINE_CURVE_WITH_KNOTS('',3,(#50032,#50033,#50034,#50035,#50036,
#50037,#50038,#50039,#50040,#50041,#50042),.UNSPECIFIED.,.F.,.F.,(4,1,1,
1,1,1,1,1,4),(252.451060993328,252.93766367645,253.937417287819,254.937170899189,
255.437047704873,255.936924510558,256.936678121927,257.936431733297,258.734246300507),
 .UNSPECIFIED.);
#462=B_SPLINE_CURVE_WITH_KNOTS('',3,(#50044,#50045,#50046,#50047,#50048,
#50049,#50050,#50051,#50052,#50053,#50054,#50055),.UNSPECIFIED.,.F.,.F.,
(4,1,1,1,1,1,1,1,1,4),(258.734246300507,258.936185344666,259.935938956035,
260.935692567405,261.935446178774,262.435322984459,262.935199790143,263.934953401513,
264.934707012882,265.017431607687),.UNSPECIFIED.);
#463=B_SPLINE_CURVE_WITH_KNOTS('',3,(#50057,#50058,#50059,#50060,#50061,
#50062,#50063,#50064,#50065,#50066,#50067,#50068,#50069,#50070,#50071,#50072,
#50073,#50074,#50075,#50076,#50077,#50078,#50079,#50080,#50081,#50082,#50083,
#50084,#50085,#50086,#50087,#50088,#50089,#50090,#50091,#50092,#50093,#50094,
#50095,#50096,#50097,#50098,#50099,#50100,#50101,#50102,#50103,#50104,#50105,
#50106,#50107,#50108,#50109,#50110,#50111,#50112,#50113,#50114,#50115,#50116,
#50117,#50118,#50119,#50120,#50121,#50122,#50123,#50124,#50125,#50126,#50127,
#50128,#50129,#50130,#50131,#50132,#50133,#50134,#50135,#50136,#50137,#50138,
#50139,#50140,#50141,#50142,#50143,#50144,#50145,#50146,#50147,#50148,#50149,
#50150,#50151,#50152,#50153,#50154,#50155,#50156,#50157,#50158,#50159,#50160,
#50161,#50162,#50163,#50164,#50165,#50166,#50167,#50168,#50169,#50170,#50171,
#50172,#50173,#50174,#50175,#50176,#50177,#50178,#50179,#50180,#50181,#50182,
#50183,#50184,#50185,#50186,#50187,#50188,#50189,#50190,#50191,#50192,#50193,
#50194,#50195,#50196,#50197,#50198,#50199,#50200,#50201,#50202,#50203,#50204,
#50205,#50206,#50207,#50208,#50209,#50210,#50211,#50212,#50213,#50214,#50215,
#50216,#50217,#50218,#50219,#50220,#50221,#50222,#50223,#50224,#50225,#50226,
#50227,#50228,#50229,#50230,#50231,#50232,#50233,#50234,#50235,#50236,#50237,
#50238,#50239,#50240,#50241,#50242,#50243,#50244,#50245,#50246,#50247,#50248,
#50249,#50250,#50251,#50252,#50253,#50254,#50255,#50256,#50257,#50258,#50259,
#50260,#50261,#50262,#50263,#50264,#50265,#50266,#50267,#50268,#50269,#50270,
#50271,#50272,#50273,#50274,#50275,#50276,#50277,#50278,#50279,#50280,#50281,
#50282,#50283,#50284,#50285,#50286,#50287,#50288,#50289,#50290,#50291,#50292,
#50293,#50294,#50295,#50296,#50297,#50298,#50299,#50300,#50301,#50302,#50303,
#50304,#50305,#50306,#50307,#50308,#50309,#50310,#50311,#50312,#50313,#50314,
#50315,#50316,#50317,#50318,#50319,#50320,#50321),.UNSPECIFIED.,.F.,.F.,
(4,3,3,3,3,3,3,3,3,3,3,3,3,3,3,3,3,3,3,3,3,3,3,3,3,3,3,3,3,3,3,3,3,3,3,
3,3,3,3,3,3,3,3,3,3,3,3,3,3,3,3,3,3,3,3,3,3,3,3,3,3,3,3,3,3,3,3,3,3,3,3,
3,3,3,3,3,3,3,3,3,3,3,3,3,3,3,3,3,4),(265.017431607687,265.091080802675,
265.164653880563,265.238165437093,265.311630019861,265.385062139806,265.458486881744,
265.531911102537,265.605347910285,265.678810418899,265.752348714647,265.825930080803,
265.899607635631,265.934460624252,266.009009349721,266.083477056199,266.15787766962,
266.232225071532,266.306533108104,266.380815598728,266.455099103966,266.529387110045,
266.603692117703,266.678026634324,266.752440496229,266.826899695921,266.90145587769,
266.934214235621,267.008093450029,267.081889846982,267.155617882127,267.229291960579,
267.302926447858,267.376535680046,267.450148232058,267.523766684185,267.597404002563,
267.671073162159,267.744828295005,267.818631503815,267.892541350503,267.93396784699,
268.008579327914,268.083104851867,268.157558327836,268.231953617221,268.306304542961,
268.380624898199,268.454938642154,268.529252128458,268.603577825149,268.677928204369,
268.752350547895,268.826814024724,268.901367984761,268.93372145836,269.012084880565,
269.090351449508,269.168526458566,269.246583759916,269.324569077196,269.402464699021,
269.433598264044,269.511504322176,269.589480441333,269.667531756376,269.745713025176,
269.823965197022,269.902337370087,269.933475069729,270.008022265226,270.08249382896,
270.156903633683,270.23126551143,270.305593262286,270.379900662817,270.454216738696,
270.528542083984,270.602889170337,270.677270478544,270.751738017127,270.82625490008,
270.900874442405,270.933228681098,271.017597248774,271.101519179819,271.185146260055,
271.268299188405,271.300616914866),.UNSPECIFIED.);
#464=B_SPLINE_CURVE_WITH_KNOTS('',3,(#50323,#50324,#50325,#50326,#50327,
#50328,#50329,#50330,#50331,#50332,#50333,#50334,#50335,#50336,#50337,#50338,
#50339,#50340),.UNSPECIFIED.,.F.,.F.,(4,2,2,2,2,2,2,2,4),(271.300616914866,
272.135533826761,272.970450738656,273.805367650551,274.640284562446,275.47520147434,
276.310118386235,277.14503529813,277.583802222046),.UNSPECIFIED.);
#465=B_SPLINE_CURVE_WITH_KNOTS('',3,(#50342,#50343,#50344,#50345,#50346,
#50347,#50348,#50349,#50350,#50351,#50352,#50353,#50354,#50355,#50356,#50357,
#50358,#50359,#50360,#50361,#50362,#50363,#50364,#50365,#50366,#50367,#50368,
#50369,#50370,#50371,#50372,#50373,#50374,#50375,#50376,#50377,#50378,#50379,
#50380,#50381,#50382,#50383,#50384,#50385,#50386,#50387,#50388,#50389,#50390,
#50391,#50392,#50393,#50394,#50395,#50396,#50397,#50398,#50399,#50400,#50401,
#50402,#50403,#50404,#50405,#50406,#50407,#50408,#50409,#50410,#50411,#50412,
#50413,#50414,#50415,#50416,#50417,#50418,#50419,#50420,#50421,#50422,#50423,
#50424,#50425,#50426,#50427,#50428,#50429,#50430,#50431,#50432,#50433,#50434,
#50435,#50436,#50437,#50438,#50439,#50440,#50441,#50442,#50443,#50444,#50445,
#50446,#50447,#50448,#50449,#50450,#50451,#50452,#50453,#50454,#50455,#50456,
#50457,#50458,#50459,#50460,#50461,#50462,#50463,#50464,#50465,#50466,#50467,
#50468,#50469,#50470,#50471,#50472,#50473,#50474,#50475,#50476,#50477,#50478,
#50479,#50480,#50481,#50482,#50483,#50484,#50485,#50486,#50487,#50488,#50489,
#50490,#50491,#50492,#50493,#50494,#50495,#50496,#50497,#50498,#50499,#50500,
#50501,#50502,#50503,#50504,#50505,#50506,#50507,#50508,#50509,#50510,#50511,
#50512,#50513,#50514,#50515,#50516,#50517,#50518,#50519,#50520,#50521,#50522,
#50523,#50524,#50525,#50526,#50527,#50528,#50529,#50530,#50531,#50532,#50533,
#50534,#50535,#50536,#50537,#50538,#50539,#50540,#50541,#50542,#50543,#50544,
#50545,#50546,#50547,#50548,#50549,#50550,#50551,#50552,#50553,#50554,#50555,
#50556,#50557,#50558,#50559,#50560,#50561,#50562,#50563,#50564,#50565,#50566,
#50567,#50568,#50569,#50570,#50571,#50572,#50573,#50574,#50575,#50576,#50577,
#50578,#50579,#50580,#50581,#50582,#50583,#50584,#50585,#50586,#50587,#50588,
#50589,#50590,#50591,#50592,#50593,#50594,#50595,#50596,#50597,#50598,#50599,
#50600,#50601,#50602,#50603),.UNSPECIFIED.,.F.,.F.,(4,3,3,3,3,3,3,3,3,3,
3,3,3,3,3,3,3,3,3,3,3,3,3,3,3,3,3,3,3,3,3,3,3,3,3,3,3,3,3,3,3,3,3,3,3,3,
3,3,3,3,3,3,3,3,3,3,3,3,3,3,3,3,3,3,3,3,3,3,3,3,3,3,3,3,3,3,3,3,3,3,3,3,
3,3,3,3,3,4),(277.583802222046,277.671324648983,277.759399580832,277.848188702518,
277.931503960684,278.005409550809,278.07922812267,278.152974148836,278.226662047954,
278.300306195967,278.373920936477,278.447532751159,278.521146595912,278.594775435239,
278.66843224023,278.742169150572,278.815950798838,278.889833991331,278.931257572053,
279.005806472993,279.080274326776,279.154675059436,279.229022552599,279.303330652497,
279.377613178569,279.451896677546,279.526184651374,279.600489600784,279.674824033135,
279.749237771833,279.82369682592,279.898252828826,279.931011183423,280.005559908927,
280.080027615441,280.154428228898,280.228775630846,280.303083667454,280.377366158114,
280.45164966339,280.525937669505,280.6002426772,280.674577193858,280.748991055799,
280.823450255528,280.898006437333,280.930764794792,281.004644009205,281.078440406163,
281.152168441314,281.225842519772,281.299477007056,281.37308623925,281.446698791268,
281.520317243401,281.593954561785,281.667623721387,281.74137885424,281.815182063056,
281.88909190975,281.930518406162,282.005129887069,282.079655411005,282.154108886956,
282.228504176325,282.302855102047,282.377175457268,282.451489201205,282.525802687492,
282.600128384164,282.674478763367,282.748901106875,282.823364583687,282.897918543707,
282.930272017531,283.008635439765,283.086902008738,283.165077017826,283.243134319204,
283.321119636513,283.399015258366,283.430148823216,283.505844145459,283.581580018405,
283.657412021233,283.73329529232,283.80929223256,283.866858317111),
 .UNSPECIFIED.);
#466=B_SPLINE_CURVE_WITH_KNOTS('',3,(#50605,#50606,#50607,#50608,#50609,
#50610,#50611,#50612,#50613,#50614,#50615,#50616,#50617,#50618,#50619,#50620,
#50621,#50622),.UNSPECIFIED.,.F.,.F.,(4,2,2,2,2,2,2,2,4),(283.86704461747,
284.70190444112,285.536821353015,286.37173826491,287.206655176805,288.0415720887,
288.876489000595,289.71140591249,290.150065821723),.UNSPECIFIED.);
#467=B_SPLINE_CURVE_WITH_KNOTS('',3,(#50624,#50625,#50626,#50627,#50628,
#50629,#50630,#50631,#50632,#50633,#50634),.UNSPECIFIED.,.F.,.F.,(4,1,1,
1,1,1,1,1,4),(290.150710098352,290.428424102801,290.928300908486,291.928054519855,
292.927808131225,293.927561742594,294.927315353963,295.927068965333,296.433358143585),
 .UNSPECIFIED.);
#468=B_SPLINE_CURVE_WITH_KNOTS('',3,(#50636,#50637,#50638,#50639,#50640,
#50641,#50642,#50643,#50644,#50645,#50646,#50647,#50648,#50649,#50650,#50651,
#50652,#50653,#50654,#50655,#50656,#50657,#50658,#50659,#50660,#50661,#50662,
#50663,#50664,#50665,#50666,#50667,#50668,#50669,#50670,#50671,#50672,#50673,
#50674,#50675,#50676,#50677,#50678,#50679,#50680,#50681,#50682,#50683,#50684,
#50685,#50686,#50687,#50688,#50689,#50690,#50691,#50692,#50693,#50694,#50695,
#50696,#50697,#50698,#50699,#50700,#50701,#50702,#50703,#50704,#50705,#50706,
#50707,#50708,#50709,#50710,#50711,#50712,#50713,#50714,#50715,#50716,#50717,
#50718,#50719,#50720,#50721,#50722,#50723,#50724,#50725,#50726,#50727,#50728,
#50729,#50730,#50731,#50732,#50733,#50734,#50735,#50736,#50737,#50738,#50739,
#50740,#50741,#50742,#50743,#50744,#50745,#50746,#50747,#50748,#50749,#50750,
#50751,#50752,#50753,#50754,#50755,#50756,#50757,#50758,#50759,#50760,#50761,
#50762,#50763,#50764,#50765,#50766,#50767,#50768,#50769,#50770,#50771,#50772,
#50773,#50774,#50775,#50776,#50777,#50778,#50779,#50780,#50781,#50782,#50783,
#50784,#50785,#50786,#50787,#50788,#50789,#50790,#50791,#50792,#50793,#50794,
#50795,#50796,#50797,#50798,#50799,#50800,#50801,#50802,#50803,#50804,#50805,
#50806,#50807,#50808,#50809,#50810,#50811,#50812,#50813,#50814,#50815,#50816,
#50817,#50818,#50819,#50820,#50821,#50822,#50823,#50824,#50825,#50826,#50827,
#50828,#50829,#50830,#50831,#50832,#50833,#50834,#50835,#50836,#50837,#50838,
#50839,#50840,#50841,#50842,#50843,#50844,#50845,#50846,#50847,#50848,#50849,
#50850,#50851,#50852,#50853,#50854,#50855,#50856,#50857,#50858,#50859,#50860,
#50861,#50862,#50863,#50864,#50865,#50866,#50867,#50868,#50869,#50870,#50871,
#50872,#50873,#50874,#50875,#50876),.UNSPECIFIED.,.F.,.F.,(4,3,3,3,3,3,
3,3,3,3,3,3,3,3,3,3,3,3,3,3,3,3,3,3,3,3,3,3,3,3,3,3,3,3,3,3,3,3,3,3,3,3,
3,3,3,3,3,3,3,3,3,3,3,3,3,3,3,3,3,3,3,3,3,3,3,3,3,3,3,3,3,3,3,3,3,3,3,3,
3,3,4),(296.433358143585,296.434193060497,296.523956293231,296.614011153268,
296.704010814826,296.793789611572,296.883272238627,296.926528890094,297.01529525035,
297.099635862482,297.167580580846,297.235456726032,297.268275055479,297.382618098477,
297.42642079471,297.541622636865,297.656981219889,297.77192883493,297.885910137167,
297.926022241522,298.037858647557,298.103191967374,298.182740066896,298.263144315382,
298.344595510271,298.394132693929,298.497551064862,298.604682910693,298.708091670656,
298.810098624463,298.908937059926,298.926078448187,298.938108879269,299.030135983696,
299.125844824944,299.222631746954,299.319787584731,299.355567335217,299.444448596844,
299.532532628507,299.619446836151,299.704089682706,299.773025791164,299.874821328605,
299.926497576467,300.029786969446,300.133648052168,300.238063752412,300.342340556559,
300.445603442629,300.517740448889,300.579586297339,300.607942703059,300.691865816354,
300.775475710615,300.858356472804,300.925694146258,301.00908707239,301.092604811342,
301.175646167532,301.189824156169,301.261772092477,301.334262910277,301.407337213651,
301.442859614954,301.526505427215,301.610283810116,301.69393111864,301.777377253097,
301.860593466713,301.925033158613,302.009335075365,302.093636992117,302.176114359061,
302.260572822167,302.277776526849,302.367060174878,302.45682417766,302.545782218094,
302.632284231065,302.716543450764),.UNSPECIFIED.);
#469=B_SPLINE_CURVE_WITH_KNOTS('',3,(#50878,#50879,#50880,#50881,#50882,
#50883,#50884,#50885,#50886,#50887,#50888,#50889,#50890,#50891,#50892,#50893,
#50894,#50895),.UNSPECIFIED.,.F.,.F.,(4,2,2,2,2,2,2,2,4),(302.716543450764,
303.551460362659,304.386377274554,305.221294186449,306.056211098343,306.891128010238,
307.726044922133,308.560961834028,308.999527974429),.UNSPECIFIED.);
#470=B_SPLINE_CURVE_WITH_KNOTS('',3,(#50897,#50898,#50899,#50900,#50901,
#50902,#50903,#50904,#50905,#50906,#50907),.UNSPECIFIED.,.F.,.F.,(4,1,1,
1,1,1,1,1,4),(309.000107393854,309.923619524504,310.923373135873,311.423249941558,
311.923126747242,312.922880358612,313.922633969981,314.922387581351,315.282906571436),
 .UNSPECIFIED.);
#471=B_SPLINE_CURVE_WITH_KNOTS('',3,(#50909,#50910,#50911,#50912,#50913,
#50914,#50915,#50916,#50917,#50918,#50919,#50920,#50921,#50922,#50923,#50924,
#50925,#50926,#50927,#50928,#50929,#50930,#50931,#50932,#50933,#50934,#50935,
#50936,#50937,#50938,#50939,#50940,#50941,#50942,#50943,#50944,#50945,#50946,
#50947,#50948,#50949,#50950,#50951,#50952,#50953,#50954,#50955,#50956,#50957,
#50958,#50959,#50960,#50961,#50962,#50963,#50964,#50965,#50966,#50967,#50968,
#50969,#50970,#50971,#50972,#50973,#50974,#50975,#50976,#50977,#50978,#50979,
#50980,#50981,#50982,#50983,#50984,#50985,#50986,#50987,#50988,#50989,#50990,
#50991,#50992,#50993,#50994,#50995,#50996,#50997,#50998,#50999,#51000,#51001,
#51002,#51003,#51004,#51005,#51006,#51007,#51008,#51009,#51010,#51011,#51012,
#51013,#51014,#51015,#51016,#51017,#51018,#51019,#51020,#51021,#51022,#51023,
#51024,#51025,#51026,#51027,#51028,#51029,#51030,#51031,#51032,#51033,#51034,
#51035,#51036,#51037,#51038,#51039,#51040,#51041,#51042,#51043,#51044,#51045,
#51046,#51047,#51048,#51049,#51050,#51051,#51052,#51053,#51054,#51055,#51056,
#51057,#51058,#51059,#51060,#51061,#51062,#51063,#51064,#51065,#51066,#51067,
#51068,#51069,#51070,#51071,#51072,#51073,#51074,#51075,#51076,#51077,#51078,
#51079,#51080,#51081,#51082,#51083,#51084,#51085,#51086,#51087,#51088,#51089,
#51090,#51091,#51092,#51093,#51094,#51095,#51096,#51097,#51098,#51099,#51100,
#51101,#51102,#51103,#51104,#51105,#51106,#51107,#51108,#51109,#51110,#51111,
#51112,#51113,#51114,#51115,#51116,#51117,#51118,#51119,#51120,#51121,#51122,
#51123,#51124,#51125,#51126,#51127,#51128,#51129,#51130,#51131,#51132,#51133,
#51134,#51135,#51136,#51137,#51138,#51139,#51140,#51141,#51142,#51143,#51144,
#51145,#51146,#51147,#51148,#51149,#51150,#51151,#51152,#51153,#51154,#51155,
#51156,#51157,#51158,#51159,#51160,#51161,#51162,#51163,#51164,#51165,#51166,
#51167,#51168,#51169,#51170,#51171,#51172,#51173),.UNSPECIFIED.,.F.,.F.,
(4,3,3,3,3,3,3,3,3,3,3,3,3,3,3,3,3,3,3,3,3,3,3,3,3,3,3,3,3,3,3,3,3,3,3,
3,3,3,3,3,3,3,3,3,3,3,3,3,3,3,3,3,3,3,3,3,3,3,3,3,3,3,3,3,3,3,3,3,3,3,3,
3,3,3,3,3,3,3,3,3,3,3,3,3,3,3,3,3,4),(315.282914065123,315.357699868323,
315.432502268467,315.507318293193,315.582159837218,315.657038806598,315.73200888131,
315.807030003138,315.882158767803,315.92214119272,315.996020407133,316.069816804091,
316.143544839241,316.217218917699,316.290853404983,316.364462637177,316.438075189195,
316.511693641327,316.585330959711,316.659000119313,316.732755252165,316.806558460981,
316.880468307675,316.921894804089,316.996506284996,317.071031808932,317.145485284884,
317.219880574253,317.294231499975,317.368551855196,317.442865599134,317.517179085421,
317.591504782093,317.665855161296,317.740277504804,317.814740981616,317.889294941636,
317.921648415459,318.000011837693,318.078278406666,318.156453415754,318.234510717131,
318.31249603444,318.390391656292,318.421525221143,318.499431279262,318.577407398407,
318.655458713436,318.733639982222,318.811892154054,318.890264327105,318.921402026828,
318.995949222326,319.070420786061,319.144830590784,319.21919246853,319.293520219386,
319.367827619918,319.442143695798,319.516469041086,319.590816127439,319.665197435647,
319.739664974231,319.814181857185,319.88880139951,319.921155638197,319.995061228322,
320.068879800183,320.142625826349,320.216313725467,320.289957873481,320.363572613991,
320.437184428674,320.510798273427,320.584427112754,320.658083917746,320.731820828088,
320.805602476354,320.879485668847,320.920909249567,320.995954235749,321.070880525398,
321.145736706182,321.220534877864,321.295287107226,321.370005534557,321.44470364888,
321.51940290023,321.566099372303),.UNSPECIFIED.);
#472=B_SPLINE_CURVE_WITH_KNOTS('',3,(#51175,#51176,#51177,#51178,#51179,
#51180,#51181,#51182,#51183,#51184,#51185),.UNSPECIFIED.,.F.,.F.,(4,1,1,
1,1,1,1,1,4),(321.566106881173,321.920662860936,322.920416472305,323.920170083675,
324.919923695044,325.419800500729,325.919677306414,326.919430917783,327.848964379533),
 .UNSPECIFIED.);
#473=B_SPLINE_CURVE_WITH_KNOTS('',3,(#51187,#51188,#51189,#51190,#51191,
#51192,#51193,#51194,#51195,#51196,#51197,#51198,#51199,#51200,#51201,#51202,
#51203,#51204),.UNSPECIFIED.,.F.,.F.,(4,2,2,2,2,2,2,2,4),(327.849512828964,
328.684201591377,329.519118503272,330.354035415167,331.188952327061,332.023869238956,
332.858786150851,333.693703062746,334.132469986662),.UNSPECIFIED.);
#474=B_SPLINE_CURVE_WITH_KNOTS('',3,(#51206,#51207,#51208,#51209,#51210,
#51211,#51212,#51213,#51214,#51215,#51216,#51217,#51218,#51219,#51220,#51221,
#51222,#51223),.UNSPECIFIED.,.F.,.F.,(4,2,2,2,2,2,2,2,4),(334.132469986662,
334.967386898557,335.802303810452,336.637220722347,337.472137634242,338.307054546136,
339.141971458031,339.976888369926,340.415655293842),.UNSPECIFIED.);
#475=B_SPLINE_CURVE_WITH_KNOTS('',3,(#51225,#51226,#51227,#51228,#51229,
#51230,#51231,#51232,#51233,#51234,#51235,#51236,#51237,#51238,#51239,#51240,
#51241,#51242,#51243,#51244,#51245,#51246,#51247,#51248,#51249,#51250,#51251,
#51252,#51253,#51254,#51255,#51256,#51257,#51258,#51259,#51260,#51261,#51262,
#51263,#51264,#51265,#51266,#51267,#51268,#51269,#51270,#51271,#51272,#51273,
#51274,#51275,#51276,#51277,#51278,#51279,#51280,#51281,#51282,#51283,#51284,
#51285,#51286,#51287,#51288,#51289,#51290,#51291,#51292,#51293,#51294,#51295,
#51296,#51297,#51298,#51299,#51300,#51301,#51302,#51303,#51304,#51305,#51306,
#51307,#51308,#51309,#51310,#51311,#51312,#51313,#51314,#51315,#51316,#51317,
#51318,#51319,#51320,#51321,#51322,#51323,#51324,#51325,#51326,#51327,#51328,
#51329,#51330,#51331,#51332,#51333,#51334,#51335,#51336,#51337,#51338,#51339,
#51340,#51341,#51342,#51343,#51344,#51345,#51346,#51347,#51348,#51349,#51350,
#51351,#51352,#51353,#51354,#51355,#51356,#51357,#51358,#51359,#51360,#51361,
#51362,#51363,#51364,#51365,#51366,#51367,#51368,#51369,#51370,#51371,#51372,
#51373,#51374,#51375,#51376,#51377,#51378,#51379,#51380,#51381,#51382,#51383,
#51384,#51385,#51386,#51387,#51388,#51389,#51390,#51391,#51392,#51393,#51394,
#51395,#51396,#51397,#51398,#51399,#51400,#51401,#51402,#51403,#51404,#51405,
#51406,#51407,#51408,#51409,#51410,#51411,#51412,#51413,#51414,#51415,#51416,
#51417,#51418,#51419,#51420,#51421,#51422,#51423,#51424,#51425,#51426,#51427,
#51428,#51429,#51430,#51431,#51432,#51433,#51434,#51435,#51436,#51437,#51438,
#51439,#51440,#51441,#51442,#51443,#51444,#51445,#51446,#51447,#51448,#51449,
#51450,#51451,#51452,#51453,#51454,#51455,#51456,#51457,#51458,#51459,#51460,
#51461,#51462,#51463,#51464,#51465,#51466,#51467,#51468,#51469,#51470,#51471,
#51472,#51473,#51474,#51475,#51476,#51477,#51478,#51479,#51480,#51481,#51482,
#51483,#51484,#51485,#51486,#51487,#51488,#51489),.UNSPECIFIED.,.F.,.F.,
(4,3,3,3,3,3,3,3,3,3,3,3,3,3,3,3,3,3,3,3,3,3,3,3,3,3,3,3,3,3,3,3,3,3,3,
3,3,3,3,3,3,3,3,3,3,3,3,3,3,3,3,3,3,3,3,3,3,3,3,3,3,3,3,3,3,3,3,3,3,3,3,
3,3,3,3,3,3,3,3,3,3,3,3,3,3,3,3,3,4),(340.415655293842,340.494481417605,
340.573436456946,340.65252149617,340.731807374889,340.81120335182,340.890766323486,
340.915981476954,340.989887067079,341.063705638941,341.137451665107,341.211139564226,
341.284783712239,341.35839845275,341.432010267432,341.505624112186,341.579252951513,
341.652909756505,341.726646666847,341.800428315114,341.874311507607,341.915735088324,
341.990283989264,342.064751843047,342.139152575706,342.213500068869,342.287808168767,
342.362090694839,342.436374193815,342.510662167644,342.584967117054,342.659301549404,
342.733715288102,342.808174342189,342.882730345094,342.915488699693,342.990037425197,
343.06450513171,343.138905745168,343.213253147116,343.287561183724,343.361843674384,
343.436127179659,343.510415185774,343.584720193469,343.659054710126,343.733468572068,
343.807927771797,343.882483953602,343.915242311062,343.989121525475,344.062917922434,
344.136645957585,344.210320036042,344.283954523327,344.357563755521,344.431176307539,
344.504794759672,344.578432078057,344.652101237659,344.725856370512,344.799659579328,
344.873569426022,344.914995922432,344.989607403339,345.064132927275,345.138586403226,
345.212981692595,345.287332618317,345.361652973537,345.435966717475,345.510280203761,
345.584605900434,345.658956279637,345.733378623144,345.807842099956,345.882396059976,
345.914749533801,345.993112956036,346.071379525009,346.149554534097,346.227611835475,
346.305597152784,346.383492774638,346.414626339486,346.486996405416,346.559377940755,
346.631822367735,346.698290813016),.UNSPECIFIED.);
#476=B_SPLINE_CURVE_WITH_KNOTS('',3,(#51491,#51492,#51493,#51494,#51495,
#51496,#51497,#51498,#51499,#51500,#51501,#51502,#51503,#51504,#51505,#51506,
#51507,#51508),.UNSPECIFIED.,.F.,.F.,(4,2,2,2,2,2,2,2,4),(346.698927745726,
347.533757512916,348.368674424811,349.203591336705,350.0385082486,350.873425160495,
351.70834207239,352.543258984284,352.981965591049),.UNSPECIFIED.);
#477=B_SPLINE_CURVE_WITH_KNOTS('',3,(#51510,#51511,#51512,#51513,#51514,
#51515,#51516,#51517,#51518,#51519,#51520,#51521,#51522,#51523,#51524,#51525,
#51526,#51527,#51528,#51529,#51530,#51531,#51532,#51533,#51534,#51535,#51536,
#51537,#51538,#51539,#51540,#51541,#51542,#51543,#51544,#51545,#51546,#51547,
#51548,#51549,#51550,#51551,#51552,#51553,#51554,#51555,#51556,#51557,#51558,
#51559,#51560,#51561,#51562,#51563,#51564,#51565,#51566,#51567,#51568,#51569,
#51570,#51571,#51572,#51573,#51574,#51575,#51576,#51577,#51578,#51579,#51580,
#51581,#51582,#51583,#51584,#51585,#51586,#51587,#51588,#51589,#51590,#51591,
#51592,#51593,#51594,#51595,#51596,#51597,#51598,#51599,#51600,#51601,#51602,
#51603,#51604,#51605,#51606,#51607,#51608,#51609,#51610,#51611,#51612,#51613,
#51614,#51615,#51616,#51617,#51618,#51619,#51620,#51621,#51622,#51623,#51624,
#51625,#51626,#51627,#51628,#51629,#51630,#51631,#51632,#51633,#51634,#51635,
#51636,#51637,#51638,#51639,#51640,#51641,#51642,#51643,#51644,#51645,#51646,
#51647,#51648,#51649,#51650,#51651,#51652,#51653,#51654,#51655,#51656,#51657,
#51658,#51659,#51660,#51661,#51662,#51663,#51664,#51665,#51666,#51667,#51668,
#51669,#51670,#51671,#51672,#51673,#51674,#51675,#51676,#51677,#51678,#51679,
#51680,#51681,#51682,#51683,#51684,#51685,#51686,#51687,#51688,#51689,#51690,
#51691,#51692,#51693,#51694,#51695,#51696,#51697,#51698,#51699,#51700,#51701,
#51702,#51703,#51704,#51705,#51706,#51707,#51708,#51709,#51710,#51711,#51712,
#51713,#51714,#51715,#51716,#51717,#51718,#51719,#51720,#51721,#51722,#51723,
#51724,#51725,#51726,#51727,#51728,#51729,#51730,#51731,#51732,#51733,#51734,
#51735,#51736,#51737,#51738,#51739,#51740,#51741,#51742,#51743,#51744,#51745,
#51746,#51747,#51748,#51749,#51750,#51751,#51752,#51753,#51754,#51755,#51756,
#51757,#51758,#51759,#51760,#51761,#51762,#51763,#51764,#51765,#51766,#51767,
#51768,#51769,#51770,#51771),.UNSPECIFIED.,.F.,.F.,(4,3,3,3,3,3,3,3,3,3,
3,3,3,3,3,3,3,3,3,3,3,3,3,3,3,3,3,3,3,3,3,3,3,3,3,3,3,3,3,3,3,3,3,3,3,3,
3,3,3,3,3,3,3,3,3,3,3,3,3,3,3,3,3,3,3,3,3,3,3,3,3,3,3,3,3,3,3,3,3,3,3,3,
3,3,3,3,3,4),(352.982179302569,353.057997125252,353.133729911659,353.209366840018,
353.284948102799,353.360473781065,353.412901619071,353.490807677191,353.568783796336,
353.646835111366,353.725016380152,353.803268551986,353.881640725038,353.912778424756,
353.987325620254,354.061797183988,354.136206988712,354.210568866458,354.284896617314,
354.359204017844,354.433520093724,354.507845439012,354.582192525365,354.656573833573,
354.731041372157,354.80555825511,354.880177797435,354.912532036125,354.98643762625,
355.060256198111,355.134002224277,355.207690123395,355.281334271409,355.354949011919,
355.428560826601,355.502174671355,355.575803510682,355.649460315673,355.723197226015,
355.796978874282,355.870862066775,355.912285647495,355.986834548435,356.061302402218,
356.135703134878,356.210050628041,356.284358727939,356.358641254011,356.432924752988,
356.507212726816,356.581517676226,356.655852108576,356.730265847275,356.804724901361,
356.879280904267,356.912039258864,356.986587984368,357.061055690881,357.135456304339,
357.209803706287,357.284111742895,357.358394233555,357.43267773883,357.506965744945,
357.58127075264,357.655605269297,357.730019131239,357.804478330968,357.879034512773,
357.911792870233,357.985672084646,358.059468481605,358.133196516756,358.206870595213,
358.280505082497,358.354114314692,358.427726866709,358.501345318843,358.574982637227,
358.64865179683,358.722406929682,358.796210138499,358.870119985193,358.911546481603,
358.999962665047,359.087819325262,359.176515270321,359.26521121538),
 .UNSPECIFIED.);
#478=B_SPLINE_CURVE_WITH_KNOTS('',3,(#51773,#51774,#51775,#51776,#51777,
#51778,#51779,#51780,#51781,#51782,#51783,#51784,#51785,#51786,#51787,#51788,
#51789,#51790),.UNSPECIFIED.,.F.,.F.,(4,2,2,2,2,2,2,2,4),(359.26521121538,
360.100128127275,360.93504503917,361.769961951065,362.60487886296,363.439795774855,
364.27471268675,365.109629598645,365.54839652256),.UNSPECIFIED.);
#479=B_SPLINE_CURVE_WITH_KNOTS('',3,(#51792,#51793,#51794,#51795,#51796,
#51797,#51798,#51799,#51800,#51801,#51802,#51803,#51804,#51805,#51806,#51807,
#51808,#51809,#51810,#51811,#51812,#51813,#51814,#51815,#51816,#51817,#51818,
#51819,#51820,#51821,#51822,#51823,#51824,#51825,#51826,#51827,#51828,#51829,
#51830,#51831,#51832,#51833,#51834,#51835,#51836,#51837,#51838,#51839,#51840,
#51841,#51842,#51843,#51844,#51845,#51846,#51847,#51848,#51849,#51850,#51851,
#51852,#51853,#51854,#51855,#51856,#51857,#51858,#51859,#51860,#51861,#51862,
#51863,#51864,#51865,#51866,#51867,#51868,#51869,#51870,#51871,#51872,#51873,
#51874,#51875,#51876,#51877,#51878,#51879,#51880,#51881,#51882,#51883,#51884,
#51885,#51886,#51887,#51888,#51889,#51890,#51891,#51892,#51893,#51894,#51895,
#51896,#51897,#51898,#51899,#51900,#51901,#51902,#51903,#51904,#51905,#51906,
#51907,#51908,#51909,#51910,#51911,#51912,#51913,#51914,#51915,#51916,#51917,
#51918,#51919,#51920,#51921,#51922,#51923,#51924,#51925,#51926,#51927,#51928,
#51929,#51930,#51931,#51932,#51933,#51934,#51935,#51936,#51937,#51938,#51939,
#51940,#51941,#51942,#51943,#51944,#51945,#51946,#51947,#51948,#51949,#51950,
#51951,#51952,#51953,#51954,#51955,#51956,#51957,#51958,#51959,#51960,#51961,
#51962,#51963,#51964,#51965,#51966,#51967,#51968,#51969,#51970,#51971,#51972,
#51973,#51974,#51975,#51976,#51977,#51978,#51979,#51980,#51981,#51982,#51983,
#51984,#51985,#51986,#51987,#51988,#51989,#51990,#51991,#51992,#51993,#51994,
#51995,#51996,#51997,#51998,#51999,#52000,#52001,#52002,#52003,#52004,#52005,
#52006,#52007,#52008,#52009,#52010,#52011,#52012,#52013,#52014,#52015,#52016,
#52017,#52018,#52019,#52020,#52021,#52022,#52023,#52024,#52025,#52026,#52027,
#52028,#52029,#52030,#52031,#52032,#52033,#52034,#52035,#52036,#52037,#52038,
#52039,#52040,#52041,#52042,#52043,#52044,#52045,#52046,#52047,#52048,#52049,
#52050,#52051,#52052,#52053,#52054,#52055,#52056),.UNSPECIFIED.,.F.,.F.,
(4,3,3,3,3,3,3,3,3,3,3,3,3,3,3,3,3,3,3,3,3,3,3,3,3,3,3,3,3,3,3,3,3,3,3,
3,3,3,3,3,3,3,3,3,3,3,3,3,3,3,3,3,3,3,3,3,3,3,3,3,3,3,3,3,3,3,3,3,3,3,3,
3,3,3,3,3,3,3,3,3,3,3,3,3,3,3,3,3,4),(365.54839652256,365.631859157807,
365.715917223977,365.800285132278,365.885043684889,365.909821761188,365.984433242095,
366.058958766032,366.133412241984,366.207807531353,366.282158457075,366.356478812296,
366.430792556234,366.505106042521,366.579431739194,366.653782118398,366.728204461906,
366.802667938719,366.877221898739,366.909575372558,366.987938794792,367.066205363764,
367.144380372852,367.222437674229,367.300422991537,367.37831861339,367.409452178242,
367.487358236361,367.565334355506,367.643385670535,367.72156693932,367.799819111153,
367.878191284204,367.909328983927,367.983876179425,368.05834774316,368.132757547883,
368.207119425629,368.281447176486,368.355754577016,368.430070652896,368.504395998184,
368.578743084538,368.653124392745,368.727591931329,368.802108814283,368.876728356608,
368.909082595296,368.982988185421,369.056806757282,369.130552783448,369.204240682566,
369.27788483058,369.35149957109,369.425111385772,369.498725230526,369.572354069853,
369.646010874844,369.719747785186,369.793529433453,369.867412625946,369.908836206666,
369.983385107606,370.057852961389,370.132253694048,370.206601187211,370.28090928711,
370.355191813181,370.429475312158,370.503763285986,370.578068235396,370.652402667747,
370.726816406445,370.801275460532,370.875831463437,370.908589818035,370.982308882286,
371.055947327308,371.129519736888,371.203040643532,371.276524540064,371.349994411399,
371.423459498714,371.496932884262,371.570427653428,371.643992705792,371.717597033695,
371.791294373935,371.831581829739),.UNSPECIFIED.);
#480=B_SPLINE_CURVE_WITH_KNOTS('',3,(#52058,#52059,#52060,#52061,#52062,
#52063,#52064,#52065,#52066,#52067,#52068,#52069,#52070),.UNSPECIFIED.,
 .F.,.F.,(4,2,1,1,1,1,1,1,1,4),(371.831581829739,371.908343429405,372.908097040774,
373.907850652143,374.407727457828,374.907604263513,375.907357874882,376.907111486251,
377.906865097621,378.114767136919),.UNSPECIFIED.);
#481=B_SPLINE_CURVE_WITH_KNOTS('',3,(#52072,#52073,#52074,#52075,#52076,
#52077,#52078,#52079,#52080,#52081,#52082),.UNSPECIFIED.,.F.,.F.,(4,1,1,
1,1,1,1,1,4),(378.114767136919,378.90661870899,379.906372320359,380.906125931729,
381.406002737414,381.905879543098,382.905633154468,383.905386765837,384.397952444099),
 .UNSPECIFIED.);
#482=B_SPLINE_CURVE_WITH_KNOTS('',3,(#52084,#52085,#52086,#52087,#52088,
#52089,#52090,#52091,#52092,#52093,#52094,#52095,#52096,#52097,#52098,#52099,
#52100,#52101),.UNSPECIFIED.,.F.,.F.,(4,2,2,2,2,2,2,2,4),(384.397952444099,
385.232869355993,386.067786267888,386.902703179783,387.737620091678,388.572537003573,
389.407453915467,390.242370827362,390.681137751278),.UNSPECIFIED.);
#483=B_SPLINE_CURVE_WITH_KNOTS('',3,(#52103,#52104,#52105,#52106,#52107,
#52108,#52109,#52110,#52111,#52112,#52113,#52114,#52115,#52116,#52117,#52118,
#52119,#52120),.UNSPECIFIED.,.F.,.F.,(4,2,2,2,2,2,2,2,4),(390.681137751278,
391.516054663173,392.350971575068,393.185888486963,394.020805398858,394.855722310753,
395.690639222648,396.525556134543,396.964110947501),.UNSPECIFIED.);
#484=B_SPLINE_CURVE_WITH_KNOTS('',3,(#52122,#52123,#52124,#52125,#52126,
#52127,#52128,#52129,#52130,#52131,#52132),.UNSPECIFIED.,.F.,.F.,(4,1,1,
1,1,1,1,1,4),(396.964751450397,397.901937325008,398.901690936378,399.901444547747,
400.901198159116,401.900951770486,402.40082857617,402.900705381855,403.247508365637),
 .UNSPECIFIED.);
#485=B_SPLINE_CURVE_WITH_KNOTS('',3,(#52134,#52135,#52136,#52137,#52138,
#52139,#52140,#52141,#52142,#52143,#52144,#52145,#52146,#52147,#52148,#52149,
#52150,#52151),.UNSPECIFIED.,.F.,.F.,(4,2,2,2,2,2,2,2,4),(403.247508365637,
404.082425277532,404.917342189427,405.752259101322,406.587176013217,407.422092925111,
408.257009837006,409.091926748901,409.530693672817),.UNSPECIFIED.);
#486=B_SPLINE_CURVE_WITH_KNOTS('',3,(#52153,#52154,#52155,#52156,#52157,
#52158,#52159,#52160,#52161,#52162,#52163,#52164,#52165,#52166,#52167,#52168,
#52169,#52170,#52171,#52172,#52173,#52174,#52175,#52176,#52177,#52178,#52179,
#52180,#52181,#52182,#52183,#52184,#52185,#52186,#52187,#52188,#52189,#52190,
#52191,#52192,#52193,#52194,#52195,#52196,#52197,#52198,#52199,#52200,#52201,
#52202,#52203,#52204,#52205,#52206,#52207,#52208,#52209,#52210,#52211,#52212,
#52213,#52214,#52215,#52216,#52217,#52218,#52219,#52220,#52221,#52222,#52223,
#52224,#52225,#52226,#52227,#52228,#52229,#52230,#52231,#52232,#52233,#52234,
#52235,#52236,#52237,#52238,#52239,#52240,#52241,#52242,#52243,#52244,#52245,
#52246,#52247,#52248,#52249,#52250,#52251,#52252,#52253,#52254,#52255,#52256,
#52257,#52258,#52259,#52260,#52261,#52262,#52263,#52264,#52265,#52266,#52267,
#52268,#52269,#52270,#52271,#52272,#52273,#52274,#52275,#52276,#52277,#52278,
#52279,#52280,#52281,#52282,#52283,#52284,#52285,#52286,#52287,#52288,#52289,
#52290,#52291,#52292,#52293,#52294,#52295,#52296,#52297,#52298,#52299,#52300,
#52301,#52302,#52303,#52304,#52305,#52306,#52307,#52308,#52309,#52310,#52311,
#52312,#52313,#52314,#52315,#52316,#52317,#52318,#52319,#52320,#52321,#52322,
#52323,#52324,#52325,#52326,#52327,#52328,#52329,#52330,#52331,#52332,#52333,
#52334,#52335,#52336,#52337,#52338,#52339,#52340,#52341,#52342,#52343,#52344,
#52345,#52346,#52347,#52348,#52349,#52350,#52351,#52352,#52353,#52354,#52355,
#52356,#52357,#52358,#52359,#52360,#52361,#52362,#52363,#52364,#52365,#52366,
#52367,#52368,#52369,#52370,#52371,#52372,#52373,#52374,#52375,#52376,#52377,
#52378,#52379,#52380,#52381,#52382,#52383,#52384,#52385,#52386,#52387,#52388,
#52389,#52390,#52391,#52392,#52393,#52394,#52395,#52396,#52397,#52398,#52399,
#52400,#52401,#52402,#52403,#52404,#52405,#52406,#52407,#52408,#52409,#52410,
#52411,#52412,#52413,#52414,#52415,#52416,#52417),.UNSPECIFIED.,.F.,.F.,
(4,3,3,3,3,3,3,3,3,3,3,3,3,3,3,3,3,3,3,3,3,3,3,3,3,3,3,3,3,3,3,3,3,3,3,
3,3,3,3,3,3,3,3,3,3,3,3,3,3,3,3,3,3,3,3,3,3,3,3,3,3,3,3,3,3,3,3,3,3,3,3,
3,3,3,3,3,3,3,3,3,3,3,3,3,3,3,3,3,4),(409.530693672817,409.613310095046,
409.696287231429,409.779442667476,409.862825827951,409.898980661441,409.973527856939,
410.047999420673,410.122409225397,410.196771103143,410.271098853999,410.34540625453,
410.419722330409,410.494047675697,410.568394762051,410.642776070258,410.717243608842,
410.791760491795,410.86638003412,410.89873427281,410.972639862935,411.046458434796,
411.120204460962,411.19389236008,411.267536508093,411.341151248603,411.414763063285,
411.488376908039,411.562005747365,411.635662552356,411.709399462699,411.783181110965,
411.857064303458,411.898487884179,411.973036785119,412.047504638902,412.121905371562,
412.196252864725,412.270560964623,412.344843490695,412.419126989672,412.4934149635,
412.56771991291,412.642054345261,412.71646808396,412.790927138046,412.865483140952,
412.898241495549,412.972790221053,413.047257927567,413.121658541024,413.196005942973,
413.270313979581,413.344596470241,413.418879975516,413.493167981632,413.567472989327,
413.641807505984,413.716221367926,413.790680567655,413.86523674946,413.897995106918,
413.971874321331,414.045670718289,414.11939875344,414.193072831897,414.266707319181,
414.340316551375,414.413929103393,414.487547555526,414.561184873909,414.634854033511,
414.708609166364,414.78241237518,414.856322221874,414.897748718287,414.971657525898,
415.045480993506,415.119233611503,415.192929817296,415.266584006522,415.340215986607,
415.413838250846,415.487463784416,415.56110557239,415.634807941336,415.708545074942,
415.782363994766,415.813507283438),.UNSPECIFIED.);
#487=B_SPLINE_CURVE_WITH_KNOTS('',3,(#52419,#52420,#52421,#52422,#52423,
#52424,#52425,#52426,#52427,#52428,#52429,#52430,#52431,#52432,#52433,#52434,
#52435,#52436),.UNSPECIFIED.,.F.,.F.,(4,2,2,2,2,2,2,2,4),(415.814026695158,
416.648795891891,417.483712803786,418.318629715681,419.153546627576,419.988463539471,
420.823380451366,421.658297363261,422.097064287176),.UNSPECIFIED.);
#488=B_SPLINE_CURVE_WITH_KNOTS('',3,(#52438,#52439,#52440,#52441,#52442,
#52443,#52444,#52445,#52446,#52447,#52448,#52449,#52450,#52451,#52452,#52453,
#52454,#52455),.UNSPECIFIED.,.F.,.F.,(4,2,2,2,2,2,2,2,4),(422.097064287176,
422.931981199071,423.766898110966,424.601815022861,425.436731934755,426.27164884665,
427.106565758545,427.94148267044,428.380249594356),.UNSPECIFIED.);
#489=B_SPLINE_CURVE_WITH_KNOTS('',3,(#52457,#52458,#52459,#52460,#52461,
#52462,#52463,#52464,#52465,#52466,#52467,#52468,#52469,#52470,#52471,#52472,
#52473,#52474),.UNSPECIFIED.,.F.,.F.,(4,2,2,2,2,2,2,2,4),(428.380249594356,
429.21516650625,430.050083418145,430.88500033004,431.719917241935,432.55483415383,
433.389751065724,434.224667977619,434.663434901535),.UNSPECIFIED.);
#490=B_SPLINE_CURVE_WITH_KNOTS('',3,(#52476,#52477,#52478,#52479,#52480,
#52481,#52482,#52483,#52484,#52485,#52486,#52487),.UNSPECIFIED.,.F.,.F.,
(4,1,1,1,1,1,1,1,1,4),(434.663434901535,434.892820945675,435.892574557044,
436.892328168413,437.392204974098,437.892081779783,438.891835391152,439.891589002521,
440.891342613891,440.946620208715),.UNSPECIFIED.);
#491=B_SPLINE_CURVE_WITH_KNOTS('',3,(#52489,#52490,#52491,#52492,#52493,
#52494,#52495,#52496,#52497,#52498,#52499,#52500,#52501,#52502,#52503,#52504,
#52505,#52506,#52507,#52508,#52509,#52510,#52511,#52512,#52513,#52514,#52515,
#52516,#52517,#52518,#52519,#52520,#52521,#52522,#52523,#52524,#52525,#52526,
#52527,#52528,#52529,#52530,#52531,#52532,#52533,#52534,#52535,#52536,#52537,
#52538,#52539,#52540,#52541,#52542,#52543,#52544,#52545,#52546,#52547,#52548,
#52549,#52550,#52551,#52552,#52553,#52554,#52555,#52556,#52557,#52558,#52559,
#52560,#52561,#52562,#52563,#52564,#52565,#52566,#52567,#52568,#52569,#52570,
#52571,#52572,#52573,#52574,#52575,#52576,#52577,#52578,#52579,#52580,#52581,
#52582,#52583,#52584,#52585,#52586,#52587,#52588,#52589,#52590,#52591,#52592,
#52593,#52594,#52595,#52596,#52597,#52598,#52599,#52600,#52601,#52602,#52603,
#52604,#52605,#52606,#52607,#52608,#52609,#52610,#52611,#52612,#52613,#52614,
#52615,#52616,#52617,#52618,#52619,#52620,#52621,#52622,#52623,#52624,#52625,
#52626,#52627,#52628,#52629,#52630,#52631,#52632,#52633,#52634,#52635,#52636,
#52637,#52638,#52639,#52640,#52641,#52642,#52643,#52644,#52645,#52646,#52647,
#52648,#52649,#52650,#52651,#52652,#52653,#52654,#52655,#52656,#52657,#52658,
#52659,#52660,#52661,#52662,#52663,#52664,#52665,#52666,#52667,#52668,#52669,
#52670,#52671,#52672,#52673,#52674,#52675,#52676,#52677,#52678,#52679,#52680,
#52681,#52682,#52683,#52684,#52685,#52686,#52687,#52688,#52689,#52690,#52691,
#52692,#52693,#52694,#52695,#52696,#52697,#52698,#52699,#52700,#52701,#52702,
#52703,#52704,#52705,#52706,#52707,#52708,#52709,#52710,#52711,#52712,#52713,
#52714,#52715,#52716,#52717,#52718,#52719,#52720,#52721,#52722,#52723,#52724,
#52725,#52726,#52727,#52728,#52729,#52730,#52731,#52732,#52733,#52734,#52735,
#52736,#52737,#52738,#52739,#52740,#52741,#52742,#52743,#52744,#52745,#52746,
#52747,#52748,#52749,#52750),.UNSPECIFIED.,.F.,.F.,(4,3,3,3,3,3,3,3,3,3,
3,3,3,3,3,3,3,3,3,3,3,3,3,3,3,3,3,3,3,3,3,3,3,3,3,3,3,3,3,3,3,3,3,3,3,3,
3,3,3,3,3,3,3,3,3,3,3,3,3,3,3,3,3,3,3,3,3,3,3,3,3,3,3,3,3,3,3,3,3,3,3,3,
3,3,3,3,3,4),(440.946620208715,441.020560156546,441.09442187872,441.168219784299,
441.241968235874,441.315681560049,441.389384092514,441.463083360364,441.536792301702,
441.61052385813,441.684330832929,441.758177779877,441.832127614359,441.89109622526,
441.964975439673,442.038771836632,442.112499871783,442.18617395024,442.259808437525,
442.333417669719,442.407030221737,442.48064867387,442.554285992254,442.627955151857,
442.701710284709,442.775513493525,442.84942334022,442.89084983663,442.965461317537,
443.039986841473,443.114440317424,443.188835606793,443.263186532514,443.337506887736,
443.411820631673,443.486134117959,443.560459814632,443.634810193835,443.709232537343,
443.783696014155,443.858249974174,443.890603447999,443.968966870234,444.047233439207,
444.125408448295,444.203465749673,444.281451066982,444.359346688836,444.390480253684,
444.468386311802,444.546362430945,444.624413745972,444.702595014756,444.780847186587,
444.859219359637,444.890357059368,444.964904254867,445.039375818601,445.113785623325,
445.188147501072,445.262475251928,445.336782652459,445.41109872834,445.485424073628,
445.559771159982,445.634152468189,445.708620006774,445.783136889728,445.857756432054,
445.890110670738,445.964016260863,446.037834832724,446.11158085889,446.185268758008,
446.258912906021,446.332527646531,446.406139461213,446.479753305967,446.553382145294,
446.627038950284,446.700775860626,446.774557508893,446.848440701386,446.889864282107,
446.977735760725,447.065254939028,447.152031804136,447.229805515894),
 .UNSPECIFIED.);
#492=B_SPLINE_CURVE_WITH_KNOTS('',3,(#52752,#52753,#52754,#52755,#52756,
#52757,#52758,#52759,#52760,#52761,#52762,#52763,#52764,#52765,#52766,#52767,
#52768,#52769),.UNSPECIFIED.,.F.,.F.,(4,2,2,2,2,2,2,2,4),(447.229805515894,
448.064722427789,448.899639339684,449.734556251579,450.569473163474,451.404390075369,
452.239306987263,453.074223899158,453.512990823074),.UNSPECIFIED.);
#493=B_SPLINE_CURVE_WITH_KNOTS('',3,(#52771,#52772,#52773,#52774,#52775,
#52776,#52777,#52778,#52779,#52780,#52781),.UNSPECIFIED.,.F.,.F.,(4,1,1,
1,1,1,1,1,4),(453.512990823074,453.888139561693,454.887893173062,455.887646784431,
456.887400395801,457.88715400717,458.387030812855,458.886907618539,459.795912565867),
 .UNSPECIFIED.);
#494=B_SPLINE_CURVE_WITH_KNOTS('',3,(#52783,#52784,#52785,#52786,#52787,
#52788,#52789,#52790,#52791,#52792,#52793,#52794,#52795,#52796,#52797,#52798,
#52799,#52800),.UNSPECIFIED.,.F.,.F.,(4,2,2,2,2,2,2,2,4),(459.796309024329,
460.631093042148,461.466009954043,462.300926865938,463.135843777833,463.970760689728,
464.805677601623,465.640594513517,466.079185816377),.UNSPECIFIED.);
#495=B_SPLINE_CURVE_WITH_KNOTS('',3,(#52802,#52803,#52804,#52805,#52806,
#52807,#52808,#52809,#52810,#52811,#52812,#52813,#52814,#52815,#52816,#52817,
#52818,#52819,#52820,#52821,#52822,#52823,#52824,#52825,#52826,#52827,#52828,
#52829,#52830,#52831,#52832,#52833,#52834,#52835,#52836,#52837,#52838,#52839,
#52840,#52841,#52842,#52843,#52844,#52845,#52846,#52847,#52848,#52849,#52850,
#52851,#52852,#52853,#52854,#52855,#52856,#52857,#52858,#52859,#52860,#52861,
#52862,#52863,#52864,#52865,#52866,#52867,#52868,#52869,#52870,#52871,#52872,
#52873,#52874,#52875,#52876,#52877,#52878,#52879,#52880,#52881,#52882,#52883,
#52884,#52885,#52886,#52887,#52888,#52889,#52890,#52891,#52892,#52893,#52894,
#52895,#52896,#52897,#52898,#52899,#52900,#52901,#52902,#52903,#52904,#52905,
#52906,#52907,#52908,#52909,#52910,#52911,#52912,#52913,#52914,#52915,#52916,
#52917,#52918,#52919,#52920,#52921,#52922,#52923,#52924,#52925,#52926,#52927,
#52928,#52929,#52930,#52931,#52932,#52933,#52934,#52935,#52936,#52937,#52938,
#52939,#52940,#52941,#52942,#52943,#52944,#52945,#52946,#52947,#52948,#52949,
#52950,#52951,#52952,#52953,#52954,#52955,#52956,#52957,#52958,#52959,#52960,
#52961,#52962,#52963,#52964,#52965,#52966,#52967,#52968,#52969,#52970,#52971,
#52972,#52973,#52974,#52975,#52976,#52977,#52978,#52979,#52980,#52981,#52982,
#52983,#52984,#52985,#52986,#52987,#52988,#52989,#52990,#52991,#52992,#52993,
#52994,#52995,#52996,#52997,#52998,#52999,#53000,#53001,#53002,#53003,#53004,
#53005,#53006,#53007,#53008,#53009,#53010,#53011,#53012,#53013,#53014,#53015,
#53016,#53017,#53018,#53019,#53020,#53021,#53022,#53023,#53024,#53025,#53026,
#53027,#53028,#53029,#53030,#53031,#53032,#53033,#53034,#53035,#53036,#53037,
#53038,#53039,#53040,#53041,#53042,#53043,#53044,#53045,#53046,#53047,#53048,
#53049,#53050,#53051,#53052,#53053,#53054,#53055,#53056,#53057,#53058,#53059,
#53060,#53061,#53062,#53063),.UNSPECIFIED.,.F.,.F.,(4,3,3,3,3,3,3,3,3,3,
3,3,3,3,3,3,3,3,3,3,3,3,3,3,3,3,3,3,3,3,3,3,3,3,3,3,3,3,3,3,3,3,3,3,3,3,
3,3,3,3,3,3,3,3,3,3,3,3,3,3,3,3,3,3,3,3,3,3,3,3,3,3,3,3,3,3,3,3,3,3,3,3,
3,3,3,3,3,4),(466.079976970098,466.153619284154,466.227213255373,466.300773314523,
466.374325227318,466.447875280061,466.521436506691,466.595021945881,466.668687639501,
466.742394771962,466.816212680748,466.884936509494,466.958842109278,467.032660690828,
467.106406726706,467.180094635551,467.253738793301,467.32735354355,467.400965367951,
467.474579222412,467.548208071428,467.621864886085,467.695601806015,467.76938346384,
467.843266665768,467.884690120864,467.959239000019,468.033706832004,468.108107542872,
468.182455014268,468.256763092443,468.331045596854,468.405329074328,468.479617026755,
468.55392195488,468.628256366081,468.702670083932,468.777129117314,468.851685099901,
468.884443732233,468.958992465446,469.033460179542,469.107860800451,469.182208209713,
469.256516253494,469.33079875118,469.405082263242,469.479370275996,469.553675290175,
469.628009813158,469.702423681156,469.776882886798,469.851439074247,469.884197343602,
469.958076624804,470.031873088724,470.105601190962,470.179275336584,470.252909891066,
470.326519190445,470.400131809449,470.473750328456,470.547387713562,470.621056939692,
470.694812138466,470.768615412974,470.842525324438,470.883950954972,470.958562234393,
471.033087557408,471.107540833182,471.181935923298,471.256286650874,471.330606809237,
471.404920358837,471.479233652386,471.553559158087,471.62790934825,471.70233150652,
471.776794800021,471.851348581114,471.883704566341,471.96265957517,472.041511482441,
472.121770297984,472.200388734976,472.281467739794,472.362546744612),
 .UNSPECIFIED.);
#496=B_SPLINE_CURVE_WITH_KNOTS('',3,(#53065,#53066,#53067,#53068,#53069,
#53070,#53071,#53072,#53073,#53074,#53075,#53076,#53077,#53078,#53079,#53080,
#53081,#53082),.UNSPECIFIED.,.F.,.F.,(4,2,2,2,2,2,2,2,4),(472.362546744612,
473.197463656507,474.032380568402,474.867297480297,475.702214392192,476.537131304087,
477.372048215982,478.206965127877,478.645732051792),.UNSPECIFIED.);
#497=B_SPLINE_CURVE_WITH_KNOTS('',3,(#53084,#53085,#53086,#53087,#53088,
#53089,#53090,#53091),.UNSPECIFIED.,.F.,.F.,(4,1,1,1,1,4),(478.645732051792,
478.881979845927,479.381856651612,479.881733457296,480.881487068666,480.943277745408),
 .UNSPECIFIED.);
#498=B_SPLINE_CURVE_WITH_KNOTS('',3,(#53095,#53096,#53097,#53098,#53099,
#53100),.UNSPECIFIED.,.F.,.F.,(4,2,4),(-483.018264218093,-482.185091679657,
-481.615013765778),.UNSPECIFIED.);
#499=B_SPLINE_CURVE_WITH_KNOTS('',3,(#53102,#53103,#53104,#53105,#53106,
#53107,#53108,#53109,#53110,#53111,#53112),.UNSPECIFIED.,.F.,.F.,(4,1,1,
1,1,1,1,1,4),(-481.615013765778,-481.232659880542,-480.234251872491,-479.23584386444,
-478.237435856389,-477.738231852364,-477.239027848338,-476.240619840287,
-475.332179850449),.UNSPECIFIED.);
#500=B_SPLINE_CURVE_WITH_KNOTS('',3,(#53114,#53115,#53116,#53117,#53118,
#53119,#53120,#53121,#53122,#53123,#53124,#53125,#53126,#53127,#53128,#53129,
#53130,#53131,#53132,#53133,#53134,#53135,#53136,#53137,#53138,#53139,#53140,
#53141,#53142,#53143,#53144,#53145,#53146,#53147,#53148,#53149,#53150,#53151,
#53152,#53153,#53154,#53155,#53156,#53157,#53158,#53159,#53160,#53161,#53162,
#53163,#53164,#53165,#53166,#53167,#53168,#53169,#53170,#53171,#53172,#53173,
#53174,#53175,#53176,#53177,#53178,#53179,#53180,#53181,#53182,#53183,#53184,
#53185,#53186,#53187,#53188,#53189,#53190,#53191,#53192,#53193,#53194,#53195,
#53196,#53197,#53198,#53199,#53200,#53201,#53202,#53203,#53204,#53205,#53206,
#53207,#53208,#53209,#53210,#53211,#53212,#53213,#53214,#53215,#53216,#53217,
#53218,#53219,#53220,#53221,#53222,#53223,#53224,#53225,#53226,#53227,#53228,
#53229,#53230,#53231,#53232,#53233,#53234,#53235,#53236,#53237,#53238,#53239,
#53240,#53241,#53242,#53243,#53244,#53245,#53246,#53247,#53248,#53249,#53250,
#53251,#53252,#53253,#53254,#53255,#53256,#53257,#53258,#53259,#53260,#53261,
#53262,#53263,#53264,#53265,#53266,#53267,#53268,#53269,#53270,#53271,#53272,
#53273,#53274,#53275,#53276,#53277,#53278,#53279,#53280,#53281,#53282,#53283,
#53284,#53285,#53286,#53287,#53288,#53289,#53290,#53291,#53292,#53293,#53294,
#53295,#53296,#53297,#53298,#53299,#53300,#53301,#53302,#53303,#53304,#53305,
#53306,#53307,#53308,#53309,#53310,#53311,#53312,#53313,#53314,#53315,#53316,
#53317,#53318,#53319,#53320,#53321,#53322,#53323,#53324,#53325,#53326,#53327,
#53328,#53329,#53330,#53331,#53332,#53333,#53334,#53335,#53336,#53337,#53338,
#53339,#53340,#53341,#53342,#53343,#53344,#53345,#53346,#53347,#53348,#53349,
#53350,#53351,#53352,#53353,#53354,#53355,#53356,#53357,#53358,#53359,#53360,
#53361,#53362,#53363,#53364,#53365,#53366,#53367,#53368,#53369,#53370,#53371,
#53372,#53373,#53374,#53375,#53376,#53377,#53378,#53379,#53380,#53381,#53382,
#53383,#53384,#53385,#53386,#53387,#53388,#53389,#53390,#53391,#53392,#53393,
#53394,#53395,#53396,#53397,#53398,#53399,#53400,#53401,#53402,#53403,#53404,
#53405,#53406,#53407,#53408,#53409,#53410,#53411,#53412,#53413,#53414,#53415,
#53416,#53417,#53418,#53419,#53420,#53421,#53422,#53423,#53424,#53425,#53426,
#53427,#53428,#53429,#53430,#53431,#53432,#53433,#53434,#53435,#53436,#53437,
#53438,#53439,#53440,#53441,#53442,#53443,#53444,#53445,#53446,#53447,#53448,
#53449,#53450,#53451,#53452,#53453,#53454,#53455,#53456,#53457,#53458,#53459,
#53460,#53461,#53462,#53463,#53464,#53465,#53466,#53467,#53468,#53469,#53470,
#53471,#53472,#53473,#53474,#53475,#53476,#53477,#53478,#53479,#53480,#53481,
#53482,#53483,#53484,#53485,#53486,#53487,#53488,#53489,#53490,#53491,#53492,
#53493,#53494,#53495,#53496,#53497,#53498,#53499,#53500,#53501,#53502,#53503,
#53504,#53505,#53506,#53507,#53508,#53509,#53510,#53511,#53512,#53513,#53514,
#53515,#53516,#53517,#53518,#53519,#53520,#53521,#53522,#53523,#53524,#53525,
#53526,#53527,#53528,#53529,#53530,#53531,#53532,#53533,#53534,#53535,#53536,
#53537,#53538,#53539,#53540,#53541,#53542,#53543,#53544,#53545,#53546,#53547,
#53548,#53549,#53550,#53551,#53552,#53553,#53554,#53555,#53556,#53557,#53558,
#53559,#53560,#53561,#53562,#53563,#53564,#53565,#53566,#53567,#53568,#53569,
#53570,#53571,#53572,#53573,#53574,#53575,#53576,#53577,#53578,#53579,#53580,
#53581,#53582,#53583,#53584,#53585,#53586,#53587,#53588,#53589,#53590,#53591,
#53592,#53593,#53594,#53595,#53596,#53597,#53598,#53599,#53600,#53601,#53602,
#53603,#53604,#53605,#53606,#53607,#53608,#53609,#53610,#53611,#53612,#53613,
#53614,#53615,#53616,#53617,#53618,#53619,#53620,#53621,#53622,#53623,#53624,
#53625,#53626,#53627,#53628,#53629,#53630,#53631,#53632,#53633,#53634,#53635,
#53636,#53637,#53638,#53639,#53640,#53641,#53642,#53643,#53644,#53645,#53646,
#53647,#53648,#53649,#53650,#53651,#53652,#53653,#53654,#53655,#53656,#53657,
#53658,#53659,#53660,#53661,#53662,#53663,#53664,#53665,#53666,#53667,#53668,
#53669,#53670,#53671,#53672,#53673,#53674,#53675,#53676,#53677,#53678,#53679,
#53680,#53681,#53682,#53683,#53684,#53685,#53686,#53687,#53688,#53689,#53690,
#53691,#53692,#53693,#53694,#53695,#53696,#53697,#53698,#53699,#53700,#53701),
 .UNSPECIFIED.,.F.,.F.,(4,2,2,2,2,2,2,2,2,2,2,2,2,2,2,2,2,2,2,2,2,2,2,2,
2,2,2,2,2,2,2,2,2,2,2,2,2,2,2,2,2,2,2,2,2,2,2,2,2,2,2,2,2,2,2,2,2,2,2,2,
2,2,2,2,2,2,2,2,2,2,2,2,2,2,2,2,2,2,2,2,2,2,2,2,2,2,2,2,2,2,2,2,2,2,2,2,
2,2,2,2,2,2,2,2,2,2,2,2,2,2,2,2,2,2,2,2,2,2,2,2,2,2,2,2,2,2,2,2,2,2,2,2,
2,2,2,2,2,2,2,2,2,2,2,2,2,2,2,2,2,2,2,2,2,2,2,2,2,2,2,2,2,2,2,2,2,2,2,2,
2,2,2,2,2,2,2,2,2,2,2,2,2,2,2,2,2,2,2,2,2,2,2,2,2,2,2,2,2,2,2,2,2,2,2,2,
2,2,2,2,2,2,2,2,2,2,2,2,2,2,2,2,2,2,2,2,2,2,2,2,2,2,2,2,2,2,2,2,2,2,2,2,
2,2,2,2,2,2,2,2,2,2,2,2,2,2,2,2,2,2,2,2,2,2,2,2,2,2,2,2,2,2,2,2,2,2,2,2,
2,2,2,2,2,2,2,2,2,2,2,2,2,2,2,2,2,4),(0.00198539612204261,0.0695281946069639,
0.0716483733971968,0.072969179381184,0.073972076551303,0.0749290983747497,
0.0758740341322982,0.0771441643805482,0.0802753384618654,0.11032324343002,
0.120039710884885,0.130454021338825,0.144461220265735,0.151158722935033,
0.363084719465787,0.454778594390875,0.4681349076702,0.471634360179192,0.473707948100735,
0.475542044892056,0.477833097855689,0.481371568867902,0.497446719655115,
0.778439388533868,0.818672492655279,0.846116047052023,0.855305827777556,
0.859172379250651,0.862094882651062,0.863455907775944,0.864442270617736,
0.865420353844057,0.866764935167273,0.869447100869893,0.892145023370465,
0.979737381538867,1.02398715311802,1.03736197047494,1.05265555968575,1.07043577687286,
1.09161394131366,1.16332718260169,1.21958320072858,1.24587362438719,1.25017773952524,
1.25242763347541,1.25408374066612,1.25587302246596,1.25844960236438,1.26565341123742,
1.27742634412946,1.53673525408729,1.60905511442089,1.63591159939473,1.64467059680943,
1.64838242997261,1.65120040753821,1.65252329121769,1.65348787930181,1.65443968533278,
1.65573652623811,1.65901300331603,1.69843339768578,1.80866273025028,1.98900072378921,
2.03584381354957,2.0446062523711,2.04753298908035,2.04942970210845,2.05122099999774,
2.05358346656273,2.05885699648111,2.10270998483147,2.10509827111799,2.11192125691502,
2.11943545989609,2.34943040262198,2.40685031023406,2.43822380802002,2.44179511876934,
2.44450865366691,2.44578773027049,2.44672257302339,2.44764719220153,2.448923625156,
2.45217539313844,2.49144714050303,2.49424509901302,2.69754764137921,2.71034855786606,
2.72487718823149,2.74179232383359,2.76235660355928,2.84197157690997,2.85423034514522,
2.85755998382333,2.85955673968097,2.86133782859566,2.86358260911417,2.86708760972244,
2.88361159567327,3.14610693198268,3.24739137343347,3.25348739652724,3.25559392926881,
3.25695616155746,3.25824599273288,3.25995271061636,3.26353756875168,3.29018256405163,
3.52810358341072,3.61108786406358,3.62601961855358,3.63080097964562,3.63385139291882,
3.63669002827845,3.64034460711267,3.64635727342268,3.67986555768184,3.88593006169828,
3.94648914665783,3.98693520425236,4.00606493204843,4.00913108619559,4.01072660008559,
4.01189780375313,4.01316011289113,4.01534920240838,4.02148880933641,4.10792534506172,
4.20914719257935,4.31736439579036,4.39842706092587,4.40403001113769,4.40649034009506,
4.40830260895753,4.40997659948598,4.41224826432733,4.41783899261654,4.47485505578666,
4.71800008987412,4.76459046956295,4.81166444119114,4.81855000693929,4.82038732051357,
4.82148241188958,4.82246306437885,4.82371014250117,4.82567954488016,4.8353260630709,
4.98259538975935,5.10994957207873,5.20750417298474,5.21401904105974,5.21643320229296,
5.21813631222369,5.219733861687,5.22193708240645,5.22626596375408,5.25648111595309,
5.3540931619433,5.58989094793188,5.61034088149828,5.61313429810774,5.61443501878184,
5.61545205917001,5.61655956749361,5.61833332045687,5.62416489431458,5.65922682939266,
5.72853199034163,5.78272325039861,5.85882676933152,5.99948411178665,6.00914421916709,
6.01237850579145,6.01419255739285,6.01584468599475,6.01804934296407,6.02213798290247,
6.04391039708453,6.08630957800502,6.13820806342962,6.2634291805327,6.37690477397915,
6.39908779934626,6.40201091950928,6.40338441389774,6.40443156985208,6.40555650373806,
6.40733606605516,6.41300200500401,6.44610734723482,6.51553803595748,6.57704285236464,
6.77430879573317,6.78735855004827,6.79092640313139,6.7930099515496,6.7946604386636,
6.79679336749758,6.80055352716823,6.81708426617341,6.87994192662831,6.93964084240221,
7.17595472550011,7.18930243288312,7.19154848261905,7.19288600902966,7.19390881611454,
7.1950001212912,7.19670600001893,7.20216479228494,7.23418971920697,7.28146810419425,
7.38223505699067,7.47687857406694,7.57869661925009,7.58545388975532,7.58812413296717,
7.58994973998226,7.59155375447143,7.59391316563354,7.59902973940588,7.67476473723677,
7.73426722392563,7.96953266292123,7.98287575677924,7.98507410654613,7.98637641689806,
7.98736832063171,7.98842611346783,7.99009391712742,7.99536731034472,8.02579760533239,
8.09520995465294,8.11571820202984,8.1683012150998,8.18949908798207,8.19744449917702,
8.20499631216658,8.21219193535937,8.29811088745238,8.38991537990947,8.39624932650762,
8.398646408409,8.40035392433461,8.40211252131302,8.4043908237084,8.4068895062419,
8.41098896619806,8.41916679068341,8.50146564518136,8.72278377822303,8.78961082403335,
8.79435638219568,8.79612479563324,8.79737560745655,8.79855126751737,8.80017644872472,
8.80338218776118,8.82624982003937,8.9350949730659,9.09991899962067,9.16097684959328,
9.16316410454399,9.16567212020523,9.16851195537729,9.17233875453396,9.17519046310607,
9.17815568852672,9.18253804083694,9.19443827821552,9.25204240797907,9.30482368907358,
9.528984484792,9.5466216554642,9.54952934708034,9.55125436302401,9.55257011153632,
9.55397084876998,9.55614764342539,9.56277813722868,9.59792562535676,9.64403532935967,
9.93113648162764,9.94273763261307,9.94626463558691,9.94851673288571,9.95021775518271,
9.95188223387109,9.9538123127537,9.95655547365957,9.96456728672837),
 .UNSPECIFIED.);
#501=B_SPLINE_CURVE_WITH_KNOTS('',3,(#53703,#53704,#53705,#53706,#53707,
#53708,#53709,#53710,#53711,#53712,#53713,#53714,#53715,#53716,#53717,#53718,
#53719,#53720,#53721,#53722,#53723,#53724,#53725,#53726,#53727,#53728,#53729,
#53730,#53731,#53732,#53733,#53734,#53735,#53736,#53737,#53738,#53739,#53740,
#53741,#53742,#53743,#53744,#53745,#53746,#53747,#53748,#53749,#53750,#53751,
#53752,#53753,#53754,#53755,#53756,#53757,#53758,#53759,#53760,#53761,#53762,
#53763,#53764,#53765,#53766,#53767,#53768,#53769,#53770,#53771,#53772,#53773,
#53774,#53775,#53776,#53777,#53778,#53779,#53780,#53781,#53782,#53783,#53784,
#53785,#53786,#53787,#53788,#53789,#53790,#53791,#53792,#53793,#53794,#53795,
#53796,#53797,#53798,#53799,#53800,#53801,#53802,#53803,#53804,#53805,#53806,
#53807,#53808,#53809,#53810,#53811,#53812,#53813,#53814,#53815,#53816,#53817,
#53818,#53819,#53820,#53821,#53822,#53823,#53824,#53825,#53826,#53827,#53828,
#53829,#53830,#53831,#53832,#53833,#53834,#53835,#53836,#53837,#53838,#53839,
#53840,#53841,#53842,#53843,#53844,#53845,#53846,#53847,#53848,#53849,#53850,
#53851,#53852,#53853,#53854,#53855,#53856,#53857,#53858,#53859,#53860,#53861,
#53862,#53863,#53864,#53865,#53866,#53867,#53868,#53869,#53870,#53871,#53872,
#53873,#53874,#53875,#53876,#53877,#53878,#53879,#53880,#53881,#53882,#53883,
#53884,#53885,#53886,#53887,#53888,#53889,#53890,#53891,#53892,#53893,#53894,
#53895,#53896,#53897,#53898,#53899,#53900,#53901,#53902,#53903,#53904,#53905,
#53906,#53907,#53908,#53909,#53910,#53911,#53912,#53913,#53914,#53915,#53916,
#53917,#53918,#53919,#53920,#53921,#53922,#53923,#53924,#53925,#53926,#53927,
#53928,#53929,#53930,#53931,#53932,#53933,#53934,#53935,#53936,#53937,#53938,
#53939,#53940,#53941,#53942,#53943,#53944,#53945,#53946,#53947,#53948,#53949,
#53950,#53951,#53952,#53953,#53954,#53955,#53956,#53957,#53958,#53959,#53960,
#53961,#53962,#53963,#53964,#53965,#53966,#53967),.UNSPECIFIED.,.F.,.F.,
(4,3,3,3,3,3,3,3,3,3,3,3,3,3,3,3,3,3,3,3,3,3,3,3,3,3,3,3,3,3,3,3,3,3,3,
3,3,3,3,3,3,3,3,3,3,3,3,3,3,3,3,3,3,3,3,3,3,3,3,3,3,3,3,3,3,3,3,3,3,3,3,
3,3,3,3,3,3,3,3,3,3,3,3,3,3,3,3,3,4),(-462.765457844239,-462.686733707007,
-462.607885241033,-462.528910893298,-462.449739943357,-462.37046153861,
-462.291017515773,-462.262907727575,-462.188987941163,-462.115154965673,
-462.041394339911,-461.96769165625,-461.894032549482,-461.82040268652,-461.746775610712,
-461.673146381543,-461.599502043651,-461.525829635064,-461.452077307501,
-461.378280156542,-461.304382129771,-461.264499719524,-461.189938657776,
-461.115458429897,-461.041045122637,-460.966684866971,-460.892363829109,
-460.818068201927,-460.743771465991,-460.669470136212,-460.595151722648,
-460.52080372868,-460.446376612285,-460.371904105249,-460.297335279547,
-460.266091711473,-460.191530725491,-460.11705056126,-460.042637305573,
-459.968277089437,-459.89395607909,-459.819660467428,-459.74536372908,-459.671062385706,
-459.596743947358,-459.522395917408,-459.447968748305,-459.373496178922,
-459.298927276623,-459.267683703422,-459.193790222148,-459.119979355985,
-459.046236660541,-458.972547741626,-458.89889824438,-458.825273843175,
-458.751645996229,-458.678012130141,-458.604359287906,-458.530674503678,
-458.456903950761,-458.383085240126,-458.30916058924,-458.269275695371,
-458.194652629911,-458.120115300983,-458.045649812182,-457.971242314493,
-457.896878997203,-457.822546079253,-457.74821961661,-457.673893284606,
-457.599554625761,-457.525191178434,-457.450755921203,-457.376279447764,
-457.301713075574,-457.27086768732,-457.1925020134,-457.114232844084,-457.036054897808,
-456.957994125735,-456.880005063599,-456.802105210717,-456.771663683295,
-456.699193493567,-456.626711514643,-456.55416419583,-456.482828943308),
 .UNSPECIFIED.);
#502=B_SPLINE_CURVE_WITH_KNOTS('',3,(#53969,#53970,#53971,#53972,#53973,
#53974,#53975,#53976,#53977,#53978,#53979,#53980,#53981,#53982,#53983,#53984,
#53985,#53986),.UNSPECIFIED.,.F.,.F.,(4,2,2,2,2,2,2,2,4),(-456.482201859304,
-455.647355625165,-454.81243871327,-453.977521801375,-453.14260488948,-452.307687977585,
-451.472771065691,-450.637854153796,-450.199157428511),.UNSPECIFIED.);
#503=B_SPLINE_CURVE_WITH_KNOTS('',3,(#53988,#53989,#53990,#53991,#53992,
#53993,#53994,#53995,#53996,#53997,#53998,#53999,#54000,#54001,#54002,#54003,
#54004,#54005,#54006,#54007,#54008,#54009,#54010,#54011,#54012,#54013,#54014,
#54015,#54016,#54017,#54018,#54019,#54020,#54021,#54022,#54023,#54024,#54025,
#54026,#54027,#54028,#54029,#54030,#54031,#54032,#54033,#54034,#54035,#54036,
#54037,#54038,#54039,#54040,#54041,#54042,#54043,#54044,#54045,#54046,#54047,
#54048,#54049,#54050,#54051,#54052,#54053,#54054,#54055,#54056,#54057,#54058,
#54059,#54060,#54061,#54062,#54063,#54064,#54065,#54066,#54067,#54068,#54069,
#54070,#54071,#54072,#54073,#54074,#54075,#54076,#54077,#54078,#54079,#54080,
#54081,#54082,#54083,#54084,#54085,#54086,#54087,#54088,#54089,#54090,#54091,
#54092,#54093,#54094,#54095,#54096,#54097,#54098,#54099,#54100,#54101,#54102,
#54103,#54104,#54105,#54106,#54107,#54108,#54109,#54110,#54111,#54112,#54113,
#54114,#54115,#54116,#54117,#54118,#54119,#54120,#54121,#54122,#54123,#54124,
#54125,#54126,#54127,#54128,#54129,#54130,#54131,#54132,#54133,#54134,#54135,
#54136,#54137,#54138,#54139,#54140,#54141,#54142,#54143,#54144,#54145,#54146,
#54147,#54148,#54149,#54150,#54151,#54152,#54153,#54154,#54155,#54156,#54157,
#54158,#54159,#54160,#54161,#54162,#54163,#54164,#54165,#54166,#54167,#54168,
#54169,#54170,#54171,#54172,#54173,#54174,#54175,#54176,#54177,#54178,#54179,
#54180,#54181,#54182,#54183,#54184,#54185,#54186,#54187,#54188,#54189,#54190,
#54191,#54192,#54193,#54194,#54195,#54196,#54197,#54198,#54199,#54200,#54201,
#54202,#54203,#54204,#54205,#54206,#54207,#54208,#54209,#54210,#54211,#54212,
#54213,#54214,#54215,#54216,#54217,#54218,#54219,#54220,#54221,#54222,#54223,
#54224,#54225,#54226,#54227,#54228,#54229,#54230,#54231,#54232,#54233,#54234,
#54235,#54236,#54237,#54238,#54239,#54240,#54241,#54242,#54243,#54244,#54245,
#54246,#54247,#54248,#54249,#54250,#54251,#54252),.UNSPECIFIED.,.F.,.F.,
(4,3,3,3,3,3,3,3,3,3,3,3,3,3,3,3,3,3,3,3,3,3,3,3,3,3,3,3,3,3,3,3,3,3,3,
3,3,3,3,3,3,3,3,3,3,3,3,3,3,3,3,3,3,3,3,3,3,3,3,3,3,3,3,3,3,3,3,3,3,3,3,
3,3,3,3,3,3,3,3,3,3,3,3,3,3,3,3,3,4),(-450.198883421911,-450.123484883473,
-450.048167901281,-449.972939821452,-449.897763337677,-449.822635356839,
-449.782807626938,-449.704897038825,-449.626916641923,-449.548861312063,
-449.470676596309,-449.392421216702,-449.314046526066,-449.283603622913,
-449.209044526386,-449.134560876773,-449.060138813668,-448.985764517231,
-448.911424199439,-448.837104095692,-448.762775226533,-448.688436993342,
-448.614076934992,-448.53968258119,-448.465202227618,-448.390672474616,
-448.316040743774,-448.285195614862,-448.211275828585,-448.137442853229,
-448.063682227601,-447.989979544073,-447.916320437438,-447.842690574608,
-447.769063498931,-447.695434269892,-447.621789932128,-447.548117523668,
-447.474365196231,-447.400568045397,-447.326670018748,-447.286787606811,
-447.212226545283,-447.137746317625,-447.063333010591,-446.988972755153,
-446.914651717522,-446.840356090572,-446.766059354873,-446.691758025332,
-446.617439612008,-446.543091618281,-446.468664502128,-446.394191995335,
-446.319623169876,-446.28837959876,-446.213818612626,-446.13933844824,-446.064925192397,
-445.990564976105,-445.9162439656,-445.841948353779,-445.767651615271,-445.693350271735,
-445.619031833226,-445.544683803114,-445.47025663385,-445.395784064305,
-445.321215161845,-445.289971590709,-445.216078109455,-445.142267243313,
-445.06852454789,-444.994835628994,-444.921186131768,-444.847561730584,
-444.773933883658,-444.70030001759,-444.626647175374,-444.552962391166,
-444.479191838268,-444.405373127653,-444.331448476786,-444.291563582658,
-444.205052052495,-444.119026734658,-444.033348198667,-443.94826036848,
-443.915901922701),.UNSPECIFIED.);
#504=B_SPLINE_CURVE_WITH_KNOTS('',3,(#54254,#54255,#54256,#54257,#54258,
#54259,#54260,#54261,#54262,#54263,#54264,#54265,#54266,#54267,#54268,#54269,
#54270,#54271),.UNSPECIFIED.,.F.,.F.,(4,2,2,2,2,2,2,2,4),(-443.915901922701,
-443.080985010806,-442.246068098911,-441.411151187016,-440.576234275121,
-439.741317363226,-438.906400451331,-438.071483539437,-437.632716615521),
 .UNSPECIFIED.);
#505=B_SPLINE_CURVE_WITH_KNOTS('',3,(#54273,#54274,#54275,#54276,#54277,
#54278,#54279,#54280,#54281,#54282,#54283),.UNSPECIFIED.,.F.,.F.,(4,1,1,
1,1,1,1,1,4),(-437.632716615521,-437.302707526302,-436.304299518251,-435.805095514225,
-435.3058915102,-434.307483502149,-433.309075494098,-432.310667486047,-431.349536372118),
 .UNSPECIFIED.);
#506=B_SPLINE_CURVE_WITH_KNOTS('',3,(#54285,#54286,#54287,#54288,#54289,
#54290,#54291,#54292,#54293,#54294,#54295,#54296,#54297,#54298,#54299,#54300,
#54301,#54302,#54303,#54304,#54305,#54306,#54307,#54308,#54309,#54310,#54311,
#54312,#54313,#54314,#54315,#54316,#54317,#54318,#54319,#54320,#54321,#54322,
#54323,#54324,#54325,#54326,#54327,#54328,#54329,#54330,#54331,#54332,#54333,
#54334,#54335,#54336,#54337,#54338,#54339,#54340,#54341,#54342,#54343,#54344,
#54345,#54346,#54347,#54348,#54349,#54350,#54351,#54352,#54353,#54354,#54355,
#54356,#54357,#54358,#54359,#54360,#54361,#54362,#54363,#54364,#54365,#54366,
#54367,#54368,#54369,#54370,#54371,#54372,#54373,#54374,#54375,#54376,#54377,
#54378,#54379,#54380,#54381,#54382,#54383,#54384,#54385,#54386,#54387,#54388,
#54389,#54390,#54391,#54392,#54393,#54394,#54395,#54396,#54397,#54398,#54399,
#54400,#54401,#54402,#54403,#54404,#54405,#54406,#54407,#54408,#54409,#54410,
#54411,#54412,#54413,#54414,#54415,#54416,#54417,#54418,#54419,#54420,#54421,
#54422,#54423,#54424,#54425,#54426,#54427,#54428,#54429,#54430,#54431,#54432,
#54433,#54434,#54435,#54436,#54437,#54438,#54439,#54440,#54441,#54442,#54443,
#54444,#54445,#54446,#54447,#54448,#54449,#54450,#54451,#54452,#54453,#54454,
#54455,#54456,#54457,#54458,#54459,#54460,#54461,#54462,#54463,#54464,#54465,
#54466,#54467,#54468,#54469,#54470,#54471,#54472,#54473,#54474,#54475,#54476,
#54477,#54478,#54479,#54480,#54481,#54482,#54483,#54484,#54485,#54486,#54487,
#54488,#54489,#54490,#54491,#54492,#54493,#54494,#54495,#54496,#54497,#54498,
#54499,#54500,#54501,#54502,#54503,#54504,#54505,#54506,#54507,#54508,#54509,
#54510,#54511,#54512,#54513,#54514,#54515,#54516,#54517,#54518,#54519,#54520,
#54521,#54522,#54523,#54524,#54525,#54526,#54527,#54528,#54529,#54530,#54531,
#54532,#54533,#54534,#54535,#54536,#54537,#54538,#54539,#54540,#54541,#54542,
#54543,#54544,#54545,#54546,#54547,#54548,#54549),.UNSPECIFIED.,.F.,.F.,
(4,3,3,3,3,3,3,3,3,3,3,3,3,3,3,3,3,3,3,3,3,3,3,3,3,3,3,3,3,3,3,3,3,3,3,
3,3,3,3,3,3,3,3,3,3,3,3,3,3,3,3,3,3,3,3,3,3,3,3,3,3,3,3,3,3,3,3,3,3,3,3,
3,3,3,3,3,3,3,3,3,3,3,3,3,3,3,3,3,4),(-431.349531308342,-431.312259477996,
-431.238365996742,-431.1645551306,-431.090812435177,-431.017123516282,-430.943474019055,
-430.869849617871,-430.796221770945,-430.722587904877,-430.648935062662,
-430.575250278454,-430.501479725556,-430.427661014941,-430.353736364073,
-430.313851469945,-430.239228404531,-430.16469107565,-430.090225586897,
-430.015818089256,-429.941454772013,-429.867121854112,-429.792795391517,
-429.718469059562,-429.644130400765,-429.569766953487,-429.495331696304,
-429.420855222913,-429.346288850772,-429.315443461894,-429.237077787853,
-429.158808618415,-429.080630672019,-429.002569899829,-428.924580837576,
-428.846680984581,-428.816239457869,-428.738328869755,-428.660348472851,
-428.58229314299,-428.504108427234,-428.425853047627,-428.347478356989,
-428.317035453843,-428.242476357316,-428.167992707704,-428.093570644599,
-428.019196348161,-427.944856030371,-427.870535926624,-427.796207057465,
-427.721868824275,-427.647508765924,-427.573114412122,-427.498634058549,
-427.424104305548,-427.349472574706,-427.318627445792,-427.244707659515,
-427.170874684159,-427.097114058531,-427.023411375003,-426.949752268368,
-426.876122405539,-426.802495329862,-426.728866100823,-426.65522176306,
-426.5815493546,-426.507797027163,-426.433999876329,-426.36010184968,-426.320219437742,
-426.245658376214,-426.171178148556,-426.096764841523,-426.022404586084,
-425.948083548453,-425.873787921505,-425.799491185805,-425.725189856265,
-425.65087144294,-425.576523449214,-425.50209633306,-425.427623826267,-425.353055000808,
-425.321811429691,-425.226177157113,-425.132161910787,-425.066346090687),
 .UNSPECIFIED.);
#507=B_SPLINE_CURVE_WITH_KNOTS('',3,(#54551,#54552,#54553,#54554,#54555,
#54556,#54557,#54558,#54559,#54560,#54561),.UNSPECIFIED.,.F.,.F.,(4,1,1,
1,1,1,1,1,4),(-425.066346001162,-424.32340342164,-423.324995413589,-422.326587405538,
-421.827383401512,-421.328179397487,-420.329771389436,-419.331363381385,
-418.783351185904),.UNSPECIFIED.);
#508=B_SPLINE_CURVE_WITH_KNOTS('',3,(#54563,#54564,#54565,#54566,#54567,
#54568,#54569,#54570,#54571,#54572,#54573,#54574,#54575,#54576,#54577,#54578,
#54579,#54580,#54581,#54582,#54583,#54584,#54585,#54586,#54587,#54588,#54589,
#54590,#54591,#54592,#54593,#54594,#54595,#54596,#54597,#54598,#54599,#54600,
#54601,#54602,#54603,#54604,#54605,#54606,#54607,#54608,#54609,#54610,#54611,
#54612,#54613,#54614,#54615,#54616,#54617,#54618,#54619,#54620,#54621,#54622,
#54623,#54624,#54625,#54626,#54627,#54628,#54629,#54630,#54631,#54632,#54633,
#54634,#54635,#54636,#54637,#54638,#54639,#54640,#54641,#54642,#54643,#54644,
#54645,#54646,#54647,#54648,#54649,#54650,#54651,#54652,#54653,#54654,#54655,
#54656,#54657,#54658,#54659,#54660,#54661,#54662,#54663,#54664,#54665,#54666,
#54667,#54668,#54669,#54670,#54671,#54672,#54673,#54674,#54675,#54676,#54677,
#54678,#54679,#54680,#54681,#54682,#54683,#54684,#54685,#54686,#54687,#54688,
#54689,#54690,#54691,#54692,#54693,#54694,#54695,#54696,#54697,#54698,#54699,
#54700,#54701,#54702,#54703,#54704,#54705,#54706,#54707,#54708,#54709,#54710,
#54711,#54712,#54713,#54714,#54715,#54716,#54717,#54718,#54719,#54720,#54721,
#54722,#54723,#54724,#54725,#54726,#54727,#54728,#54729,#54730,#54731,#54732,
#54733,#54734,#54735,#54736,#54737,#54738,#54739,#54740,#54741,#54742,#54743,
#54744,#54745,#54746,#54747,#54748,#54749,#54750,#54751,#54752,#54753,#54754,
#54755,#54756,#54757,#54758,#54759,#54760,#54761,#54762,#54763,#54764,#54765,
#54766,#54767,#54768,#54769,#54770,#54771,#54772,#54773,#54774,#54775,#54776,
#54777,#54778,#54779,#54780,#54781,#54782,#54783,#54784,#54785,#54786,#54787,
#54788,#54789,#54790,#54791,#54792,#54793,#54794,#54795,#54796,#54797,#54798,
#54799,#54800,#54801,#54802,#54803,#54804,#54805,#54806,#54807,#54808,#54809,
#54810,#54811,#54812,#54813,#54814,#54815,#54816,#54817,#54818,#54819,#54820,
#54821,#54822,#54823,#54824,#54825,#54826,#54827,#54828,#54829,#54830,#54831,
#54832,#54833,#54834,#54835,#54836,#54837,#54838,#54839,#54840,#54841,#54842,
#54843,#54844,#54845,#54846,#54847,#54848,#54849,#54850,#54851,#54852,#54853,
#54854,#54855,#54856,#54857,#54858,#54859,#54860,#54861,#54862,#54863,#54864,
#54865,#54866,#54867,#54868,#54869,#54870,#54871,#54872,#54873,#54874,#54875,
#54876,#54877,#54878,#54879,#54880,#54881,#54882,#54883,#54884,#54885,#54886,
#54887,#54888,#54889,#54890,#54891,#54892,#54893,#54894,#54895,#54896,#54897,
#54898,#54899,#54900,#54901,#54902,#54903,#54904,#54905,#54906,#54907,#54908,
#54909,#54910,#54911,#54912,#54913,#54914,#54915,#54916,#54917,#54918,#54919,
#54920,#54921,#54922,#54923,#54924,#54925,#54926,#54927,#54928,#54929,#54930,
#54931,#54932,#54933,#54934,#54935,#54936,#54937,#54938,#54939,#54940,#54941,
#54942,#54943,#54944,#54945,#54946,#54947,#54948,#54949,#54950,#54951,#54952,
#54953,#54954,#54955,#54956,#54957,#54958,#54959,#54960,#54961,#54962,#54963,
#54964,#54965,#54966,#54967,#54968,#54969,#54970,#54971,#54972,#54973,#54974,
#54975,#54976,#54977,#54978,#54979,#54980,#54981,#54982,#54983,#54984,#54985,
#54986,#54987,#54988,#54989,#54990,#54991,#54992,#54993,#54994,#54995,#54996,
#54997,#54998,#54999,#55000,#55001,#55002,#55003,#55004,#55005,#55006,#55007,
#55008,#55009,#55010,#55011,#55012,#55013,#55014,#55015,#55016,#55017,#55018,
#55019,#55020,#55021,#55022,#55023,#55024,#55025,#55026,#55027,#55028,#55029,
#55030,#55031,#55032,#55033,#55034,#55035,#55036,#55037,#55038,#55039,#55040,
#55041,#55042,#55043,#55044,#55045,#55046,#55047,#55048,#55049,#55050,#55051,
#55052,#55053,#55054,#55055,#55056,#55057,#55058,#55059,#55060,#55061,#55062,
#55063,#55064,#55065,#55066,#55067,#55068,#55069,#55070,#55071,#55072,#55073,
#55074,#55075,#55076,#55077,#55078,#55079,#55080,#55081,#55082,#55083,#55084,
#55085,#55086,#55087,#55088,#55089,#55090,#55091,#55092,#55093,#55094,#55095,
#55096,#55097,#55098,#55099,#55100,#55101,#55102,#55103,#55104,#55105,#55106,
#55107,#55108,#55109,#55110,#55111,#55112,#55113,#55114,#55115,#55116,#55117,
#55118,#55119,#55120,#55121,#55122,#55123,#55124,#55125,#55126,#55127,#55128,
#55129,#55130,#55131,#55132,#55133,#55134,#55135,#55136,#55137,#55138,#55139,
#55140,#55141,#55142,#55143,#55144,#55145,#55146,#55147,#55148,#55149,#55150,
#55151,#55152,#55153,#55154),.UNSPECIFIED.,.F.,.F.,(4,2,2,2,2,2,2,2,2,2,
2,2,2,2,2,2,2,2,2,2,2,2,2,2,2,2,2,2,2,2,2,2,2,2,2,2,2,2,2,2,2,2,2,2,2,2,
2,2,2,2,2,2,2,2,2,2,2,2,2,2,2,2,2,2,2,2,2,2,2,2,2,2,2,2,2,2,2,2,2,2,2,2,
2,2,2,2,2,2,2,2,2,2,2,2,2,2,2,2,2,2,2,2,2,2,2,2,2,2,2,2,2,2,2,2,2,2,2,2,
2,2,2,2,2,2,2,2,2,2,2,2,2,2,2,2,2,2,2,2,2,2,2,2,2,2,2,2,2,2,2,2,2,2,2,2,
2,2,2,2,2,2,2,2,2,2,2,2,2,2,2,2,2,2,2,2,2,2,2,2,2,2,2,2,2,2,2,2,2,2,2,2,
2,2,2,2,2,2,2,2,2,2,2,2,2,2,2,2,2,2,2,2,2,2,2,2,2,2,2,2,2,2,2,2,2,2,2,2,
2,2,2,2,2,2,2,2,2,2,2,2,2,2,2,2,2,2,2,2,2,2,2,2,2,2,2,2,2,2,2,2,2,2,2,2,
2,2,2,2,2,2,2,2,2,2,2,2,2,2,2,2,2,2,2,2,2,2,2,2,2,2,2,2,2,2,2,2,2,4),(0.0021107734850337,
0.313958519844044,0.35040009996185,0.356414794478,0.358234174092905,0.359367833469475,
0.360411547344041,0.361764528000124,0.364011936012669,0.376799783573237,
0.610136391080713,0.709427024510122,0.730459732642549,0.738807201515291,
0.74300297259584,0.745566374542952,0.747906260804457,0.749718256613466,
0.751482239056741,0.754467720453203,0.76242615398281,0.881084939228714,
0.943057554476376,1.05754177401902,1.10690754537228,1.13994018172288,1.14555813163525,
1.14730694929582,1.14840860341799,1.14942692467963,1.15073853363265,1.15292213128534,
1.16584495672315,1.41761405142509,1.47114434912135,1.50807569858058,1.52754146018385,
1.53534526331003,1.53929710978713,1.54172707645712,1.54395167436626,1.54568969179015,
1.54739382466881,1.54981364562728,1.55636884984881,1.65947926616869,1.71676694856147,
1.80926600952225,1.88350406002921,1.93135050162504,1.93830418565468,1.94015507138977,
1.94125709112926,1.94223511845872,1.94347238781967,1.94589446340493,1.95961792695883,
2.18939210654088,2.28466327834053,2.32641266982843,2.34055748272365,2.34671893492178,
2.35005225632904,2.35292677757035,2.35480362396226,2.35660681880789,2.35897650316781,
2.36298023110404,2.38744458822538,2.56296029065471,2.68577795450005,2.73572196891867,
2.74681664312659,2.74942953153049,2.75092662239325,2.75209028838396,2.75361256664475,
2.75626691324694,2.76663282861866,2.89765207232179,3.01540506199868,3.10413029830975,
3.11969968012748,3.12455575079131,3.12762226235055,3.13039514591027,3.13353090684597,
3.13992000122609,3.15489959781632,3.2387503322446,3.29730431605276,3.49307247223651,
3.5010405471248,3.5033702255634,3.50480406808172,3.5061071054925,3.5077551964859,
3.51040369774838,3.52370596033994,3.74780677769619,3.83375470821287,3.87399720222095,
3.89471535369585,3.8986551141331,3.90078571943595,3.90254130743241,3.90461426504689,
3.90819267942106,3.92175629212439,3.92611242701271,4.18472193881074,4.24569611785408,
4.30426635552552,4.31192408655437,4.31382892776188,4.31493854565035,4.31591604467966,
4.31713831127566,4.31902890203739,4.32764366944064,4.46092035292842,4.5860030993019,
4.64114574747391,4.68308640231368,4.70472185691645,4.70868771916486,4.71081361127814,
4.7124012303178,4.71413897389492,4.71722239298175,4.7263317306843,4.86088035479531,
4.9808557402363,5.07974238317828,5.10279583585837,5.10568588946089,5.10700354057489,
5.10802247424256,5.10912074299932,5.11085560287205,5.1163583990433,5.14832171989804,
5.19498872041594,5.34843151741666,5.4914573274337,5.50056617173629,5.50425602016166,
5.50639445823782,5.50820609593985,5.51040548387486,5.51447478919789,5.53593545284701,
5.57764565809867,5.69335417614501,5.73932978047868,5.79106841834415,5.79704213794616,
5.88710299665648,5.89293648269095,5.89480768164182,5.89583814499682,5.8968610469622,
5.89814341094205,5.90064554655125,5.917417671647,5.95724678085269,6.06865881566324,
6.26562322194229,6.27899833269172,6.28262774946748,6.28475201514421,6.28658169613875,
6.2888049579093,6.29298606283135,6.31661398042449,6.35908644372054,6.40676331601866,
6.48890429532695,6.57109364956328,6.67422177707237,6.68114943143726,6.68310097960942,
6.68414326941422,6.68504850002454,6.68616573584713,6.68806108720513,6.69035183626345,
6.69495640776353,6.74309228077589,6.85939758094755,7.06047579780178,7.07440238761392,
7.0779972087994,7.08006372959954,7.08164562436041,7.08368390545715,7.0872493771952,
7.10250905509153,7.27521357952129,7.40685581788151,7.42664699329201,7.43609456650022,
7.47177256101591,7.4749550738992,7.47622244352291,7.47714701563913,7.47813968857575,
7.47946069698554,7.48209105780349,7.48571292366267,7.51791370995304,7.58070347329138,
7.651120675881,7.72935355111975,7.87443180766461,7.88470691150223,7.88795956147616,
7.88974043937623,7.89133709218482,7.8934315626451,7.89720497949486,7.91513257216186,
7.94858233456759,8.01250701867857,8.04518093084793,8.06746826838991,8.07666828331565,
8.08514756286795,8.24409158714607,8.24937568939075,8.25298852654768,8.28038015810245,
8.28397846039894,8.28566266907478,8.28697065857906,8.28835756373514,8.29048447282631,
8.29300654727658,8.29775442611662,8.30899987232049,8.34497437531431,8.42743360480842,
8.60517709048041,8.65052731091322,8.65787307928605,8.66147492406709,8.6642970083782,
8.66739991386669,8.67242037805708,8.68946802306027,8.75152402116829,8.78755807143131,
8.81316434163601,8.83336111729128,8.85006462654123,8.8875679004826,8.98576628035345,
9.03282087370896,9.03698430486048,9.03865553493356,9.03987964687302,9.0411147379669,
9.04280756699977,9.04628535077753,9.05082977772171,9.06118002366665,9.08542244214113,
9.13110559744123,9.41322450409757,9.42992203620607,9.43343800885111,9.43568510058897,
9.43746498511733,9.43945720287359,9.4427717990269,9.45489497949568,9.53299488055051,
9.74268265674979,9.74993515641069,9.79522814704126,9.80157339631034,9.80832310078216,
9.81131441410182,9.81453324129582,9.8172532933142,9.81983574340087,9.82307430044125,
9.84510581793936,9.84793592067282,9.84922249928725,9.85020888203762,9.85127375306111,
9.85236422937948,9.85394563582332,9.85670926869068,9.95650252222412),
 .UNSPECIFIED.);
#509=B_SPLINE_CURVE_WITH_KNOTS('',3,(#55156,#55157,#55158,#55159,#55160,
#55161,#55162,#55163,#55164,#55165,#55166,#55167,#55168,#55169,#55170,#55171,
#55172,#55173,#55174,#55175,#55176,#55177,#55178,#55179,#55180,#55181,#55182,
#55183,#55184,#55185,#55186,#55187,#55188,#55189,#55190,#55191,#55192,#55193,
#55194,#55195,#55196,#55197,#55198,#55199,#55200,#55201,#55202,#55203,#55204,
#55205,#55206,#55207,#55208,#55209,#55210,#55211,#55212,#55213,#55214,#55215,
#55216,#55217,#55218,#55219,#55220,#55221,#55222,#55223,#55224,#55225,#55226,
#55227,#55228,#55229,#55230,#55231,#55232,#55233,#55234,#55235,#55236,#55237,
#55238,#55239,#55240,#55241,#55242,#55243,#55244,#55245,#55246,#55247,#55248,
#55249,#55250,#55251,#55252,#55253,#55254,#55255,#55256,#55257,#55258,#55259,
#55260,#55261,#55262,#55263,#55264,#55265,#55266,#55267,#55268,#55269,#55270,
#55271,#55272,#55273,#55274,#55275,#55276,#55277,#55278,#55279,#55280,#55281,
#55282,#55283,#55284,#55285,#55286,#55287,#55288,#55289,#55290,#55291,#55292,
#55293,#55294,#55295,#55296,#55297,#55298,#55299,#55300,#55301,#55302,#55303,
#55304,#55305,#55306,#55307,#55308,#55309,#55310,#55311,#55312,#55313,#55314,
#55315,#55316,#55317,#55318,#55319,#55320,#55321,#55322,#55323,#55324,#55325,
#55326,#55327,#55328,#55329,#55330,#55331,#55332,#55333,#55334,#55335,#55336,
#55337,#55338,#55339,#55340,#55341,#55342,#55343,#55344,#55345,#55346,#55347,
#55348,#55349,#55350,#55351,#55352,#55353,#55354,#55355,#55356,#55357,#55358,
#55359,#55360,#55361,#55362,#55363,#55364,#55365,#55366,#55367,#55368,#55369,
#55370,#55371,#55372,#55373,#55374,#55375,#55376,#55377,#55378,#55379,#55380,
#55381,#55382,#55383,#55384,#55385,#55386,#55387,#55388,#55389,#55390,#55391,
#55392,#55393,#55394,#55395,#55396,#55397,#55398,#55399,#55400,#55401,#55402,
#55403,#55404,#55405,#55406,#55407,#55408,#55409,#55410,#55411,#55412,#55413,
#55414,#55415,#55416,#55417,#55418,#55419,#55420),.UNSPECIFIED.,.F.,.F.,
(4,3,3,3,3,3,3,3,3,3,3,3,3,3,3,3,3,3,3,3,3,3,3,3,3,3,3,3,3,3,3,3,3,3,3,
3,3,3,3,3,3,3,3,3,3,3,3,3,3,3,3,3,3,3,3,3,3,3,3,3,3,3,3,3,3,3,3,3,3,3,3,
3,3,3,3,3,3,3,3,3,3,3,3,3,3,3,3,3,4),(-406.216115345406,-406.143347772459,
-406.070651068475,-405.998010215403,-405.925410253742,-405.8528277308,-405.780252578522,
-405.707671314702,-405.635070452466,-405.5623959866,-405.489683307801,-405.41686606389,
-405.353651268672,-405.279090207144,-405.204609979486,-405.130196672452,
-405.055836417014,-404.981515379383,-404.907219752434,-404.832923016735,
-404.758621687194,-404.684303273869,-404.609955280143,-404.53552816399,
-404.461055657197,-404.386486831737,-404.355243260621,-404.280682274487,
-404.206202110101,-404.131788854258,-404.057428637965,-403.983107627461,
-403.908812015639,-403.834515277131,-403.760213933595,-403.685895495086,
-403.611547464975,-403.53712029571,-403.462647726165,-403.388078823705,
-403.35683525257,-403.282941771316,-403.209130905174,-403.135388209751,
-403.061699290857,-402.988049793631,-402.914425392447,-402.840797545522,
-402.767163679453,-402.693510837238,-402.61982605303,-402.546055500133,
-402.472236789517,-402.39831213865,-402.35842724452,-402.283804179106,-402.209266850226,
-402.134801361473,-402.060393863831,-401.986030546589,-401.911697628688,
-401.837371166093,-401.763044834138,-401.688706175342,-401.614342728064,
-401.539907470881,-401.46543099749,-401.390864625349,-401.360019236469,
-401.281653562426,-401.203384392987,-401.12520644659,-401.047145674397,
-400.969156612141,-400.891256759144,-400.860815232443,-400.78290464433,
-400.704924247428,-400.626868917569,-400.548684201815,-400.470428822209,
-400.392054131574,-400.361611228418,-400.281649493689,-400.201825534484,
-400.122201686956,-400.042702288608,-399.963379286285,-399.933604772444),
 .UNSPECIFIED.);
#510=B_SPLINE_CURVE_WITH_KNOTS('',3,(#55422,#55423,#55424,#55425,#55426,
#55427,#55428,#55429,#55430,#55431,#55432,#55433,#55434,#55435,#55436,#55437,
#55438,#55439,#55440,#55441,#55442,#55443,#55444,#55445,#55446,#55447,#55448,
#55449,#55450,#55451,#55452,#55453,#55454,#55455,#55456,#55457,#55458,#55459,
#55460,#55461,#55462,#55463,#55464,#55465,#55466,#55467,#55468,#55469,#55470,
#55471,#55472,#55473,#55474,#55475,#55476,#55477,#55478,#55479,#55480,#55481,
#55482,#55483,#55484,#55485,#55486,#55487,#55488,#55489,#55490,#55491,#55492,
#55493,#55494,#55495,#55496,#55497,#55498,#55499,#55500,#55501,#55502,#55503,
#55504,#55505,#55506,#55507,#55508,#55509,#55510,#55511,#55512,#55513,#55514,
#55515,#55516,#55517,#55518,#55519,#55520,#55521,#55522,#55523,#55524,#55525,
#55526,#55527,#55528,#55529,#55530,#55531,#55532,#55533,#55534,#55535,#55536,
#55537,#55538,#55539,#55540,#55541,#55542,#55543,#55544,#55545,#55546,#55547,
#55548,#55549,#55550,#55551,#55552,#55553,#55554,#55555,#55556,#55557,#55558,
#55559,#55560,#55561,#55562,#55563,#55564,#55565,#55566,#55567,#55568,#55569,
#55570,#55571,#55572,#55573,#55574,#55575,#55576,#55577,#55578,#55579,#55580,
#55581,#55582,#55583,#55584,#55585,#55586,#55587,#55588,#55589,#55590,#55591,
#55592,#55593,#55594,#55595,#55596,#55597,#55598,#55599,#55600,#55601,#55602,
#55603,#55604,#55605,#55606,#55607,#55608,#55609,#55610,#55611,#55612,#55613,
#55614,#55615,#55616,#55617,#55618,#55619,#55620,#55621,#55622,#55623,#55624,
#55625,#55626,#55627,#55628,#55629,#55630,#55631,#55632,#55633,#55634,#55635,
#55636,#55637,#55638,#55639,#55640,#55641,#55642,#55643,#55644,#55645,#55646,
#55647,#55648,#55649,#55650,#55651,#55652,#55653),.UNSPECIFIED.,.F.,.F.,
(4,3,3,3,3,3,3,3,3,3,3,3,3,3,3,3,3,3,3,3,3,3,3,3,3,3,3,3,3,3,3,3,3,3,3,
3,3,3,3,3,3,3,3,3,3,3,3,3,3,3,3,3,3,3,3,3,3,3,3,3,3,3,3,3,3,3,3,3,3,3,3,
3,3,3,3,3,3,4),(-399.933604772444,-399.840724028374,-399.747275322167,-399.651442442894,
-399.558193843029,-399.461068824051,-399.363943805073,-399.272254036915,
-399.189836347056,-399.144188462362,-399.098687860549,-398.993531946425,
-398.88744788438,-398.78060582744,-398.673880337361,-398.568532952472,-398.466721211401,
-398.36490947033,-398.263770948654,-398.169261401944,-398.070080276303,
-397.968351387849,-397.865062762489,-397.76182249299,-397.661460916396,
-397.563608224494,-397.469619049145,-397.428854036759,-397.366376810785,
-397.269810333766,-397.1728740931,-397.075644374962,-397.011395580811,-396.923204173434,
-396.834237371584,-396.745961779209,-396.659945332695,-396.593937124864,
-396.499407545471,-396.40630905662,-396.368017440488,-396.274530703769,
-396.180063933608,-396.085912867677,-396.012055671754,-395.936942422972,
-395.861310605271,-395.78560057235,-395.759020212969,-395.681056354592,
-395.603177911801,-395.525486571131,-395.447574940006,-395.369663308881,
-395.292190873668,-395.215031932995,-395.17713875986,-395.106168378275,
-395.034791684364,-394.962843271554,-394.924103301075,-394.829321125232,
-394.734159677891,-394.638919242863,-394.543896244866,-394.449330934484,
-394.371456442117,-394.27823634382,-394.225892546488,-394.167925634083,
-394.110000407008,-394.08918638918,-393.995395485879,-393.900068996454,
-393.871945671379,-393.776560664005,-393.682731182159,-393.650419465264),
 .UNSPECIFIED.);
#511=B_SPLINE_CURVE_WITH_KNOTS('',3,(#55655,#55656,#55657,#55658,#55659,
#55660,#55661,#55662,#55663,#55664,#55665,#55666,#55667,#55668,#55669,#55670,
#55671,#55672,#55673,#55674,#55675,#55676,#55677,#55678,#55679,#55680,#55681,
#55682,#55683,#55684,#55685,#55686,#55687,#55688,#55689,#55690,#55691,#55692,
#55693,#55694,#55695,#55696,#55697,#55698,#55699,#55700,#55701,#55702,#55703,
#55704,#55705,#55706,#55707,#55708,#55709,#55710,#55711,#55712,#55713,#55714,
#55715,#55716,#55717,#55718,#55719,#55720,#55721,#55722,#55723,#55724,#55725,
#55726,#55727,#55728,#55729,#55730,#55731,#55732,#55733,#55734,#55735,#55736,
#55737,#55738,#55739,#55740,#55741,#55742,#55743,#55744,#55745,#55746,#55747,
#55748,#55749,#55750,#55751,#55752,#55753,#55754,#55755,#55756,#55757,#55758,
#55759,#55760,#55761,#55762,#55763,#55764,#55765,#55766,#55767,#55768,#55769,
#55770,#55771,#55772,#55773,#55774,#55775,#55776,#55777,#55778,#55779,#55780,
#55781,#55782,#55783,#55784,#55785,#55786,#55787,#55788,#55789,#55790,#55791,
#55792,#55793,#55794,#55795,#55796,#55797,#55798,#55799,#55800,#55801,#55802,
#55803,#55804,#55805,#55806,#55807,#55808,#55809,#55810,#55811,#55812,#55813,
#55814,#55815,#55816,#55817,#55818,#55819,#55820,#55821,#55822,#55823,#55824,
#55825,#55826,#55827,#55828,#55829,#55830,#55831,#55832,#55833,#55834,#55835,
#55836,#55837,#55838,#55839,#55840,#55841,#55842,#55843,#55844,#55845,#55846,
#55847,#55848,#55849,#55850,#55851,#55852,#55853,#55854,#55855,#55856,#55857,
#55858,#55859,#55860,#55861,#55862,#55863,#55864,#55865,#55866,#55867,#55868,
#55869,#55870,#55871,#55872,#55873,#55874,#55875,#55876,#55877,#55878,#55879,
#55880,#55881,#55882,#55883,#55884,#55885,#55886,#55887,#55888,#55889,#55890,
#55891,#55892,#55893,#55894,#55895,#55896,#55897,#55898,#55899,#55900,#55901,
#55902,#55903,#55904,#55905,#55906,#55907,#55908,#55909,#55910,#55911,#55912,
#55913,#55914,#55915,#55916,#55917,#55918,#55919,#55920,#55921,#55922,#55923,
#55924,#55925,#55926,#55927,#55928,#55929,#55930,#55931,#55932,#55933,#55934,
#55935,#55936,#55937,#55938,#55939,#55940,#55941,#55942,#55943,#55944,#55945,
#55946,#55947,#55948,#55949,#55950,#55951,#55952,#55953,#55954,#55955,#55956,
#55957,#55958,#55959,#55960,#55961,#55962,#55963,#55964,#55965,#55966,#55967,
#55968,#55969,#55970,#55971,#55972,#55973,#55974,#55975,#55976,#55977,#55978,
#55979,#55980,#55981,#55982,#55983,#55984,#55985,#55986,#55987,#55988,#55989,
#55990,#55991,#55992,#55993,#55994,#55995,#55996,#55997,#55998,#55999,#56000,
#56001,#56002,#56003,#56004,#56005,#56006,#56007,#56008,#56009,#56010,#56011,
#56012,#56013,#56014,#56015,#56016,#56017,#56018,#56019,#56020,#56021,#56022,
#56023,#56024,#56025,#56026,#56027,#56028,#56029,#56030,#56031,#56032,#56033,
#56034,#56035,#56036,#56037,#56038,#56039,#56040,#56041,#56042,#56043,#56044,
#56045,#56046,#56047,#56048,#56049,#56050,#56051,#56052,#56053,#56054,#56055,
#56056,#56057,#56058,#56059,#56060,#56061,#56062,#56063,#56064,#56065,#56066,
#56067,#56068,#56069,#56070,#56071,#56072,#56073,#56074,#56075,#56076,#56077,
#56078,#56079,#56080,#56081,#56082,#56083,#56084,#56085,#56086,#56087,#56088,
#56089,#56090,#56091,#56092,#56093,#56094,#56095,#56096,#56097,#56098,#56099,
#56100,#56101,#56102,#56103,#56104,#56105,#56106,#56107,#56108,#56109,#56110,
#56111,#56112,#56113,#56114,#56115,#56116,#56117,#56118,#56119,#56120,#56121,
#56122,#56123,#56124,#56125,#56126,#56127,#56128,#56129,#56130,#56131,#56132,
#56133,#56134,#56135,#56136,#56137,#56138,#56139,#56140,#56141,#56142,#56143,
#56144,#56145,#56146,#56147,#56148,#56149,#56150,#56151,#56152,#56153,#56154,
#56155,#56156,#56157,#56158,#56159,#56160,#56161,#56162,#56163,#56164,#56165,
#56166,#56167,#56168,#56169,#56170,#56171,#56172,#56173,#56174,#56175,#56176,
#56177,#56178,#56179,#56180,#56181,#56182,#56183,#56184,#56185,#56186,#56187,
#56188,#56189,#56190,#56191,#56192,#56193,#56194,#56195,#56196,#56197,#56198,
#56199,#56200,#56201,#56202,#56203,#56204,#56205,#56206,#56207,#56208,#56209,
#56210,#56211,#56212,#56213,#56214,#56215,#56216,#56217,#56218,#56219,#56220,
#56221,#56222,#56223,#56224,#56225,#56226,#56227,#56228,#56229,#56230,#56231,
#56232,#56233,#56234,#56235,#56236,#56237,#56238,#56239,#56240,#56241,#56242,
#56243,#56244),.UNSPECIFIED.,.F.,.F.,(4,2,2,2,2,2,2,2,2,2,2,2,2,2,2,2,2,
2,2,2,2,2,2,2,2,2,2,2,2,2,2,2,2,2,2,2,2,2,2,2,2,2,2,2,2,2,2,2,2,2,2,2,2,
2,2,2,2,2,2,2,2,2,2,2,2,2,2,2,2,2,2,2,2,2,2,2,2,2,2,2,2,2,2,2,2,2,2,2,2,
2,2,2,2,2,2,2,2,2,2,2,2,2,2,2,2,2,2,2,2,2,2,2,2,2,2,2,2,2,2,2,2,2,2,2,2,
2,2,2,2,2,2,2,2,2,2,2,2,2,2,2,2,2,2,2,2,2,2,2,2,2,2,2,2,2,2,2,2,2,2,2,2,
2,2,2,2,2,2,2,2,2,2,2,2,2,2,2,2,2,2,2,2,2,2,2,2,2,2,2,2,2,2,2,2,2,2,2,2,
2,2,2,2,2,2,2,2,2,2,2,2,2,2,2,2,2,2,2,2,2,2,2,2,2,2,2,2,2,2,2,2,2,2,2,2,
2,2,2,2,2,2,2,2,2,2,2,2,2,2,2,2,2,2,2,2,2,2,2,2,2,2,2,2,2,2,2,2,2,2,2,2,
2,2,2,2,2,2,2,2,2,2,2,2,2,2,2,2,2,2,2,2,2,2,2,2,2,4),(0.00126251356552906,
0.186225059591935,0.193990259317628,0.19760417431679,0.200513629682513,
0.202075751102413,0.203357019082192,0.204863069230799,0.207445693352058,
0.217043998252016,0.363438211244255,0.385024522634687,0.412253677348794,
0.463411052219837,0.589938340080337,0.595362951279272,0.597790581231296,
0.599596968016022,0.601278560374348,0.60358068419683,0.609349117916951,
0.673470367871833,0.815646411707306,0.850951794127492,0.883100220265274,
0.963169023255109,1.00316234601866,1.00941479613643,1.0111898642275,1.01227087534843,
1.01325421597341,1.01452547891397,1.01657474515715,1.02739808771365,1.19545040087695,
1.28545896032165,1.30012866446307,1.31921566201163,1.39961935540532,1.40518634575801,
1.40762792674758,1.40942523852921,1.41108462242251,1.41333526615407,1.41886827989882,
1.47516475895015,1.59923116554963,1.69608774112018,1.77531724775118,1.79240853360536,
1.80162765909149,1.80366953286933,1.80483324203958,1.80573882835393,1.8069250295385,
1.80899669625365,1.81777797401388,1.82144251627647,1.82694939923977,1.82768564840291,
1.8281272919608,1.82846786651528,1.82879097821014,1.82916813151138,1.97959339451667,
2.10481190919764,2.16856630786246,2.19695407305411,2.20134383698661,2.20361162585582,
2.20542782710451,2.20724670270543,2.21050818559859,2.22037974297078,2.37069746840366,
2.46801654513442,2.56231872042902,2.58041103267246,2.59013680425805,2.59228294034795,
2.59348923116391,2.59441703281646,2.59563059322422,2.59775137647423,2.60607319936642,
2.73929801363221,2.88638187638445,2.94784061656243,2.97551697690295,2.97987835971894,
2.98214016573425,2.98397267867294,2.98579897459387,2.98909752837871,2.99924785939877,
3.14531770463246,3.29548641033746,3.34214176984737,3.37410469665941,3.37960816752188,
3.38134334966396,3.38244184976096,3.38346101705703,3.38477899723267,3.38766988365334,
3.41073407474417,3.44353826910841,3.46033621650893,3.48689805699996,3.59984625278181,
3.69377985621534,3.74649184098769,3.77147094980812,3.77559627682108,3.77775641769902,
3.77934798960353,3.78106900517781,3.78406762974939,3.79257334228811,3.92214011435952,
4.08876382243618,4.16885607214697,4.17282109331017,4.17431925568893,4.17534357396199,
4.17634200162114,4.17755046195423,4.18060513669474,4.20944701402957,4.21008013036782,
4.21131496566917,4.21263018757763,4.21590635348096,4.22406982146714,4.23191199517075,
4.25921489352442,4.39448143441191,4.49878153598755,4.57899386313192,4.58466603679844,
4.58713836939801,4.58895236935687,4.59062299209048,4.59288254643806,4.59840607784595,
4.6531828280249,4.69205436451527,4.69627726121,4.72394140779277,4.90593207451306,
4.97864316905341,4.98239412207399,4.98410750791603,4.98542041403811,4.98682383866322,
4.98901660506026,4.99578648733437,5.0349271777167,5.09219180809043,5.33876318346483,
5.35359507428902,5.35854968084249,5.36132921066024,5.36411125609756,5.36756599164354,
5.37419198588687,5.41588391906643,5.51032462913216,5.60195616938288,5.65110888612536,
5.68822270573462,5.73191871970059,5.73600781058292,5.7376663761029,5.738887422315,
5.74020824652171,5.74199993481398,5.74607375590731,5.82727778891642,6.02621304286717,
6.03337671366783,6.06454240512269,6.12570791758827,6.1313948625272,6.13368270076109,
6.13536037415255,6.1371687624287,6.13961002527876,6.14498962286527,6.1521777570633,
6.21763669954722,6.2537116853726,6.37703636536662,6.52067717600832,6.54385969572138,
6.54644599819678,6.54772689175005,6.54865235206963,6.54964535379951,6.55098124091396,
6.55397118779999,6.62022197992257,6.72685954668408,6.87584332601442,6.88227289479219,
6.93579800087975,6.94125595077556,6.94349319513139,6.94514899073363,6.9469485092749,
6.94935474901434,6.9547594861787,6.96201258104655,7.02903448389256,7.14691191469804,
7.27480465632261,7.33517892825819,7.33883721822377,7.34019468783558,7.34116201489244,
7.34207784751574,7.34335428844533,7.3459096666313,7.36561724102622,7.45243821239467,
7.62550618070714,7.67417071886145,7.73084580485863,7.73654600221541,7.73887723907269,
7.74060068810342,7.74247190382012,7.74497089728739,7.75057061015039,7.7908098537416,
7.85992648875509,7.93703573742161,7.99171721680425,8.10653411768252,8.12498075648566,
8.12778318624607,8.1291263341347,8.13016503574707,8.13131385358631,8.13320261284503,
8.13987331763765,8.18297928745175,8.29028902764492,8.39675307603804,8.45614085496303,
8.47734992691092,8.51028366880833,8.51526937847719,8.51763204860301,8.51947969075598,
8.52149221508219,8.52355508731986,8.5300520652502,8.58940030098077,8.6778791210809,
8.90114226955788,8.91417096930859,8.91639817338624,8.9177296525736,8.91875087812554,
8.91984346061239,8.9215576849172,8.9270960936443,8.95988641600577,9.02854047039999,
9.10066765360362,9.13741325629974,9.18282148614484,9.23334694231122,9.23651186310549,
9.30452298112913,9.31033940470826,9.3126387099953,9.31431054129882,9.31609919802679,
9.31785429841102,9.32016630842972,9.33048866102472,9.4142135474803,9.46108141916866,
9.69379765100659,9.70707939134416,9.70927339045581,9.71057395287453,9.71156500734078,
9.71262237429131,9.71429050094163,9.71957287421535,9.75009918684513,9.95560876709398),
 .UNSPECIFIED.);
#512=B_SPLINE_CURVE_WITH_KNOTS('',3,(#56246,#56247,#56248,#56249,#56250,
#56251,#56252,#56253,#56254,#56255,#56256,#56257,#56258,#56259,#56260,#56261,
#56262,#56263),.UNSPECIFIED.,.F.,.F.,(4,2,2,2,2,2,2,2,4),(-381.084048850905,
-380.24913193901,-379.414215027115,-378.579298115221,-377.744381203326,
-376.909464291431,-376.074547379536,-375.239630467641,-374.800863543726),
 .UNSPECIFIED.);
#513=B_SPLINE_CURVE_WITH_KNOTS('',3,(#56265,#56266,#56267,#56268,#56269,
#56270,#56271,#56272,#56273,#56274,#56275,#56276,#56277,#56278,#56279,#56280,
#56281,#56282,#56283,#56284,#56285,#56286,#56287,#56288,#56289,#56290,#56291,
#56292,#56293,#56294,#56295,#56296,#56297,#56298,#56299,#56300,#56301,#56302,
#56303,#56304,#56305,#56306,#56307,#56308,#56309,#56310,#56311,#56312,#56313,
#56314,#56315,#56316,#56317,#56318,#56319,#56320,#56321,#56322,#56323,#56324,
#56325,#56326,#56327,#56328,#56329,#56330,#56331,#56332,#56333,#56334,#56335,
#56336,#56337,#56338,#56339,#56340,#56341,#56342,#56343,#56344,#56345,#56346,
#56347,#56348,#56349,#56350,#56351,#56352,#56353,#56354,#56355,#56356,#56357,
#56358,#56359,#56360,#56361,#56362,#56363,#56364,#56365,#56366,#56367,#56368,
#56369,#56370,#56371,#56372,#56373,#56374,#56375,#56376,#56377,#56378,#56379,
#56380,#56381,#56382,#56383,#56384,#56385,#56386,#56387,#56388,#56389,#56390,
#56391,#56392,#56393,#56394,#56395,#56396,#56397,#56398,#56399,#56400,#56401,
#56402,#56403,#56404,#56405,#56406,#56407,#56408,#56409,#56410,#56411,#56412,
#56413,#56414,#56415,#56416,#56417,#56418,#56419,#56420,#56421,#56422,#56423,
#56424,#56425,#56426,#56427,#56428,#56429,#56430,#56431,#56432,#56433,#56434,
#56435,#56436,#56437,#56438,#56439,#56440,#56441,#56442,#56443,#56444,#56445,
#56446,#56447,#56448,#56449,#56450,#56451,#56452,#56453,#56454,#56455,#56456,
#56457,#56458,#56459,#56460,#56461,#56462,#56463,#56464,#56465,#56466,#56467,
#56468,#56469,#56470,#56471,#56472,#56473,#56474,#56475,#56476,#56477,#56478,
#56479,#56480,#56481,#56482,#56483,#56484,#56485,#56486,#56487,#56488,#56489,
#56490,#56491,#56492,#56493,#56494,#56495,#56496,#56497,#56498,#56499,#56500,
#56501,#56502,#56503,#56504,#56505,#56506,#56507,#56508,#56509,#56510,#56511,
#56512,#56513,#56514,#56515,#56516,#56517,#56518,#56519,#56520,#56521,#56522,
#56523,#56524,#56525,#56526,#56527,#56528,#56529),.UNSPECIFIED.,.F.,.F.,
(4,3,3,3,3,3,3,3,3,3,3,3,3,3,3,3,3,3,3,3,3,3,3,3,3,3,3,3,3,3,3,3,3,3,3,
3,3,3,3,3,3,3,3,3,3,3,3,3,3,3,3,3,3,3,3,3,3,3,3,3,3,3,3,3,3,3,3,3,3,3,3,
3,3,3,3,3,3,3,3,3,3,3,3,3,3,3,3,3,4),(-374.800863543726,-374.719546014481,
-374.637804672318,-374.555849675824,-374.473567339188,-374.403003019094,
-374.32837995368,-374.2538426248,-374.179377136047,-374.104969638405,-374.030606321163,
-373.956273403262,-373.881946940668,-373.807620608713,-373.733281949916,
-373.658918502638,-373.584483245456,-373.510006772065,-373.435440399924,
-373.404595011043,-373.326229337001,-373.247960167562,-373.169782221164,
-373.091721448973,-373.013732386718,-372.935832533722,-372.905391007017,
-372.827480418904,-372.749500022002,-372.671444692142,-372.593259976388,
-372.515004596782,-372.436629906146,-372.406187002992,-372.331627906465,
-372.257144256853,-372.182722193748,-372.10834789731,-372.034007579519,
-371.959687475773,-371.885358606614,-371.811020373423,-371.736660315073,
-371.66226596127,-371.587785607698,-371.513255854697,-371.438624123855,
-371.407778994941,-371.333859208664,-371.260026233307,-371.186265607679,
-371.112562924151,-371.038903817516,-370.965273954686,-370.891646879009,
-370.818017649969,-370.744373312206,-370.670700903746,-370.596948576309,
-370.523151425474,-370.449253398825,-370.40937098689,-370.334809925361,
-370.260329697704,-370.18591639067,-370.111556135232,-370.0372350976,-369.962939470652,
-369.888642734953,-369.814341405412,-369.740022992087,-369.66567499836,
-369.591247882207,-369.516775375414,-369.442206549955,-369.410962978839,
-369.337414086104,-369.263945524044,-369.190542599154,-369.117190671653,
-369.042251617264,-368.968950350266,-368.895652939365,-368.822346207468,
-368.746179214737,-368.672781983367,-368.599343700407,-368.525824158253,
-368.517678236546),.UNSPECIFIED.);
#514=B_SPLINE_CURVE_WITH_KNOTS('',3,(#56531,#56532,#56533,#56534,#56535,
#56536,#56537,#56538,#56539,#56540,#56541,#56542,#56543,#56544,#56545,#56546,
#56547,#56548,#56549,#56550,#56551,#56552,#56553,#56554,#56555,#56556,#56557,
#56558,#56559,#56560,#56561,#56562,#56563,#56564,#56565,#56566,#56567,#56568,
#56569,#56570,#56571,#56572,#56573,#56574,#56575,#56576,#56577,#56578,#56579,
#56580,#56581,#56582,#56583,#56584,#56585,#56586,#56587,#56588,#56589,#56590,
#56591,#56592,#56593,#56594,#56595,#56596,#56597,#56598,#56599,#56600,#56601,
#56602,#56603,#56604,#56605,#56606,#56607,#56608,#56609,#56610,#56611,#56612,
#56613,#56614,#56615,#56616,#56617,#56618,#56619,#56620,#56621,#56622,#56623,
#56624,#56625,#56626,#56627,#56628,#56629,#56630,#56631,#56632,#56633,#56634,
#56635,#56636,#56637,#56638,#56639,#56640,#56641,#56642,#56643,#56644,#56645,
#56646,#56647,#56648,#56649,#56650,#56651,#56652,#56653,#56654,#56655,#56656,
#56657,#56658,#56659,#56660,#56661,#56662,#56663,#56664,#56665,#56666,#56667,
#56668,#56669,#56670,#56671,#56672,#56673,#56674,#56675,#56676,#56677,#56678,
#56679,#56680,#56681,#56682,#56683,#56684,#56685,#56686,#56687,#56688,#56689,
#56690,#56691,#56692,#56693,#56694,#56695,#56696,#56697,#56698,#56699,#56700,
#56701,#56702,#56703,#56704,#56705,#56706,#56707,#56708,#56709,#56710,#56711,
#56712,#56713,#56714,#56715,#56716,#56717,#56718,#56719,#56720,#56721,#56722,
#56723,#56724,#56725,#56726,#56727,#56728,#56729,#56730,#56731,#56732,#56733,
#56734,#56735,#56736,#56737,#56738,#56739,#56740,#56741,#56742,#56743,#56744,
#56745,#56746,#56747,#56748,#56749,#56750,#56751,#56752,#56753,#56754,#56755,
#56756,#56757,#56758,#56759,#56760,#56761,#56762,#56763,#56764,#56765,#56766,
#56767,#56768,#56769,#56770,#56771,#56772,#56773,#56774,#56775,#56776,#56777,
#56778,#56779,#56780,#56781,#56782,#56783,#56784,#56785,#56786,#56787,#56788,
#56789,#56790,#56791,#56792,#56793,#56794,#56795,#56796,#56797,#56798,#56799,
#56800,#56801,#56802,#56803,#56804,#56805,#56806,#56807,#56808,#56809,#56810,
#56811,#56812,#56813,#56814,#56815,#56816,#56817,#56818,#56819,#56820,#56821,
#56822,#56823,#56824,#56825,#56826,#56827,#56828,#56829,#56830,#56831,#56832,
#56833,#56834,#56835,#56836,#56837,#56838,#56839,#56840,#56841,#56842,#56843,
#56844,#56845,#56846,#56847,#56848,#56849,#56850,#56851,#56852,#56853,#56854,
#56855,#56856,#56857,#56858,#56859,#56860,#56861,#56862,#56863,#56864,#56865,
#56866,#56867,#56868,#56869,#56870,#56871,#56872,#56873,#56874,#56875,#56876,
#56877,#56878,#56879,#56880,#56881,#56882,#56883,#56884,#56885,#56886,#56887,
#56888,#56889,#56890,#56891,#56892,#56893,#56894,#56895,#56896,#56897,#56898,
#56899,#56900,#56901,#56902,#56903,#56904,#56905,#56906,#56907,#56908,#56909,
#56910,#56911,#56912,#56913,#56914,#56915,#56916,#56917,#56918,#56919,#56920,
#56921,#56922,#56923,#56924,#56925,#56926,#56927,#56928,#56929,#56930,#56931,
#56932,#56933,#56934,#56935,#56936,#56937,#56938,#56939,#56940,#56941,#56942,
#56943,#56944,#56945,#56946,#56947,#56948,#56949,#56950,#56951,#56952,#56953,
#56954,#56955,#56956,#56957,#56958,#56959,#56960,#56961,#56962,#56963,#56964,
#56965,#56966,#56967,#56968,#56969,#56970,#56971,#56972,#56973,#56974,#56975,
#56976,#56977,#56978,#56979,#56980,#56981,#56982,#56983,#56984,#56985,#56986,
#56987,#56988,#56989,#56990,#56991,#56992,#56993,#56994,#56995,#56996,#56997,
#56998,#56999,#57000,#57001,#57002,#57003,#57004,#57005,#57006,#57007,#57008,
#57009,#57010,#57011,#57012,#57013,#57014,#57015,#57016,#57017,#57018,#57019,
#57020,#57021,#57022,#57023,#57024,#57025,#57026,#57027,#57028,#57029,#57030,
#57031,#57032,#57033,#57034,#57035,#57036,#57037,#57038,#57039,#57040,#57041,
#57042,#57043,#57044,#57045,#57046,#57047,#57048,#57049,#57050,#57051,#57052,
#57053,#57054,#57055,#57056,#57057,#57058,#57059,#57060,#57061,#57062,#57063,
#57064,#57065,#57066,#57067,#57068,#57069,#57070,#57071,#57072,#57073,#57074,
#57075,#57076,#57077,#57078,#57079,#57080,#57081,#57082,#57083,#57084,#57085,
#57086,#57087,#57088,#57089,#57090,#57091,#57092,#57093,#57094,#57095,#57096,
#57097,#57098,#57099,#57100,#57101,#57102,#57103,#57104),.UNSPECIFIED.,
 .F.,.F.,(4,2,2,2,2,2,2,2,2,2,2,2,2,2,2,2,2,2,2,2,2,2,2,2,2,2,2,2,2,2,2,
2,2,2,2,2,2,2,2,2,2,2,2,2,2,2,2,2,2,2,2,2,2,2,2,2,2,2,2,2,2,2,2,2,2,2,2,
2,2,2,2,2,2,2,2,2,2,2,2,2,2,2,2,2,2,2,2,2,2,2,2,2,2,2,2,2,2,2,2,2,2,2,2,
2,2,2,2,2,2,2,2,2,2,2,2,2,2,2,2,2,2,2,2,2,2,2,2,2,2,2,2,2,2,2,2,2,2,2,2,
2,2,2,2,2,2,2,2,2,2,2,2,2,2,2,2,2,2,2,2,2,2,2,2,2,2,2,2,2,2,2,2,2,2,2,2,
2,2,2,2,2,2,2,2,2,2,2,2,2,2,2,2,2,2,2,2,2,2,2,2,2,2,2,2,2,2,2,2,2,2,2,2,
2,2,2,2,2,2,2,2,2,2,2,2,2,2,2,2,2,2,2,2,2,2,2,2,2,2,2,2,2,2,2,2,2,2,2,2,
2,2,2,2,2,2,2,2,2,2,2,2,2,2,2,2,2,2,2,2,2,2,2,2,2,2,2,2,2,2,2,2,2,2,2,2,
2,2,2,4),(0.00175903982440652,0.0619033949982958,0.0773251103339988,0.0793500364310013,
0.0806404128587861,0.0816337458300343,0.0826032683097308,0.0835626793958884,
0.0848899579511312,0.0883523287965929,0.13715083610504,0.157413074338618,
0.164171423162419,0.339089179933081,0.417864966959503,0.464742709937004,
0.47350788403339,0.476434200940765,0.478330286045617,0.480120734003368,
0.482481703792499,0.487750323666294,0.531505480165916,0.534036325308417,
0.540303918898397,0.545528498615362,0.562145795789653,0.780130183370125,
0.835391076207062,0.859452222108224,0.871355019724401,0.873545253277799,
0.874511497419455,0.875447174514417,0.876373425657873,0.877657157433084,
0.880254562304033,0.903782286123755,0.907724907334266,0.937361825917045,
0.948168304158819,1.02756118071958,1.03679852734077,1.04720568688562,1.05901661766314,
1.07253732293115,1.08819529895498,1.10663396019865,1.16988511765201,1.27926667323192,
1.28463039311485,1.28704670078533,1.28885109600663,1.29053551032943,1.29284879527928,
1.29868312701384,1.36607439219648,1.49035282391027,1.60717879828619,1.64604329211697,
1.66788418346017,1.67581966402046,1.67953857275252,1.68166549731746,1.68312526544564,
1.68452927587427,1.68580461329873,1.68746787804002,1.69086477157092,1.71162488274356,
1.84610989817839,2.04056119865127,2.05393970939231,2.05852490886575,2.06153214825909,
2.06438863731001,2.06815180312257,2.07654525239088,2.15045665748907,2.3221263790503,
2.38171141127265,2.41687348194745,2.42789281003331,2.43257060862904,2.43506600303702,
2.43667891686166,2.43818605243424,2.43942716000428,2.44093952712982,2.44354948377633,
2.4534205953433,2.59011544409689,2.68090675441139,2.73966728565225,2.81502691635214,
2.82907683762242,2.83256627392893,2.83459854643679,2.8363746279343,2.83856539076809,
2.84189738186162,2.85627590056278,2.8603892452858,3.13703601602355,3.20541644448914,
3.24039705374321,3.24420575138112,3.24619416785437,3.2478775302273,3.24892895054535,
3.24991464050417,3.25118042953033,3.2532565238506,3.26449720238799,3.44281498087408,
3.5522529640981,3.62823985548881,3.6401125495251,3.64338722574311,3.64536141320717,
3.64712899430856,3.64936570382018,3.65287525861323,3.66970782740594,3.95572751606245,
4.00264534326786,4.03440094833861,4.0398309353522,4.04153329595158,4.04262371744316,
4.04364663764598,4.04498566811218,4.04793243059222,4.07096687403263,4.07601931075552,
4.07801948007068,4.0832477480956,4.08871767295861,4.10029896442959,4.33481028609234,
4.4233746373646,4.43651076981224,4.43999197069271,4.44206254036525,4.44389882548904,
4.44619904581248,4.44976383328471,4.46614762519994,4.74400952150499,4.77572423849033,
4.82225795153851,4.82924474520577,4.83116587782632,4.83232247843113,4.83325197579703,
4.83452850708019,4.8364782614903,4.84499939117204,4.98069672908429,5.160018458876,
5.17487295770866,5.21314063518914,5.21835418281805,5.22076134320313,5.22261669443289,
5.22461075519972,5.22774900273032,5.23761755817871,5.42006113909995,5.60613756515104,
5.60839688187197,5.61806223719701,5.62007415904981,5.6213551636993,5.62236698397053,
5.62349644945202,5.62537809546184,5.63256420611471,5.6831709036341,5.73920533537026,
5.78748703504006,5.88912268771359,6.00592908500263,6.01346612221099,6.01631885317761,
6.01801161062242,6.01961320755682,6.02184384889773,6.02630544781578,6.06073129983565,
6.15390288875623,6.39004414485309,6.41061090996926,6.41339980704797,6.41468471264851,
6.41567369960073,6.41673882154944,6.41844018530934,6.42400253278825,6.4571395404516,
6.53159202589756,6.59237132618945,6.71768849745545,6.81773254002068,6.82440984208749,
6.82686140267966,6.82858365021243,6.83031193086043,6.83253688150836,6.83697302979643,
6.84264203086998,6.88715528697601,6.96510940595954,7.20692725140058,7.22076437161491,
7.22345093128765,7.22512950898651,7.22643411553023,7.22786889930314,7.23019835318589,
7.23814923026575,7.43340579013368,7.58605908205236,7.59624568242833,7.60005874858824,
7.60301523198508,7.60586806609863,7.60966441949961,7.61800433433649,7.80136421371316,
7.93302758586372,7.97373420887745,7.97783600506985,7.97945435497719,7.98066614718158,
7.98199698234236,7.98383866049691,7.98818978065292,8.09208681021082,8.18490874218475,
8.3150025855144,8.36800820606732,8.37303973938585,8.37546000281852,8.3771739963735,
8.37889618165677,8.38113941090526,8.38532662697681,8.39080289884384,8.40287658238937,
8.43746430230672,8.51477168194802,8.77353773155922,8.78740062702841,8.78983264510202,
8.79107295264083,8.79205234488855,8.7931548385238,8.79500399991749,8.80192305162432,
8.84930216261481,8.92330365192968,9.01454515107542,9.06891042081912,9.17661297365186,
9.18385459680458,9.18638021289148,9.18811494060852,9.18984723203075,9.19200841457564,
9.19434986416638,9.19808861922751,9.20532140466049,9.22289991172767,9.26823496600275,
9.3264499243663,9.56070762949262,9.58073970506991,9.58351779358425,9.58481628221867,
9.58583361657385,9.58694351643894,9.58872561496557,9.59462416432671,9.63031753343889,
9.67840012039954,9.96492602872158),.UNSPECIFIED.);
#515=B_SPLINE_CURVE_WITH_KNOTS('',3,(#57106,#57107,#57108,#57109,#57110,
#57111,#57112,#57113,#57114,#57115,#57116,#57117,#57118,#57119,#57120,#57121,
#57122,#57123),.UNSPECIFIED.,.F.,.F.,(4,2,2,2,2,2,2,2,4),(-355.951307622187,
-355.116390710292,-354.281473798397,-353.446556886502,-352.611639974607,
-351.776723062712,-350.941806150818,-350.106889238923,-349.668122315007),
 .UNSPECIFIED.);
#516=B_SPLINE_CURVE_WITH_KNOTS('',3,(#57125,#57126,#57127,#57128,#57129,
#57130,#57131,#57132,#57133,#57134,#57135,#57136,#57137,#57138,#57139,#57140,
#57141,#57142),.UNSPECIFIED.,.F.,.F.,(4,2,2,2,2,2,2,2,4),(-349.668122315007,
-348.833205403113,-347.998288491218,-347.163371579323,-346.328454667428,
-345.493537755533,-344.658620843639,-343.823703931744,-343.385155491413),
 .UNSPECIFIED.);
#517=B_SPLINE_CURVE_WITH_KNOTS('',3,(#57144,#57145,#57146,#57147,#57148,
#57149,#57150,#57151,#57152,#57153,#57154),.UNSPECIFIED.,.F.,.F.,(4,1,1,
1,1,1,1,1,4),(-343.384486891376,-342.453946761465,-341.455538753414,-340.457130745363,
-339.458722737312,-338.460314729261,-337.961110725235,-337.46190672121,
-337.101751700648),.UNSPECIFIED.);
#518=B_SPLINE_CURVE_WITH_KNOTS('',3,(#57156,#57157,#57158,#57159,#57160,
#57161,#57162,#57163,#57164,#57165,#57166,#57167,#57168,#57169,#57170,#57171,
#57172,#57173),.UNSPECIFIED.,.F.,.F.,(4,2,2,2,2,2,2,2,4),(-337.101751700648,
-336.266834788753,-335.431917876858,-334.597000964964,-333.762084053069,
-332.927167141174,-332.092250229279,-331.257333317384,-330.818566393469),
 .UNSPECIFIED.);
#519=B_SPLINE_CURVE_WITH_KNOTS('',3,(#57175,#57176,#57177,#57178,#57179,
#57180,#57181,#57182,#57183,#57184,#57185,#57186,#57187,#57188,#57189,#57190,
#57191,#57192,#57193,#57194,#57195,#57196,#57197,#57198,#57199,#57200,#57201,
#57202,#57203,#57204,#57205,#57206,#57207,#57208,#57209,#57210,#57211,#57212,
#57213,#57214,#57215,#57216,#57217,#57218,#57219,#57220,#57221,#57222,#57223,
#57224,#57225,#57226,#57227,#57228,#57229,#57230,#57231,#57232,#57233,#57234,
#57235,#57236,#57237,#57238,#57239,#57240,#57241,#57242,#57243,#57244,#57245,
#57246,#57247,#57248,#57249,#57250,#57251,#57252,#57253,#57254,#57255,#57256,
#57257,#57258,#57259,#57260,#57261,#57262,#57263,#57264,#57265,#57266,#57267,
#57268,#57269,#57270,#57271,#57272,#57273,#57274,#57275,#57276,#57277,#57278,
#57279,#57280,#57281,#57282,#57283,#57284,#57285,#57286,#57287,#57288,#57289,
#57290,#57291,#57292,#57293,#57294,#57295,#57296,#57297,#57298,#57299,#57300,
#57301,#57302,#57303,#57304,#57305,#57306,#57307,#57308,#57309,#57310,#57311,
#57312,#57313,#57314,#57315,#57316,#57317,#57318,#57319,#57320,#57321,#57322,
#57323,#57324,#57325,#57326,#57327,#57328,#57329,#57330,#57331,#57332,#57333,
#57334,#57335,#57336,#57337,#57338,#57339,#57340,#57341,#57342,#57343,#57344,
#57345,#57346,#57347,#57348,#57349,#57350,#57351,#57352,#57353,#57354,#57355,
#57356,#57357,#57358,#57359,#57360,#57361,#57362,#57363,#57364,#57365,#57366,
#57367,#57368,#57369,#57370,#57371,#57372,#57373,#57374,#57375,#57376,#57377,
#57378,#57379,#57380,#57381,#57382,#57383,#57384,#57385,#57386,#57387,#57388,
#57389,#57390,#57391,#57392,#57393,#57394,#57395,#57396,#57397,#57398,#57399,
#57400,#57401,#57402,#57403,#57404,#57405,#57406,#57407,#57408,#57409,#57410,
#57411,#57412,#57413,#57414,#57415,#57416,#57417,#57418,#57419,#57420,#57421,
#57422,#57423,#57424,#57425,#57426,#57427,#57428,#57429,#57430,#57431,#57432,
#57433,#57434,#57435,#57436),.UNSPECIFIED.,.F.,.F.,(4,3,3,3,3,3,3,3,3,3,
3,3,3,3,3,3,3,3,3,3,3,3,3,3,3,3,3,3,3,3,3,3,3,3,3,3,3,3,3,3,3,3,3,3,3,3,
3,3,3,3,3,3,3,3,3,3,3,3,3,3,3,3,3,3,3,3,3,3,3,3,3,3,3,3,3,3,3,3,3,3,3,3,
3,3,3,3,3,4),(-330.818566393469,-330.732187461315,-330.647974550361,-330.560512607607,
-330.473050664853,-330.398491568327,-330.324007918715,-330.249585855612,
-330.175211559175,-330.100871241385,-330.026551137639,-329.952222268481,
-329.877884035291,-329.803523976941,-329.72912962314,-329.654649269568,
-329.580119516568,-329.505487785727,-329.474642656803,-329.400722870526,
-329.326889895169,-329.253129269541,-329.179426586013,-329.105767479378,
-329.032137616548,-328.958510540871,-328.884881311831,-328.811236974068,
-328.737564565608,-328.663812238171,-328.590015087337,-328.516117060688,
-328.476234648752,-328.401673587223,-328.327193359566,-328.252780052532,
-328.178419797093,-328.104098759462,-328.029803132513,-327.955506396813,
-327.881205067272,-327.806886653947,-327.732538660221,-327.658111544067,
-327.583639037274,-327.509070211814,-327.477826640701,-327.403265654567,
-327.328785490181,-327.254372234338,-327.180012018046,-327.105691007541,
-327.03139539572,-326.957098657212,-326.882797313677,-326.808478875168,
-326.734130845056,-326.659703675792,-326.585231106247,-326.510662203788,
-326.47941863265,-326.405525151396,-326.331714285254,-326.257971589831,
-326.184282670936,-326.110633173709,-326.037008772525,-325.963380925599,
-325.889747059531,-325.816094217316,-325.742409433107,-325.668638880209,
-325.594820169594,-325.520895518727,-325.481010624599,-325.406897287707,
-325.332869248636,-325.258912171831,-325.185011772281,-325.11115380508,
-325.037318033266,-324.963492534632,-324.889664458657,-324.815820955436,
-324.741913564608,-324.667972525697,-324.593939371745,-324.535655273961),
 .UNSPECIFIED.);
#520=B_SPLINE_CURVE_WITH_KNOTS('',3,(#57438,#57439,#57440,#57441,#57442,
#57443,#57444,#57445,#57446,#57447,#57448,#57449,#57450,#57451,#57452,#57453,
#57454,#57455,#57456,#57457,#57458,#57459,#57460,#57461,#57462,#57463,#57464,
#57465,#57466,#57467,#57468,#57469,#57470,#57471,#57472,#57473,#57474,#57475,
#57476,#57477,#57478,#57479,#57480,#57481,#57482,#57483,#57484,#57485,#57486,
#57487,#57488,#57489,#57490,#57491,#57492,#57493,#57494,#57495,#57496,#57497,
#57498,#57499,#57500,#57501,#57502,#57503,#57504,#57505,#57506,#57507,#57508,
#57509,#57510,#57511,#57512,#57513,#57514,#57515,#57516,#57517,#57518,#57519,
#57520,#57521,#57522,#57523,#57524,#57525,#57526,#57527,#57528,#57529,#57530,
#57531,#57532,#57533,#57534,#57535,#57536,#57537,#57538,#57539,#57540,#57541,
#57542,#57543,#57544,#57545,#57546,#57547,#57548,#57549,#57550,#57551,#57552,
#57553,#57554,#57555,#57556,#57557,#57558,#57559,#57560,#57561,#57562,#57563,
#57564,#57565,#57566,#57567,#57568,#57569,#57570,#57571,#57572,#57573,#57574,
#57575,#57576,#57577,#57578,#57579,#57580,#57581,#57582,#57583,#57584,#57585,
#57586,#57587,#57588,#57589,#57590,#57591,#57592,#57593,#57594,#57595,#57596,
#57597,#57598,#57599,#57600,#57601,#57602,#57603,#57604,#57605,#57606,#57607,
#57608,#57609,#57610,#57611,#57612,#57613,#57614,#57615,#57616,#57617,#57618,
#57619,#57620,#57621,#57622,#57623,#57624,#57625,#57626,#57627,#57628,#57629,
#57630,#57631,#57632,#57633,#57634,#57635,#57636,#57637,#57638,#57639,#57640,
#57641,#57642,#57643,#57644,#57645,#57646,#57647,#57648,#57649,#57650,#57651,
#57652,#57653,#57654,#57655,#57656,#57657,#57658,#57659,#57660,#57661,#57662,
#57663,#57664,#57665,#57666,#57667,#57668,#57669,#57670,#57671,#57672,#57673,
#57674,#57675,#57676,#57677,#57678,#57679,#57680,#57681,#57682,#57683,#57684,
#57685,#57686,#57687,#57688,#57689,#57690,#57691,#57692,#57693,#57694,#57695,
#57696,#57697,#57698,#57699,#57700,#57701,#57702,#57703,#57704,#57705,#57706,
#57707,#57708,#57709,#57710,#57711,#57712,#57713,#57714,#57715,#57716,#57717,
#57718,#57719,#57720,#57721,#57722,#57723,#57724,#57725,#57726,#57727,#57728,
#57729,#57730,#57731,#57732,#57733,#57734,#57735,#57736,#57737,#57738,#57739,
#57740,#57741,#57742,#57743,#57744,#57745,#57746,#57747,#57748,#57749,#57750,
#57751,#57752,#57753,#57754,#57755,#57756,#57757,#57758,#57759,#57760,#57761,
#57762,#57763,#57764,#57765,#57766,#57767,#57768,#57769,#57770,#57771,#57772,
#57773,#57774,#57775,#57776,#57777,#57778,#57779,#57780,#57781,#57782,#57783,
#57784,#57785,#57786,#57787,#57788,#57789,#57790,#57791,#57792,#57793,#57794,
#57795,#57796,#57797,#57798,#57799,#57800,#57801,#57802,#57803,#57804,#57805,
#57806,#57807,#57808,#57809,#57810,#57811,#57812,#57813,#57814,#57815,#57816,
#57817,#57818,#57819,#57820,#57821,#57822,#57823,#57824,#57825,#57826,#57827,
#57828,#57829,#57830,#57831,#57832,#57833,#57834,#57835,#57836,#57837,#57838,
#57839,#57840,#57841,#57842,#57843,#57844,#57845,#57846,#57847,#57848,#57849,
#57850,#57851,#57852,#57853,#57854,#57855,#57856,#57857,#57858,#57859,#57860,
#57861,#57862,#57863,#57864,#57865,#57866,#57867,#57868,#57869,#57870,#57871,
#57872,#57873,#57874,#57875,#57876,#57877,#57878,#57879,#57880,#57881,#57882,
#57883,#57884,#57885,#57886,#57887,#57888,#57889,#57890,#57891,#57892,#57893,
#57894,#57895,#57896,#57897,#57898,#57899,#57900,#57901,#57902,#57903,#57904,
#57905,#57906,#57907,#57908,#57909,#57910,#57911,#57912,#57913,#57914,#57915,
#57916,#57917,#57918,#57919,#57920,#57921,#57922,#57923,#57924,#57925,#57926,
#57927,#57928,#57929,#57930,#57931,#57932,#57933,#57934,#57935,#57936,#57937,
#57938,#57939,#57940,#57941,#57942,#57943,#57944,#57945,#57946,#57947,#57948,
#57949,#57950,#57951,#57952,#57953,#57954,#57955,#57956,#57957,#57958,#57959,
#57960,#57961,#57962,#57963,#57964,#57965,#57966,#57967,#57968,#57969,#57970,
#57971,#57972,#57973,#57974,#57975,#57976,#57977,#57978,#57979,#57980,#57981,
#57982,#57983,#57984,#57985,#57986,#57987,#57988,#57989,#57990,#57991,#57992,
#57993,#57994,#57995,#57996,#57997,#57998,#57999,#58000,#58001,#58002,#58003,
#58004,#58005,#58006,#58007,#58008,#58009,#58010,#58011,#58012,#58013,#58014,
#58015,#58016,#58017,#58018,#58019,#58020,#58021,#58022,#58023,#58024,#58025,
#58026,#58027,#58028,#58029,#58030,#58031,#58032,#58033,#58034,#58035,#58036,
#58037,#58038,#58039,#58040,#58041),.UNSPECIFIED.,.F.,.F.,(4,2,2,2,2,2,
2,2,2,2,2,2,2,2,2,2,2,2,2,2,2,2,2,2,2,2,2,2,2,2,2,2,2,2,2,2,2,2,2,2,2,2,
2,2,2,2,2,2,2,2,2,2,2,2,2,2,2,2,2,2,2,2,2,2,2,2,2,2,2,2,2,2,2,2,2,2,2,2,
2,2,2,2,2,2,2,2,2,2,2,2,2,2,2,2,2,2,2,2,2,2,2,2,2,2,2,2,2,2,2,2,2,2,2,2,
2,2,2,2,2,2,2,2,2,2,2,2,2,2,2,2,2,2,2,2,2,2,2,2,2,2,2,2,2,2,2,2,2,2,2,2,
2,2,2,2,2,2,2,2,2,2,2,2,2,2,2,2,2,2,2,2,2,2,2,2,2,2,2,2,2,2,2,2,2,2,2,2,
2,2,2,2,2,2,2,2,2,2,2,2,2,2,2,2,2,2,2,2,2,2,2,2,2,2,2,2,2,2,2,2,2,2,2,2,
2,2,2,2,2,2,2,2,2,2,2,2,2,2,2,2,2,2,2,2,2,2,2,2,2,2,2,2,2,2,2,2,2,2,2,2,
2,2,2,2,2,2,2,2,2,2,2,2,2,2,2,2,2,2,2,2,2,2,2,2,2,2,2,2,2,2,2,2,2,2,2,2,
2,2,2,2,2,2,2,4),(0.00136622398944564,0.0549836364701191,0.0575959087568496,
0.0592608135368877,0.0605382522441885,0.0617743502663625,0.0629998489473684,
0.0646756916742249,0.0688645621889766,0.117084529607065,0.122773462059413,
0.131153634355164,0.286044438208657,0.416698022472885,0.430356651377554,
0.434978118346523,0.437992946900742,0.440845169366185,0.444585637914629,
0.450889687103354,0.489749078850845,0.678371606139728,0.715457827701584,
0.760840216312113,0.794122201000565,0.804664488038609,0.809191877773913,
0.812650380643149,0.814320638478753,0.815567921817461,0.816801443060079,
0.818508273664927,0.821943405844319,0.857651705652357,0.864479611526515,
0.949966848352646,0.95910782349341,0.969254789920635,0.980633977839693,
0.993514584864171,1.00825465634677,1.02537115364427,1.08927684796378,1.14284207435874,
1.18362711403943,1.20458526833659,1.20853892283229,1.21067288315403,1.21242906244085,
1.21450016788585,1.21806911105161,1.23153069266861,1.2362757338985,1.49769581269447,
1.57066913504191,1.60142769380722,1.61446364800677,1.62194620323438,1.62383802512198,
1.62476978795356,1.62565040248645,1.6266121987789,1.62831307267665,1.63329999502228,
1.71295078896719,1.71418957342121,1.71541308076413,1.8497374604961,1.86952998751965,
1.89339093147479,1.92900566308549,1.98784532404182,2.01445110218426,2.0186448123843,
2.0208194381931,2.02256497192871,2.02431636472182,2.02746582337276,2.03705831081284,
2.17538338123192,2.2501173478525,2.32373024868085,2.38301787396716,2.40360973903664,
2.41056452709298,2.41367113400105,2.41609819913882,2.41733147041691,2.41824578572452,
2.41921866868889,2.42059477541822,2.42346414283281,2.45399887021593,2.45659144852119,
2.46171223807594,2.46735964086411,2.49994789575026,2.70620281969758,2.79800967133651,
2.81137728312264,2.81487888535627,2.8169535903507,2.81878857839893,2.82108061743515,
2.82462037436985,2.84069759150573,3.08851743177993,3.15465042485733,3.19724728495318,
3.20162231904173,3.20385802729046,3.20573937989056,3.20687343205009,3.2079105908883,
3.20923885952927,3.21135672789564,3.2221000053344,3.39602945880976,3.57417923007587,
3.59008530784042,3.59379763156706,3.5959193330896,3.59756573602103,3.59943285089433,
3.60293355083198,3.61472892441595,3.78405069555577,3.90958447925468,3.9558138625686,
3.98760663077307,3.99309194459957,3.99482503010733,3.99592310314843,3.99694249903544,
3.99826165531829,4.00115883574194,4.02439597057315,4.02960656921686,4.26303270142273,
4.31796713796737,4.37698536162458,4.38713644308349,4.39022951490476,4.39216262995934,
4.39393925279675,4.39621366149945,4.39992804579904,4.40943918638269,4.56584757678512,
4.71857283327626,4.78398178686849,4.78696839442891,4.78830369079372,4.789296614296,
4.79022226772311,4.79150384800621,4.794092828011,4.8173582560741,4.82158581797852,
4.97965523899293,5.04492006435551,5.18681921727791,5.19681175350678,5.20002885019111,
5.2018028506433,5.20357820608608,5.20576248821886,5.20995259080822,5.23586466223165,
5.2920027714497,5.45318364419068,5.58514695881448,5.59431102188089,5.59684829061204,
5.5983435640978,5.59963758623534,5.60121759023072,5.60421174616796,5.62171113723449,
5.65857146842216,5.73879280155077,5.81441968449108,5.95952002348252,5.96884073603031,
5.97251220589428,5.97518045712044,5.97802485511338,5.98178156826293,5.98992144889064,
6.13176725819743,6.32677201448762,6.34678635488243,6.35010334537974,6.35177334704772,
6.35307580732724,6.35451281960426,6.35685617663271,6.36495066419743,6.41383363022294,
6.52942198157384,6.68100534345652,6.7393630837497,6.74497997674114,6.74725575642469,
6.74893041267137,6.75070487577116,6.7530877507837,6.75573102537095,6.76017892325509,
6.86177418736654,7.09448149964857,7.15640282301169,7.16015983454559,7.16151563532281,
7.16246111029065,7.16334629923613,7.16456855205924,7.16697430236636,7.18384376998072,
7.26144323897518,7.38021574846885,7.45359341050738,7.54845133480444,7.55479333226655,
7.55717946658029,7.55887459186821,7.56061637997025,7.56273655802658,7.56513975324901,
7.56902744471967,7.57665887900283,7.64967118996528,7.75679329987061,7.93993301467533,
7.9457540224234,7.95218578688714,7.95407799716185,7.95509618311438,7.9560932114186,
7.95730943038514,7.95957618455766,7.97186221326425,7.99667471615725,8.04469830972115,
8.06734237235833,8.0848381807374,8.12548588831923,8.13470375109014,8.14338038425575,
8.15158103720518,8.1593586919536,8.2692530898096,8.34433037548595,8.35046734830483,
8.35308804001049,8.35495251093868,8.35682064337513,8.35871488630855,8.36369865466696,
8.41508239995064,8.50948338263502,8.71465462538405,8.7391166583074,8.74212183058371,
8.74338626291622,8.74444025812886,8.74552948658939,8.74714718567329,8.75157568685505,
8.85833700198782,8.88400487569615,8.90543087084854,8.98081582127137,9.02742663224101,
9.12254138325966,9.12903743372827,9.13172278728915,9.13360111154788,9.1354565067724,
9.13804303010381,9.14427691528408,9.26741577166684,9.48091372007006,9.52736250495282,
9.53085492284987,9.53219854562552,9.53316282357872,9.53408084640659,9.53536843485012,
9.53801825382757,9.56409286876191,9.64588370684354,9.89942030683067,9.90961703703559,
9.92357694107525,9.9271762621359,9.92924454040451,9.93084517391125,9.93250872590421,
9.93451244944676,9.93745080181594,9.9580269971825),.UNSPECIFIED.);
#521=B_SPLINE_CURVE_WITH_KNOTS('',3,(#58043,#58044,#58045,#58046,#58047,
#58048,#58049,#58050,#58051,#58052,#58053,#58054,#58055,#58056,#58057,#58058,
#58059,#58060,#58061,#58062,#58063,#58064,#58065,#58066,#58067,#58068,#58069,
#58070,#58071,#58072,#58073,#58074,#58075,#58076,#58077,#58078,#58079,#58080,
#58081,#58082,#58083,#58084,#58085,#58086,#58087,#58088,#58089,#58090,#58091,
#58092,#58093,#58094,#58095,#58096,#58097,#58098,#58099,#58100,#58101,#58102,
#58103,#58104,#58105,#58106,#58107,#58108,#58109,#58110,#58111,#58112,#58113,
#58114,#58115,#58116,#58117,#58118,#58119,#58120,#58121,#58122,#58123,#58124,
#58125,#58126,#58127,#58128,#58129,#58130,#58131,#58132,#58133,#58134,#58135,
#58136,#58137,#58138,#58139,#58140,#58141,#58142,#58143,#58144,#58145,#58146,
#58147,#58148,#58149,#58150,#58151,#58152,#58153,#58154,#58155,#58156,#58157,
#58158,#58159,#58160,#58161,#58162,#58163,#58164,#58165,#58166,#58167,#58168,
#58169,#58170,#58171,#58172,#58173,#58174,#58175,#58176,#58177,#58178,#58179,
#58180,#58181,#58182,#58183,#58184,#58185,#58186,#58187,#58188,#58189,#58190,
#58191,#58192,#58193,#58194,#58195,#58196,#58197,#58198,#58199,#58200,#58201,
#58202,#58203,#58204,#58205,#58206,#58207,#58208,#58209,#58210,#58211,#58212,
#58213,#58214,#58215,#58216,#58217,#58218,#58219,#58220,#58221,#58222,#58223,
#58224,#58225,#58226,#58227,#58228,#58229,#58230,#58231,#58232,#58233,#58234,
#58235,#58236,#58237,#58238,#58239,#58240,#58241,#58242,#58243,#58244,#58245,
#58246,#58247,#58248,#58249,#58250,#58251,#58252,#58253,#58254,#58255,#58256,
#58257,#58258,#58259,#58260,#58261,#58262,#58263,#58264,#58265,#58266,#58267,
#58268,#58269,#58270,#58271,#58272,#58273,#58274,#58275,#58276,#58277,#58278,
#58279,#58280,#58281,#58282,#58283,#58284,#58285,#58286,#58287,#58288,#58289,
#58290,#58291,#58292,#58293,#58294,#58295,#58296,#58297,#58298,#58299,#58300,
#58301,#58302,#58303,#58304,#58305,#58306,#58307,#58308,#58309,#58310,#58311,
#58312,#58313,#58314,#58315,#58316,#58317,#58318,#58319,#58320,#58321,#58322,
#58323,#58324,#58325,#58326,#58327,#58328,#58329,#58330,#58331,#58332,#58333,
#58334,#58335,#58336,#58337,#58338,#58339,#58340,#58341,#58342,#58343,#58344,
#58345,#58346,#58347,#58348,#58349,#58350,#58351,#58352,#58353,#58354,#58355,
#58356,#58357,#58358,#58359,#58360,#58361,#58362,#58363,#58364,#58365,#58366,
#58367,#58368,#58369,#58370,#58371,#58372,#58373,#58374,#58375,#58376,#58377,
#58378,#58379,#58380,#58381,#58382,#58383,#58384,#58385,#58386,#58387,#58388,
#58389,#58390,#58391,#58392,#58393,#58394,#58395,#58396,#58397,#58398,#58399,
#58400,#58401,#58402,#58403,#58404,#58405,#58406,#58407,#58408,#58409,#58410,
#58411,#58412,#58413,#58414,#58415,#58416,#58417,#58418,#58419,#58420,#58421,
#58422,#58423,#58424,#58425,#58426,#58427,#58428,#58429,#58430,#58431,#58432,
#58433,#58434,#58435,#58436,#58437,#58438,#58439,#58440,#58441,#58442,#58443,
#58444,#58445,#58446,#58447,#58448,#58449,#58450,#58451,#58452,#58453,#58454,
#58455,#58456,#58457,#58458,#58459,#58460,#58461,#58462,#58463,#58464,#58465,
#58466,#58467,#58468,#58469,#58470,#58471,#58472,#58473,#58474,#58475,#58476,
#58477,#58478,#58479,#58480,#58481,#58482,#58483,#58484,#58485,#58486,#58487,
#58488,#58489,#58490,#58491,#58492,#58493,#58494,#58495,#58496,#58497,#58498,
#58499,#58500,#58501,#58502,#58503,#58504,#58505,#58506,#58507,#58508,#58509,
#58510,#58511,#58512,#58513,#58514,#58515,#58516,#58517,#58518,#58519,#58520,
#58521,#58522,#58523,#58524,#58525,#58526,#58527,#58528,#58529,#58530,#58531,
#58532,#58533,#58534,#58535,#58536,#58537,#58538,#58539,#58540,#58541,#58542,
#58543,#58544,#58545,#58546,#58547,#58548,#58549,#58550,#58551,#58552,#58553,
#58554,#58555,#58556,#58557,#58558,#58559,#58560,#58561,#58562,#58563,#58564,
#58565,#58566,#58567,#58568,#58569,#58570,#58571,#58572,#58573,#58574,#58575,
#58576,#58577,#58578,#58579,#58580,#58581,#58582,#58583,#58584,#58585,#58586,
#58587,#58588,#58589,#58590,#58591,#58592,#58593,#58594,#58595,#58596,#58597,
#58598,#58599,#58600,#58601,#58602,#58603,#58604,#58605,#58606,#58607,#58608,
#58609,#58610,#58611,#58612,#58613,#58614,#58615,#58616,#58617,#58618,#58619,
#58620,#58621,#58622,#58623,#58624,#58625,#58626,#58627,#58628,#58629,#58630,
#58631,#58632,#58633,#58634,#58635,#58636,#58637,#58638,#58639,#58640,#58641,
#58642),.UNSPECIFIED.,.F.,.F.,(4,2,2,2,2,2,2,2,2,2,2,2,2,2,2,2,2,2,2,2,
2,2,2,2,2,2,2,2,2,2,2,2,2,2,2,2,2,2,2,2,2,2,2,2,2,2,2,2,2,2,2,2,2,2,2,2,
2,2,2,2,2,2,2,2,2,2,2,2,2,2,2,2,2,2,2,2,2,2,2,2,2,2,2,2,2,2,2,2,2,2,2,2,
2,2,2,2,2,2,2,2,2,2,2,2,2,2,2,2,2,2,2,2,2,2,2,2,2,2,2,2,2,2,2,2,2,2,2,2,
2,2,2,2,2,2,2,2,2,2,2,2,2,2,2,2,2,2,2,2,2,2,2,2,2,2,2,2,2,2,2,2,2,2,2,2,
2,2,2,2,2,2,2,2,2,2,2,2,2,2,2,2,2,2,2,2,2,2,2,2,2,2,2,2,2,2,2,2,2,2,2,2,
2,2,2,2,2,2,2,2,2,2,2,2,2,2,2,2,2,2,2,2,2,2,2,2,2,2,2,2,2,2,2,2,2,2,2,2,
2,2,2,2,2,2,2,2,2,2,2,2,2,2,2,2,2,2,2,2,2,2,2,2,2,2,2,2,2,2,2,2,2,2,2,2,
2,2,2,2,2,2,2,2,2,2,2,2,2,2,2,2,2,2,2,2,2,2,2,2,2,2,2,4),(0.00206444117643367,
0.25427431608748,0.339067277347239,0.366399914497447,0.369061434760028,
0.370335247392758,0.371228429494803,0.372155344558195,0.373441236097224,
0.376046839704919,0.399823501786385,0.40241207047523,0.4026545356114,0.404864726580252,
0.407130600099304,0.409767078590461,0.411645952746294,0.419848751972015,
0.427270563141598,0.444946466908281,0.673772008220203,0.713191162614711,
0.7555123015024,0.777504155471055,0.78150229940178,0.783259178941547,0.784957261209794,
0.78663663324531,0.788930496568503,0.794651364311366,0.857185395057024,
0.926461665957577,0.972825146685942,1.05650480205845,1.12550004865115,1.15920049507532,
1.17569845060946,1.17864228241125,1.18021179553869,1.18138039652398,1.1826559664504,
1.1849094593692,1.19150880487733,1.30059208763602,1.40326557985149,1.5397807850755,
1.55065497057407,1.55488116716038,1.55781249227586,1.560652047084,1.56457398684755,
1.57348018923723,1.67899289130392,1.83091352603107,1.88509382078349,1.92414976652091,
1.93091139458827,1.93310332441546,1.93450668512066,1.9358198647796,1.93753408548038,
1.94128878902606,1.97433812524604,2.22326212126178,2.31257757723106,2.32109345218367,
2.32531609963515,2.32879963531253,2.33081733474463,2.33241286389285,2.33449352633316,
2.33810369138847,2.35198610581368,2.53765465498566,2.64981294354697,2.69618541992743,
2.73558363437747,2.74177836078784,2.74354731857468,2.74462686089695,2.74561037614764,
2.74688394018323,2.74894112955727,2.7598907940736,2.92997030265151,3.04230941574737,
3.13091685377812,3.13518458002826,3.13774633050417,3.14006615415957,3.14181852299347,
3.14349091243715,3.14579263247026,3.15162383273341,3.22031097737794,3.44198244811632,
3.53238790623307,3.53556798627373,3.53695164468424,3.53797767127976,3.53893043805087,
3.54023103646255,3.54346969333043,3.5783825105287,3.58367792980028,3.59541906151467,
3.78245951239566,3.92769609853722,3.93332771277499,3.93583849792533,3.93770303021958,
3.93943612865611,3.94180474663939,3.94771935640704,4.01307630757973,4.22564608669173,
4.28082937555888,4.31752831320715,4.3235686323625,4.32539047917649,4.32652444061578,
4.32756757043276,4.32891860880413,4.33116026160005,4.3438594230423,4.57367390309785,
4.63301584912154,4.69939728164292,4.71047233928644,4.71374672727321,4.71577036987524,
4.71761500046117,4.71999492430083,4.72493778518826,4.75692456115181,4.76082680167905,
4.76969162719881,4.77577112103574,4.79694903348135,4.98078786716294,5.01442476688674,
5.08069816059329,5.0830339466468,5.08494521092472,5.11037248331752,5.11340204678713,
5.1147558829414,5.11578085566193,5.11686461758359,5.11853806882708,5.12372880799352,
5.15328219438149,5.22180857063446,5.3691834022681,5.49819792987428,5.50657693398901,
5.50955679095335,5.51127388586721,5.51286612230062,5.51503369824752,5.51919526687294,
5.5450350833803,5.60114540550497,5.69772539950262,5.73745491140066,5.78091176263103,
5.89676209437594,5.90454857878548,5.90654815858638,5.90769532102681,5.90857228003648,
5.90970739990934,5.91172770244974,5.92089420512607,5.93789589720552,6.01546775262138,
6.12973379528788,6.30335351632527,6.3153507533736,6.31876683451587,6.32080212768807,
6.32257743616542,6.3247628737941,6.32895894639734,6.35501921408713,6.41172079298135,
6.51948258252078,6.63158643549496,6.70853586175171,6.7140851858047,6.71618358385647,
6.71742755931257,6.71870862528055,6.72036767146531,6.72219237612246,6.72519473094039,
6.73122800761504,6.78456977716475,6.93329597709434,7.07831315188783,7.08767636887057,
7.09135480854045,7.09402454255856,7.09686727712101,7.10061619099023,7.10871717976492,
7.24318436812602,7.43386226117847,7.46483461022097,7.46864804590523,7.47037291523631,
7.4716874519614,7.47305756489847,7.47515999696972,7.47758980986699,7.4820625745571,
7.51836372627306,7.57311000537312,7.80863370073895,7.85860202587526,7.86354818627313,
7.86594588987164,7.86765231124158,7.86926508762447,7.87150850442997,7.87598550855356,
7.9100650954623,8.00298056291935,8.02811508438221,8.04787397645065,8.05574823112596,
8.18274243880661,8.22431862697358,8.23345964133844,8.23630691607363,8.2430612220221,
8.27569808155605,8.27879071212485,8.28003919289574,8.28095624728956,8.2819547313747,
8.28294216818475,8.28533428064562,8.30204550286421,8.31565383282046,8.37478252038758,
8.42915885616388,8.65585175120397,8.67103334244475,8.67441359293433,8.67660937778111,
8.67837188007698,8.68036951869516,8.6837527936194,8.69680390794285,8.78801852432739,
8.81460594920854,8.83513705550795,8.85186178914556,8.86588208597962,8.877843906523,
8.88816962342697,8.89715695700585,8.96897369035021,8.99595240162936,9.01300327628705,
9.0456575410992,9.06850891022486,9.07139106781341,9.07270705278876,9.07372547807939,
9.07482397217211,9.07594845958547,9.07941229017193,9.08421522023498,9.09661652830864,
9.14387530061798,9.19667652314135,9.44942145331006,9.45607473128349,9.46528147473302,
9.46924659903031,9.47164214120946,9.47349396662997,9.47548960372275,9.47864165148474,
9.48864509131477,9.67383961418688,9.76497271985972,9.77251460448592,9.8537716397057,
9.85899437679942,9.86078353544733,9.8617972301364,9.86272925281889,9.86372016723375,
9.86496178249052,9.86684782188861,9.87030959177873,9.95674259834603),
 .UNSPECIFIED.);
#522=B_SPLINE_CURVE_WITH_KNOTS('',3,(#58644,#58645,#58646,#58647,#58648,
#58649,#58650,#58651,#58652,#58653,#58654),.UNSPECIFIED.,.F.,.F.,(4,1,1,
1,1,1,1,1,4),(-299.40224579153,-298.523994407224,-297.525586399173,-296.527178391122,
-296.027974387097,-295.528770383071,-294.530362375021,-293.53195436697,
-293.119454550391),.UNSPECIFIED.);
#523=B_SPLINE_CURVE_WITH_KNOTS('',3,(#58656,#58657,#58658,#58659,#58660,
#58661,#58662,#58663,#58664,#58665,#58666,#58667,#58668,#58669,#58670,#58671,
#58672,#58673,#58674,#58675,#58676,#58677,#58678,#58679,#58680,#58681,#58682,
#58683,#58684,#58685,#58686,#58687,#58688,#58689,#58690,#58691,#58692,#58693,
#58694,#58695,#58696,#58697,#58698,#58699,#58700,#58701,#58702,#58703,#58704,
#58705,#58706,#58707,#58708,#58709,#58710,#58711,#58712,#58713,#58714,#58715,
#58716,#58717,#58718,#58719,#58720,#58721,#58722,#58723,#58724,#58725,#58726,
#58727,#58728,#58729,#58730,#58731,#58732,#58733,#58734,#58735,#58736,#58737,
#58738,#58739,#58740,#58741,#58742,#58743,#58744,#58745,#58746,#58747,#58748,
#58749,#58750,#58751,#58752,#58753,#58754,#58755,#58756,#58757,#58758,#58759,
#58760,#58761,#58762,#58763,#58764,#58765,#58766,#58767,#58768,#58769,#58770,
#58771,#58772,#58773,#58774,#58775,#58776,#58777,#58778,#58779,#58780,#58781,
#58782,#58783,#58784,#58785,#58786,#58787,#58788,#58789,#58790,#58791,#58792,
#58793,#58794,#58795,#58796,#58797,#58798,#58799,#58800,#58801,#58802,#58803,
#58804,#58805,#58806,#58807,#58808,#58809,#58810,#58811,#58812,#58813,#58814,
#58815,#58816,#58817,#58818,#58819,#58820,#58821,#58822,#58823,#58824,#58825,
#58826,#58827,#58828,#58829,#58830,#58831,#58832,#58833,#58834,#58835,#58836,
#58837,#58838,#58839,#58840,#58841,#58842,#58843,#58844,#58845,#58846,#58847,
#58848,#58849,#58850,#58851,#58852,#58853,#58854,#58855,#58856,#58857,#58858,
#58859,#58860,#58861,#58862,#58863,#58864,#58865,#58866,#58867,#58868,#58869,
#58870,#58871,#58872,#58873,#58874,#58875,#58876,#58877,#58878,#58879,#58880,
#58881,#58882,#58883,#58884,#58885,#58886,#58887,#58888,#58889,#58890,#58891,
#58892,#58893,#58894,#58895,#58896,#58897,#58898,#58899,#58900,#58901,#58902,
#58903,#58904,#58905,#58906,#58907,#58908,#58909,#58910,#58911,#58912,#58913,
#58914,#58915,#58916,#58917,#58918,#58919,#58920,#58921,#58922,#58923,#58924,
#58925,#58926,#58927,#58928,#58929,#58930,#58931,#58932,#58933,#58934,#58935,
#58936,#58937,#58938,#58939,#58940,#58941,#58942,#58943,#58944,#58945,#58946,
#58947,#58948,#58949,#58950,#58951,#58952,#58953,#58954,#58955,#58956,#58957,
#58958,#58959,#58960,#58961,#58962,#58963,#58964,#58965,#58966,#58967,#58968,
#58969,#58970,#58971,#58972,#58973,#58974,#58975,#58976,#58977,#58978,#58979,
#58980,#58981,#58982,#58983,#58984,#58985,#58986,#58987,#58988,#58989,#58990,
#58991,#58992,#58993,#58994,#58995,#58996,#58997,#58998,#58999,#59000,#59001,
#59002,#59003,#59004,#59005,#59006,#59007,#59008,#59009,#59010,#59011,#59012,
#59013,#59014,#59015,#59016,#59017,#59018,#59019,#59020,#59021,#59022,#59023,
#59024,#59025,#59026,#59027,#59028,#59029,#59030,#59031,#59032,#59033,#59034,
#59035,#59036,#59037,#59038,#59039,#59040,#59041,#59042,#59043,#59044,#59045,
#59046,#59047,#59048,#59049,#59050,#59051,#59052,#59053,#59054,#59055,#59056,
#59057,#59058,#59059,#59060,#59061,#59062,#59063,#59064,#59065,#59066,#59067,
#59068,#59069,#59070,#59071,#59072,#59073,#59074,#59075,#59076,#59077,#59078,
#59079,#59080,#59081,#59082,#59083,#59084,#59085,#59086,#59087,#59088,#59089,
#59090,#59091,#59092,#59093,#59094,#59095,#59096,#59097,#59098,#59099,#59100,
#59101,#59102,#59103,#59104,#59105,#59106,#59107,#59108,#59109,#59110,#59111,
#59112,#59113,#59114,#59115,#59116,#59117,#59118,#59119,#59120,#59121,#59122,
#59123,#59124,#59125,#59126,#59127,#59128,#59129,#59130,#59131,#59132,#59133,
#59134,#59135,#59136,#59137,#59138,#59139,#59140,#59141,#59142,#59143,#59144,
#59145,#59146,#59147,#59148,#59149,#59150,#59151,#59152,#59153,#59154,#59155,
#59156,#59157,#59158,#59159,#59160,#59161,#59162,#59163,#59164,#59165,#59166,
#59167,#59168,#59169,#59170,#59171,#59172,#59173,#59174,#59175,#59176,#59177,
#59178,#59179,#59180,#59181,#59182,#59183,#59184,#59185,#59186,#59187,#59188,
#59189,#59190,#59191,#59192,#59193,#59194,#59195,#59196,#59197,#59198,#59199,
#59200,#59201,#59202,#59203,#59204,#59205,#59206,#59207,#59208,#59209,#59210,
#59211,#59212,#59213,#59214,#59215),.UNSPECIFIED.,.F.,.F.,(4,2,2,2,2,2,
2,2,2,2,2,2,2,2,2,2,2,2,2,2,2,2,2,2,2,2,2,2,2,2,2,2,2,2,2,2,2,2,2,2,2,2,
2,2,2,2,2,2,2,2,2,2,2,2,2,2,2,2,2,2,2,2,2,2,2,2,2,2,2,2,2,2,2,2,2,2,2,2,
2,2,2,2,2,2,2,2,2,2,2,2,2,2,2,2,2,2,2,2,2,2,2,2,2,2,2,2,2,2,2,2,2,2,2,2,
2,2,2,2,2,2,2,2,2,2,2,2,2,2,2,2,2,2,2,2,2,2,2,2,2,2,2,2,2,2,2,2,2,2,2,2,
2,2,2,2,2,2,2,2,2,2,2,2,2,2,2,2,2,2,2,2,2,2,2,2,2,2,2,2,2,2,2,2,2,2,2,2,
2,2,2,2,2,2,2,2,2,2,2,2,2,2,2,2,2,2,2,2,2,2,2,2,2,2,2,2,2,2,2,2,2,2,2,2,
2,2,2,2,2,2,2,2,2,2,2,2,2,2,2,2,2,2,2,2,2,2,2,2,2,2,2,2,2,2,2,2,2,2,2,2,
2,2,2,2,2,2,2,2,2,2,2,2,2,2,2,2,2,2,2,2,2,4),(0.00182729117505357,0.0654996008145292,
0.0701074088737819,0.0728422120533014,0.0747943813940611,0.0765090142978765,
0.0783641644564241,0.080774520517057,0.0860086466192052,0.124845090641752,
0.144694040278344,0.154702975825758,0.40987014630865,0.45616129617932,0.463125478905227,
0.465043948671223,0.46619968573496,0.467237281011554,0.46856891796434,0.470697699179319,
0.481601163029537,0.747138396296082,0.792862962430324,0.829746281241003,
0.842481204638353,0.851037642781539,0.854000319653516,0.855717376106154,
0.85755893755648,0.859913651506986,0.864729058813973,0.894106271274702,
0.898618119695143,0.904633638535121,0.914247332001024,1.00742449286921,
1.05992933584833,1.07452584042807,1.0910717537891,1.11014411552814,1.16817491732573,
1.2148914464747,1.24687716946578,1.25238282492018,1.25411813001952,1.25521656794703,
1.25623558051963,1.25755322401423,1.2597585799249,1.27308654478159,1.50799210840985,
1.57744093902551,1.6208103577681,1.63640662173346,1.64301766962169,1.6480362705988,
1.65036613427066,1.65204407236765,1.65370002848432,1.65593869058125,1.66029091512886,
1.69286389726613,1.69658950861984,1.69919706376264,1.70186714832853,1.85697384184988,
1.88999843290375,1.91007005830308,1.93830949810155,2.00972820820729,2.03997228620068,
2.04522850700231,2.04689998095725,2.04796169750311,2.04894968195724,2.05024496313522,
2.05243649565854,2.06585448731704,2.28666978807397,2.38758047806079,2.44595834684701,
2.45265771901319,2.45764652238093,2.46003501494346,2.46184226625668,2.46352016713626,
2.46581029355287,2.47151377129052,2.53340074968265,2.68552969186938,2.78920195806079,
2.81177295072392,2.84727143189108,2.85394022484021,2.85611999235643,2.85752015022534,
2.8588335815403,2.86055300183686,2.8641993442349,2.89180785181045,3.0844444269064,
3.2065262221986,3.22534029125046,3.23054063340928,3.23368342094688,3.23643460942883,
3.2398320113717,3.24619211114061,3.2768870628765,3.47482396011193,3.57602025212566,
3.60543698590955,3.60882080164138,3.61048091455183,3.6116605155399,3.61289607808051,
3.61461164743346,3.61903934258769,3.68129429164791,3.84926009682395,3.93761416976383,
3.99262975945702,4.0023472315729,4.00540544075515,4.00734064232026,4.00913564451352,
4.01145658949688,4.01645224879046,4.05208268913113,4.31609399402479,4.41456176489621,
4.4187237504521,4.42024472938987,4.42127034980716,4.42226755846087,4.42346247212247,
4.42640738688737,4.45133822809549,4.66761540676287,4.76016208375238,4.79344126570143,
4.81129208296053,4.81503909602459,4.81711739238437,4.81870103731314,4.82046670605492,
4.82368956615312,4.8338563599165,4.97962355324292,5.18130508682964,5.18543676865487,
5.20911706154826,5.21202919657863,5.21335075455124,5.21437024168725,5.21546667281263,
5.2171935044951,5.22262961720931,5.25397463473391,5.32605112253785,5.58958983290153,
5.60339136798987,5.6094498917172,5.61184253879933,5.61358144901017,5.61544115194774,
5.61792622678755,5.62342132276256,5.73049487927807,5.78318288577994,5.98658317891159,
5.99874789909316,6.00095682330009,6.00229784382983,6.00333912369449,6.00447715089883,
6.00631853299332,6.01254098034217,6.17263244944631,6.37221731355809,6.38582911113373,
6.38948215627375,6.39161168307753,6.39344071902455,6.39565677762603,6.39980535924009,
6.42278950143117,6.46683055893895,6.56887134550894,6.77491237108166,6.78008815612838,
6.78802695125784,6.79006455851089,6.79122749114294,6.79221293317646,6.79316562617901,
6.79502272608746,6.80195385427695,6.8493630658064,6.88121561979771,7.16418361515147,
7.18129963686276,7.18482787705405,7.18706927550078,7.18883595048827,7.19080433197611,
7.19405826928279,7.20574046382023,7.27969874357913,7.38453879689245,7.56898986283093,
7.58046465038643,7.5827391770487,7.58393386760999,7.58488706536052,7.5858004939159,
7.58745229944187,7.59260531876554,7.62195727914172,7.68963173470231,7.93040852785828,
7.98811522345443,7.99371927006413,7.99599174943956,7.99766467407823,7.99947418775777,
8.00192793984711,8.00750374231509,8.08846485719693,8.11953028399923,8.25009379231305,
8.25821453492117,8.26603424871818,8.38140637541629,8.38955344340338,8.39195618198125,
8.39339978113528,8.39468910491681,8.39627956338108,8.39932666436457,8.41806127250395,
8.44177118949497,8.49341867941202,8.63771858293601,8.75464344580777,8.7637076713746,
8.7673341891042,8.76998938803991,8.77283784285586,8.77663137687114,8.78497728089117,
8.97350939317952,9.06406468418882,9.13916442045584,9.14036422609357,9.14223971689198,
9.14489216603862,9.14639406936621,9.14758057811493,9.14906387107188,9.15161754904803,
9.16198573584434,9.31856172853097,9.3922476959119,9.52838779727184,9.53771523847683,
9.54084242042248,9.5425974340325,9.54419637600433,9.54633087455309,9.55029192990362,
9.57142843442649,9.61230281067081,9.66818508581611,9.82376476595195,9.93627842990203,
9.94235955118631,9.95222662661329,9.95437668741503,9.95538583871127),
 .UNSPECIFIED.);
#524=B_SPLINE_CURVE_WITH_KNOTS('',3,(#59217,#59218,#59219,#59220,#59221,
#59222,#59223,#59224,#59225,#59226,#59227,#59228,#59229,#59230,#59231,#59232,
#59233,#59234,#59235,#59236,#59237,#59238,#59239,#59240,#59241,#59242,#59243,
#59244,#59245,#59246,#59247,#59248,#59249,#59250,#59251,#59252,#59253,#59254,
#59255,#59256,#59257,#59258,#59259,#59260,#59261,#59262,#59263,#59264,#59265,
#59266,#59267,#59268,#59269,#59270,#59271,#59272,#59273,#59274,#59275,#59276,
#59277,#59278,#59279,#59280,#59281,#59282,#59283,#59284,#59285,#59286,#59287,
#59288,#59289,#59290,#59291,#59292,#59293,#59294,#59295,#59296,#59297,#59298,
#59299,#59300,#59301,#59302,#59303,#59304,#59305,#59306,#59307,#59308,#59309,
#59310,#59311,#59312,#59313,#59314,#59315,#59316,#59317,#59318,#59319,#59320,
#59321,#59322,#59323,#59324,#59325,#59326,#59327,#59328,#59329,#59330,#59331,
#59332,#59333,#59334,#59335,#59336,#59337,#59338,#59339,#59340,#59341,#59342,
#59343,#59344,#59345,#59346,#59347,#59348,#59349,#59350,#59351,#59352,#59353,
#59354,#59355,#59356,#59357,#59358,#59359,#59360,#59361,#59362,#59363,#59364,
#59365,#59366,#59367,#59368,#59369,#59370,#59371,#59372,#59373,#59374,#59375,
#59376,#59377,#59378,#59379,#59380,#59381,#59382,#59383,#59384,#59385,#59386,
#59387,#59388,#59389,#59390,#59391,#59392,#59393,#59394,#59395,#59396,#59397,
#59398,#59399,#59400,#59401,#59402,#59403,#59404,#59405,#59406,#59407,#59408,
#59409,#59410,#59411,#59412,#59413,#59414,#59415,#59416,#59417,#59418,#59419,
#59420,#59421,#59422,#59423,#59424,#59425,#59426,#59427,#59428,#59429,#59430,
#59431,#59432,#59433,#59434,#59435,#59436,#59437,#59438,#59439,#59440,#59441,
#59442,#59443,#59444,#59445,#59446,#59447,#59448,#59449,#59450,#59451,#59452,
#59453,#59454,#59455,#59456,#59457,#59458,#59459,#59460,#59461,#59462,#59463,
#59464,#59465,#59466,#59467,#59468,#59469,#59470,#59471,#59472,#59473,#59474,
#59475,#59476,#59477,#59478,#59479,#59480,#59481),.UNSPECIFIED.,.F.,.F.,
(4,3,3,3,3,3,3,3,3,3,3,3,3,3,3,3,3,3,3,3,3,3,3,3,3,3,3,3,3,3,3,3,3,3,3,
3,3,3,3,3,3,3,3,3,3,3,3,3,3,3,3,3,3,3,3,3,3,3,3,3,3,3,3,3,3,3,3,3,3,3,3,
3,3,3,3,3,3,3,3,3,3,3,3,3,3,3,3,3,4),(-280.552952748318,-280.479027221112,
-280.405188492471,-280.33142210548,-280.257713656703,-280.184048785067,
-280.110413161578,-280.036780331792,-279.963145359955,-279.889495294389,
-279.815817176824,-279.742059132793,-279.668256289114,-279.594352502714,
-279.554242254257,-279.479681192729,-279.405200965071,-279.330787658037,
-279.256427402599,-279.182106364968,-279.10781073802,-279.03351400232,-278.959212672779,
-278.884894259454,-278.810546265728,-278.736119149574,-278.661646642781,
-278.587077817322,-278.555834246206,-278.481273260072,-278.406793095686,
-278.332379839843,-278.258019623551,-278.183698613046,-278.109403001225,
-278.035106262717,-277.960804919181,-277.886486480672,-277.81213845056,
-277.737711281296,-277.663238711751,-277.588669809291,-277.557426238155,
-277.483532756901,-277.409721890759,-277.335979195336,-277.262290276441,
-277.188640779214,-277.11501637803,-277.041388531105,-276.967754665036,
-276.894101822821,-276.820417038612,-276.746646485715,-276.672827775099,
-276.598903124232,-276.559018230104,-276.48439516469,-276.409857835809,
-276.335392347056,-276.260984849414,-276.186621532172,-276.11228861427,
-276.037962151675,-275.96363581972,-275.889297160923,-275.814933713645,
-275.740498456463,-275.666021983071,-275.59145561093,-275.560610222053,
-275.482244548012,-275.403975378574,-275.325797432178,-275.247736659987,
-275.169747597733,-275.091847744738,-275.061406218028,-274.983495629914,
-274.905515233012,-274.827459903152,-274.749275187397,-274.67101980779,
-274.592645117153,-274.562202214002,-274.473533367918,-274.385256001682,
-274.297705320811,-274.269898628852),.UNSPECIFIED.);
#525=B_SPLINE_CURVE_WITH_KNOTS('',3,(#59483,#59484,#59485,#59486,#59487,
#59488,#59489,#59490,#59491,#59492,#59493,#59494,#59495,#59496,#59497,#59498,
#59499,#59500),.UNSPECIFIED.,.F.,.F.,(4,2,2,2,2,2,2,2,4),(-274.269898628852,
-273.434981716958,-272.600064805063,-271.765147893168,-270.930230981273,
-270.095314069378,-269.260397157483,-268.425480245588,-267.986713321673),
 .UNSPECIFIED.);
#526=B_SPLINE_CURVE_WITH_KNOTS('',3,(#59502,#59503,#59504,#59505,#59506,
#59507,#59508,#59509,#59510,#59511,#59512,#59513,#59514,#59515,#59516,#59517,
#59518,#59519,#59520,#59521,#59522,#59523,#59524,#59525,#59526,#59527,#59528,
#59529,#59530,#59531,#59532,#59533,#59534,#59535,#59536,#59537,#59538,#59539,
#59540,#59541,#59542,#59543,#59544,#59545,#59546,#59547,#59548,#59549,#59550,
#59551,#59552,#59553,#59554,#59555,#59556,#59557,#59558,#59559,#59560,#59561,
#59562,#59563,#59564,#59565,#59566,#59567,#59568,#59569,#59570,#59571,#59572,
#59573,#59574,#59575,#59576,#59577,#59578,#59579,#59580,#59581,#59582,#59583,
#59584,#59585,#59586,#59587,#59588,#59589,#59590,#59591,#59592,#59593,#59594,
#59595,#59596,#59597,#59598,#59599,#59600,#59601,#59602,#59603,#59604,#59605,
#59606,#59607,#59608,#59609,#59610,#59611,#59612,#59613,#59614,#59615,#59616,
#59617,#59618,#59619,#59620,#59621,#59622,#59623,#59624,#59625,#59626,#59627,
#59628,#59629,#59630,#59631,#59632,#59633,#59634,#59635,#59636,#59637,#59638,
#59639,#59640,#59641,#59642,#59643,#59644,#59645,#59646,#59647,#59648,#59649,
#59650,#59651,#59652,#59653,#59654,#59655,#59656,#59657,#59658,#59659,#59660,
#59661,#59662,#59663,#59664,#59665,#59666,#59667,#59668,#59669,#59670,#59671,
#59672,#59673,#59674,#59675,#59676,#59677,#59678,#59679,#59680,#59681,#59682,
#59683,#59684,#59685,#59686,#59687,#59688,#59689,#59690,#59691,#59692,#59693,
#59694,#59695,#59696,#59697,#59698,#59699,#59700,#59701,#59702,#59703,#59704,
#59705,#59706,#59707,#59708,#59709,#59710,#59711,#59712,#59713,#59714,#59715,
#59716,#59717,#59718,#59719,#59720,#59721,#59722,#59723,#59724,#59725,#59726,
#59727,#59728,#59729,#59730,#59731,#59732,#59733,#59734,#59735,#59736,#59737,
#59738,#59739,#59740,#59741,#59742,#59743,#59744,#59745,#59746,#59747,#59748,
#59749,#59750,#59751,#59752,#59753,#59754,#59755,#59756,#59757,#59758,#59759,
#59760,#59761,#59762,#59763),.UNSPECIFIED.,.F.,.F.,(4,3,3,3,3,3,3,3,3,3,
3,3,3,3,3,3,3,3,3,3,3,3,3,3,3,3,3,3,3,3,3,3,3,3,3,3,3,3,3,3,3,3,3,3,3,3,
3,3,3,3,3,3,3,3,3,3,3,3,3,3,3,3,3,3,3,3,3,3,3,3,3,3,3,3,3,3,3,3,3,3,3,3,
3,3,3,3,3,4),(-267.986713321673,-267.906108764019,-267.822918112426,-267.741928442518,
-267.657637300082,-267.573346157646,-267.498787061105,-267.424303411479,
-267.349881348361,-267.275507051909,-267.201166734104,-267.126846630343,
-267.052517761171,-266.978179527966,-266.903819469602,-266.829425115786,
-266.7549447622,-266.680415009185,-266.605783278329,-266.574938149595,-266.501018363321,
-266.427185387969,-266.353424762344,-266.27972207882,-266.206062972188,
-266.132433109361,-266.058806033688,-265.985176804652,-265.911532466892,
-265.837860058435,-265.764107731001,-265.69031058017,-265.616412553523,
-265.576530141544,-265.501969080047,-265.42748885242,-265.353075545418,
-265.278715290011,-265.204394252411,-265.130098625494,-265.055801889826,
-264.981500560316,-264.907182147023,-264.832834153328,-264.758407037205,
-264.683934530443,-264.609365705014,-264.578122133493,-264.503561147286,
-264.429080982827,-264.354667726912,-264.280307510546,-264.20598649997,
-264.131690888076,-264.057394149496,-263.983092805889,-263.908774367309,
-263.834426337128,-263.759999167794,-263.68552659818,-263.610957695652,
-263.579714125442,-263.505820644216,-263.432009778101,-263.358267082705,
-263.284578163837,-263.210928666637,-263.137304265478,-263.063676418577,
-262.990042552533,-262.916389710342,-262.842704926157,-262.768934373282,
-262.695115662688,-262.621191011842,-262.581306117391,-262.507515619813,
-262.433810262704,-262.360175471895,-262.286596727781,-262.213059860217,
-262.13954538831,-262.066040247222,-261.992531379277,-261.918974420258,
-261.84539359123,-261.771731328759,-261.704055150649),.UNSPECIFIED.);
#527=B_SPLINE_CURVE_WITH_KNOTS('',3,(#59765,#59766,#59767,#59768,#59769,
#59770,#59771,#59772,#59773,#59774,#59775,#59776,#59777,#59778,#59779,#59780,
#59781,#59782,#59783,#59784,#59785,#59786,#59787,#59788,#59789,#59790,#59791,
#59792,#59793,#59794,#59795,#59796,#59797,#59798,#59799,#59800,#59801,#59802,
#59803,#59804,#59805,#59806,#59807,#59808,#59809,#59810,#59811,#59812,#59813,
#59814,#59815,#59816,#59817,#59818,#59819,#59820,#59821,#59822,#59823,#59824,
#59825,#59826,#59827,#59828,#59829,#59830,#59831,#59832,#59833,#59834,#59835,
#59836,#59837,#59838,#59839,#59840,#59841,#59842,#59843,#59844,#59845,#59846,
#59847,#59848,#59849,#59850,#59851,#59852,#59853,#59854,#59855,#59856,#59857,
#59858,#59859,#59860,#59861,#59862,#59863,#59864,#59865,#59866,#59867,#59868,
#59869,#59870,#59871,#59872,#59873,#59874,#59875,#59876,#59877,#59878,#59879,
#59880,#59881,#59882,#59883,#59884,#59885,#59886,#59887,#59888,#59889,#59890,
#59891,#59892,#59893,#59894,#59895,#59896,#59897,#59898,#59899,#59900,#59901,
#59902,#59903,#59904,#59905,#59906,#59907,#59908,#59909,#59910,#59911,#59912,
#59913,#59914,#59915,#59916,#59917,#59918,#59919,#59920,#59921,#59922,#59923,
#59924,#59925,#59926,#59927,#59928,#59929,#59930,#59931,#59932,#59933,#59934,
#59935,#59936,#59937,#59938,#59939,#59940,#59941,#59942,#59943,#59944,#59945,
#59946,#59947,#59948,#59949,#59950,#59951,#59952,#59953,#59954,#59955,#59956,
#59957,#59958,#59959,#59960,#59961,#59962,#59963,#59964,#59965,#59966,#59967,
#59968,#59969,#59970,#59971,#59972,#59973,#59974,#59975,#59976,#59977,#59978,
#59979,#59980,#59981,#59982,#59983,#59984,#59985,#59986,#59987,#59988,#59989,
#59990,#59991,#59992,#59993,#59994,#59995,#59996,#59997,#59998,#59999,#60000,
#60001,#60002,#60003,#60004,#60005,#60006,#60007,#60008,#60009,#60010,#60011,
#60012,#60013,#60014,#60015,#60016,#60017,#60018,#60019,#60020,#60021,#60022,
#60023,#60024,#60025,#60026,#60027,#60028,#60029,#60030,#60031,#60032,#60033,
#60034,#60035,#60036,#60037,#60038,#60039,#60040,#60041,#60042,#60043,#60044,
#60045,#60046,#60047,#60048,#60049,#60050,#60051,#60052,#60053,#60054,#60055,
#60056,#60057,#60058,#60059,#60060,#60061,#60062,#60063,#60064,#60065,#60066,
#60067,#60068,#60069,#60070,#60071,#60072,#60073,#60074,#60075,#60076,#60077,
#60078,#60079,#60080,#60081,#60082,#60083,#60084,#60085,#60086,#60087,#60088,
#60089,#60090,#60091,#60092,#60093,#60094,#60095,#60096,#60097,#60098,#60099,
#60100,#60101,#60102,#60103,#60104,#60105,#60106,#60107,#60108,#60109,#60110,
#60111,#60112,#60113,#60114,#60115,#60116,#60117,#60118,#60119,#60120,#60121,
#60122,#60123,#60124,#60125,#60126,#60127,#60128,#60129,#60130,#60131,#60132,
#60133,#60134,#60135,#60136,#60137,#60138,#60139,#60140,#60141,#60142,#60143,
#60144,#60145,#60146,#60147,#60148,#60149,#60150,#60151,#60152,#60153,#60154,
#60155,#60156,#60157,#60158,#60159,#60160,#60161,#60162,#60163,#60164,#60165,
#60166,#60167,#60168,#60169,#60170,#60171,#60172,#60173,#60174,#60175,#60176,
#60177,#60178,#60179,#60180,#60181,#60182,#60183,#60184,#60185,#60186,#60187,
#60188,#60189,#60190,#60191,#60192,#60193,#60194,#60195,#60196,#60197,#60198,
#60199,#60200,#60201,#60202,#60203,#60204,#60205,#60206,#60207,#60208,#60209,
#60210,#60211,#60212,#60213,#60214,#60215,#60216,#60217,#60218,#60219,#60220,
#60221,#60222,#60223,#60224,#60225,#60226,#60227,#60228,#60229,#60230,#60231,
#60232,#60233,#60234,#60235,#60236,#60237,#60238,#60239,#60240,#60241,#60242,
#60243,#60244,#60245,#60246,#60247,#60248,#60249,#60250,#60251,#60252,#60253,
#60254,#60255,#60256,#60257,#60258,#60259,#60260,#60261,#60262,#60263,#60264,
#60265,#60266,#60267,#60268,#60269,#60270,#60271,#60272,#60273,#60274,#60275,
#60276,#60277,#60278,#60279,#60280,#60281,#60282,#60283,#60284,#60285,#60286,
#60287,#60288,#60289,#60290,#60291,#60292,#60293,#60294,#60295,#60296,#60297,
#60298,#60299,#60300,#60301,#60302,#60303,#60304,#60305,#60306,#60307,#60308,
#60309,#60310,#60311,#60312,#60313,#60314,#60315,#60316,#60317,#60318,#60319,
#60320,#60321,#60322,#60323,#60324,#60325,#60326,#60327,#60328,#60329,#60330,
#60331,#60332,#60333,#60334,#60335,#60336,#60337,#60338,#60339,#60340),
 .UNSPECIFIED.,.F.,.F.,(4,2,2,2,2,2,2,2,2,2,2,2,2,2,2,2,2,2,2,2,2,2,2,2,
2,2,2,2,2,2,2,2,2,2,2,2,2,2,2,2,2,2,2,2,2,2,2,2,2,2,2,2,2,2,2,2,2,2,2,2,
2,2,2,2,2,2,2,2,2,2,2,2,2,2,2,2,2,2,2,2,2,2,2,2,2,2,2,2,2,2,2,2,2,2,2,2,
2,2,2,2,2,2,2,2,2,2,2,2,2,2,2,2,2,2,2,2,2,2,2,2,2,2,2,2,2,2,2,2,2,2,2,2,
2,2,2,2,2,2,2,2,2,2,2,2,2,2,2,2,2,2,2,2,2,2,2,2,2,2,2,2,2,2,2,2,2,2,2,2,
2,2,2,2,2,2,2,2,2,2,2,2,2,2,2,2,2,2,2,2,2,2,2,2,2,2,2,2,2,2,2,2,2,2,2,2,
2,2,2,2,2,2,2,2,2,2,2,2,2,2,2,2,2,2,2,2,2,2,2,2,2,2,2,2,2,2,2,2,2,2,2,2,
2,2,2,2,2,2,2,2,2,2,2,2,2,2,2,2,2,2,2,2,2,2,2,2,2,2,2,2,2,2,2,2,2,2,2,2,
2,2,2,2,2,2,2,2,2,2,2,4),(0.00135467936860461,0.105905930347926,0.109781162785451,
0.111971599148687,0.113457851424939,0.114902647586442,0.116203225236225,
0.117858513503175,0.120476298019936,0.133391480944711,0.242813923920672,
0.254956640849107,0.437672197329887,0.477662082861804,0.486041402095746,
0.489842763732373,0.492694103771591,0.49534988272335,0.498973832276405,
0.508014324551167,0.622732808646861,0.696276497028578,0.723696217518591,
0.794401940169627,0.842975615310469,0.856494980750388,0.864683171939286,
0.866427018531058,0.867733985107433,0.869056540279512,0.870274573891002,
0.871921959007485,0.875949218922695,0.926505973886985,0.975494227105744,
1.04932196243803,1.05858070480526,1.069232921339,1.08159728199511,1.096132785653,
1.14426648409367,1.19730391518818,1.25035727062657,1.25985354027119,1.2628859183482,
1.26481576058556,1.26661346119229,1.2689487512867,1.27283496982685,1.28145053066355,
1.43512062978405,1.5200757110767,1.61755590934972,1.65760373379746,1.66858440667646,
1.67293352300218,1.67611277346537,1.67748866140144,1.67848626687923,1.67940466161041,
1.68064735337387,1.68368655596113,1.71373931107317,1.75671962746866,1.81136529901845,
1.9477769258085,1.97150830227803,2.00615049657611,2.04687088502283,2.06784821882593,
2.07177970623093,2.0738983549376,2.07564019400885,2.07769235081026,2.08122368923301,
2.09449282191791,2.29013857515821,2.38491141486254,2.42869334652271,2.45361764704357,
2.4669851894006,2.46925575352262,2.47047702433452,2.47148355053888,2.47265366486427,
2.47465640774287,2.48206850930876,2.59218348615894,2.74717041969454,2.80325040293928,
2.83904097737279,2.86300500251538,2.86720307836638,2.86943026323644,2.87126052566002,
2.87338247474936,2.87700070248533,2.89026193690734,3.08611885385599,3.2502463267109,
3.25445744657098,3.25758780895534,3.2589890650467,3.26004111515289,3.26101924152143,
3.262363868879,3.26504608623641,3.28774287235409,3.32255572966217,3.35329934152961,
3.55296650186679,3.61397157562832,3.64151943120264,3.64587535615561,3.6481359042926,
3.64996818586396,3.65179490400689,3.65509603630614,3.66526739576775,3.81328358323173,
3.943884280613,3.99187330242446,4.02847341842462,4.04428348811881,4.04670845846484,
4.04795802045265,4.0488701693116,4.04984833325476,4.05153662365964,4.05635834462272,
4.13185719284762,4.32090066557039,4.38176762556886,4.430648694589,4.43964937652221,
4.44260545367139,4.44450803499917,4.44629547384494,4.44863921353242,4.45362274715417,
4.49131402928216,4.49298098767543,4.4940723283588,4.49748049918456,4.50036729068039,
4.5067399248079,4.51150395115702,4.58217694522431,4.73464532075125,4.80411363501906,
4.83319291843746,4.83832249637584,4.83997875602932,4.84103719292627,4.84202666524086,
4.84333059408172,4.8462528534955,4.87086724271372,4.87189624476929,4.97793406782097,
5.08840400771867,5.23809519846542,5.24694095567933,5.25079643720284,5.25312254623189,
5.25491872044257,5.25685239417388,5.25990229748367,5.26954564224272,5.32389195446405,
5.4226108409505,5.63286354251302,5.64583364080445,5.64845888757635,5.65011780321481,
5.65141892171266,5.65286194054345,5.655232127965,5.66358743332866,5.71903089472145,
5.78437674262154,5.98512045033842,6.01637918488383,6.02225639943245,6.02587022251524,
6.02870245508081,6.031770781023,6.03663415163201,6.05226394773474,6.14152795757657,
6.25955863475273,6.38585091922345,6.39953468820055,6.40220526203005,6.40385891252999,
6.40516272185708,6.40659381889168,6.40891102236911,6.41676080627408,6.46309497171556,
6.53550357264128,6.77870743965064,6.79470629261983,6.79817002131697,6.80040153322107,
6.80218066925732,6.80414379072952,6.80733911484718,6.81117303003682,6.81863737892238,
6.88832271622816,6.99800239906012,7.19835282047591,7.20067573968731,7.21094644236082,
7.21295024848259,7.21418986680626,7.21517028977066,7.21625910313221,7.21805109503241,
7.22439814698596,7.26535678174477,7.32944300393575,7.40395566010084,7.54091378183065,
7.60153121281455,7.60717384761469,7.609443344494,7.61110739117516,7.61286434970071,
7.61521408922589,7.61781774980441,7.62218648233486,7.63112688574736,7.69057513380319,
7.7486400408186,7.98359329986033,8.0029422908334,8.00541587966643,8.00668319994108,
8.00762739005743,8.00865980031254,8.01007950197134,8.01339186615285,8.10549354228159,
8.22094636824289,8.30951005776843,8.39619016231785,8.40255255250107,8.40521377229103,
8.40708657694722,8.40894553172706,8.41082591555787,8.41568024097913,8.46028577977377,
8.5344087007939,8.77987993903232,8.79234537718995,8.79457326394936,8.7959202825172,
8.79696287278316,8.79809884642329,8.79992956171754,8.80604952056384,8.90638692857541,
9.00918948901993,9.0689030627306,9.17457944142369,9.18130774150486,9.18403339794349,
9.18592030380121,9.18776827571486,9.18962987628439,9.19430613881731,9.23146619108504,
9.32707261236817,9.53714990258149,9.55732759127054,9.58051070062318,9.58346242184171,
9.58480219008999,9.5858250473158,9.586914795481,9.58861503086718,9.59402837030787,
9.62563108756224,9.67216786306517,9.95668469293117),.UNSPECIFIED.);
#528=B_SPLINE_CURVE_WITH_KNOTS('',3,(#60342,#60343,#60344,#60345,#60346,
#60347,#60348,#60349,#60350,#60351,#60352,#60353,#60354,#60355,#60356,#60357,
#60358,#60359,#60360,#60361,#60362,#60363,#60364,#60365,#60366,#60367,#60368,
#60369,#60370,#60371,#60372,#60373,#60374,#60375,#60376,#60377,#60378,#60379,
#60380,#60381,#60382,#60383,#60384,#60385,#60386,#60387,#60388,#60389,#60390,
#60391,#60392,#60393,#60394,#60395,#60396,#60397,#60398,#60399,#60400,#60401,
#60402,#60403,#60404,#60405,#60406,#60407,#60408,#60409,#60410,#60411,#60412,
#60413,#60414,#60415,#60416,#60417,#60418,#60419,#60420,#60421,#60422,#60423,
#60424,#60425,#60426,#60427,#60428,#60429,#60430,#60431,#60432,#60433,#60434,
#60435,#60436,#60437,#60438,#60439,#60440,#60441,#60442,#60443,#60444,#60445,
#60446,#60447,#60448,#60449,#60450,#60451,#60452,#60453,#60454,#60455,#60456,
#60457,#60458,#60459,#60460,#60461,#60462,#60463,#60464,#60465,#60466,#60467,
#60468,#60469,#60470,#60471,#60472,#60473,#60474,#60475,#60476,#60477,#60478,
#60479,#60480,#60481,#60482,#60483,#60484,#60485,#60486,#60487,#60488,#60489,
#60490,#60491,#60492,#60493,#60494,#60495,#60496,#60497,#60498,#60499,#60500,
#60501,#60502,#60503,#60504,#60505,#60506,#60507,#60508,#60509,#60510,#60511,
#60512,#60513,#60514,#60515,#60516,#60517,#60518,#60519,#60520,#60521,#60522,
#60523,#60524,#60525,#60526,#60527,#60528,#60529,#60530,#60531,#60532,#60533,
#60534,#60535,#60536,#60537,#60538,#60539,#60540,#60541,#60542,#60543,#60544,
#60545,#60546,#60547,#60548,#60549,#60550,#60551,#60552,#60553,#60554,#60555,
#60556,#60557,#60558,#60559,#60560,#60561,#60562,#60563,#60564,#60565,#60566,
#60567,#60568,#60569,#60570,#60571,#60572,#60573,#60574,#60575,#60576,#60577,
#60578,#60579,#60580,#60581,#60582,#60583,#60584,#60585,#60586,#60587,#60588,
#60589,#60590,#60591,#60592,#60593,#60594,#60595,#60596,#60597,#60598,#60599,
#60600,#60601,#60602,#60603,#60604,#60605,#60606,#60607,#60608,#60609,#60610,
#60611,#60612,#60613,#60614,#60615,#60616,#60617,#60618,#60619,#60620,#60621,
#60622,#60623,#60624,#60625,#60626,#60627,#60628,#60629,#60630,#60631,#60632,
#60633,#60634,#60635,#60636,#60637,#60638,#60639,#60640,#60641,#60642,#60643,
#60644,#60645,#60646,#60647,#60648,#60649,#60650,#60651,#60652,#60653,#60654,
#60655,#60656,#60657,#60658,#60659,#60660,#60661,#60662,#60663,#60664,#60665,
#60666,#60667,#60668,#60669,#60670,#60671,#60672,#60673,#60674,#60675,#60676,
#60677,#60678,#60679,#60680,#60681,#60682,#60683,#60684,#60685,#60686,#60687,
#60688,#60689,#60690,#60691,#60692,#60693,#60694,#60695,#60696,#60697,#60698,
#60699,#60700,#60701,#60702,#60703,#60704,#60705,#60706,#60707,#60708,#60709,
#60710,#60711,#60712,#60713,#60714,#60715,#60716,#60717,#60718,#60719,#60720,
#60721,#60722,#60723,#60724,#60725,#60726,#60727,#60728,#60729,#60730,#60731,
#60732,#60733,#60734,#60735,#60736,#60737,#60738,#60739,#60740,#60741,#60742,
#60743,#60744,#60745,#60746,#60747,#60748,#60749,#60750,#60751,#60752,#60753,
#60754,#60755,#60756,#60757,#60758,#60759,#60760,#60761,#60762,#60763,#60764,
#60765,#60766,#60767,#60768,#60769,#60770,#60771,#60772,#60773,#60774,#60775,
#60776,#60777,#60778,#60779,#60780,#60781,#60782,#60783,#60784,#60785,#60786,
#60787,#60788,#60789,#60790,#60791,#60792,#60793,#60794,#60795,#60796,#60797,
#60798,#60799,#60800,#60801,#60802,#60803,#60804,#60805,#60806,#60807,#60808,
#60809,#60810,#60811,#60812,#60813,#60814,#60815,#60816,#60817,#60818,#60819,
#60820,#60821,#60822,#60823,#60824,#60825,#60826,#60827,#60828,#60829,#60830,
#60831,#60832,#60833,#60834,#60835,#60836,#60837,#60838,#60839,#60840,#60841,
#60842,#60843,#60844,#60845,#60846,#60847,#60848,#60849,#60850,#60851,#60852,
#60853,#60854,#60855,#60856,#60857,#60858,#60859,#60860,#60861,#60862,#60863,
#60864,#60865,#60866,#60867,#60868,#60869,#60870,#60871,#60872,#60873,#60874,
#60875,#60876,#60877,#60878,#60879,#60880,#60881,#60882,#60883,#60884,#60885,
#60886,#60887,#60888,#60889,#60890,#60891,#60892,#60893,#60894,#60895,#60896,
#60897,#60898,#60899,#60900,#60901,#60902,#60903,#60904,#60905,#60906,#60907,
#60908,#60909,#60910,#60911,#60912,#60913,#60914,#60915,#60916,#60917,#60918,
#60919,#60920,#60921,#60922,#60923,#60924,#60925,#60926,#60927,#60928,#60929,
#60930,#60931,#60932,#60933,#60934,#60935,#60936,#60937,#60938,#60939,#60940,
#60941,#60942,#60943,#60944,#60945,#60946,#60947,#60948,#60949,#60950,#60951,
#60952,#60953,#60954,#60955,#60956,#60957),.UNSPECIFIED.,.F.,.F.,(4,2,2,
2,2,2,2,2,2,2,2,2,2,2,2,2,2,2,2,2,2,2,2,2,2,2,2,2,2,2,2,2,2,2,2,2,2,2,2,
2,2,2,2,2,2,2,2,2,2,2,2,2,2,2,2,2,2,2,2,2,2,2,2,2,2,2,2,2,2,2,2,2,2,2,2,
2,2,2,2,2,2,2,2,2,2,2,2,2,2,2,2,2,2,2,2,2,2,2,2,2,2,2,2,2,2,2,2,2,2,2,2,
2,2,2,2,2,2,2,2,2,2,2,2,2,2,2,2,2,2,2,2,2,2,2,2,2,2,2,2,2,2,2,2,2,2,2,2,
2,2,2,2,2,2,2,2,2,2,2,2,2,2,2,2,2,2,2,2,2,2,2,2,2,2,2,2,2,2,2,2,2,2,2,2,
2,2,2,2,2,2,2,2,2,2,2,2,2,2,2,2,2,2,2,2,2,2,2,2,2,2,2,2,2,2,2,2,2,2,2,2,
2,2,2,2,2,2,2,2,2,2,2,2,2,2,2,2,2,2,2,2,2,2,2,2,2,2,2,2,2,2,2,2,2,2,2,2,
2,2,2,2,2,2,2,2,2,2,2,2,2,2,2,2,2,2,2,2,2,2,2,2,2,2,2,2,2,2,2,2,2,2,2,2,
2,2,2,2,2,2,2,2,2,2,2,2,2,2,2,2,4),(0.00211751522266133,0.0203487448140315,
0.0233396307185236,0.0253653093889092,0.0270336021014908,0.0286196489711016,
0.030659105402196,0.0341342840646406,0.0468442262904942,0.0571183188809527,
0.316321449506284,0.395751492788939,0.420267752109709,0.422876291006466,
0.424139781454416,0.425031367887155,0.425961656823417,0.427260319795774,
0.430647443332828,0.476474940746983,0.507710315873694,0.730301566755093,
0.787060668938419,0.815861512614544,0.826363351505926,0.831297980995632,
0.835260252259935,0.837013278865553,0.838714072668814,0.840397629460644,
0.842707959867446,0.848525574761595,0.915190192337002,1.00193201257549,
1.05720940702609,1.0729715832019,1.09121513166381,1.11291192374864,1.18937277439881,
1.22422821879501,1.23081620325662,1.23298393024763,1.2343801078656,1.23569248272775,
1.237414390011,1.2403197432154,1.25801580912919,1.4819056695185,1.59425643394248,
1.60454838385065,1.60866481023985,1.61155935843278,1.6143966928691,1.61836815298445,
1.62760665685734,1.76458571087279,1.81666939983119,1.92138790386485,1.97625768192028,
1.98455080994873,1.9869083107692,1.98834466710389,1.98964046489571,1.99129353898145,
1.99391139597964,2.00687735020665,2.21718586094031,2.31546325484413,2.35724971268514,
2.3712906343388,2.37741059905734,2.38212766163794,2.3844076171033,2.3861122670254,
2.38780253568542,2.39014582662124,2.39487937829662,2.4375911564596,2.43956161201346,
2.65576998447692,2.66686773035628,2.67909885614578,2.69280758762909,2.79330917507329,
2.79652034191443,2.79788984819507,2.79888806682704,2.79980973866556,2.80105993755311,
2.8041331024341,2.83525153894454,3.08501857729282,3.18479383091183,3.18919981722481,
3.19182092445397,3.19418461154305,3.19594794683303,3.19761428528336,3.19988210259741,
3.20549624124599,3.26457633020326,3.4932706543862,3.51121705408484,3.5339494150222,
3.58139667457577,3.58834186258623,3.59020584733558,3.59133489081425,3.59235211872347,
3.59364788731741,3.59628004112941,3.61192187379014,3.6137383468532,3.61469144542661,
3.61558556795375,3.61730132765294,3.78879717761604,3.89682821902251,3.97084445696559,
3.98271980814225,3.98608095971661,3.98812578930755,3.98996860745907,3.99231696832411,
3.99709176562342,4.02561526800418,4.05123023666428,4.27966376196531,4.33428677642955,
4.36075601936324,4.37482004753219,4.3772057779469,4.37846148719029,4.37948815117661,
4.38051936564364,4.38243297405945,4.38877492573883,4.39639657938534,4.62074094072661,
4.71407607525427,4.74784684285249,4.76599460048085,4.76982928282915,4.77196012567408,
4.7735856172384,4.77566988753082,4.77920066379627,4.7919121724557,4.98045649906709,
5.14409075109595,5.16606871388247,5.16867196448299,5.16997721804109,5.17092677626253,
5.17194666156686,5.17333154224294,5.17648855019712,5.28439301281565,5.54310583802784,
5.54628458262641,5.56038490960152,5.56404227423261,5.56614821749934,5.5677621494078,
5.56984391937517,5.57349180811749,5.58919852054118,5.76533791401445,5.78982001376208,
5.93634422093143,5.95748166191959,5.96033706293842,5.96165163101424,5.9626638106372,
5.96376152842931,5.96551659476634,5.97126070006308,6.00563847826581,6.05883319512685,
6.18077101822055,6.29721809301472,6.2996479486732,6.29999652052559,6.30043104665369,
6.30110290585124,6.30332587178196,6.30358048667121,6.30426593787041,6.30490516887891,
6.3510756476589,6.35652212497748,6.35873314166507,6.36057943820299,6.36247562674068,
6.36524872907727,6.37259017757667,6.47187054765089,6.58050447474925,6.66845716110728,
6.74607744046733,6.75086522706987,6.75257326311576,6.75356465897043,6.75449613534523,
6.75575726779103,6.75819951934292,6.76130053405256,6.89538876504119,6.91549323463673,
6.99076059734671,7.12886539503232,7.13834341256229,7.14155379664398,7.14336361679277,
7.14501742303726,7.14723246973909,7.15136649406493,7.17397342926271,7.21777182334469,
7.29472515593811,7.46594430939503,7.50457923786179,7.53534236269615,7.53854613213906,
7.53981025003095,7.54075677254305,7.54179618322441,7.54320406815022,7.5465293574908,
7.55111973660279,7.59885560848396,7.69077888710198,7.91515756527117,7.93015405108597,
7.9335248281765,7.9357208071321,7.93748768400637,7.93949484121496,7.94290534822238,
7.95619456365978,8.05092493716908,8.07868267668072,8.10007413126194,8.12447838308061,
8.24596209586379,8.32518337536583,8.33013098903248,8.3318280711429,8.33279014516939,
8.33367239690127,8.33460573872196,8.33650472997047,8.34410241683171,8.35740711634689,
8.38918401789272,8.46030480267807,8.72163530912242,8.72559484678511,8.7397273709299,
8.74335643954359,8.74543870407977,8.74703053515841,8.74907915527874,8.75265565819566,
8.76786106833943,8.79478730330389,8.90586407638577,8.92726267398728,8.94514962832429,
8.96047244303898,8.97381213396143,8.98556166739383,8.99600921616865,9.0053870515391,
9.09248539067258,9.10127087357609,9.1038711528879,9.13624403661262,9.13996784021801,
9.14167122072968,9.14297745772833,9.14418620214296,9.14616551954953,9.15143824292911,
9.15911227454543,9.18077152512064,9.23705469809105,9.49673734620167,9.5114402685722,
9.51635838158552,9.51911917847084,9.52188136759699,9.52531268356329,9.53190188606939,
9.57359579554831,9.6684620470765,9.82787860058392,9.83620678294941,9.85876088194946,
9.88984309728776,9.89365342576422,9.89537514938782,9.89668657238815,9.89789282009943,
9.89925572239684,9.90115071667791,9.9043124389687,9.95584215760787),
 .UNSPECIFIED.);
#529=B_SPLINE_CURVE_WITH_KNOTS('',3,(#60959,#60960,#60961,#60962,#60963,
#60964,#60965,#60966,#60967,#60968,#60969,#60970,#60971,#60972,#60973,#60974,
#60975,#60976,#60977,#60978,#60979,#60980,#60981,#60982,#60983,#60984,#60985,
#60986,#60987,#60988,#60989,#60990,#60991,#60992,#60993,#60994,#60995,#60996,
#60997,#60998,#60999,#61000,#61001,#61002,#61003,#61004,#61005,#61006,#61007,
#61008,#61009,#61010,#61011,#61012,#61013,#61014,#61015,#61016,#61017,#61018,
#61019,#61020,#61021,#61022,#61023,#61024,#61025,#61026,#61027,#61028,#61029,
#61030,#61031,#61032,#61033,#61034,#61035,#61036,#61037,#61038,#61039,#61040,
#61041,#61042,#61043,#61044,#61045,#61046,#61047,#61048,#61049,#61050,#61051,
#61052,#61053,#61054,#61055,#61056,#61057,#61058,#61059,#61060,#61061,#61062,
#61063,#61064,#61065,#61066,#61067,#61068,#61069,#61070,#61071,#61072,#61073,
#61074,#61075,#61076,#61077,#61078,#61079,#61080,#61081,#61082,#61083,#61084,
#61085,#61086,#61087,#61088,#61089,#61090,#61091,#61092,#61093,#61094,#61095,
#61096,#61097,#61098,#61099,#61100,#61101,#61102,#61103,#61104,#61105,#61106,
#61107,#61108,#61109,#61110,#61111,#61112,#61113,#61114,#61115,#61116,#61117,
#61118,#61119,#61120,#61121,#61122,#61123,#61124,#61125,#61126,#61127,#61128,
#61129,#61130,#61131,#61132,#61133,#61134,#61135,#61136,#61137,#61138,#61139,
#61140,#61141,#61142,#61143,#61144,#61145,#61146,#61147,#61148,#61149,#61150,
#61151,#61152,#61153,#61154,#61155,#61156,#61157,#61158,#61159,#61160,#61161,
#61162,#61163,#61164,#61165,#61166,#61167,#61168,#61169,#61170,#61171,#61172,
#61173,#61174,#61175,#61176,#61177,#61178,#61179,#61180,#61181,#61182,#61183,
#61184,#61185,#61186,#61187,#61188,#61189,#61190,#61191,#61192,#61193,#61194,
#61195,#61196,#61197,#61198,#61199,#61200,#61201,#61202,#61203,#61204,#61205,
#61206,#61207,#61208,#61209,#61210,#61211,#61212,#61213,#61214,#61215,#61216,
#61217,#61218,#61219,#61220),.UNSPECIFIED.,.F.,.F.,(4,3,3,3,3,3,3,3,3,3,
3,3,3,3,3,3,3,3,3,3,3,3,3,3,3,3,3,3,3,3,3,3,3,3,3,3,3,3,3,3,3,3,3,3,3,3,
3,3,3,3,3,3,3,3,3,3,3,3,3,3,3,3,3,3,3,3,3,3,3,3,3,3,3,3,3,3,3,3,3,3,3,3,
3,3,3,3,3,4),(-236.570517887855,-236.496478268965,-236.422511351756,-236.348602846773,
-236.274738505804,-236.200904112088,-236.127072919686,-236.053240372639,
-235.979393621018,-235.905519809121,-235.831563950077,-235.757564442011,
-235.683456355741,-235.624289900016,-235.550367529142,-235.476531943763,
-235.402768684695,-235.329063346266,-235.255401565183,-235.18176901024,
-235.108139222922,-235.034507269787,-234.960860197126,-234.887185044625,
-234.813429971543,-234.73963006972,-234.665729306294,-234.625881891966,
-234.551321119513,-234.476841179748,-234.402428159158,-234.32806818845,
-234.253747433568,-234.179452087123,-234.105155627678,-234.030854571707,
-233.956536429025,-233.882188702768,-233.807761847989,-233.733289599446,
-233.658721025371,-233.627473883915,-233.552913435452,-233.478433816586,
-233.404021113575,-233.329661456895,-233.255341012262,-233.181045972053,
-233.106749812024,-233.032449051203,-232.958131199188,-232.883783758897,
-232.809357181721,-232.73488520639,-232.660316896702,-232.629065875864,
-232.55517201873,-232.481360773344,-232.407617695596,-232.333928391571,
-232.260278506677,-232.186653715553,-232.113025476293,-232.03939121634,
-231.965737978926,-231.892052798438,-231.818281849421,-231.744462742115,
-231.67053769699,-231.630657867813,-231.556034821066,-231.481497510767,
-231.407032040494,-231.332624561216,-231.258261262204,-231.183928362384,
-231.109601917595,-231.035275603271,-230.960936961917,-230.886573531877,
-230.812138291546,-230.737661834807,-230.663095478887,-230.632249859762,
-230.54608776447,-230.46167604618,-230.374638762388,-230.287601478596),
 .UNSPECIFIED.);
#530=B_SPLINE_CURVE_WITH_KNOTS('',3,(#61222,#61223,#61224,#61225,#61226,
#61227,#61228,#61229,#61230,#61231,#61232,#61233,#61234,#61235,#61236,#61237,
#61238,#61239),.UNSPECIFIED.,.F.,.F.,(4,2,2,2,2,2,2,2,4),(-230.287601478596,
-229.452684566701,-228.617767654806,-227.782850742911,-226.947933831016,
-226.113016919122,-225.278100007227,-224.443183095332,-224.004416171416),
 .UNSPECIFIED.);
#531=B_SPLINE_CURVE_WITH_KNOTS('',3,(#61241,#61242,#61243,#61244,#61245,
#61246,#61247,#61248,#61249,#61250,#61251),.UNSPECIFIED.,.F.,.F.,(4,1,1,
1,1,1,1,1,4),(-224.004416171416,-223.643393803405,-223.14418979938,-222.644985795355,
-221.646577787304,-220.648169779253,-219.649761771202,-218.651353763151,
-217.72156918778),.UNSPECIFIED.);
#532=B_SPLINE_CURVE_WITH_KNOTS('',3,(#61253,#61254,#61255,#61256,#61257,
#61258,#61259,#61260,#61261,#61262,#61263,#61264,#61265,#61266,#61267,#61268,
#61269,#61270,#61271,#61272,#61273,#61274,#61275,#61276,#61277,#61278,#61279,
#61280,#61281,#61282,#61283,#61284,#61285,#61286,#61287,#61288,#61289,#61290,
#61291,#61292,#61293,#61294,#61295,#61296,#61297,#61298,#61299,#61300,#61301,
#61302,#61303,#61304,#61305,#61306,#61307,#61308,#61309,#61310,#61311,#61312,
#61313,#61314,#61315,#61316,#61317,#61318,#61319,#61320,#61321,#61322,#61323,
#61324,#61325,#61326,#61327,#61328,#61329,#61330,#61331,#61332,#61333,#61334,
#61335,#61336,#61337,#61338,#61339,#61340,#61341,#61342,#61343,#61344,#61345,
#61346,#61347,#61348,#61349,#61350,#61351,#61352,#61353,#61354,#61355,#61356,
#61357,#61358,#61359,#61360,#61361,#61362,#61363,#61364,#61365,#61366,#61367,
#61368,#61369,#61370,#61371,#61372,#61373,#61374,#61375,#61376,#61377,#61378,
#61379,#61380,#61381,#61382,#61383,#61384,#61385,#61386,#61387,#61388,#61389,
#61390,#61391,#61392,#61393,#61394,#61395,#61396,#61397,#61398,#61399,#61400,
#61401,#61402,#61403,#61404,#61405,#61406,#61407,#61408,#61409,#61410,#61411,
#61412,#61413,#61414,#61415,#61416,#61417,#61418,#61419,#61420,#61421,#61422,
#61423,#61424,#61425,#61426,#61427,#61428,#61429,#61430,#61431,#61432,#61433,
#61434,#61435,#61436,#61437,#61438,#61439,#61440,#61441,#61442,#61443,#61444,
#61445,#61446,#61447,#61448,#61449,#61450,#61451,#61452,#61453,#61454,#61455,
#61456,#61457,#61458,#61459,#61460,#61461,#61462,#61463,#61464,#61465,#61466,
#61467,#61468,#61469,#61470,#61471,#61472,#61473,#61474,#61475,#61476,#61477,
#61478,#61479,#61480,#61481,#61482,#61483,#61484,#61485,#61486,#61487,#61488,
#61489,#61490,#61491,#61492,#61493,#61494,#61495,#61496,#61497,#61498,#61499,
#61500,#61501,#61502,#61503,#61504,#61505,#61506,#61507,#61508,#61509,#61510,
#61511,#61512,#61513,#61514,#61515,#61516,#61517,#61518,#61519,#61520,#61521,
#61522,#61523,#61524,#61525,#61526,#61527,#61528,#61529,#61530,#61531,#61532,
#61533,#61534,#61535,#61536,#61537,#61538,#61539,#61540,#61541,#61542,#61543,
#61544,#61545,#61546,#61547,#61548,#61549,#61550,#61551,#61552,#61553,#61554,
#61555,#61556,#61557,#61558,#61559,#61560,#61561,#61562,#61563,#61564,#61565,
#61566,#61567,#61568,#61569,#61570,#61571,#61572,#61573,#61574,#61575,#61576,
#61577,#61578,#61579,#61580,#61581,#61582,#61583,#61584,#61585,#61586,#61587,
#61588,#61589,#61590,#61591,#61592,#61593,#61594,#61595,#61596,#61597,#61598,
#61599,#61600,#61601,#61602,#61603,#61604,#61605,#61606,#61607,#61608,#61609,
#61610,#61611,#61612,#61613,#61614,#61615,#61616,#61617,#61618,#61619,#61620,
#61621,#61622,#61623,#61624,#61625,#61626,#61627,#61628,#61629,#61630,#61631,
#61632,#61633,#61634,#61635,#61636,#61637,#61638,#61639,#61640,#61641,#61642,
#61643,#61644,#61645,#61646,#61647,#61648,#61649,#61650,#61651,#61652,#61653,
#61654,#61655,#61656,#61657,#61658,#61659,#61660,#61661,#61662,#61663,#61664,
#61665,#61666,#61667,#61668,#61669,#61670,#61671,#61672,#61673,#61674,#61675,
#61676,#61677,#61678,#61679,#61680,#61681,#61682,#61683,#61684,#61685,#61686,
#61687,#61688,#61689,#61690,#61691,#61692,#61693,#61694,#61695,#61696,#61697,
#61698,#61699,#61700,#61701,#61702,#61703,#61704,#61705,#61706,#61707,#61708,
#61709,#61710,#61711,#61712,#61713,#61714,#61715,#61716,#61717,#61718,#61719,
#61720,#61721,#61722,#61723,#61724,#61725,#61726,#61727,#61728,#61729,#61730,
#61731,#61732,#61733,#61734,#61735,#61736,#61737,#61738,#61739,#61740,#61741,
#61742,#61743,#61744,#61745,#61746,#61747,#61748,#61749,#61750,#61751,#61752,
#61753,#61754,#61755,#61756,#61757,#61758,#61759,#61760,#61761,#61762,#61763,
#61764,#61765,#61766,#61767,#61768,#61769,#61770,#61771,#61772,#61773,#61774,
#61775,#61776,#61777,#61778,#61779,#61780,#61781,#61782,#61783,#61784,#61785,
#61786,#61787,#61788,#61789,#61790,#61791,#61792,#61793,#61794,#61795,#61796,
#61797,#61798,#61799,#61800,#61801,#61802,#61803,#61804,#61805,#61806,#61807,
#61808,#61809,#61810,#61811,#61812,#61813,#61814,#61815,#61816,#61817,#61818,
#61819,#61820,#61821,#61822,#61823,#61824,#61825,#61826,#61827,#61828,#61829,
#61830,#61831,#61832,#61833,#61834,#61835,#61836,#61837,#61838,#61839,#61840),
 .UNSPECIFIED.,.F.,.F.,(4,2,2,2,2,2,2,2,2,2,2,2,2,2,2,2,2,2,2,2,2,2,2,2,
2,2,2,2,2,2,2,2,2,2,2,2,2,2,2,2,2,2,2,2,2,2,2,2,2,2,2,2,2,2,2,2,2,2,2,2,
2,2,2,2,2,2,2,2,2,2,2,2,2,2,2,2,2,2,2,2,2,2,2,2,2,2,2,2,2,2,2,2,2,2,2,2,
2,2,2,2,2,2,2,2,2,2,2,2,2,2,2,2,2,2,2,2,2,2,2,2,2,2,2,2,2,2,2,2,2,2,2,2,
2,2,2,2,2,2,2,2,2,2,2,2,2,2,2,2,2,2,2,2,2,2,2,2,2,2,2,2,2,2,2,2,2,2,2,2,
2,2,2,2,2,2,2,2,2,2,2,2,2,2,2,2,2,2,2,2,2,2,2,2,2,2,2,2,2,2,2,2,2,2,2,2,
2,2,2,2,2,2,2,2,2,2,2,2,2,2,2,2,2,2,2,2,2,2,2,2,2,2,2,2,2,2,2,2,2,2,2,2,
2,2,2,2,2,2,2,2,2,2,2,2,2,2,2,2,2,2,2,2,2,2,2,2,2,2,2,2,2,2,2,2,2,2,2,2,
2,2,2,2,2,2,2,2,2,2,2,2,2,2,2,2,2,4),(0.00206310016479781,0.0503830808988502,
0.0524268792653076,0.0537113840937123,0.0546855606875728,0.0556157387795359,
0.0565331450836818,0.0577822267195454,0.0608769462524458,0.0935667358570958,
0.1050112952103,0.111035653215168,0.314970378675905,0.401194488205747,0.438624331519552,
0.461707117851576,0.465769564042696,0.467926747858301,0.469528949649375,
0.471273994897825,0.47434733835435,0.483275900280479,0.615286404134497,
0.779705853341372,0.809798541705046,0.853665089400275,0.861264784104124,
0.863554516051205,0.864772757973366,0.865954029160069,0.867445851268963,
0.870051938062555,0.880138893397435,0.924874815266039,0.936994950550609,
0.994714499242434,1.2123573467069,1.23277386820493,1.23812548660565,1.24130270669334,
1.24411220545776,1.24759068569905,1.25290262742621,1.27631830806268,1.48964407782103,
1.55146882682353,1.60674164603289,1.61508168623236,1.61745016216806,1.61867848455857,
1.61994433840325,1.62144310093537,1.62407871012408,1.63444026869955,1.77621953920154,
1.78426404396731,1.79278687508964,1.80185911913089,1.81161153821605,1.82273199832761,
1.83565044281444,1.8760704311336,1.97107068491241,2.0076309153499,2.01217817501339,
2.01443619117316,2.01605140115547,2.01775300509979,2.02060734889288,2.02807630094551,
2.03850181331873,2.27302087060922,2.33280349377825,2.38408334667411,2.42022489038964,
2.42410898851928,2.42612583156773,2.42739626748279,2.4285707187389,2.42952722188195,
2.43050431717203,2.43228148880858,2.43784170035034,2.52175079767785,2.66773110152632,
2.68062829070292,2.69527981906675,2.71238587228607,2.73332634436571,2.80813180918227,
2.81989523498609,2.82315863662191,2.82512998084907,2.82689754568116,2.82913766797792,
2.8326592287791,2.84966268797417,3.11256124669895,3.18219832174056,3.21388663176762,
3.21748591363248,3.21940002903702,3.221038478741,3.22209825401321,3.22312074147338,
3.22445873952079,3.22740134016791,3.25034111695839,3.25843999198882,3.27085456177941,
3.51214882728638,3.53475104444254,3.6047200735571,3.61619208221541,3.61950899512696,
3.62154231425786,3.62338483797292,3.62574679157748,3.63043574870699,3.65853730710928,
3.67356311277806,3.69050409043141,3.70590656980858,3.91032771053457,3.96549540892021,
4.00215786217311,4.00819452700101,4.01001600897586,4.0111499157126,4.01219311549608,
4.01354440980433,4.01578683988271,4.02849820005397,4.26180438945362,4.35871582069006,
4.3928242017781,4.39741112977155,4.39971954046507,4.40138299013086,4.40314672016327,
4.4056309907901,4.41224320552322,4.51384354609371,4.63504977813863,4.79018231719396,
4.79696018365848,4.798832716037,4.79996187339252,4.80097293518431,4.80225232568065,
4.80427852685768,4.81464032610943,4.9804847213518,5.17699161328337,5.19028798177488,
5.19382180852563,5.19587441880517,5.19761605201889,5.19973372719817,5.20366129217755,
5.22457098790241,5.26514513426225,5.32120287336182,5.44559659092256,5.58052483305719,
5.58928706209074,5.59118928099527,5.59241515470495,5.59339298482172,5.59450014689056,
5.5963939414982,5.60392141263613,5.66015899823546,5.7215552360471,5.77432099869787,
5.935069984782,5.99637252378493,6.00207093649415,6.00436045967791,6.00603843468076,
6.00784625333532,6.01028511648299,6.01577378256877,6.16866215801806,6.38430459804151,
6.39765430389124,6.40030628043358,6.40197341546939,6.40327551592991,6.40471404085846,
6.4070641912719,6.41522512405134,6.46852745557286,6.60612801272068,6.76284545390843,
6.77271232154962,6.77681114385611,6.77969007276274,6.78258451836723,6.7866260816601,
6.79636235057872,6.93074609026676,7.12197422784265,7.15032312910918,7.1540446765417,
7.15575265618913,7.15706465232665,7.15847040969394,7.1606736765203,7.16752856212847,
7.2046198739944,7.24680847773683,7.34191888203779,7.52801785552134,7.54619237175491,
7.54981657912374,7.55209781692984,7.55388260738899,7.55581775232708,7.55894617490725,
7.56264338306019,7.56974643342612,7.74261913193179,7.94333614781604,7.96217241167257,
7.9646072101625,7.96584979040548,7.96676565124097,7.96776589714003,7.96914230870995,
7.97235786706012,8.06367268210611,8.08306778812237,8.11984415901366,8.14127209378237,
8.14974394819524,8.15773510773838,8.16529839580869,8.27254291014769,8.35295157072723,
8.35902442377338,8.36136680065576,8.36305015096787,8.36479717037477,8.36708132604246,
8.36959434710459,8.37374464171974,8.38208473358466,8.403355825419,8.4988422555759,
8.73452908597825,8.75501855572248,8.75781282705858,8.75911342753162,8.76013015564565,
8.76123710290569,8.76300947734345,8.76883235216942,8.80381803636421,8.88752819026766,
8.94302869918772,9.01134908143064,9.0542897768729,9.14819909920552,9.15468928526942,
9.157154366426,9.15891331450244,9.16072757532108,9.16308176044369,9.16566544862633,
9.16990964051844,9.17838792908977,9.19986146006793,9.29844891000985,9.53174040719135,
9.54452699237474,9.54677433952639,9.54812730814649,9.5491710263944,9.55030470425575,
9.55212414289312,9.55813928698537,9.59458800176715,9.64485976923376,9.91441346941936,
9.92561650147807,9.9335914794583,9.93657942754645,9.93834386281007,9.94011759325285,
9.94190715232923,9.94420607027357,9.95041883173145,9.95922074868957),
 .UNSPECIFIED.);
#533=B_SPLINE_CURVE_WITH_KNOTS('',3,(#61842,#61843,#61844,#61845,#61846,
#61847,#61848,#61849,#61850,#61851,#61852,#61853,#61854,#61855,#61856,#61857,
#61858,#61859,#61860,#61861,#61862,#61863,#61864,#61865,#61866,#61867,#61868,
#61869,#61870,#61871,#61872,#61873,#61874,#61875,#61876,#61877,#61878,#61879,
#61880,#61881,#61882,#61883,#61884,#61885,#61886,#61887,#61888,#61889,#61890,
#61891,#61892,#61893,#61894,#61895,#61896,#61897,#61898,#61899,#61900,#61901,
#61902,#61903,#61904,#61905,#61906,#61907,#61908,#61909,#61910,#61911,#61912,
#61913,#61914,#61915,#61916,#61917,#61918,#61919,#61920,#61921,#61922,#61923,
#61924,#61925,#61926,#61927,#61928,#61929,#61930,#61931,#61932,#61933,#61934,
#61935,#61936,#61937,#61938,#61939,#61940,#61941,#61942,#61943,#61944,#61945,
#61946,#61947,#61948,#61949,#61950,#61951,#61952,#61953,#61954,#61955,#61956,
#61957,#61958,#61959,#61960,#61961,#61962,#61963,#61964,#61965,#61966,#61967,
#61968,#61969,#61970,#61971,#61972,#61973,#61974,#61975,#61976,#61977,#61978,
#61979,#61980,#61981,#61982,#61983,#61984,#61985,#61986,#61987,#61988,#61989,
#61990,#61991,#61992,#61993,#61994,#61995,#61996,#61997,#61998,#61999,#62000,
#62001,#62002,#62003,#62004,#62005,#62006,#62007,#62008,#62009,#62010,#62011,
#62012,#62013,#62014,#62015,#62016,#62017,#62018,#62019,#62020,#62021,#62022,
#62023,#62024,#62025,#62026,#62027,#62028,#62029,#62030,#62031,#62032,#62033,
#62034,#62035,#62036,#62037,#62038,#62039,#62040,#62041,#62042,#62043,#62044,
#62045,#62046,#62047,#62048,#62049,#62050,#62051,#62052,#62053,#62054,#62055,
#62056,#62057,#62058,#62059,#62060,#62061,#62062,#62063,#62064,#62065,#62066,
#62067,#62068,#62069,#62070,#62071,#62072,#62073,#62074,#62075,#62076,#62077,
#62078,#62079,#62080,#62081,#62082,#62083,#62084,#62085,#62086,#62087,#62088,
#62089,#62090,#62091,#62092,#62093,#62094,#62095,#62096,#62097,#62098,#62099,
#62100,#62101,#62102,#62103,#62104,#62105,#62106,#62107,#62108,#62109,#62110,
#62111,#62112,#62113,#62114,#62115,#62116,#62117,#62118,#62119,#62120,#62121,
#62122,#62123,#62124,#62125,#62126,#62127,#62128,#62129,#62130,#62131,#62132,
#62133,#62134,#62135,#62136,#62137,#62138,#62139,#62140,#62141,#62142,#62143,
#62144,#62145,#62146,#62147,#62148,#62149,#62150,#62151,#62152,#62153,#62154,
#62155,#62156,#62157,#62158,#62159,#62160,#62161,#62162,#62163,#62164,#62165,
#62166,#62167,#62168,#62169,#62170,#62171,#62172,#62173,#62174,#62175,#62176,
#62177,#62178,#62179,#62180,#62181,#62182,#62183,#62184,#62185,#62186,#62187,
#62188,#62189,#62190,#62191,#62192,#62193,#62194,#62195,#62196,#62197,#62198,
#62199,#62200,#62201,#62202,#62203,#62204,#62205,#62206,#62207,#62208,#62209,
#62210,#62211,#62212,#62213,#62214,#62215,#62216,#62217,#62218,#62219,#62220,
#62221,#62222,#62223,#62224,#62225,#62226,#62227,#62228,#62229,#62230,#62231,
#62232,#62233,#62234,#62235,#62236,#62237,#62238,#62239,#62240,#62241,#62242,
#62243,#62244,#62245,#62246,#62247,#62248,#62249,#62250,#62251,#62252,#62253,
#62254,#62255,#62256,#62257,#62258,#62259,#62260,#62261,#62262,#62263,#62264,
#62265,#62266,#62267,#62268,#62269,#62270,#62271,#62272,#62273,#62274,#62275,
#62276,#62277,#62278,#62279,#62280,#62281,#62282,#62283,#62284,#62285,#62286,
#62287,#62288,#62289,#62290,#62291,#62292,#62293,#62294,#62295,#62296,#62297,
#62298,#62299,#62300,#62301,#62302,#62303,#62304,#62305,#62306,#62307,#62308,
#62309,#62310,#62311,#62312,#62313,#62314,#62315,#62316,#62317,#62318,#62319,
#62320,#62321,#62322,#62323,#62324,#62325,#62326,#62327,#62328,#62329,#62330,
#62331,#62332,#62333,#62334,#62335,#62336,#62337,#62338,#62339,#62340,#62341,
#62342,#62343,#62344,#62345,#62346,#62347,#62348,#62349,#62350,#62351,#62352,
#62353,#62354,#62355,#62356,#62357,#62358,#62359,#62360,#62361,#62362,#62363,
#62364,#62365,#62366,#62367,#62368,#62369,#62370,#62371,#62372,#62373,#62374,
#62375,#62376,#62377,#62378,#62379,#62380,#62381,#62382,#62383,#62384,#62385,
#62386,#62387,#62388,#62389,#62390,#62391,#62392,#62393,#62394,#62395,#62396,
#62397,#62398,#62399,#62400,#62401,#62402,#62403,#62404,#62405,#62406,#62407),
 .UNSPECIFIED.,.F.,.F.,(4,2,2,2,2,2,2,2,2,2,2,2,2,2,2,2,2,2,2,2,2,2,2,2,
2,2,2,2,2,2,2,2,2,2,2,2,2,2,2,2,2,2,2,2,2,2,2,2,2,2,2,2,2,2,2,2,2,2,2,2,
2,2,2,2,2,2,2,2,2,2,2,2,2,2,2,2,2,2,2,2,2,2,2,2,2,2,2,2,2,2,2,2,2,2,2,2,
2,2,2,2,2,2,2,2,2,2,2,2,2,2,2,2,2,2,2,2,2,2,2,2,2,2,2,2,2,2,2,2,2,2,2,2,
2,2,2,2,2,2,2,2,2,2,2,2,2,2,2,2,2,2,2,2,2,2,2,2,2,2,2,2,2,2,2,2,2,2,2,2,
2,2,2,2,2,2,2,2,2,2,2,2,2,2,2,2,2,2,2,2,2,2,2,2,2,2,2,2,2,2,2,2,2,2,2,2,
2,2,2,2,2,2,2,2,2,2,2,2,2,2,2,2,2,2,2,2,2,2,2,2,2,2,2,2,2,2,2,2,2,2,2,2,
2,2,2,2,2,2,2,2,2,2,2,2,2,2,2,2,2,2,2,2,2,2,2,2,2,2,2,2,2,2,2,2,2,2,2,2,
2,2,2,2,2,2,4),(0.00297604451504543,0.307437594455464,0.371161582836229,
0.379255930588295,0.381247520469777,0.382403600670181,0.383309176057065,
0.384345273648609,0.386278223922282,0.393296840400095,0.395251204720802,
0.398779986928545,0.593253181120357,0.691488307478245,0.743883918454952,
0.762198970999362,0.769655411505022,0.773477566485675,0.775853344079466,
0.778038881741714,0.779772412711776,0.781493345206249,0.78449037278834,
0.792982494912627,0.915805534751877,0.979539837164022,1.10465434478413,
1.17036313763555,1.1735306101825,1.17489870280763,1.17589756473639,1.17681548228123,
1.17806592797039,1.18116733851056,1.21409251601541,1.21593559283684,1.22744211855453,
1.44952133152978,1.52092898355953,1.55842920282579,1.57395891958729,1.58056674656611,
1.58558795220044,1.58793303887868,1.58962626431515,1.59129807907288,1.59356216125344,
1.59911117744845,1.65484153748527,1.79242955617571,1.89923289445484,1.95089881172431,
1.97005669899383,1.98111263644824,1.98372308061504,1.98521991715767,1.98638393472394,
1.98790746088799,1.99056597055898,2.00096940227494,2.22509849381014,2.34676947668228,
2.35626025360985,2.36026027329891,2.36314700288535,2.36603848037698,2.36964317389163,
2.37856060223993,2.48473765140089,2.64649835660391,2.73302726055399,2.73695610015258,
2.7387215099047,2.74003802516155,2.74126542759059,2.74294856164591,2.74628966608516,
2.77775701226603,2.78175289936853,2.78928274531461,3.00484017421296,3.12598854685781,
3.13021172120628,3.13276123370063,3.13507577787528,3.13671210928667,3.13838279165264,
3.1406434214609,3.14504422548245,3.17816986231892,3.46132153087943,3.54456974636974,
3.54800428252614,3.54941266875121,3.55041630498528,3.55132839782235,3.55254522833223,
3.55562205260018,3.58479459260071,3.62643865815275,3.74345924115258,3.8530262304217,
3.92922045931211,3.94111141824744,3.94438767945159,3.94636210433657,3.9481294400624,
3.95036521914059,3.95387211645877,3.97067168829991,4.25778194441792,4.3039555196626,
4.33541480080938,4.34081291708075,4.34251147315146,4.34360100664821,4.3446241634064,
4.34596504757275,4.34892217336037,4.37224606333591,4.37340568177209,4.37854279327014,
4.6074609443119,4.66508628406531,4.7272497041009,4.73789784371986,4.74112600388234,
4.74313979742355,4.74498806245511,4.74735078358507,4.75233381235465,4.78517478513079,
4.80684465962293,4.98433108496847,5.12055812093897,5.1291405271459,5.13109510562046,
5.13237296979,5.13330232349179,5.13445752615367,5.13637327528557,5.1433083719927,
5.18927518278472,5.2668165488979,5.46399155217598,5.47532633709226,5.51340949858671,
5.51809439553617,5.52046418719999,5.52219792213742,5.52406292820472,5.52657398371105,
5.53220466867101,5.67642466639299,5.72053638009082,5.76500723477777,5.90896649712754,
5.91417333741174,5.91896864453272,5.9206743033543,5.92165729671086,5.92256875403068,
5.92380933825557,5.92622024849291,5.94295877815542,6.00738768862343,6.29512649075997,
6.31187547115639,6.31537819654718,6.31761247268939,6.31937936536836,6.32135407368037,
6.32463261972384,6.33655099305369,6.41305219834724,6.49526811434365,6.56925826906714,
6.69111758263847,6.71042500927461,6.71316101123142,6.71443528017928,6.71542196401978,
6.71646875238109,6.71813284813966,6.72009355819043,6.72383004418041,6.75773049938111,
6.8266694698301,7.10388523573989,7.10798986267781,7.12239621138787,7.12572980339555,
7.12792063962473,7.12969612359525,7.131726991057,7.13521221963925,7.14922218997859,
7.25763239225117,7.4131035066815,7.51399770638478,7.5211549643648,7.52348475684752,
7.52477484031725,7.52596616939829,7.52748700439794,7.52911928285559,7.53166135700761,
7.57745200546682,7.63557718244864,7.76599743200456,7.88612986163292,7.89523816174119,
7.89887334340797,7.90153171623142,7.90438066997776,7.90816976331211,7.91648526544872,
7.92741268943911,7.98828338399325,8.03065488990954,8.06294655311029,8.21280309397782,
8.2541827693215,8.27287353881204,8.27609479471951,8.27775780835643,8.2790327298689,
8.28043597663861,8.28189482683876,8.28402014868918,8.28773580088015,8.38895564237337,
8.65202188565386,8.66852788552615,8.67203001351949,8.67427312774102,8.67605300868926,
8.6780485304051,8.68137639368066,8.69363168376002,8.77323978297454,8.84243184117943,
8.86339574401253,8.88090405450091,8.89586133592198,8.90883022829153,8.92019388978084,
8.93023225685929,8.93916413156648,9.01647757493111,9.06093313200018,9.08345251082273,
9.08630076212298,9.08759082221684,9.08857785133288,9.08949221786674,9.09053709880988,
9.0934679614785,9.1280133170749,9.18304705224816,9.39561539070965,9.47449716416361,
9.48053747718202,9.48287356665185,9.48455452351055,9.48615841483564,9.48841403280086,
9.49300685956648,9.53261967100893,9.64047168806455,9.7997260697482,9.8064626528913,
9.82537131618962,9.87484558918037,9.87831908295523,9.87964774310392,9.8806071984042,
9.88157659059722,9.8825689995385,9.88385749356293,9.88587848619483,9.90123656120509,
9.96079208582225),.UNSPECIFIED.);
#534=B_SPLINE_CURVE_WITH_KNOTS('',3,(#62409,#62410,#62411,#62412,#62413,
#62414,#62415,#62416,#62417,#62418,#62419,#62420,#62421,#62422,#62423,#62424,
#62425,#62426,#62427,#62428,#62429,#62430,#62431,#62432,#62433,#62434,#62435,
#62436,#62437,#62438,#62439,#62440,#62441,#62442,#62443,#62444,#62445,#62446,
#62447,#62448,#62449,#62450,#62451,#62452,#62453,#62454,#62455,#62456,#62457,
#62458,#62459,#62460,#62461,#62462,#62463,#62464,#62465,#62466,#62467,#62468,
#62469,#62470,#62471,#62472,#62473,#62474,#62475,#62476,#62477,#62478,#62479,
#62480,#62481,#62482,#62483,#62484,#62485,#62486,#62487,#62488,#62489,#62490,
#62491,#62492,#62493,#62494,#62495,#62496,#62497,#62498,#62499,#62500,#62501,
#62502,#62503,#62504,#62505,#62506,#62507,#62508,#62509,#62510,#62511,#62512,
#62513,#62514,#62515,#62516,#62517,#62518,#62519,#62520,#62521,#62522,#62523,
#62524,#62525,#62526,#62527,#62528,#62529,#62530,#62531,#62532,#62533,#62534,
#62535,#62536,#62537,#62538,#62539,#62540,#62541,#62542,#62543,#62544,#62545,
#62546,#62547,#62548,#62549,#62550,#62551,#62552,#62553,#62554,#62555,#62556,
#62557,#62558,#62559,#62560,#62561,#62562,#62563,#62564,#62565,#62566,#62567,
#62568,#62569,#62570,#62571,#62572,#62573,#62574,#62575,#62576,#62577,#62578,
#62579,#62580,#62581,#62582,#62583,#62584,#62585,#62586,#62587,#62588,#62589,
#62590,#62591,#62592,#62593,#62594,#62595,#62596,#62597,#62598,#62599,#62600,
#62601,#62602,#62603,#62604,#62605,#62606,#62607,#62608,#62609,#62610,#62611,
#62612,#62613,#62614,#62615,#62616,#62617,#62618,#62619,#62620,#62621,#62622,
#62623,#62624,#62625,#62626,#62627,#62628,#62629,#62630,#62631,#62632,#62633,
#62634,#62635,#62636,#62637,#62638,#62639,#62640,#62641,#62642,#62643,#62644,
#62645,#62646,#62647,#62648,#62649,#62650,#62651,#62652,#62653,#62654,#62655,
#62656,#62657,#62658,#62659,#62660,#62661,#62662,#62663,#62664,#62665,#62666,
#62667,#62668,#62669,#62670,#62671,#62672,#62673),.UNSPECIFIED.,.F.,.F.,
(4,3,3,3,3,3,3,3,3,3,3,3,3,3,3,3,3,3,3,3,3,3,3,3,3,3,3,3,3,3,3,3,3,3,3,
3,3,3,3,3,3,3,3,3,3,3,3,3,3,3,3,3,3,3,3,3,3,3,3,3,3,3,3,3,3,3,3,3,3,3,3,
3,3,3,3,3,3,3,3,3,3,3,3,3,3,3,3,3,4),(-192.588489635518,-192.514976588221,
-192.441536697609,-192.368155301087,-192.294817783453,-192.219757753744,
-192.146453138469,-192.073145745637,-191.999822398974,-191.923451185674,
-191.850020602564,-191.776543231949,-191.702976492768,-191.694337545776,
-191.619776559642,-191.545296395256,-191.470883139413,-191.39652292312,
-191.322201912616,-191.247906300795,-191.173609562286,-191.099308218751,
-191.024989780242,-190.95064175013,-190.876214580866,-190.801742011321,
-190.727173108861,-190.695929537725,-190.622036056471,-190.548225190329,
-190.474482494906,-190.400793576011,-190.327144078784,-190.2535196776,-190.179891830674,
-190.106257964606,-190.032605122391,-189.958920338183,-189.885149785285,
-189.81133107467,-189.737406423803,-189.697521529674,-189.62289846426,-189.548361135379,
-189.473895646626,-189.399488148984,-189.325124831742,-189.250791913841,
-189.176465451246,-189.102139119291,-189.027800460494,-188.953437013215,
-188.879001756033,-188.804525282641,-188.7299589105,-188.699113521623,-188.620747847582,
-188.542478678145,-188.464300731748,-188.386239959557,-188.308250897303,
-188.230351044309,-188.199909517598,-188.121998929484,-188.04401853258,
-187.965963202718,-187.887778486963,-187.809523107355,-187.731148416719,
-187.700705513572,-187.626146417045,-187.551662767433,-187.477240704328,
-187.40286640789,-187.328526090098,-187.254205986351,-187.179877117193,
-187.105538884002,-187.031178825652,-186.95678447185,-186.882304118277,
-186.807774365277,-186.733142634435,-186.702297505521,-186.619885579121,
-186.537828525829,-186.455989679252,-186.374521751061,-186.305304328339),
 .UNSPECIFIED.);
#535=B_SPLINE_CURVE_WITH_KNOTS('',3,(#62675,#62676,#62677,#62678,#62679,
#62680,#62681,#62682,#62683,#62684,#62685,#62686,#62687,#62688,#62689,#62690,
#62691,#62692),.UNSPECIFIED.,.F.,.F.,(4,2,2,2,2,2,2,2,4),(-186.305304328339,
-185.470387416444,-184.635470504549,-183.800553592654,-182.965636680759,
-182.130719768864,-181.29580285697,-180.460885945075,-180.022119021159),
 .UNSPECIFIED.);
#536=B_SPLINE_CURVE_WITH_KNOTS('',3,(#62694,#62695,#62696,#62697,#62698,
#62699,#62700,#62701,#62702,#62703,#62704,#62705,#62706,#62707,#62708,#62709,
#62710,#62711,#62712,#62713,#62714,#62715,#62716,#62717,#62718,#62719,#62720,
#62721,#62722,#62723,#62724,#62725,#62726,#62727,#62728,#62729,#62730,#62731,
#62732,#62733,#62734,#62735,#62736,#62737,#62738,#62739,#62740,#62741,#62742,
#62743,#62744,#62745,#62746,#62747,#62748,#62749,#62750,#62751,#62752,#62753,
#62754,#62755,#62756,#62757,#62758,#62759,#62760,#62761,#62762,#62763,#62764,
#62765,#62766,#62767,#62768,#62769,#62770,#62771,#62772,#62773,#62774,#62775,
#62776,#62777,#62778,#62779,#62780,#62781,#62782,#62783,#62784,#62785,#62786,
#62787,#62788,#62789,#62790,#62791,#62792,#62793,#62794,#62795,#62796,#62797,
#62798,#62799,#62800,#62801,#62802,#62803,#62804,#62805,#62806,#62807,#62808,
#62809,#62810,#62811,#62812,#62813,#62814,#62815,#62816,#62817,#62818,#62819,
#62820,#62821,#62822,#62823,#62824,#62825,#62826,#62827,#62828,#62829,#62830,
#62831,#62832,#62833,#62834,#62835,#62836,#62837,#62838,#62839,#62840,#62841,
#62842,#62843,#62844,#62845,#62846,#62847,#62848,#62849,#62850,#62851,#62852,
#62853,#62854,#62855,#62856,#62857,#62858,#62859,#62860,#62861,#62862,#62863,
#62864,#62865,#62866,#62867,#62868,#62869,#62870,#62871,#62872,#62873,#62874,
#62875,#62876,#62877,#62878,#62879,#62880,#62881,#62882,#62883,#62884,#62885,
#62886,#62887,#62888,#62889,#62890,#62891,#62892,#62893,#62894,#62895,#62896,
#62897,#62898,#62899,#62900,#62901,#62902,#62903,#62904,#62905,#62906,#62907,
#62908,#62909,#62910,#62911,#62912,#62913,#62914,#62915,#62916,#62917,#62918,
#62919,#62920,#62921,#62922,#62923,#62924,#62925,#62926,#62927,#62928,#62929,
#62930,#62931,#62932,#62933,#62934,#62935,#62936,#62937,#62938,#62939,#62940,
#62941,#62942,#62943,#62944,#62945,#62946,#62947,#62948,#62949,#62950,#62951,
#62952,#62953,#62954,#62955,#62956,#62957,#62958,#62959,#62960,#62961,#62962,
#62963,#62964,#62965,#62966,#62967,#62968,#62969,#62970,#62971,#62972,#62973,
#62974,#62975,#62976,#62977,#62978,#62979,#62980,#62981,#62982,#62983,#62984,
#62985,#62986,#62987,#62988,#62989,#62990,#62991,#62992,#62993,#62994,#62995,
#62996,#62997,#62998,#62999,#63000,#63001,#63002,#63003,#63004,#63005,#63006,
#63007,#63008,#63009,#63010,#63011,#63012,#63013,#63014,#63015,#63016,#63017,
#63018,#63019,#63020,#63021,#63022,#63023,#63024,#63025,#63026,#63027,#63028,
#63029,#63030,#63031,#63032,#63033,#63034,#63035,#63036,#63037,#63038,#63039,
#63040,#63041,#63042,#63043,#63044,#63045,#63046,#63047,#63048,#63049,#63050,
#63051,#63052,#63053,#63054,#63055,#63056,#63057,#63058,#63059,#63060,#63061,
#63062,#63063,#63064,#63065,#63066,#63067,#63068,#63069,#63070,#63071,#63072,
#63073,#63074,#63075,#63076,#63077,#63078,#63079,#63080,#63081,#63082,#63083,
#63084,#63085,#63086,#63087,#63088,#63089,#63090,#63091,#63092,#63093,#63094,
#63095,#63096,#63097,#63098,#63099,#63100,#63101,#63102,#63103,#63104,#63105,
#63106,#63107,#63108,#63109,#63110,#63111,#63112,#63113,#63114,#63115,#63116,
#63117,#63118,#63119,#63120,#63121,#63122,#63123,#63124,#63125,#63126,#63127,
#63128,#63129,#63130,#63131,#63132,#63133,#63134,#63135,#63136,#63137,#63138,
#63139,#63140,#63141,#63142,#63143,#63144,#63145,#63146,#63147,#63148,#63149,
#63150,#63151,#63152,#63153,#63154,#63155,#63156,#63157,#63158,#63159,#63160,
#63161,#63162,#63163,#63164,#63165,#63166,#63167,#63168,#63169,#63170,#63171,
#63172,#63173,#63174,#63175,#63176,#63177,#63178,#63179,#63180,#63181,#63182,
#63183,#63184,#63185,#63186,#63187,#63188,#63189,#63190,#63191,#63192,#63193,
#63194,#63195,#63196,#63197,#63198,#63199,#63200,#63201,#63202,#63203,#63204,
#63205,#63206,#63207,#63208,#63209,#63210,#63211,#63212,#63213,#63214,#63215,
#63216,#63217,#63218,#63219,#63220,#63221,#63222,#63223,#63224,#63225,#63226,
#63227,#63228,#63229,#63230,#63231,#63232,#63233,#63234,#63235,#63236,#63237,
#63238,#63239,#63240,#63241,#63242,#63243,#63244,#63245,#63246,#63247,#63248,
#63249,#63250,#63251,#63252,#63253,#63254,#63255,#63256,#63257,#63258,#63259,
#63260,#63261,#63262,#63263,#63264,#63265),.UNSPECIFIED.,.F.,.F.,(4,2,2,
2,2,2,2,2,2,2,2,2,2,2,2,2,2,2,2,2,2,2,2,2,2,2,2,2,2,2,2,2,2,2,2,2,2,2,2,
2,2,2,2,2,2,2,2,2,2,2,2,2,2,2,2,2,2,2,2,2,2,2,2,2,2,2,2,2,2,2,2,2,2,2,2,
2,2,2,2,2,2,2,2,2,2,2,2,2,2,2,2,2,2,2,2,2,2,2,2,2,2,2,2,2,2,2,2,2,2,2,2,
2,2,2,2,2,2,2,2,2,2,2,2,2,2,2,2,2,2,2,2,2,2,2,2,2,2,2,2,2,2,2,2,2,2,2,2,
2,2,2,2,2,2,2,2,2,2,2,2,2,2,2,2,2,2,2,2,2,2,2,2,2,2,2,2,2,2,2,2,2,2,2,2,
2,2,2,2,2,2,2,2,2,2,2,2,2,2,2,2,2,2,2,2,2,2,2,2,2,2,2,2,2,2,2,2,2,2,2,2,
2,2,2,2,2,2,2,2,2,2,2,2,2,2,2,2,2,2,2,2,2,2,2,2,2,2,2,2,2,2,2,2,2,2,2,2,
2,2,2,2,2,2,2,2,2,2,2,2,2,2,2,2,2,2,2,2,2,2,2,2,2,2,2,2,2,2,4),(0.000947724590819553,
0.207127724815813,0.237603480675008,0.242880588191167,0.24454806825737,
0.245605280156748,0.246596370893857,0.247897236940394,0.250092317633511,
0.263394818606918,0.496507780731943,0.539185768320658,0.599368239939017,
0.634092615263434,0.637474689143311,0.639664733503269,0.641378320251603,
0.642982115041705,0.644665732403467,0.647009945005304,0.653095635135978,
0.734265729789568,0.773633675436147,0.819428004846183,0.856468935458509,
0.929244616464085,0.999233698146093,1.03022547919743,1.03557229837192,1.03726426378135,
1.03835197678722,1.03937509229096,1.04071833863366,1.04369056265577,1.0674666751502,
1.27624187269221,1.34623592121595,1.40374887419738,1.43034062201941,1.4346437913907,
1.43647496164993,1.4383384309352,1.44007228993145,1.4424446574652,1.44838257809628,
1.51476299402155,1.55646798687329,1.65235350094941,1.81737909797484,1.8238598955143,
1.82572896985573,1.8268733157138,1.827913039325,1.82924217797162,1.8314109894856,
1.84292941111115,2.03102121289364,2.12302884815369,2.1817880146853,2.20868202223375,
2.21299716790313,2.21482971293008,2.21669376305457,2.21842644585236,2.22079454252517,
2.2254751322135,2.26345451814496,2.27094355871683,2.28894276717766,2.31901202130812,
2.44949235498463,2.60306616486844,2.61198456835532,2.61404002566128,2.61520983217603,
2.61611504403584,2.61729391293099,2.61935073984407,2.62766473763541,2.62928427099797,
2.78180023384879,2.87161662808824,2.95461954995335,2.99833013804605,3.0066737908653,
3.00953933817333,3.0114346507468,3.0132248437297,3.01558617153086,3.02085848856206,
3.06473938636343,3.06689176072869,3.06916191466725,3.07195523109899,3.08300676476133,
3.11198134261111,3.30343586960334,3.37146407445748,3.40019193855557,3.4052826712274,
3.40693402441988,3.40799128650385,3.40898106329199,3.41028747428738,3.41311212533903,
3.43598862706669,3.58713352953827,3.72251472077341,3.75227710124463,3.79320537088694,
3.81399809294732,3.81814728721038,3.82034046925134,3.82211611135656,3.82388468192189,
3.82707588579124,3.83687548282645,3.97970191705428,4.04970671255117,4.20587742081602,
4.21364676360052,4.21595483122959,4.21738362840693,4.21868757051583,4.2203720321278,
4.2238779960294,4.24695270637007,4.44631528050854,4.50564934072617,4.5683005823847,
4.58560334600116,4.59065052253146,4.59375915044009,4.59657948134747,4.60016936102526,
4.60584209023865,4.63403131682417,4.83859635114614,4.90122413516529,4.95862180999879,
4.96714953793225,4.96953656223199,4.9709830153505,4.97228283698306,4.97393408972684,
4.97727355566071,5.00650734117506,5.05894188475831,5.23631852131014,5.30267282766002,
5.35800922620107,5.36354529296927,5.36580632297705,5.3674766998798,5.36928914001459,
5.37175703927016,5.37740899425566,5.45757053311368,5.56165006970578,5.69696259849524,
5.72505125436997,5.73199767945725,5.74020723493719,5.74476234725454,5.74609425635309,
5.77544634877715,5.77820838015913,5.77953238662084,5.78046893703126,5.78135663674325,
5.78259923590203,5.78510667275141,5.80537919524097,5.83797031438553,5.89430820420481,
6.0440600310955,6.10294065133863,6.16708229607079,6.1728082112456,6.17509146660627,
6.17675860445949,6.17854883283052,6.18095368266124,6.18632300231797,6.30901879048983,
6.44281263648507,6.56181357330139,6.56939936258579,6.57138800788964,6.5725513919714,
6.57355783712935,6.57478616210781,6.57711182033334,6.59060677539225,6.61745918219728,
6.67180106212564,6.81263421994436,6.9564195293122,6.9664508242804,6.96973273109896,
6.97155506533697,6.97336957680026,6.9756275973213,6.97997429000239,7.00732987835108,
7.06765779865156,7.21628891010548,7.34902065517395,7.35744415785545,7.35957373785265,
7.3607889421538,7.36171617998268,7.36291956779403,7.36505431775467,7.37462947939665,
7.53411564240847,7.61622079936947,7.68534691114172,7.7404325119529,7.7456231821168,
7.74811823503617,7.74988443080237,7.75154603463036,7.75384529441409,7.75839047130692,
7.79121409287726,7.88837602215563,7.98157722973941,8.11129590771979,8.11637557863732,
8.12021939221516,8.14426574416599,8.14720831103851,8.14844488823968,8.14947498136198,
8.15053045560553,8.15207130223126,8.15625492477782,8.25410494204454,8.35429125495423,
8.52727441100835,8.53935536900768,8.54276233626839,8.5447848800462,8.54654452689706,
8.54870490193997,8.55283506466141,8.57796827436248,8.63136356925425,8.65162069698498,
8.66698800859803,8.759453349192,8.926934974668,8.9377322885196,8.93977895374562,
8.94104898698024,8.94203161175717,8.94311207996608,8.94488680188714,8.95114340844106,
8.99120102300993,9.07084470575175,9.1028393295956,9.13798902689615,9.27685845217146,
9.344676829327,9.35052880258044,9.35284428392076,9.3545286206513,9.35633135059043,
9.35874263609865,9.36408382080603,9.46995219416744,9.53371155654059,9.56286865554598,
9.5903721922408,9.73669576998189,9.74629825936004,9.74888018862983,9.75038544466215,
9.7516658036195,9.75322652959894,9.75613253866614,9.75974179342287,9.76749543643411,
9.95163942614331),.UNSPECIFIED.);
#537=B_SPLINE_CURVE_WITH_KNOTS('',3,(#63267,#63268,#63269,#63270,#63271,
#63272,#63273,#63274,#63275,#63276,#63277,#63278,#63279,#63280,#63281,#63282,
#63283,#63284),.UNSPECIFIED.,.F.,.F.,(4,2,2,2,2,2,2,2,4),(-167.4557484068,
-166.620831494905,-165.78591458301,-164.950997671115,-164.11608075922,-163.281163847326,
-162.446246935431,-161.611330023536,-161.17256309962),.UNSPECIFIED.);
#538=B_SPLINE_CURVE_WITH_KNOTS('',3,(#63286,#63287,#63288,#63289,#63290,
#63291,#63292,#63293,#63294,#63295,#63296,#63297,#63298,#63299,#63300,#63301,
#63302,#63303,#63304,#63305,#63306,#63307,#63308,#63309,#63310,#63311,#63312,
#63313,#63314,#63315,#63316,#63317,#63318,#63319,#63320,#63321,#63322,#63323,
#63324,#63325,#63326,#63327,#63328,#63329,#63330,#63331,#63332,#63333,#63334,
#63335,#63336,#63337,#63338,#63339,#63340,#63341,#63342,#63343,#63344,#63345,
#63346,#63347,#63348,#63349,#63350,#63351,#63352,#63353,#63354,#63355,#63356,
#63357,#63358,#63359,#63360,#63361,#63362,#63363,#63364,#63365,#63366,#63367,
#63368,#63369,#63370,#63371,#63372,#63373,#63374,#63375,#63376,#63377,#63378,
#63379,#63380,#63381,#63382,#63383,#63384,#63385,#63386,#63387,#63388,#63389,
#63390,#63391,#63392,#63393,#63394,#63395,#63396,#63397,#63398,#63399,#63400,
#63401,#63402,#63403,#63404,#63405,#63406,#63407,#63408,#63409,#63410,#63411,
#63412,#63413,#63414,#63415,#63416,#63417,#63418,#63419,#63420,#63421,#63422,
#63423,#63424,#63425,#63426,#63427,#63428,#63429,#63430,#63431,#63432,#63433,
#63434,#63435,#63436,#63437,#63438,#63439,#63440,#63441,#63442,#63443,#63444,
#63445,#63446,#63447,#63448,#63449,#63450,#63451,#63452,#63453,#63454,#63455,
#63456,#63457,#63458,#63459,#63460,#63461,#63462,#63463,#63464,#63465,#63466,
#63467,#63468,#63469,#63470,#63471,#63472,#63473,#63474,#63475,#63476,#63477,
#63478,#63479,#63480,#63481,#63482,#63483,#63484,#63485,#63486,#63487,#63488,
#63489,#63490,#63491,#63492,#63493,#63494,#63495,#63496,#63497,#63498,#63499,
#63500,#63501,#63502,#63503,#63504,#63505,#63506,#63507,#63508,#63509,#63510,
#63511,#63512,#63513,#63514,#63515,#63516,#63517,#63518,#63519,#63520,#63521,
#63522,#63523,#63524,#63525,#63526,#63527,#63528,#63529,#63530,#63531,#63532,
#63533,#63534,#63535,#63536,#63537,#63538,#63539,#63540,#63541,#63542,#63543,
#63544,#63545,#63546,#63547,#63548,#63549,#63550),.UNSPECIFIED.,.F.,.F.,
(4,3,3,3,3,3,3,3,3,3,3,3,3,3,3,3,3,3,3,3,3,3,3,3,3,3,3,3,3,3,3,3,3,3,3,
3,3,3,3,3,3,3,3,3,3,3,3,3,3,3,3,3,3,3,3,3,3,3,3,3,3,3,3,3,3,3,3,3,3,3,3,
3,3,3,3,3,3,3,3,3,3,3,3,3,3,3,3,3,4),(-161.17256309962,-161.093277609603,
-161.013852914826,-160.93421691605,-160.85446750119,-160.774546868961,-160.743689296198,
-160.665323622154,-160.587054452714,-160.508876506316,-160.430815734123,
-160.352826671867,-160.27492681887,-160.244485292172,-160.166574704059,
-160.088594307158,-160.010538977298,-159.932354261544,-159.854098881938,
-159.775724191303,-159.745281288147,-159.67072219162,-159.596238542007,
-159.521816478903,-159.447442182465,-159.373101864674,-159.298781760927,
-159.224452891769,-159.150114658578,-159.075754600227,-159.001360246425,
-158.926879892853,-158.852350139852,-158.777718409009,-158.746873280096,
-158.672953493819,-158.599120518462,-158.525359892834,-158.451657209306,
-158.377998102671,-158.304368239841,-158.230741164164,-158.157111935124,
-158.083467597361,-158.009795188901,-157.936042861464,-157.862245710629,
-157.78834768398,-157.748465272045,-157.673904210517,-157.599423982859,
-157.525010675825,-157.450650420387,-157.376329382756,-157.302033755808,
-157.227737020108,-157.153435690567,-157.079117277243,-157.004769283516,
-156.930342167363,-156.85586966057,-156.78130083511,-156.750057263994,-156.67549627786,
-156.601016113474,-156.526602857631,-156.452242641338,-156.377921630834,
-156.303626019013,-156.229329280504,-156.155027936969,-156.080709498459,
-156.006361468348,-155.931934299084,-155.857461729539,-155.782892827079,
-155.751649255943,-155.678823428956,-155.606079482122,-155.533402341825,
-155.460777006045,-155.388185732948,-155.315611970161,-155.243042231707,
-155.170463035149,-155.097826176621,-155.025159832957,-154.952403540713,
-154.890004205893),.UNSPECIFIED.);
#539=B_SPLINE_CURVE_WITH_KNOTS('',3,(#63552,#63553,#63554,#63555,#63556,
#63557,#63558,#63559,#63560,#63561,#63562,#63563,#63564,#63565,#63566,#63567,
#63568,#63569,#63570,#63571,#63572,#63573,#63574,#63575,#63576,#63577,#63578,
#63579,#63580,#63581,#63582,#63583,#63584,#63585,#63586,#63587,#63588,#63589,
#63590,#63591,#63592,#63593,#63594,#63595,#63596,#63597,#63598,#63599,#63600,
#63601,#63602,#63603,#63604,#63605,#63606,#63607,#63608,#63609,#63610,#63611,
#63612,#63613,#63614,#63615,#63616,#63617,#63618,#63619,#63620,#63621,#63622,
#63623,#63624,#63625,#63626,#63627,#63628,#63629,#63630,#63631,#63632,#63633,
#63634,#63635,#63636,#63637,#63638,#63639,#63640,#63641,#63642,#63643,#63644,
#63645,#63646,#63647,#63648,#63649,#63650,#63651,#63652,#63653,#63654,#63655,
#63656,#63657,#63658,#63659,#63660,#63661,#63662,#63663,#63664,#63665,#63666,
#63667,#63668,#63669,#63670,#63671,#63672,#63673,#63674,#63675,#63676,#63677,
#63678,#63679,#63680,#63681,#63682,#63683,#63684,#63685,#63686,#63687,#63688,
#63689,#63690,#63691,#63692,#63693,#63694,#63695,#63696,#63697,#63698,#63699,
#63700,#63701,#63702,#63703,#63704,#63705,#63706,#63707,#63708,#63709,#63710,
#63711,#63712,#63713,#63714,#63715,#63716,#63717,#63718,#63719,#63720,#63721,
#63722,#63723,#63724,#63725,#63726,#63727,#63728,#63729,#63730,#63731,#63732,
#63733,#63734,#63735,#63736,#63737,#63738,#63739,#63740,#63741,#63742,#63743,
#63744,#63745,#63746,#63747,#63748,#63749,#63750,#63751,#63752,#63753,#63754,
#63755,#63756,#63757,#63758,#63759,#63760,#63761,#63762,#63763,#63764,#63765,
#63766,#63767,#63768,#63769,#63770,#63771,#63772,#63773,#63774,#63775,#63776,
#63777,#63778,#63779,#63780,#63781,#63782,#63783,#63784,#63785,#63786,#63787,
#63788,#63789,#63790,#63791,#63792,#63793,#63794,#63795,#63796,#63797,#63798,
#63799,#63800,#63801,#63802,#63803,#63804,#63805,#63806,#63807,#63808,#63809,
#63810,#63811,#63812,#63813,#63814,#63815,#63816,#63817,#63818,#63819,#63820,
#63821,#63822,#63823,#63824,#63825,#63826,#63827,#63828,#63829,#63830,#63831,
#63832,#63833,#63834,#63835,#63836,#63837,#63838,#63839,#63840,#63841,#63842,
#63843,#63844,#63845,#63846,#63847,#63848,#63849,#63850,#63851,#63852,#63853,
#63854,#63855,#63856,#63857,#63858,#63859,#63860,#63861,#63862,#63863,#63864,
#63865,#63866,#63867,#63868,#63869,#63870,#63871,#63872,#63873,#63874,#63875,
#63876,#63877,#63878,#63879,#63880,#63881,#63882,#63883,#63884,#63885,#63886,
#63887,#63888,#63889,#63890,#63891,#63892,#63893,#63894,#63895,#63896,#63897,
#63898,#63899,#63900,#63901,#63902,#63903,#63904,#63905,#63906,#63907,#63908,
#63909,#63910,#63911,#63912,#63913,#63914,#63915,#63916,#63917,#63918,#63919,
#63920,#63921,#63922,#63923,#63924,#63925,#63926,#63927,#63928,#63929,#63930,
#63931,#63932,#63933,#63934,#63935,#63936,#63937,#63938,#63939,#63940,#63941,
#63942,#63943,#63944,#63945,#63946,#63947,#63948,#63949,#63950,#63951,#63952,
#63953,#63954,#63955,#63956,#63957,#63958,#63959,#63960,#63961,#63962,#63963,
#63964,#63965,#63966,#63967,#63968,#63969,#63970,#63971,#63972,#63973,#63974,
#63975,#63976,#63977,#63978,#63979,#63980,#63981,#63982,#63983,#63984,#63985,
#63986,#63987,#63988,#63989,#63990,#63991,#63992,#63993,#63994,#63995,#63996,
#63997,#63998,#63999,#64000,#64001,#64002,#64003,#64004,#64005,#64006,#64007,
#64008,#64009,#64010,#64011,#64012,#64013,#64014,#64015,#64016,#64017,#64018,
#64019,#64020,#64021,#64022,#64023,#64024,#64025,#64026,#64027,#64028,#64029,
#64030,#64031,#64032,#64033,#64034,#64035,#64036,#64037,#64038,#64039,#64040,
#64041,#64042,#64043,#64044,#64045,#64046,#64047,#64048,#64049,#64050,#64051,
#64052,#64053,#64054,#64055,#64056,#64057,#64058,#64059,#64060,#64061,#64062,
#64063,#64064,#64065,#64066,#64067,#64068,#64069,#64070,#64071,#64072,#64073,
#64074,#64075,#64076,#64077,#64078,#64079,#64080,#64081,#64082,#64083,#64084,
#64085,#64086,#64087,#64088,#64089,#64090,#64091,#64092,#64093,#64094,#64095,
#64096,#64097,#64098,#64099,#64100,#64101,#64102,#64103,#64104,#64105,#64106,
#64107,#64108,#64109,#64110,#64111,#64112,#64113,#64114,#64115),
 .UNSPECIFIED.,.F.,.F.,(4,2,2,2,2,2,2,2,2,2,2,2,2,2,2,2,2,2,2,2,2,2,2,2,
2,2,2,2,2,2,2,2,2,2,2,2,2,2,2,2,2,2,2,2,2,2,2,2,2,2,2,2,2,2,2,2,2,2,2,2,
2,2,2,2,2,2,2,2,2,2,2,2,2,2,2,2,2,2,2,2,2,2,2,2,2,2,2,2,2,2,2,2,2,2,2,2,
2,2,2,2,2,2,2,2,2,2,2,2,2,2,2,2,2,2,2,2,2,2,2,2,2,2,2,2,2,2,2,2,2,2,2,2,
2,2,2,2,2,2,2,2,2,2,2,2,2,2,2,2,2,2,2,2,2,2,2,2,2,2,2,2,2,2,2,2,2,2,2,2,
2,2,2,2,2,2,2,2,2,2,2,2,2,2,2,2,2,2,2,2,2,2,2,2,2,2,2,2,2,2,2,2,2,2,2,2,
2,2,2,2,2,2,2,2,2,2,2,2,2,2,2,2,2,2,2,2,2,2,2,2,2,2,2,2,2,2,2,2,2,2,2,2,
2,2,2,2,2,2,2,2,2,2,2,2,2,2,2,2,2,2,2,2,2,2,2,2,2,2,2,2,2,2,2,2,2,2,2,2,
2,2,2,2,2,4),(0.00136600686276613,0.0861468345095725,0.103286173672408,
0.105373964908813,0.106676925466201,0.107657746315892,0.10865265629107,
0.109575320646033,0.110845213942466,0.114060655613495,0.151757518273064,
0.156809171672282,0.163055226769575,0.209266853378583,0.216547421283818,
0.432110891827582,0.512367810499585,0.517965862907182,0.520424619489773,
0.522235952003031,0.523909266231999,0.526180307013929,0.531770917615309,
0.589125755379268,0.697272092775012,0.82379549412045,0.864509470399254,
0.887701450714803,0.903999804991615,0.913749035427492,0.91625083056306,
0.917488942525277,0.918776243759128,0.920266188472274,0.922781350083865,
0.931760480025448,0.950370262315602,0.977948905461798,1.09450731135067,
1.10865866835453,1.12530295012558,1.14542820669018,1.17093726968923,1.2067966486548,
1.268978719982,1.28607505907945,1.29110145481201,1.29420613596962,1.29702861093301,
1.300629237588,1.30772314675413,1.34982398311746,1.53276313042715,1.61743233918193,
1.65068686328156,1.66122248493384,1.66574779953149,1.66818418622269,1.67027716421508,
1.6716453578029,1.67296107897272,1.67469173577668,1.67853615939151,1.71539429179514,
1.87224544842473,1.88058948601965,1.88963349541841,1.9113939115549,1.94260291976575,
2.00028853939063,2.05344262619743,2.06295045486912,2.06598427246075,2.0679144650741,
2.06971209646244,2.07204673543636,2.07593065931185,2.08456506657105,2.23864592516649,
2.32393838946969,2.40584696597568,2.47014098353738,2.47804323091178,2.47996444983278,
2.48089876871747,2.48178029957768,2.4827367827063,2.48441175993337,2.48921637258699,
2.56439651998784,2.74276847862193,2.83798814175757,2.87030720078494,2.87470299444743,
2.87691920665452,2.87851777973851,2.8802141521766,2.88308957390748,2.89077852321149,
3.00413339824161,3.07121444470293,3.16757410578299,3.2664649406515,3.26966174368101,
3.27210303007129,3.27336282293146,3.27428072352468,3.27524370852951,3.27658366359109,
3.2793068765687,3.30459764013293,3.34171191024698,3.56054341550202,3.65391684390414,
3.6673888278488,3.67089919276305,3.67297548701912,3.67480965277939,3.67709773266258,
3.68062587118442,3.69656613203174,3.94930892915765,4.03379691011564,4.05837980696131,
4.0611045654401,4.0624323682412,4.06337269692271,4.0643627973657,4.06575277651548,
4.06941810537744,4.12253580750349,4.35079256456728,4.4160289390183,4.44478297554158,
4.44918576238912,4.45145585467486,4.45327174637383,4.45535456201974,4.45889405834353,
4.46829170226635,4.61060278415822,4.76385048314198,4.81110072473817,4.84329713795082,
4.84882505055077,4.85056282480903,4.85166170424352,4.85268035020252,4.85399642861372,
4.85687798331519,4.87969858920732,4.9782208780694,5.2253300020657,5.24147362636173,
5.24492979600868,5.24714924526974,5.24891404704051,5.25089656967671,5.25421199118372,
5.26652271472088,5.347607468908,5.40227272981092,5.61630040225658,5.6398141836146,
5.64242164436536,5.64371186013077,5.64464245064138,5.64553268844385,5.64680013967281,
5.649456495844,5.67736949713039,5.73311576741655,5.77719678197101,6.03416471666612,
6.03749772886747,6.05181438378162,6.05513986073624,6.05732793140271,6.05910290403764,
6.0611350882833,6.06462731658767,6.07872639889206,6.25263287093517,6.43756495177981,
6.44972603413614,6.45229119825805,6.45393125526195,6.45522988086817,6.45668295962764,
6.459099442793,6.46792626434181,6.52881805723823,6.607811574523,6.77817220742128,
6.81898443050167,6.82595628968731,6.82920689186231,6.83200340772601,6.83500520561845,
6.83956938870991,6.85279883187459,7.04839531567641,7.15554940331971,7.20119473475273,
7.20532738852862,7.20699329486049,7.20821603078815,7.2095351301934,7.21131821437206,
7.21534582194712,7.2831612644692,7.36460895089989,7.55297555133023,7.59571865231594,
7.60045529364844,7.60280104683527,7.60449361501895,7.60620028825252,7.60848436925048,
7.6132110686816,7.61934024256664,7.63338613307489,7.6748716473014,7.77036760075454,
8.00020123064167,8.01392019750202,8.01634178781049,8.01757885037082,8.01855673477646,
8.01965861477876,8.02150931633003,8.02846286996565,8.07631794101876,8.15053235444009,
8.24299298516318,8.29952484148184,8.40341962736315,8.41003791124797,8.41246743126957,
8.41417406971254,8.41591089235737,8.41812808918061,8.42054789967341,8.42447576776836,
8.43221557099516,8.45146875308431,8.48481393795657,8.54030331559143,8.66540516577765,
8.79846844145902,8.80693154051052,8.80881956019495,8.81005731332172,8.81096378510183,
8.8120866951413,8.81393167806943,8.82043554155496,8.86226390722535,8.90536531506369,
9.01765357074381,9.0790168544491,9.19688483061321,9.20480501830483,9.20778382824276,
9.20954605287822,9.21135780171077,9.21369986517822,9.2162665220373,9.22047080346694,
9.22884233802831,9.24995825136854,9.34904089158242,9.58222851194488,9.59500949045565,
9.59725584660048,9.59860821774252,9.59965147456159,9.60078465069335,9.60260328298588,
9.60861575143648,9.64504819585966,9.9560577309929),.UNSPECIFIED.);
#540=B_SPLINE_CURVE_WITH_KNOTS('',3,(#64117,#64118,#64119,#64120,#64121,
#64122,#64123,#64124,#64125,#64126,#64127),.UNSPECIFIED.,.F.,.F.,(4,1,1,
1,1,1,1,1,4),(-142.322804428922,-141.77393714323,-140.775529135179,-139.777121127128,
-139.277917123103,-138.778713119077,-137.780305111027,-136.781897102976,
-136.039821870902),.UNSPECIFIED.);
#541=B_SPLINE_CURVE_WITH_KNOTS('',3,(#64129,#64130,#64131,#64132,#64133,
#64134,#64135,#64136,#64137,#64138,#64139,#64140,#64141,#64142,#64143,#64144,
#64145,#64146,#64147,#64148,#64149,#64150,#64151,#64152,#64153,#64154,#64155,
#64156,#64157,#64158,#64159,#64160,#64161,#64162,#64163,#64164,#64165,#64166,
#64167,#64168,#64169,#64170,#64171,#64172,#64173,#64174,#64175,#64176,#64177,
#64178,#64179,#64180,#64181,#64182,#64183,#64184,#64185,#64186,#64187,#64188,
#64189,#64190,#64191,#64192,#64193,#64194,#64195,#64196,#64197,#64198,#64199,
#64200,#64201,#64202,#64203,#64204,#64205,#64206,#64207,#64208,#64209,#64210,
#64211,#64212,#64213,#64214,#64215,#64216,#64217,#64218,#64219,#64220,#64221,
#64222,#64223,#64224,#64225,#64226,#64227,#64228,#64229,#64230,#64231,#64232,
#64233,#64234,#64235,#64236,#64237,#64238,#64239,#64240,#64241,#64242,#64243,
#64244,#64245,#64246,#64247,#64248,#64249,#64250,#64251,#64252,#64253,#64254,
#64255,#64256,#64257,#64258,#64259,#64260,#64261,#64262,#64263,#64264,#64265,
#64266,#64267,#64268,#64269,#64270,#64271,#64272,#64273,#64274,#64275,#64276,
#64277,#64278,#64279,#64280,#64281,#64282,#64283,#64284,#64285,#64286,#64287,
#64288,#64289,#64290,#64291,#64292,#64293,#64294,#64295,#64296,#64297,#64298,
#64299,#64300,#64301,#64302,#64303,#64304,#64305,#64306,#64307,#64308,#64309,
#64310,#64311,#64312,#64313,#64314,#64315,#64316,#64317,#64318,#64319,#64320,
#64321,#64322,#64323,#64324,#64325,#64326,#64327,#64328,#64329,#64330,#64331,
#64332,#64333,#64334,#64335,#64336,#64337,#64338,#64339,#64340,#64341,#64342,
#64343,#64344,#64345,#64346,#64347,#64348,#64349,#64350,#64351,#64352,#64353,
#64354,#64355,#64356,#64357,#64358,#64359,#64360,#64361,#64362,#64363,#64364,
#64365,#64366,#64367,#64368,#64369,#64370,#64371,#64372,#64373,#64374,#64375,
#64376,#64377,#64378,#64379,#64380,#64381,#64382,#64383,#64384,#64385,#64386,
#64387,#64388,#64389,#64390,#64391,#64392,#64393),.UNSPECIFIED.,.F.,.F.,
(4,3,3,3,3,3,3,3,3,3,3,3,3,3,3,3,3,3,3,3,3,3,3,3,3,3,3,3,3,3,3,3,3,3,3,
3,3,3,3,3,3,3,3,3,3,3,3,3,3,3,3,3,3,3,3,3,3,3,3,3,3,3,3,3,3,3,3,3,3,3,3,
3,3,3,3,3,3,3,3,3,3,3,3,3,3,3,3,3,4),(-136.039821779079,-135.94619225248,
-135.850900439115,-135.783489094925,-135.70892810879,-135.634447944404,
-135.560034688561,-135.485674472268,-135.411353461763,-135.337057849942,
-135.262761111433,-135.188459767897,-135.114141329388,-135.039793299276,
-134.965366130011,-134.890893560466,-134.816324658006,-134.785081086874,
-134.71118760562,-134.637376739478,-134.563634044055,-134.48994512516,-134.416295627933,
-134.342671226749,-134.269043379823,-134.195409513755,-134.12175667154,
-134.048071887332,-133.974301334434,-133.900482623819,-133.826557972951,
-133.786673078823,-133.712050013409,-133.637512684528,-133.563047195775,
-133.488639698134,-133.414276380892,-133.339943462991,-133.265617000396,
-133.191290668441,-133.116952009644,-133.042588562366,-132.968153305183,
-132.893676831792,-132.819110459651,-132.788265070772,-132.709899396731,
-132.631630227293,-132.553452280897,-132.475391508706,-132.397402446453,
-132.319502593457,-132.289061066747,-132.211150478633,-132.133170081729,
-132.055114751869,-131.976930036113,-131.898674656506,-131.820299965869,
-131.789857062721,-131.715297966194,-131.640814316582,-131.566392253477,
-131.49201795704,-131.417677639249,-131.343357535502,-131.269028666344,
-131.194690433153,-131.120330374802,-131.045936021,-130.971455667428,-130.896925914427,
-130.822294183585,-130.79144905467,-130.717529268393,-130.643696293037,
-130.569935667409,-130.496232983881,-130.422573877246,-130.348944014416,
-130.275316938739,-130.2016877097,-130.128043371937,-130.054370963477,-129.98061863604,
-129.906821485206,-129.832923458557,-129.793041046619,-129.756636563722),
 .UNSPECIFIED.);
#542=B_SPLINE_CURVE_WITH_KNOTS('',3,(#64395,#64396,#64397,#64398,#64399,
#64400,#64401,#64402,#64403,#64404,#64405),.UNSPECIFIED.,.F.,.F.,(4,1,1,
1,1,1,1,1,4),(-129.75663160721,-128.794633038568,-127.796225030517,-126.797817022466,
-125.799409014416,-125.30020501039,-124.801001006365,-123.802592998314,
-123.473451256543),.UNSPECIFIED.);
#543=B_SPLINE_CURVE_WITH_KNOTS('',3,(#64407,#64408,#64409,#64410,#64411,
#64412,#64413,#64414,#64415,#64416,#64417,#64418,#64419,#64420,#64421,#64422,
#64423,#64424),.UNSPECIFIED.,.F.,.F.,(4,2,2,2,2,2,2,2,4),(-123.473451256543,
-122.638534344648,-121.803617432753,-120.968700520858,-120.133783608963,
-119.298866697069,-118.463949785174,-117.629032873279,-117.190265949363),
 .UNSPECIFIED.);
#544=B_SPLINE_CURVE_WITH_KNOTS('',3,(#64426,#64427,#64428,#64429,#64430,
#64431,#64432,#64433,#64434,#64435,#64436,#64437,#64438,#64439,#64440,#64441,
#64442,#64443,#64444,#64445,#64446,#64447,#64448,#64449,#64450,#64451,#64452,
#64453,#64454,#64455,#64456,#64457,#64458,#64459,#64460,#64461,#64462,#64463,
#64464,#64465,#64466,#64467,#64468,#64469,#64470,#64471,#64472,#64473,#64474,
#64475,#64476,#64477,#64478,#64479,#64480,#64481,#64482,#64483,#64484,#64485,
#64486,#64487,#64488,#64489,#64490,#64491,#64492,#64493,#64494,#64495,#64496,
#64497,#64498,#64499,#64500,#64501,#64502,#64503,#64504,#64505,#64506,#64507,
#64508,#64509,#64510,#64511,#64512,#64513,#64514,#64515,#64516,#64517,#64518,
#64519,#64520,#64521,#64522,#64523,#64524,#64525,#64526,#64527,#64528,#64529,
#64530,#64531,#64532,#64533,#64534,#64535,#64536,#64537,#64538,#64539,#64540,
#64541,#64542,#64543,#64544,#64545,#64546,#64547,#64548,#64549,#64550,#64551,
#64552,#64553,#64554,#64555,#64556,#64557,#64558,#64559,#64560,#64561,#64562,
#64563,#64564,#64565,#64566,#64567,#64568,#64569,#64570,#64571,#64572,#64573,
#64574,#64575,#64576,#64577,#64578,#64579,#64580,#64581,#64582,#64583,#64584,
#64585,#64586,#64587,#64588,#64589,#64590,#64591,#64592,#64593,#64594,#64595,
#64596,#64597,#64598,#64599,#64600,#64601,#64602,#64603,#64604,#64605,#64606,
#64607,#64608,#64609,#64610,#64611,#64612,#64613,#64614,#64615,#64616,#64617,
#64618,#64619,#64620,#64621,#64622,#64623,#64624,#64625,#64626,#64627,#64628,
#64629,#64630,#64631,#64632,#64633,#64634,#64635,#64636,#64637,#64638,#64639,
#64640,#64641,#64642,#64643,#64644,#64645,#64646,#64647,#64648,#64649,#64650,
#64651,#64652,#64653,#64654,#64655,#64656,#64657,#64658,#64659,#64660,#64661,
#64662,#64663,#64664,#64665,#64666,#64667,#64668,#64669,#64670,#64671,#64672,
#64673,#64674,#64675,#64676,#64677,#64678,#64679,#64680,#64681,#64682,#64683,
#64684,#64685,#64686,#64687,#64688,#64689,#64690),.UNSPECIFIED.,.F.,.F.,
(4,3,3,3,3,3,3,3,3,3,3,3,3,3,3,3,3,3,3,3,3,3,3,3,3,3,3,3,3,3,3,3,3,3,3,
3,3,3,3,3,3,3,3,3,3,3,3,3,3,3,3,3,3,3,3,3,3,3,3,3,3,3,3,3,3,3,3,3,3,3,3,
3,3,3,3,3,3,3,3,3,3,3,3,3,3,3,3,3,4),(-117.190265949363,-117.105316619372,
-117.019674410368,-116.933688950344,-116.84729407057,-116.813736941957,
-116.73981715568,-116.665984180324,-116.592223554695,-116.518520871167,
-116.444861764532,-116.371231901702,-116.297604826025,-116.223975596986,
-116.150331259222,-116.076658850763,-116.002906523325,-115.929109372491,
-115.855211345842,-115.815328933906,-115.740767872377,-115.66628764472,
-115.591874337686,-115.517514082247,-115.443193044616,-115.368897417668,
-115.294600681968,-115.220299352427,-115.145980939102,-115.071632945376,
-114.997205829222,-114.922733322429,-114.84816449697,-114.816920925855,
-114.742359939721,-114.667879775335,-114.593466519493,-114.5191063032,-114.444785292696,
-114.370489680875,-114.296192942367,-114.221891598831,-114.147573160322,
-114.073225130211,-113.998797960947,-113.924325391403,-113.849756488943,
-113.818512917805,-113.744619436551,-113.670808570409,-113.597065874986,
-113.523376956091,-113.449727458864,-113.37610305768,-113.302475210754,
-113.228841344686,-113.155188502471,-113.081503718263,-113.007733165365,
-112.93391445475,-112.859989803883,-112.820104909754,-112.74548184434,-112.670944515459,
-112.596479026706,-112.522071529065,-112.447708211822,-112.373375293921,
-112.299048831326,-112.224722499371,-112.150383840575,-112.076020393296,
-112.001585136114,-111.927108662723,-111.852542290581,-111.821696901703,
-111.743331227661,-111.665062058222,-111.586884111824,-111.508823339632,
-111.430834277378,-111.352934424382,-111.322492897677,-111.247393740118,
-111.172260130373,-111.097041135258,-111.021774372652,-110.946406268164,
-110.907282228194),.UNSPECIFIED.);
#545=B_SPLINE_CURVE_WITH_KNOTS('',3,(#64692,#64693,#64694,#64695,#64696,
#64697,#64698,#64699,#64700,#64701,#64702,#64703,#64704,#64705,#64706,#64707,
#64708,#64709),.UNSPECIFIED.,.F.,.F.,(4,2,2,2,2,2,2,2,4),(-110.907004517659,
-110.072163730289,-109.237246818394,-108.402329906499,-107.567412994604,
-106.732496082709,-105.897579170815,-105.06266225892,-104.623985027996),
 .UNSPECIFIED.);
#546=B_SPLINE_CURVE_WITH_KNOTS('',3,(#64711,#64712,#64713,#64714,#64715,
#64716,#64717,#64718,#64719,#64720,#64721,#64722,#64723,#64724,#64725,#64726,
#64727,#64728,#64729,#64730,#64731,#64732,#64733,#64734,#64735,#64736,#64737,
#64738,#64739,#64740,#64741,#64742,#64743,#64744,#64745,#64746,#64747,#64748,
#64749,#64750,#64751,#64752,#64753,#64754,#64755,#64756,#64757,#64758,#64759,
#64760,#64761,#64762,#64763,#64764,#64765,#64766,#64767,#64768,#64769,#64770,
#64771,#64772,#64773,#64774,#64775,#64776,#64777,#64778,#64779,#64780,#64781,
#64782,#64783,#64784,#64785,#64786,#64787,#64788,#64789,#64790,#64791,#64792,
#64793,#64794,#64795,#64796,#64797,#64798,#64799,#64800,#64801,#64802,#64803,
#64804,#64805,#64806,#64807,#64808,#64809,#64810,#64811,#64812,#64813,#64814,
#64815,#64816,#64817,#64818,#64819,#64820,#64821,#64822,#64823,#64824,#64825,
#64826,#64827,#64828,#64829,#64830,#64831,#64832,#64833,#64834,#64835,#64836,
#64837,#64838,#64839,#64840,#64841,#64842,#64843,#64844,#64845,#64846,#64847,
#64848,#64849,#64850,#64851,#64852,#64853,#64854,#64855,#64856,#64857,#64858,
#64859,#64860,#64861,#64862,#64863,#64864,#64865,#64866,#64867,#64868,#64869,
#64870,#64871,#64872,#64873,#64874,#64875,#64876,#64877,#64878,#64879,#64880,
#64881,#64882,#64883,#64884,#64885,#64886,#64887,#64888,#64889,#64890,#64891,
#64892,#64893,#64894,#64895,#64896,#64897,#64898,#64899,#64900,#64901,#64902,
#64903,#64904,#64905,#64906,#64907,#64908,#64909,#64910,#64911,#64912,#64913,
#64914,#64915,#64916,#64917,#64918,#64919,#64920,#64921,#64922,#64923,#64924,
#64925,#64926,#64927,#64928,#64929,#64930,#64931,#64932,#64933,#64934,#64935,
#64936,#64937,#64938,#64939,#64940,#64941,#64942,#64943,#64944,#64945,#64946,
#64947,#64948,#64949,#64950,#64951,#64952,#64953,#64954,#64955,#64956,#64957,
#64958,#64959,#64960,#64961,#64962,#64963,#64964,#64965,#64966,#64967,#64968,
#64969,#64970,#64971,#64972,#64973,#64974,#64975),.UNSPECIFIED.,.F.,.F.,
(4,3,3,3,3,3,3,3,3,3,3,3,3,3,3,3,3,3,3,3,3,3,3,3,3,3,3,3,3,3,3,3,3,3,3,
3,3,3,3,3,3,3,3,3,3,3,3,3,3,3,3,3,3,3,3,3,3,3,3,3,3,3,3,3,3,3,3,3,3,3,3,
3,3,3,3,3,3,3,3,3,3,3,3,3,3,3,3,3,4),(-104.623358907686,-104.550797753273,
-104.47828304321,-104.405799590655,-104.333636841321,-104.255726253206,
-104.177745856302,-104.09969052644,-104.021505810683,-103.943250431075,
-103.864875740437,-103.834432837295,-103.759873740768,-103.685390091156,
-103.610968028051,-103.536593731613,-103.462253413823,-103.387933310076,
-103.313604440918,-103.239266207727,-103.164906149377,-103.090511795574,
-103.016031442002,-102.941501689001,-102.866869958159,-102.836024829244,
-102.762105042967,-102.688272067611,-102.614511441983,-102.540808758455,
-102.467149651821,-102.393519788992,-102.319892713315,-102.246263484276,
-102.172619146513,-102.098946738052,-102.025194410616,-101.951397259782,
-101.877499233133,-101.837616821194,-101.763055759665,-101.688575532008,
-101.614162224974,-101.539801969536,-101.465480931905,-101.391185304956,
-101.316888569256,-101.242587239716,-101.168268826391,-101.093920832665,
-101.019493716511,-100.945021209718,-100.870452384259,-100.839208813143,
-100.764647827009,-100.690167662623,-100.61575440678,-100.541394190487,
-100.467073179983,-100.392777568161,-100.318480829653,-100.244179486117,
-100.169861047607,-100.095513017496,-100.021085848232,-99.9466132786866,
-99.8720443762267,-99.8408008050917,-99.7669073238381,-99.6930964576958,
-99.619353762273,-99.5456648433779,-99.4720153461518,-99.3983909449678,
-99.3247630980424,-99.2511292319739,-99.177476389759,-99.1037916055511,
-99.0300210526534,-98.9562023420383,-98.8822776911711,-98.8423927970408,
-98.7629300258068,-98.683602234694,-98.604407958319,-98.5254009471871,-98.4465090550021,
-98.3677746029374,-98.3407100278245),.UNSPECIFIED.);
#547=B_SPLINE_CURVE_WITH_KNOTS('',3,(#64977,#64978,#64979,#64980,#64981,
#64982,#64983,#64984,#64985,#64986,#64987,#64988,#64989,#64990,#64991,#64992,
#64993,#64994,#64995,#64996,#64997,#64998,#64999,#65000,#65001,#65002,#65003,
#65004,#65005,#65006,#65007,#65008,#65009,#65010,#65011,#65012,#65013,#65014,
#65015,#65016,#65017,#65018,#65019,#65020,#65021,#65022,#65023,#65024,#65025,
#65026,#65027,#65028,#65029,#65030,#65031,#65032,#65033,#65034,#65035,#65036,
#65037,#65038,#65039,#65040,#65041,#65042,#65043,#65044,#65045,#65046,#65047,
#65048,#65049,#65050,#65051,#65052,#65053,#65054,#65055,#65056,#65057,#65058,
#65059,#65060,#65061,#65062,#65063,#65064,#65065,#65066,#65067,#65068,#65069,
#65070,#65071,#65072,#65073,#65074,#65075,#65076,#65077,#65078,#65079,#65080,
#65081,#65082,#65083,#65084,#65085,#65086,#65087,#65088,#65089,#65090,#65091,
#65092,#65093,#65094,#65095,#65096,#65097,#65098,#65099,#65100,#65101,#65102,
#65103,#65104,#65105,#65106,#65107,#65108,#65109,#65110,#65111,#65112,#65113,
#65114,#65115,#65116,#65117,#65118,#65119,#65120,#65121,#65122,#65123,#65124,
#65125,#65126,#65127,#65128,#65129,#65130,#65131,#65132,#65133,#65134,#65135,
#65136,#65137,#65138,#65139,#65140,#65141,#65142,#65143,#65144,#65145,#65146,
#65147,#65148,#65149,#65150,#65151,#65152,#65153,#65154,#65155,#65156,#65157,
#65158,#65159,#65160,#65161,#65162,#65163,#65164,#65165,#65166,#65167,#65168,
#65169,#65170,#65171,#65172,#65173,#65174,#65175,#65176,#65177,#65178,#65179,
#65180,#65181,#65182,#65183,#65184,#65185,#65186,#65187,#65188,#65189,#65190,
#65191,#65192,#65193,#65194,#65195,#65196,#65197,#65198,#65199,#65200,#65201,
#65202,#65203,#65204,#65205,#65206,#65207,#65208,#65209,#65210,#65211,#65212,
#65213,#65214,#65215,#65216,#65217),.UNSPECIFIED.,.F.,.F.,(4,3,3,3,3,3,
3,3,3,3,3,3,3,3,3,3,3,3,3,3,3,3,3,3,3,3,3,3,3,3,3,3,3,3,3,3,3,3,3,3,3,3,
3,3,3,3,3,3,3,3,3,3,3,3,3,3,3,3,3,3,3,3,3,3,3,3,3,3,3,3,3,3,3,3,3,3,3,3,
3,3,4),(-98.3407100278245,-98.3398751109126,-98.2497923383696,-98.1594093744117,
-98.0690731139765,-97.9789567735724,-97.8891402262143,-97.8442804143033,
-97.7552175859449,-97.6724974832672,-97.6057318876503,-97.5390372049508,
-97.5057931159296,-97.3913563601377,-97.3450651360715,-97.2298028424745,
-97.1144050455794,-96.9994261646693,-96.8854619929382,-96.8461239064708,
-96.7342773273762,-96.6708762040348,-96.5912548848605,-96.5107793206893,
-96.4292551225898,-96.3799354774799,-96.2761438716762,-96.1689624435349,
-96.0652171864929,-95.9629223065681,-95.8638736849662,-95.847418159111,
-95.8359592921399,-95.7438149252361,-95.6479844699747,-95.5510733494601,
-95.4537908365631,-95.4185008361925,-95.3295095279158,-95.2413177536157,
-95.1543001375577,-95.0695592780133,-95.001042380245,-94.8989066470248,
-94.8483475199855,-94.7446888282949,-94.6404310244062,-94.5356081345725,
-94.43092383478,-94.3272430696066,-94.2541340789527,-94.1932522994489,-94.1661254683501,
-94.0819039095132,-93.9980018643696,-93.9148482355806,-93.8504898373246,
-93.7668082244376,-93.682989170877,-93.59965070049,-93.5842440152402,-93.5121655571065,
-93.4395403317008,-93.3663365921562,-93.3312085564552,-93.2476744079394,
-93.1640127763708,-93.0804884793871,-92.9971666819597,-92.9140745743315,
-92.8524988242307,-92.7672692310056,-92.6820396377804,-92.6021855545101,
-92.5207460562211,-92.4962916445604,-92.4066331146904,-92.3166043445123,
-92.2274393260093,-92.1407699558148,-92.0575247206449),.UNSPECIFIED.);
#548=B_SPLINE_CURVE_WITH_KNOTS('',3,(#65219,#65220,#65221,#65222,#65223,
#65224,#65225,#65226,#65227,#65228,#65229,#65230,#65231,#65232,#65233,#65234,
#65235,#65236),.UNSPECIFIED.,.F.,.F.,(4,2,2,2,2,2,2,2,4),(-92.0575247206449,
-91.2226078087501,-90.3876908968552,-89.5527739849604,-88.7178570730655,
-87.8829401611707,-87.0480232492758,-86.213106337381,-85.774546795447),
 .UNSPECIFIED.);
#549=B_SPLINE_CURVE_WITH_KNOTS('',3,(#65238,#65239,#65240,#65241,#65242,
#65243,#65244,#65245,#65246,#65247,#65248),.UNSPECIFIED.,.F.,.F.,(4,1,1,
1,1,1,1,1,4),(-85.7739081130952,-84.864680684328,-83.866272676277,-83.3670686722516,
-82.8678646682261,-81.8694566601752,-80.8710486521243,-79.8726406440734,
-79.4911610665801),.UNSPECIFIED.);
#550=B_SPLINE_CURVE_WITH_KNOTS('',3,(#65250,#65251,#65252,#65253,#65254,
#65255,#65256,#65257,#65258,#65259,#65260,#65261,#65262,#65263,#65264,#65265,
#65266,#65267,#65268,#65269,#65270,#65271,#65272,#65273,#65274,#65275,#65276,
#65277,#65278,#65279,#65280,#65281,#65282,#65283,#65284,#65285,#65286,#65287,
#65288,#65289,#65290,#65291,#65292,#65293,#65294,#65295,#65296,#65297,#65298,
#65299,#65300,#65301,#65302,#65303,#65304,#65305,#65306,#65307,#65308,#65309,
#65310,#65311,#65312,#65313,#65314,#65315,#65316,#65317,#65318,#65319,#65320,
#65321,#65322,#65323,#65324,#65325,#65326,#65327,#65328,#65329,#65330,#65331,
#65332,#65333,#65334,#65335,#65336,#65337,#65338,#65339,#65340,#65341,#65342,
#65343,#65344,#65345,#65346,#65347,#65348,#65349,#65350,#65351,#65352,#65353,
#65354,#65355,#65356,#65357,#65358,#65359,#65360,#65361,#65362,#65363,#65364,
#65365,#65366,#65367,#65368,#65369,#65370,#65371,#65372,#65373,#65374,#65375,
#65376,#65377,#65378,#65379,#65380,#65381,#65382,#65383,#65384,#65385,#65386,
#65387,#65388,#65389,#65390,#65391,#65392,#65393,#65394,#65395,#65396,#65397,
#65398,#65399,#65400,#65401,#65402,#65403,#65404,#65405,#65406,#65407,#65408,
#65409,#65410,#65411,#65412,#65413,#65414,#65415,#65416,#65417,#65418,#65419,
#65420,#65421,#65422,#65423,#65424,#65425,#65426,#65427,#65428,#65429,#65430,
#65431,#65432,#65433,#65434,#65435,#65436,#65437,#65438,#65439,#65440,#65441,
#65442,#65443,#65444,#65445,#65446,#65447,#65448,#65449,#65450,#65451,#65452,
#65453,#65454,#65455,#65456,#65457,#65458,#65459,#65460,#65461,#65462,#65463,
#65464,#65465,#65466,#65467,#65468,#65469,#65470,#65471,#65472,#65473,#65474,
#65475,#65476,#65477,#65478,#65479,#65480,#65481,#65482,#65483,#65484,#65485,
#65486,#65487,#65488,#65489,#65490,#65491,#65492,#65493,#65494,#65495,#65496,
#65497,#65498,#65499,#65500,#65501,#65502,#65503,#65504,#65505,#65506,#65507,
#65508,#65509,#65510,#65511,#65512,#65513,#65514),.UNSPECIFIED.,.F.,.F.,
(4,3,3,3,3,3,3,3,3,3,3,3,3,3,3,3,3,3,3,3,3,3,3,3,3,3,3,3,3,3,3,3,3,3,3,
3,3,3,3,3,3,3,3,3,3,3,3,3,3,3,3,3,3,3,3,3,3,3,3,3,3,3,3,3,3,3,3,3,3,3,3,
3,3,3,3,3,3,3,3,3,3,3,3,3,3,3,3,3,4),(-79.4911541062857,-79.4140389225028,
-79.3388515225128,-79.2636409863518,-79.1883959109838,-79.1098550922435,
-79.0344649991889,-78.9590167596919,-78.8834664025531,-78.8742326360225,
-78.8003391547687,-78.7265282886263,-78.652785593203,-78.5790966743082,
-78.5054471770817,-78.4318227758969,-78.3581949289715,-78.2845610629028,
-78.210908220688,-78.13722343648,-78.0634528835819,-77.9896341729666,-77.9157095220992,
-77.8758246279715,-77.8012015625577,-77.7266642336767,-77.6521987449237,
-77.5777912472822,-77.5034279300403,-77.4290950121387,-77.354768549544,
-77.2804422175887,-77.2061035587924,-77.1317401115139,-77.0573048543314,
-76.9828283809401,-76.9082620087988,-76.8774166199206,-76.7990509458789,
-76.7207817764409,-76.6426038300442,-76.564543057853,-76.4865539955989,
-76.4086541426038,-76.3782126158952,-76.3003020277817,-76.2223216308785,
-76.1442663010181,-76.0660815852632,-75.9878262056562,-75.9094515150197,
-75.8790086118697,-75.8044495153425,-75.7299658657305,-75.6555438026262,
-75.5811695061888,-75.5068291883977,-75.4325090846501,-75.3581802154919,
-75.2838419823009,-75.2094819239501,-75.1350875701474,-75.0606072165753,
-74.9860774635745,-74.9114457327325,-74.8806006038188,-74.8066808175414,
-74.7328478421853,-74.6590872165573,-74.5853845330293,-74.5117254263945,
-74.4380955635651,-74.3644684878882,-74.2908392588486,-74.2171949210857,
-74.1435225126251,-74.0697701851881,-73.9959730343537,-73.9220750077044,
-73.8821925957679,-73.8075920945069,-73.7326391825818,-73.6582186814261,
-73.5838517352182,-73.5095258513851,-73.4341365883154,-73.3598492930203,
-73.2839090460632,-73.2079687991061),.UNSPECIFIED.);
#551=B_SPLINE_CURVE_WITH_KNOTS('',3,(#65516,#65517,#65518,#65519,#65520,
#65521,#65522,#65523,#65524,#65525,#65526),.UNSPECIFIED.,.F.,.F.,(4,1,1,
1,1,1,1,1,4),(-73.2079618312794,-72.8837845877169,-71.885376579666,-70.8869685716151,
-69.8885605635642,-69.3893565595387,-68.8901525555133,-67.8917445474624,
-66.9249979083913),.UNSPECIFIED.);
#552=B_SPLINE_CURVE_WITH_KNOTS('',3,(#65528,#65529,#65530,#65531,#65532,
#65533,#65534,#65535,#65536,#65537,#65538,#65539,#65540,#65541,#65542,#65543,
#65544,#65545),.UNSPECIFIED.,.F.,.F.,(4,2,2,2,2,2,2,2,4),(-66.9246686944173,
-66.0898665800317,-65.2549496681368,-64.420032756242,-63.5851158443471,
-62.7501989324523,-61.9152820205574,-61.0803651086626,-60.641598184747),
 .UNSPECIFIED.);
#553=B_SPLINE_CURVE_WITH_KNOTS('',3,(#65547,#65548,#65549,#65550,#65551,
#65552,#65553,#65554,#65555,#65556,#65557,#65558,#65559,#65560,#65561,#65562,
#65563,#65564),.UNSPECIFIED.,.F.,.F.,(4,2,2,2,2,2,2,2,4),(-60.641598184747,
-59.8066812728521,-58.9717643609573,-58.1368474490624,-57.3019305371676,
-56.4670136252727,-55.6320967133778,-54.797179801483,-54.3584128775674),
 .UNSPECIFIED.);
#554=B_SPLINE_CURVE_WITH_KNOTS('',3,(#65566,#65567,#65568,#65569,#65570,
#65571,#65572,#65573,#65574,#65575,#65576),.UNSPECIFIED.,.F.,.F.,(4,1,1,
1,1,1,1,1,4),(-54.3584128775674,-53.9140324347495,-52.9156244266986,-51.9172164186477,
-50.9188084105968,-49.9204004025459,-48.9219923944949,-48.4227883904695,
-48.0756242030887),.UNSPECIFIED.);
#555=B_SPLINE_CURVE_WITH_KNOTS('',3,(#65578,#65579,#65580,#65581,#65582,
#65583,#65584,#65585,#65586,#65587,#65588,#65589,#65590,#65591,#65592,#65593,
#65594,#65595),.UNSPECIFIED.,.F.,.F.,(4,2,2,2,2,2,2,2,4),(-48.0751022683111,
-47.2403106584929,-46.405393746598,-45.5704768347031,-44.7355599228082,
-43.9006430109134,-43.0657260990185,-42.2308091871236,-41.792165349807),
 .UNSPECIFIED.);
#556=B_SPLINE_CURVE_WITH_KNOTS('',3,(#65597,#65598,#65599,#65600,#65601,
#65602,#65603,#65604,#65605,#65606,#65607),.UNSPECIFIED.,.F.,.F.,(4,1,1,
1,1,1,1,1,4),(-41.7916731482383,-41.4339323341131,-40.9347283300876,-39.9363203220367,
-38.9379123139858,-37.9395043059348,-36.9410962978839,-35.942688289833,
-35.5088569560286),.UNSPECIFIED.);
#557=B_SPLINE_CURVE_WITH_KNOTS('',3,(#65609,#65610,#65611,#65612,#65613,
#65614,#65615,#65616,#65617,#65618,#65619,#65620,#65621,#65622,#65623,#65624,
#65625,#65626,#65627,#65628,#65629,#65630,#65631,#65632,#65633,#65634,#65635,
#65636,#65637,#65638,#65639,#65640,#65641,#65642,#65643,#65644,#65645,#65646,
#65647,#65648,#65649,#65650,#65651,#65652,#65653,#65654,#65655,#65656,#65657,
#65658,#65659,#65660,#65661,#65662,#65663,#65664,#65665,#65666,#65667,#65668,
#65669,#65670,#65671,#65672,#65673,#65674,#65675,#65676,#65677,#65678,#65679,
#65680,#65681,#65682,#65683,#65684,#65685,#65686,#65687,#65688,#65689,#65690,
#65691,#65692,#65693,#65694,#65695,#65696,#65697,#65698,#65699,#65700,#65701,
#65702,#65703,#65704,#65705,#65706,#65707,#65708,#65709,#65710,#65711,#65712,
#65713,#65714,#65715,#65716,#65717,#65718,#65719,#65720,#65721,#65722,#65723,
#65724,#65725,#65726,#65727,#65728,#65729,#65730,#65731,#65732,#65733,#65734,
#65735,#65736,#65737,#65738,#65739,#65740,#65741,#65742,#65743,#65744,#65745,
#65746,#65747,#65748,#65749,#65750,#65751,#65752,#65753,#65754,#65755,#65756,
#65757,#65758,#65759,#65760,#65761,#65762,#65763,#65764,#65765,#65766,#65767,
#65768,#65769,#65770,#65771,#65772,#65773,#65774,#65775,#65776,#65777,#65778,
#65779,#65780,#65781,#65782,#65783,#65784,#65785,#65786,#65787,#65788,#65789,
#65790,#65791,#65792,#65793,#65794,#65795,#65796,#65797,#65798,#65799,#65800,
#65801,#65802,#65803,#65804,#65805,#65806,#65807,#65808,#65809,#65810,#65811,
#65812,#65813,#65814,#65815,#65816,#65817,#65818,#65819,#65820,#65821,#65822,
#65823,#65824,#65825,#65826,#65827,#65828,#65829,#65830,#65831,#65832,#65833,
#65834,#65835,#65836,#65837,#65838,#65839,#65840,#65841,#65842,#65843,#65844,
#65845,#65846),.UNSPECIFIED.,.F.,.F.,(4,3,3,3,3,3,3,3,3,3,3,3,3,3,3,3,3,
3,3,3,3,3,3,3,3,3,3,3,3,3,3,3,3,3,3,3,3,3,3,3,3,3,3,3,3,3,3,3,3,3,3,3,3,
3,3,3,3,3,3,3,3,3,3,3,3,3,3,3,3,3,3,3,3,3,3,3,3,3,3,4),(-35.5088569560286,
-35.5080220391167,-35.4078226390595,-35.3069421369146,-35.2059486885099,
-35.105244626726,-35.0050126956435,-34.9446638723629,-34.8458356537844,
-34.7591101236746,-34.7092184675934,-34.6739400441337,-34.5831464955377,
-34.4908340657363,-34.4450138153475,-34.3507477017669,-34.2564815881863,
-34.1463815848413,-34.0363558288672,-33.9460902199452,-33.8390231322389,
-33.7510601187875,-33.6605691285795,-33.5688148214294,-33.4758388293184,
-33.4215646762915,-33.3042274288324,-33.1904896172914,-33.0844504646164,
-33.004106220344,-32.9476783657108,-32.8536744421173,-32.7592046327776,
-32.6643487376451,-32.5866477643965,-32.4997781842343,-32.4120965402195,
-32.3250698966745,-32.2402926429357,-32.1691893084491,-32.0750415190886,
-31.9820995782183,-31.9488402515311,-31.8561241312604,-31.7622897538461,
-31.6684546500954,-31.5873078553393,-31.5117019803102,-31.4355870580904,
-31.3593882068004,-31.3342723965543,-31.2551135477029,-31.1760459938561,
-31.0971771530997,-31.0185521244204,-30.9509227757793,-30.8721831335571,
-30.7937911100304,-30.7523909434444,-30.6822918968919,-30.6117873185264,
-30.5407351827176,-30.4993554846594,-30.4114258939849,-30.3232470914475,
-30.230635044061,-30.1426420911496,-30.0548682539713,-29.9674611296698,
-29.9527989019017,-29.8663222153201,-29.8142264196547,-29.757682515458,
-29.7011770307223,-29.6644385727646,-29.578284095983,-29.4901309841995,
-29.4022684992888,-29.3139700740689,-29.225671648849),.UNSPECIFIED.);
#558=B_SPLINE_CURVE_WITH_KNOTS('',3,(#65848,#65849,#65850,#65851,#65852,
#65853,#65854,#65855,#65856,#65857,#65858,#65859,#65860,#65861,#65862,#65863,
#65864,#65865,#65866,#65867,#65868,#65869,#65870,#65871,#65872,#65873,#65874,
#65875,#65876,#65877,#65878,#65879,#65880,#65881,#65882,#65883,#65884,#65885,
#65886,#65887,#65888,#65889,#65890,#65891,#65892,#65893,#65894,#65895,#65896,
#65897,#65898,#65899,#65900,#65901,#65902,#65903,#65904,#65905,#65906,#65907,
#65908,#65909,#65910,#65911,#65912,#65913,#65914,#65915,#65916,#65917,#65918,
#65919,#65920,#65921,#65922,#65923,#65924,#65925,#65926,#65927,#65928,#65929,
#65930,#65931,#65932,#65933,#65934,#65935,#65936,#65937,#65938,#65939,#65940,
#65941,#65942,#65943,#65944,#65945,#65946,#65947,#65948,#65949,#65950,#65951,
#65952,#65953,#65954,#65955,#65956,#65957,#65958,#65959,#65960,#65961,#65962,
#65963,#65964,#65965,#65966,#65967,#65968,#65969,#65970,#65971,#65972,#65973,
#65974,#65975,#65976,#65977,#65978,#65979,#65980,#65981,#65982,#65983,#65984,
#65985,#65986,#65987,#65988,#65989,#65990,#65991,#65992,#65993,#65994,#65995,
#65996,#65997,#65998,#65999,#66000,#66001,#66002,#66003,#66004,#66005,#66006,
#66007,#66008,#66009,#66010,#66011,#66012,#66013,#66014,#66015,#66016,#66017,
#66018,#66019,#66020,#66021,#66022,#66023,#66024,#66025,#66026,#66027,#66028,
#66029,#66030,#66031,#66032,#66033,#66034,#66035,#66036,#66037,#66038,#66039,
#66040,#66041,#66042,#66043,#66044,#66045,#66046,#66047,#66048,#66049,#66050,
#66051,#66052,#66053,#66054,#66055,#66056,#66057,#66058,#66059,#66060,#66061,
#66062,#66063,#66064,#66065,#66066,#66067,#66068,#66069,#66070,#66071,#66072,
#66073,#66074,#66075,#66076,#66077,#66078,#66079,#66080,#66081,#66082,#66083,
#66084,#66085,#66086,#66087,#66088,#66089,#66090,#66091,#66092,#66093,#66094,
#66095,#66096,#66097,#66098,#66099,#66100,#66101,#66102,#66103,#66104,#66105,
#66106,#66107,#66108,#66109,#66110,#66111,#66112,#66113,#66114,#66115,#66116,
#66117,#66118,#66119,#66120,#66121,#66122,#66123,#66124,#66125,#66126,#66127,
#66128,#66129,#66130,#66131,#66132,#66133,#66134,#66135,#66136,#66137,#66138,
#66139,#66140,#66141,#66142,#66143,#66144,#66145,#66146,#66147,#66148,#66149,
#66150,#66151,#66152,#66153,#66154,#66155,#66156,#66157,#66158,#66159,#66160,
#66161,#66162,#66163,#66164,#66165,#66166,#66167,#66168,#66169,#66170,#66171,
#66172,#66173,#66174,#66175,#66176,#66177,#66178,#66179,#66180,#66181,#66182,
#66183,#66184,#66185,#66186,#66187,#66188,#66189,#66190,#66191,#66192,#66193,
#66194,#66195,#66196,#66197,#66198,#66199,#66200,#66201,#66202,#66203,#66204,
#66205,#66206,#66207,#66208,#66209,#66210,#66211,#66212,#66213,#66214,#66215,
#66216,#66217,#66218,#66219,#66220,#66221,#66222,#66223,#66224,#66225,#66226,
#66227,#66228,#66229,#66230,#66231,#66232,#66233,#66234,#66235,#66236,#66237,
#66238,#66239,#66240,#66241,#66242,#66243,#66244,#66245,#66246,#66247,#66248,
#66249,#66250,#66251,#66252,#66253,#66254,#66255,#66256,#66257,#66258,#66259,
#66260,#66261,#66262,#66263,#66264,#66265,#66266,#66267,#66268,#66269,#66270,
#66271,#66272,#66273,#66274,#66275,#66276,#66277,#66278,#66279,#66280,#66281,
#66282,#66283,#66284,#66285,#66286,#66287,#66288,#66289,#66290,#66291,#66292,
#66293,#66294,#66295,#66296,#66297,#66298,#66299,#66300,#66301,#66302,#66303,
#66304,#66305,#66306,#66307,#66308,#66309,#66310,#66311,#66312,#66313,#66314,
#66315,#66316,#66317,#66318,#66319,#66320,#66321,#66322,#66323,#66324,#66325,
#66326,#66327,#66328,#66329,#66330,#66331,#66332,#66333,#66334,#66335,#66336,
#66337,#66338,#66339,#66340,#66341,#66342,#66343,#66344,#66345,#66346,#66347,
#66348,#66349,#66350,#66351,#66352,#66353,#66354,#66355,#66356,#66357,#66358,
#66359,#66360,#66361,#66362,#66363,#66364,#66365,#66366,#66367,#66368,#66369,
#66370,#66371,#66372,#66373,#66374,#66375,#66376,#66377,#66378,#66379,#66380,
#66381,#66382,#66383,#66384,#66385,#66386,#66387,#66388,#66389,#66390,#66391,
#66392,#66393,#66394,#66395,#66396,#66397,#66398,#66399,#66400,#66401,#66402,
#66403,#66404,#66405,#66406,#66407),.UNSPECIFIED.,.F.,.F.,(4,2,2,2,2,2,
2,2,2,2,2,2,2,2,2,2,2,2,2,2,2,2,2,2,2,2,2,2,2,2,2,2,2,2,2,2,2,2,2,2,2,2,
2,2,2,2,2,2,2,2,2,2,2,2,2,2,2,2,2,2,2,2,2,2,2,2,2,2,2,2,2,2,2,2,2,2,2,2,
2,2,2,2,2,2,2,2,2,2,2,2,2,2,2,2,2,2,2,2,2,2,2,2,2,2,2,2,2,2,2,2,2,2,2,2,
2,2,2,2,2,2,2,2,2,2,2,2,2,2,2,2,2,2,2,2,2,2,2,2,2,2,2,2,2,2,2,2,2,2,2,2,
2,2,2,2,2,2,2,2,2,2,2,2,2,2,2,2,2,2,2,2,2,2,2,2,2,2,2,2,2,2,2,2,2,2,2,2,
2,2,2,2,2,2,2,2,2,2,2,2,2,2,2,2,2,2,2,2,2,2,2,2,2,2,2,2,2,2,2,2,2,2,2,2,
2,2,2,2,2,2,2,2,2,2,2,2,2,2,2,2,2,2,2,2,2,2,2,2,2,2,2,2,2,2,2,2,2,2,2,2,
2,2,2,2,2,2,2,2,2,2,2,2,2,2,2,2,2,2,2,2,2,4),(0.00156532237835257,0.17091198575568,
0.207222044334215,0.213114571822337,0.214859008958513,0.21593723683326,
0.216920339048251,0.218180441939555,0.220252266223459,0.231571329861011,
0.232374313989906,0.421839154393626,0.441471010575572,0.45895600194081,
0.496527568298866,0.620284332679301,0.625704004424397,0.628130491401357,
0.629936452366404,0.631617985894264,0.633920560157569,0.639692817873232,
0.704397104304271,0.831718616604965,0.897726105172791,0.979889125669097,
1.01542845563187,1.02210293679107,1.02428389357666,1.02568464164343,1.02699850312874,
1.02871830861566,1.03161118657523,1.0490064374067,1.23167620699884,1.32241227949923,
1.36745586561959,1.39252393554242,1.39823731160618,1.4009526180676,1.40350295568623,
1.40619311151654,1.40994760655908,1.4176164505781,1.49633768409118,1.61407369888607,
1.70869963385546,1.76494143491077,1.77504926126684,1.77758213928747,1.77906146779443,
1.78035682133211,1.78195784055565,1.78439717193456,1.79498606567316,1.94322770270387,
2.03919426651885,2.13822307967879,2.15423385763598,2.16956404976285,2.17315533580032,
2.1752099541776,2.1768052663174,2.1786154504831,2.18201236143277,2.19348056050792,
2.35556996007128,2.47745658925013,2.52751920776311,2.57868561417901,2.5858835663221,
2.58774864820281,2.58884947920185,2.58982835895663,2.59106415765009,2.59299829580082,
2.60217579955307,2.74132338282202,2.83059035182472,2.91432313816549,2.95587350324658,
2.97831503175031,2.98245753596772,2.98462106226711,2.98621278202622,2.98793169076646,
2.99092079530467,2.99936298900047,3.12377123290145,3.27438478098718,3.344449639781,
3.37694349084083,3.3796949179669,3.38100138450275,3.38192206805785,3.38287946950333,
3.38419822687073,3.38683677495832,3.40947362848246,3.53937227605842,3.69126386474088,
3.76354160547186,3.7712511287355,3.77697651393606,3.77952774811514,3.78139913749344,
3.7831222778922,3.78545238950731,3.79114632494279,3.84772510466974,3.89428917158918,
4.0797698411106,4.11179213214894,4.14970406585538,4.16597163644554,4.16845506224293,
4.169733632886,4.17076587052824,4.17195526839645,4.17397262786818,4.18125801802497,
4.29057331604547,4.46630886885966,4.55034907080562,4.55570588938883,4.55816553348199,
4.56002159322068,4.56176837821911,4.56418972654398,4.56908033885465,4.6133189880826,
4.6335836262616,4.83742579194341,4.90010496954302,4.94859638373132,4.95569551757532,
4.95759889516182,4.95873495671618,4.95974483635744,4.96101287277483,4.96348016474068,
4.97764364645044,5.00914422764245,5.06583248171667,5.33250055608807,5.34879440441641,
5.35226230016677,5.3544855010552,5.35625083866129,5.35823138303028,5.36153740835061,
5.3737467498349,5.45360670002394,5.60629983614269,5.73985202249173,5.74834712965012,
5.75022802371263,5.75144721071487,5.7524243432637,5.75353588678314,5.75544973085389,
5.76321694698121,5.82397826486286,5.88385225661824,6.06049972388032,6.09418470132512,
6.15538855396458,6.16108400927817,6.16337286417672,6.16505053529474,6.16685820374977,
6.16929717513358,6.17466579819149,6.18184257204658,6.2475354714967,6.39663328727209,
6.49356792896584,6.55407445078301,6.55837994976079,6.56007512299525,6.56130534236182,
6.5624876963338,6.5641646236099,6.56763252385029,6.60099662200162,6.6654308425079,
6.91498632094265,6.92983507866367,6.93479076784127,6.93756979963217,6.940320018155,
6.94368831065719,6.94731092978816,6.9530111204984,6.96385462201226,7.0243742017623,
7.08283889007759,7.29986043561504,7.31061465140634,7.31306549767383,7.31466883456716,
7.31583470102624,7.31726951457356,7.3196046408652,7.32762656154413,7.37575038783523,
7.40613398370776,7.5658047327608,7.69753177017189,7.70642659746195,7.70949467328503,
7.71123834266517,7.71284027042881,7.71499856283841,7.71898658129515,7.73639492694558,
7.76950801501643,7.8501973758505,7.92069692995797,8.10892538928674,8.10945343827896,
8.12089009653594,8.12296859413053,8.12423041706083,8.1252134091904,8.12629006813002,
8.12802879177178,8.13387312449858,8.1697202082136,8.23781482028477,8.31223464550103,
8.40171163419133,8.45150171697918,8.45997506133572,8.46625489428652,8.46826786736495,
8.51216207554354,8.51743462767127,8.51979593742876,8.52158606653488,8.52348126375185,
8.52540708939205,8.53107899814716,8.5915877747844,8.67948461743734,8.9001746809301,
8.91319202847375,8.91538019121428,8.91669279506628,8.91771089239394,8.9188113106224,
8.92055604854181,8.92614334966688,8.95889910609161,9.02907506070383,9.10307630689263,
9.14101548565173,9.18836401865907,9.30373870124536,9.31159270675471,9.31456095996236,
9.31632104103345,9.31798555639991,9.31976121288474,9.32201769810091,9.32548479189891,
9.36082397496341,9.41954965255361,9.46215601694711,9.66516308305237,9.68232515367044,
9.70106288747595,9.70359777460581,9.70490459607476,9.70587290571473,9.70693226598835,
9.70840375989528,9.71190547133014,9.81939241609079,9.95375608942013),
 .UNSPECIFIED.);
#559=B_SPLINE_CURVE_WITH_KNOTS('',3,(#66408,#66409,#66410,#66411,#66412,
#66413,#66414,#66415,#66416,#66417,#66418,#66419,#66420,#66421,#66422,#66423,
#66424,#66425,#66426,#66427,#66428,#66429,#66430,#66431,#66432,#66433,#66434,
#66435,#66436,#66437,#66438,#66439,#66440,#66441,#66442,#66443,#66444,#66445,
#66446,#66447,#66448,#66449,#66450,#66451,#66452,#66453,#66454,#66455,#66456,
#66457,#66458,#66459,#66460,#66461,#66462,#66463,#66464,#66465,#66466,#66467,
#66468,#66469,#66470,#66471,#66472,#66473,#66474,#66475,#66476,#66477,#66478,
#66479,#66480,#66481,#66482,#66483,#66484,#66485,#66486,#66487,#66488,#66489,
#66490,#66491,#66492,#66493,#66494,#66495,#66496,#66497,#66498,#66499,#66500,
#66501,#66502,#66503,#66504,#66505,#66506,#66507,#66508,#66509,#66510,#66511,
#66512,#66513,#66514,#66515,#66516,#66517,#66518,#66519,#66520,#66521,#66522,
#66523,#66524,#66525,#66526,#66527,#66528,#66529,#66530,#66531,#66532,#66533,
#66534,#66535,#66536,#66537,#66538,#66539,#66540,#66541,#66542,#66543,#66544,
#66545,#66546,#66547,#66548,#66549,#66550,#66551,#66552,#66553,#66554,#66555,
#66556,#66557,#66558,#66559,#66560,#66561,#66562,#66563,#66564,#66565,#66566,
#66567,#66568,#66569,#66570,#66571,#66572,#66573,#66574,#66575,#66576,#66577,
#66578,#66579,#66580,#66581,#66582,#66583,#66584,#66585,#66586,#66587,#66588,
#66589,#66590,#66591,#66592,#66593,#66594,#66595,#66596,#66597,#66598,#66599,
#66600,#66601,#66602,#66603,#66604,#66605,#66606,#66607,#66608,#66609,#66610,
#66611,#66612,#66613,#66614,#66615,#66616,#66617,#66618,#66619,#66620,#66621,
#66622,#66623,#66624,#66625,#66626,#66627,#66628,#66629,#66630,#66631,#66632,
#66633,#66634,#66635,#66636,#66637,#66638,#66639,#66640,#66641,#66642,#66643,
#66644,#66645,#66646,#66647,#66648,#66649,#66650,#66651,#66652,#66653,#66654,
#66655,#66656,#66657,#66658,#66659,#66660,#66661,#66662,#66663,#66664,#66665,
#66666,#66667,#66668,#66669,#66670,#66671,#66672,#66673,#66674,#66675,#66676,
#66677,#66678,#66679,#66680,#66681,#66682,#66683,#66684,#66685,#66686,#66687,
#66688,#66689,#66690,#66691,#66692,#66693,#66694,#66695,#66696,#66697,#66698,
#66699,#66700,#66701,#66702,#66703,#66704,#66705,#66706,#66707,#66708,#66709,
#66710,#66711,#66712,#66713,#66714,#66715,#66716,#66717,#66718,#66719,#66720,
#66721,#66722,#66723,#66724,#66725,#66726,#66727,#66728,#66729,#66730,#66731,
#66732,#66733,#66734,#66735,#66736,#66737,#66738,#66739,#66740,#66741,#66742,
#66743,#66744,#66745,#66746,#66747,#66748,#66749,#66750,#66751,#66752,#66753,
#66754,#66755,#66756,#66757,#66758,#66759,#66760,#66761,#66762,#66763,#66764,
#66765,#66766,#66767,#66768,#66769,#66770,#66771,#66772,#66773,#66774,#66775,
#66776,#66777,#66778,#66779,#66780,#66781,#66782,#66783,#66784,#66785,#66786,
#66787,#66788,#66789,#66790,#66791,#66792,#66793,#66794,#66795,#66796,#66797,
#66798,#66799,#66800,#66801,#66802,#66803,#66804,#66805,#66806,#66807,#66808,
#66809,#66810,#66811,#66812,#66813,#66814,#66815,#66816,#66817,#66818,#66819,
#66820,#66821,#66822,#66823,#66824,#66825,#66826,#66827,#66828,#66829,#66830,
#66831,#66832,#66833,#66834,#66835,#66836,#66837,#66838,#66839,#66840,#66841,
#66842,#66843,#66844,#66845,#66846,#66847,#66848,#66849,#66850,#66851,#66852,
#66853,#66854,#66855,#66856,#66857,#66858,#66859,#66860,#66861,#66862,#66863,
#66864,#66865,#66866,#66867,#66868,#66869,#66870,#66871,#66872,#66873,#66874,
#66875,#66876,#66877,#66878,#66879,#66880,#66881,#66882,#66883,#66884,#66885,
#66886,#66887,#66888,#66889,#66890,#66891,#66892,#66893,#66894,#66895,#66896,
#66897,#66898,#66899,#66900,#66901,#66902,#66903,#66904,#66905,#66906,#66907,
#66908,#66909,#66910,#66911,#66912,#66913,#66914,#66915,#66916,#66917,#66918,
#66919,#66920,#66921,#66922,#66923,#66924,#66925,#66926,#66927,#66928,#66929,
#66930,#66931,#66932,#66933,#66934,#66935,#66936,#66937,#66938,#66939,#66940,
#66941,#66942,#66943,#66944,#66945,#66946,#66947,#66948,#66949,#66950,#66951,
#66952,#66953,#66954,#66955,#66956,#66957,#66958,#66959,#66960,#66961,#66962,
#66963,#66964,#66965,#66966,#66967,#66968,#66969,#66970,#66971,#66972,#66973,
#66974,#66975,#66976,#66977,#66978,#66979),.UNSPECIFIED.,.F.,.F.,(4,2,2,
2,2,2,2,2,2,2,2,2,2,2,2,2,2,2,2,2,2,2,2,2,2,2,2,2,2,2,2,2,2,2,2,2,2,2,2,
2,2,2,2,2,2,2,2,2,2,2,2,2,2,2,2,2,2,2,2,2,2,2,2,2,2,2,2,2,2,2,2,2,2,2,2,
2,2,2,2,2,2,2,2,2,2,2,2,2,2,2,2,2,2,2,2,2,2,2,2,2,2,2,2,2,2,2,2,2,2,2,2,
2,2,2,2,2,2,2,2,2,2,2,2,2,2,2,2,2,2,2,2,2,2,2,2,2,2,2,2,2,2,2,2,2,2,2,2,
2,2,2,2,2,2,2,2,2,2,2,2,2,2,2,2,2,2,2,2,2,2,2,2,2,2,2,2,2,2,2,2,2,2,2,2,
2,2,2,2,2,2,2,2,2,2,2,2,2,2,2,2,2,2,2,2,2,2,2,2,2,2,2,2,2,2,2,2,2,2,2,2,
2,2,2,2,2,2,2,2,2,2,2,2,2,2,2,2,2,2,2,2,2,2,2,2,2,2,2,2,2,2,2,2,2,2,2,2,
2,2,2,2,2,2,2,2,2,2,2,2,2,2,2,2,2,2,2,2,2,2,2,2,2,2,2,2,2,2,4),(0.00230660127850738,
0.128345221299926,0.134920681005092,0.138444386242725,0.140724949474323,
0.142508472062085,0.144177389799666,0.145928375692367,0.148364814814351,
0.154681539308349,0.238875327581102,0.276509332655191,0.287233309423933,
0.473069833707347,0.537672296612725,0.540906916335336,0.542312915935396,
0.543342879364206,0.544290082307809,0.545569450243708,0.5487438631145,0.583747592806631,
0.78634720366351,0.847112789003208,0.905598660780656,0.923021431936684,
0.933872207622032,0.936219605831329,0.937987456768179,0.939783021604548,
0.941444244688455,0.943702663790448,0.949281257397128,1.00734723993167,
1.07414691052537,1.157715840318,1.16787183435951,1.17948683764632,1.19290049275817,
1.20863044925713,1.22756443935456,1.29639674228562,1.32754297526308,1.33289680491233,
1.33458009829973,1.33564457361223,1.3366317942913,1.33792121116186,1.34076453027969,
1.36312884601792,1.56197401493471,1.66178182418684,1.71630562546323,1.73307022502847,
1.74362884824775,1.74596989535025,1.74816415585285,1.74994003945794,1.75170832830087,
1.75489757584768,1.76468077755972,1.90701099886728,2.05730317281499,2.08461541888431,
2.1333582496924,2.14143935599111,2.14378098857757,2.14521741964217,2.14638333802988,
2.14798473875959,2.15042892032036,2.16110029256818,2.37628271934823,2.43521607290879,
2.49681578006484,2.50792333901872,2.51372459313611,2.51738987593,2.52078648865102,
2.52354038564477,2.52630310747086,2.53117715381897,2.54542750470412,2.7918392715674,
2.84929342443344,2.88896022903573,2.8957843922249,2.89798335465623,2.89938784519667,
2.90069970591071,2.90240880974919,2.9061387035619,2.93826085567872,2.94174329558787,
2.95514697192867,2.97924175159734,3.05224976599085,3.15913856134385,3.25331654834907,
3.28677108277123,3.29199599100632,3.2944331146302,3.29624057798281,3.29791888993328,
3.30020990163617,3.30591727664759,3.36758624221959,3.42175484108784,3.58915467387187,
3.65151698971242,3.69894673490316,3.70585918591164,3.70769819521392,3.70879321949632,
3.70977317851828,3.71101843987944,3.71298314717672,3.72257483818995,3.87303308975443,
4.01914424311439,4.09605319841951,4.10164296966842,4.10408832386243,4.1058860006037,
4.10754402157203,4.1097902289916,4.11529947943244,4.1707324262075,4.39503258938269,
4.45173176096255,4.4833223073281,4.49778884667176,4.50011295118531,4.50133568971659,
4.50234226643736,4.50351112526991,4.50550853085898,4.51286867514984,4.62210180040717,
4.77700987720342,4.83307348977952,4.88616788589078,4.89579457589138,4.89890218937483,
4.90088856190432,4.90274504239576,4.90516547629103,4.90921284607816,4.93293175548031,
4.94410876979255,4.95209591288574,4.98036213696699,5.03851983158081,5.26493346155454,
5.28560182345081,5.28850058350351,5.2898478001113,5.29089006673285,5.29202497430403,
5.29385308129089,5.2999563389031,5.36670758665547,5.48510936851614,5.66216643158317,
5.6739141294271,5.67740818314465,5.67927338924316,5.68091900195438,5.68304090309669,
5.6867570949866,5.70273044109283,5.73111623245015,5.78306163032006,6.00348430390019,
6.04266633459154,6.04552718570898,6.04809754522921,6.05131497396005,6.07448089261174,
6.07743121040447,6.07877042537367,6.07979289479764,6.08088226325311,6.08258262450377,
6.08799872927215,6.11962239041733,6.16620548944169,6.28477887436226,6.45786471015039,
6.4696825710734,6.47310373408216,6.47511130885555,6.47685817416462,6.47903750820815,
6.48324994677044,6.51027789042411,6.57055824293226,6.6805624832239,6.85933012443352,
6.86849540404132,6.87042968254335,6.87166606881031,6.87264573403327,6.8737251276232,
6.87553041241013,6.87769673323445,6.88197942829283,7.01139060248478,7.21690260981582,
7.27565974944715,7.28129550649728,7.28357496460972,7.28525090397973,7.28706164310502,
7.28951346022059,7.29506951458921,7.3761168334038,7.47051139731932,7.66410799346736,
7.6764962685436,7.6790635898108,7.68069669816208,7.68195812208696,7.68335631094932,
7.6856149414343,7.68829790976247,7.69348615884106,7.70620794947686,7.74904395165377,
7.81074717894133,8.03568726524247,8.04944531275463,8.05417144639542,8.05685485940246,
8.05931959978896,8.06262292863043,8.06875449169653,8.10189391594875,8.1656505340179,
8.28216252427989,8.40883989268998,8.43040719690892,8.43381011908805,8.43546047111226,
8.43669707232212,8.43806938165352,8.44023563622075,8.44276388066525,8.44751142388798,
8.45853056711512,8.49505075917323,8.52664168920347,8.81104765590495,8.82767841720906,
8.83117233643037,8.83340383151837,8.83517038255303,8.83714664447517,8.84043226537289,
8.85242323119308,8.92947229407872,9.05134171018654,9.10292432586987,9.16474973800832,
9.21340043738603,9.24164175279483,9.24436266525319,9.24567287580225,9.24660748479505,
9.24749783839472,9.24845060594464,9.24966918715297,9.25447493580103,9.31035283527648,
9.34706401935888,9.58339405392858,9.63639247904457,9.64141583360316,9.64383091101246,
9.64554061864745,9.64714914952137,9.64937505856541,9.65377537708792,9.6855358940007,
9.78208413797257,9.95839499409821),.UNSPECIFIED.);
#560=B_SPLINE_CURVE_WITH_KNOTS('',3,(#67039,#67040,#67041,#67042,#67043,
#67044,#67045,#67046,#67047,#67048,#67049,#67050,#67051,#67052,#67053,#67054,
#67055,#67056,#67057,#67058,#67059,#67060,#67061,#67062,#67063,#67064,#67065,
#67066,#67067,#67068),.UNSPECIFIED.,.F.,.F.,(4,2,2,2,2,2,2,2,2,2,2,2,2,
2,4),(-5.1172649587789,-4.77125985892989,-4.39072557177308,-3.78322541506865,
-3.21302721090485,-2.63736934344719,-2.17538637120503,-1.75347930631198,
-1.43774045964503,-1.15825087501937,-0.854608089732673,-0.620651733076443,
-0.367068559363653,-0.196690632762468,-0.000776879412541869),
 .UNSPECIFIED.);
#561=B_SPLINE_CURVE_WITH_KNOTS('',3,(#67069,#67070,#67071,#67072,#67073,
#67074,#67075,#67076,#67077,#67078,#67079,#67080,#67081,#67082,#67083,#67084,
#67085,#67086,#67087,#67088,#67089,#67090,#67091,#67092,#67093,#67094,#67095,
#67096,#67097,#67098,#67099,#67100,#67101,#67102,#67103,#67104,#67105,#67106,
#67107,#67108,#67109,#67110,#67111,#67112,#67113,#67114,#67115,#67116,#67117,
#67118,#67119,#67120,#67121,#67122,#67123,#67124,#67125,#67126,#67127,#67128,
#67129,#67130,#67131,#67132,#67133,#67134,#67135,#67136,#67137,#67138),
 .UNSPECIFIED.,.F.,.F.,(4,3,3,3,3,3,3,3,3,3,3,3,3,3,3,3,3,3,3,3,3,3,3,4),
(-1.12803176442304,-1.06660631931699,-1.00636787721923,-0.961112508690392,
-0.899376762802759,-0.85939191897837,-0.849462260101921,-0.842475058397111,
-0.782885726971055,-0.72274595667072,-0.662901991936166,-0.604134381573305,
-0.579498012207646,-0.565265641437903,-0.554476152855422,-0.547373062825023,
-0.489041380710527,-0.430655486338116,-0.372940968315836,-0.315893092681781,
-0.290970068308981,-0.275474495988932,-0.266102779271428,-0.216200995190583),
 .UNSPECIFIED.);
#562=B_SPLINE_CURVE_WITH_KNOTS('',3,(#69371,#69372,#69373,#69374,#69375,
#69376,#69377,#69378,#69379,#69380,#69381,#69382,#69383,#69384,#69385,#69386,
#69387,#69388,#69389,#69390,#69391,#69392,#69393,#69394,#69395,#69396,#69397,
#69398,#69399,#69400,#69401,#69402,#69403,#69404,#69405,#69406,#69407,#69408,
#69409,#69410,#69411,#69412,#69413,#69414,#69415,#69416,#69417,#69418,#69419,
#69420,#69421,#69422,#69423,#69424,#69425,#69426,#69427,#69428,#69429,#69430,
#69431,#69432,#69433,#69434,#69435,#69436,#69437,#69438,#69439,#69440,#69441,
#69442,#69443,#69444,#69445,#69446,#69447,#69448,#69449,#69450,#69451,#69452,
#69453,#69454,#69455,#69456,#69457,#69458,#69459,#69460,#69461,#69462,#69463,
#69464,#69465,#69466,#69467,#69468,#69469,#69470,#69471,#69472,#69473,#69474,
#69475,#69476,#69477,#69478,#69479),.UNSPECIFIED.,.F.,.F.,(4,3,3,3,3,3,
3,3,3,3,3,3,3,3,3,3,3,3,3,3,3,3,3,3,3,3,3,3,3,3,3,3,3,3,3,3,4),(-1.52870610664526,
-1.4669968085376,-1.40516063220429,-1.34270018454279,-1.32404855442001,
-1.31376060856527,-1.25232916205104,-1.19058262877584,-1.12913545396555,
-1.1198174668383,-1.11189637748511,-1.05127683134977,-0.9908173650714,-0.93102541318309,
-0.875002691406706,-0.832985650074418,-0.821141831585003,-0.762941140003209,
-0.706934526077554,-0.648166878086584,-0.589327029396728,-0.558993140800858,
-0.547233056843969,-0.537331142832007,-0.47987739433253,-0.42225444188307,
-0.365147363201414,-0.346655920629775,-0.30332393055107,-0.283703366897939,
-0.271772304256833,-0.26150992201455,-0.205232539959138,-0.149113591098172,
-0.0934593024883868,-0.0388976662899543,-1.34448406245148E-13),
 .UNSPECIFIED.);
#563=B_SPLINE_CURVE_WITH_KNOTS('',3,(#71716,#71717,#71718,#71719,#71720,
#71721,#71722,#71723,#71724,#71725,#71726,#71727,#71728,#71729,#71730,#71731,
#71732,#71733,#71734,#71735,#71736,#71737,#71738,#71739,#71740,#71741,#71742,
#71743,#71744,#71745,#71746,#71747,#71748,#71749,#71750,#71751,#71752,#71753,
#71754,#71755,#71756,#71757,#71758,#71759,#71760,#71761,#71762,#71763,#71764,
#71765,#71766,#71767,#71768,#71769,#71770,#71771,#71772,#71773,#71774,#71775,
#71776,#71777,#71778,#71779,#71780,#71781,#71782,#71783,#71784,#71785,#71786,
#71787,#71788,#71789,#71790,#71791,#71792,#71793,#71794,#71795,#71796,#71797,
#71798,#71799,#71800,#71801,#71802,#71803,#71804,#71805,#71806,#71807,#71808,
#71809,#71810,#71811,#71812,#71813,#71814,#71815,#71816,#71817,#71818,#71819,
#71820,#71821,#71822,#71823,#71824),.UNSPECIFIED.,.F.,.F.,(4,3,3,3,3,3,
3,3,3,3,3,3,3,3,3,3,3,3,3,3,3,3,3,3,3,3,3,3,3,3,3,3,3,3,3,3,4),(-1.53373699248731,
-1.4821365546276,-1.42770923574272,-1.37225914868662,-1.35730091972004,
-1.3456492103406,-1.2887137341168,-1.23163095606003,-1.1889477616213,-1.17417243892694,
-1.16116852269338,-1.14054366009933,-1.08259591133439,-1.02385609453003,
-0.965203361155031,-0.907403642265373,-0.890165400550202,-0.883312518347464,
-0.823389257062025,-0.768413556573938,-0.710270076125937,-0.651296044762335,
-0.618741054482267,-0.600604850453944,-0.581663798302628,-0.522138221798477,
-0.461815506006418,-0.400951391085016,-0.39085612252179,-0.330016377059625,
-0.310377881025886,-0.303327250694008,-0.241908819659544,-0.179747915445459,
-0.117618730811708,-0.0562544900865141,0.),.UNSPECIFIED.);
#894=SHAPE_REPRESENTATION_RELATIONSHIP('SRR','None',#105862,#906);
#906=ADVANCED_BREP_SHAPE_REPRESENTATION('',(#930),#105797);
#918=STYLED_ITEM('',(#105931),#930);
#930=MANIFOLD_SOLID_BREP('Body1',#7205);
#959=FACE_BOUND('',#1463,.T.);
#960=FACE_BOUND('',#1465,.T.);
#961=FACE_BOUND('',#1470,.T.);
#962=FACE_BOUND('',#1473,.T.);
#963=FACE_BOUND('',#1489,.T.);
#964=FACE_BOUND('',#1490,.T.);
#965=FACE_BOUND('',#1491,.T.);
#966=FACE_BOUND('',#1492,.T.);
#967=FACE_BOUND('',#1493,.T.);
#968=FACE_BOUND('',#1496,.T.);
#969=FACE_BOUND('',#1497,.T.);
#970=FACE_BOUND('',#1498,.T.);
#971=FACE_BOUND('',#1499,.T.);
#972=FACE_BOUND('',#1500,.T.);
#1012=PLANE('',#7485);
#1013=PLANE('',#7487);
#1014=PLANE('',#7493);
#1015=PLANE('',#7494);
#1016=PLANE('',#7501);
#1017=PLANE('',#7515);
#1018=PLANE('',#7516);
#1019=PLANE('',#7517);
#1020=PLANE('',#7518);
#1021=PLANE('',#7519);
#1022=PLANE('',#7520);
#1023=PLANE('',#7521);
#1024=PLANE('',#7522);
#1025=PLANE('',#7526);
#1090=FACE_OUTER_BOUND('',#1382,.T.);
#1091=FACE_OUTER_BOUND('',#1383,.T.);
#1092=FACE_OUTER_BOUND('',#1384,.T.);
#1093=FACE_OUTER_BOUND('',#1385,.T.);
#1094=FACE_OUTER_BOUND('',#1386,.T.);
#1095=FACE_OUTER_BOUND('',#1387,.T.);
#1096=FACE_OUTER_BOUND('',#1388,.T.);
#1097=FACE_OUTER_BOUND('',#1389,.T.);
#1098=FACE_OUTER_BOUND('',#1390,.T.);
#1099=FACE_OUTER_BOUND('',#1391,.T.);
#1100=FACE_OUTER_BOUND('',#1392,.T.);
#1101=FACE_OUTER_BOUND('',#1393,.T.);
#1102=FACE_OUTER_BOUND('',#1394,.T.);
#1103=FACE_OUTER_BOUND('',#1395,.T.);
#1104=FACE_OUTER_BOUND('',#1396,.T.);
#1105=FACE_OUTER_BOUND('',#1397,.T.);
#1106=FACE_OUTER_BOUND('',#1398,.T.);
#1107=FACE_OUTER_BOUND('',#1399,.T.);
#1108=FACE_OUTER_BOUND('',#1400,.T.);
#1109=FACE_OUTER_BOUND('',#1401,.T.);
#1110=FACE_OUTER_BOUND('',#1402,.T.);
#1111=FACE_OUTER_BOUND('',#1403,.T.);
#1112=FACE_OUTER_BOUND('',#1404,.T.);
#1113=FACE_OUTER_BOUND('',#1405,.T.);
#1114=FACE_OUTER_BOUND('',#1406,.T.);
#1115=FACE_OUTER_BOUND('',#1407,.T.);
#1116=FACE_OUTER_BOUND('',#1408,.T.);
#1117=FACE_OUTER_BOUND('',#1409,.T.);
#1118=FACE_OUTER_BOUND('',#1410,.T.);
#1119=FACE_OUTER_BOUND('',#1411,.T.);
#1120=FACE_OUTER_BOUND('',#1412,.T.);
#1121=FACE_OUTER_BOUND('',#1413,.T.);
#1122=FACE_OUTER_BOUND('',#1414,.T.);
#1123=FACE_OUTER_BOUND('',#1415,.T.);
#1124=FACE_OUTER_BOUND('',#1416,.T.);
#1125=FACE_OUTER_BOUND('',#1417,.T.);
#1126=FACE_OUTER_BOUND('',#1418,.T.);
#1127=FACE_OUTER_BOUND('',#1419,.T.);
#1128=FACE_OUTER_BOUND('',#1420,.T.);
#1129=FACE_OUTER_BOUND('',#1421,.T.);
#1130=FACE_OUTER_BOUND('',#1422,.T.);
#1131=FACE_OUTER_BOUND('',#1423,.T.);
#1132=FACE_OUTER_BOUND('',#1424,.T.);
#1133=FACE_OUTER_BOUND('',#1425,.T.);
#1134=FACE_OUTER_BOUND('',#1426,.T.);
#1135=FACE_OUTER_BOUND('',#1427,.T.);
#1136=FACE_OUTER_BOUND('',#1428,.T.);
#1137=FACE_OUTER_BOUND('',#1429,.T.);
#1138=FACE_OUTER_BOUND('',#1430,.T.);
#1139=FACE_OUTER_BOUND('',#1431,.T.);
#1140=FACE_OUTER_BOUND('',#1432,.T.);
#1141=FACE_OUTER_BOUND('',#1433,.T.);
#1142=FACE_OUTER_BOUND('',#1434,.T.);
#1143=FACE_OUTER_BOUND('',#1435,.T.);
#1144=FACE_OUTER_BOUND('',#1436,.T.);
#1145=FACE_OUTER_BOUND('',#1437,.T.);
#1146=FACE_OUTER_BOUND('',#1438,.T.);
#1147=FACE_OUTER_BOUND('',#1439,.T.);
#1148=FACE_OUTER_BOUND('',#1440,.T.);
#1149=FACE_OUTER_BOUND('',#1441,.T.);
#1150=FACE_OUTER_BOUND('',#1442,.T.);
#1151=FACE_OUTER_BOUND('',#1443,.T.);
#1152=FACE_OUTER_BOUND('',#1444,.T.);
#1153=FACE_OUTER_BOUND('',#1445,.T.);
#1154=FACE_OUTER_BOUND('',#1446,.T.);
#1155=FACE_OUTER_BOUND('',#1447,.T.);
#1156=FACE_OUTER_BOUND('',#1448,.T.);
#1157=FACE_OUTER_BOUND('',#1449,.T.);
#1158=FACE_OUTER_BOUND('',#1450,.T.);
#1159=FACE_OUTER_BOUND('',#1451,.T.);
#1160=FACE_OUTER_BOUND('',#1452,.T.);
#1161=FACE_OUTER_BOUND('',#1453,.T.);
#1162=FACE_OUTER_BOUND('',#1454,.T.);
#1163=FACE_OUTER_BOUND('',#1455,.T.);
#1164=FACE_OUTER_BOUND('',#1456,.T.);
#1165=FACE_OUTER_BOUND('',#1457,.T.);
#1166=FACE_OUTER_BOUND('',#1458,.T.);
#1167=FACE_OUTER_BOUND('',#1459,.T.);
#1168=FACE_OUTER_BOUND('',#1460,.T.);
#1169=FACE_OUTER_BOUND('',#1461,.T.);
#1170=FACE_OUTER_BOUND('',#1462,.T.);
#1171=FACE_OUTER_BOUND('',#1464,.T.);
#1172=FACE_OUTER_BOUND('',#1466,.T.);
#1173=FACE_OUTER_BOUND('',#1467,.T.);
#1174=FACE_OUTER_BOUND('',#1468,.T.);
#1175=FACE_OUTER_BOUND('',#1469,.T.);
#1176=FACE_OUTER_BOUND('',#1471,.T.);
#1177=FACE_OUTER_BOUND('',#1472,.T.);
#1178=FACE_OUTER_BOUND('',#1474,.T.);
#1179=FACE_OUTER_BOUND('',#1475,.T.);
#1180=FACE_OUTER_BOUND('',#1476,.T.);
#1181=FACE_OUTER_BOUND('',#1477,.T.);
#1182=FACE_OUTER_BOUND('',#1478,.T.);
#1183=FACE_OUTER_BOUND('',#1479,.T.);
#1184=FACE_OUTER_BOUND('',#1480,.T.);
#1185=FACE_OUTER_BOUND('',#1481,.T.);
#1186=FACE_OUTER_BOUND('',#1482,.T.);
#1187=FACE_OUTER_BOUND('',#1483,.T.);
#1188=FACE_OUTER_BOUND('',#1484,.T.);
#1189=FACE_OUTER_BOUND('',#1485,.T.);
#1190=FACE_OUTER_BOUND('',#1486,.T.);
#1191=FACE_OUTER_BOUND('',#1487,.T.);
#1192=FACE_OUTER_BOUND('',#1488,.T.);
#1193=FACE_OUTER_BOUND('',#1494,.T.);
#1194=FACE_OUTER_BOUND('',#1495,.T.);
#1382=EDGE_LOOP('',(#4527,#4528,#4529,#4530));
#1383=EDGE_LOOP('',(#4531,#4532,#4533,#4534,#4535,#4536));
#1384=EDGE_LOOP('',(#4537,#4538,#4539,#4540,#4541,#4542));
#1385=EDGE_LOOP('',(#4543,#4544,#4545,#4546,#4547,#4548));
#1386=EDGE_LOOP('',(#4549,#4550,#4551,#4552,#4553,#4554));
#1387=EDGE_LOOP('',(#4555,#4556,#4557,#4558,#4559,#4560));
#1388=EDGE_LOOP('',(#4561,#4562,#4563,#4564,#4565,#4566));
#1389=EDGE_LOOP('',(#4567,#4568,#4569,#4570,#4571,#4572));
#1390=EDGE_LOOP('',(#4573,#4574,#4575,#4576,#4577,#4578));
#1391=EDGE_LOOP('',(#4579,#4580,#4581,#4582,#4583,#4584));
#1392=EDGE_LOOP('',(#4585,#4586,#4587,#4588,#4589,#4590));
#1393=EDGE_LOOP('',(#4591,#4592,#4593,#4594,#4595,#4596));
#1394=EDGE_LOOP('',(#4597,#4598,#4599,#4600,#4601,#4602));
#1395=EDGE_LOOP('',(#4603,#4604,#4605,#4606,#4607,#4608));
#1396=EDGE_LOOP('',(#4609,#4610,#4611,#4612,#4613,#4614));
#1397=EDGE_LOOP('',(#4615,#4616,#4617,#4618,#4619,#4620));
#1398=EDGE_LOOP('',(#4621,#4622,#4623,#4624,#4625,#4626));
#1399=EDGE_LOOP('',(#4627,#4628,#4629,#4630,#4631,#4632));
#1400=EDGE_LOOP('',(#4633,#4634,#4635,#4636,#4637,#4638));
#1401=EDGE_LOOP('',(#4639,#4640,#4641,#4642,#4643,#4644));
#1402=EDGE_LOOP('',(#4645,#4646,#4647,#4648,#4649,#4650));
#1403=EDGE_LOOP('',(#4651,#4652,#4653,#4654,#4655,#4656));
#1404=EDGE_LOOP('',(#4657,#4658,#4659,#4660,#4661,#4662));
#1405=EDGE_LOOP('',(#4663,#4664,#4665,#4666,#4667,#4668));
#1406=EDGE_LOOP('',(#4669,#4670,#4671,#4672,#4673,#4674));
#1407=EDGE_LOOP('',(#4675,#4676,#4677,#4678,#4679,#4680));
#1408=EDGE_LOOP('',(#4681,#4682,#4683,#4684,#4685,#4686));
#1409=EDGE_LOOP('',(#4687,#4688,#4689,#4690,#4691,#4692));
#1410=EDGE_LOOP('',(#4693,#4694,#4695,#4696,#4697,#4698));
#1411=EDGE_LOOP('',(#4699,#4700,#4701,#4702,#4703,#4704));
#1412=EDGE_LOOP('',(#4705,#4706,#4707,#4708,#4709,#4710));
#1413=EDGE_LOOP('',(#4711,#4712,#4713,#4714,#4715,#4716));
#1414=EDGE_LOOP('',(#4717,#4718,#4719,#4720,#4721,#4722));
#1415=EDGE_LOOP('',(#4723,#4724,#4725,#4726,#4727,#4728));
#1416=EDGE_LOOP('',(#4729,#4730,#4731,#4732,#4733,#4734));
#1417=EDGE_LOOP('',(#4735,#4736,#4737,#4738,#4739,#4740));
#1418=EDGE_LOOP('',(#4741,#4742,#4743,#4744,#4745,#4746));
#1419=EDGE_LOOP('',(#4747,#4748,#4749,#4750,#4751,#4752));
#1420=EDGE_LOOP('',(#4753,#4754,#4755,#4756,#4757,#4758));
#1421=EDGE_LOOP('',(#4759,#4760,#4761,#4762,#4763,#4764));
#1422=EDGE_LOOP('',(#4765,#4766,#4767,#4768,#4769,#4770));
#1423=EDGE_LOOP('',(#4771,#4772,#4773,#4774,#4775,#4776));
#1424=EDGE_LOOP('',(#4777,#4778,#4779,#4780,#4781,#4782));
#1425=EDGE_LOOP('',(#4783,#4784,#4785,#4786,#4787,#4788));
#1426=EDGE_LOOP('',(#4789,#4790,#4791,#4792,#4793,#4794));
#1427=EDGE_LOOP('',(#4795,#4796,#4797,#4798,#4799,#4800));
#1428=EDGE_LOOP('',(#4801,#4802,#4803,#4804,#4805,#4806));
#1429=EDGE_LOOP('',(#4807,#4808,#4809,#4810,#4811,#4812));
#1430=EDGE_LOOP('',(#4813,#4814,#4815,#4816,#4817,#4818));
#1431=EDGE_LOOP('',(#4819,#4820,#4821,#4822,#4823,#4824));
#1432=EDGE_LOOP('',(#4825,#4826,#4827,#4828,#4829,#4830));
#1433=EDGE_LOOP('',(#4831,#4832,#4833,#4834,#4835,#4836));
#1434=EDGE_LOOP('',(#4837,#4838,#4839,#4840,#4841,#4842));
#1435=EDGE_LOOP('',(#4843,#4844,#4845,#4846,#4847,#4848));
#1436=EDGE_LOOP('',(#4849,#4850,#4851,#4852,#4853,#4854));
#1437=EDGE_LOOP('',(#4855,#4856,#4857,#4858,#4859,#4860));
#1438=EDGE_LOOP('',(#4861,#4862,#4863,#4864,#4865,#4866));
#1439=EDGE_LOOP('',(#4867,#4868,#4869,#4870,#4871,#4872));
#1440=EDGE_LOOP('',(#4873,#4874,#4875,#4876,#4877,#4878));
#1441=EDGE_LOOP('',(#4879,#4880,#4881,#4882,#4883,#4884));
#1442=EDGE_LOOP('',(#4885,#4886,#4887,#4888,#4889,#4890));
#1443=EDGE_LOOP('',(#4891,#4892,#4893,#4894,#4895,#4896));
#1444=EDGE_LOOP('',(#4897,#4898,#4899,#4900,#4901,#4902));
#1445=EDGE_LOOP('',(#4903,#4904,#4905,#4906,#4907,#4908));
#1446=EDGE_LOOP('',(#4909,#4910,#4911,#4912,#4913,#4914));
#1447=EDGE_LOOP('',(#4915,#4916,#4917,#4918,#4919,#4920));
#1448=EDGE_LOOP('',(#4921,#4922,#4923,#4924,#4925,#4926));
#1449=EDGE_LOOP('',(#4927,#4928,#4929,#4930,#4931,#4932));
#1450=EDGE_LOOP('',(#4933,#4934,#4935,#4936,#4937,#4938));
#1451=EDGE_LOOP('',(#4939,#4940,#4941,#4942,#4943,#4944));
#1452=EDGE_LOOP('',(#4945,#4946,#4947,#4948,#4949,#4950));
#1453=EDGE_LOOP('',(#4951,#4952,#4953,#4954,#4955,#4956));
#1454=EDGE_LOOP('',(#4957,#4958,#4959,#4960,#4961,#4962));
#1455=EDGE_LOOP('',(#4963,#4964,#4965,#4966,#4967,#4968));
#1456=EDGE_LOOP('',(#4969,#4970,#4971,#4972,#4973,#4974));
#1457=EDGE_LOOP('',(#4975,#4976,#4977,#4978,#4979,#4980));
#1458=EDGE_LOOP('',(#4981,#4982,#4983,#4984,#4985,#4986));
#1459=EDGE_LOOP('',(#4987,#4988,#4989,#4990,#4991,#4992));
#1460=EDGE_LOOP('',(#4993,#4994,#4995,#4996,#4997,#4998,#4999,#5000,#5001,
#5002,#5003,#5004,#5005,#5006,#5007,#5008,#5009,#5010,#5011,#5012,#5013,
#5014,#5015,#5016,#5017,#5018,#5019,#5020,#5021,#5022,#5023,#5024,#5025,
#5026,#5027,#5028,#5029,#5030,#5031,#5032,#5033,#5034,#5035,#5036,#5037,
#5038,#5039,#5040,#5041,#5042,#5043,#5044,#5045,#5046,#5047,#5048,#5049,
#5050,#5051,#5052,#5053,#5054,#5055,#5056,#5057,#5058,#5059,#5060,#5061,
#5062,#5063,#5064,#5065,#5066,#5067,#5068,#5069,#5070,#5071,#5072,#5073,
#5074,#5075,#5076,#5077,#5078,#5079,#5080,#5081,#5082,#5083,#5084,#5085,
#5086,#5087,#5088,#5089,#5090,#5091,#5092,#5093,#5094,#5095,#5096,#5097,
#5098,#5099,#5100,#5101,#5102,#5103,#5104,#5105,#5106,#5107,#5108,#5109,
#5110,#5111,#5112,#5113,#5114,#5115,#5116,#5117,#5118,#5119,#5120,#5121,
#5122,#5123,#5124,#5125,#5126,#5127,#5128,#5129,#5130,#5131,#5132,#5133,
#5134,#5135));
#1461=EDGE_LOOP('',(#5136,#5137,#5138,#5139));
#1462=EDGE_LOOP('',(#5140));
#1463=EDGE_LOOP('',(#5141));
#1464=EDGE_LOOP('',(#5142));
#1465=EDGE_LOOP('',(#5143));
#1466=EDGE_LOOP('',(#5144,#5145,#5146,#5147));
#1467=EDGE_LOOP('',(#5148,#5149,#5150,#5151));
#1468=EDGE_LOOP('',(#5152));
#1469=EDGE_LOOP('',(#5153));
#1470=EDGE_LOOP('',(#5154,#5155,#5156,#5157));
#1471=EDGE_LOOP('',(#5158,#5159,#5160,#5161));
#1472=EDGE_LOOP('',(#5162));
#1473=EDGE_LOOP('',(#5163));
#1474=EDGE_LOOP('',(#5164,#5165,#5166,#5167));
#1475=EDGE_LOOP('',(#5168,#5169,#5170,#5171));
#1476=EDGE_LOOP('',(#5172,#5173,#5174,#5175));
#1477=EDGE_LOOP('',(#5176,#5177,#5178,#5179));
#1478=EDGE_LOOP('',(#5180,#5181,#5182,#5183));
#1479=EDGE_LOOP('',(#5184,#5185,#5186,#5187,#5188,#5189,#5190,#5191,#5192,
#5193,#5194,#5195,#5196,#5197,#5198,#5199,#5200,#5201,#5202,#5203,#5204,
#5205,#5206,#5207,#5208,#5209,#5210,#5211,#5212,#5213,#5214,#5215,#5216,
#5217,#5218,#5219,#5220,#5221,#5222,#5223,#5224,#5225,#5226,#5227,#5228,
#5229,#5230,#5231,#5232,#5233,#5234,#5235,#5236,#5237,#5238,#5239,#5240,
#5241,#5242,#5243,#5244,#5245,#5246,#5247,#5248,#5249,#5250,#5251,#5252,
#5253,#5254,#5255,#5256,#5257,#5258,#5259,#5260,#5261,#5262,#5263,#5264,
#5265,#5266,#5267,#5268,#5269,#5270,#5271,#5272,#5273,#5274,#5275,#5276,
#5277,#5278,#5279,#5280,#5281,#5282,#5283,#5284,#5285,#5286,#5287,#5288,
#5289,#5290,#5291,#5292,#5293,#5294,#5295,#5296,#5297,#5298,#5299,#5300,
#5301,#5302,#5303,#5304,#5305,#5306,#5307,#5308,#5309,#5310,#5311,#5312,
#5313,#5314,#5315,#5316,#5317,#5318,#5319,#5320,#5321,#5322,#5323,#5324,
#5325,#5326,#5327,#5328,#5329,#5330,#5331,#5332,#5333,#5334,#5335,#5336,
#5337,#5338,#5339,#5340,#5341,#5342,#5343,#5344,#5345,#5346,#5347,#5348,
#5349,#5350,#5351,#5352,#5353,#5354,#5355,#5356,#5357,#5358,#5359,#5360,
#5361,#5362,#5363,#5364,#5365,#5366,#5367,#5368,#5369,#5370,#5371,#5372,
#5373,#5374,#5375,#5376,#5377,#5378,#5379,#5380,#5381,#5382,#5383,#5384,
#5385,#5386,#5387,#5388,#5389,#5390,#5391,#5392,#5393,#5394,#5395,#5396,
#5397,#5398,#5399,#5400,#5401,#5402,#5403,#5404));
#1480=EDGE_LOOP('',(#5405,#5406,#5407,#5408,#5409,#5410,#5411,#5412,#5413,
#5414,#5415,#5416,#5417,#5418,#5419,#5420,#5421,#5422,#5423,#5424,#5425,
#5426,#5427,#5428,#5429,#5430,#5431,#5432,#5433,#5434,#5435,#5436,#5437,
#5438,#5439,#5440,#5441,#5442,#5443,#5444,#5445,#5446,#5447,#5448,#5449,
#5450,#5451,#5452,#5453,#5454,#5455,#5456,#5457,#5458,#5459,#5460,#5461,
#5462,#5463,#5464,#5465,#5466,#5467,#5468,#5469,#5470,#5471,#5472,#5473,
#5474,#5475,#5476,#5477,#5478,#5479,#5480,#5481,#5482,#5483,#5484,#5485,
#5486,#5487,#5488,#5489,#5490,#5491,#5492,#5493,#5494,#5495,#5496,#5497,
#5498,#5499,#5500,#5501,#5502,#5503,#5504,#5505,#5506,#5507,#5508,#5509,
#5510,#5511,#5512,#5513,#5514,#5515,#5516,#5517,#5518,#5519,#5520,#5521,
#5522,#5523,#5524,#5525,#5526,#5527,#5528,#5529,#5530,#5531,#5532,#5533,
#5534,#5535,#5536,#5537,#5538,#5539,#5540,#5541,#5542,#5543,#5544,#5545,
#5546,#5547,#5548,#5549,#5550,#5551,#5552,#5553,#5554,#5555,#5556,#5557,
#5558,#5559,#5560,#5561,#5562,#5563,#5564,#5565,#5566,#5567,#5568,#5569,
#5570,#5571,#5572,#5573,#5574,#5575,#5576,#5577,#5578,#5579,#5580,#5581,
#5582,#5583,#5584,#5585,#5586,#5587,#5588,#5589,#5590,#5591,#5592,#5593,
#5594,#5595,#5596,#5597,#5598,#5599,#5600,#5601,#5602,#5603,#5604,#5605,
#5606,#5607,#5608,#5609,#5610,#5611,#5612,#5613,#5614,#5615,#5616,#5617,
#5618,#5619,#5620,#5621,#5622,#5623,#5624,#5625,#5626,#5627,#5628,#5629,
#5630,#5631,#5632,#5633,#5634,#5635,#5636,#5637,#5638,#5639,#5640));
#1481=EDGE_LOOP('',(#5641,#5642,#5643,#5644));
#1482=EDGE_LOOP('',(#5645,#5646,#5647,#5648));
#1483=EDGE_LOOP('',(#5649,#5650,#5651,#5652));
#1484=EDGE_LOOP('',(#5653,#5654,#5655,#5656));
#1485=EDGE_LOOP('',(#5657,#5658,#5659,#5660));
#1486=EDGE_LOOP('',(#5661,#5662,#5663,#5664));
#1487=EDGE_LOOP('',(#5665,#5666,#5667,#5668,#5669,#5670));
#1488=EDGE_LOOP('',(#5671));
#1489=EDGE_LOOP('',(#5672,#5673,#5674,#5675));
#1490=EDGE_LOOP('',(#5676));
#1491=EDGE_LOOP('',(#5677));
#1492=EDGE_LOOP('',(#5678));
#1493=EDGE_LOOP('',(#5679));
#1494=EDGE_LOOP('',(#5680,#5681,#5682,#5683));
#1495=EDGE_LOOP('',(#5684));
#1496=EDGE_LOOP('',(#5685,#5686,#5687,#5688,#5689,#5690));
#1497=EDGE_LOOP('',(#5691));
#1498=EDGE_LOOP('',(#5692));
#1499=EDGE_LOOP('',(#5693));
#1500=EDGE_LOOP('',(#5694));
#1703=LINE('',#8943,#1983);
#1704=LINE('',#9159,#1984);
#1705=LINE('',#9655,#1985);
#1706=LINE('',#10157,#1986);
#1707=LINE('',#10668,#1987);
#1708=LINE('',#11161,#1988);
#1709=LINE('',#11654,#1989);
#1710=LINE('',#12153,#1990);
#1711=LINE('',#12652,#1991);
#1712=LINE('',#13142,#1992);
#1713=LINE('',#13629,#1993);
#1714=LINE('',#14134,#1994);
#1715=LINE('',#14639,#1995);
#1716=LINE('',#15141,#1996);
#1717=LINE('',#15637,#1997);
#1718=LINE('',#16130,#1998);
#1719=LINE('',#16620,#1999);
#1720=LINE('',#17122,#2000);
#1721=LINE('',#17636,#2001);
#1722=LINE('',#18135,#2002);
#1723=LINE('',#18622,#2003);
#1724=LINE('',#19115,#2004);
#1725=LINE('',#19623,#2005);
#1726=LINE('',#20122,#2006);
#1727=LINE('',#20624,#2007);
#1728=LINE('',#21111,#2008);
#1729=LINE('',#21595,#2009);
#1730=LINE('',#22097,#2010);
#1731=LINE('',#22605,#2011);
#1732=LINE('',#23113,#2012);
#1733=LINE('',#23597,#2013);
#1734=LINE('',#24090,#2014);
#1735=LINE('',#24601,#2015);
#1736=LINE('',#25112,#2016);
#1737=LINE('',#25608,#2017);
#1738=LINE('',#26089,#2018);
#1739=LINE('',#26588,#2019);
#1740=LINE('',#27087,#2020);
#1741=LINE('',#27583,#2021);
#1742=LINE('',#28100,#2022);
#1743=LINE('',#28584,#2023);
#1744=LINE('',#29077,#2024);
#1745=LINE('',#29579,#2025);
#1746=LINE('',#30078,#2026);
#1747=LINE('',#30565,#2027);
#1748=LINE('',#30898,#2028);
#1749=LINE('',#31336,#2029);
#1750=LINE('',#31832,#2030);
#1751=LINE('',#32334,#2031);
#1752=LINE('',#32836,#2032);
#1753=LINE('',#33338,#2033);
#1754=LINE('',#33834,#2034);
#1755=LINE('',#34336,#2035);
#1756=LINE('',#34838,#2036);
#1757=LINE('',#35325,#2037);
#1758=LINE('',#35830,#2038);
#1759=LINE('',#36332,#2039);
#1760=LINE('',#36822,#2040);
#1761=LINE('',#37309,#2041);
#1762=LINE('',#37811,#2042);
#1763=LINE('',#38322,#2043);
#1764=LINE('',#38818,#2044);
#1765=LINE('',#39308,#2045);
#1766=LINE('',#39798,#2046);
#1767=LINE('',#40297,#2047);
#1768=LINE('',#40796,#2048);
#1769=LINE('',#41289,#2049);
#1770=LINE('',#41782,#2050);
#1771=LINE('',#42287,#2051);
#1772=LINE('',#42780,#2052);
#1773=LINE('',#43288,#2053);
#1774=LINE('',#43787,#2054);
#1775=LINE('',#44274,#2055);
#1776=LINE('',#44773,#2056);
#1777=LINE('',#45269,#2057);
#1778=LINE('',#45771,#2058);
#1779=LINE('',#46273,#2059);
#1780=LINE('',#66984,#2060);
#1781=LINE('',#66995,#2061);
#1782=LINE('',#66998,#2062);
#1783=LINE('',#67012,#2063);
#1784=LINE('',#67018,#2064);
#1785=LINE('',#67024,#2065);
#1786=LINE('',#67030,#2066);
#1787=LINE('',#67036,#2067);
#1788=LINE('',#71828,#2068);
#1789=LINE('',#71830,#2069);
#1790=LINE('',#71832,#2070);
#1791=LINE('',#71833,#2071);
#1792=LINE('',#71836,#2072);
#1793=LINE('',#71838,#2073);
#1794=LINE('',#71839,#2074);
#1795=LINE('',#71842,#2075);
#1796=LINE('',#71844,#2076);
#1797=LINE('',#71845,#2077);
#1798=LINE('',#71848,#2078);
#1799=LINE('',#71850,#2079);
#1800=LINE('',#71851,#2080);
#1801=LINE('',#71854,#2081);
#1802=LINE('',#71856,#2082);
#1803=LINE('',#71857,#2083);
#1804=LINE('',#71859,#2084);
#1805=LINE('',#71860,#2085);
#1806=LINE('',#71867,#2086);
#1983=VECTOR('',#7884,6.767);
#1984=VECTOR('',#7889,6.767);
#1985=VECTOR('',#7892,6.767);
#1986=VECTOR('',#7895,6.767);
#1987=VECTOR('',#7898,6.767);
#1988=VECTOR('',#7901,6.767);
#1989=VECTOR('',#7904,6.767);
#1990=VECTOR('',#7907,6.767);
#1991=VECTOR('',#7910,6.767);
#1992=VECTOR('',#7913,6.767);
#1993=VECTOR('',#7916,6.767);
#1994=VECTOR('',#7919,6.767);
#1995=VECTOR('',#7922,6.767);
#1996=VECTOR('',#7925,6.767);
#1997=VECTOR('',#7928,6.767);
#1998=VECTOR('',#7931,6.767);
#1999=VECTOR('',#7934,6.767);
#2000=VECTOR('',#7937,6.767);
#2001=VECTOR('',#7940,6.767);
#2002=VECTOR('',#7943,6.767);
#2003=VECTOR('',#7946,6.767);
#2004=VECTOR('',#7949,6.767);
#2005=VECTOR('',#7952,6.767);
#2006=VECTOR('',#7955,6.767);
#2007=VECTOR('',#7958,6.767);
#2008=VECTOR('',#7961,6.767);
#2009=VECTOR('',#7964,6.767);
#2010=VECTOR('',#7967,6.767);
#2011=VECTOR('',#7970,6.767);
#2012=VECTOR('',#7973,6.767);
#2013=VECTOR('',#7976,6.767);
#2014=VECTOR('',#7979,6.767);
#2015=VECTOR('',#7982,6.767);
#2016=VECTOR('',#7985,6.767);
#2017=VECTOR('',#7988,6.767);
#2018=VECTOR('',#7991,6.767);
#2019=VECTOR('',#7994,6.767);
#2020=VECTOR('',#7997,6.767);
#2021=VECTOR('',#8000,6.767);
#2022=VECTOR('',#8003,6.767);
#2023=VECTOR('',#8006,6.767);
#2024=VECTOR('',#8009,6.767);
#2025=VECTOR('',#8012,6.767);
#2026=VECTOR('',#8015,6.767);
#2027=VECTOR('',#8018,6.767);
#2028=VECTOR('',#8021,6.767);
#2029=VECTOR('',#8024,6.767);
#2030=VECTOR('',#8027,6.767);
#2031=VECTOR('',#8030,6.767);
#2032=VECTOR('',#8033,6.767);
#2033=VECTOR('',#8036,6.767);
#2034=VECTOR('',#8039,6.767);
#2035=VECTOR('',#8042,6.767);
#2036=VECTOR('',#8045,6.767);
#2037=VECTOR('',#8048,6.767);
#2038=VECTOR('',#8051,6.767);
#2039=VECTOR('',#8054,6.767);
#2040=VECTOR('',#8057,6.767);
#2041=VECTOR('',#8060,6.767);
#2042=VECTOR('',#8063,6.767);
#2043=VECTOR('',#8066,6.767);
#2044=VECTOR('',#8069,6.767);
#2045=VECTOR('',#8072,6.767);
#2046=VECTOR('',#8075,6.767);
#2047=VECTOR('',#8078,6.767);
#2048=VECTOR('',#8081,6.767);
#2049=VECTOR('',#8084,6.767);
#2050=VECTOR('',#8087,6.767);
#2051=VECTOR('',#8090,6.767);
#2052=VECTOR('',#8093,6.767);
#2053=VECTOR('',#8096,6.767);
#2054=VECTOR('',#8099,6.767);
#2055=VECTOR('',#8102,6.767);
#2056=VECTOR('',#8105,6.767);
#2057=VECTOR('',#8108,6.767);
#2058=VECTOR('',#8111,6.767);
#2059=VECTOR('',#8114,6.767);
#2060=VECTOR('',#8129,4.);
#2061=VECTOR('',#8144,5.);
#2062=VECTOR('',#8147,5.);
#2063=VECTOR('',#8166,10.);
#2064=VECTOR('',#8173,8.);
#2065=VECTOR('',#8180,8.);
#2066=VECTOR('',#8187,8.);
#2067=VECTOR('',#8194,8.);
#2068=VECTOR('',#8201,10.);
#2069=VECTOR('',#8202,10.);
#2070=VECTOR('',#8203,10.);
#2071=VECTOR('',#8204,10.);
#2072=VECTOR('',#8207,10.);
#2073=VECTOR('',#8208,10.);
#2074=VECTOR('',#8209,10.);
#2075=VECTOR('',#8212,10.);
#2076=VECTOR('',#8213,10.);
#2077=VECTOR('',#8214,10.);
#2078=VECTOR('',#8217,10.);
#2079=VECTOR('',#8218,10.);
#2080=VECTOR('',#8219,10.);
#2081=VECTOR('',#8222,10.);
#2082=VECTOR('',#8223,10.);
#2083=VECTOR('',#8224,10.);
#2084=VECTOR('',#8227,10.);
#2085=VECTOR('',#8228,10.);
#2086=VECTOR('',#8237,45.);
#2250=CIRCLE('',#7400,6.767);
#2251=CIRCLE('',#7478,6.767);
#2252=CIRCLE('',#7480,7.911);
#2253=CIRCLE('',#7481,7.911);
#2254=CIRCLE('',#7483,4.);
#2255=CIRCLE('',#7484,4.);
#2256=CIRCLE('',#7486,5.);
#2257=CIRCLE('',#7488,5.);
#2258=CIRCLE('',#7490,5.);
#2259=CIRCLE('',#7492,5.);
#2260=CIRCLE('',#7495,10.);
#2261=CIRCLE('',#7496,7.);
#2262=CIRCLE('',#7500,10.);
#2263=CIRCLE('',#7503,8.);
#2264=CIRCLE('',#7504,8.);
#2265=CIRCLE('',#7506,8.);
#2266=CIRCLE('',#7507,8.);
#2267=CIRCLE('',#7509,8.);
#2268=CIRCLE('',#7510,8.);
#2269=CIRCLE('',#7512,8.);
#2270=CIRCLE('',#7513,8.);
#2271=CIRCLE('',#7523,45.);
#2272=CIRCLE('',#7525,45.);
#2364=VERTEX_POINT('',#8941);
#2365=VERTEX_POINT('',#8942);
#2366=VERTEX_POINT('',#8944);
#2367=VERTEX_POINT('',#9078);
#2368=VERTEX_POINT('',#9157);
#2369=VERTEX_POINT('',#9158);
#2370=VERTEX_POINT('',#9160);
#2371=VERTEX_POINT('',#9403);
#2372=VERTEX_POINT('',#9653);
#2373=VERTEX_POINT('',#9654);
#2374=VERTEX_POINT('',#9656);
#2375=VERTEX_POINT('',#9899);
#2376=VERTEX_POINT('',#10155);
#2377=VERTEX_POINT('',#10156);
#2378=VERTEX_POINT('',#10158);
#2379=VERTEX_POINT('',#10413);
#2380=VERTEX_POINT('',#10666);
#2381=VERTEX_POINT('',#10667);
#2382=VERTEX_POINT('',#10669);
#2383=VERTEX_POINT('',#10906);
#2384=VERTEX_POINT('',#11159);
#2385=VERTEX_POINT('',#11160);
#2386=VERTEX_POINT('',#11162);
#2387=VERTEX_POINT('',#11411);
#2388=VERTEX_POINT('',#11652);
#2389=VERTEX_POINT('',#11653);
#2390=VERTEX_POINT('',#11655);
#2391=VERTEX_POINT('',#11907);
#2392=VERTEX_POINT('',#12151);
#2393=VERTEX_POINT('',#12152);
#2394=VERTEX_POINT('',#12154);
#2395=VERTEX_POINT('',#12406);
#2396=VERTEX_POINT('',#12650);
#2397=VERTEX_POINT('',#12651);
#2398=VERTEX_POINT('',#12653);
#2399=VERTEX_POINT('',#12893);
#2400=VERTEX_POINT('',#13140);
#2401=VERTEX_POINT('',#13141);
#2402=VERTEX_POINT('',#13143);
#2403=VERTEX_POINT('',#13386);
#2404=VERTEX_POINT('',#13627);
#2405=VERTEX_POINT('',#13628);
#2406=VERTEX_POINT('',#13630);
#2407=VERTEX_POINT('',#13885);
#2408=VERTEX_POINT('',#14132);
#2409=VERTEX_POINT('',#14133);
#2410=VERTEX_POINT('',#14135);
#2411=VERTEX_POINT('',#14378);
#2412=VERTEX_POINT('',#14637);
#2413=VERTEX_POINT('',#14638);
#2414=VERTEX_POINT('',#14640);
#2415=VERTEX_POINT('',#14883);
#2416=VERTEX_POINT('',#15139);
#2417=VERTEX_POINT('',#15140);
#2418=VERTEX_POINT('',#15142);
#2419=VERTEX_POINT('',#15382);
#2420=VERTEX_POINT('',#15635);
#2421=VERTEX_POINT('',#15636);
#2422=VERTEX_POINT('',#15638);
#2423=VERTEX_POINT('',#15887);
#2424=VERTEX_POINT('',#16128);
#2425=VERTEX_POINT('',#16129);
#2426=VERTEX_POINT('',#16131);
#2427=VERTEX_POINT('',#16371);
#2428=VERTEX_POINT('',#16618);
#2429=VERTEX_POINT('',#16619);
#2430=VERTEX_POINT('',#16621);
#2431=VERTEX_POINT('',#16867);
#2432=VERTEX_POINT('',#17120);
#2433=VERTEX_POINT('',#17121);
#2434=VERTEX_POINT('',#17123);
#2435=VERTEX_POINT('',#17381);
#2436=VERTEX_POINT('',#17634);
#2437=VERTEX_POINT('',#17635);
#2438=VERTEX_POINT('',#17637);
#2439=VERTEX_POINT('',#17877);
#2440=VERTEX_POINT('',#18133);
#2441=VERTEX_POINT('',#18134);
#2442=VERTEX_POINT('',#18136);
#2443=VERTEX_POINT('',#18379);
#2444=VERTEX_POINT('',#18620);
#2445=VERTEX_POINT('',#18621);
#2446=VERTEX_POINT('',#18623);
#2447=VERTEX_POINT('',#18866);
#2448=VERTEX_POINT('',#19113);
#2449=VERTEX_POINT('',#19114);
#2450=VERTEX_POINT('',#19116);
#2451=VERTEX_POINT('',#19362);
#2452=VERTEX_POINT('',#19621);
#2453=VERTEX_POINT('',#19622);
#2454=VERTEX_POINT('',#19624);
#2455=VERTEX_POINT('',#19864);
#2456=VERTEX_POINT('',#20120);
#2457=VERTEX_POINT('',#20121);
#2458=VERTEX_POINT('',#20123);
#2459=VERTEX_POINT('',#20369);
#2460=VERTEX_POINT('',#20622);
#2461=VERTEX_POINT('',#20623);
#2462=VERTEX_POINT('',#20625);
#2463=VERTEX_POINT('',#20868);
#2464=VERTEX_POINT('',#21109);
#2465=VERTEX_POINT('',#21110);
#2466=VERTEX_POINT('',#21112);
#2467=VERTEX_POINT('',#21346);
#2468=VERTEX_POINT('',#21593);
#2469=VERTEX_POINT('',#21594);
#2470=VERTEX_POINT('',#21596);
#2471=VERTEX_POINT('',#21842);
#2472=VERTEX_POINT('',#22095);
#2473=VERTEX_POINT('',#22096);
#2474=VERTEX_POINT('',#22098);
#2475=VERTEX_POINT('',#22350);
#2476=VERTEX_POINT('',#22603);
#2477=VERTEX_POINT('',#22604);
#2478=VERTEX_POINT('',#22606);
#2479=VERTEX_POINT('',#22855);
#2480=VERTEX_POINT('',#23111);
#2481=VERTEX_POINT('',#23112);
#2482=VERTEX_POINT('',#23114);
#2483=VERTEX_POINT('',#23354);
#2484=VERTEX_POINT('',#23595);
#2485=VERTEX_POINT('',#23596);
#2486=VERTEX_POINT('',#23598);
#2487=VERTEX_POINT('',#23841);
#2488=VERTEX_POINT('',#24088);
#2489=VERTEX_POINT('',#24089);
#2490=VERTEX_POINT('',#24091);
#2491=VERTEX_POINT('',#24346);
#2492=VERTEX_POINT('',#24599);
#2493=VERTEX_POINT('',#24600);
#2494=VERTEX_POINT('',#24602);
#2495=VERTEX_POINT('',#24854);
#2496=VERTEX_POINT('',#25110);
#2497=VERTEX_POINT('',#25111);
#2498=VERTEX_POINT('',#25113);
#2499=VERTEX_POINT('',#25365);
#2500=VERTEX_POINT('',#25606);
#2501=VERTEX_POINT('',#25607);
#2502=VERTEX_POINT('',#25609);
#2503=VERTEX_POINT('',#25852);
#2504=VERTEX_POINT('',#26087);
#2505=VERTEX_POINT('',#26088);
#2506=VERTEX_POINT('',#26090);
#2507=VERTEX_POINT('',#26339);
#2508=VERTEX_POINT('',#26586);
#2509=VERTEX_POINT('',#26587);
#2510=VERTEX_POINT('',#26589);
#2511=VERTEX_POINT('',#26841);
#2512=VERTEX_POINT('',#27085);
#2513=VERTEX_POINT('',#27086);
#2514=VERTEX_POINT('',#27088);
#2515=VERTEX_POINT('',#27337);
#2516=VERTEX_POINT('',#27581);
#2517=VERTEX_POINT('',#27582);
#2518=VERTEX_POINT('',#27584);
#2519=VERTEX_POINT('',#27839);
#2520=VERTEX_POINT('',#28098);
#2521=VERTEX_POINT('',#28099);
#2522=VERTEX_POINT('',#28101);
#2523=VERTEX_POINT('',#28341);
#2524=VERTEX_POINT('',#28582);
#2525=VERTEX_POINT('',#28583);
#2526=VERTEX_POINT('',#28585);
#2527=VERTEX_POINT('',#28831);
#2528=VERTEX_POINT('',#29075);
#2529=VERTEX_POINT('',#29076);
#2530=VERTEX_POINT('',#29078);
#2531=VERTEX_POINT('',#29333);
#2532=VERTEX_POINT('',#29577);
#2533=VERTEX_POINT('',#29578);
#2534=VERTEX_POINT('',#29580);
#2535=VERTEX_POINT('',#29829);
#2536=VERTEX_POINT('',#30076);
#2537=VERTEX_POINT('',#30077);
#2538=VERTEX_POINT('',#30079);
#2539=VERTEX_POINT('',#30322);
#2540=VERTEX_POINT('',#30563);
#2541=VERTEX_POINT('',#30564);
#2542=VERTEX_POINT('',#30566);
#2543=VERTEX_POINT('',#30809);
#2544=VERTEX_POINT('',#30896);
#2545=VERTEX_POINT('',#30897);
#2546=VERTEX_POINT('',#30899);
#2547=VERTEX_POINT('',#31154);
#2548=VERTEX_POINT('',#31334);
#2549=VERTEX_POINT('',#31335);
#2550=VERTEX_POINT('',#31337);
#2551=VERTEX_POINT('',#31589);
#2552=VERTEX_POINT('',#31830);
#2553=VERTEX_POINT('',#31831);
#2554=VERTEX_POINT('',#31833);
#2555=VERTEX_POINT('',#32085);
#2556=VERTEX_POINT('',#32332);
#2557=VERTEX_POINT('',#32333);
#2558=VERTEX_POINT('',#32335);
#2559=VERTEX_POINT('',#32578);
#2560=VERTEX_POINT('',#32834);
#2561=VERTEX_POINT('',#32835);
#2562=VERTEX_POINT('',#32837);
#2563=VERTEX_POINT('',#33086);
#2564=VERTEX_POINT('',#33336);
#2565=VERTEX_POINT('',#33337);
#2566=VERTEX_POINT('',#33339);
#2567=VERTEX_POINT('',#33591);
#2568=VERTEX_POINT('',#33832);
#2569=VERTEX_POINT('',#33833);
#2570=VERTEX_POINT('',#33835);
#2571=VERTEX_POINT('',#34087);
#2572=VERTEX_POINT('',#34334);
#2573=VERTEX_POINT('',#34335);
#2574=VERTEX_POINT('',#34337);
#2575=VERTEX_POINT('',#34580);
#2576=VERTEX_POINT('',#34836);
#2577=VERTEX_POINT('',#34837);
#2578=VERTEX_POINT('',#34839);
#2579=VERTEX_POINT('',#35085);
#2580=VERTEX_POINT('',#35323);
#2581=VERTEX_POINT('',#35324);
#2582=VERTEX_POINT('',#35326);
#2583=VERTEX_POINT('',#35578);
#2584=VERTEX_POINT('',#35828);
#2585=VERTEX_POINT('',#35829);
#2586=VERTEX_POINT('',#35831);
#2587=VERTEX_POINT('',#36086);
#2588=VERTEX_POINT('',#36330);
#2589=VERTEX_POINT('',#36331);
#2590=VERTEX_POINT('',#36333);
#2591=VERTEX_POINT('',#36585);
#2592=VERTEX_POINT('',#36820);
#2593=VERTEX_POINT('',#36821);
#2594=VERTEX_POINT('',#36823);
#2595=VERTEX_POINT('',#37060);
#2596=VERTEX_POINT('',#37307);
#2597=VERTEX_POINT('',#37308);
#2598=VERTEX_POINT('',#37310);
#2599=VERTEX_POINT('',#37556);
#2600=VERTEX_POINT('',#37809);
#2601=VERTEX_POINT('',#37810);
#2602=VERTEX_POINT('',#37812);
#2603=VERTEX_POINT('',#38067);
#2604=VERTEX_POINT('',#38320);
#2605=VERTEX_POINT('',#38321);
#2606=VERTEX_POINT('',#38323);
#2607=VERTEX_POINT('',#38575);
#2608=VERTEX_POINT('',#38816);
#2609=VERTEX_POINT('',#38817);
#2610=VERTEX_POINT('',#38819);
#2611=VERTEX_POINT('',#39059);
#2612=VERTEX_POINT('',#39306);
#2613=VERTEX_POINT('',#39307);
#2614=VERTEX_POINT('',#39309);
#2615=VERTEX_POINT('',#39543);
#2616=VERTEX_POINT('',#39796);
#2617=VERTEX_POINT('',#39797);
#2618=VERTEX_POINT('',#39799);
#2619=VERTEX_POINT('',#40045);
#2620=VERTEX_POINT('',#40295);
#2621=VERTEX_POINT('',#40296);
#2622=VERTEX_POINT('',#40298);
#2623=VERTEX_POINT('',#40538);
#2624=VERTEX_POINT('',#40794);
#2625=VERTEX_POINT('',#40795);
#2626=VERTEX_POINT('',#40797);
#2627=VERTEX_POINT('',#41043);
#2628=VERTEX_POINT('',#41287);
#2629=VERTEX_POINT('',#41288);
#2630=VERTEX_POINT('',#41290);
#2631=VERTEX_POINT('',#41530);
#2632=VERTEX_POINT('',#41780);
#2633=VERTEX_POINT('',#41781);
#2634=VERTEX_POINT('',#41783);
#2635=VERTEX_POINT('',#42032);
#2636=VERTEX_POINT('',#42285);
#2637=VERTEX_POINT('',#42286);
#2638=VERTEX_POINT('',#42288);
#2639=VERTEX_POINT('',#42528);
#2640=VERTEX_POINT('',#42778);
#2641=VERTEX_POINT('',#42779);
#2642=VERTEX_POINT('',#42781);
#2643=VERTEX_POINT('',#43030);
#2644=VERTEX_POINT('',#43286);
#2645=VERTEX_POINT('',#43287);
#2646=VERTEX_POINT('',#43289);
#2647=VERTEX_POINT('',#43544);
#2648=VERTEX_POINT('',#43785);
#2649=VERTEX_POINT('',#43786);
#2650=VERTEX_POINT('',#43788);
#2651=VERTEX_POINT('',#44025);
#2652=VERTEX_POINT('',#44272);
#2653=VERTEX_POINT('',#44273);
#2654=VERTEX_POINT('',#44275);
#2655=VERTEX_POINT('',#44518);
#2656=VERTEX_POINT('',#44771);
#2657=VERTEX_POINT('',#44772);
#2658=VERTEX_POINT('',#44774);
#2659=VERTEX_POINT('',#45017);
#2660=VERTEX_POINT('',#45267);
#2661=VERTEX_POINT('',#45268);
#2662=VERTEX_POINT('',#45270);
#2663=VERTEX_POINT('',#45516);
#2664=VERTEX_POINT('',#45769);
#2665=VERTEX_POINT('',#45770);
#2666=VERTEX_POINT('',#45772);
#2667=VERTEX_POINT('',#46027);
#2668=VERTEX_POINT('',#46271);
#2669=VERTEX_POINT('',#46272);
#2670=VERTEX_POINT('',#46274);
#2671=VERTEX_POINT('',#46529);
#2672=VERTEX_POINT('',#46776);
#2673=VERTEX_POINT('',#46859);
#2674=VERTEX_POINT('',#46942);
#2675=VERTEX_POINT('',#46944);
#2676=VERTEX_POINT('',#47065);
#2677=VERTEX_POINT('',#47066);
#2678=VERTEX_POINT('',#47075);
#2679=VERTEX_POINT('',#47077);
#2680=VERTEX_POINT('',#47121);
#2681=VERTEX_POINT('',#47384);
#2682=VERTEX_POINT('',#47403);
#2683=VERTEX_POINT('',#47669);
#2684=VERTEX_POINT('',#47688);
#2685=VERTEX_POINT('',#47707);
#2686=VERTEX_POINT('',#47719);
#2687=VERTEX_POINT('',#47738);
#2688=VERTEX_POINT('',#47750);
#2689=VERTEX_POINT('',#47769);
#2690=VERTEX_POINT('',#47788);
#2691=VERTEX_POINT('',#47807);
#2692=VERTEX_POINT('',#47826);
#2693=VERTEX_POINT('',#47837);
#2694=VERTEX_POINT('',#47856);
#2695=VERTEX_POINT('',#48119);
#2696=VERTEX_POINT('',#48138);
#2697=VERTEX_POINT('',#48401);
#2698=VERTEX_POINT('',#48415);
#2699=VERTEX_POINT('',#48434);
#2700=VERTEX_POINT('',#48453);
#2701=VERTEX_POINT('',#48472);
#2702=VERTEX_POINT('',#48738);
#2703=VERTEX_POINT('',#48757);
#2704=VERTEX_POINT('',#48769);
#2705=VERTEX_POINT('',#48788);
#2706=VERTEX_POINT('',#48807);
#2707=VERTEX_POINT('',#48819);
#2708=VERTEX_POINT('',#48832);
#2709=VERTEX_POINT('',#49098);
#2710=VERTEX_POINT('',#49117);
#2711=VERTEX_POINT('',#49380);
#2712=VERTEX_POINT('',#49399);
#2713=VERTEX_POINT('',#49418);
#2714=VERTEX_POINT('',#49684);
#2715=VERTEX_POINT('',#49703);
#2716=VERTEX_POINT('',#49715);
#2717=VERTEX_POINT('',#49981);
#2718=VERTEX_POINT('',#49993);
#2719=VERTEX_POINT('',#50012);
#2720=VERTEX_POINT('',#50031);
#2721=VERTEX_POINT('',#50043);
#2722=VERTEX_POINT('',#50056);
#2723=VERTEX_POINT('',#50322);
#2724=VERTEX_POINT('',#50341);
#2725=VERTEX_POINT('',#50604);
#2726=VERTEX_POINT('',#50623);
#2727=VERTEX_POINT('',#50635);
#2728=VERTEX_POINT('',#50877);
#2729=VERTEX_POINT('',#50896);
#2730=VERTEX_POINT('',#50908);
#2731=VERTEX_POINT('',#51174);
#2732=VERTEX_POINT('',#51186);
#2733=VERTEX_POINT('',#51205);
#2734=VERTEX_POINT('',#51224);
#2735=VERTEX_POINT('',#51490);
#2736=VERTEX_POINT('',#51509);
#2737=VERTEX_POINT('',#51772);
#2738=VERTEX_POINT('',#51791);
#2739=VERTEX_POINT('',#52057);
#2740=VERTEX_POINT('',#52071);
#2741=VERTEX_POINT('',#52083);
#2742=VERTEX_POINT('',#52102);
#2743=VERTEX_POINT('',#52121);
#2744=VERTEX_POINT('',#52133);
#2745=VERTEX_POINT('',#52152);
#2746=VERTEX_POINT('',#52418);
#2747=VERTEX_POINT('',#52437);
#2748=VERTEX_POINT('',#52456);
#2749=VERTEX_POINT('',#52475);
#2750=VERTEX_POINT('',#52488);
#2751=VERTEX_POINT('',#52751);
#2752=VERTEX_POINT('',#52770);
#2753=VERTEX_POINT('',#52782);
#2754=VERTEX_POINT('',#52801);
#2755=VERTEX_POINT('',#53064);
#2756=VERTEX_POINT('',#53083);
#2757=VERTEX_POINT('',#53092);
#2758=VERTEX_POINT('',#53094);
#2759=VERTEX_POINT('',#53101);
#2760=VERTEX_POINT('',#53113);
#2761=VERTEX_POINT('',#53702);
#2762=VERTEX_POINT('',#53968);
#2763=VERTEX_POINT('',#53987);
#2764=VERTEX_POINT('',#54253);
#2765=VERTEX_POINT('',#54272);
#2766=VERTEX_POINT('',#54284);
#2767=VERTEX_POINT('',#54550);
#2768=VERTEX_POINT('',#54562);
#2769=VERTEX_POINT('',#55155);
#2770=VERTEX_POINT('',#55421);
#2771=VERTEX_POINT('',#55654);
#2772=VERTEX_POINT('',#56245);
#2773=VERTEX_POINT('',#56264);
#2774=VERTEX_POINT('',#56530);
#2775=VERTEX_POINT('',#57105);
#2776=VERTEX_POINT('',#57124);
#2777=VERTEX_POINT('',#57143);
#2778=VERTEX_POINT('',#57155);
#2779=VERTEX_POINT('',#57174);
#2780=VERTEX_POINT('',#57437);
#2781=VERTEX_POINT('',#58042);
#2782=VERTEX_POINT('',#58643);
#2783=VERTEX_POINT('',#58655);
#2784=VERTEX_POINT('',#59216);
#2785=VERTEX_POINT('',#59482);
#2786=VERTEX_POINT('',#59501);
#2787=VERTEX_POINT('',#59764);
#2788=VERTEX_POINT('',#60341);
#2789=VERTEX_POINT('',#60958);
#2790=VERTEX_POINT('',#61221);
#2791=VERTEX_POINT('',#61240);
#2792=VERTEX_POINT('',#61252);
#2793=VERTEX_POINT('',#61841);
#2794=VERTEX_POINT('',#62408);
#2795=VERTEX_POINT('',#62674);
#2796=VERTEX_POINT('',#62693);
#2797=VERTEX_POINT('',#63266);
#2798=VERTEX_POINT('',#63285);
#2799=VERTEX_POINT('',#63551);
#2800=VERTEX_POINT('',#64116);
#2801=VERTEX_POINT('',#64128);
#2802=VERTEX_POINT('',#64394);
#2803=VERTEX_POINT('',#64406);
#2804=VERTEX_POINT('',#64425);
#2805=VERTEX_POINT('',#64691);
#2806=VERTEX_POINT('',#64710);
#2807=VERTEX_POINT('',#64976);
#2808=VERTEX_POINT('',#65218);
#2809=VERTEX_POINT('',#65237);
#2810=VERTEX_POINT('',#65249);
#2811=VERTEX_POINT('',#65515);
#2812=VERTEX_POINT('',#65527);
#2813=VERTEX_POINT('',#65546);
#2814=VERTEX_POINT('',#65565);
#2815=VERTEX_POINT('',#65577);
#2816=VERTEX_POINT('',#65596);
#2817=VERTEX_POINT('',#65608);
#2818=VERTEX_POINT('',#65847);
#2819=VERTEX_POINT('',#66981);
#2820=VERTEX_POINT('',#66983);
#2821=VERTEX_POINT('',#66987);
#2822=VERTEX_POINT('',#66990);
#2823=VERTEX_POINT('',#66993);
#2824=VERTEX_POINT('',#66997);
#2825=VERTEX_POINT('',#67002);
#2826=VERTEX_POINT('',#67004);
#2827=VERTEX_POINT('',#67005);
#2828=VERTEX_POINT('',#67010);
#2829=VERTEX_POINT('',#67015);
#2830=VERTEX_POINT('',#67017);
#2831=VERTEX_POINT('',#67021);
#2832=VERTEX_POINT('',#67023);
#2833=VERTEX_POINT('',#67027);
#2834=VERTEX_POINT('',#67029);
#2835=VERTEX_POINT('',#67033);
#2836=VERTEX_POINT('',#67035);
#2837=VERTEX_POINT('',#71826);
#2838=VERTEX_POINT('',#71827);
#2839=VERTEX_POINT('',#71829);
#2840=VERTEX_POINT('',#71831);
#2841=VERTEX_POINT('',#71835);
#2842=VERTEX_POINT('',#71837);
#2843=VERTEX_POINT('',#71841);
#2844=VERTEX_POINT('',#71843);
#2845=VERTEX_POINT('',#71847);
#2846=VERTEX_POINT('',#71849);
#2847=VERTEX_POINT('',#71853);
#2848=VERTEX_POINT('',#71855);
#2849=VERTEX_POINT('',#71863);
#2850=VERTEX_POINT('',#71866);
#3308=EDGE_CURVE('',#2364,#2365,#1703,.T.);
#3309=EDGE_CURVE('',#2366,#2364,#109,.T.);
#3310=EDGE_CURVE('',#2367,#2366,#2250,.T.);
#3311=EDGE_CURVE('',#2367,#2365,#110,.T.);
#3312=EDGE_CURVE('',#2368,#2369,#1704,.T.);
#3313=EDGE_CURVE('',#2370,#2368,#111,.T.);
#3314=EDGE_CURVE('',#2364,#2370,#112,.T.);
#3315=EDGE_CURVE('',#2365,#2371,#113,.T.);
#3316=EDGE_CURVE('',#2371,#2369,#114,.T.);
#3317=EDGE_CURVE('',#2372,#2373,#1705,.T.);
#3318=EDGE_CURVE('',#2374,#2372,#115,.T.);
#3319=EDGE_CURVE('',#2368,#2374,#116,.T.);
#3320=EDGE_CURVE('',#2369,#2375,#117,.T.);
#3321=EDGE_CURVE('',#2375,#2373,#118,.T.);
#3322=EDGE_CURVE('',#2376,#2377,#1706,.T.);
#3323=EDGE_CURVE('',#2378,#2376,#119,.T.);
#3324=EDGE_CURVE('',#2372,#2378,#120,.T.);
#3325=EDGE_CURVE('',#2373,#2379,#121,.T.);
#3326=EDGE_CURVE('',#2379,#2377,#122,.T.);
#3327=EDGE_CURVE('',#2380,#2381,#1707,.T.);
#3328=EDGE_CURVE('',#2382,#2380,#123,.T.);
#3329=EDGE_CURVE('',#2376,#2382,#124,.T.);
#3330=EDGE_CURVE('',#2377,#2383,#125,.T.);
#3331=EDGE_CURVE('',#2383,#2381,#126,.T.);
#3332=EDGE_CURVE('',#2384,#2385,#1708,.T.);
#3333=EDGE_CURVE('',#2386,#2384,#127,.T.);
#3334=EDGE_CURVE('',#2380,#2386,#128,.T.);
#3335=EDGE_CURVE('',#2381,#2387,#129,.T.);
#3336=EDGE_CURVE('',#2387,#2385,#130,.T.);
#3337=EDGE_CURVE('',#2388,#2389,#1709,.T.);
#3338=EDGE_CURVE('',#2390,#2388,#131,.T.);
#3339=EDGE_CURVE('',#2384,#2390,#132,.T.);
#3340=EDGE_CURVE('',#2385,#2391,#133,.T.);
#3341=EDGE_CURVE('',#2391,#2389,#134,.T.);
#3342=EDGE_CURVE('',#2392,#2393,#1710,.T.);
#3343=EDGE_CURVE('',#2394,#2392,#135,.T.);
#3344=EDGE_CURVE('',#2388,#2394,#136,.T.);
#3345=EDGE_CURVE('',#2389,#2395,#137,.T.);
#3346=EDGE_CURVE('',#2395,#2393,#138,.T.);
#3347=EDGE_CURVE('',#2396,#2397,#1711,.T.);
#3348=EDGE_CURVE('',#2398,#2396,#139,.T.);
#3349=EDGE_CURVE('',#2392,#2398,#140,.T.);
#3350=EDGE_CURVE('',#2393,#2399,#141,.T.);
#3351=EDGE_CURVE('',#2399,#2397,#142,.T.);
#3352=EDGE_CURVE('',#2400,#2401,#1712,.T.);
#3353=EDGE_CURVE('',#2402,#2400,#143,.T.);
#3354=EDGE_CURVE('',#2396,#2402,#144,.T.);
#3355=EDGE_CURVE('',#2397,#2403,#145,.T.);
#3356=EDGE_CURVE('',#2403,#2401,#146,.T.);
#3357=EDGE_CURVE('',#2404,#2405,#1713,.T.);
#3358=EDGE_CURVE('',#2406,#2404,#147,.T.);
#3359=EDGE_CURVE('',#2400,#2406,#148,.T.);
#3360=EDGE_CURVE('',#2401,#2407,#149,.T.);
#3361=EDGE_CURVE('',#2407,#2405,#150,.T.);
#3362=EDGE_CURVE('',#2408,#2409,#1714,.T.);
#3363=EDGE_CURVE('',#2410,#2408,#151,.T.);
#3364=EDGE_CURVE('',#2404,#2410,#152,.T.);
#3365=EDGE_CURVE('',#2405,#2411,#153,.T.);
#3366=EDGE_CURVE('',#2411,#2409,#154,.T.);
#3367=EDGE_CURVE('',#2412,#2413,#1715,.T.);
#3368=EDGE_CURVE('',#2414,#2412,#155,.T.);
#3369=EDGE_CURVE('',#2408,#2414,#156,.T.);
#3370=EDGE_CURVE('',#2409,#2415,#157,.T.);
#3371=EDGE_CURVE('',#2415,#2413,#158,.T.);
#3372=EDGE_CURVE('',#2416,#2417,#1716,.T.);
#3373=EDGE_CURVE('',#2418,#2416,#159,.T.);
#3374=EDGE_CURVE('',#2412,#2418,#160,.T.);
#3375=EDGE_CURVE('',#2413,#2419,#161,.T.);
#3376=EDGE_CURVE('',#2419,#2417,#162,.T.);
#3377=EDGE_CURVE('',#2420,#2421,#1717,.T.);
#3378=EDGE_CURVE('',#2422,#2420,#163,.T.);
#3379=EDGE_CURVE('',#2416,#2422,#164,.T.);
#3380=EDGE_CURVE('',#2417,#2423,#165,.T.);
#3381=EDGE_CURVE('',#2423,#2421,#166,.T.);
#3382=EDGE_CURVE('',#2424,#2425,#1718,.T.);
#3383=EDGE_CURVE('',#2426,#2424,#167,.T.);
#3384=EDGE_CURVE('',#2420,#2426,#168,.T.);
#3385=EDGE_CURVE('',#2421,#2427,#169,.T.);
#3386=EDGE_CURVE('',#2427,#2425,#170,.T.);
#3387=EDGE_CURVE('',#2428,#2429,#1719,.T.);
#3388=EDGE_CURVE('',#2430,#2428,#171,.T.);
#3389=EDGE_CURVE('',#2424,#2430,#172,.T.);
#3390=EDGE_CURVE('',#2425,#2431,#173,.T.);
#3391=EDGE_CURVE('',#2431,#2429,#174,.T.);
#3392=EDGE_CURVE('',#2432,#2433,#1720,.T.);
#3393=EDGE_CURVE('',#2434,#2432,#175,.T.);
#3394=EDGE_CURVE('',#2428,#2434,#176,.T.);
#3395=EDGE_CURVE('',#2429,#2435,#177,.T.);
#3396=EDGE_CURVE('',#2435,#2433,#178,.T.);
#3397=EDGE_CURVE('',#2436,#2437,#1721,.T.);
#3398=EDGE_CURVE('',#2438,#2436,#179,.T.);
#3399=EDGE_CURVE('',#2432,#2438,#180,.T.);
#3400=EDGE_CURVE('',#2433,#2439,#181,.T.);
#3401=EDGE_CURVE('',#2439,#2437,#182,.T.);
#3402=EDGE_CURVE('',#2440,#2441,#1722,.T.);
#3403=EDGE_CURVE('',#2442,#2440,#183,.T.);
#3404=EDGE_CURVE('',#2436,#2442,#184,.T.);
#3405=EDGE_CURVE('',#2437,#2443,#185,.T.);
#3406=EDGE_CURVE('',#2443,#2441,#186,.T.);
#3407=EDGE_CURVE('',#2444,#2445,#1723,.T.);
#3408=EDGE_CURVE('',#2446,#2444,#187,.T.);
#3409=EDGE_CURVE('',#2440,#2446,#188,.T.);
#3410=EDGE_CURVE('',#2441,#2447,#189,.T.);
#3411=EDGE_CURVE('',#2447,#2445,#190,.T.);
#3412=EDGE_CURVE('',#2448,#2449,#1724,.T.);
#3413=EDGE_CURVE('',#2450,#2448,#191,.T.);
#3414=EDGE_CURVE('',#2444,#2450,#192,.T.);
#3415=EDGE_CURVE('',#2445,#2451,#193,.T.);
#3416=EDGE_CURVE('',#2451,#2449,#194,.T.);
#3417=EDGE_CURVE('',#2452,#2453,#1725,.T.);
#3418=EDGE_CURVE('',#2454,#2452,#195,.T.);
#3419=EDGE_CURVE('',#2448,#2454,#196,.T.);
#3420=EDGE_CURVE('',#2449,#2455,#197,.T.);
#3421=EDGE_CURVE('',#2455,#2453,#198,.T.);
#3422=EDGE_CURVE('',#2456,#2457,#1726,.T.);
#3423=EDGE_CURVE('',#2458,#2456,#199,.T.);
#3424=EDGE_CURVE('',#2452,#2458,#200,.T.);
#3425=EDGE_CURVE('',#2453,#2459,#201,.T.);
#3426=EDGE_CURVE('',#2459,#2457,#202,.T.);
#3427=EDGE_CURVE('',#2460,#2461,#1727,.T.);
#3428=EDGE_CURVE('',#2462,#2460,#203,.T.);
#3429=EDGE_CURVE('',#2456,#2462,#204,.T.);
#3430=EDGE_CURVE('',#2457,#2463,#205,.T.);
#3431=EDGE_CURVE('',#2463,#2461,#206,.T.);
#3432=EDGE_CURVE('',#2464,#2465,#1728,.T.);
#3433=EDGE_CURVE('',#2466,#2464,#207,.T.);
#3434=EDGE_CURVE('',#2460,#2466,#208,.T.);
#3435=EDGE_CURVE('',#2461,#2467,#209,.T.);
#3436=EDGE_CURVE('',#2467,#2465,#210,.T.);
#3437=EDGE_CURVE('',#2468,#2469,#1729,.T.);
#3438=EDGE_CURVE('',#2470,#2468,#211,.T.);
#3439=EDGE_CURVE('',#2464,#2470,#212,.T.);
#3440=EDGE_CURVE('',#2465,#2471,#213,.T.);
#3441=EDGE_CURVE('',#2471,#2469,#214,.T.);
#3442=EDGE_CURVE('',#2472,#2473,#1730,.T.);
#3443=EDGE_CURVE('',#2474,#2472,#215,.T.);
#3444=EDGE_CURVE('',#2468,#2474,#216,.T.);
#3445=EDGE_CURVE('',#2469,#2475,#217,.T.);
#3446=EDGE_CURVE('',#2475,#2473,#218,.T.);
#3447=EDGE_CURVE('',#2476,#2477,#1731,.T.);
#3448=EDGE_CURVE('',#2478,#2476,#219,.T.);
#3449=EDGE_CURVE('',#2472,#2478,#220,.T.);
#3450=EDGE_CURVE('',#2473,#2479,#221,.T.);
#3451=EDGE_CURVE('',#2479,#2477,#222,.T.);
#3452=EDGE_CURVE('',#2480,#2481,#1732,.T.);
#3453=EDGE_CURVE('',#2482,#2480,#223,.T.);
#3454=EDGE_CURVE('',#2476,#2482,#224,.T.);
#3455=EDGE_CURVE('',#2477,#2483,#225,.T.);
#3456=EDGE_CURVE('',#2483,#2481,#226,.T.);
#3457=EDGE_CURVE('',#2484,#2485,#1733,.T.);
#3458=EDGE_CURVE('',#2486,#2484,#227,.T.);
#3459=EDGE_CURVE('',#2480,#2486,#228,.T.);
#3460=EDGE_CURVE('',#2481,#2487,#229,.T.);
#3461=EDGE_CURVE('',#2487,#2485,#230,.T.);
#3462=EDGE_CURVE('',#2488,#2489,#1734,.T.);
#3463=EDGE_CURVE('',#2490,#2488,#231,.T.);
#3464=EDGE_CURVE('',#2484,#2490,#232,.T.);
#3465=EDGE_CURVE('',#2485,#2491,#233,.T.);
#3466=EDGE_CURVE('',#2491,#2489,#234,.T.);
#3467=EDGE_CURVE('',#2492,#2493,#1735,.T.);
#3468=EDGE_CURVE('',#2494,#2492,#235,.T.);
#3469=EDGE_CURVE('',#2488,#2494,#236,.T.);
#3470=EDGE_CURVE('',#2489,#2495,#237,.T.);
#3471=EDGE_CURVE('',#2495,#2493,#238,.T.);
#3472=EDGE_CURVE('',#2496,#2497,#1736,.T.);
#3473=EDGE_CURVE('',#2498,#2496,#239,.T.);
#3474=EDGE_CURVE('',#2492,#2498,#240,.T.);
#3475=EDGE_CURVE('',#2493,#2499,#241,.T.);
#3476=EDGE_CURVE('',#2499,#2497,#242,.T.);
#3477=EDGE_CURVE('',#2500,#2501,#1737,.T.);
#3478=EDGE_CURVE('',#2502,#2500,#243,.T.);
#3479=EDGE_CURVE('',#2496,#2502,#244,.T.);
#3480=EDGE_CURVE('',#2497,#2503,#245,.T.);
#3481=EDGE_CURVE('',#2503,#2501,#246,.T.);
#3482=EDGE_CURVE('',#2504,#2505,#1738,.T.);
#3483=EDGE_CURVE('',#2506,#2504,#247,.T.);
#3484=EDGE_CURVE('',#2500,#2506,#248,.T.);
#3485=EDGE_CURVE('',#2501,#2507,#249,.T.);
#3486=EDGE_CURVE('',#2507,#2505,#250,.T.);
#3487=EDGE_CURVE('',#2508,#2509,#1739,.T.);
#3488=EDGE_CURVE('',#2510,#2508,#251,.T.);
#3489=EDGE_CURVE('',#2504,#2510,#252,.T.);
#3490=EDGE_CURVE('',#2505,#2511,#253,.T.);
#3491=EDGE_CURVE('',#2511,#2509,#254,.T.);
#3492=EDGE_CURVE('',#2512,#2513,#1740,.T.);
#3493=EDGE_CURVE('',#2514,#2512,#255,.T.);
#3494=EDGE_CURVE('',#2508,#2514,#256,.T.);
#3495=EDGE_CURVE('',#2509,#2515,#257,.T.);
#3496=EDGE_CURVE('',#2515,#2513,#258,.T.);
#3497=EDGE_CURVE('',#2516,#2517,#1741,.T.);
#3498=EDGE_CURVE('',#2518,#2516,#259,.T.);
#3499=EDGE_CURVE('',#2512,#2518,#260,.T.);
#3500=EDGE_CURVE('',#2513,#2519,#261,.T.);
#3501=EDGE_CURVE('',#2519,#2517,#262,.T.);
#3502=EDGE_CURVE('',#2520,#2521,#1742,.T.);
#3503=EDGE_CURVE('',#2522,#2520,#263,.T.);
#3504=EDGE_CURVE('',#2516,#2522,#264,.T.);
#3505=EDGE_CURVE('',#2517,#2523,#265,.T.);
#3506=EDGE_CURVE('',#2523,#2521,#266,.T.);
#3507=EDGE_CURVE('',#2524,#2525,#1743,.T.);
#3508=EDGE_CURVE('',#2526,#2524,#267,.T.);
#3509=EDGE_CURVE('',#2520,#2526,#268,.T.);
#3510=EDGE_CURVE('',#2521,#2527,#269,.T.);
#3511=EDGE_CURVE('',#2527,#2525,#270,.T.);
#3512=EDGE_CURVE('',#2528,#2529,#1744,.T.);
#3513=EDGE_CURVE('',#2530,#2528,#271,.T.);
#3514=EDGE_CURVE('',#2524,#2530,#272,.T.);
#3515=EDGE_CURVE('',#2525,#2531,#273,.T.);
#3516=EDGE_CURVE('',#2531,#2529,#274,.T.);
#3517=EDGE_CURVE('',#2532,#2533,#1745,.T.);
#3518=EDGE_CURVE('',#2534,#2532,#275,.T.);
#3519=EDGE_CURVE('',#2528,#2534,#276,.T.);
#3520=EDGE_CURVE('',#2529,#2535,#277,.T.);
#3521=EDGE_CURVE('',#2535,#2533,#278,.T.);
#3522=EDGE_CURVE('',#2536,#2537,#1746,.T.);
#3523=EDGE_CURVE('',#2538,#2536,#279,.T.);
#3524=EDGE_CURVE('',#2532,#2538,#280,.T.);
#3525=EDGE_CURVE('',#2533,#2539,#281,.T.);
#3526=EDGE_CURVE('',#2539,#2537,#282,.T.);
#3527=EDGE_CURVE('',#2540,#2541,#1747,.T.);
#3528=EDGE_CURVE('',#2542,#2540,#283,.T.);
#3529=EDGE_CURVE('',#2536,#2542,#284,.T.);
#3530=EDGE_CURVE('',#2537,#2543,#285,.T.);
#3531=EDGE_CURVE('',#2543,#2541,#286,.T.);
#3532=EDGE_CURVE('',#2544,#2545,#1748,.T.);
#3533=EDGE_CURVE('',#2546,#2544,#287,.T.);
#3534=EDGE_CURVE('',#2540,#2546,#288,.T.);
#3535=EDGE_CURVE('',#2541,#2547,#289,.T.);
#3536=EDGE_CURVE('',#2547,#2545,#290,.T.);
#3537=EDGE_CURVE('',#2548,#2549,#1749,.T.);
#3538=EDGE_CURVE('',#2550,#2548,#291,.T.);
#3539=EDGE_CURVE('',#2544,#2550,#292,.T.);
#3540=EDGE_CURVE('',#2545,#2551,#293,.T.);
#3541=EDGE_CURVE('',#2551,#2549,#294,.T.);
#3542=EDGE_CURVE('',#2552,#2553,#1750,.T.);
#3543=EDGE_CURVE('',#2554,#2552,#295,.T.);
#3544=EDGE_CURVE('',#2548,#2554,#296,.T.);
#3545=EDGE_CURVE('',#2549,#2555,#297,.T.);
#3546=EDGE_CURVE('',#2555,#2553,#298,.T.);
#3547=EDGE_CURVE('',#2556,#2557,#1751,.T.);
#3548=EDGE_CURVE('',#2558,#2556,#299,.T.);
#3549=EDGE_CURVE('',#2552,#2558,#300,.T.);
#3550=EDGE_CURVE('',#2553,#2559,#301,.T.);
#3551=EDGE_CURVE('',#2559,#2557,#302,.T.);
#3552=EDGE_CURVE('',#2560,#2561,#1752,.T.);
#3553=EDGE_CURVE('',#2562,#2560,#303,.T.);
#3554=EDGE_CURVE('',#2556,#2562,#304,.T.);
#3555=EDGE_CURVE('',#2557,#2563,#305,.T.);
#3556=EDGE_CURVE('',#2563,#2561,#306,.T.);
#3557=EDGE_CURVE('',#2564,#2565,#1753,.T.);
#3558=EDGE_CURVE('',#2566,#2564,#307,.T.);
#3559=EDGE_CURVE('',#2560,#2566,#308,.T.);
#3560=EDGE_CURVE('',#2561,#2567,#309,.T.);
#3561=EDGE_CURVE('',#2567,#2565,#310,.T.);
#3562=EDGE_CURVE('',#2568,#2569,#1754,.T.);
#3563=EDGE_CURVE('',#2570,#2568,#311,.T.);
#3564=EDGE_CURVE('',#2564,#2570,#312,.T.);
#3565=EDGE_CURVE('',#2565,#2571,#313,.T.);
#3566=EDGE_CURVE('',#2571,#2569,#314,.T.);
#3567=EDGE_CURVE('',#2572,#2573,#1755,.T.);
#3568=EDGE_CURVE('',#2574,#2572,#315,.T.);
#3569=EDGE_CURVE('',#2568,#2574,#316,.T.);
#3570=EDGE_CURVE('',#2569,#2575,#317,.T.);
#3571=EDGE_CURVE('',#2575,#2573,#318,.T.);
#3572=EDGE_CURVE('',#2576,#2577,#1756,.T.);
#3573=EDGE_CURVE('',#2578,#2576,#319,.T.);
#3574=EDGE_CURVE('',#2572,#2578,#320,.T.);
#3575=EDGE_CURVE('',#2573,#2579,#321,.T.);
#3576=EDGE_CURVE('',#2579,#2577,#322,.T.);
#3577=EDGE_CURVE('',#2580,#2581,#1757,.T.);
#3578=EDGE_CURVE('',#2582,#2580,#323,.T.);
#3579=EDGE_CURVE('',#2576,#2582,#324,.T.);
#3580=EDGE_CURVE('',#2577,#2583,#325,.T.);
#3581=EDGE_CURVE('',#2583,#2581,#326,.T.);
#3582=EDGE_CURVE('',#2584,#2585,#1758,.T.);
#3583=EDGE_CURVE('',#2586,#2584,#327,.T.);
#3584=EDGE_CURVE('',#2580,#2586,#328,.T.);
#3585=EDGE_CURVE('',#2581,#2587,#329,.T.);
#3586=EDGE_CURVE('',#2587,#2585,#330,.T.);
#3587=EDGE_CURVE('',#2588,#2589,#1759,.T.);
#3588=EDGE_CURVE('',#2590,#2588,#331,.T.);
#3589=EDGE_CURVE('',#2584,#2590,#332,.T.);
#3590=EDGE_CURVE('',#2585,#2591,#333,.T.);
#3591=EDGE_CURVE('',#2591,#2589,#334,.T.);
#3592=EDGE_CURVE('',#2592,#2593,#1760,.T.);
#3593=EDGE_CURVE('',#2594,#2592,#335,.T.);
#3594=EDGE_CURVE('',#2588,#2594,#336,.T.);
#3595=EDGE_CURVE('',#2589,#2595,#337,.T.);
#3596=EDGE_CURVE('',#2595,#2593,#338,.T.);
#3597=EDGE_CURVE('',#2596,#2597,#1761,.T.);
#3598=EDGE_CURVE('',#2598,#2596,#339,.T.);
#3599=EDGE_CURVE('',#2592,#2598,#340,.T.);
#3600=EDGE_CURVE('',#2593,#2599,#341,.T.);
#3601=EDGE_CURVE('',#2599,#2597,#342,.T.);
#3602=EDGE_CURVE('',#2600,#2601,#1762,.T.);
#3603=EDGE_CURVE('',#2602,#2600,#343,.T.);
#3604=EDGE_CURVE('',#2596,#2602,#344,.T.);
#3605=EDGE_CURVE('',#2597,#2603,#345,.T.);
#3606=EDGE_CURVE('',#2603,#2601,#346,.T.);
#3607=EDGE_CURVE('',#2604,#2605,#1763,.T.);
#3608=EDGE_CURVE('',#2606,#2604,#347,.T.);
#3609=EDGE_CURVE('',#2600,#2606,#348,.T.);
#3610=EDGE_CURVE('',#2601,#2607,#349,.T.);
#3611=EDGE_CURVE('',#2607,#2605,#350,.T.);
#3612=EDGE_CURVE('',#2608,#2609,#1764,.T.);
#3613=EDGE_CURVE('',#2610,#2608,#351,.T.);
#3614=EDGE_CURVE('',#2604,#2610,#352,.T.);
#3615=EDGE_CURVE('',#2605,#2611,#353,.T.);
#3616=EDGE_CURVE('',#2611,#2609,#354,.T.);
#3617=EDGE_CURVE('',#2612,#2613,#1765,.T.);
#3618=EDGE_CURVE('',#2614,#2612,#355,.T.);
#3619=EDGE_CURVE('',#2608,#2614,#356,.T.);
#3620=EDGE_CURVE('',#2609,#2615,#357,.T.);
#3621=EDGE_CURVE('',#2615,#2613,#358,.T.);
#3622=EDGE_CURVE('',#2616,#2617,#1766,.T.);
#3623=EDGE_CURVE('',#2618,#2616,#359,.T.);
#3624=EDGE_CURVE('',#2612,#2618,#360,.T.);
#3625=EDGE_CURVE('',#2613,#2619,#361,.T.);
#3626=EDGE_CURVE('',#2619,#2617,#362,.T.);
#3627=EDGE_CURVE('',#2620,#2621,#1767,.T.);
#3628=EDGE_CURVE('',#2622,#2620,#363,.T.);
#3629=EDGE_CURVE('',#2616,#2622,#364,.T.);
#3630=EDGE_CURVE('',#2617,#2623,#365,.T.);
#3631=EDGE_CURVE('',#2623,#2621,#366,.T.);
#3632=EDGE_CURVE('',#2624,#2625,#1768,.T.);
#3633=EDGE_CURVE('',#2626,#2624,#367,.T.);
#3634=EDGE_CURVE('',#2620,#2626,#368,.T.);
#3635=EDGE_CURVE('',#2621,#2627,#369,.T.);
#3636=EDGE_CURVE('',#2627,#2625,#370,.T.);
#3637=EDGE_CURVE('',#2628,#2629,#1769,.T.);
#3638=EDGE_CURVE('',#2630,#2628,#371,.T.);
#3639=EDGE_CURVE('',#2624,#2630,#372,.T.);
#3640=EDGE_CURVE('',#2625,#2631,#373,.T.);
#3641=EDGE_CURVE('',#2631,#2629,#374,.T.);
#3642=EDGE_CURVE('',#2632,#2633,#1770,.T.);
#3643=EDGE_CURVE('',#2634,#2632,#375,.T.);
#3644=EDGE_CURVE('',#2628,#2634,#376,.T.);
#3645=EDGE_CURVE('',#2629,#2635,#377,.T.);
#3646=EDGE_CURVE('',#2635,#2633,#378,.T.);
#3647=EDGE_CURVE('',#2636,#2637,#1771,.T.);
#3648=EDGE_CURVE('',#2638,#2636,#379,.T.);
#3649=EDGE_CURVE('',#2632,#2638,#380,.T.);
#3650=EDGE_CURVE('',#2633,#2639,#381,.T.);
#3651=EDGE_CURVE('',#2639,#2637,#382,.T.);
#3652=EDGE_CURVE('',#2640,#2641,#1772,.T.);
#3653=EDGE_CURVE('',#2642,#2640,#383,.T.);
#3654=EDGE_CURVE('',#2636,#2642,#384,.T.);
#3655=EDGE_CURVE('',#2637,#2643,#385,.T.);
#3656=EDGE_CURVE('',#2643,#2641,#386,.T.);
#3657=EDGE_CURVE('',#2644,#2645,#1773,.T.);
#3658=EDGE_CURVE('',#2646,#2644,#387,.T.);
#3659=EDGE_CURVE('',#2640,#2646,#388,.T.);
#3660=EDGE_CURVE('',#2641,#2647,#389,.T.);
#3661=EDGE_CURVE('',#2647,#2645,#390,.T.);
#3662=EDGE_CURVE('',#2648,#2649,#1774,.T.);
#3663=EDGE_CURVE('',#2650,#2648,#391,.T.);
#3664=EDGE_CURVE('',#2644,#2650,#392,.T.);
#3665=EDGE_CURVE('',#2645,#2651,#393,.T.);
#3666=EDGE_CURVE('',#2651,#2649,#394,.T.);
#3667=EDGE_CURVE('',#2652,#2653,#1775,.T.);
#3668=EDGE_CURVE('',#2654,#2652,#395,.T.);
#3669=EDGE_CURVE('',#2648,#2654,#396,.T.);
#3670=EDGE_CURVE('',#2649,#2655,#397,.T.);
#3671=EDGE_CURVE('',#2655,#2653,#398,.T.);
#3672=EDGE_CURVE('',#2656,#2657,#1776,.T.);
#3673=EDGE_CURVE('',#2658,#2656,#399,.T.);
#3674=EDGE_CURVE('',#2652,#2658,#400,.T.);
#3675=EDGE_CURVE('',#2653,#2659,#401,.T.);
#3676=EDGE_CURVE('',#2659,#2657,#402,.T.);
#3677=EDGE_CURVE('',#2660,#2661,#1777,.T.);
#3678=EDGE_CURVE('',#2662,#2660,#403,.T.);
#3679=EDGE_CURVE('',#2656,#2662,#404,.T.);
#3680=EDGE_CURVE('',#2657,#2663,#405,.T.);
#3681=EDGE_CURVE('',#2663,#2661,#406,.T.);
#3682=EDGE_CURVE('',#2664,#2665,#1778,.T.);
#3683=EDGE_CURVE('',#2666,#2664,#407,.T.);
#3684=EDGE_CURVE('',#2660,#2666,#408,.T.);
#3685=EDGE_CURVE('',#2661,#2667,#409,.T.);
#3686=EDGE_CURVE('',#2667,#2665,#410,.T.);
#3687=EDGE_CURVE('',#2668,#2669,#1779,.T.);
#3688=EDGE_CURVE('',#2670,#2668,#411,.T.);
#3689=EDGE_CURVE('',#2664,#2670,#412,.T.);
#3690=EDGE_CURVE('',#2665,#2671,#413,.T.);
#3691=EDGE_CURVE('',#2671,#2669,#414,.T.);
#3692=EDGE_CURVE('',#2669,#2672,#415,.T.);
#3693=EDGE_CURVE('',#2672,#2673,#416,.T.);
#3694=EDGE_CURVE('',#2674,#2673,#2251,.T.);
#3695=EDGE_CURVE('',#2675,#2674,#417,.T.);
#3696=EDGE_CURVE('',#2668,#2675,#418,.T.);
#3697=EDGE_CURVE('',#2676,#2677,#419,.T.);
#3698=EDGE_CURVE('',#2677,#2678,#2252,.F.);
#3699=EDGE_CURVE('',#2678,#2679,#420,.T.);
#3700=EDGE_CURVE('',#2679,#2680,#421,.T.);
#3701=EDGE_CURVE('',#2680,#2681,#422,.T.);
#3702=EDGE_CURVE('',#2681,#2682,#423,.T.);
#3703=EDGE_CURVE('',#2682,#2683,#424,.T.);
#3704=EDGE_CURVE('',#2683,#2684,#425,.T.);
#3705=EDGE_CURVE('',#2684,#2685,#426,.T.);
#3706=EDGE_CURVE('',#2685,#2686,#427,.T.);
#3707=EDGE_CURVE('',#2686,#2687,#428,.T.);
#3708=EDGE_CURVE('',#2687,#2688,#429,.T.);
#3709=EDGE_CURVE('',#2688,#2689,#430,.T.);
#3710=EDGE_CURVE('',#2689,#2690,#431,.T.);
#3711=EDGE_CURVE('',#2690,#2691,#432,.T.);
#3712=EDGE_CURVE('',#2691,#2692,#433,.T.);
#3713=EDGE_CURVE('',#2692,#2693,#434,.T.);
#3714=EDGE_CURVE('',#2693,#2694,#435,.T.);
#3715=EDGE_CURVE('',#2694,#2695,#436,.T.);
#3716=EDGE_CURVE('',#2695,#2696,#437,.T.);
#3717=EDGE_CURVE('',#2696,#2697,#438,.T.);
#3718=EDGE_CURVE('',#2697,#2698,#439,.T.);
#3719=EDGE_CURVE('',#2698,#2699,#440,.T.);
#3720=EDGE_CURVE('',#2699,#2700,#441,.T.);
#3721=EDGE_CURVE('',#2700,#2701,#442,.T.);
#3722=EDGE_CURVE('',#2701,#2702,#443,.T.);
#3723=EDGE_CURVE('',#2702,#2703,#444,.T.);
#3724=EDGE_CURVE('',#2703,#2704,#445,.T.);
#3725=EDGE_CURVE('',#2704,#2705,#446,.T.);
#3726=EDGE_CURVE('',#2705,#2706,#447,.T.);
#3727=EDGE_CURVE('',#2706,#2707,#448,.T.);
#3728=EDGE_CURVE('',#2707,#2708,#449,.T.);
#3729=EDGE_CURVE('',#2708,#2709,#450,.T.);
#3730=EDGE_CURVE('',#2709,#2710,#451,.T.);
#3731=EDGE_CURVE('',#2710,#2711,#452,.T.);
#3732=EDGE_CURVE('',#2711,#2712,#453,.T.);
#3733=EDGE_CURVE('',#2712,#2713,#454,.T.);
#3734=EDGE_CURVE('',#2713,#2714,#455,.T.);
#3735=EDGE_CURVE('',#2714,#2715,#456,.T.);
#3736=EDGE_CURVE('',#2715,#2716,#457,.T.);
#3737=EDGE_CURVE('',#2716,#2717,#458,.T.);
#3738=EDGE_CURVE('',#2717,#2718,#459,.T.);
#3739=EDGE_CURVE('',#2718,#2719,#460,.T.);
#3740=EDGE_CURVE('',#2719,#2720,#461,.T.);
#3741=EDGE_CURVE('',#2720,#2721,#462,.T.);
#3742=EDGE_CURVE('',#2721,#2722,#463,.T.);
#3743=EDGE_CURVE('',#2722,#2723,#464,.T.);
#3744=EDGE_CURVE('',#2723,#2724,#465,.T.);
#3745=EDGE_CURVE('',#2724,#2725,#466,.T.);
#3746=EDGE_CURVE('',#2725,#2726,#467,.T.);
#3747=EDGE_CURVE('',#2726,#2727,#468,.T.);
#3748=EDGE_CURVE('',#2727,#2728,#469,.T.);
#3749=EDGE_CURVE('',#2728,#2729,#470,.T.);
#3750=EDGE_CURVE('',#2729,#2730,#471,.T.);
#3751=EDGE_CURVE('',#2730,#2731,#472,.T.);
#3752=EDGE_CURVE('',#2731,#2732,#473,.T.);
#3753=EDGE_CURVE('',#2732,#2733,#474,.T.);
#3754=EDGE_CURVE('',#2733,#2734,#475,.T.);
#3755=EDGE_CURVE('',#2734,#2735,#476,.T.);
#3756=EDGE_CURVE('',#2735,#2736,#477,.T.);
#3757=EDGE_CURVE('',#2736,#2737,#478,.T.);
#3758=EDGE_CURVE('',#2737,#2738,#479,.T.);
#3759=EDGE_CURVE('',#2738,#2739,#480,.T.);
#3760=EDGE_CURVE('',#2739,#2740,#481,.T.);
#3761=EDGE_CURVE('',#2740,#2741,#482,.T.);
#3762=EDGE_CURVE('',#2741,#2742,#483,.T.);
#3763=EDGE_CURVE('',#2742,#2743,#484,.T.);
#3764=EDGE_CURVE('',#2743,#2744,#485,.T.);
#3765=EDGE_CURVE('',#2744,#2745,#486,.T.);
#3766=EDGE_CURVE('',#2745,#2746,#487,.T.);
#3767=EDGE_CURVE('',#2746,#2747,#488,.T.);
#3768=EDGE_CURVE('',#2747,#2748,#489,.T.);
#3769=EDGE_CURVE('',#2748,#2749,#490,.T.);
#3770=EDGE_CURVE('',#2749,#2750,#491,.T.);
#3771=EDGE_CURVE('',#2750,#2751,#492,.T.);
#3772=EDGE_CURVE('',#2751,#2752,#493,.T.);
#3773=EDGE_CURVE('',#2752,#2753,#494,.T.);
#3774=EDGE_CURVE('',#2753,#2754,#495,.T.);
#3775=EDGE_CURVE('',#2754,#2755,#496,.T.);
#3776=EDGE_CURVE('',#2755,#2756,#497,.T.);
#3777=EDGE_CURVE('',#2756,#2757,#2253,.T.);
#3778=EDGE_CURVE('',#2757,#2758,#498,.T.);
#3779=EDGE_CURVE('',#2758,#2759,#499,.T.);
#3780=EDGE_CURVE('',#2759,#2760,#500,.T.);
#3781=EDGE_CURVE('',#2760,#2761,#501,.T.);
#3782=EDGE_CURVE('',#2761,#2762,#502,.T.);
#3783=EDGE_CURVE('',#2762,#2763,#503,.T.);
#3784=EDGE_CURVE('',#2763,#2764,#504,.T.);
#3785=EDGE_CURVE('',#2764,#2765,#505,.T.);
#3786=EDGE_CURVE('',#2765,#2766,#506,.T.);
#3787=EDGE_CURVE('',#2766,#2767,#507,.T.);
#3788=EDGE_CURVE('',#2767,#2768,#508,.T.);
#3789=EDGE_CURVE('',#2768,#2769,#509,.T.);
#3790=EDGE_CURVE('',#2769,#2770,#510,.T.);
#3791=EDGE_CURVE('',#2770,#2771,#511,.T.);
#3792=EDGE_CURVE('',#2771,#2772,#512,.T.);
#3793=EDGE_CURVE('',#2772,#2773,#513,.T.);
#3794=EDGE_CURVE('',#2773,#2774,#514,.T.);
#3795=EDGE_CURVE('',#2774,#2775,#515,.T.);
#3796=EDGE_CURVE('',#2775,#2776,#516,.T.);
#3797=EDGE_CURVE('',#2776,#2777,#517,.T.);
#3798=EDGE_CURVE('',#2777,#2778,#518,.T.);
#3799=EDGE_CURVE('',#2778,#2779,#519,.T.);
#3800=EDGE_CURVE('',#2779,#2780,#520,.T.);
#3801=EDGE_CURVE('',#2780,#2781,#521,.T.);
#3802=EDGE_CURVE('',#2781,#2782,#522,.T.);
#3803=EDGE_CURVE('',#2782,#2783,#523,.T.);
#3804=EDGE_CURVE('',#2783,#2784,#524,.T.);
#3805=EDGE_CURVE('',#2784,#2785,#525,.T.);
#3806=EDGE_CURVE('',#2785,#2786,#526,.T.);
#3807=EDGE_CURVE('',#2786,#2787,#527,.T.);
#3808=EDGE_CURVE('',#2787,#2788,#528,.T.);
#3809=EDGE_CURVE('',#2788,#2789,#529,.T.);
#3810=EDGE_CURVE('',#2789,#2790,#530,.T.);
#3811=EDGE_CURVE('',#2790,#2791,#531,.T.);
#3812=EDGE_CURVE('',#2791,#2792,#532,.T.);
#3813=EDGE_CURVE('',#2792,#2793,#533,.T.);
#3814=EDGE_CURVE('',#2793,#2794,#534,.T.);
#3815=EDGE_CURVE('',#2794,#2795,#535,.T.);
#3816=EDGE_CURVE('',#2795,#2796,#536,.T.);
#3817=EDGE_CURVE('',#2796,#2797,#537,.T.);
#3818=EDGE_CURVE('',#2797,#2798,#538,.T.);
#3819=EDGE_CURVE('',#2798,#2799,#539,.T.);
#3820=EDGE_CURVE('',#2799,#2800,#540,.T.);
#3821=EDGE_CURVE('',#2800,#2801,#541,.T.);
#3822=EDGE_CURVE('',#2801,#2802,#542,.T.);
#3823=EDGE_CURVE('',#2802,#2803,#543,.T.);
#3824=EDGE_CURVE('',#2803,#2804,#544,.T.);
#3825=EDGE_CURVE('',#2804,#2805,#545,.T.);
#3826=EDGE_CURVE('',#2805,#2806,#546,.T.);
#3827=EDGE_CURVE('',#2806,#2807,#547,.T.);
#3828=EDGE_CURVE('',#2807,#2808,#548,.T.);
#3829=EDGE_CURVE('',#2808,#2809,#549,.T.);
#3830=EDGE_CURVE('',#2809,#2810,#550,.T.);
#3831=EDGE_CURVE('',#2810,#2811,#551,.T.);
#3832=EDGE_CURVE('',#2811,#2812,#552,.T.);
#3833=EDGE_CURVE('',#2812,#2813,#553,.T.);
#3834=EDGE_CURVE('',#2813,#2814,#554,.T.);
#3835=EDGE_CURVE('',#2814,#2815,#555,.T.);
#3836=EDGE_CURVE('',#2815,#2816,#556,.T.);
#3837=EDGE_CURVE('',#2816,#2817,#557,.T.);
#3838=EDGE_CURVE('',#2817,#2818,#558,.T.);
#3839=EDGE_CURVE('',#2818,#2676,#559,.T.);
#3840=EDGE_CURVE('',#2819,#2819,#2254,.T.);
#3841=EDGE_CURVE('',#2819,#2820,#1780,.T.);
#3842=EDGE_CURVE('',#2820,#2820,#2255,.T.);
#3843=EDGE_CURVE('',#2821,#2821,#2256,.T.);
#3844=EDGE_CURVE('',#2822,#2822,#2257,.T.);
#3845=EDGE_CURVE('',#2823,#2823,#2258,.T.);
#3846=EDGE_CURVE('',#2823,#2822,#1781,.T.);
#3847=EDGE_CURVE('',#2821,#2824,#1782,.T.);
#3848=EDGE_CURVE('',#2824,#2824,#2259,.T.);
#3849=EDGE_CURVE('',#2825,#2825,#2260,.T.);
#3850=EDGE_CURVE('',#2826,#2827,#2261,.T.);
#3851=EDGE_CURVE('',#2827,#2674,#107,.T.);
#3852=EDGE_CURVE('',#2673,#2826,#108,.T.);
#3853=EDGE_CURVE('',#2828,#2828,#2262,.T.);
#3854=EDGE_CURVE('',#2828,#2825,#1783,.T.);
#3855=EDGE_CURVE('',#2829,#2829,#2263,.T.);
#3856=EDGE_CURVE('',#2829,#2830,#1784,.T.);
#3857=EDGE_CURVE('',#2830,#2830,#2264,.T.);
#3858=EDGE_CURVE('',#2831,#2831,#2265,.T.);
#3859=EDGE_CURVE('',#2831,#2832,#1785,.T.);
#3860=EDGE_CURVE('',#2832,#2832,#2266,.T.);
#3861=EDGE_CURVE('',#2833,#2833,#2267,.T.);
#3862=EDGE_CURVE('',#2833,#2834,#1786,.T.);
#3863=EDGE_CURVE('',#2834,#2834,#2268,.T.);
#3864=EDGE_CURVE('',#2835,#2835,#2269,.T.);
#3865=EDGE_CURVE('',#2835,#2836,#1787,.T.);
#3866=EDGE_CURVE('',#2836,#2836,#2270,.T.);
#3867=EDGE_CURVE('',#2827,#2756,#560,.T.);
#3868=EDGE_CURVE('',#2757,#2826,#561,.T.);
#3869=EDGE_CURVE('',#2677,#2367,#562,.T.);
#3870=EDGE_CURVE('',#2366,#2678,#563,.T.);
#3871=EDGE_CURVE('',#2837,#2838,#1788,.T.);
#3872=EDGE_CURVE('',#2837,#2839,#1789,.T.);
#3873=EDGE_CURVE('',#2839,#2840,#1790,.T.);
#3874=EDGE_CURVE('',#2838,#2840,#1791,.T.);
#3875=EDGE_CURVE('',#2841,#2837,#1792,.T.);
#3876=EDGE_CURVE('',#2841,#2842,#1793,.T.);
#3877=EDGE_CURVE('',#2842,#2839,#1794,.T.);
#3878=EDGE_CURVE('',#2843,#2841,#1795,.T.);
#3879=EDGE_CURVE('',#2843,#2844,#1796,.T.);
#3880=EDGE_CURVE('',#2844,#2842,#1797,.T.);
#3881=EDGE_CURVE('',#2845,#2843,#1798,.T.);
#3882=EDGE_CURVE('',#2845,#2846,#1799,.T.);
#3883=EDGE_CURVE('',#2846,#2844,#1800,.T.);
#3884=EDGE_CURVE('',#2847,#2845,#1801,.T.);
#3885=EDGE_CURVE('',#2847,#2848,#1802,.T.);
#3886=EDGE_CURVE('',#2848,#2846,#1803,.T.);
#3887=EDGE_CURVE('',#2838,#2847,#1804,.T.);
#3888=EDGE_CURVE('',#2840,#2848,#1805,.T.);
#3889=EDGE_CURVE('',#2849,#2849,#2271,.F.);
#3890=EDGE_CURVE('',#2849,#2850,#1806,.T.);
#3891=EDGE_CURVE('',#2850,#2850,#2272,.F.);
#4527=ORIENTED_EDGE('',*,*,#3308,.F.);
#4528=ORIENTED_EDGE('',*,*,#3309,.F.);
#4529=ORIENTED_EDGE('',*,*,#3310,.F.);
#4530=ORIENTED_EDGE('',*,*,#3311,.T.);
#4531=ORIENTED_EDGE('',*,*,#3312,.F.);
#4532=ORIENTED_EDGE('',*,*,#3313,.F.);
#4533=ORIENTED_EDGE('',*,*,#3314,.F.);
#4534=ORIENTED_EDGE('',*,*,#3308,.T.);
#4535=ORIENTED_EDGE('',*,*,#3315,.T.);
#4536=ORIENTED_EDGE('',*,*,#3316,.T.);
#4537=ORIENTED_EDGE('',*,*,#3317,.F.);
#4538=ORIENTED_EDGE('',*,*,#3318,.F.);
#4539=ORIENTED_EDGE('',*,*,#3319,.F.);
#4540=ORIENTED_EDGE('',*,*,#3312,.T.);
#4541=ORIENTED_EDGE('',*,*,#3320,.T.);
#4542=ORIENTED_EDGE('',*,*,#3321,.T.);
#4543=ORIENTED_EDGE('',*,*,#3322,.F.);
#4544=ORIENTED_EDGE('',*,*,#3323,.F.);
#4545=ORIENTED_EDGE('',*,*,#3324,.F.);
#4546=ORIENTED_EDGE('',*,*,#3317,.T.);
#4547=ORIENTED_EDGE('',*,*,#3325,.T.);
#4548=ORIENTED_EDGE('',*,*,#3326,.T.);
#4549=ORIENTED_EDGE('',*,*,#3327,.F.);
#4550=ORIENTED_EDGE('',*,*,#3328,.F.);
#4551=ORIENTED_EDGE('',*,*,#3329,.F.);
#4552=ORIENTED_EDGE('',*,*,#3322,.T.);
#4553=ORIENTED_EDGE('',*,*,#3330,.T.);
#4554=ORIENTED_EDGE('',*,*,#3331,.T.);
#4555=ORIENTED_EDGE('',*,*,#3332,.F.);
#4556=ORIENTED_EDGE('',*,*,#3333,.F.);
#4557=ORIENTED_EDGE('',*,*,#3334,.F.);
#4558=ORIENTED_EDGE('',*,*,#3327,.T.);
#4559=ORIENTED_EDGE('',*,*,#3335,.T.);
#4560=ORIENTED_EDGE('',*,*,#3336,.T.);
#4561=ORIENTED_EDGE('',*,*,#3337,.F.);
#4562=ORIENTED_EDGE('',*,*,#3338,.F.);
#4563=ORIENTED_EDGE('',*,*,#3339,.F.);
#4564=ORIENTED_EDGE('',*,*,#3332,.T.);
#4565=ORIENTED_EDGE('',*,*,#3340,.T.);
#4566=ORIENTED_EDGE('',*,*,#3341,.T.);
#4567=ORIENTED_EDGE('',*,*,#3342,.F.);
#4568=ORIENTED_EDGE('',*,*,#3343,.F.);
#4569=ORIENTED_EDGE('',*,*,#3344,.F.);
#4570=ORIENTED_EDGE('',*,*,#3337,.T.);
#4571=ORIENTED_EDGE('',*,*,#3345,.T.);
#4572=ORIENTED_EDGE('',*,*,#3346,.T.);
#4573=ORIENTED_EDGE('',*,*,#3347,.F.);
#4574=ORIENTED_EDGE('',*,*,#3348,.F.);
#4575=ORIENTED_EDGE('',*,*,#3349,.F.);
#4576=ORIENTED_EDGE('',*,*,#3342,.T.);
#4577=ORIENTED_EDGE('',*,*,#3350,.T.);
#4578=ORIENTED_EDGE('',*,*,#3351,.T.);
#4579=ORIENTED_EDGE('',*,*,#3352,.F.);
#4580=ORIENTED_EDGE('',*,*,#3353,.F.);
#4581=ORIENTED_EDGE('',*,*,#3354,.F.);
#4582=ORIENTED_EDGE('',*,*,#3347,.T.);
#4583=ORIENTED_EDGE('',*,*,#3355,.T.);
#4584=ORIENTED_EDGE('',*,*,#3356,.T.);
#4585=ORIENTED_EDGE('',*,*,#3357,.F.);
#4586=ORIENTED_EDGE('',*,*,#3358,.F.);
#4587=ORIENTED_EDGE('',*,*,#3359,.F.);
#4588=ORIENTED_EDGE('',*,*,#3352,.T.);
#4589=ORIENTED_EDGE('',*,*,#3360,.T.);
#4590=ORIENTED_EDGE('',*,*,#3361,.T.);
#4591=ORIENTED_EDGE('',*,*,#3362,.F.);
#4592=ORIENTED_EDGE('',*,*,#3363,.F.);
#4593=ORIENTED_EDGE('',*,*,#3364,.F.);
#4594=ORIENTED_EDGE('',*,*,#3357,.T.);
#4595=ORIENTED_EDGE('',*,*,#3365,.T.);
#4596=ORIENTED_EDGE('',*,*,#3366,.T.);
#4597=ORIENTED_EDGE('',*,*,#3367,.F.);
#4598=ORIENTED_EDGE('',*,*,#3368,.F.);
#4599=ORIENTED_EDGE('',*,*,#3369,.F.);
#4600=ORIENTED_EDGE('',*,*,#3362,.T.);
#4601=ORIENTED_EDGE('',*,*,#3370,.T.);
#4602=ORIENTED_EDGE('',*,*,#3371,.T.);
#4603=ORIENTED_EDGE('',*,*,#3372,.F.);
#4604=ORIENTED_EDGE('',*,*,#3373,.F.);
#4605=ORIENTED_EDGE('',*,*,#3374,.F.);
#4606=ORIENTED_EDGE('',*,*,#3367,.T.);
#4607=ORIENTED_EDGE('',*,*,#3375,.T.);
#4608=ORIENTED_EDGE('',*,*,#3376,.T.);
#4609=ORIENTED_EDGE('',*,*,#3377,.F.);
#4610=ORIENTED_EDGE('',*,*,#3378,.F.);
#4611=ORIENTED_EDGE('',*,*,#3379,.F.);
#4612=ORIENTED_EDGE('',*,*,#3372,.T.);
#4613=ORIENTED_EDGE('',*,*,#3380,.T.);
#4614=ORIENTED_EDGE('',*,*,#3381,.T.);
#4615=ORIENTED_EDGE('',*,*,#3382,.F.);
#4616=ORIENTED_EDGE('',*,*,#3383,.F.);
#4617=ORIENTED_EDGE('',*,*,#3384,.F.);
#4618=ORIENTED_EDGE('',*,*,#3377,.T.);
#4619=ORIENTED_EDGE('',*,*,#3385,.T.);
#4620=ORIENTED_EDGE('',*,*,#3386,.T.);
#4621=ORIENTED_EDGE('',*,*,#3387,.F.);
#4622=ORIENTED_EDGE('',*,*,#3388,.F.);
#4623=ORIENTED_EDGE('',*,*,#3389,.F.);
#4624=ORIENTED_EDGE('',*,*,#3382,.T.);
#4625=ORIENTED_EDGE('',*,*,#3390,.T.);
#4626=ORIENTED_EDGE('',*,*,#3391,.T.);
#4627=ORIENTED_EDGE('',*,*,#3392,.F.);
#4628=ORIENTED_EDGE('',*,*,#3393,.F.);
#4629=ORIENTED_EDGE('',*,*,#3394,.F.);
#4630=ORIENTED_EDGE('',*,*,#3387,.T.);
#4631=ORIENTED_EDGE('',*,*,#3395,.T.);
#4632=ORIENTED_EDGE('',*,*,#3396,.T.);
#4633=ORIENTED_EDGE('',*,*,#3397,.F.);
#4634=ORIENTED_EDGE('',*,*,#3398,.F.);
#4635=ORIENTED_EDGE('',*,*,#3399,.F.);
#4636=ORIENTED_EDGE('',*,*,#3392,.T.);
#4637=ORIENTED_EDGE('',*,*,#3400,.T.);
#4638=ORIENTED_EDGE('',*,*,#3401,.T.);
#4639=ORIENTED_EDGE('',*,*,#3402,.F.);
#4640=ORIENTED_EDGE('',*,*,#3403,.F.);
#4641=ORIENTED_EDGE('',*,*,#3404,.F.);
#4642=ORIENTED_EDGE('',*,*,#3397,.T.);
#4643=ORIENTED_EDGE('',*,*,#3405,.T.);
#4644=ORIENTED_EDGE('',*,*,#3406,.T.);
#4645=ORIENTED_EDGE('',*,*,#3407,.F.);
#4646=ORIENTED_EDGE('',*,*,#3408,.F.);
#4647=ORIENTED_EDGE('',*,*,#3409,.F.);
#4648=ORIENTED_EDGE('',*,*,#3402,.T.);
#4649=ORIENTED_EDGE('',*,*,#3410,.T.);
#4650=ORIENTED_EDGE('',*,*,#3411,.T.);
#4651=ORIENTED_EDGE('',*,*,#3412,.F.);
#4652=ORIENTED_EDGE('',*,*,#3413,.F.);
#4653=ORIENTED_EDGE('',*,*,#3414,.F.);
#4654=ORIENTED_EDGE('',*,*,#3407,.T.);
#4655=ORIENTED_EDGE('',*,*,#3415,.T.);
#4656=ORIENTED_EDGE('',*,*,#3416,.T.);
#4657=ORIENTED_EDGE('',*,*,#3417,.F.);
#4658=ORIENTED_EDGE('',*,*,#3418,.F.);
#4659=ORIENTED_EDGE('',*,*,#3419,.F.);
#4660=ORIENTED_EDGE('',*,*,#3412,.T.);
#4661=ORIENTED_EDGE('',*,*,#3420,.T.);
#4662=ORIENTED_EDGE('',*,*,#3421,.T.);
#4663=ORIENTED_EDGE('',*,*,#3422,.F.);
#4664=ORIENTED_EDGE('',*,*,#3423,.F.);
#4665=ORIENTED_EDGE('',*,*,#3424,.F.);
#4666=ORIENTED_EDGE('',*,*,#3417,.T.);
#4667=ORIENTED_EDGE('',*,*,#3425,.T.);
#4668=ORIENTED_EDGE('',*,*,#3426,.T.);
#4669=ORIENTED_EDGE('',*,*,#3427,.F.);
#4670=ORIENTED_EDGE('',*,*,#3428,.F.);
#4671=ORIENTED_EDGE('',*,*,#3429,.F.);
#4672=ORIENTED_EDGE('',*,*,#3422,.T.);
#4673=ORIENTED_EDGE('',*,*,#3430,.T.);
#4674=ORIENTED_EDGE('',*,*,#3431,.T.);
#4675=ORIENTED_EDGE('',*,*,#3432,.F.);
#4676=ORIENTED_EDGE('',*,*,#3433,.F.);
#4677=ORIENTED_EDGE('',*,*,#3434,.F.);
#4678=ORIENTED_EDGE('',*,*,#3427,.T.);
#4679=ORIENTED_EDGE('',*,*,#3435,.T.);
#4680=ORIENTED_EDGE('',*,*,#3436,.T.);
#4681=ORIENTED_EDGE('',*,*,#3437,.F.);
#4682=ORIENTED_EDGE('',*,*,#3438,.F.);
#4683=ORIENTED_EDGE('',*,*,#3439,.F.);
#4684=ORIENTED_EDGE('',*,*,#3432,.T.);
#4685=ORIENTED_EDGE('',*,*,#3440,.T.);
#4686=ORIENTED_EDGE('',*,*,#3441,.T.);
#4687=ORIENTED_EDGE('',*,*,#3442,.F.);
#4688=ORIENTED_EDGE('',*,*,#3443,.F.);
#4689=ORIENTED_EDGE('',*,*,#3444,.F.);
#4690=ORIENTED_EDGE('',*,*,#3437,.T.);
#4691=ORIENTED_EDGE('',*,*,#3445,.T.);
#4692=ORIENTED_EDGE('',*,*,#3446,.T.);
#4693=ORIENTED_EDGE('',*,*,#3447,.F.);
#4694=ORIENTED_EDGE('',*,*,#3448,.F.);
#4695=ORIENTED_EDGE('',*,*,#3449,.F.);
#4696=ORIENTED_EDGE('',*,*,#3442,.T.);
#4697=ORIENTED_EDGE('',*,*,#3450,.T.);
#4698=ORIENTED_EDGE('',*,*,#3451,.T.);
#4699=ORIENTED_EDGE('',*,*,#3452,.F.);
#4700=ORIENTED_EDGE('',*,*,#3453,.F.);
#4701=ORIENTED_EDGE('',*,*,#3454,.F.);
#4702=ORIENTED_EDGE('',*,*,#3447,.T.);
#4703=ORIENTED_EDGE('',*,*,#3455,.T.);
#4704=ORIENTED_EDGE('',*,*,#3456,.T.);
#4705=ORIENTED_EDGE('',*,*,#3457,.F.);
#4706=ORIENTED_EDGE('',*,*,#3458,.F.);
#4707=ORIENTED_EDGE('',*,*,#3459,.F.);
#4708=ORIENTED_EDGE('',*,*,#3452,.T.);
#4709=ORIENTED_EDGE('',*,*,#3460,.T.);
#4710=ORIENTED_EDGE('',*,*,#3461,.T.);
#4711=ORIENTED_EDGE('',*,*,#3462,.F.);
#4712=ORIENTED_EDGE('',*,*,#3463,.F.);
#4713=ORIENTED_EDGE('',*,*,#3464,.F.);
#4714=ORIENTED_EDGE('',*,*,#3457,.T.);
#4715=ORIENTED_EDGE('',*,*,#3465,.T.);
#4716=ORIENTED_EDGE('',*,*,#3466,.T.);
#4717=ORIENTED_EDGE('',*,*,#3467,.F.);
#4718=ORIENTED_EDGE('',*,*,#3468,.F.);
#4719=ORIENTED_EDGE('',*,*,#3469,.F.);
#4720=ORIENTED_EDGE('',*,*,#3462,.T.);
#4721=ORIENTED_EDGE('',*,*,#3470,.T.);
#4722=ORIENTED_EDGE('',*,*,#3471,.T.);
#4723=ORIENTED_EDGE('',*,*,#3472,.F.);
#4724=ORIENTED_EDGE('',*,*,#3473,.F.);
#4725=ORIENTED_EDGE('',*,*,#3474,.F.);
#4726=ORIENTED_EDGE('',*,*,#3467,.T.);
#4727=ORIENTED_EDGE('',*,*,#3475,.T.);
#4728=ORIENTED_EDGE('',*,*,#3476,.T.);
#4729=ORIENTED_EDGE('',*,*,#3477,.F.);
#4730=ORIENTED_EDGE('',*,*,#3478,.F.);
#4731=ORIENTED_EDGE('',*,*,#3479,.F.);
#4732=ORIENTED_EDGE('',*,*,#3472,.T.);
#4733=ORIENTED_EDGE('',*,*,#3480,.T.);
#4734=ORIENTED_EDGE('',*,*,#3481,.T.);
#4735=ORIENTED_EDGE('',*,*,#3482,.F.);
#4736=ORIENTED_EDGE('',*,*,#3483,.F.);
#4737=ORIENTED_EDGE('',*,*,#3484,.F.);
#4738=ORIENTED_EDGE('',*,*,#3477,.T.);
#4739=ORIENTED_EDGE('',*,*,#3485,.T.);
#4740=ORIENTED_EDGE('',*,*,#3486,.T.);
#4741=ORIENTED_EDGE('',*,*,#3487,.F.);
#4742=ORIENTED_EDGE('',*,*,#3488,.F.);
#4743=ORIENTED_EDGE('',*,*,#3489,.F.);
#4744=ORIENTED_EDGE('',*,*,#3482,.T.);
#4745=ORIENTED_EDGE('',*,*,#3490,.T.);
#4746=ORIENTED_EDGE('',*,*,#3491,.T.);
#4747=ORIENTED_EDGE('',*,*,#3492,.F.);
#4748=ORIENTED_EDGE('',*,*,#3493,.F.);
#4749=ORIENTED_EDGE('',*,*,#3494,.F.);
#4750=ORIENTED_EDGE('',*,*,#3487,.T.);
#4751=ORIENTED_EDGE('',*,*,#3495,.T.);
#4752=ORIENTED_EDGE('',*,*,#3496,.T.);
#4753=ORIENTED_EDGE('',*,*,#3497,.F.);
#4754=ORIENTED_EDGE('',*,*,#3498,.F.);
#4755=ORIENTED_EDGE('',*,*,#3499,.F.);
#4756=ORIENTED_EDGE('',*,*,#3492,.T.);
#4757=ORIENTED_EDGE('',*,*,#3500,.T.);
#4758=ORIENTED_EDGE('',*,*,#3501,.T.);
#4759=ORIENTED_EDGE('',*,*,#3502,.F.);
#4760=ORIENTED_EDGE('',*,*,#3503,.F.);
#4761=ORIENTED_EDGE('',*,*,#3504,.F.);
#4762=ORIENTED_EDGE('',*,*,#3497,.T.);
#4763=ORIENTED_EDGE('',*,*,#3505,.T.);
#4764=ORIENTED_EDGE('',*,*,#3506,.T.);
#4765=ORIENTED_EDGE('',*,*,#3507,.F.);
#4766=ORIENTED_EDGE('',*,*,#3508,.F.);
#4767=ORIENTED_EDGE('',*,*,#3509,.F.);
#4768=ORIENTED_EDGE('',*,*,#3502,.T.);
#4769=ORIENTED_EDGE('',*,*,#3510,.T.);
#4770=ORIENTED_EDGE('',*,*,#3511,.T.);
#4771=ORIENTED_EDGE('',*,*,#3512,.F.);
#4772=ORIENTED_EDGE('',*,*,#3513,.F.);
#4773=ORIENTED_EDGE('',*,*,#3514,.F.);
#4774=ORIENTED_EDGE('',*,*,#3507,.T.);
#4775=ORIENTED_EDGE('',*,*,#3515,.T.);
#4776=ORIENTED_EDGE('',*,*,#3516,.T.);
#4777=ORIENTED_EDGE('',*,*,#3517,.F.);
#4778=ORIENTED_EDGE('',*,*,#3518,.F.);
#4779=ORIENTED_EDGE('',*,*,#3519,.F.);
#4780=ORIENTED_EDGE('',*,*,#3512,.T.);
#4781=ORIENTED_EDGE('',*,*,#3520,.T.);
#4782=ORIENTED_EDGE('',*,*,#3521,.T.);
#4783=ORIENTED_EDGE('',*,*,#3522,.F.);
#4784=ORIENTED_EDGE('',*,*,#3523,.F.);
#4785=ORIENTED_EDGE('',*,*,#3524,.F.);
#4786=ORIENTED_EDGE('',*,*,#3517,.T.);
#4787=ORIENTED_EDGE('',*,*,#3525,.T.);
#4788=ORIENTED_EDGE('',*,*,#3526,.T.);
#4789=ORIENTED_EDGE('',*,*,#3527,.F.);
#4790=ORIENTED_EDGE('',*,*,#3528,.F.);
#4791=ORIENTED_EDGE('',*,*,#3529,.F.);
#4792=ORIENTED_EDGE('',*,*,#3522,.T.);
#4793=ORIENTED_EDGE('',*,*,#3530,.T.);
#4794=ORIENTED_EDGE('',*,*,#3531,.T.);
#4795=ORIENTED_EDGE('',*,*,#3532,.F.);
#4796=ORIENTED_EDGE('',*,*,#3533,.F.);
#4797=ORIENTED_EDGE('',*,*,#3534,.F.);
#4798=ORIENTED_EDGE('',*,*,#3527,.T.);
#4799=ORIENTED_EDGE('',*,*,#3535,.T.);
#4800=ORIENTED_EDGE('',*,*,#3536,.T.);
#4801=ORIENTED_EDGE('',*,*,#3537,.F.);
#4802=ORIENTED_EDGE('',*,*,#3538,.F.);
#4803=ORIENTED_EDGE('',*,*,#3539,.F.);
#4804=ORIENTED_EDGE('',*,*,#3532,.T.);
#4805=ORIENTED_EDGE('',*,*,#3540,.T.);
#4806=ORIENTED_EDGE('',*,*,#3541,.T.);
#4807=ORIENTED_EDGE('',*,*,#3542,.F.);
#4808=ORIENTED_EDGE('',*,*,#3543,.F.);
#4809=ORIENTED_EDGE('',*,*,#3544,.F.);
#4810=ORIENTED_EDGE('',*,*,#3537,.T.);
#4811=ORIENTED_EDGE('',*,*,#3545,.T.);
#4812=ORIENTED_EDGE('',*,*,#3546,.T.);
#4813=ORIENTED_EDGE('',*,*,#3547,.F.);
#4814=ORIENTED_EDGE('',*,*,#3548,.F.);
#4815=ORIENTED_EDGE('',*,*,#3549,.F.);
#4816=ORIENTED_EDGE('',*,*,#3542,.T.);
#4817=ORIENTED_EDGE('',*,*,#3550,.T.);
#4818=ORIENTED_EDGE('',*,*,#3551,.T.);
#4819=ORIENTED_EDGE('',*,*,#3552,.F.);
#4820=ORIENTED_EDGE('',*,*,#3553,.F.);
#4821=ORIENTED_EDGE('',*,*,#3554,.F.);
#4822=ORIENTED_EDGE('',*,*,#3547,.T.);
#4823=ORIENTED_EDGE('',*,*,#3555,.T.);
#4824=ORIENTED_EDGE('',*,*,#3556,.T.);
#4825=ORIENTED_EDGE('',*,*,#3557,.F.);
#4826=ORIENTED_EDGE('',*,*,#3558,.F.);
#4827=ORIENTED_EDGE('',*,*,#3559,.F.);
#4828=ORIENTED_EDGE('',*,*,#3552,.T.);
#4829=ORIENTED_EDGE('',*,*,#3560,.T.);
#4830=ORIENTED_EDGE('',*,*,#3561,.T.);
#4831=ORIENTED_EDGE('',*,*,#3562,.F.);
#4832=ORIENTED_EDGE('',*,*,#3563,.F.);
#4833=ORIENTED_EDGE('',*,*,#3564,.F.);
#4834=ORIENTED_EDGE('',*,*,#3557,.T.);
#4835=ORIENTED_EDGE('',*,*,#3565,.T.);
#4836=ORIENTED_EDGE('',*,*,#3566,.T.);
#4837=ORIENTED_EDGE('',*,*,#3567,.F.);
#4838=ORIENTED_EDGE('',*,*,#3568,.F.);
#4839=ORIENTED_EDGE('',*,*,#3569,.F.);
#4840=ORIENTED_EDGE('',*,*,#3562,.T.);
#4841=ORIENTED_EDGE('',*,*,#3570,.T.);
#4842=ORIENTED_EDGE('',*,*,#3571,.T.);
#4843=ORIENTED_EDGE('',*,*,#3572,.F.);
#4844=ORIENTED_EDGE('',*,*,#3573,.F.);
#4845=ORIENTED_EDGE('',*,*,#3574,.F.);
#4846=ORIENTED_EDGE('',*,*,#3567,.T.);
#4847=ORIENTED_EDGE('',*,*,#3575,.T.);
#4848=ORIENTED_EDGE('',*,*,#3576,.T.);
#4849=ORIENTED_EDGE('',*,*,#3577,.F.);
#4850=ORIENTED_EDGE('',*,*,#3578,.F.);
#4851=ORIENTED_EDGE('',*,*,#3579,.F.);
#4852=ORIENTED_EDGE('',*,*,#3572,.T.);
#4853=ORIENTED_EDGE('',*,*,#3580,.T.);
#4854=ORIENTED_EDGE('',*,*,#3581,.T.);
#4855=ORIENTED_EDGE('',*,*,#3582,.F.);
#4856=ORIENTED_EDGE('',*,*,#3583,.F.);
#4857=ORIENTED_EDGE('',*,*,#3584,.F.);
#4858=ORIENTED_EDGE('',*,*,#3577,.T.);
#4859=ORIENTED_EDGE('',*,*,#3585,.T.);
#4860=ORIENTED_EDGE('',*,*,#3586,.T.);
#4861=ORIENTED_EDGE('',*,*,#3587,.F.);
#4862=ORIENTED_EDGE('',*,*,#3588,.F.);
#4863=ORIENTED_EDGE('',*,*,#3589,.F.);
#4864=ORIENTED_EDGE('',*,*,#3582,.T.);
#4865=ORIENTED_EDGE('',*,*,#3590,.T.);
#4866=ORIENTED_EDGE('',*,*,#3591,.T.);
#4867=ORIENTED_EDGE('',*,*,#3592,.F.);
#4868=ORIENTED_EDGE('',*,*,#3593,.F.);
#4869=ORIENTED_EDGE('',*,*,#3594,.F.);
#4870=ORIENTED_EDGE('',*,*,#3587,.T.);
#4871=ORIENTED_EDGE('',*,*,#3595,.T.);
#4872=ORIENTED_EDGE('',*,*,#3596,.T.);
#4873=ORIENTED_EDGE('',*,*,#3597,.F.);
#4874=ORIENTED_EDGE('',*,*,#3598,.F.);
#4875=ORIENTED_EDGE('',*,*,#3599,.F.);
#4876=ORIENTED_EDGE('',*,*,#3592,.T.);
#4877=ORIENTED_EDGE('',*,*,#3600,.T.);
#4878=ORIENTED_EDGE('',*,*,#3601,.T.);
#4879=ORIENTED_EDGE('',*,*,#3602,.F.);
#4880=ORIENTED_EDGE('',*,*,#3603,.F.);
#4881=ORIENTED_EDGE('',*,*,#3604,.F.);
#4882=ORIENTED_EDGE('',*,*,#3597,.T.);
#4883=ORIENTED_EDGE('',*,*,#3605,.T.);
#4884=ORIENTED_EDGE('',*,*,#3606,.T.);
#4885=ORIENTED_EDGE('',*,*,#3607,.F.);
#4886=ORIENTED_EDGE('',*,*,#3608,.F.);
#4887=ORIENTED_EDGE('',*,*,#3609,.F.);
#4888=ORIENTED_EDGE('',*,*,#3602,.T.);
#4889=ORIENTED_EDGE('',*,*,#3610,.T.);
#4890=ORIENTED_EDGE('',*,*,#3611,.T.);
#4891=ORIENTED_EDGE('',*,*,#3612,.F.);
#4892=ORIENTED_EDGE('',*,*,#3613,.F.);
#4893=ORIENTED_EDGE('',*,*,#3614,.F.);
#4894=ORIENTED_EDGE('',*,*,#3607,.T.);
#4895=ORIENTED_EDGE('',*,*,#3615,.T.);
#4896=ORIENTED_EDGE('',*,*,#3616,.T.);
#4897=ORIENTED_EDGE('',*,*,#3617,.F.);
#4898=ORIENTED_EDGE('',*,*,#3618,.F.);
#4899=ORIENTED_EDGE('',*,*,#3619,.F.);
#4900=ORIENTED_EDGE('',*,*,#3612,.T.);
#4901=ORIENTED_EDGE('',*,*,#3620,.T.);
#4902=ORIENTED_EDGE('',*,*,#3621,.T.);
#4903=ORIENTED_EDGE('',*,*,#3622,.F.);
#4904=ORIENTED_EDGE('',*,*,#3623,.F.);
#4905=ORIENTED_EDGE('',*,*,#3624,.F.);
#4906=ORIENTED_EDGE('',*,*,#3617,.T.);
#4907=ORIENTED_EDGE('',*,*,#3625,.T.);
#4908=ORIENTED_EDGE('',*,*,#3626,.T.);
#4909=ORIENTED_EDGE('',*,*,#3627,.F.);
#4910=ORIENTED_EDGE('',*,*,#3628,.F.);
#4911=ORIENTED_EDGE('',*,*,#3629,.F.);
#4912=ORIENTED_EDGE('',*,*,#3622,.T.);
#4913=ORIENTED_EDGE('',*,*,#3630,.T.);
#4914=ORIENTED_EDGE('',*,*,#3631,.T.);
#4915=ORIENTED_EDGE('',*,*,#3632,.F.);
#4916=ORIENTED_EDGE('',*,*,#3633,.F.);
#4917=ORIENTED_EDGE('',*,*,#3634,.F.);
#4918=ORIENTED_EDGE('',*,*,#3627,.T.);
#4919=ORIENTED_EDGE('',*,*,#3635,.T.);
#4920=ORIENTED_EDGE('',*,*,#3636,.T.);
#4921=ORIENTED_EDGE('',*,*,#3637,.F.);
#4922=ORIENTED_EDGE('',*,*,#3638,.F.);
#4923=ORIENTED_EDGE('',*,*,#3639,.F.);
#4924=ORIENTED_EDGE('',*,*,#3632,.T.);
#4925=ORIENTED_EDGE('',*,*,#3640,.T.);
#4926=ORIENTED_EDGE('',*,*,#3641,.T.);
#4927=ORIENTED_EDGE('',*,*,#3642,.F.);
#4928=ORIENTED_EDGE('',*,*,#3643,.F.);
#4929=ORIENTED_EDGE('',*,*,#3644,.F.);
#4930=ORIENTED_EDGE('',*,*,#3637,.T.);
#4931=ORIENTED_EDGE('',*,*,#3645,.T.);
#4932=ORIENTED_EDGE('',*,*,#3646,.T.);
#4933=ORIENTED_EDGE('',*,*,#3647,.F.);
#4934=ORIENTED_EDGE('',*,*,#3648,.F.);
#4935=ORIENTED_EDGE('',*,*,#3649,.F.);
#4936=ORIENTED_EDGE('',*,*,#3642,.T.);
#4937=ORIENTED_EDGE('',*,*,#3650,.T.);
#4938=ORIENTED_EDGE('',*,*,#3651,.T.);
#4939=ORIENTED_EDGE('',*,*,#3652,.F.);
#4940=ORIENTED_EDGE('',*,*,#3653,.F.);
#4941=ORIENTED_EDGE('',*,*,#3654,.F.);
#4942=ORIENTED_EDGE('',*,*,#3647,.T.);
#4943=ORIENTED_EDGE('',*,*,#3655,.T.);
#4944=ORIENTED_EDGE('',*,*,#3656,.T.);
#4945=ORIENTED_EDGE('',*,*,#3657,.F.);
#4946=ORIENTED_EDGE('',*,*,#3658,.F.);
#4947=ORIENTED_EDGE('',*,*,#3659,.F.);
#4948=ORIENTED_EDGE('',*,*,#3652,.T.);
#4949=ORIENTED_EDGE('',*,*,#3660,.T.);
#4950=ORIENTED_EDGE('',*,*,#3661,.T.);
#4951=ORIENTED_EDGE('',*,*,#3662,.F.);
#4952=ORIENTED_EDGE('',*,*,#3663,.F.);
#4953=ORIENTED_EDGE('',*,*,#3664,.F.);
#4954=ORIENTED_EDGE('',*,*,#3657,.T.);
#4955=ORIENTED_EDGE('',*,*,#3665,.T.);
#4956=ORIENTED_EDGE('',*,*,#3666,.T.);
#4957=ORIENTED_EDGE('',*,*,#3667,.F.);
#4958=ORIENTED_EDGE('',*,*,#3668,.F.);
#4959=ORIENTED_EDGE('',*,*,#3669,.F.);
#4960=ORIENTED_EDGE('',*,*,#3662,.T.);
#4961=ORIENTED_EDGE('',*,*,#3670,.T.);
#4962=ORIENTED_EDGE('',*,*,#3671,.T.);
#4963=ORIENTED_EDGE('',*,*,#3672,.F.);
#4964=ORIENTED_EDGE('',*,*,#3673,.F.);
#4965=ORIENTED_EDGE('',*,*,#3674,.F.);
#4966=ORIENTED_EDGE('',*,*,#3667,.T.);
#4967=ORIENTED_EDGE('',*,*,#3675,.T.);
#4968=ORIENTED_EDGE('',*,*,#3676,.T.);
#4969=ORIENTED_EDGE('',*,*,#3677,.F.);
#4970=ORIENTED_EDGE('',*,*,#3678,.F.);
#4971=ORIENTED_EDGE('',*,*,#3679,.F.);
#4972=ORIENTED_EDGE('',*,*,#3672,.T.);
#4973=ORIENTED_EDGE('',*,*,#3680,.T.);
#4974=ORIENTED_EDGE('',*,*,#3681,.T.);
#4975=ORIENTED_EDGE('',*,*,#3682,.F.);
#4976=ORIENTED_EDGE('',*,*,#3683,.F.);
#4977=ORIENTED_EDGE('',*,*,#3684,.F.);
#4978=ORIENTED_EDGE('',*,*,#3677,.T.);
#4979=ORIENTED_EDGE('',*,*,#3685,.T.);
#4980=ORIENTED_EDGE('',*,*,#3686,.T.);
#4981=ORIENTED_EDGE('',*,*,#3687,.F.);
#4982=ORIENTED_EDGE('',*,*,#3688,.F.);
#4983=ORIENTED_EDGE('',*,*,#3689,.F.);
#4984=ORIENTED_EDGE('',*,*,#3682,.T.);
#4985=ORIENTED_EDGE('',*,*,#3690,.T.);
#4986=ORIENTED_EDGE('',*,*,#3691,.T.);
#4987=ORIENTED_EDGE('',*,*,#3687,.T.);
#4988=ORIENTED_EDGE('',*,*,#3692,.T.);
#4989=ORIENTED_EDGE('',*,*,#3693,.T.);
#4990=ORIENTED_EDGE('',*,*,#3694,.F.);
#4991=ORIENTED_EDGE('',*,*,#3695,.F.);
#4992=ORIENTED_EDGE('',*,*,#3696,.F.);
#4993=ORIENTED_EDGE('',*,*,#3697,.T.);
#4994=ORIENTED_EDGE('',*,*,#3698,.T.);
#4995=ORIENTED_EDGE('',*,*,#3699,.T.);
#4996=ORIENTED_EDGE('',*,*,#3700,.T.);
#4997=ORIENTED_EDGE('',*,*,#3701,.T.);
#4998=ORIENTED_EDGE('',*,*,#3702,.T.);
#4999=ORIENTED_EDGE('',*,*,#3703,.T.);
#5000=ORIENTED_EDGE('',*,*,#3704,.T.);
#5001=ORIENTED_EDGE('',*,*,#3705,.T.);
#5002=ORIENTED_EDGE('',*,*,#3706,.T.);
#5003=ORIENTED_EDGE('',*,*,#3707,.T.);
#5004=ORIENTED_EDGE('',*,*,#3708,.T.);
#5005=ORIENTED_EDGE('',*,*,#3709,.T.);
#5006=ORIENTED_EDGE('',*,*,#3710,.T.);
#5007=ORIENTED_EDGE('',*,*,#3711,.T.);
#5008=ORIENTED_EDGE('',*,*,#3712,.T.);
#5009=ORIENTED_EDGE('',*,*,#3713,.T.);
#5010=ORIENTED_EDGE('',*,*,#3714,.T.);
#5011=ORIENTED_EDGE('',*,*,#3715,.T.);
#5012=ORIENTED_EDGE('',*,*,#3716,.T.);
#5013=ORIENTED_EDGE('',*,*,#3717,.T.);
#5014=ORIENTED_EDGE('',*,*,#3718,.T.);
#5015=ORIENTED_EDGE('',*,*,#3719,.T.);
#5016=ORIENTED_EDGE('',*,*,#3720,.T.);
#5017=ORIENTED_EDGE('',*,*,#3721,.T.);
#5018=ORIENTED_EDGE('',*,*,#3722,.T.);
#5019=ORIENTED_EDGE('',*,*,#3723,.T.);
#5020=ORIENTED_EDGE('',*,*,#3724,.T.);
#5021=ORIENTED_EDGE('',*,*,#3725,.T.);
#5022=ORIENTED_EDGE('',*,*,#3726,.T.);
#5023=ORIENTED_EDGE('',*,*,#3727,.T.);
#5024=ORIENTED_EDGE('',*,*,#3728,.T.);
#5025=ORIENTED_EDGE('',*,*,#3729,.T.);
#5026=ORIENTED_EDGE('',*,*,#3730,.T.);
#5027=ORIENTED_EDGE('',*,*,#3731,.T.);
#5028=ORIENTED_EDGE('',*,*,#3732,.T.);
#5029=ORIENTED_EDGE('',*,*,#3733,.T.);
#5030=ORIENTED_EDGE('',*,*,#3734,.T.);
#5031=ORIENTED_EDGE('',*,*,#3735,.T.);
#5032=ORIENTED_EDGE('',*,*,#3736,.T.);
#5033=ORIENTED_EDGE('',*,*,#3737,.T.);
#5034=ORIENTED_EDGE('',*,*,#3738,.T.);
#5035=ORIENTED_EDGE('',*,*,#3739,.T.);
#5036=ORIENTED_EDGE('',*,*,#3740,.T.);
#5037=ORIENTED_EDGE('',*,*,#3741,.T.);
#5038=ORIENTED_EDGE('',*,*,#3742,.T.);
#5039=ORIENTED_EDGE('',*,*,#3743,.T.);
#5040=ORIENTED_EDGE('',*,*,#3744,.T.);
#5041=ORIENTED_EDGE('',*,*,#3745,.T.);
#5042=ORIENTED_EDGE('',*,*,#3746,.T.);
#5043=ORIENTED_EDGE('',*,*,#3747,.T.);
#5044=ORIENTED_EDGE('',*,*,#3748,.T.);
#5045=ORIENTED_EDGE('',*,*,#3749,.T.);
#5046=ORIENTED_EDGE('',*,*,#3750,.T.);
#5047=ORIENTED_EDGE('',*,*,#3751,.T.);
#5048=ORIENTED_EDGE('',*,*,#3752,.T.);
#5049=ORIENTED_EDGE('',*,*,#3753,.T.);
#5050=ORIENTED_EDGE('',*,*,#3754,.T.);
#5051=ORIENTED_EDGE('',*,*,#3755,.T.);
#5052=ORIENTED_EDGE('',*,*,#3756,.T.);
#5053=ORIENTED_EDGE('',*,*,#3757,.T.);
#5054=ORIENTED_EDGE('',*,*,#3758,.T.);
#5055=ORIENTED_EDGE('',*,*,#3759,.T.);
#5056=ORIENTED_EDGE('',*,*,#3760,.T.);
#5057=ORIENTED_EDGE('',*,*,#3761,.T.);
#5058=ORIENTED_EDGE('',*,*,#3762,.T.);
#5059=ORIENTED_EDGE('',*,*,#3763,.T.);
#5060=ORIENTED_EDGE('',*,*,#3764,.T.);
#5061=ORIENTED_EDGE('',*,*,#3765,.T.);
#5062=ORIENTED_EDGE('',*,*,#3766,.T.);
#5063=ORIENTED_EDGE('',*,*,#3767,.T.);
#5064=ORIENTED_EDGE('',*,*,#3768,.T.);
#5065=ORIENTED_EDGE('',*,*,#3769,.T.);
#5066=ORIENTED_EDGE('',*,*,#3770,.T.);
#5067=ORIENTED_EDGE('',*,*,#3771,.T.);
#5068=ORIENTED_EDGE('',*,*,#3772,.T.);
#5069=ORIENTED_EDGE('',*,*,#3773,.T.);
#5070=ORIENTED_EDGE('',*,*,#3774,.T.);
#5071=ORIENTED_EDGE('',*,*,#3775,.T.);
#5072=ORIENTED_EDGE('',*,*,#3776,.T.);
#5073=ORIENTED_EDGE('',*,*,#3777,.T.);
#5074=ORIENTED_EDGE('',*,*,#3778,.T.);
#5075=ORIENTED_EDGE('',*,*,#3779,.T.);
#5076=ORIENTED_EDGE('',*,*,#3780,.T.);
#5077=ORIENTED_EDGE('',*,*,#3781,.T.);
#5078=ORIENTED_EDGE('',*,*,#3782,.T.);
#5079=ORIENTED_EDGE('',*,*,#3783,.T.);
#5080=ORIENTED_EDGE('',*,*,#3784,.T.);
#5081=ORIENTED_EDGE('',*,*,#3785,.T.);
#5082=ORIENTED_EDGE('',*,*,#3786,.T.);
#5083=ORIENTED_EDGE('',*,*,#3787,.T.);
#5084=ORIENTED_EDGE('',*,*,#3788,.T.);
#5085=ORIENTED_EDGE('',*,*,#3789,.T.);
#5086=ORIENTED_EDGE('',*,*,#3790,.T.);
#5087=ORIENTED_EDGE('',*,*,#3791,.T.);
#5088=ORIENTED_EDGE('',*,*,#3792,.T.);
#5089=ORIENTED_EDGE('',*,*,#3793,.T.);
#5090=ORIENTED_EDGE('',*,*,#3794,.T.);
#5091=ORIENTED_EDGE('',*,*,#3795,.T.);
#5092=ORIENTED_EDGE('',*,*,#3796,.T.);
#5093=ORIENTED_EDGE('',*,*,#3797,.T.);
#5094=ORIENTED_EDGE('',*,*,#3798,.T.);
#5095=ORIENTED_EDGE('',*,*,#3799,.T.);
#5096=ORIENTED_EDGE('',*,*,#3800,.T.);
#5097=ORIENTED_EDGE('',*,*,#3801,.T.);
#5098=ORIENTED_EDGE('',*,*,#3802,.T.);
#5099=ORIENTED_EDGE('',*,*,#3803,.T.);
#5100=ORIENTED_EDGE('',*,*,#3804,.T.);
#5101=ORIENTED_EDGE('',*,*,#3805,.T.);
#5102=ORIENTED_EDGE('',*,*,#3806,.T.);
#5103=ORIENTED_EDGE('',*,*,#3807,.T.);
#5104=ORIENTED_EDGE('',*,*,#3808,.T.);
#5105=ORIENTED_EDGE('',*,*,#3809,.T.);
#5106=ORIENTED_EDGE('',*,*,#3810,.T.);
#5107=ORIENTED_EDGE('',*,*,#3811,.T.);
#5108=ORIENTED_EDGE('',*,*,#3812,.T.);
#5109=ORIENTED_EDGE('',*,*,#3813,.T.);
#5110=ORIENTED_EDGE('',*,*,#3814,.T.);
#5111=ORIENTED_EDGE('',*,*,#3815,.T.);
#5112=ORIENTED_EDGE('',*,*,#3816,.T.);
#5113=ORIENTED_EDGE('',*,*,#3817,.T.);
#5114=ORIENTED_EDGE('',*,*,#3818,.T.);
#5115=ORIENTED_EDGE('',*,*,#3819,.T.);
#5116=ORIENTED_EDGE('',*,*,#3820,.T.);
#5117=ORIENTED_EDGE('',*,*,#3821,.T.);
#5118=ORIENTED_EDGE('',*,*,#3822,.T.);
#5119=ORIENTED_EDGE('',*,*,#3823,.T.);
#5120=ORIENTED_EDGE('',*,*,#3824,.T.);
#5121=ORIENTED_EDGE('',*,*,#3825,.T.);
#5122=ORIENTED_EDGE('',*,*,#3826,.T.);
#5123=ORIENTED_EDGE('',*,*,#3827,.T.);
#5124=ORIENTED_EDGE('',*,*,#3828,.T.);
#5125=ORIENTED_EDGE('',*,*,#3829,.T.);
#5126=ORIENTED_EDGE('',*,*,#3830,.T.);
#5127=ORIENTED_EDGE('',*,*,#3831,.T.);
#5128=ORIENTED_EDGE('',*,*,#3832,.T.);
#5129=ORIENTED_EDGE('',*,*,#3833,.T.);
#5130=ORIENTED_EDGE('',*,*,#3834,.T.);
#5131=ORIENTED_EDGE('',*,*,#3835,.T.);
#5132=ORIENTED_EDGE('',*,*,#3836,.T.);
#5133=ORIENTED_EDGE('',*,*,#3837,.T.);
#5134=ORIENTED_EDGE('',*,*,#3838,.T.);
#5135=ORIENTED_EDGE('',*,*,#3839,.T.);
#5136=ORIENTED_EDGE('',*,*,#3840,.F.);
#5137=ORIENTED_EDGE('',*,*,#3841,.T.);
#5138=ORIENTED_EDGE('',*,*,#3842,.T.);
#5139=ORIENTED_EDGE('',*,*,#3841,.F.);
#5140=ORIENTED_EDGE('',*,*,#3843,.F.);
#5141=ORIENTED_EDGE('',*,*,#3842,.F.);
#5142=ORIENTED_EDGE('',*,*,#3844,.F.);
#5143=ORIENTED_EDGE('',*,*,#3840,.T.);
#5144=ORIENTED_EDGE('',*,*,#3845,.F.);
#5145=ORIENTED_EDGE('',*,*,#3846,.T.);
#5146=ORIENTED_EDGE('',*,*,#3844,.T.);
#5147=ORIENTED_EDGE('',*,*,#3846,.F.);
#5148=ORIENTED_EDGE('',*,*,#3843,.T.);
#5149=ORIENTED_EDGE('',*,*,#3847,.T.);
#5150=ORIENTED_EDGE('',*,*,#3848,.F.);
#5151=ORIENTED_EDGE('',*,*,#3847,.F.);
#5152=ORIENTED_EDGE('',*,*,#3845,.T.);
#5153=ORIENTED_EDGE('',*,*,#3849,.F.);
#5154=ORIENTED_EDGE('',*,*,#3850,.T.);
#5155=ORIENTED_EDGE('',*,*,#3851,.T.);
#5156=ORIENTED_EDGE('',*,*,#3694,.T.);
#5157=ORIENTED_EDGE('',*,*,#3852,.T.);
#5158=ORIENTED_EDGE('',*,*,#3853,.F.);
#5159=ORIENTED_EDGE('',*,*,#3854,.T.);
#5160=ORIENTED_EDGE('',*,*,#3849,.T.);
#5161=ORIENTED_EDGE('',*,*,#3854,.F.);
#5162=ORIENTED_EDGE('',*,*,#3853,.T.);
#5163=ORIENTED_EDGE('',*,*,#3848,.T.);
#5164=ORIENTED_EDGE('',*,*,#3855,.F.);
#5165=ORIENTED_EDGE('',*,*,#3856,.T.);
#5166=ORIENTED_EDGE('',*,*,#3857,.F.);
#5167=ORIENTED_EDGE('',*,*,#3856,.F.);
#5168=ORIENTED_EDGE('',*,*,#3858,.F.);
#5169=ORIENTED_EDGE('',*,*,#3859,.T.);
#5170=ORIENTED_EDGE('',*,*,#3860,.F.);
#5171=ORIENTED_EDGE('',*,*,#3859,.F.);
#5172=ORIENTED_EDGE('',*,*,#3861,.F.);
#5173=ORIENTED_EDGE('',*,*,#3862,.T.);
#5174=ORIENTED_EDGE('',*,*,#3863,.F.);
#5175=ORIENTED_EDGE('',*,*,#3862,.F.);
#5176=ORIENTED_EDGE('',*,*,#3864,.F.);
#5177=ORIENTED_EDGE('',*,*,#3865,.T.);
#5178=ORIENTED_EDGE('',*,*,#3866,.F.);
#5179=ORIENTED_EDGE('',*,*,#3865,.F.);
#5180=ORIENTED_EDGE('',*,*,#3867,.F.);
#5181=ORIENTED_EDGE('',*,*,#3850,.F.);
#5182=ORIENTED_EDGE('',*,*,#3868,.F.);
#5183=ORIENTED_EDGE('',*,*,#3777,.F.);
#5184=ORIENTED_EDGE('',*,*,#3868,.T.);
#5185=ORIENTED_EDGE('',*,*,#3852,.F.);
#5186=ORIENTED_EDGE('',*,*,#3693,.F.);
#5187=ORIENTED_EDGE('',*,*,#3692,.F.);
#5188=ORIENTED_EDGE('',*,*,#3691,.F.);
#5189=ORIENTED_EDGE('',*,*,#3690,.F.);
#5190=ORIENTED_EDGE('',*,*,#3686,.F.);
#5191=ORIENTED_EDGE('',*,*,#3685,.F.);
#5192=ORIENTED_EDGE('',*,*,#3681,.F.);
#5193=ORIENTED_EDGE('',*,*,#3680,.F.);
#5194=ORIENTED_EDGE('',*,*,#3676,.F.);
#5195=ORIENTED_EDGE('',*,*,#3675,.F.);
#5196=ORIENTED_EDGE('',*,*,#3671,.F.);
#5197=ORIENTED_EDGE('',*,*,#3670,.F.);
#5198=ORIENTED_EDGE('',*,*,#3666,.F.);
#5199=ORIENTED_EDGE('',*,*,#3665,.F.);
#5200=ORIENTED_EDGE('',*,*,#3661,.F.);
#5201=ORIENTED_EDGE('',*,*,#3660,.F.);
#5202=ORIENTED_EDGE('',*,*,#3656,.F.);
#5203=ORIENTED_EDGE('',*,*,#3655,.F.);
#5204=ORIENTED_EDGE('',*,*,#3651,.F.);
#5205=ORIENTED_EDGE('',*,*,#3650,.F.);
#5206=ORIENTED_EDGE('',*,*,#3646,.F.);
#5207=ORIENTED_EDGE('',*,*,#3645,.F.);
#5208=ORIENTED_EDGE('',*,*,#3641,.F.);
#5209=ORIENTED_EDGE('',*,*,#3640,.F.);
#5210=ORIENTED_EDGE('',*,*,#3636,.F.);
#5211=ORIENTED_EDGE('',*,*,#3635,.F.);
#5212=ORIENTED_EDGE('',*,*,#3631,.F.);
#5213=ORIENTED_EDGE('',*,*,#3630,.F.);
#5214=ORIENTED_EDGE('',*,*,#3626,.F.);
#5215=ORIENTED_EDGE('',*,*,#3625,.F.);
#5216=ORIENTED_EDGE('',*,*,#3621,.F.);
#5217=ORIENTED_EDGE('',*,*,#3620,.F.);
#5218=ORIENTED_EDGE('',*,*,#3616,.F.);
#5219=ORIENTED_EDGE('',*,*,#3615,.F.);
#5220=ORIENTED_EDGE('',*,*,#3611,.F.);
#5221=ORIENTED_EDGE('',*,*,#3610,.F.);
#5222=ORIENTED_EDGE('',*,*,#3606,.F.);
#5223=ORIENTED_EDGE('',*,*,#3605,.F.);
#5224=ORIENTED_EDGE('',*,*,#3601,.F.);
#5225=ORIENTED_EDGE('',*,*,#3600,.F.);
#5226=ORIENTED_EDGE('',*,*,#3596,.F.);
#5227=ORIENTED_EDGE('',*,*,#3595,.F.);
#5228=ORIENTED_EDGE('',*,*,#3591,.F.);
#5229=ORIENTED_EDGE('',*,*,#3590,.F.);
#5230=ORIENTED_EDGE('',*,*,#3586,.F.);
#5231=ORIENTED_EDGE('',*,*,#3585,.F.);
#5232=ORIENTED_EDGE('',*,*,#3581,.F.);
#5233=ORIENTED_EDGE('',*,*,#3580,.F.);
#5234=ORIENTED_EDGE('',*,*,#3576,.F.);
#5235=ORIENTED_EDGE('',*,*,#3575,.F.);
#5236=ORIENTED_EDGE('',*,*,#3571,.F.);
#5237=ORIENTED_EDGE('',*,*,#3570,.F.);
#5238=ORIENTED_EDGE('',*,*,#3566,.F.);
#5239=ORIENTED_EDGE('',*,*,#3565,.F.);
#5240=ORIENTED_EDGE('',*,*,#3561,.F.);
#5241=ORIENTED_EDGE('',*,*,#3560,.F.);
#5242=ORIENTED_EDGE('',*,*,#3556,.F.);
#5243=ORIENTED_EDGE('',*,*,#3555,.F.);
#5244=ORIENTED_EDGE('',*,*,#3551,.F.);
#5245=ORIENTED_EDGE('',*,*,#3550,.F.);
#5246=ORIENTED_EDGE('',*,*,#3546,.F.);
#5247=ORIENTED_EDGE('',*,*,#3545,.F.);
#5248=ORIENTED_EDGE('',*,*,#3541,.F.);
#5249=ORIENTED_EDGE('',*,*,#3540,.F.);
#5250=ORIENTED_EDGE('',*,*,#3536,.F.);
#5251=ORIENTED_EDGE('',*,*,#3535,.F.);
#5252=ORIENTED_EDGE('',*,*,#3531,.F.);
#5253=ORIENTED_EDGE('',*,*,#3530,.F.);
#5254=ORIENTED_EDGE('',*,*,#3526,.F.);
#5255=ORIENTED_EDGE('',*,*,#3525,.F.);
#5256=ORIENTED_EDGE('',*,*,#3521,.F.);
#5257=ORIENTED_EDGE('',*,*,#3520,.F.);
#5258=ORIENTED_EDGE('',*,*,#3516,.F.);
#5259=ORIENTED_EDGE('',*,*,#3515,.F.);
#5260=ORIENTED_EDGE('',*,*,#3511,.F.);
#5261=ORIENTED_EDGE('',*,*,#3510,.F.);
#5262=ORIENTED_EDGE('',*,*,#3506,.F.);
#5263=ORIENTED_EDGE('',*,*,#3505,.F.);
#5264=ORIENTED_EDGE('',*,*,#3501,.F.);
#5265=ORIENTED_EDGE('',*,*,#3500,.F.);
#5266=ORIENTED_EDGE('',*,*,#3496,.F.);
#5267=ORIENTED_EDGE('',*,*,#3495,.F.);
#5268=ORIENTED_EDGE('',*,*,#3491,.F.);
#5269=ORIENTED_EDGE('',*,*,#3490,.F.);
#5270=ORIENTED_EDGE('',*,*,#3486,.F.);
#5271=ORIENTED_EDGE('',*,*,#3485,.F.);
#5272=ORIENTED_EDGE('',*,*,#3481,.F.);
#5273=ORIENTED_EDGE('',*,*,#3480,.F.);
#5274=ORIENTED_EDGE('',*,*,#3476,.F.);
#5275=ORIENTED_EDGE('',*,*,#3475,.F.);
#5276=ORIENTED_EDGE('',*,*,#3471,.F.);
#5277=ORIENTED_EDGE('',*,*,#3470,.F.);
#5278=ORIENTED_EDGE('',*,*,#3466,.F.);
#5279=ORIENTED_EDGE('',*,*,#3465,.F.);
#5280=ORIENTED_EDGE('',*,*,#3461,.F.);
#5281=ORIENTED_EDGE('',*,*,#3460,.F.);
#5282=ORIENTED_EDGE('',*,*,#3456,.F.);
#5283=ORIENTED_EDGE('',*,*,#3455,.F.);
#5284=ORIENTED_EDGE('',*,*,#3451,.F.);
#5285=ORIENTED_EDGE('',*,*,#3450,.F.);
#5286=ORIENTED_EDGE('',*,*,#3446,.F.);
#5287=ORIENTED_EDGE('',*,*,#3445,.F.);
#5288=ORIENTED_EDGE('',*,*,#3441,.F.);
#5289=ORIENTED_EDGE('',*,*,#3440,.F.);
#5290=ORIENTED_EDGE('',*,*,#3436,.F.);
#5291=ORIENTED_EDGE('',*,*,#3435,.F.);
#5292=ORIENTED_EDGE('',*,*,#3431,.F.);
#5293=ORIENTED_EDGE('',*,*,#3430,.F.);
#5294=ORIENTED_EDGE('',*,*,#3426,.F.);
#5295=ORIENTED_EDGE('',*,*,#3425,.F.);
#5296=ORIENTED_EDGE('',*,*,#3421,.F.);
#5297=ORIENTED_EDGE('',*,*,#3420,.F.);
#5298=ORIENTED_EDGE('',*,*,#3416,.F.);
#5299=ORIENTED_EDGE('',*,*,#3415,.F.);
#5300=ORIENTED_EDGE('',*,*,#3411,.F.);
#5301=ORIENTED_EDGE('',*,*,#3410,.F.);
#5302=ORIENTED_EDGE('',*,*,#3406,.F.);
#5303=ORIENTED_EDGE('',*,*,#3405,.F.);
#5304=ORIENTED_EDGE('',*,*,#3401,.F.);
#5305=ORIENTED_EDGE('',*,*,#3400,.F.);
#5306=ORIENTED_EDGE('',*,*,#3396,.F.);
#5307=ORIENTED_EDGE('',*,*,#3395,.F.);
#5308=ORIENTED_EDGE('',*,*,#3391,.F.);
#5309=ORIENTED_EDGE('',*,*,#3390,.F.);
#5310=ORIENTED_EDGE('',*,*,#3386,.F.);
#5311=ORIENTED_EDGE('',*,*,#3385,.F.);
#5312=ORIENTED_EDGE('',*,*,#3381,.F.);
#5313=ORIENTED_EDGE('',*,*,#3380,.F.);
#5314=ORIENTED_EDGE('',*,*,#3376,.F.);
#5315=ORIENTED_EDGE('',*,*,#3375,.F.);
#5316=ORIENTED_EDGE('',*,*,#3371,.F.);
#5317=ORIENTED_EDGE('',*,*,#3370,.F.);
#5318=ORIENTED_EDGE('',*,*,#3366,.F.);
#5319=ORIENTED_EDGE('',*,*,#3365,.F.);
#5320=ORIENTED_EDGE('',*,*,#3361,.F.);
#5321=ORIENTED_EDGE('',*,*,#3360,.F.);
#5322=ORIENTED_EDGE('',*,*,#3356,.F.);
#5323=ORIENTED_EDGE('',*,*,#3355,.F.);
#5324=ORIENTED_EDGE('',*,*,#3351,.F.);
#5325=ORIENTED_EDGE('',*,*,#3350,.F.);
#5326=ORIENTED_EDGE('',*,*,#3346,.F.);
#5327=ORIENTED_EDGE('',*,*,#3345,.F.);
#5328=ORIENTED_EDGE('',*,*,#3341,.F.);
#5329=ORIENTED_EDGE('',*,*,#3340,.F.);
#5330=ORIENTED_EDGE('',*,*,#3336,.F.);
#5331=ORIENTED_EDGE('',*,*,#3335,.F.);
#5332=ORIENTED_EDGE('',*,*,#3331,.F.);
#5333=ORIENTED_EDGE('',*,*,#3330,.F.);
#5334=ORIENTED_EDGE('',*,*,#3326,.F.);
#5335=ORIENTED_EDGE('',*,*,#3325,.F.);
#5336=ORIENTED_EDGE('',*,*,#3321,.F.);
#5337=ORIENTED_EDGE('',*,*,#3320,.F.);
#5338=ORIENTED_EDGE('',*,*,#3316,.F.);
#5339=ORIENTED_EDGE('',*,*,#3315,.F.);
#5340=ORIENTED_EDGE('',*,*,#3311,.F.);
#5341=ORIENTED_EDGE('',*,*,#3869,.F.);
#5342=ORIENTED_EDGE('',*,*,#3697,.F.);
#5343=ORIENTED_EDGE('',*,*,#3839,.F.);
#5344=ORIENTED_EDGE('',*,*,#3838,.F.);
#5345=ORIENTED_EDGE('',*,*,#3837,.F.);
#5346=ORIENTED_EDGE('',*,*,#3836,.F.);
#5347=ORIENTED_EDGE('',*,*,#3835,.F.);
#5348=ORIENTED_EDGE('',*,*,#3834,.F.);
#5349=ORIENTED_EDGE('',*,*,#3833,.F.);
#5350=ORIENTED_EDGE('',*,*,#3832,.F.);
#5351=ORIENTED_EDGE('',*,*,#3831,.F.);
#5352=ORIENTED_EDGE('',*,*,#3830,.F.);
#5353=ORIENTED_EDGE('',*,*,#3829,.F.);
#5354=ORIENTED_EDGE('',*,*,#3828,.F.);
#5355=ORIENTED_EDGE('',*,*,#3827,.F.);
#5356=ORIENTED_EDGE('',*,*,#3826,.F.);
#5357=ORIENTED_EDGE('',*,*,#3825,.F.);
#5358=ORIENTED_EDGE('',*,*,#3824,.F.);
#5359=ORIENTED_EDGE('',*,*,#3823,.F.);
#5360=ORIENTED_EDGE('',*,*,#3822,.F.);
#5361=ORIENTED_EDGE('',*,*,#3821,.F.);
#5362=ORIENTED_EDGE('',*,*,#3820,.F.);
#5363=ORIENTED_EDGE('',*,*,#3819,.F.);
#5364=ORIENTED_EDGE('',*,*,#3818,.F.);
#5365=ORIENTED_EDGE('',*,*,#3817,.F.);
#5366=ORIENTED_EDGE('',*,*,#3816,.F.);
#5367=ORIENTED_EDGE('',*,*,#3815,.F.);
#5368=ORIENTED_EDGE('',*,*,#3814,.F.);
#5369=ORIENTED_EDGE('',*,*,#3813,.F.);
#5370=ORIENTED_EDGE('',*,*,#3812,.F.);
#5371=ORIENTED_EDGE('',*,*,#3811,.F.);
#5372=ORIENTED_EDGE('',*,*,#3810,.F.);
#5373=ORIENTED_EDGE('',*,*,#3809,.F.);
#5374=ORIENTED_EDGE('',*,*,#3808,.F.);
#5375=ORIENTED_EDGE('',*,*,#3807,.F.);
#5376=ORIENTED_EDGE('',*,*,#3806,.F.);
#5377=ORIENTED_EDGE('',*,*,#3805,.F.);
#5378=ORIENTED_EDGE('',*,*,#3804,.F.);
#5379=ORIENTED_EDGE('',*,*,#3803,.F.);
#5380=ORIENTED_EDGE('',*,*,#3802,.F.);
#5381=ORIENTED_EDGE('',*,*,#3801,.F.);
#5382=ORIENTED_EDGE('',*,*,#3800,.F.);
#5383=ORIENTED_EDGE('',*,*,#3799,.F.);
#5384=ORIENTED_EDGE('',*,*,#3798,.F.);
#5385=ORIENTED_EDGE('',*,*,#3797,.F.);
#5386=ORIENTED_EDGE('',*,*,#3796,.F.);
#5387=ORIENTED_EDGE('',*,*,#3795,.F.);
#5388=ORIENTED_EDGE('',*,*,#3794,.F.);
#5389=ORIENTED_EDGE('',*,*,#3793,.F.);
#5390=ORIENTED_EDGE('',*,*,#3792,.F.);
#5391=ORIENTED_EDGE('',*,*,#3791,.F.);
#5392=ORIENTED_EDGE('',*,*,#3790,.F.);
#5393=ORIENTED_EDGE('',*,*,#3789,.F.);
#5394=ORIENTED_EDGE('',*,*,#3788,.F.);
#5395=ORIENTED_EDGE('',*,*,#3787,.F.);
#5396=ORIENTED_EDGE('',*,*,#3786,.F.);
#5397=ORIENTED_EDGE('',*,*,#3785,.F.);
#5398=ORIENTED_EDGE('',*,*,#3784,.F.);
#5399=ORIENTED_EDGE('',*,*,#3783,.F.);
#5400=ORIENTED_EDGE('',*,*,#3782,.F.);
#5401=ORIENTED_EDGE('',*,*,#3781,.F.);
#5402=ORIENTED_EDGE('',*,*,#3780,.F.);
#5403=ORIENTED_EDGE('',*,*,#3779,.F.);
#5404=ORIENTED_EDGE('',*,*,#3778,.F.);
#5405=ORIENTED_EDGE('',*,*,#3867,.T.);
#5406=ORIENTED_EDGE('',*,*,#3776,.F.);
#5407=ORIENTED_EDGE('',*,*,#3775,.F.);
#5408=ORIENTED_EDGE('',*,*,#3774,.F.);
#5409=ORIENTED_EDGE('',*,*,#3773,.F.);
#5410=ORIENTED_EDGE('',*,*,#3772,.F.);
#5411=ORIENTED_EDGE('',*,*,#3771,.F.);
#5412=ORIENTED_EDGE('',*,*,#3770,.F.);
#5413=ORIENTED_EDGE('',*,*,#3769,.F.);
#5414=ORIENTED_EDGE('',*,*,#3768,.F.);
#5415=ORIENTED_EDGE('',*,*,#3767,.F.);
#5416=ORIENTED_EDGE('',*,*,#3766,.F.);
#5417=ORIENTED_EDGE('',*,*,#3765,.F.);
#5418=ORIENTED_EDGE('',*,*,#3764,.F.);
#5419=ORIENTED_EDGE('',*,*,#3763,.F.);
#5420=ORIENTED_EDGE('',*,*,#3762,.F.);
#5421=ORIENTED_EDGE('',*,*,#3761,.F.);
#5422=ORIENTED_EDGE('',*,*,#3760,.F.);
#5423=ORIENTED_EDGE('',*,*,#3759,.F.);
#5424=ORIENTED_EDGE('',*,*,#3758,.F.);
#5425=ORIENTED_EDGE('',*,*,#3757,.F.);
#5426=ORIENTED_EDGE('',*,*,#3756,.F.);
#5427=ORIENTED_EDGE('',*,*,#3755,.F.);
#5428=ORIENTED_EDGE('',*,*,#3754,.F.);
#5429=ORIENTED_EDGE('',*,*,#3753,.F.);
#5430=ORIENTED_EDGE('',*,*,#3752,.F.);
#5431=ORIENTED_EDGE('',*,*,#3751,.F.);
#5432=ORIENTED_EDGE('',*,*,#3750,.F.);
#5433=ORIENTED_EDGE('',*,*,#3749,.F.);
#5434=ORIENTED_EDGE('',*,*,#3748,.F.);
#5435=ORIENTED_EDGE('',*,*,#3747,.F.);
#5436=ORIENTED_EDGE('',*,*,#3746,.F.);
#5437=ORIENTED_EDGE('',*,*,#3745,.F.);
#5438=ORIENTED_EDGE('',*,*,#3744,.F.);
#5439=ORIENTED_EDGE('',*,*,#3743,.F.);
#5440=ORIENTED_EDGE('',*,*,#3742,.F.);
#5441=ORIENTED_EDGE('',*,*,#3741,.F.);
#5442=ORIENTED_EDGE('',*,*,#3740,.F.);
#5443=ORIENTED_EDGE('',*,*,#3739,.F.);
#5444=ORIENTED_EDGE('',*,*,#3738,.F.);
#5445=ORIENTED_EDGE('',*,*,#3737,.F.);
#5446=ORIENTED_EDGE('',*,*,#3736,.F.);
#5447=ORIENTED_EDGE('',*,*,#3735,.F.);
#5448=ORIENTED_EDGE('',*,*,#3734,.F.);
#5449=ORIENTED_EDGE('',*,*,#3733,.F.);
#5450=ORIENTED_EDGE('',*,*,#3732,.F.);
#5451=ORIENTED_EDGE('',*,*,#3731,.F.);
#5452=ORIENTED_EDGE('',*,*,#3730,.F.);
#5453=ORIENTED_EDGE('',*,*,#3729,.F.);
#5454=ORIENTED_EDGE('',*,*,#3728,.F.);
#5455=ORIENTED_EDGE('',*,*,#3727,.F.);
#5456=ORIENTED_EDGE('',*,*,#3726,.F.);
#5457=ORIENTED_EDGE('',*,*,#3725,.F.);
#5458=ORIENTED_EDGE('',*,*,#3724,.F.);
#5459=ORIENTED_EDGE('',*,*,#3723,.F.);
#5460=ORIENTED_EDGE('',*,*,#3722,.F.);
#5461=ORIENTED_EDGE('',*,*,#3721,.F.);
#5462=ORIENTED_EDGE('',*,*,#3720,.F.);
#5463=ORIENTED_EDGE('',*,*,#3719,.F.);
#5464=ORIENTED_EDGE('',*,*,#3718,.F.);
#5465=ORIENTED_EDGE('',*,*,#3717,.F.);
#5466=ORIENTED_EDGE('',*,*,#3716,.F.);
#5467=ORIENTED_EDGE('',*,*,#3715,.F.);
#5468=ORIENTED_EDGE('',*,*,#3714,.F.);
#5469=ORIENTED_EDGE('',*,*,#3713,.F.);
#5470=ORIENTED_EDGE('',*,*,#3712,.F.);
#5471=ORIENTED_EDGE('',*,*,#3711,.F.);
#5472=ORIENTED_EDGE('',*,*,#3710,.F.);
#5473=ORIENTED_EDGE('',*,*,#3709,.F.);
#5474=ORIENTED_EDGE('',*,*,#3708,.F.);
#5475=ORIENTED_EDGE('',*,*,#3707,.F.);
#5476=ORIENTED_EDGE('',*,*,#3706,.F.);
#5477=ORIENTED_EDGE('',*,*,#3705,.F.);
#5478=ORIENTED_EDGE('',*,*,#3704,.F.);
#5479=ORIENTED_EDGE('',*,*,#3703,.F.);
#5480=ORIENTED_EDGE('',*,*,#3702,.F.);
#5481=ORIENTED_EDGE('',*,*,#3701,.F.);
#5482=ORIENTED_EDGE('',*,*,#3700,.F.);
#5483=ORIENTED_EDGE('',*,*,#3699,.F.);
#5484=ORIENTED_EDGE('',*,*,#3870,.F.);
#5485=ORIENTED_EDGE('',*,*,#3309,.T.);
#5486=ORIENTED_EDGE('',*,*,#3314,.T.);
#5487=ORIENTED_EDGE('',*,*,#3313,.T.);
#5488=ORIENTED_EDGE('',*,*,#3319,.T.);
#5489=ORIENTED_EDGE('',*,*,#3318,.T.);
#5490=ORIENTED_EDGE('',*,*,#3324,.T.);
#5491=ORIENTED_EDGE('',*,*,#3323,.T.);
#5492=ORIENTED_EDGE('',*,*,#3329,.T.);
#5493=ORIENTED_EDGE('',*,*,#3328,.T.);
#5494=ORIENTED_EDGE('',*,*,#3334,.T.);
#5495=ORIENTED_EDGE('',*,*,#3333,.T.);
#5496=ORIENTED_EDGE('',*,*,#3339,.T.);
#5497=ORIENTED_EDGE('',*,*,#3338,.T.);
#5498=ORIENTED_EDGE('',*,*,#3344,.T.);
#5499=ORIENTED_EDGE('',*,*,#3343,.T.);
#5500=ORIENTED_EDGE('',*,*,#3349,.T.);
#5501=ORIENTED_EDGE('',*,*,#3348,.T.);
#5502=ORIENTED_EDGE('',*,*,#3354,.T.);
#5503=ORIENTED_EDGE('',*,*,#3353,.T.);
#5504=ORIENTED_EDGE('',*,*,#3359,.T.);
#5505=ORIENTED_EDGE('',*,*,#3358,.T.);
#5506=ORIENTED_EDGE('',*,*,#3364,.T.);
#5507=ORIENTED_EDGE('',*,*,#3363,.T.);
#5508=ORIENTED_EDGE('',*,*,#3369,.T.);
#5509=ORIENTED_EDGE('',*,*,#3368,.T.);
#5510=ORIENTED_EDGE('',*,*,#3374,.T.);
#5511=ORIENTED_EDGE('',*,*,#3373,.T.);
#5512=ORIENTED_EDGE('',*,*,#3379,.T.);
#5513=ORIENTED_EDGE('',*,*,#3378,.T.);
#5514=ORIENTED_EDGE('',*,*,#3384,.T.);
#5515=ORIENTED_EDGE('',*,*,#3383,.T.);
#5516=ORIENTED_EDGE('',*,*,#3389,.T.);
#5517=ORIENTED_EDGE('',*,*,#3388,.T.);
#5518=ORIENTED_EDGE('',*,*,#3394,.T.);
#5519=ORIENTED_EDGE('',*,*,#3393,.T.);
#5520=ORIENTED_EDGE('',*,*,#3399,.T.);
#5521=ORIENTED_EDGE('',*,*,#3398,.T.);
#5522=ORIENTED_EDGE('',*,*,#3404,.T.);
#5523=ORIENTED_EDGE('',*,*,#3403,.T.);
#5524=ORIENTED_EDGE('',*,*,#3409,.T.);
#5525=ORIENTED_EDGE('',*,*,#3408,.T.);
#5526=ORIENTED_EDGE('',*,*,#3414,.T.);
#5527=ORIENTED_EDGE('',*,*,#3413,.T.);
#5528=ORIENTED_EDGE('',*,*,#3419,.T.);
#5529=ORIENTED_EDGE('',*,*,#3418,.T.);
#5530=ORIENTED_EDGE('',*,*,#3424,.T.);
#5531=ORIENTED_EDGE('',*,*,#3423,.T.);
#5532=ORIENTED_EDGE('',*,*,#3429,.T.);
#5533=ORIENTED_EDGE('',*,*,#3428,.T.);
#5534=ORIENTED_EDGE('',*,*,#3434,.T.);
#5535=ORIENTED_EDGE('',*,*,#3433,.T.);
#5536=ORIENTED_EDGE('',*,*,#3439,.T.);
#5537=ORIENTED_EDGE('',*,*,#3438,.T.);
#5538=ORIENTED_EDGE('',*,*,#3444,.T.);
#5539=ORIENTED_EDGE('',*,*,#3443,.T.);
#5540=ORIENTED_EDGE('',*,*,#3449,.T.);
#5541=ORIENTED_EDGE('',*,*,#3448,.T.);
#5542=ORIENTED_EDGE('',*,*,#3454,.T.);
#5543=ORIENTED_EDGE('',*,*,#3453,.T.);
#5544=ORIENTED_EDGE('',*,*,#3459,.T.);
#5545=ORIENTED_EDGE('',*,*,#3458,.T.);
#5546=ORIENTED_EDGE('',*,*,#3464,.T.);
#5547=ORIENTED_EDGE('',*,*,#3463,.T.);
#5548=ORIENTED_EDGE('',*,*,#3469,.T.);
#5549=ORIENTED_EDGE('',*,*,#3468,.T.);
#5550=ORIENTED_EDGE('',*,*,#3474,.T.);
#5551=ORIENTED_EDGE('',*,*,#3473,.T.);
#5552=ORIENTED_EDGE('',*,*,#3479,.T.);
#5553=ORIENTED_EDGE('',*,*,#3478,.T.);
#5554=ORIENTED_EDGE('',*,*,#3484,.T.);
#5555=ORIENTED_EDGE('',*,*,#3483,.T.);
#5556=ORIENTED_EDGE('',*,*,#3489,.T.);
#5557=ORIENTED_EDGE('',*,*,#3488,.T.);
#5558=ORIENTED_EDGE('',*,*,#3494,.T.);
#5559=ORIENTED_EDGE('',*,*,#3493,.T.);
#5560=ORIENTED_EDGE('',*,*,#3499,.T.);
#5561=ORIENTED_EDGE('',*,*,#3498,.T.);
#5562=ORIENTED_EDGE('',*,*,#3504,.T.);
#5563=ORIENTED_EDGE('',*,*,#3503,.T.);
#5564=ORIENTED_EDGE('',*,*,#3509,.T.);
#5565=ORIENTED_EDGE('',*,*,#3508,.T.);
#5566=ORIENTED_EDGE('',*,*,#3514,.T.);
#5567=ORIENTED_EDGE('',*,*,#3513,.T.);
#5568=ORIENTED_EDGE('',*,*,#3519,.T.);
#5569=ORIENTED_EDGE('',*,*,#3518,.T.);
#5570=ORIENTED_EDGE('',*,*,#3524,.T.);
#5571=ORIENTED_EDGE('',*,*,#3523,.T.);
#5572=ORIENTED_EDGE('',*,*,#3529,.T.);
#5573=ORIENTED_EDGE('',*,*,#3528,.T.);
#5574=ORIENTED_EDGE('',*,*,#3534,.T.);
#5575=ORIENTED_EDGE('',*,*,#3533,.T.);
#5576=ORIENTED_EDGE('',*,*,#3539,.T.);
#5577=ORIENTED_EDGE('',*,*,#3538,.T.);
#5578=ORIENTED_EDGE('',*,*,#3544,.T.);
#5579=ORIENTED_EDGE('',*,*,#3543,.T.);
#5580=ORIENTED_EDGE('',*,*,#3549,.T.);
#5581=ORIENTED_EDGE('',*,*,#3548,.T.);
#5582=ORIENTED_EDGE('',*,*,#3554,.T.);
#5583=ORIENTED_EDGE('',*,*,#3553,.T.);
#5584=ORIENTED_EDGE('',*,*,#3559,.T.);
#5585=ORIENTED_EDGE('',*,*,#3558,.T.);
#5586=ORIENTED_EDGE('',*,*,#3564,.T.);
#5587=ORIENTED_EDGE('',*,*,#3563,.T.);
#5588=ORIENTED_EDGE('',*,*,#3569,.T.);
#5589=ORIENTED_EDGE('',*,*,#3568,.T.);
#5590=ORIENTED_EDGE('',*,*,#3574,.T.);
#5591=ORIENTED_EDGE('',*,*,#3573,.T.);
#5592=ORIENTED_EDGE('',*,*,#3579,.T.);
#5593=ORIENTED_EDGE('',*,*,#3578,.T.);
#5594=ORIENTED_EDGE('',*,*,#3584,.T.);
#5595=ORIENTED_EDGE('',*,*,#3583,.T.);
#5596=ORIENTED_EDGE('',*,*,#3589,.T.);
#5597=ORIENTED_EDGE('',*,*,#3588,.T.);
#5598=ORIENTED_EDGE('',*,*,#3594,.T.);
#5599=ORIENTED_EDGE('',*,*,#3593,.T.);
#5600=ORIENTED_EDGE('',*,*,#3599,.T.);
#5601=ORIENTED_EDGE('',*,*,#3598,.T.);
#5602=ORIENTED_EDGE('',*,*,#3604,.T.);
#5603=ORIENTED_EDGE('',*,*,#3603,.T.);
#5604=ORIENTED_EDGE('',*,*,#3609,.T.);
#5605=ORIENTED_EDGE('',*,*,#3608,.T.);
#5606=ORIENTED_EDGE('',*,*,#3614,.T.);
#5607=ORIENTED_EDGE('',*,*,#3613,.T.);
#5608=ORIENTED_EDGE('',*,*,#3619,.T.);
#5609=ORIENTED_EDGE('',*,*,#3618,.T.);
#5610=ORIENTED_EDGE('',*,*,#3624,.T.);
#5611=ORIENTED_EDGE('',*,*,#3623,.T.);
#5612=ORIENTED_EDGE('',*,*,#3629,.T.);
#5613=ORIENTED_EDGE('',*,*,#3628,.T.);
#5614=ORIENTED_EDGE('',*,*,#3634,.T.);
#5615=ORIENTED_EDGE('',*,*,#3633,.T.);
#5616=ORIENTED_EDGE('',*,*,#3639,.T.);
#5617=ORIENTED_EDGE('',*,*,#3638,.T.);
#5618=ORIENTED_EDGE('',*,*,#3644,.T.);
#5619=ORIENTED_EDGE('',*,*,#3643,.T.);
#5620=ORIENTED_EDGE('',*,*,#3649,.T.);
#5621=ORIENTED_EDGE('',*,*,#3648,.T.);
#5622=ORIENTED_EDGE('',*,*,#3654,.T.);
#5623=ORIENTED_EDGE('',*,*,#3653,.T.);
#5624=ORIENTED_EDGE('',*,*,#3659,.T.);
#5625=ORIENTED_EDGE('',*,*,#3658,.T.);
#5626=ORIENTED_EDGE('',*,*,#3664,.T.);
#5627=ORIENTED_EDGE('',*,*,#3663,.T.);
#5628=ORIENTED_EDGE('',*,*,#3669,.T.);
#5629=ORIENTED_EDGE('',*,*,#3668,.T.);
#5630=ORIENTED_EDGE('',*,*,#3674,.T.);
#5631=ORIENTED_EDGE('',*,*,#3673,.T.);
#5632=ORIENTED_EDGE('',*,*,#3679,.T.);
#5633=ORIENTED_EDGE('',*,*,#3678,.T.);
#5634=ORIENTED_EDGE('',*,*,#3684,.T.);
#5635=ORIENTED_EDGE('',*,*,#3683,.T.);
#5636=ORIENTED_EDGE('',*,*,#3689,.T.);
#5637=ORIENTED_EDGE('',*,*,#3688,.T.);
#5638=ORIENTED_EDGE('',*,*,#3696,.T.);
#5639=ORIENTED_EDGE('',*,*,#3695,.T.);
#5640=ORIENTED_EDGE('',*,*,#3851,.F.);
#5641=ORIENTED_EDGE('',*,*,#3871,.F.);
#5642=ORIENTED_EDGE('',*,*,#3872,.T.);
#5643=ORIENTED_EDGE('',*,*,#3873,.T.);
#5644=ORIENTED_EDGE('',*,*,#3874,.F.);
#5645=ORIENTED_EDGE('',*,*,#3875,.F.);
#5646=ORIENTED_EDGE('',*,*,#3876,.T.);
#5647=ORIENTED_EDGE('',*,*,#3877,.T.);
#5648=ORIENTED_EDGE('',*,*,#3872,.F.);
#5649=ORIENTED_EDGE('',*,*,#3878,.F.);
#5650=ORIENTED_EDGE('',*,*,#3879,.T.);
#5651=ORIENTED_EDGE('',*,*,#3880,.T.);
#5652=ORIENTED_EDGE('',*,*,#3876,.F.);
#5653=ORIENTED_EDGE('',*,*,#3881,.F.);
#5654=ORIENTED_EDGE('',*,*,#3882,.T.);
#5655=ORIENTED_EDGE('',*,*,#3883,.T.);
#5656=ORIENTED_EDGE('',*,*,#3879,.F.);
#5657=ORIENTED_EDGE('',*,*,#3884,.F.);
#5658=ORIENTED_EDGE('',*,*,#3885,.T.);
#5659=ORIENTED_EDGE('',*,*,#3886,.T.);
#5660=ORIENTED_EDGE('',*,*,#3882,.F.);
#5661=ORIENTED_EDGE('',*,*,#3887,.F.);
#5662=ORIENTED_EDGE('',*,*,#3874,.T.);
#5663=ORIENTED_EDGE('',*,*,#3888,.T.);
#5664=ORIENTED_EDGE('',*,*,#3885,.F.);
#5665=ORIENTED_EDGE('',*,*,#3888,.F.);
#5666=ORIENTED_EDGE('',*,*,#3873,.F.);
#5667=ORIENTED_EDGE('',*,*,#3877,.F.);
#5668=ORIENTED_EDGE('',*,*,#3880,.F.);
#5669=ORIENTED_EDGE('',*,*,#3883,.F.);
#5670=ORIENTED_EDGE('',*,*,#3886,.F.);
#5671=ORIENTED_EDGE('',*,*,#3889,.T.);
#5672=ORIENTED_EDGE('',*,*,#3869,.T.);
#5673=ORIENTED_EDGE('',*,*,#3310,.T.);
#5674=ORIENTED_EDGE('',*,*,#3870,.T.);
#5675=ORIENTED_EDGE('',*,*,#3698,.F.);
#5676=ORIENTED_EDGE('',*,*,#3864,.T.);
#5677=ORIENTED_EDGE('',*,*,#3861,.T.);
#5678=ORIENTED_EDGE('',*,*,#3858,.T.);
#5679=ORIENTED_EDGE('',*,*,#3855,.T.);
#5680=ORIENTED_EDGE('',*,*,#3889,.F.);
#5681=ORIENTED_EDGE('',*,*,#3890,.T.);
#5682=ORIENTED_EDGE('',*,*,#3891,.T.);
#5683=ORIENTED_EDGE('',*,*,#3890,.F.);
#5684=ORIENTED_EDGE('',*,*,#3891,.F.);
#5685=ORIENTED_EDGE('',*,*,#3871,.T.);
#5686=ORIENTED_EDGE('',*,*,#3887,.T.);
#5687=ORIENTED_EDGE('',*,*,#3884,.T.);
#5688=ORIENTED_EDGE('',*,*,#3881,.T.);
#5689=ORIENTED_EDGE('',*,*,#3878,.T.);
#5690=ORIENTED_EDGE('',*,*,#3875,.T.);
#5691=ORIENTED_EDGE('',*,*,#3866,.T.);
#5692=ORIENTED_EDGE('',*,*,#3863,.T.);
#5693=ORIENTED_EDGE('',*,*,#3860,.T.);
#5694=ORIENTED_EDGE('',*,*,#3857,.T.);
#6748=CYLINDRICAL_SURFACE('',#7399,6.767);
#6749=CYLINDRICAL_SURFACE('',#7401,6.767);
#6750=CYLINDRICAL_SURFACE('',#7402,6.767);
#6751=CYLINDRICAL_SURFACE('',#7403,6.767);
#6752=CYLINDRICAL_SURFACE('',#7404,6.767);
#6753=CYLINDRICAL_SURFACE('',#7405,6.767);
#6754=CYLINDRICAL_SURFACE('',#7406,6.767);
#6755=CYLINDRICAL_SURFACE('',#7407,6.767);
#6756=CYLINDRICAL_SURFACE('',#7408,6.767);
#6757=CYLINDRICAL_SURFACE('',#7409,6.767);
#6758=CYLINDRICAL_SURFACE('',#7410,6.767);
#6759=CYLINDRICAL_SURFACE('',#7411,6.767);
#6760=CYLINDRICAL_SURFACE('',#7412,6.767);
#6761=CYLINDRICAL_SURFACE('',#7413,6.767);
#6762=CYLINDRICAL_SURFACE('',#7414,6.767);
#6763=CYLINDRICAL_SURFACE('',#7415,6.767);
#6764=CYLINDRICAL_SURFACE('',#7416,6.767);
#6765=CYLINDRICAL_SURFACE('',#7417,6.767);
#6766=CYLINDRICAL_SURFACE('',#7418,6.767);
#6767=CYLINDRICAL_SURFACE('',#7419,6.767);
#6768=CYLINDRICAL_SURFACE('',#7420,6.767);
#6769=CYLINDRICAL_SURFACE('',#7421,6.767);
#6770=CYLINDRICAL_SURFACE('',#7422,6.767);
#6771=CYLINDRICAL_SURFACE('',#7423,6.767);
#6772=CYLINDRICAL_SURFACE('',#7424,6.767);
#6773=CYLINDRICAL_SURFACE('',#7425,6.767);
#6774=CYLINDRICAL_SURFACE('',#7426,6.767);
#6775=CYLINDRICAL_SURFACE('',#7427,6.767);
#6776=CYLINDRICAL_SURFACE('',#7428,6.767);
#6777=CYLINDRICAL_SURFACE('',#7429,6.767);
#6778=CYLINDRICAL_SURFACE('',#7430,6.767);
#6779=CYLINDRICAL_SURFACE('',#7431,6.767);
#6780=CYLINDRICAL_SURFACE('',#7432,6.767);
#6781=CYLINDRICAL_SURFACE('',#7433,6.767);
#6782=CYLINDRICAL_SURFACE('',#7434,6.767);
#6783=CYLINDRICAL_SURFACE('',#7435,6.767);
#6784=CYLINDRICAL_SURFACE('',#7436,6.767);
#6785=CYLINDRICAL_SURFACE('',#7437,6.767);
#6786=CYLINDRICAL_SURFACE('',#7438,6.767);
#6787=CYLINDRICAL_SURFACE('',#7439,6.767);
#6788=CYLINDRICAL_SURFACE('',#7440,6.767);
#6789=CYLINDRICAL_SURFACE('',#7441,6.767);
#6790=CYLINDRICAL_SURFACE('',#7442,6.767);
#6791=CYLINDRICAL_SURFACE('',#7443,6.767);
#6792=CYLINDRICAL_SURFACE('',#7444,6.767);
#6793=CYLINDRICAL_SURFACE('',#7445,6.767);
#6794=CYLINDRICAL_SURFACE('',#7446,6.767);
#6795=CYLINDRICAL_SURFACE('',#7447,6.767);
#6796=CYLINDRICAL_SURFACE('',#7448,6.767);
#6797=CYLINDRICAL_SURFACE('',#7449,6.767);
#6798=CYLINDRICAL_SURFACE('',#7450,6.767);
#6799=CYLINDRICAL_SURFACE('',#7451,6.767);
#6800=CYLINDRICAL_SURFACE('',#7452,6.767);
#6801=CYLINDRICAL_SURFACE('',#7453,6.767);
#6802=CYLINDRICAL_SURFACE('',#7454,6.767);
#6803=CYLINDRICAL_SURFACE('',#7455,6.767);
#6804=CYLINDRICAL_SURFACE('',#7456,6.767);
#6805=CYLINDRICAL_SURFACE('',#7457,6.767);
#6806=CYLINDRICAL_SURFACE('',#7458,6.767);
#6807=CYLINDRICAL_SURFACE('',#7459,6.767);
#6808=CYLINDRICAL_SURFACE('',#7460,6.767);
#6809=CYLINDRICAL_SURFACE('',#7461,6.767);
#6810=CYLINDRICAL_SURFACE('',#7462,6.767);
#6811=CYLINDRICAL_SURFACE('',#7463,6.767);
#6812=CYLINDRICAL_SURFACE('',#7464,6.767);
#6813=CYLINDRICAL_SURFACE('',#7465,6.767);
#6814=CYLINDRICAL_SURFACE('',#7466,6.767);
#6815=CYLINDRICAL_SURFACE('',#7467,6.767);
#6816=CYLINDRICAL_SURFACE('',#7468,6.767);
#6817=CYLINDRICAL_SURFACE('',#7469,6.767);
#6818=CYLINDRICAL_SURFACE('',#7470,6.767);
#6819=CYLINDRICAL_SURFACE('',#7471,6.767);
#6820=CYLINDRICAL_SURFACE('',#7472,6.767);
#6821=CYLINDRICAL_SURFACE('',#7473,6.767);
#6822=CYLINDRICAL_SURFACE('',#7474,6.767);
#6823=CYLINDRICAL_SURFACE('',#7475,6.767);
#6824=CYLINDRICAL_SURFACE('',#7476,6.767);
#6825=CYLINDRICAL_SURFACE('',#7477,6.767);
#6826=CYLINDRICAL_SURFACE('',#7479,7.911);
#6827=CYLINDRICAL_SURFACE('',#7482,4.);
#6828=CYLINDRICAL_SURFACE('',#7489,5.);
#6829=CYLINDRICAL_SURFACE('',#7491,5.);
#6830=CYLINDRICAL_SURFACE('',#7499,10.);
#6831=CYLINDRICAL_SURFACE('',#7502,8.);
#6832=CYLINDRICAL_SURFACE('',#7505,8.);
#6833=CYLINDRICAL_SURFACE('',#7508,8.);
#6834=CYLINDRICAL_SURFACE('',#7511,8.);
#6835=CYLINDRICAL_SURFACE('',#7524,45.);
#6955=ADVANCED_FACE('',(#1090),#6748,.T.);
#6956=ADVANCED_FACE('',(#1091),#6749,.T.);
#6957=ADVANCED_FACE('',(#1092),#6750,.T.);
#6958=ADVANCED_FACE('',(#1093),#6751,.T.);
#6959=ADVANCED_FACE('',(#1094),#6752,.T.);
#6960=ADVANCED_FACE('',(#1095),#6753,.T.);
#6961=ADVANCED_FACE('',(#1096),#6754,.T.);
#6962=ADVANCED_FACE('',(#1097),#6755,.T.);
#6963=ADVANCED_FACE('',(#1098),#6756,.T.);
#6964=ADVANCED_FACE('',(#1099),#6757,.T.);
#6965=ADVANCED_FACE('',(#1100),#6758,.T.);
#6966=ADVANCED_FACE('',(#1101),#6759,.T.);
#6967=ADVANCED_FACE('',(#1102),#6760,.T.);
#6968=ADVANCED_FACE('',(#1103),#6761,.T.);
#6969=ADVANCED_FACE('',(#1104),#6762,.T.);
#6970=ADVANCED_FACE('',(#1105),#6763,.T.);
#6971=ADVANCED_FACE('',(#1106),#6764,.T.);
#6972=ADVANCED_FACE('',(#1107),#6765,.T.);
#6973=ADVANCED_FACE('',(#1108),#6766,.T.);
#6974=ADVANCED_FACE('',(#1109),#6767,.T.);
#6975=ADVANCED_FACE('',(#1110),#6768,.T.);
#6976=ADVANCED_FACE('',(#1111),#6769,.T.);
#6977=ADVANCED_FACE('',(#1112),#6770,.T.);
#6978=ADVANCED_FACE('',(#1113),#6771,.T.);
#6979=ADVANCED_FACE('',(#1114),#6772,.T.);
#6980=ADVANCED_FACE('',(#1115),#6773,.T.);
#6981=ADVANCED_FACE('',(#1116),#6774,.T.);
#6982=ADVANCED_FACE('',(#1117),#6775,.T.);
#6983=ADVANCED_FACE('',(#1118),#6776,.T.);
#6984=ADVANCED_FACE('',(#1119),#6777,.T.);
#6985=ADVANCED_FACE('',(#1120),#6778,.T.);
#6986=ADVANCED_FACE('',(#1121),#6779,.T.);
#6987=ADVANCED_FACE('',(#1122),#6780,.T.);
#6988=ADVANCED_FACE('',(#1123),#6781,.T.);
#6989=ADVANCED_FACE('',(#1124),#6782,.T.);
#6990=ADVANCED_FACE('',(#1125),#6783,.T.);
#6991=ADVANCED_FACE('',(#1126),#6784,.T.);
#6992=ADVANCED_FACE('',(#1127),#6785,.T.);
#6993=ADVANCED_FACE('',(#1128),#6786,.T.);
#6994=ADVANCED_FACE('',(#1129),#6787,.T.);
#6995=ADVANCED_FACE('',(#1130),#6788,.T.);
#6996=ADVANCED_FACE('',(#1131),#6789,.T.);
#6997=ADVANCED_FACE('',(#1132),#6790,.T.);
#6998=ADVANCED_FACE('',(#1133),#6791,.T.);
#6999=ADVANCED_FACE('',(#1134),#6792,.T.);
#7000=ADVANCED_FACE('',(#1135),#6793,.T.);
#7001=ADVANCED_FACE('',(#1136),#6794,.T.);
#7002=ADVANCED_FACE('',(#1137),#6795,.T.);
#7003=ADVANCED_FACE('',(#1138),#6796,.T.);
#7004=ADVANCED_FACE('',(#1139),#6797,.T.);
#7005=ADVANCED_FACE('',(#1140),#6798,.T.);
#7006=ADVANCED_FACE('',(#1141),#6799,.T.);
#7007=ADVANCED_FACE('',(#1142),#6800,.T.);
#7008=ADVANCED_FACE('',(#1143),#6801,.T.);
#7009=ADVANCED_FACE('',(#1144),#6802,.T.);
#7010=ADVANCED_FACE('',(#1145),#6803,.T.);
#7011=ADVANCED_FACE('',(#1146),#6804,.T.);
#7012=ADVANCED_FACE('',(#1147),#6805,.T.);
#7013=ADVANCED_FACE('',(#1148),#6806,.T.);
#7014=ADVANCED_FACE('',(#1149),#6807,.T.);
#7015=ADVANCED_FACE('',(#1150),#6808,.T.);
#7016=ADVANCED_FACE('',(#1151),#6809,.T.);
#7017=ADVANCED_FACE('',(#1152),#6810,.T.);
#7018=ADVANCED_FACE('',(#1153),#6811,.T.);
#7019=ADVANCED_FACE('',(#1154),#6812,.T.);
#7020=ADVANCED_FACE('',(#1155),#6813,.T.);
#7021=ADVANCED_FACE('',(#1156),#6814,.T.);
#7022=ADVANCED_FACE('',(#1157),#6815,.T.);
#7023=ADVANCED_FACE('',(#1158),#6816,.T.);
#7024=ADVANCED_FACE('',(#1159),#6817,.T.);
#7025=ADVANCED_FACE('',(#1160),#6818,.T.);
#7026=ADVANCED_FACE('',(#1161),#6819,.T.);
#7027=ADVANCED_FACE('',(#1162),#6820,.T.);
#7028=ADVANCED_FACE('',(#1163),#6821,.T.);
#7029=ADVANCED_FACE('',(#1164),#6822,.T.);
#7030=ADVANCED_FACE('',(#1165),#6823,.T.);
#7031=ADVANCED_FACE('',(#1166),#6824,.T.);
#7032=ADVANCED_FACE('',(#1167),#6825,.T.);
#7033=ADVANCED_FACE('',(#1168),#6826,.T.);
#7034=ADVANCED_FACE('',(#1169),#6827,.T.);
#7035=ADVANCED_FACE('',(#1170,#959),#1012,.F.);
#7036=ADVANCED_FACE('',(#1171,#960),#1013,.F.);
#7037=ADVANCED_FACE('',(#1172),#6828,.T.);
#7038=ADVANCED_FACE('',(#1173),#6829,.T.);
#7039=ADVANCED_FACE('',(#1174),#1014,.T.);
#7040=ADVANCED_FACE('',(#1175,#961),#1015,.F.);
#7041=ADVANCED_FACE('',(#1176),#6830,.T.);
#7042=ADVANCED_FACE('',(#1177,#962),#1016,.T.);
#7043=ADVANCED_FACE('',(#1178),#6831,.F.);
#7044=ADVANCED_FACE('',(#1179),#6832,.F.);
#7045=ADVANCED_FACE('',(#1180),#6833,.F.);
#7046=ADVANCED_FACE('',(#1181),#6834,.F.);
#7047=ADVANCED_FACE('',(#1182),#105,.T.);
#7048=ADVANCED_FACE('',(#1183),#95,.F.);
#7049=ADVANCED_FACE('',(#1184),#96,.F.);
#7050=ADVANCED_FACE('',(#1185),#1017,.F.);
#7051=ADVANCED_FACE('',(#1186),#1018,.F.);
#7052=ADVANCED_FACE('',(#1187),#1019,.F.);
#7053=ADVANCED_FACE('',(#1188),#1020,.F.);
#7054=ADVANCED_FACE('',(#1189),#1021,.F.);
#7055=ADVANCED_FACE('',(#1190),#1022,.F.);
#7056=ADVANCED_FACE('',(#1191),#1023,.F.);
#7057=ADVANCED_FACE('',(#1192,#963,#964,#965,#966,#967),#1024,.T.);
#7058=ADVANCED_FACE('',(#1193),#6835,.T.);
#7059=ADVANCED_FACE('',(#1194,#968,#969,#970,#971,#972),#1025,.F.);
#7205=CLOSED_SHELL('',(#6955,#6956,#6957,#6958,#6959,#6960,#6961,#6962,
#6963,#6964,#6965,#6966,#6967,#6968,#6969,#6970,#6971,#6972,#6973,#6974,
#6975,#6976,#6977,#6978,#6979,#6980,#6981,#6982,#6983,#6984,#6985,#6986,
#6987,#6988,#6989,#6990,#6991,#6992,#6993,#6994,#6995,#6996,#6997,#6998,
#6999,#7000,#7001,#7002,#7003,#7004,#7005,#7006,#7007,#7008,#7009,#7010,
#7011,#7012,#7013,#7014,#7015,#7016,#7017,#7018,#7019,#7020,#7021,#7022,
#7023,#7024,#7025,#7026,#7027,#7028,#7029,#7030,#7031,#7032,#7033,#7034,
#7035,#7036,#7037,#7038,#7039,#7040,#7041,#7042,#7043,#7044,#7045,#7046,
#7047,#7048,#7049,#7050,#7051,#7052,#7053,#7054,#7055,#7056,#7057,#7058,
#7059));
#7398=AXIS2_PLACEMENT_3D('',#8939,#7880,#7881);
#7399=AXIS2_PLACEMENT_3D('',#8940,#7882,#7883);
#7400=AXIS2_PLACEMENT_3D('',#9079,#7885,#7886);
#7401=AXIS2_PLACEMENT_3D('',#9156,#7887,#7888);
#7402=AXIS2_PLACEMENT_3D('',#9652,#7890,#7891);
#7403=AXIS2_PLACEMENT_3D('',#10154,#7893,#7894);
#7404=AXIS2_PLACEMENT_3D('',#10665,#7896,#7897);
#7405=AXIS2_PLACEMENT_3D('',#11158,#7899,#7900);
#7406=AXIS2_PLACEMENT_3D('',#11651,#7902,#7903);
#7407=AXIS2_PLACEMENT_3D('',#12150,#7905,#7906);
#7408=AXIS2_PLACEMENT_3D('',#12649,#7908,#7909);
#7409=AXIS2_PLACEMENT_3D('',#13139,#7911,#7912);
#7410=AXIS2_PLACEMENT_3D('',#13626,#7914,#7915);
#7411=AXIS2_PLACEMENT_3D('',#14131,#7917,#7918);
#7412=AXIS2_PLACEMENT_3D('',#14636,#7920,#7921);
#7413=AXIS2_PLACEMENT_3D('',#15138,#7923,#7924);
#7414=AXIS2_PLACEMENT_3D('',#15634,#7926,#7927);
#7415=AXIS2_PLACEMENT_3D('',#16127,#7929,#7930);
#7416=AXIS2_PLACEMENT_3D('',#16617,#7932,#7933);
#7417=AXIS2_PLACEMENT_3D('',#17119,#7935,#7936);
#7418=AXIS2_PLACEMENT_3D('',#17633,#7938,#7939);
#7419=AXIS2_PLACEMENT_3D('',#18132,#7941,#7942);
#7420=AXIS2_PLACEMENT_3D('',#18619,#7944,#7945);
#7421=AXIS2_PLACEMENT_3D('',#19112,#7947,#7948);
#7422=AXIS2_PLACEMENT_3D('',#19620,#7950,#7951);
#7423=AXIS2_PLACEMENT_3D('',#20119,#7953,#7954);
#7424=AXIS2_PLACEMENT_3D('',#20621,#7956,#7957);
#7425=AXIS2_PLACEMENT_3D('',#21108,#7959,#7960);
#7426=AXIS2_PLACEMENT_3D('',#21592,#7962,#7963);
#7427=AXIS2_PLACEMENT_3D('',#22094,#7965,#7966);
#7428=AXIS2_PLACEMENT_3D('',#22602,#7968,#7969);
#7429=AXIS2_PLACEMENT_3D('',#23110,#7971,#7972);
#7430=AXIS2_PLACEMENT_3D('',#23594,#7974,#7975);
#7431=AXIS2_PLACEMENT_3D('',#24087,#7977,#7978);
#7432=AXIS2_PLACEMENT_3D('',#24598,#7980,#7981);
#7433=AXIS2_PLACEMENT_3D('',#25109,#7983,#7984);
#7434=AXIS2_PLACEMENT_3D('',#25605,#7986,#7987);
#7435=AXIS2_PLACEMENT_3D('',#26086,#7989,#7990);
#7436=AXIS2_PLACEMENT_3D('',#26585,#7992,#7993);
#7437=AXIS2_PLACEMENT_3D('',#27084,#7995,#7996);
#7438=AXIS2_PLACEMENT_3D('',#27580,#7998,#7999);
#7439=AXIS2_PLACEMENT_3D('',#28097,#8001,#8002);
#7440=AXIS2_PLACEMENT_3D('',#28581,#8004,#8005);
#7441=AXIS2_PLACEMENT_3D('',#29074,#8007,#8008);
#7442=AXIS2_PLACEMENT_3D('',#29576,#8010,#8011);
#7443=AXIS2_PLACEMENT_3D('',#30075,#8013,#8014);
#7444=AXIS2_PLACEMENT_3D('',#30562,#8016,#8017);
#7445=AXIS2_PLACEMENT_3D('',#30895,#8019,#8020);
#7446=AXIS2_PLACEMENT_3D('',#31333,#8022,#8023);
#7447=AXIS2_PLACEMENT_3D('',#31829,#8025,#8026);
#7448=AXIS2_PLACEMENT_3D('',#32331,#8028,#8029);
#7449=AXIS2_PLACEMENT_3D('',#32833,#8031,#8032);
#7450=AXIS2_PLACEMENT_3D('',#33335,#8034,#8035);
#7451=AXIS2_PLACEMENT_3D('',#33831,#8037,#8038);
#7452=AXIS2_PLACEMENT_3D('',#34333,#8040,#8041);
#7453=AXIS2_PLACEMENT_3D('',#34835,#8043,#8044);
#7454=AXIS2_PLACEMENT_3D('',#35322,#8046,#8047);
#7455=AXIS2_PLACEMENT_3D('',#35827,#8049,#8050);
#7456=AXIS2_PLACEMENT_3D('',#36329,#8052,#8053);
#7457=AXIS2_PLACEMENT_3D('',#36819,#8055,#8056);
#7458=AXIS2_PLACEMENT_3D('',#37306,#8058,#8059);
#7459=AXIS2_PLACEMENT_3D('',#37808,#8061,#8062);
#7460=AXIS2_PLACEMENT_3D('',#38319,#8064,#8065);
#7461=AXIS2_PLACEMENT_3D('',#38815,#8067,#8068);
#7462=AXIS2_PLACEMENT_3D('',#39305,#8070,#8071);
#7463=AXIS2_PLACEMENT_3D('',#39795,#8073,#8074);
#7464=AXIS2_PLACEMENT_3D('',#40294,#8076,#8077);
#7465=AXIS2_PLACEMENT_3D('',#40793,#8079,#8080);
#7466=AXIS2_PLACEMENT_3D('',#41286,#8082,#8083);
#7467=AXIS2_PLACEMENT_3D('',#41779,#8085,#8086);
#7468=AXIS2_PLACEMENT_3D('',#42284,#8088,#8089);
#7469=AXIS2_PLACEMENT_3D('',#42777,#8091,#8092);
#7470=AXIS2_PLACEMENT_3D('',#43285,#8094,#8095);
#7471=AXIS2_PLACEMENT_3D('',#43784,#8097,#8098);
#7472=AXIS2_PLACEMENT_3D('',#44271,#8100,#8101);
#7473=AXIS2_PLACEMENT_3D('',#44770,#8103,#8104);
#7474=AXIS2_PLACEMENT_3D('',#45266,#8106,#8107);
#7475=AXIS2_PLACEMENT_3D('',#45768,#8109,#8110);
#7476=AXIS2_PLACEMENT_3D('',#46270,#8112,#8113);
#7477=AXIS2_PLACEMENT_3D('',#46775,#8115,#8116);
#7478=AXIS2_PLACEMENT_3D('',#46943,#8117,#8118);
#7479=AXIS2_PLACEMENT_3D('',#47064,#8119,#8120);
#7480=AXIS2_PLACEMENT_3D('',#47076,#8121,#8122);
#7481=AXIS2_PLACEMENT_3D('',#53093,#8123,#8124);
#7482=AXIS2_PLACEMENT_3D('',#66980,#8125,#8126);
#7483=AXIS2_PLACEMENT_3D('',#66982,#8127,#8128);
#7484=AXIS2_PLACEMENT_3D('',#66985,#8130,#8131);
#7485=AXIS2_PLACEMENT_3D('',#66986,#8132,#8133);
#7486=AXIS2_PLACEMENT_3D('',#66988,#8134,#8135);
#7487=AXIS2_PLACEMENT_3D('',#66989,#8136,#8137);
#7488=AXIS2_PLACEMENT_3D('',#66991,#8138,#8139);
#7489=AXIS2_PLACEMENT_3D('',#66992,#8140,#8141);
#7490=AXIS2_PLACEMENT_3D('',#66994,#8142,#8143);
#7491=AXIS2_PLACEMENT_3D('',#66996,#8145,#8146);
#7492=AXIS2_PLACEMENT_3D('',#66999,#8148,#8149);
#7493=AXIS2_PLACEMENT_3D('',#67000,#8150,#8151);
#7494=AXIS2_PLACEMENT_3D('',#67001,#8152,#8153);
#7495=AXIS2_PLACEMENT_3D('',#67003,#8154,#8155);
#7496=AXIS2_PLACEMENT_3D('',#67006,#8156,#8157);
#7497=AXIS2_PLACEMENT_3D('',#67007,#8158,#8159);
#7498=AXIS2_PLACEMENT_3D('',#67008,#8160,#8161);
#7499=AXIS2_PLACEMENT_3D('',#67009,#8162,#8163);
#7500=AXIS2_PLACEMENT_3D('',#67011,#8164,#8165);
#7501=AXIS2_PLACEMENT_3D('',#67013,#8167,#8168);
#7502=AXIS2_PLACEMENT_3D('',#67014,#8169,#8170);
#7503=AXIS2_PLACEMENT_3D('',#67016,#8171,#8172);
#7504=AXIS2_PLACEMENT_3D('',#67019,#8174,#8175);
#7505=AXIS2_PLACEMENT_3D('',#67020,#8176,#8177);
#7506=AXIS2_PLACEMENT_3D('',#67022,#8178,#8179);
#7507=AXIS2_PLACEMENT_3D('',#67025,#8181,#8182);
#7508=AXIS2_PLACEMENT_3D('',#67026,#8183,#8184);
#7509=AXIS2_PLACEMENT_3D('',#67028,#8185,#8186);
#7510=AXIS2_PLACEMENT_3D('',#67031,#8188,#8189);
#7511=AXIS2_PLACEMENT_3D('',#67032,#8190,#8191);
#7512=AXIS2_PLACEMENT_3D('',#67034,#8192,#8193);
#7513=AXIS2_PLACEMENT_3D('',#67037,#8195,#8196);
#7514=AXIS2_PLACEMENT_3D('',#67038,#8197,#8198);
#7515=AXIS2_PLACEMENT_3D('',#71825,#8199,#8200);
#7516=AXIS2_PLACEMENT_3D('',#71834,#8205,#8206);
#7517=AXIS2_PLACEMENT_3D('',#71840,#8210,#8211);
#7518=AXIS2_PLACEMENT_3D('',#71846,#8215,#8216);
#7519=AXIS2_PLACEMENT_3D('',#71852,#8220,#8221);
#7520=AXIS2_PLACEMENT_3D('',#71858,#8225,#8226);
#7521=AXIS2_PLACEMENT_3D('',#71861,#8229,#8230);
#7522=AXIS2_PLACEMENT_3D('',#71862,#8231,#8232);
#7523=AXIS2_PLACEMENT_3D('',#71864,#8233,#8234);
#7524=AXIS2_PLACEMENT_3D('',#71865,#8235,#8236);
#7525=AXIS2_PLACEMENT_3D('',#71868,#8238,#8239);
#7526=AXIS2_PLACEMENT_3D('',#71869,#8240,#8241);
#7880=DIRECTION('axis',(0.,0.,1.));
#7881=DIRECTION('refdir',(1.,0.,0.));
#7882=DIRECTION('center_axis',(0.,0.,1.));
#7883=DIRECTION('ref_axis',(-0.457983707777832,-0.888960585971093,0.));
#7884=DIRECTION('',(0.,0.,-1.));
#7885=DIRECTION('center_axis',(0.,0.,-1.));
#7886=DIRECTION('ref_axis',(1.,-1.35784937511192E-12,0.));
#7887=DIRECTION('center_axis',(0.,0.,1.));
#7888=DIRECTION('ref_axis',(-0.457983707777832,-0.888960585971093,0.));
#7889=DIRECTION('',(0.,0.,-1.));
#7890=DIRECTION('center_axis',(0.,0.,1.));
#7891=DIRECTION('ref_axis',(-0.457983707777832,-0.888960585971093,0.));
#7892=DIRECTION('',(0.,0.,-1.));
#7893=DIRECTION('center_axis',(0.,0.,1.));
#7894=DIRECTION('ref_axis',(-0.457983707777832,-0.888960585971093,0.));
#7895=DIRECTION('',(0.,0.,-1.));
#7896=DIRECTION('center_axis',(0.,0.,1.));
#7897=DIRECTION('ref_axis',(-0.457983707777832,-0.888960585971093,0.));
#7898=DIRECTION('',(0.,0.,-1.));
#7899=DIRECTION('center_axis',(0.,0.,1.));
#7900=DIRECTION('ref_axis',(-0.457983707777832,-0.888960585971093,0.));
#7901=DIRECTION('',(0.,0.,-1.));
#7902=DIRECTION('center_axis',(0.,0.,1.));
#7903=DIRECTION('ref_axis',(-0.457983707777832,-0.888960585971093,0.));
#7904=DIRECTION('',(0.,0.,-1.));
#7905=DIRECTION('center_axis',(0.,0.,1.));
#7906=DIRECTION('ref_axis',(-0.457983707777832,-0.888960585971093,0.));
#7907=DIRECTION('',(0.,0.,-1.));
#7908=DIRECTION('center_axis',(0.,0.,1.));
#7909=DIRECTION('ref_axis',(-0.457983707777832,-0.888960585971093,0.));
#7910=DIRECTION('',(0.,0.,-1.));
#7911=DIRECTION('center_axis',(0.,0.,1.));
#7912=DIRECTION('ref_axis',(-0.457983707777832,-0.888960585971093,0.));
#7913=DIRECTION('',(0.,0.,-1.));
#7914=DIRECTION('center_axis',(0.,0.,1.));
#7915=DIRECTION('ref_axis',(-0.457983707777832,-0.888960585971093,0.));
#7916=DIRECTION('',(0.,0.,-1.));
#7917=DIRECTION('center_axis',(0.,0.,1.));
#7918=DIRECTION('ref_axis',(-0.457983707777832,-0.888960585971093,0.));
#7919=DIRECTION('',(0.,0.,-1.));
#7920=DIRECTION('center_axis',(0.,0.,1.));
#7921=DIRECTION('ref_axis',(-0.457983707777832,-0.888960585971093,0.));
#7922=DIRECTION('',(0.,0.,-1.));
#7923=DIRECTION('center_axis',(0.,0.,1.));
#7924=DIRECTION('ref_axis',(-0.457983707777832,-0.888960585971093,0.));
#7925=DIRECTION('',(0.,0.,-1.));
#7926=DIRECTION('center_axis',(0.,0.,1.));
#7927=DIRECTION('ref_axis',(-0.457983707777832,-0.888960585971093,0.));
#7928=DIRECTION('',(0.,0.,-1.));
#7929=DIRECTION('center_axis',(0.,0.,1.));
#7930=DIRECTION('ref_axis',(-0.457983707777832,-0.888960585971093,0.));
#7931=DIRECTION('',(0.,0.,-1.));
#7932=DIRECTION('center_axis',(0.,0.,1.));
#7933=DIRECTION('ref_axis',(-0.457983707777832,-0.888960585971093,0.));
#7934=DIRECTION('',(0.,0.,-1.));
#7935=DIRECTION('center_axis',(0.,0.,1.));
#7936=DIRECTION('ref_axis',(-0.457983707777832,-0.888960585971093,0.));
#7937=DIRECTION('',(0.,0.,-1.));
#7938=DIRECTION('center_axis',(0.,0.,1.));
#7939=DIRECTION('ref_axis',(-0.457983707777832,-0.888960585971093,0.));
#7940=DIRECTION('',(0.,0.,-1.));
#7941=DIRECTION('center_axis',(0.,0.,1.));
#7942=DIRECTION('ref_axis',(-0.457983707777832,-0.888960585971093,0.));
#7943=DIRECTION('',(0.,0.,-1.));
#7944=DIRECTION('center_axis',(0.,0.,1.));
#7945=DIRECTION('ref_axis',(-0.457983707777832,-0.888960585971093,0.));
#7946=DIRECTION('',(0.,0.,-1.));
#7947=DIRECTION('center_axis',(0.,0.,1.));
#7948=DIRECTION('ref_axis',(-0.457983707777832,-0.888960585971093,0.));
#7949=DIRECTION('',(0.,0.,-1.));
#7950=DIRECTION('center_axis',(0.,0.,1.));
#7951=DIRECTION('ref_axis',(-0.457983707777832,-0.888960585971093,0.));
#7952=DIRECTION('',(0.,0.,-1.));
#7953=DIRECTION('center_axis',(0.,0.,1.));
#7954=DIRECTION('ref_axis',(-0.457983707777832,-0.888960585971093,0.));
#7955=DIRECTION('',(0.,0.,-1.));
#7956=DIRECTION('center_axis',(0.,0.,1.));
#7957=DIRECTION('ref_axis',(-0.457983707777832,-0.888960585971093,0.));
#7958=DIRECTION('',(0.,0.,-1.));
#7959=DIRECTION('center_axis',(0.,0.,1.));
#7960=DIRECTION('ref_axis',(-0.457983707777832,-0.888960585971093,0.));
#7961=DIRECTION('',(0.,0.,-1.));
#7962=DIRECTION('center_axis',(0.,0.,1.));
#7963=DIRECTION('ref_axis',(-0.457983707777832,-0.888960585971093,0.));
#7964=DIRECTION('',(0.,0.,-1.));
#7965=DIRECTION('center_axis',(0.,0.,1.));
#7966=DIRECTION('ref_axis',(-0.457983707777832,-0.888960585971093,0.));
#7967=DIRECTION('',(0.,0.,-1.));
#7968=DIRECTION('center_axis',(0.,0.,1.));
#7969=DIRECTION('ref_axis',(-0.457983707777832,-0.888960585971093,0.));
#7970=DIRECTION('',(0.,0.,-1.));
#7971=DIRECTION('center_axis',(0.,0.,1.));
#7972=DIRECTION('ref_axis',(-0.457983707777832,-0.888960585971093,0.));
#7973=DIRECTION('',(0.,0.,-1.));
#7974=DIRECTION('center_axis',(0.,0.,1.));
#7975=DIRECTION('ref_axis',(-0.457983707777832,-0.888960585971093,0.));
#7976=DIRECTION('',(0.,0.,-1.));
#7977=DIRECTION('center_axis',(0.,0.,1.));
#7978=DIRECTION('ref_axis',(-0.457983707777832,-0.888960585971093,0.));
#7979=DIRECTION('',(0.,0.,-1.));
#7980=DIRECTION('center_axis',(0.,0.,1.));
#7981=DIRECTION('ref_axis',(-0.457983707777832,-0.888960585971093,0.));
#7982=DIRECTION('',(0.,0.,-1.));
#7983=DIRECTION('center_axis',(0.,0.,1.));
#7984=DIRECTION('ref_axis',(-0.457983707777832,-0.888960585971093,0.));
#7985=DIRECTION('',(0.,0.,-1.));
#7986=DIRECTION('center_axis',(0.,0.,1.));
#7987=DIRECTION('ref_axis',(-0.457983707777832,-0.888960585971093,0.));
#7988=DIRECTION('',(0.,0.,-1.));
#7989=DIRECTION('center_axis',(0.,0.,1.));
#7990=DIRECTION('ref_axis',(-0.457983707777832,-0.888960585971093,0.));
#7991=DIRECTION('',(0.,0.,-1.));
#7992=DIRECTION('center_axis',(0.,0.,1.));
#7993=DIRECTION('ref_axis',(-0.457983707777832,-0.888960585971093,0.));
#7994=DIRECTION('',(0.,0.,-1.));
#7995=DIRECTION('center_axis',(0.,0.,1.));
#7996=DIRECTION('ref_axis',(-0.457983707777832,-0.888960585971093,0.));
#7997=DIRECTION('',(0.,0.,-1.));
#7998=DIRECTION('center_axis',(0.,0.,1.));
#7999=DIRECTION('ref_axis',(-0.457983707777832,-0.888960585971093,0.));
#8000=DIRECTION('',(0.,0.,-1.));
#8001=DIRECTION('center_axis',(0.,0.,1.));
#8002=DIRECTION('ref_axis',(-0.457983707777832,-0.888960585971093,0.));
#8003=DIRECTION('',(0.,0.,-1.));
#8004=DIRECTION('center_axis',(0.,0.,1.));
#8005=DIRECTION('ref_axis',(-0.457983707777832,-0.888960585971093,0.));
#8006=DIRECTION('',(0.,0.,-1.));
#8007=DIRECTION('center_axis',(0.,0.,1.));
#8008=DIRECTION('ref_axis',(-0.457983707777832,-0.888960585971093,0.));
#8009=DIRECTION('',(0.,0.,-1.));
#8010=DIRECTION('center_axis',(0.,0.,1.));
#8011=DIRECTION('ref_axis',(-0.457983707777832,-0.888960585971093,0.));
#8012=DIRECTION('',(0.,0.,-1.));
#8013=DIRECTION('center_axis',(0.,0.,1.));
#8014=DIRECTION('ref_axis',(-0.457983707777832,-0.888960585971093,0.));
#8015=DIRECTION('',(0.,0.,-1.));
#8016=DIRECTION('center_axis',(0.,0.,1.));
#8017=DIRECTION('ref_axis',(-0.457983707777832,-0.888960585971093,0.));
#8018=DIRECTION('',(0.,0.,-1.));
#8019=DIRECTION('center_axis',(0.,0.,1.));
#8020=DIRECTION('ref_axis',(-0.457983707777832,-0.888960585971093,0.));
#8021=DIRECTION('',(0.,0.,-1.));
#8022=DIRECTION('center_axis',(0.,0.,1.));
#8023=DIRECTION('ref_axis',(-0.457983707777832,-0.888960585971093,0.));
#8024=DIRECTION('',(0.,0.,-1.));
#8025=DIRECTION('center_axis',(0.,0.,1.));
#8026=DIRECTION('ref_axis',(-0.457983707777832,-0.888960585971093,0.));
#8027=DIRECTION('',(0.,0.,-1.));
#8028=DIRECTION('center_axis',(0.,0.,1.));
#8029=DIRECTION('ref_axis',(-0.457983707777832,-0.888960585971093,0.));
#8030=DIRECTION('',(0.,0.,-1.));
#8031=DIRECTION('center_axis',(0.,0.,1.));
#8032=DIRECTION('ref_axis',(-0.457983707777832,-0.888960585971093,0.));
#8033=DIRECTION('',(0.,0.,-1.));
#8034=DIRECTION('center_axis',(0.,0.,1.));
#8035=DIRECTION('ref_axis',(-0.457983707777832,-0.888960585971093,0.));
#8036=DIRECTION('',(0.,0.,-1.));
#8037=DIRECTION('center_axis',(0.,0.,1.));
#8038=DIRECTION('ref_axis',(-0.457983707777832,-0.888960585971093,0.));
#8039=DIRECTION('',(0.,0.,-1.));
#8040=DIRECTION('center_axis',(0.,0.,1.));
#8041=DIRECTION('ref_axis',(-0.457983707777832,-0.888960585971093,0.));
#8042=DIRECTION('',(0.,0.,-1.));
#8043=DIRECTION('center_axis',(0.,0.,1.));
#8044=DIRECTION('ref_axis',(-0.457983707777832,-0.888960585971093,0.));
#8045=DIRECTION('',(0.,0.,-1.));
#8046=DIRECTION('center_axis',(0.,0.,1.));
#8047=DIRECTION('ref_axis',(-0.457983707777832,-0.888960585971093,0.));
#8048=DIRECTION('',(0.,0.,-1.));
#8049=DIRECTION('center_axis',(0.,0.,1.));
#8050=DIRECTION('ref_axis',(-0.457983707777832,-0.888960585971093,0.));
#8051=DIRECTION('',(0.,0.,-1.));
#8052=DIRECTION('center_axis',(0.,0.,1.));
#8053=DIRECTION('ref_axis',(-0.457983707777832,-0.888960585971093,0.));
#8054=DIRECTION('',(0.,0.,-1.));
#8055=DIRECTION('center_axis',(0.,0.,1.));
#8056=DIRECTION('ref_axis',(-0.457983707777832,-0.888960585971093,0.));
#8057=DIRECTION('',(0.,0.,-1.));
#8058=DIRECTION('center_axis',(0.,0.,1.));
#8059=DIRECTION('ref_axis',(-0.457983707777832,-0.888960585971093,0.));
#8060=DIRECTION('',(0.,0.,-1.));
#8061=DIRECTION('center_axis',(0.,0.,1.));
#8062=DIRECTION('ref_axis',(-0.457983707777832,-0.888960585971093,0.));
#8063=DIRECTION('',(0.,0.,-1.));
#8064=DIRECTION('center_axis',(0.,0.,1.));
#8065=DIRECTION('ref_axis',(-0.457983707777832,-0.888960585971093,0.));
#8066=DIRECTION('',(0.,0.,-1.));
#8067=DIRECTION('center_axis',(0.,0.,1.));
#8068=DIRECTION('ref_axis',(-0.457983707777832,-0.888960585971093,0.));
#8069=DIRECTION('',(0.,0.,-1.));
#8070=DIRECTION('center_axis',(0.,0.,1.));
#8071=DIRECTION('ref_axis',(-0.457983707777832,-0.888960585971093,0.));
#8072=DIRECTION('',(0.,0.,-1.));
#8073=DIRECTION('center_axis',(0.,0.,1.));
#8074=DIRECTION('ref_axis',(-0.457983707777832,-0.888960585971093,0.));
#8075=DIRECTION('',(0.,0.,-1.));
#8076=DIRECTION('center_axis',(0.,0.,1.));
#8077=DIRECTION('ref_axis',(-0.457983707777832,-0.888960585971093,0.));
#8078=DIRECTION('',(0.,0.,-1.));
#8079=DIRECTION('center_axis',(0.,0.,1.));
#8080=DIRECTION('ref_axis',(-0.457983707777832,-0.888960585971093,0.));
#8081=DIRECTION('',(0.,0.,-1.));
#8082=DIRECTION('center_axis',(0.,0.,1.));
#8083=DIRECTION('ref_axis',(-0.457983707777832,-0.888960585971093,0.));
#8084=DIRECTION('',(0.,0.,-1.));
#8085=DIRECTION('center_axis',(0.,0.,1.));
#8086=DIRECTION('ref_axis',(-0.457983707777832,-0.888960585971093,0.));
#8087=DIRECTION('',(0.,0.,-1.));
#8088=DIRECTION('center_axis',(0.,0.,1.));
#8089=DIRECTION('ref_axis',(-0.457983707777832,-0.888960585971093,0.));
#8090=DIRECTION('',(0.,0.,-1.));
#8091=DIRECTION('center_axis',(0.,0.,1.));
#8092=DIRECTION('ref_axis',(-0.457983707777832,-0.888960585971093,0.));
#8093=DIRECTION('',(0.,0.,-1.));
#8094=DIRECTION('center_axis',(0.,0.,1.));
#8095=DIRECTION('ref_axis',(-0.457983707777832,-0.888960585971093,0.));
#8096=DIRECTION('',(0.,0.,-1.));
#8097=DIRECTION('center_axis',(0.,0.,1.));
#8098=DIRECTION('ref_axis',(-0.457983707777832,-0.888960585971093,0.));
#8099=DIRECTION('',(0.,0.,-1.));
#8100=DIRECTION('center_axis',(0.,0.,1.));
#8101=DIRECTION('ref_axis',(-0.457983707777832,-0.888960585971093,0.));
#8102=DIRECTION('',(0.,0.,-1.));
#8103=DIRECTION('center_axis',(0.,0.,1.));
#8104=DIRECTION('ref_axis',(-0.457983707777832,-0.888960585971093,0.));
#8105=DIRECTION('',(0.,0.,-1.));
#8106=DIRECTION('center_axis',(0.,0.,1.));
#8107=DIRECTION('ref_axis',(-0.457983707777832,-0.888960585971093,0.));
#8108=DIRECTION('',(0.,0.,-1.));
#8109=DIRECTION('center_axis',(0.,0.,1.));
#8110=DIRECTION('ref_axis',(-0.457983707777832,-0.888960585971093,0.));
#8111=DIRECTION('',(0.,0.,-1.));
#8112=DIRECTION('center_axis',(0.,0.,1.));
#8113=DIRECTION('ref_axis',(-0.457983707777832,-0.888960585971093,0.));
#8114=DIRECTION('',(0.,0.,-1.));
#8115=DIRECTION('center_axis',(0.,0.,1.));
#8116=DIRECTION('ref_axis',(-0.457983707777832,-0.888960585971093,0.));
#8117=DIRECTION('center_axis',(0.,0.,1.));
#8118=DIRECTION('ref_axis',(1.,-1.35784937511192E-12,0.));
#8119=DIRECTION('center_axis',(0.,0.,1.));
#8120=DIRECTION('ref_axis',(1.,0.,0.));
#8121=DIRECTION('center_axis',(0.,0.,-1.));
#8122=DIRECTION('ref_axis',(1.,0.,0.));
#8123=DIRECTION('center_axis',(0.,0.,-1.));
#8124=DIRECTION('ref_axis',(1.,0.,0.));
#8125=DIRECTION('center_axis',(0.,0.,1.));
#8126=DIRECTION('ref_axis',(1.,0.,0.));
#8127=DIRECTION('center_axis',(0.,0.,1.));
#8128=DIRECTION('ref_axis',(1.,0.,0.));
#8129=DIRECTION('',(0.,0.,-1.));
#8130=DIRECTION('center_axis',(0.,0.,1.));
#8131=DIRECTION('ref_axis',(1.,0.,0.));
#8132=DIRECTION('center_axis',(0.,0.,-1.));
#8133=DIRECTION('ref_axis',(-1.,0.,0.));
#8134=DIRECTION('center_axis',(0.,0.,-1.));
#8135=DIRECTION('ref_axis',(1.,0.,0.));
#8136=DIRECTION('center_axis',(0.,0.,1.));
#8137=DIRECTION('ref_axis',(1.,0.,0.));
#8138=DIRECTION('center_axis',(0.,0.,1.));
#8139=DIRECTION('ref_axis',(1.,0.,0.));
#8140=DIRECTION('center_axis',(0.,0.,1.));
#8141=DIRECTION('ref_axis',(1.,0.,0.));
#8142=DIRECTION('center_axis',(0.,0.,1.));
#8143=DIRECTION('ref_axis',(1.,0.,0.));
#8144=DIRECTION('',(0.,0.,-1.));
#8145=DIRECTION('center_axis',(0.,0.,1.));
#8146=DIRECTION('ref_axis',(1.,0.,0.));
#8147=DIRECTION('',(0.,0.,-1.));
#8148=DIRECTION('center_axis',(0.,0.,-1.));
#8149=DIRECTION('ref_axis',(1.,0.,0.));
#8150=DIRECTION('center_axis',(0.,0.,1.));
#8151=DIRECTION('ref_axis',(1.,0.,0.));
#8152=DIRECTION('center_axis',(0.,0.,1.));
#8153=DIRECTION('ref_axis',(1.,0.,0.));
#8154=DIRECTION('center_axis',(0.,0.,1.));
#8155=DIRECTION('ref_axis',(1.,0.,0.));
#8156=DIRECTION('center_axis',(0.,0.,1.));
#8157=DIRECTION('ref_axis',(1.,0.,0.));
#8158=DIRECTION('center_axis',(6.78567850819536E-13,5.53097019214562E-13,
1.));
#8159=DIRECTION('ref_axis',(0.504160107343572,-0.86361020499026,1.35553389634315E-13));
#8160=DIRECTION('center_axis',(-6.40020660077179E-13,6.68075341414769E-13,
1.));
#8161=DIRECTION('ref_axis',(0.774139656364633,0.633014843778287,7.25637659806176E-14));
#8162=DIRECTION('center_axis',(0.,0.,1.));
#8163=DIRECTION('ref_axis',(1.,0.,0.));
#8164=DIRECTION('center_axis',(0.,0.,1.));
#8165=DIRECTION('ref_axis',(1.,0.,0.));
#8166=DIRECTION('',(0.,0.,-1.));
#8167=DIRECTION('center_axis',(0.,0.,1.));
#8168=DIRECTION('ref_axis',(1.,0.,0.));
#8169=DIRECTION('center_axis',(0.,0.,-1.));
#8170=DIRECTION('ref_axis',(1.,0.,0.));
#8171=DIRECTION('center_axis',(0.,0.,-1.));
#8172=DIRECTION('ref_axis',(1.,0.,0.));
#8173=DIRECTION('',(0.,0.,-1.));
#8174=DIRECTION('center_axis',(0.,0.,1.));
#8175=DIRECTION('ref_axis',(1.,0.,0.));
#8176=DIRECTION('center_axis',(0.,0.,-1.));
#8177=DIRECTION('ref_axis',(1.,0.,0.));
#8178=DIRECTION('center_axis',(0.,0.,-1.));
#8179=DIRECTION('ref_axis',(1.,0.,0.));
#8180=DIRECTION('',(0.,0.,-1.));
#8181=DIRECTION('center_axis',(0.,0.,1.));
#8182=DIRECTION('ref_axis',(1.,0.,0.));
#8183=DIRECTION('center_axis',(0.,0.,-1.));
#8184=DIRECTION('ref_axis',(1.,0.,0.));
#8185=DIRECTION('center_axis',(0.,0.,-1.));
#8186=DIRECTION('ref_axis',(1.,0.,0.));
#8187=DIRECTION('',(0.,0.,-1.));
#8188=DIRECTION('center_axis',(0.,0.,1.));
#8189=DIRECTION('ref_axis',(1.,0.,0.));
#8190=DIRECTION('center_axis',(0.,0.,-1.));
#8191=DIRECTION('ref_axis',(1.,0.,0.));
#8192=DIRECTION('center_axis',(0.,0.,-1.));
#8193=DIRECTION('ref_axis',(1.,0.,0.));
#8194=DIRECTION('',(0.,0.,-1.));
#8195=DIRECTION('center_axis',(0.,0.,1.));
#8196=DIRECTION('ref_axis',(1.,0.,0.));
#8197=DIRECTION('center_axis',(0.,0.,-1.));
#8198=DIRECTION('ref_axis',(0.568605661693349,0.822610236679722,0.));
#8199=DIRECTION('center_axis',(-2.40370335797945E-16,-1.,0.));
#8200=DIRECTION('ref_axis',(1.,-2.40370335797945E-16,0.));
#8201=DIRECTION('',(1.,-2.40370335797945E-16,0.));
#8202=DIRECTION('',(0.,0.,1.));
#8203=DIRECTION('',(1.,-2.40370335797945E-16,0.));
#8204=DIRECTION('',(0.,0.,1.));
#8205=DIRECTION('center_axis',(-0.866025403784439,-0.5,0.));
#8206=DIRECTION('ref_axis',(0.5,-0.866025403784439,0.));
#8207=DIRECTION('',(0.5,-0.866025403784439,0.));
#8208=DIRECTION('',(0.,0.,1.));
#8209=DIRECTION('',(0.5,-0.866025403784439,0.));
#8210=DIRECTION('center_axis',(-0.866025403784439,0.5,0.));
#8211=DIRECTION('ref_axis',(-0.5,-0.866025403784439,0.));
#8212=DIRECTION('',(-0.5,-0.866025403784439,0.));
#8213=DIRECTION('',(0.,0.,1.));
#8214=DIRECTION('',(-0.5,-0.866025403784439,0.));
#8215=DIRECTION('center_axis',(1.20185167898973E-16,1.,0.));
#8216=DIRECTION('ref_axis',(-1.,1.20185167898973E-16,0.));
#8217=DIRECTION('',(-1.,1.20185167898973E-16,0.));
#8218=DIRECTION('',(0.,0.,1.));
#8219=DIRECTION('',(-1.,1.20185167898973E-16,0.));
#8220=DIRECTION('center_axis',(0.866025403784439,0.5,0.));
#8221=DIRECTION('ref_axis',(-0.5,0.866025403784439,0.));
#8222=DIRECTION('',(-0.5,0.866025403784439,0.));
#8223=DIRECTION('',(0.,0.,1.));
#8224=DIRECTION('',(-0.5,0.866025403784439,0.));
#8225=DIRECTION('center_axis',(0.866025403784439,-0.5,0.));
#8226=DIRECTION('ref_axis',(0.5,0.866025403784439,0.));
#8227=DIRECTION('',(0.5,0.866025403784439,0.));
#8228=DIRECTION('',(0.5,0.866025403784439,0.));
#8229=DIRECTION('center_axis',(0.,0.,1.));
#8230=DIRECTION('ref_axis',(1.,0.,0.));
#8231=DIRECTION('center_axis',(0.,0.,1.));
#8232=DIRECTION('ref_axis',(1.,0.,0.));
#8233=DIRECTION('center_axis',(0.,0.,-1.));
#8234=DIRECTION('ref_axis',(1.,0.,0.));
#8235=DIRECTION('center_axis',(0.,0.,1.));
#8236=DIRECTION('ref_axis',(1.,0.,0.));
#8237=DIRECTION('',(0.,0.,-1.));
#8238=DIRECTION('center_axis',(0.,0.,-1.));
#8239=DIRECTION('ref_axis',(1.,0.,0.));
#8240=DIRECTION('center_axis',(0.,0.,1.));
#8241=DIRECTION('ref_axis',(1.,0.,0.));
#8939=CARTESIAN_POINT('',(0.,0.,0.));
#8940=CARTESIAN_POINT('Origin',(0.,0.,-3.69717978381041));
#8941=CARTESIAN_POINT('',(3.0991757505326,6.01559628526639,1.04590194808422));
#8942=CARTESIAN_POINT('',(3.09917575053259,6.01559628526639,0.651392015122069));
#8943=CARTESIAN_POINT('',(3.09917575053259,6.01559628526639,-3.69717978381041));
#8944=CARTESIAN_POINT('',(-3.92961407736517,-5.50997186835842,0.000232560444541066));
#8945=CARTESIAN_POINT('Ctrl Pts',(-3.92889204432313,-5.50963667622961,0.00025114599476872));
#8946=CARTESIAN_POINT('Ctrl Pts',(-3.79038240896438,-5.60840714629906,0.00830193321678136));
#8947=CARTESIAN_POINT('Ctrl Pts',(-3.6479042510226,-5.70212321738183,0.0163527204387951));
#8948=CARTESIAN_POINT('Ctrl Pts',(-3.50187062022184,-5.79043963436517,0.0244035076608076));
#8949=CARTESIAN_POINT('Ctrl Pts',(-3.35600620203666,-5.87865371703119,0.0324449662456032));
#8950=CARTESIAN_POINT('Ctrl Pts',(-3.2065948255179,-5.96148040292313,0.0404864248303983));
#8951=CARTESIAN_POINT('Ctrl Pts',(-3.05408187353037,-6.03861514834098,0.0485278834151939));
#8952=CARTESIAN_POINT('Ctrl Pts',(-2.90171192392777,-6.11567756906503,0.0565618019993478));
#8953=CARTESIAN_POINT('Ctrl Pts',(-2.74624651834304,-6.18705850218575,0.0645957205835019));
#8954=CARTESIAN_POINT('Ctrl Pts',(-2.58815912298106,-6.25249720944599,0.0726296391676557));
#8955=CARTESIAN_POINT('Ctrl Pts',(-2.43018506105976,-6.31788900345404,0.0806577982057483));
#8956=CARTESIAN_POINT('Ctrl Pts',(-2.26959309568702,-6.37734690791538,0.0886859572438399));
#8957=CARTESIAN_POINT('Ctrl Pts',(-2.10688022797297,-6.43065663093409,0.0967141162819325));
#8958=CARTESIAN_POINT('Ctrl Pts',(-1.94010051972161,-6.48529877557163,0.104942930886329));
#8959=CARTESIAN_POINT('Ctrl Pts',(-1.77109285526961,-6.53348118862384,0.113171745490725));
#8960=CARTESIAN_POINT('Ctrl Pts',(-1.6004136702066,-6.57502586186669,0.121400560095122));
#8961=CARTESIAN_POINT('Ctrl Pts',(-1.43400115166054,-6.61553199449185,0.129423669430104));
#8962=CARTESIAN_POINT('Ctrl Pts',(-1.26600007280295,-6.64972821013253,0.137446778765087));
#8963=CARTESIAN_POINT('Ctrl Pts',(-1.09694043186167,-6.67750033238091,0.145469888100069));
#8964=CARTESIAN_POINT('Ctrl Pts',(-0.927881956037865,-6.70527226323065,
0.153492942141754));
#8965=CARTESIAN_POINT('Ctrl Pts',(-0.757765302814855,-6.72662012752097,
0.161515996183439));
#8966=CARTESIAN_POINT('Ctrl Pts',(-0.587129013611443,-6.74148118156356,
0.169539050225124));
#8967=CARTESIAN_POINT('Ctrl Pts',(-0.416459841795382,-6.75634509941833,
0.177563650356328));
#8968=CARTESIAN_POINT('Ctrl Pts',(-0.245271208442629,-6.76471968690886,
0.185588250487533));
#8969=CARTESIAN_POINT('Ctrl Pts',(-0.0741049318708623,-6.76659422893618,
0.193612850618737));
#8970=CARTESIAN_POINT('Ctrl Pts',(0.104700424075701,-6.76855243099061,0.201995585299463));
#8971=CARTESIAN_POINT('Ctrl Pts',(0.283480924655757,-6.76341705142668,0.210378319980189));
#8972=CARTESIAN_POINT('Ctrl Pts',(0.461622104329729,-6.75123648177089,0.218761054660915));
#8973=CARTESIAN_POINT('Ctrl Pts',(0.632409631117175,-6.73955872500415,0.22679775076036));
#8974=CARTESIAN_POINT('Ctrl Pts',(0.80260919751235,-6.72140587627492,0.234834446859806));
#8975=CARTESIAN_POINT('Ctrl Pts',(0.97168796157606,-6.69687326334672,0.242871142959252));
#8976=CARTESIAN_POINT('Ctrl Pts',(1.14087936821317,-6.67232430645796,0.250913193215));
#8977=CARTESIAN_POINT('Ctrl Pts',(1.30894811887766,-6.64138719044629,0.258955243470749));
#8978=CARTESIAN_POINT('Ctrl Pts',(1.47537431408813,-6.60420772184893,0.266997293726497));
#8979=CARTESIAN_POINT('Ctrl Pts',(1.64201671727433,-6.5669799525761,0.275049791588792));
#8980=CARTESIAN_POINT('Ctrl Pts',(1.80701194770951,-6.52349374575839,0.283102289451085));
#8981=CARTESIAN_POINT('Ctrl Pts',(1.96985743028625,-6.47394398372013,0.291154787313379));
#8982=CARTESIAN_POINT('Ctrl Pts',(1.99042338587475,-6.46768628354095,0.292171747138067));
#8983=CARTESIAN_POINT('Ctrl Pts',(2.010955083382,-6.46133193442697,0.293188706962756));
#8984=CARTESIAN_POINT('Ctrl Pts',(2.03145153667316,-6.45488138188056,0.294205666787444));
#8985=CARTESIAN_POINT('Ctrl Pts',(2.19747654241461,-6.40263073108063,0.302443226639107));
#8986=CARTESIAN_POINT('Ctrl Pts',(2.3617135116338,-6.3438984024491,0.31068078649077));
#8987=CARTESIAN_POINT('Ctrl Pts',(2.52362070621982,-6.27882373786194,0.318918346342433));
#8988=CARTESIAN_POINT('Ctrl Pts',(2.68534576630942,-6.21382227781208,0.327146639503884));
#8989=CARTESIAN_POINT('Ctrl Pts',(2.84474594209345,-6.14249282172973,0.335374932665337));
#8990=CARTESIAN_POINT('Ctrl Pts',(3.0012937929869,-6.06502469641949,0.343603225826788));
#8991=CARTESIAN_POINT('Ctrl Pts',(3.15769669554932,-5.98762829918093,0.351823900376077));
#8992=CARTESIAN_POINT('Ctrl Pts',(3.3112522146734,-5.90410471035315,0.360044574925363));
#8993=CARTESIAN_POINT('Ctrl Pts',(3.4614519757946,-5.8146916701806,0.368265249474652));
#8994=CARTESIAN_POINT('Ctrl Pts',(3.6115425504235,-5.72534362808894,0.376479948071571));
#8995=CARTESIAN_POINT('Ctrl Pts',(3.75828192028324,-5.63011484475562,0.38469464666849));
#8996=CARTESIAN_POINT('Ctrl Pts',(3.90118536821696,-5.52928944104122,0.392909345265409));
#8997=CARTESIAN_POINT('Ctrl Pts',(4.04401335933728,-5.42851727581604,0.401119706283438));
#8998=CARTESIAN_POINT('Ctrl Pts',(4.18300917239897,-5.3221545832726,0.409330067301468));
#8999=CARTESIAN_POINT('Ctrl Pts',(4.31771611726011,-5.21052939064278,0.417540428319497));
#9000=CARTESIAN_POINT('Ctrl Pts',(4.45239570423667,-5.09892686818146,0.425749121879999));
#9001=CARTESIAN_POINT('Ctrl Pts',(4.58278787946917,-4.98206419803764,0.433957815440499));
#9002=CARTESIAN_POINT('Ctrl Pts',(4.70846792674628,-4.86031056443944,0.442166509001001));
#9003=CARTESIAN_POINT('Ctrl Pts',(4.83413768807839,-4.73856689543948,0.450374530743085));
#9004=CARTESIAN_POINT('Ctrl Pts',(4.95509583218291,-4.61193330837405,0.45858255248517));
#9005=CARTESIAN_POINT('Ctrl Pts',(5.07095353957911,-4.48081680047624,0.466790574227254));
#9006=CARTESIAN_POINT('Ctrl Pts',(5.18682264631825,-4.34968739190852,0.474999403563902));
#9007=CARTESIAN_POINT('Ctrl Pts',(5.29759007971564,-4.21407445167993,0.483208232900549));
#9008=CARTESIAN_POINT('Ctrl Pts',(5.40290641236495,-4.07441913642003,0.491417062237197));
#9009=CARTESIAN_POINT('Ctrl Pts',(5.50825208868729,-3.93472490981746,0.499628178751893));
#9010=CARTESIAN_POINT('Ctrl Pts',(5.60814342364821,-3.79098635003299,0.507839295266589));
#9011=CARTESIAN_POINT('Ctrl Pts',(5.70227349625691,-3.64367478980851,0.516050411781285));
#9012=CARTESIAN_POINT('Ctrl Pts',(5.7964993705027,-3.49621330206095,0.524269885225734));
#9013=CARTESIAN_POINT('Ctrl Pts',(5.88495207482346,-3.34517185030215,0.532489358670184));
#9014=CARTESIAN_POINT('Ctrl Pts',(5.96736947095795,-3.19104851061201,0.540708832114634));
#9015=CARTESIAN_POINT('Ctrl Pts',(6.04982999095192,-3.0368445278349,0.54893260629454));
#9016=CARTESIAN_POINT('Ctrl Pts',(6.12624875071037,-2.8795557634772,0.557156380474448));
#9017=CARTESIAN_POINT('Ctrl Pts',(6.19641126214192,-2.71970154068435,0.565380154654354));
#9018=CARTESIAN_POINT('Ctrl Pts',(6.26667455633474,-2.55961770025602,0.573615741619366));
#9019=CARTESIAN_POINT('Ctrl Pts',(6.33066351158858,-2.3969613695239,0.581851328584376));
#9020=CARTESIAN_POINT('Ctrl Pts',(6.38821271033491,-2.23226955529915,0.590086915549388));
#9021=CARTESIAN_POINT('Ctrl Pts',(6.44027281862399,-2.08328618333845,0.597536985377683));
#9022=CARTESIAN_POINT('Ctrl Pts',(6.48706363804092,-1.93263748079221,0.604987055205977));
#9023=CARTESIAN_POINT('Ctrl Pts',(6.52849874228747,-1.78072827010495,0.612437125034272));
#9024=CARTESIAN_POINT('Ctrl Pts',(6.57393130962719,-1.6141635764817,0.620605942400958));
#9025=CARTESIAN_POINT('Ctrl Pts',(6.61305351986596,-1.44560879889593,0.628774759767645));
#9026=CARTESIAN_POINT('Ctrl Pts',(6.64568796898957,-1.27558630395096,0.636943577134332));
#9027=CARTESIAN_POINT('Ctrl Pts',(6.67828553118715,-1.10575598651667,0.645103161234637));
#9028=CARTESIAN_POINT('Ctrl Pts',(6.704409862946,-0.934461608373648,0.653262745334943));
#9029=CARTESIAN_POINT('Ctrl Pts',(6.72393320152799,-0.762240973308022,0.661422329435248));
#9030=CARTESIAN_POINT('Ctrl Pts',(6.74343853720231,-0.590179146746397,0.669574389400343));
#9031=CARTESIAN_POINT('Ctrl Pts',(6.75635495829404,-0.417193123190283,0.677726449365437));
#9032=CARTESIAN_POINT('Ctrl Pts',(6.76260566212413,-0.24383120925473,0.685878509330532));
#9033=CARTESIAN_POINT('Ctrl Pts',(6.76885190277121,-0.0705930807313588,
0.69402474848943));
#9034=CARTESIAN_POINT('Ctrl Pts',(6.76844189092621,0.103020041389537,0.70217098764833));
#9035=CARTESIAN_POINT('Ctrl Pts',(6.76135060250933,0.276454390355338,0.710317226807228));
#9036=CARTESIAN_POINT('Ctrl Pts',(6.75426290225783,0.449800982190343,0.718459343999632));
#9037=CARTESIAN_POINT('Ctrl Pts',(6.74050067365104,0.622968618117431,0.726601461192037));
#9038=CARTESIAN_POINT('Ctrl Pts',(6.72009098117132,0.795403171215613,0.734743578384441));
#9039=CARTESIAN_POINT('Ctrl Pts',(6.69962758385231,0.968291458243047,0.742907120255134));
#9040=CARTESIAN_POINT('Ctrl Pts',(6.67248169599599,1.14044243079594,0.751070662125828));
#9041=CARTESIAN_POINT('Ctrl Pts',(6.63873304122902,1.3113018749678,0.759234203996522));
#9042=CARTESIAN_POINT('Ctrl Pts',(6.60507898639243,1.48168238770861,0.767374862866457));
#9043=CARTESIAN_POINT('Ctrl Pts',(6.56485921978189,1.65077824737774,0.775515521736392));
#9044=CARTESIAN_POINT('Ctrl Pts',(6.51820410356284,1.81804957696335,0.783656180606327));
#9045=CARTESIAN_POINT('Ctrl Pts',(6.47154210487086,1.98534558209348,0.791798040370587));
#9046=CARTESIAN_POINT('Ctrl Pts',(6.41844296343186,2.15081617013514,0.799939900134848));
#9047=CARTESIAN_POINT('Ctrl Pts',(6.35908705673205,2.31393621452774,0.808081759899108));
#9048=CARTESIAN_POINT('Ctrl Pts',(6.29971120841759,2.47711106184132,0.816226355058021));
#9049=CARTESIAN_POINT('Ctrl Pts',(6.23407453305535,2.6379334507201,0.824370950216934));
#9050=CARTESIAN_POINT('Ctrl Pts',(6.16240571227708,2.79589785888091,0.832515545375847));
#9051=CARTESIAN_POINT('Ctrl Pts',(6.09043044989734,2.95453769138503,0.840694965201285));
#9052=CARTESIAN_POINT('Ctrl Pts',(6.01237149959967,3.11029471312419,0.848874385026722));
#9053=CARTESIAN_POINT('Ctrl Pts',(5.92850683918757,3.26268227961385,0.857053804852159));
#9054=CARTESIAN_POINT('Ctrl Pts',(5.84485364385698,3.41468560023628,0.865212600237317));
#9055=CARTESIAN_POINT('Ctrl Pts',(5.75542421689786,3.5633361542509,0.873371395622476));
#9056=CARTESIAN_POINT('Ctrl Pts',(5.66053745414438,3.70818078445868,0.881530191007635));
#9057=CARTESIAN_POINT('Ctrl Pts',(5.56529089813482,3.85357463902209,0.889719923053211));
#9058=CARTESIAN_POINT('Ctrl Pts',(5.46454576871104,3.99513336137898,0.897909655098788));
#9059=CARTESIAN_POINT('Ctrl Pts',(5.35866457522277,4.13243305695962,0.906099387144364));
#9060=CARTESIAN_POINT('Ctrl Pts',(5.25278338173449,4.26973275254026,0.91428911918994));
#9061=CARTESIAN_POINT('Ctrl Pts',(5.14176640573001,4.40277318243318,0.922478851235517));
#9062=CARTESIAN_POINT('Ctrl Pts',(5.02601218914608,4.53116877577464,0.930668583281093));
#9063=CARTESIAN_POINT('Ctrl Pts',(4.90985584864106,4.66001040849997,0.938886766015206));
#9064=CARTESIAN_POINT('Ctrl Pts',(4.78856616752597,4.78457774688426,0.947104948749321));
#9065=CARTESIAN_POINT('Ctrl Pts',(4.66248925298099,4.90443503023914,0.955323131483434));
#9066=CARTESIAN_POINT('Ctrl Pts',(4.53660699102111,5.02410726361772,0.963528626006388));
#9067=CARTESIAN_POINT('Ctrl Pts',(4.40595248216271,5.13908368708086,0.971734120529341));
#9068=CARTESIAN_POINT('Ctrl Pts',(4.27091134853337,5.24896230249074,0.979939615052295));
#9069=CARTESIAN_POINT('Ctrl Pts',(4.13599006363772,5.35874340085109,0.988137827215413));
#9070=CARTESIAN_POINT('Ctrl Pts',(3.99669017928062,5.46343547027293,0.99633603937853));
#9071=CARTESIAN_POINT('Ctrl Pts',(3.8534339375994,5.56267344795263,1.00453425154165));
#9072=CARTESIAN_POINT('Ctrl Pts',(3.71030282712495,5.66182474342038,1.01272530274501));
#9073=CARTESIAN_POINT('Ctrl Pts',(3.5632225385651,5.75553123438426,1.02091635394837));
#9074=CARTESIAN_POINT('Ctrl Pts',(3.41264795723443,5.8434683981334,1.02910740515173));
#9075=CARTESIAN_POINT('Ctrl Pts',(3.30973763034577,5.9035691281976,1.03470558612923));
#9076=CARTESIAN_POINT('Ctrl Pts',(3.20519580383802,5.96097580166128,1.04030376710673));
#9077=CARTESIAN_POINT('Ctrl Pts',(3.0991757505326,6.01559628526639,1.04590194808422));
#9078=CARTESIAN_POINT('',(3.92888236737287,-5.50964357679755,0.));
#9079=CARTESIAN_POINT('Origin',(0.,0.,0.));
#9080=CARTESIAN_POINT('Ctrl Pts',(3.92888236737286,-5.50964357679756,-4.44089209850063E-16));
#9081=CARTESIAN_POINT('Ctrl Pts',(4.08032704765413,-5.40164959756899,0.00874944781300858));
#9082=CARTESIAN_POINT('Ctrl Pts',(4.2273164115086,-5.28740798007164,0.0174988956260169));
#9083=CARTESIAN_POINT('Ctrl Pts',(4.36935121050034,-5.16730674522998,0.0262483434390259));
#9084=CARTESIAN_POINT('Ctrl Pts',(4.51138486261615,-5.04720648015923,0.0349977206036361));
#9085=CARTESIAN_POINT('Ctrl Pts',(4.64846381108604,-4.9212468774719,0.0437470977682466));
#9086=CARTESIAN_POINT('Ctrl Pts',(4.78012247564787,-4.78985575125245,0.0524964749328567));
#9087=CARTESIAN_POINT('Ctrl Pts',(4.91178012085318,-4.65846564231811,0.0612457843561254));
#9088=CARTESIAN_POINT('Ctrl Pts',(5.03801736328267,-4.52164429644009,0.0699950937793945));
#9089=CARTESIAN_POINT('Ctrl Pts',(5.15840545249789,-4.37985641176056,0.0787444032026632));
#9090=CARTESIAN_POINT('Ctrl Pts',(5.27879264960788,-4.23806957776398,0.0874936477914066));
#9091=CARTESIAN_POINT('Ctrl Pts',(5.39333059476267,-4.09131649706054,0.0962428923801495));
#9092=CARTESIAN_POINT('Ctrl Pts',(5.50163027861608,-3.94009559242092,0.104992136968893));
#9093=CARTESIAN_POINT('Ctrl Pts',(5.60992919591457,-3.78887575813648,0.113741319629695));
#9094=CARTESIAN_POINT('Ctrl Pts',(5.71198977342317,-3.63318839617191,0.122490502290497));
#9095=CARTESIAN_POINT('Ctrl Pts',(5.80746538403055,-3.47356226564127,0.131239684951299));
#9096=CARTESIAN_POINT('Ctrl Pts',(5.90294035056408,-3.3139372119408,0.139988808590537));
#9097=CARTESIAN_POINT('Ctrl Pts',(5.99183029200292,-3.15037368876134,0.148737932229775));
#9098=CARTESIAN_POINT('Ctrl Pts',(6.07383331657755,-2.98342719744131,0.157487055869014));
#9099=CARTESIAN_POINT('Ctrl Pts',(6.15583581519874,-2.81648177688769,0.166236123392861));
#9100=CARTESIAN_POINT('Ctrl Pts',(6.23095135902003,-2.64615368880009,0.174985190916708));
#9101=CARTESIAN_POINT('Ctrl Pts',(6.2989248407314,-2.4730214012048,0.183734258440555));
#9102=CARTESIAN_POINT('Ctrl Pts',(6.36689790904675,-2.29989016655244,0.192483272754981));
#9103=CARTESIAN_POINT('Ctrl Pts',(6.4277288974603,-2.12395503322982,0.201232287069408));
#9104=CARTESIAN_POINT('Ctrl Pts',(6.48121121436041,-1.94581350464243,0.209981301383834));
#9105=CARTESIAN_POINT('Ctrl Pts',(6.53742627953525,-1.75856960384828,0.219177357920047));
#9106=CARTESIAN_POINT('Ctrl Pts',(6.5855219277559,-1.56888825318548,0.22837341445626));
#9107=CARTESIAN_POINT('Ctrl Pts',(6.62531771926539,-1.37748107747006,0.237569470992473));
#9108=CARTESIAN_POINT('Ctrl Pts',(6.6631831972433,-1.19535819658355,0.246319468493404));
#9109=CARTESIAN_POINT('Ctrl Pts',(6.69353484894203,-1.01167324970243,0.255069465994336));
#9110=CARTESIAN_POINT('Ctrl Pts',(6.71626957222991,-0.827050199890335,0.263819463495267));
#9111=CARTESIAN_POINT('Ctrl Pts',(6.73900383447862,-0.642430894063015,0.272569283554338));
#9112=CARTESIAN_POINT('Ctrl Pts',(6.75412144238072,-0.456873807891365,0.281319103613409));
#9113=CARTESIAN_POINT('Ctrl Pts',(6.76157104471273,-0.271009238407965,0.29006892367248));
#9114=CARTESIAN_POINT('Ctrl Pts',(6.76902050587629,-0.085148191020104,0.298818577924252));
#9115=CARTESIAN_POINT('Ctrl Pts',(6.76880224076615,0.101020041610374,0.307568232176024));
#9116=CARTESIAN_POINT('Ctrl Pts',(6.76091699075328,0.286863110461421,0.316317886427796));
#9117=CARTESIAN_POINT('Ctrl Pts',(6.75303187968407,0.472702904626974,0.32506738650451));
#9118=CARTESIAN_POINT('Ctrl Pts',(6.73748006620785,0.658217260123046,0.333816886581225));
#9119=CARTESIAN_POINT('Ctrl Pts',(6.71431437259024,0.842776071105572,0.342566386657939));
#9120=CARTESIAN_POINT('Ctrl Pts',(6.69114905638314,1.02733187529549,0.351315744189673));
#9121=CARTESIAN_POINT('Ctrl Pts',(6.66037014395277,1.21093188176617,0.360065101721407));
#9122=CARTESIAN_POINT('Ctrl Pts',(6.62208217352349,1.39295250712377,0.368814459253141));
#9123=CARTESIAN_POINT('Ctrl Pts',(6.58379477599824,1.57497040890141,0.377563685867982));
#9124=CARTESIAN_POINT('Ctrl Pts',(6.53799860430444,1.75540869642656,0.386312912482823));
#9125=CARTESIAN_POINT('Ctrl Pts',(6.48484919699013,1.9336545431634,0.395062139097663));
#9126=CARTESIAN_POINT('Ctrl Pts',(6.43170051433729,2.11189795962108,0.403811246421853));
#9127=CARTESIAN_POINT('Ctrl Pts',(6.37119887857043,2.28794872050952,0.412560353746043));
#9128=CARTESIAN_POINT('Ctrl Pts',(6.30354976713205,2.46120891703438,0.421309461070233));
#9129=CARTESIAN_POINT('Ctrl Pts',(6.23590148818025,2.63446698142792,0.430058460728346));
#9130=CARTESIAN_POINT('Ctrl Pts',(6.16110601378106,2.80493428327179,0.438807460386459));
#9131=CARTESIAN_POINT('Ctrl Pts',(6.07941736028839,2.97203189071453,0.447556460044571));
#9132=CARTESIAN_POINT('Ctrl Pts',(5.99771978801279,3.13914774190625,0.456306414920151));
#9133=CARTESIAN_POINT('Ctrl Pts',(5.90912765640074,3.30289290492367,0.465056369795731));
#9134=CARTESIAN_POINT('Ctrl Pts',(5.81394190290397,3.46271115596687,0.473806324671311));
#9135=CARTESIAN_POINT('Ctrl Pts',(5.71875982413551,3.6225232370883,0.482555941747317));
#9136=CARTESIAN_POINT('Ctrl Pts',(5.6169847795414,3.77840846333365,0.491305558823323));
#9137=CARTESIAN_POINT('Ctrl Pts',(5.50896246077205,3.92983735106231,0.500055175899329));
#9138=CARTESIAN_POINT('Ctrl Pts',(5.40094373802236,4.08126119778403,0.508804501704092));
#9139=CARTESIAN_POINT('Ctrl Pts',(5.28667832369811,4.22822876953944,0.517553827508855));
#9140=CARTESIAN_POINT('Ctrl Pts',(5.16655430873675,4.37024090581672,0.526303153313617));
#9141=CARTESIAN_POINT('Ctrl Pts',(5.04643365420422,4.51224906935235,0.535052234358939));
#9142=CARTESIAN_POINT('Ctrl Pts',(4.9204549120583,4.64930185603789,0.543801315404261));
#9143=CARTESIAN_POINT('Ctrl Pts',(4.78904593245666,4.78093380594422,0.552550396449583));
#9144=CARTESIAN_POINT('Ctrl Pts',(4.65762507998344,4.91257764886762,0.561300267979057));
#9145=CARTESIAN_POINT('Ctrl Pts',(4.52077321070996,5.0387994720143,0.57005013950853));
#9146=CARTESIAN_POINT('Ctrl Pts',(4.37895518611181,5.15917052228597,0.578800011038004));
#9147=CARTESIAN_POINT('Ctrl Pts',(4.23714700417698,5.27953321838881,0.587549275296012));
#9148=CARTESIAN_POINT('Ctrl Pts',(4.09037357512216,5.3940457687175,0.59629853955402));
#9149=CARTESIAN_POINT('Ctrl Pts',(3.9391333930669,5.50231924842836,0.605047803812028));
#9150=CARTESIAN_POINT('Ctrl Pts',(3.78788546298275,5.61059827498556,0.613797516294519));
#9151=CARTESIAN_POINT('Ctrl Pts',(3.63217055501693,5.71263742444897,0.62254722877701));
#9152=CARTESIAN_POINT('Ctrl Pts',(3.47251758582549,5.80809010055222,0.6312969412595));
#9153=CARTESIAN_POINT('Ctrl Pts',(3.35029497128432,5.8811640665259,0.63799529921369));
#9154=CARTESIAN_POINT('Ctrl Pts',(3.22576502399092,5.95037874273607,0.64469365716788));
#9155=CARTESIAN_POINT('Ctrl Pts',(3.09917575053259,6.01559628526639,0.651392015122069));
#9156=CARTESIAN_POINT('Origin',(0.,0.,-3.69717978381041));
#9157=CARTESIAN_POINT('',(3.09917575053259,6.01559628526639,3.04575158274221));
#9158=CARTESIAN_POINT('',(3.09917575053259,6.01559628526639,2.65160425626863));
#9159=CARTESIAN_POINT('',(3.09917575053259,6.01559628526639,-3.69717978381041));
#9160=CARTESIAN_POINT('',(-6.767,1.71693117622523E-12,1.69717978381002));
#9161=CARTESIAN_POINT('Ctrl Pts',(-6.767,1.71693091881772E-12,1.69717978381002));
#9162=CARTESIAN_POINT('Ctrl Pts',(-6.76700000000005,-0.186007249414028,
1.70592929561597));
#9163=CARTESIAN_POINT('Ctrl Pts',(-6.75932637295447,-0.372014355525948,
1.71467880742193));
#9164=CARTESIAN_POINT('Ctrl Pts',(-6.7440051826694,-0.557389537153533,1.72342831922788));
#9165=CARTESIAN_POINT('Ctrl Pts',(-6.72868405709661,-0.742763935809962,
1.73217779407843));
#9166=CARTESIAN_POINT('Ctrl Pts',(-6.7057154565301,-0.927506129693684,1.74092726892897));
#9167=CARTESIAN_POINT('Ctrl Pts',(-6.67517739415671,-1.11098863924849,1.74967674377952));
#9168=CARTESIAN_POINT('Ctrl Pts',(-6.64463945823092,-1.29447038906543,1.7584261824015));
#9169=CARTESIAN_POINT('Ctrl Pts',(-6.60653217027148,-1.47669218228261,1.76717562102349));
#9170=CARTESIAN_POINT('Ctrl Pts',(-6.560984961167,-1.65703510504169,1.77592505964547));
#9171=CARTESIAN_POINT('Ctrl Pts',(-6.51543793687501,-1.83737729604078,1.78467446276571));
#9172=CARTESIAN_POINT('Ctrl Pts',(-6.46245112202619,-2.0158403539712,1.79342386588594));
#9173=CARTESIAN_POINT('Ctrl Pts',(-6.40220448416217,-2.19181813638219,1.80217326900618));
#9174=CARTESIAN_POINT('Ctrl Pts',(-6.34195808575155,-2.36779521936031,1.81092263735146));
#9175=CARTESIAN_POINT('Ctrl Pts',(-6.27445201489195,-2.54128677544927,1.81967200569673));
#9176=CARTESIAN_POINT('Ctrl Pts',(-6.19991555136135,-2.71170355237951,1.82842137404201));
#9177=CARTESIAN_POINT('Ctrl Pts',(-6.12537937788984,-2.88211966613188,1.83717070833907));
#9178=CARTESIAN_POINT('Ctrl Pts',(-6.04381298133556,-3.04946076210566,1.84592004263613));
#9179=CARTESIAN_POINT('Ctrl Pts',(-5.95549339426238,-3.21315848206981,1.85466937693319));
#9180=CARTESIAN_POINT('Ctrl Pts',(-5.86717414355079,-3.37685557859778,1.86341867790876));
#9181=CARTESIAN_POINT('Ctrl Pts',(-5.77210188986143,-3.53690907467468,1.87216797888434));
#9182=CARTESIAN_POINT('Ctrl Pts',(-5.67059953466957,-3.69277536785075,1.88091727985991));
#9183=CARTESIAN_POINT('Ctrl Pts',(-5.56909755761648,-3.84864108035964,1.88966654824067));
#9184=CARTESIAN_POINT('Ctrl Pts',(-5.46116568337945,-4.0003193810445,1.89841581662144));
#9185=CARTESIAN_POINT('Ctrl Pts',(-5.34717048685982,-4.14729511663389,1.9071650850022));
#9186=CARTESIAN_POINT('Ctrl Pts',(-5.23317570555385,-4.29427031688201,1.91591432151482));
#9187=CARTESIAN_POINT('Ctrl Pts',(-5.11311782178674,-4.4365427598728,1.92466355802743));
#9188=CARTESIAN_POINT('Ctrl Pts',(-4.98740459171885,-4.57362924147791,1.93341279454005));
#9189=CARTESIAN_POINT('Ctrl Pts',(-4.86169180910691,-4.7107152351458,1.94216199991117));
#9190=CARTESIAN_POINT('Ctrl Pts',(-4.73032391415281,-4.8426150931667,1.95091120528229));
#9191=CARTESIAN_POINT('Ctrl Pts',(-4.59374707237132,-4.96888084331672,1.95966041065341));
#9192=CARTESIAN_POINT('Ctrl Pts',(-4.45717070537233,-5.09514615452872,1.96840958560964));
#9193=CARTESIAN_POINT('Ctrl Pts',(-4.31538563819332,-5.21577720253779,1.97715876056588));
#9194=CARTESIAN_POINT('Ctrl Pts',(-4.16887341290463,-5.33036429028795,1.98590793552211));
#9195=CARTESIAN_POINT('Ctrl Pts',(-4.02236168477139,-5.44495098921324,1.99465708079003));
#9196=CARTESIAN_POINT('Ctrl Pts',(-3.87112305634225,-5.55349359238908,2.00340622605795));
#9197=CARTESIAN_POINT('Ctrl Pts',(-3.71567117316504,-5.65562346102623,2.01215537132588));
#9198=CARTESIAN_POINT('Ctrl Pts',(-3.56021980457083,-5.75775299158903,2.02090448763203));
#9199=CARTESIAN_POINT('Ctrl Pts',(-3.40055544862183,-5.85346967275472,2.02965360393819));
#9200=CARTESIAN_POINT('Ctrl Pts',(-3.23722036323211,-5.94244842803666,2.03840272024434));
#9201=CARTESIAN_POINT('Ctrl Pts',(-3.07388580495863,-6.03142689616568,2.04715180831528));
#9202=CARTESIAN_POINT('Ctrl Pts',(-2.90688079257533,-6.11366734484905,2.05590089638622));
#9203=CARTESIAN_POINT('Ctrl Pts',(-2.73677251094451,-6.18889046787375,2.06464998445716));
#9204=CARTESIAN_POINT('Ctrl Pts',(-2.56666476416466,-6.26411335438344,2.0733990450194));
#9205=CARTESIAN_POINT('Ctrl Pts',(-2.39345402971899,-6.33231884350364,2.08214810558163));
#9206=CARTESIAN_POINT('Ctrl Pts',(-2.21772856473829,-6.39327529621116,2.09089716614387));
#9207=CARTESIAN_POINT('Ctrl Pts',(-2.04200363768054,-6.4542315623215,2.09964619992387));
#9208=CARTESIAN_POINT('Ctrl Pts',(-1.86376426619872,-6.50793874252119,2.10839523370387));
#9209=CARTESIAN_POINT('Ctrl Pts',(-1.6836157819446,-6.55421443796181,2.11714426748388));
#9210=CARTESIAN_POINT('Ctrl Pts',(-1.50346783419614,-6.60048999558738,2.12589327520812));
#9211=CARTESIAN_POINT('Ctrl Pts',(-1.32141106256967,-6.63933404145552,2.13464228293236));
#9212=CARTESIAN_POINT('Ctrl Pts',(-1.13806375958738,-6.67061465527082,2.1433912906566));
#9213=CARTESIAN_POINT('Ctrl Pts',(-0.954716987416449,-6.70189517852518,
2.15214027305146));
#9214=CARTESIAN_POINT('Ctrl Pts',(-0.770079973807536,-6.72561226535854,
2.16088925544633));
#9215=CARTESIAN_POINT('Ctrl Pts',(-0.584779770550486,-6.74168536939799,
2.1696382378412));
#9216=CARTESIAN_POINT('Ctrl Pts',(-0.391490647551969,-6.75845143942405,
2.17876441851725));
#9217=CARTESIAN_POINT('Ctrl Pts',(-0.19748021310242,-6.76689975924032,2.1878905991933));
#9218=CARTESIAN_POINT('Ctrl Pts',(-0.00346532629591402,-6.76699911271708,
2.19701677986935));
#9219=CARTESIAN_POINT('Ctrl Pts',(0.184486595297895,-6.76709536139768,2.20585776739928));
#9220=CARTESIAN_POINT('Ctrl Pts',(0.372442378187021,-6.7593565972676,2.2146987549292));
#9221=CARTESIAN_POINT('Ctrl Pts',(0.559750217723831,-6.74380965729002,2.22353974245913));
#9222=CARTESIAN_POINT('Ctrl Pts',(0.745129914459458,-6.72842275717234,2.23228972105689));
#9223=CARTESIAN_POINT('Ctrl Pts',(0.929874656315847,-6.7053877227345,2.24103969965466));
#9224=CARTESIAN_POINT('Ctrl Pts',(1.11335688289939,-6.67478280180715,2.24978967825243));
#9225=CARTESIAN_POINT('Ctrl Pts',(1.29683723119015,-6.64417819417992,2.25853956727737));
#9226=CARTESIAN_POINT('Ctrl Pts',(1.4790548073039,-6.6060039023004,2.26728945630231));
#9227=CARTESIAN_POINT('Ctrl Pts',(1.65939064804959,-6.56038959797096,2.27603934532725));
#9228=CARTESIAN_POINT('Ctrl Pts',(1.83972470264408,-6.51477574543215,2.28478914768819));
#9229=CARTESIAN_POINT('Ctrl Pts',(2.01817678125982,-6.46172209820058,2.29353895004914));
#9230=CARTESIAN_POINT('Ctrl Pts',(2.19414072347805,-6.40140886723971,2.30228875241008));
#9231=CARTESIAN_POINT('Ctrl Pts',(2.37010298132218,-6.34109621361329,2.31103847101557));
#9232=CARTESIAN_POINT('Ctrl Pts',(2.5435768792703,-6.27352420825923,2.31978818962105));
#9233=CARTESIAN_POINT('Ctrl Pts',(2.71397317790084,-6.19892237325447,2.32853790822654));
#9234=CARTESIAN_POINT('Ctrl Pts',(2.88436790207312,-6.12432122756911,2.33728754598481));
#9235=CARTESIAN_POINT('Ctrl Pts',(3.05168482126366,-6.04269049717362,2.34603718374307));
#9236=CARTESIAN_POINT('Ctrl Pts',(3.21535561997496,-5.95430745234871,2.35478682150134));
#9237=CARTESIAN_POINT('Ctrl Pts',(3.3790249607538,-5.86592519481459,2.36353638132035));
#9238=CARTESIAN_POINT('Ctrl Pts',(3.53904799384966,-5.77079087940176,2.37228594113936));
#9239=CARTESIAN_POINT('Ctrl Pts',(3.69488118815067,-5.66922763746971,2.38103550095836));
#9240=CARTESIAN_POINT('Ctrl Pts',(3.85071304610917,-5.56766526648994,2.3897849857458));
#9241=CARTESIAN_POINT('Ctrl Pts',(4.00235489706053,-5.45967423580651,2.39853447053324));
#9242=CARTESIAN_POINT('Ctrl Pts',(4.1492916860774,-5.34562133936262,2.40728395532068));
#9243=CARTESIAN_POINT('Ctrl Pts',(4.29622726385845,-5.23156938308459,2.41603336798399));
#9244=CARTESIAN_POINT('Ctrl Pts',(4.43845763092155,-5.11145583677126,2.42478278064729));
#9245=CARTESIAN_POINT('Ctrl Pts',(4.57549970661051,-4.9856886620413,2.43353219331059));
#9246=CARTESIAN_POINT('Ctrl Pts',(4.71254069815378,-4.85992248226081,2.44228153675691));
#9247=CARTESIAN_POINT('Ctrl Pts',(4.8443932693139,-4.72850295733924,2.45103088020324));
#9248=CARTESIAN_POINT('Ctrl Pts',(4.97060959434769,-4.59187644221605,2.45978022364957));
#9249=CARTESIAN_POINT('Ctrl Pts',(5.09682496280587,-4.45525096256581,2.46852950078586));
#9250=CARTESIAN_POINT('Ctrl Pts',(5.21740397615913,-4.31341878218237,2.47727877792216));
#9251=CARTESIAN_POINT('Ctrl Pts',(5.33193710452009,-4.16686161438582,2.48602805505845));
#9252=CARTESIAN_POINT('Ctrl Pts',(5.44646940289459,-4.02030550864411,2.49477726879142));
#9253=CARTESIAN_POINT('Ctrl Pts',(5.55495572749741,-3.86902470980024,2.50352648252438));
#9254=CARTESIAN_POINT('Ctrl Pts',(5.65702762491532,-3.71353301465665,2.51227569625735));
#9255=CARTESIAN_POINT('Ctrl Pts',(5.75909881655227,-3.55804239466774,2.52102484949346));
#9256=CARTESIAN_POINT('Ctrl Pts',(5.85475551250852,-3.39834117619432,2.52977400272958));
#9257=CARTESIAN_POINT('Ctrl Pts',(5.94367283728161,-3.23497174691847,2.53852315596569));
#9258=CARTESIAN_POINT('Ctrl Pts',(6.03258957676374,-3.07160339300843,2.54727225161123));
#9259=CARTESIAN_POINT('Ctrl Pts',(6.11476689685343,-2.9045671282938,2.55602134725676));
#9260=CARTESIAN_POINT('Ctrl Pts',(6.18992570525316,-2.7344302447578,2.56477044290229));
#9261=CARTESIAN_POINT('Ctrl Pts',(6.2650840438876,-2.56429442462879,2.57351948386333));
#9262=CARTESIAN_POINT('Ctrl Pts',(6.33322384283383,-2.39105828655815,2.58226852482437));
#9263=CARTESIAN_POINT('Ctrl Pts',(6.39411368720104,-2.21531017131876,2.59101756578541));
#9264=CARTESIAN_POINT('Ctrl Pts',(6.45500317120952,-2.03956309619317,2.59976655496781));
#9265=CARTESIAN_POINT('Ctrl Pts',(6.50864269270127,-1.86130434438443,2.60851554415021));
#9266=CARTESIAN_POINT('Ctrl Pts',(6.5548500844638,-1.68113930719762,2.61726453333261));
#9267=CARTESIAN_POINT('Ctrl Pts',(6.60199664749445,-1.49731239211659,2.62619134686198));
#9268=CARTESIAN_POINT('Ctrl Pts',(6.64140563640942,-1.31150116499492,2.63511816039135));
#9269=CARTESIAN_POINT('Ctrl Pts',(6.67293772282202,-1.12436255155483,2.64404497392071));
#9270=CARTESIAN_POINT('Ctrl Pts',(6.70384494949896,-0.940932395049558,2.65279488807624));
#9271=CARTESIAN_POINT('Ctrl Pts',(6.72718449348951,-0.756227260504914,2.66154480223177));
#9272=CARTESIAN_POINT('Ctrl Pts',(6.74287707373947,-0.57087456453988,2.67029471638729));
#9273=CARTESIAN_POINT('Ctrl Pts',(6.7585693453868,-0.385525513630672,2.67904445847127));
#9274=CARTESIAN_POINT('Ctrl Pts',(6.76661493004108,-0.199529212416435,2.68779420055525));
#9275=CARTESIAN_POINT('Ctrl Pts',(6.76698649908907,-0.0135174385986461,
2.69654394263923));
#9276=CARTESIAN_POINT('Ctrl Pts',(6.76735806132385,0.172490924447578,2.70529352428513));
#9277=CARTESIAN_POINT('Ctrl Pts',(6.7600558889628,0.358514472903222,2.71404310593102));
#9278=CARTESIAN_POINT('Ctrl Pts',(6.7451047845457,0.543921359664041,2.72279268757692));
#9279=CARTESIAN_POINT('Ctrl Pts',(6.73015393440668,0.729325093152314,2.73154212041597));
#9280=CARTESIAN_POINT('Ctrl Pts',(6.70755443556871,0.914111900258259,2.74029155325501));
#9281=CARTESIAN_POINT('Ctrl Pts',(6.67738304682287,1.09765415591732,2.74904098609406));
#9282=CARTESIAN_POINT('Ctrl Pts',(6.64721213111822,1.2811935339147,2.75779028175539));
#9283=CARTESIAN_POINT('Ctrl Pts',(6.6094696095545,1.46348811672852,2.76653957741671));
#9284=CARTESIAN_POINT('Ctrl Pts',(6.56428366991132,1.64391876348423,2.77528887307804));
#9285=CARTESIAN_POINT('Ctrl Pts',(6.51909837867661,1.82434682109917,2.78403804318887));
#9286=CARTESIAN_POINT('Ctrl Pts',(6.46646995271859,2.00291071820645,2.79278721329969));
#9287=CARTESIAN_POINT('Ctrl Pts',(6.40657713281481,2.17900400212903,2.80153638341052));
#9288=CARTESIAN_POINT('Ctrl Pts',(6.34668509278988,2.3550949930985,2.81028543959629));
#9289=CARTESIAN_POINT('Ctrl Pts',(6.27952894037451,2.52871516398307,2.81903449578206));
#9290=CARTESIAN_POINT('Ctrl Pts',(6.2053367506137,2.69927486771596,2.82778355196784));
#9291=CARTESIAN_POINT('Ctrl Pts',(6.12832117907839,2.87632521636088,2.8368655532501));
#9292=CARTESIAN_POINT('Ctrl Pts',(6.04372366626002,3.05007728920149,2.84594755453237));
#9293=CARTESIAN_POINT('Ctrl Pts',(5.95185378007792,3.21989527478336,2.85502955581463));
#9294=CARTESIAN_POINT('Ctrl Pts',(5.8633445081729,3.38350129286893,2.86377933612176));
#9295=CARTESIAN_POINT('Ctrl Pts',(5.76808562057168,3.54345567125104,2.87252911642888));
#9296=CARTESIAN_POINT('Ctrl Pts',(5.66640068804391,3.69921508465452,2.881278896736));
#9297=CARTESIAN_POINT('Ctrl Pts',(5.56471941107827,3.85496889852422,2.89002836248949));
#9298=CARTESIAN_POINT('Ctrl Pts',(5.45661270815014,4.00652780919772,2.89877782824297));
#9299=CARTESIAN_POINT('Ctrl Pts',(5.34244776449012,4.1533770456936,2.90752729399645));
#9300=CARTESIAN_POINT('Ctrl Pts',(5.22828631819485,4.30022178356384,2.91627649171605));
#9301=CARTESIAN_POINT('Ctrl Pts',(5.1080671784395,4.44235690972816,2.92502568943565));
#9302=CARTESIAN_POINT('Ctrl Pts',(4.98219864544591,4.57929969070785,2.93377488715526));
#9303=CARTESIAN_POINT('Ctrl Pts',(4.85633329943897,4.71623900430132,2.94252386334549));
#9304=CARTESIAN_POINT('Ctrl Pts',(4.72481904033522,4.84798602483739,2.95127283953573));
#9305=CARTESIAN_POINT('Ctrl Pts',(4.58810250737074,4.9740933225924,2.96002181572596));
#9306=CARTESIAN_POINT('Ctrl Pts',(4.45137708685513,5.10020881822248,2.96877136066214));
#9307=CARTESIAN_POINT('Ctrl Pts',(4.30944892635918,5.22068366308043,2.97752090559831));
#9308=CARTESIAN_POINT('Ctrl Pts',(4.16280009466523,5.33510865604958,2.98627045053449));
#9309=CARTESIAN_POINT('Ctrl Pts',(4.01615988348655,5.4495269227299,2.99501948114276));
#9310=CARTESIAN_POINT('Ctrl Pts',(3.86479978232101,5.55789587288716,3.00376851175104));
#9311=CARTESIAN_POINT('Ctrl Pts',(3.70923383580943,5.65984746713959,3.01251754235931));
#9312=CARTESIAN_POINT('Ctrl Pts',(3.5536657779941,5.76180044505463,3.02126669170734));
#9313=CARTESIAN_POINT('Ctrl Pts',(3.39389200026703,5.85733573571139,3.03001584105536));
#9314=CARTESIAN_POINT('Ctrl Pts',(3.23045513625898,5.94612887622006,3.03876499040338));
#9315=CARTESIAN_POINT('Ctrl Pts',(3.18695122151483,5.96976399206739,3.04109385451632));
#9316=CARTESIAN_POINT('Ctrl Pts',(3.14318791262616,5.99292165435357,3.04342271862927));
#9317=CARTESIAN_POINT('Ctrl Pts',(3.09917575053259,6.01559628526639,3.04575158274221));
#9318=CARTESIAN_POINT('Ctrl Pts',(3.0991757505326,6.01559628526639,1.04590194808422));
#9319=CARTESIAN_POINT('Ctrl Pts',(2.93899076682749,6.0981220056699,1.05436020197771));
#9320=CARTESIAN_POINT('Ctrl Pts',(2.77543011409295,6.17428487827924,1.0628184558712));
#9321=CARTESIAN_POINT('Ctrl Pts',(2.60904700143327,6.24380995421162,1.07127670976468));
#9322=CARTESIAN_POINT('Ctrl Pts',(2.44807637543265,6.31107336103624,1.07945981442202));
#9323=CARTESIAN_POINT('Ctrl Pts',(2.28446439899782,6.37212391638201,1.08764291907935));
#9324=CARTESIAN_POINT('Ctrl Pts',(2.11873390604186,6.42676089763643,1.09582602373668));
#9325=CARTESIAN_POINT('Ctrl Pts',(1.95300550772517,6.48139718834342,1.10400902496916));
#9326=CARTESIAN_POINT('Ctrl Pts',(1.7851589879776,6.52961995329728,1.11219202620163));
#9327=CARTESIAN_POINT('Ctrl Pts',(1.61573361158904,6.57127795001714,1.12037502743411));
#9328=CARTESIAN_POINT('Ctrl Pts',(1.44627930262977,6.61294306062373,1.12855942606801));
#9329=CARTESIAN_POINT('Ctrl Pts',(1.27524594961246,6.64804108434614,1.13674382470191));
#9330=CARTESIAN_POINT('Ctrl Pts',(1.10318434504944,6.67647162061203,1.1449282233358));
#9331=CARTESIAN_POINT('Ctrl Pts',(0.931061800160809,6.70491222633033,1.15311552069844));
#9332=CARTESIAN_POINT('Ctrl Pts',(0.757910633300328,6.72668058281044,1.16130281806107));
#9333=CARTESIAN_POINT('Ctrl Pts',(0.584288150258786,6.74172799491845,1.16949011542371));
#9334=CARTESIAN_POINT('Ctrl Pts',(0.410491565226955,6.75679049599623,1.17768562269523));
#9335=CARTESIAN_POINT('Ctrl Pts',(0.23622307891755,6.76511856369256,1.18588112996675));
#9336=CARTESIAN_POINT('Ctrl Pts',(0.0620422149731795,6.76671558169554,1.19407663723826));
#9337=CARTESIAN_POINT('Ctrl Pts',(-0.112242861460377,6.76831355519512,1.20227704788547));
#9338=CARTESIAN_POINT('Ctrl Pts',(-0.286439852232708,6.76317246294877,1.21047745853267));
#9339=CARTESIAN_POINT('Ctrl Pts',(-0.459993091321101,6.75134766960915,1.21867786917987));
#9340=CARTESIAN_POINT('Ctrl Pts',(-0.633758091792142,6.73950844822082,1.22688828557693));
#9341=CARTESIAN_POINT('Ctrl Pts',(-0.806877415747976,6.72096928098195,1.23509870197399));
#9342=CARTESIAN_POINT('Ctrl Pts',(-0.978803580777068,6.69583695666628,1.24330911837105));
#9343=CARTESIAN_POINT('Ctrl Pts',(-1.01782823477954,6.69013229699141,1.24517275942334));
#9344=CARTESIAN_POINT('Ctrl Pts',(-1.05679146850773,6.68408814897662,1.24703640047563));
#9345=CARTESIAN_POINT('Ctrl Pts',(-1.09568698135607,6.67770612103339,1.24890004152792));
#9346=CARTESIAN_POINT('Ctrl Pts',(-1.27638429160621,6.64805706388433,1.25755797918603));
#9347=CARTESIAN_POINT('Ctrl Pts',(-1.4560377233974,6.61104300179464,1.26621591684414));
#9348=CARTESIAN_POINT('Ctrl Pts',(-1.63403926172985,6.56674993365252,1.27487385450225));
#9349=CARTESIAN_POINT('Ctrl Pts',(-1.8118097449023,6.52251436019299,1.28352055371158));
#9350=CARTESIAN_POINT('Ctrl Pts',(-1.98793231762334,6.4710186949504,1.29216725292091));
#9351=CARTESIAN_POINT('Ctrl Pts',(-2.16180789265776,6.41240014622003,1.30081395213024));
#9352=CARTESIAN_POINT('Ctrl Pts',(-2.34145041084909,6.35183739205194,1.309747437007));
#9353=CARTESIAN_POINT('Ctrl Pts',(-2.51869400074864,6.2836711745779,1.31868092188375));
#9354=CARTESIAN_POINT('Ctrl Pts',(-2.69289047092689,6.20811001123459,1.32761440676051));
#9355=CARTESIAN_POINT('Ctrl Pts',(-2.86101743343772,6.13518161685499,1.33623662324646));
#9356=CARTESIAN_POINT('Ctrl Pts',(-3.0263057022571,6.05536500245165,1.34485883973241));
#9357=CARTESIAN_POINT('Ctrl Pts',(-3.18818833214442,5.96889806905581,1.35348105621836));
#9358=CARTESIAN_POINT('Ctrl Pts',(-3.34991343823498,5.88251527439463,1.36209488264864));
#9359=CARTESIAN_POINT('Ctrl Pts',(-3.50823924606549,5.78949520530867,1.37070870907892));
#9360=CARTESIAN_POINT('Ctrl Pts',(-3.66262035967817,5.69012311825245,1.37932253550919));
#9361=CARTESIAN_POINT('Ctrl Pts',(-3.81682114161615,5.59086710714916,1.38792630017926));
#9362=CARTESIAN_POINT('Ctrl Pts',(-3.96708616736431,5.4852740441412,1.39653006484934));
#9363=CARTESIAN_POINT('Ctrl Pts',(-4.11289597547628,5.37367431976585,1.40513382951941));
#9364=CARTESIAN_POINT('Ctrl Pts',(-4.12917626282904,5.36121373426173,1.40609447656337));
#9365=CARTESIAN_POINT('Ctrl Pts',(-4.14540103557206,5.34867831175663,1.40705512360734));
#9366=CARTESIAN_POINT('Ctrl Pts',(-4.16156959154005,5.33606854667078,1.40801577065131));
#9367=CARTESIAN_POINT('Ctrl Pts',(-4.30619743622049,5.22327411098318,1.41660876508709));
#9368=CARTESIAN_POINT('Ctrl Pts',(-4.44615136592851,5.10466300999673,1.42520175952288));
#9369=CARTESIAN_POINT('Ctrl Pts',(-4.58098069078672,4.98065306065773,1.43379475395866));
#9370=CARTESIAN_POINT('Ctrl Pts',(-4.71593654636555,4.85652673405237,1.44239581249904));
#9371=CARTESIAN_POINT('Ctrl Pts',(-4.84575797284515,4.72699165302455,1.45099687103942));
#9372=CARTESIAN_POINT('Ctrl Pts',(-4.97003164824036,4.59250197773384,1.4595979295798));
#9373=CARTESIAN_POINT('Ctrl Pts',(-5.09950788202557,4.45238206429071,1.46855906042938));
#9374=CARTESIAN_POINT('Ctrl Pts',(-5.22296162407326,4.3068840874192,1.47752019127895));
#9375=CARTESIAN_POINT('Ctrl Pts',(-5.33997329198447,4.15655797997485,1.48648132212853));
#9376=CARTESIAN_POINT('Ctrl Pts',(-5.45259162315717,4.01187603795759,1.49510599708373));
#9377=CARTESIAN_POINT('Ctrl Pts',(-5.55924268538611,3.86272218531277,1.50373067203892));
#9378=CARTESIAN_POINT('Ctrl Pts',(-5.659597629749,3.70961502980289,1.51235534699412));
#9379=CARTESIAN_POINT('Ctrl Pts',(-5.76004892269622,3.55636087946602,1.52098830231086));
#9380=CARTESIAN_POINT('Ctrl Pts',(-5.85419187260608,3.39914611040372,1.5296212576276));
#9381=CARTESIAN_POINT('Ctrl Pts',(-5.94174325319159,3.23851449173108,1.53825421294434));
#9382=CARTESIAN_POINT('Ctrl Pts',(-6.02942535205559,3.07764304258949,1.54690005766443));
#9383=CARTESIAN_POINT('Ctrl Pts',(-6.11049607590235,2.91334482106544,1.55554590238451));
#9384=CARTESIAN_POINT('Ctrl Pts',(-6.18471940918936,2.74618550531395,1.56419174710459));
#9385=CARTESIAN_POINT('Ctrl Pts',(-6.1931318604605,2.72723971648984,1.5651716646613));
#9386=CARTESIAN_POINT('Ctrl Pts',(-6.2014564030209,2.70825719217792,1.56615158221801));
#9387=CARTESIAN_POINT('Ctrl Pts',(-6.209692733347,2.68923876913477,1.56713149977472));
#9388=CARTESIAN_POINT('Ctrl Pts',(-6.2847318510522,2.51596673792696,1.57605928022646));
#9389=CARTESIAN_POINT('Ctrl Pts',(-6.35258133209611,2.33939829260565,1.58498706067819));
#9390=CARTESIAN_POINT('Ctrl Pts',(-6.41296689791982,2.16012605330908,1.59391484112993));
#9391=CARTESIAN_POINT('Ctrl Pts',(-6.47316786112979,1.98140186094215,1.60281532877446));
#9392=CARTESIAN_POINT('Ctrl Pts',(-6.52595035309913,1.7999906094939,1.61171581641899));
#9393=CARTESIAN_POINT('Ctrl Pts',(-6.57108874529099,1.61650292344622,1.62061630406351));
#9394=CARTESIAN_POINT('Ctrl Pts',(-6.61614205175235,1.43336111112258,1.6295000143162));
#9395=CARTESIAN_POINT('Ctrl Pts',(-6.65357993410146,1.24815091814942,1.63838372456888));
#9396=CARTESIAN_POINT('Ctrl Pts',(-6.68322586262152,1.06149944379957,1.64726743482156));
#9397=CARTESIAN_POINT('Ctrl Pts',(-6.71278037808465,0.875423508240538,1.65612375220271));
#9398=CARTESIAN_POINT('Ctrl Pts',(-6.73459082912758,0.687915409948818,1.66498006958387));
#9399=CARTESIAN_POINT('Ctrl Pts',(-6.74853140626713,0.499612708631656,1.67383638696503));
#9400=CARTESIAN_POINT('Ctrl Pts',(-6.76077955300093,0.334170554191592,1.68161751924669));
#9401=CARTESIAN_POINT('Ctrl Pts',(-6.76695336728736,0.168115363848341,1.68939865152836));
#9402=CARTESIAN_POINT('Ctrl Pts',(-6.76699973671697,0.00188766322821155,
1.69717978381002));
#9403=CARTESIAN_POINT('',(-6.7669988871634,0.00388086708922883,1.30263766580882));
#9404=CARTESIAN_POINT('Ctrl Pts',(3.09917575053259,6.01559628526639,0.651392015122069));
#9405=CARTESIAN_POINT('Ctrl Pts',(2.93382385406851,6.10078394805573,0.660141462533071));
#9406=CARTESIAN_POINT('Ctrl Pts',(2.76495774058454,6.17915009368906,0.668890909944073));
#9407=CARTESIAN_POINT('Ctrl Pts',(2.59315096270441,6.25042855207747,0.677640357355075));
#9408=CARTESIAN_POINT('Ctrl Pts',(2.42134557177907,6.32170643505203,0.686389734133892));
#9409=CARTESIAN_POINT('Ctrl Pts',(2.2465998286745,6.38589663545787,0.695139110912711));
#9410=CARTESIAN_POINT('Ctrl Pts',(2.06950724656412,6.44278113522558,0.703888487691529));
#9411=CARTESIAN_POINT('Ctrl Pts',(1.89241603525059,6.49966519467506,0.712637796745217));
#9412=CARTESIAN_POINT('Ctrl Pts',(1.71297829413072,6.54924357900826,0.721387105798904));
#9413=CARTESIAN_POINT('Ctrl Pts',(1.53180346303543,6.59134790089498,0.730136414852592));
#9414=CARTESIAN_POINT('Ctrl Pts',(1.35062997415456,6.63345191085632,0.738885659087957));
#9415=CARTESIAN_POINT('Ctrl Pts',(1.16771970017938,6.6680819043066,0.747634903323322));
#9416=CARTESIAN_POINT('Ctrl Pts',(0.983693865807499,6.69512026616197,0.756384147558687));
#9417=CARTESIAN_POINT('Ctrl Pts',(0.79966933364614,6.72215843668747,0.765133329882321));
#9418=CARTESIAN_POINT('Ctrl Pts',(0.614529540397793,6.74160504146313,0.773882512205955));
#9419=CARTESIAN_POINT('Ctrl Pts',(0.428903274066081,6.75339403422423,0.782631694529589));
#9420=CARTESIAN_POINT('Ctrl Pts',(0.243278259616313,6.76518294747919,0.79138081784787));
#9421=CARTESIAN_POINT('Ctrl Pts',(0.0571670646193069,6.76931433390325,0.80012994116615));
#9422=CARTESIAN_POINT('Ctrl Pts',(-0.128798232278501,6.76577416230855,0.808879064484431));
#9423=CARTESIAN_POINT('Ctrl Pts',(-0.314762336770819,6.76223401341335,0.817628131703521));
#9424=CARTESIAN_POINT('Ctrl Pts',(-0.500580258550281,6.75102241038819,0.826377198922611));
#9425=CARTESIAN_POINT('Ctrl Pts',(-0.685620923081958,6.73217743006171,0.835126266141701));
#9426=CARTESIAN_POINT('Ctrl Pts',(-0.870660462589858,6.71333256431032,0.843875280167572));
#9427=CARTESIAN_POINT('Ctrl Pts',(-1.05492246925224,6.68685444316035,0.852624294193443));
#9428=CARTESIAN_POINT('Ctrl Pts',(-1.23778116033235,6.65283299047303,0.861373308219314));
#9429=CARTESIAN_POINT('Ctrl Pts',(-1.42991953208325,6.6170850230927,0.870566315669095));
#9430=CARTESIAN_POINT('Ctrl Pts',(-1.62050811672427,6.57300825457429,0.879759323118877));
#9431=CARTESIAN_POINT('Ctrl Pts',(-1.808832359327,6.52076793758615,0.888952330568658));
#9432=CARTESIAN_POINT('Ctrl Pts',(-1.98808125918661,6.47104508077799,0.897702327111858));
#9433=CARTESIAN_POINT('Ctrl Pts',(-2.16527861796168,6.41392703709576,0.906452323655057));
#9434=CARTESIAN_POINT('Ctrl Pts',(-2.33982251053777,6.34960783192007,0.915202320198256));
#9435=CARTESIAN_POINT('Ctrl Pts',(-2.51436286473782,6.28528993063151,0.92395213936041));
#9436=CARTESIAN_POINT('Ctrl Pts',(-2.68624959139652,6.21377125909801,0.932701958522564));
#9437=CARTESIAN_POINT('Ctrl Pts',(-2.85489882883657,6.13529475062996,0.941451777684718));
#9438=CARTESIAN_POINT('Ctrl Pts',(-3.02354487157988,6.05681972873043,0.950201431100385));
#9439=CARTESIAN_POINT('Ctrl Pts',(-3.18895328794629,5.97138725457424,0.958951084516051));
#9440=CARTESIAN_POINT('Ctrl Pts',(-3.35056224292841,5.87928751263812,0.967700737931717));
#9441=CARTESIAN_POINT('Ctrl Pts',(-3.5121683513698,5.7871893929244,0.976450237233122));
#9442=CARTESIAN_POINT('Ctrl Pts',(-3.66997488333246,5.68842438234431,0.985199736534526));
#9443=CARTESIAN_POINT('Ctrl Pts',(-3.82344584363613,5.58332793956987,0.99394923583593));
#9444=CARTESIAN_POINT('Ctrl Pts',(-3.97691430468979,5.47823320827418,1.00269859265314));
#9445=CARTESIAN_POINT('Ctrl Pts',(-4.12604709891178,5.36680741303859,1.01144794947035));
#9446=CARTESIAN_POINT('Ctrl Pts',(-4.27033770824381,5.24942900300129,1.02019730628756));
#9447=CARTESIAN_POINT('Ctrl Pts',(-4.41462615955329,5.1320523484854,1.02894653224865));
#9448=CARTESIAN_POINT('Ctrl Pts',(-4.55407234859234,5.008723438162,1.03769575820974));
#9449=CARTESIAN_POINT('Ctrl Pts',(-4.68820267126408,4.87986113666694,1.04644498417083));
#9450=CARTESIAN_POINT('Ctrl Pts',(-4.82233116607775,4.75100059124012,1.05519409090203));
#9451=CARTESIAN_POINT('Ctrl Pts',(-4.95114373285208,4.61660700405917,1.06394319763323));
#9452=CARTESIAN_POINT('Ctrl Pts',(-5.07420289460218,4.47713680653282,1.07269230436443));
#9453=CARTESIAN_POINT('Ctrl Pts',(-5.19726054284679,4.33766832435139,1.08144130349031));
#9454=CARTESIAN_POINT('Ctrl Pts',(-5.31456473809728,4.19312357162134,1.09019030261618));
#9455=CARTESIAN_POINT('Ctrl Pts',(-5.42571709822437,4.04399344337201,1.09893930174206));
#9456=CARTESIAN_POINT('Ctrl Pts',(-5.53688157678416,3.89484705614786,1.10768925473124));
#9457=CARTESIAN_POINT('Ctrl Pts',(-5.64189270668245,3.74111452275908,1.11643920772042));
#9458=CARTESIAN_POINT('Ctrl Pts',(-5.7403937771409,3.5833180550102,1.12518916070959));
#9459=CARTESIAN_POINT('Ctrl Pts',(-5.83889104761745,3.42552767474563,1.13393877614241));
#9460=CARTESIAN_POINT('Ctrl Pts',(-5.93087860943509,3.2636739170053,1.14268839157523));
#9461=CARTESIAN_POINT('Ctrl Pts',(-6.01604401546832,3.09830653808622,1.15143800700804));
#9462=CARTESIAN_POINT('Ctrl Pts',(-6.10120658874526,2.93294465958691,1.16018733141274));
#9463=CARTESIAN_POINT('Ctrl Pts',(-6.17954732910422,2.76406964856331,1.16893665581743));
#9464=CARTESIAN_POINT('Ctrl Pts',(-6.25080016021907,2.59225507174839,1.17768598022213));
#9465=CARTESIAN_POINT('Ctrl Pts',(-6.32205100003899,2.4204452966163,1.18643506011043));
#9466=CARTESIAN_POINT('Ctrl Pts',(-6.38621421723416,2.24569638477739,1.19518413999873));
#9467=CARTESIAN_POINT('Ctrl Pts',(-6.44307190015638,2.06860181992941,1.20393321988703));
#9468=CARTESIAN_POINT('Ctrl Pts',(-6.49993470395433,1.89149130509521,1.21268308775944));
#9469=CARTESIAN_POINT('Ctrl Pts',(-6.54949056911377,1.71203498737916,1.22143295563185));
#9470=CARTESIAN_POINT('Ctrl Pts',(-6.5915711633095,1.53084244748656,1.23018282350427));
#9471=CARTESIAN_POINT('Ctrl Pts',(-6.63364884164169,1.34966246285206,1.23893208507771));
#9472=CARTESIAN_POINT('Ctrl Pts',(-6.66825222068406,1.16674677594928,1.24768134665116));
#9473=CARTESIAN_POINT('Ctrl Pts',(-6.69526377527894,0.982716632319621,1.25643060822461));
#9474=CARTESIAN_POINT('Ctrl Pts',(-6.72227670080852,0.798677148490385,1.26518031385493));
#9475=CARTESIAN_POINT('Ctrl Pts',(-6.74169698918657,0.613523378321138,1.27393001948524));
#9476=CARTESIAN_POINT('Ctrl Pts',(-6.75345867564419,0.427884232434633,1.28267972511556));
#9477=CARTESIAN_POINT('Ctrl Pts',(-6.76240141614664,0.286737576745467,1.28933237201331));
#9478=CARTESIAN_POINT('Ctrl Pts',(-6.76691777740362,0.145310511934777,1.29598501891107));
#9479=CARTESIAN_POINT('Ctrl Pts',(-6.7669988871634,0.00388086708923183,
1.30263766580882));
#9480=CARTESIAN_POINT('Ctrl Pts',(-6.76699888234511,0.00388925958011982,
1.30282022489417));
#9481=CARTESIAN_POINT('Ctrl Pts',(-6.76709704828634,-0.166911583330251,
1.31088823850834));
#9482=CARTESIAN_POINT('Ctrl Pts',(-6.76072447256501,-0.337975125809719,
1.31895625212251));
#9483=CARTESIAN_POINT('Ctrl Pts',(-6.74784790637245,-0.508760879456122,
1.32702426573667));
#9484=CARTESIAN_POINT('Ctrl Pts',(-6.73498437417603,-0.679373759308398,
1.33508411269704));
#9485=CARTESIAN_POINT('Ctrl Pts',(-6.71562998115061,-0.849709041106061,
1.3431439596574));
#9486=CARTESIAN_POINT('Ctrl Pts',(-6.68980346698226,-1.01922449595371,1.35120380661777));
#9487=CARTESIAN_POINT('Ctrl Pts',(-6.66399744413831,-1.18860545351101,1.35925725871828));
#9488=CARTESIAN_POINT('Ctrl Pts',(-6.631729577102,-1.3571675119843,1.36731071081879));
#9489=CARTESIAN_POINT('Ctrl Pts',(-6.59307054474703,-1.52437193361366,1.3753641629193));
#9490=CARTESIAN_POINT('Ctrl Pts',(-6.55443373493223,-1.69148024039619,1.38341298561882));
#9491=CARTESIAN_POINT('Ctrl Pts',(-6.50941315756628,-1.8572321015694,1.39146180831834));
#9492=CARTESIAN_POINT('Ctrl Pts',(-6.45813084501019,-2.02109747135758,1.39951063101786));
#9493=CARTESIAN_POINT('Ctrl Pts',(-6.40685982948131,-2.18492674309461,1.40755768063491));
#9494=CARTESIAN_POINT('Ctrl Pts',(-6.34932992906808,-2.34686999290344,1.41560473025197));
#9495=CARTESIAN_POINT('Ctrl Pts',(-6.28571348724989,-2.50641077164235,1.42365177986902));
#9496=CARTESIAN_POINT('Ctrl Pts',(-6.22210246312151,-2.66593796360361,1.43169814418496));
#9497=CARTESIAN_POINT('Ctrl Pts',(-6.15240606641361,-2.82306274460335,1.4397445085009));
#9498=CARTESIAN_POINT('Ctrl Pts',(-6.07684530578212,-2.97728737773058,1.44779087281684));
#9499=CARTESIAN_POINT('Ctrl Pts',(-6.00127603156627,-3.13152938766044,1.45583814373299));
#9500=CARTESIAN_POINT('Ctrl Pts',(-5.91984124224131,-3.28287026394481,1.46388541464914));
#9501=CARTESIAN_POINT('Ctrl Pts',(-5.83280847428983,-3.43083580228679,1.47193268556529));
#9502=CARTESIAN_POINT('Ctrl Pts',(-5.74574867847249,-3.57884729105428,1.47998245554661));
#9503=CARTESIAN_POINT('Ctrl Pts',(-5.65308763304491,-3.72348103402496,1.48803222552792));
#9504=CARTESIAN_POINT('Ctrl Pts',(-5.55513677578713,-3.86429093137375,1.49608199550924));
#9505=CARTESIAN_POINT('Ctrl Pts',(-5.45707735362938,-4.0052568969066,1.50414068754083));
#9506=CARTESIAN_POINT('Ctrl Pts',(-5.35371662344936,-4.14239024572985,1.51219937957242));
#9507=CARTESIAN_POINT('Ctrl Pts',(-5.24540748325654,-4.27527652141897,1.52025807160401));
#9508=CARTESIAN_POINT('Ctrl Pts',(-5.13703552073096,-4.40823987486733,1.52832143790253));
#9509=CARTESIAN_POINT('Ctrl Pts',(-5.02370967782438,-4.53695096962361,1.53638480420105));
#9510=CARTESIAN_POINT('Ctrl Pts',(-4.90582009191361,-4.66103188422658,1.54444817049957));
#9511=CARTESIAN_POINT('Ctrl Pts',(-4.78774817794154,-4.78530470240126,1.55252400760231));
#9512=CARTESIAN_POINT('Ctrl Pts',(-4.66509868858995,-4.90493277636546,1.56059984470504));
#9513=CARTESIAN_POINT('Ctrl Pts',(-4.53829604923321,-5.01957746922131,1.56867568180778));
#9514=CARTESIAN_POINT('Ctrl Pts',(-4.43183989767127,-5.11582651309254,1.57545568688464));
#9515=CARTESIAN_POINT('Ctrl Pts',(-4.32245714146461,-5.20856377686059,1.5822356919615));
#9516=CARTESIAN_POINT('Ctrl Pts',(-4.21041417240527,-5.29761281114512,1.58901569703837));
#9517=CARTESIAN_POINT('Ctrl Pts',(-4.07461375508114,-5.40554368909021,1.59723332574482));
#9518=CARTESIAN_POINT('Ctrl Pts',(-3.93445583250538,-5.50841221031713,1.60545095445126));
#9519=CARTESIAN_POINT('Ctrl Pts',(-3.79035361516694,-5.6058459193944,1.61366858315771));
#9520=CARTESIAN_POINT('Ctrl Pts',(-3.64642540015359,-5.70316197801332,1.62187628914036));
#9521=CARTESIAN_POINT('Ctrl Pts',(-3.49856266833718,-5.7950560916103,1.63008399512301));
#9522=CARTESIAN_POINT('Ctrl Pts',(-3.34721244403314,-5.88119527430519,1.63829170110566));
#9523=CARTESIAN_POINT('Ctrl Pts',(-3.19601434056076,-5.96724787923536,1.64649115759237));
#9524=CARTESIAN_POINT('Ctrl Pts',(-3.04133603523146,-6.04755689511507,1.65469061407908));
#9525=CARTESIAN_POINT('Ctrl Pts',(-2.88365440396457,-6.12183193811262,1.66289007056579));
#9526=CARTESIAN_POINT('Ctrl Pts',(-2.72609935444989,-6.19604735548979,1.67108294479203));
#9527=CARTESIAN_POINT('Ctrl Pts',(-2.56554610473802,-6.26423829474248,1.67927581901827));
#9528=CARTESIAN_POINT('Ctrl Pts',(-2.40249712904587,-6.32615969960657,1.68746869324451));
#9529=CARTESIAN_POINT('Ctrl Pts',(-2.2395460639878,-6.3880439207718,1.69565664766363));
#9530=CARTESIAN_POINT('Ctrl Pts',(-2.07410259367583,-6.44366597973139,1.70384460208275));
#9531=CARTESIAN_POINT('Ctrl Pts',(-1.9066902882976,-6.49282843947933,1.71203255650188));
#9532=CARTESIAN_POINT('Ctrl Pts',(-1.73932881463813,-6.54197597193551,1.72021802479673));
#9533=CARTESIAN_POINT('Ctrl Pts',(-1.57000004024041,-6.58466770686101,1.72840349309158));
#9534=CARTESIAN_POINT('Ctrl Pts',(-1.39924407841513,-6.62075562220961,1.73658896138643));
#9535=CARTESIAN_POINT('Ctrl Pts',(-1.2285124106804,-6.65683840319527,1.74477326510403));
#9536=CARTESIAN_POINT('Ctrl Pts',(-1.0563543116645,-6.6863191605116,1.75295756882163));
#9537=CARTESIAN_POINT('Ctrl Pts',(-0.883321511936119,-6.70910069283141,
1.76114187253924));
#9538=CARTESIAN_POINT('Ctrl Pts',(-0.71028162461133,-6.73188315830555,1.7693265114941));
#9539=CARTESIAN_POINT('Ctrl Pts',(-0.536367321981056,-6.74796580506379,
1.77751115044896));
#9540=CARTESIAN_POINT('Ctrl Pts',(-0.362136944529296,-6.75730314795829,
1.78569578940383));
#9541=CARTESIAN_POINT('Ctrl Pts',(-0.187867505324042,-6.7666425842477,1.79388226332199));
#9542=CARTESIAN_POINT('Ctrl Pts',(-0.0132822094303347,-6.76923368560635,
1.80206873724016));
#9543=CARTESIAN_POINT('Ctrl Pts',(0.161059064643997,-6.76508307249039,1.81025521115833));
#9544=CARTESIAN_POINT('Ctrl Pts',(0.335565213747655,-6.76092853412802,1.81844942704772));
#9545=CARTESIAN_POINT('Ctrl Pts',(0.509826519751691,-6.75001955194915,1.82664364293712));
#9546=CARTESIAN_POINT('Ctrl Pts',(0.683285754315221,-6.73241484000725,1.83483785882651));
#9547=CARTESIAN_POINT('Ctrl Pts',(0.856828512439003,-6.71480165109829,1.84303602036968));
#9548=CARTESIAN_POINT('Ctrl Pts',(1.02956807303185,-6.69048635478854,1.85123418191286));
#9549=CARTESIAN_POINT('Ctrl Pts',(1.20095600065172,-6.65957909214228,1.85943234345603));
#9550=CARTESIAN_POINT('Ctrl Pts',(1.37258163648686,-6.62862896235629,1.86764187552207));
#9551=CARTESIAN_POINT('Ctrl Pts',(1.54285154136209,-6.59106867194669,1.8758514075881));
#9552=CARTESIAN_POINT('Ctrl Pts',(1.71122987766881,-6.54705898138803,1.88406093965413));
#9553=CARTESIAN_POINT('Ctrl Pts',(1.86681880238214,-6.50639210831407,1.89164690525144));
#9554=CARTESIAN_POINT('Ctrl Pts',(2.02079255608343,-6.46021898958428,1.89923287084874));
#9555=CARTESIAN_POINT('Ctrl Pts',(2.17274339940872,-6.40870307631161,1.90681883644604));
#9556=CARTESIAN_POINT('Ctrl Pts',(2.34617658434546,-6.34990400209602,1.9154772824643));
#9557=CARTESIAN_POINT('Ctrl Pts',(2.51737466941937,-6.28400871360894,1.92413572848256));
#9558=CARTESIAN_POINT('Ctrl Pts',(2.68575184058637,-6.21120165916282,1.93279417450082));
#9559=CARTESIAN_POINT('Ctrl Pts',(2.85391124251773,-6.13848876912442,1.94144142218881));
#9560=CARTESIAN_POINT('Ctrl Pts',(3.01925672896684,-6.05888205885241,1.95008866987681));
#9561=CARTESIAN_POINT('Ctrl Pts',(3.18121968350465,-5.97261503240269,1.95873591756481));
#9562=CARTESIAN_POINT('Ctrl Pts',(3.34820464494508,-5.88367311277425,1.96765129161356));
#9563=CARTESIAN_POINT('Ctrl Pts',(3.51159362552328,-5.7876512745346,1.97656666566232));
#9564=CARTESIAN_POINT('Ctrl Pts',(3.67078501067243,-5.68485940067322,1.98548203971107));
#9565=CARTESIAN_POINT('Ctrl Pts',(3.8247536597855,-5.58543991297035,1.99410491900406));
#9566=CARTESIAN_POINT('Ctrl Pts',(3.97479546597253,-5.47968771741926,2.00272779829704));
#9567=CARTESIAN_POINT('Ctrl Pts',(4.12038995361317,-5.36793029296801,2.01135067759003));
#9568=CARTESIAN_POINT('Ctrl Pts',(4.27339245822644,-5.25048652069846,2.02041229901667));
#9569=CARTESIAN_POINT('Ctrl Pts',(4.42148297714327,-5.12641061677613,2.02947392044331));
#9570=CARTESIAN_POINT('Ctrl Pts',(4.56409038230586,-4.99613530462728,2.03853554186995));
#9571=CARTESIAN_POINT('Ctrl Pts',(4.69949920388821,-4.87243607260469,2.04713974778483));
#9572=CARTESIAN_POINT('Ctrl Pts',(4.82996451064429,-4.74314806876094,2.05574395369972));
#9573=CARTESIAN_POINT('Ctrl Pts',(4.95502957298067,-4.60868429498995,2.0643481596146));
#9574=CARTESIAN_POINT('Ctrl Pts',(4.96167826317439,-4.60153595190051,2.06480557512635));
#9575=CARTESIAN_POINT('Ctrl Pts',(4.96831169919643,-4.59437299049623,2.06526299063811));
#9576=CARTESIAN_POINT('Ctrl Pts',(4.9749298151216,-4.58719547595415,2.06572040614986));
#9577=CARTESIAN_POINT('Ctrl Pts',(5.09926231861951,-4.45235372310475,2.07431373034638));
#9578=CARTESIAN_POINT('Ctrl Pts',(5.21803628917243,-4.31253349391377,2.08290705454289));
#9579=CARTESIAN_POINT('Ctrl Pts',(5.33087497953295,-4.16822035796928,2.09150037873941));
#9580=CARTESIAN_POINT('Ctrl Pts',(5.44381910882233,-4.02377237268877,2.10010173272514));
#9581=CARTESIAN_POINT('Ctrl Pts',(5.55081669959559,-3.87482334158127,2.10870308671086));
#9582=CARTESIAN_POINT('Ctrl Pts',(5.65153378452362,-3.72188861767627,2.11730444069659));
#9583=CARTESIAN_POINT('Ctrl Pts',(5.75625285279107,-3.56287704774733,2.12624756862635));
#9584=CARTESIAN_POINT('Ctrl Pts',(5.85418190555349,-3.39955689125769,2.13519069655611));
#9585=CARTESIAN_POINT('Ctrl Pts',(5.94499829711266,-3.2325352662156,2.14413382448587));
#9586=CARTESIAN_POINT('Ctrl Pts',(6.03258260228007,-3.0714578139397,2.15275867328578));
#9587=CARTESIAN_POINT('Ctrl Pts',(6.11355169969962,-2.90693810381944,2.16138352208569));
#9588=CARTESIAN_POINT('Ctrl Pts',(6.18766535016368,-2.73954129634576,2.1700083708856));
#9589=CARTESIAN_POINT('Ctrl Pts',(6.26184988137288,-2.57198439406669,2.1786414683105));
#9590=CARTESIAN_POINT('Ctrl Pts',(6.32916576362738,-2.40154518468651,2.18727456573541));
#9591=CARTESIAN_POINT('Ctrl Pts',(6.38942186041684,-2.2288062476643,2.19590766316031));
#9592=CARTESIAN_POINT('Ctrl Pts',(6.44976743376656,-2.05581080405222,2.20455358019855));
#9593=CARTESIAN_POINT('Ctrl Pts',(6.50303217958239,-1.88050909936569,2.21319949723679));
#9594=CARTESIAN_POINT('Ctrl Pts',(6.54907510496199,-1.70349765763476,2.22184541427503));
#9595=CARTESIAN_POINT('Ctrl Pts',(6.55400386756034,-1.68454909243631,2.22277093480126));
#9596=CARTESIAN_POINT('Ctrl Pts',(6.55884992321818,-1.66558094336064,2.22369645532748));
#9597=CARTESIAN_POINT('Ctrl Pts',(6.5636131339237,-1.64659394757308,2.22462197585371));
#9598=CARTESIAN_POINT('Ctrl Pts',(6.60594263129275,-1.47786112470964,2.23284685211935));
#9599=CARTESIAN_POINT('Ctrl Pts',(6.64181725648561,-1.30727253348678,2.24107172838499));
#9600=CARTESIAN_POINT('Ctrl Pts',(6.6710748893297,-1.13536285871732,2.24929660465063));
#9601=CARTESIAN_POINT('Ctrl Pts',(6.7003017416724,-0.963634041572632,2.25751282793273));
#9602=CARTESIAN_POINT('Ctrl Pts',(6.72292540467277,-0.790587258972482,2.26572905121483));
#9603=CARTESIAN_POINT('Ctrl Pts',(6.7388339249604,-0.616770890852404,2.27394527449693));
#9604=CARTESIAN_POINT('Ctrl Pts',(6.7547288948653,-0.443102574107876,2.28215449945561));
#9605=CARTESIAN_POINT('Ctrl Pts',(6.76392008114605,-0.268666332271811,2.2903637244143));
#9606=CARTESIAN_POINT('Ctrl Pts',(6.76634682560446,-0.0940193364815904,
2.29857294937299));
#9607=CARTESIAN_POINT('Ctrl Pts',(6.76877198893167,0.0805138690767463,2.30677682565902));
#9608=CARTESIAN_POINT('Ctrl Pts',(6.76444148450205,0.255257197980979,2.31498070194504));
#9609=CARTESIAN_POINT('Ctrl Pts',(6.75334658911855,0.429649679670336,2.32318457823107));
#9610=CARTESIAN_POINT('Ctrl Pts',(6.74225670153002,0.603963447522276,2.33138475161329));
#9611=CARTESIAN_POINT('Ctrl Pts',(6.72440852847687,0.777926326716095,2.33958492499551));
#9612=CARTESIAN_POINT('Ctrl Pts',(6.69984542688093,0.950978578046184,2.34778509837773));
#9613=CARTESIAN_POINT('Ctrl Pts',(6.6752843512477,1.12401655604,2.35598459541029));
#9614=CARTESIAN_POINT('Ctrl Pts',(6.64400949203572,1.29614369999235,2.36418409244284));
#9615=CARTESIAN_POINT('Ctrl Pts',(6.60611598786299,1.46680624313542,2.3723835894754));
#9616=CARTESIAN_POINT('Ctrl Pts',(6.56822277133648,1.63746749079427,2.3805830242663));
#9617=CARTESIAN_POINT('Ctrl Pts',(6.52371108658861,1.8066638095827,2.3887824590572));
#9618=CARTESIAN_POINT('Ctrl Pts',(6.47272701235145,1.9738525840538,2.3969818938481));
#9619=CARTESIAN_POINT('Ctrl Pts',(6.42173407708048,2.14107041593953,2.40518275370104));
#9620=CARTESIAN_POINT('Ctrl Pts',(6.36426661572915,2.30627966545076,2.41338361355399));
#9621=CARTESIAN_POINT('Ctrl Pts',(6.30052032183935,2.46895376102699,2.42158447340693));
#9622=CARTESIAN_POINT('Ctrl Pts',(6.23675138571998,2.63168563728338,2.42978824614688));
#9623=CARTESIAN_POINT('Ctrl Pts',(6.16669930513151,2.79188023225607,2.43799201888684));
#9624=CARTESIAN_POINT('Ctrl Pts',(6.09060758166292,2.94903175401524,2.44619579162679));
#9625=CARTESIAN_POINT('Ctrl Pts',(6.01442912047239,3.10636241437681,2.45440891592992));
#9626=CARTESIAN_POINT('Ctrl Pts',(5.93219741848239,3.26064274842366,2.46262204023304));
#9627=CARTESIAN_POINT('Ctrl Pts',(5.84420205173538,3.41139141385037,2.47083516453617));
#9628=CARTESIAN_POINT('Ctrl Pts',(5.75615469141516,3.56222915171421,2.4790531417048));
#9629=CARTESIAN_POINT('Ctrl Pts',(5.66233707004052,3.70953075941405,2.48727111887342));
#9630=CARTESIAN_POINT('Ctrl Pts',(5.56308156368259,3.85284473030188,2.49548909604205));
#9631=CARTESIAN_POINT('Ctrl Pts',(5.46367237026505,3.9963806083019,2.50371979791275));
#9632=CARTESIAN_POINT('Ctrl Pts',(5.35880868062565,4.13591622413822,2.51195049978345));
#9633=CARTESIAN_POINT('Ctrl Pts',(5.24886338443184,4.27103291623593,2.52018120165414));
#9634=CARTESIAN_POINT('Ctrl Pts',(5.14981902958912,4.39275295393276,2.52759583952322));
#9635=CARTESIAN_POINT('Ctrl Pts',(5.04665142495269,4.51088722119783,2.5350104773923));
#9636=CARTESIAN_POINT('Ctrl Pts',(4.93965759606199,4.62515641180567,2.54242511526138));
#9637=CARTESIAN_POINT('Ctrl Pts',(4.82192603404906,4.75089347944494,2.55058387457617));
#9638=CARTESIAN_POINT('Ctrl Pts',(4.69919892592138,4.87233694864273,2.55874263389096));
#9639=CARTESIAN_POINT('Ctrl Pts',(4.57182321124844,4.9890601845528,2.56690139320575));
#9640=CARTESIAN_POINT('Ctrl Pts',(4.44464415896944,5.10560320501866,2.57504755576187));
#9641=CARTESIAN_POINT('Ctrl Pts',(4.31283106579809,5.21744026702449,2.58319371831799));
#9642=CARTESIAN_POINT('Ctrl Pts',(4.17677003524039,5.32417891066012,2.59133988087411));
#9643=CARTESIAN_POINT('Ctrl Pts',(4.04083006405777,5.4308225843147,2.59947879543758));
#9644=CARTESIAN_POINT('Ctrl Pts',(3.900649961062,5.53237664176759,2.60761771000106));
#9645=CARTESIAN_POINT('Ctrl Pts',(3.75665199545179,5.62848601180354,2.61575662456454));
#9646=CARTESIAN_POINT('Ctrl Pts',(3.61277866478679,5.72451219603879,2.62388849463147));
#9647=CARTESIAN_POINT('Ctrl Pts',(3.46509435600694,5.81510287755278,2.63202036469841));
#9648=CARTESIAN_POINT('Ctrl Pts',(3.31405342985844,5.89994397126308,2.64015223476534));
#9649=CARTESIAN_POINT('Ctrl Pts',(3.24315034852982,5.93977089182523,2.64396957526644));
#9650=CARTESIAN_POINT('Ctrl Pts',(3.17150803856598,5.97833140537366,2.64778691576753));
#9651=CARTESIAN_POINT('Ctrl Pts',(3.09917575053259,6.01559628526639,2.65160425626863));
#9652=CARTESIAN_POINT('Origin',(0.,0.,-3.69717978381041));
#9653=CARTESIAN_POINT('',(3.09917575053259,6.01559628526639,5.04568623149126));
#9654=CARTESIAN_POINT('',(3.09917575053259,6.01559628526639,4.6512641878525));
#9655=CARTESIAN_POINT('',(3.09917575053259,6.01559628526639,-3.69717978381041));
#9656=CARTESIAN_POINT('',(-6.767,1.74262947821857E-12,3.69717978381002));
#9657=CARTESIAN_POINT('Ctrl Pts',(-6.76699874815404,-0.00411612459687825,
3.69717978381002));
#9658=CARTESIAN_POINT('Ctrl Pts',(-6.76687514509871,-0.207322247497207,
3.70672388776635));
#9659=CARTESIAN_POINT('Ctrl Pts',(-6.75759441333246,-0.410217053170746,
3.71626799172269));
#9660=CARTESIAN_POINT('Ctrl Pts',(-6.73926461418622,-0.612046942625711,
3.72581209567903));
#9661=CARTESIAN_POINT('Ctrl Pts',(-6.72085546075771,-0.814750604122016,
3.73539751844705));
#9662=CARTESIAN_POINT('Ctrl Pts',(-6.69331880047275,-1.01638001069333,3.74498294121508));
#9663=CARTESIAN_POINT('Ctrl Pts',(-6.65681420104171,-1.21618818149556,3.75456836398311));
#9664=CARTESIAN_POINT('Ctrl Pts',(-6.62013581135308,-1.41694759444292,3.76419942081144));
#9665=CARTESIAN_POINT('Ctrl Pts',(-6.57440394949044,-1.61586829355856,3.77383047763978));
#9666=CARTESIAN_POINT('Ctrl Pts',(-6.51982988362059,-1.81221060824836,3.78346153446811));
#9667=CARTESIAN_POINT('Ctrl Pts',(-6.49850475257701,-1.88893250029406,3.78722492547955));
#9668=CARTESIAN_POINT('Ctrl Pts',(-6.47583003097947,-1.9652609000595,3.79098831649099));
#9669=CARTESIAN_POINT('Ctrl Pts',(-6.45182033297249,-2.04115246638823,3.79475170750244));
#9670=CARTESIAN_POINT('Ctrl Pts',(-6.39934861310573,-2.20700882191145,3.80297636733964));
#9671=CARTESIAN_POINT('Ctrl Pts',(-6.34040815136586,-2.37105913358796,3.81120102717685));
#9672=CARTESIAN_POINT('Ctrl Pts',(-6.27514141282242,-2.53276316482239,3.81942568701406));
#9673=CARTESIAN_POINT('Ctrl Pts',(-6.20994328005258,-2.69429721927526,3.82764170141925));
#9674=CARTESIAN_POINT('Ctrl Pts',(-6.13843224588407,-2.85348957496219,3.83585771582444));
#9675=CARTESIAN_POINT('Ctrl Pts',(-6.06080066937938,-3.00981465310582,3.84407373022964));
#9676=CARTESIAN_POINT('Ctrl Pts',(-5.98323514607949,-3.16600672129568,3.85228275399897));
#9677=CARTESIAN_POINT('Ctrl Pts',(-5.89955961069964,-3.31933605155709,3.86049177776831));
#9678=CARTESIAN_POINT('Ctrl Pts',(-5.81001470431116,-3.46929649002331,3.86870080153765));
#9679=CARTESIAN_POINT('Ctrl Pts',(-5.72052805641934,-3.61915936325602,3.8769044844629));
#9680=CARTESIAN_POINT('Ctrl Pts',(-5.6251798270287,-3.76565740397587,3.88510816738816));
#9681=CARTESIAN_POINT('Ctrl Pts',(-5.52425686518469,-3.90830846882124,3.89331185031341));
#9682=CARTESIAN_POINT('Ctrl Pts',(-5.42337935892376,-4.05089528379511,3.90151183830954));
#9683=CARTESIAN_POINT('Ctrl Pts',(-5.3169323290966,-4.18963828286598,3.90971182630567));
#9684=CARTESIAN_POINT('Ctrl Pts',(-5.2052463170163,-4.32408369243569,3.9179118143018));
#9685=CARTESIAN_POINT('Ctrl Pts',(-5.09356924072396,-4.45851834528081,3.9261111462323));
#9686=CARTESIAN_POINT('Ctrl Pts',(-4.97665423921318,-4.58865581243468,3.9343104781628));
#9687=CARTESIAN_POINT('Ctrl Pts',(-4.85487280636697,-4.7140745681415,3.94250981009329));
#9688=CARTESIAN_POINT('Ctrl Pts',(-4.73309217086887,-4.83949250268532,3.95070908833973));
#9689=CARTESIAN_POINT('Ctrl Pts',(-4.60644541647417,-4.96019152935117,3.95890836658617));
#9690=CARTESIAN_POINT('Ctrl Pts',(-4.47534155471156,-5.07578633993512,3.96710764483261));
#9691=CARTESIAN_POINT('Ctrl Pts',(-4.34421476743135,-5.1914013640416,3.97530835684839));
#9692=CARTESIAN_POINT('Ctrl Pts',(-4.20862958889401,-5.30191015669955,3.98350906886417));
#9693=CARTESIAN_POINT('Ctrl Pts',(-4.06902885310209,-5.40696709742372,3.99170978087996));
#9694=CARTESIAN_POINT('Ctrl Pts',(-3.92937838036582,-5.51206146783037,3.99991341464507));
#9695=CARTESIAN_POINT('Ctrl Pts',(-3.78570978670595,-5.61169990152915,4.00811704841019));
#9696=CARTESIAN_POINT('Ctrl Pts',(-3.63849570577419,-5.7055795497971,4.01632068217531));
#9697=CARTESIAN_POINT('Ctrl Pts',(-3.49111298434392,-5.79956674151865,4.0245337135801));
#9698=CARTESIAN_POINT('Ctrl Pts',(-3.3401769639609,-5.88778177515888,4.0327467449849));
#9699=CARTESIAN_POINT('Ctrl Pts',(-3.18618668325835,-5.96996678545427,4.04095977638969));
#9700=CARTESIAN_POINT('Ctrl Pts',(-3.0321052852362,-6.05220042529832,4.04917766751293));
#9701=CARTESIAN_POINT('Ctrl Pts',(-2.87496634646817,-6.12839677324508,4.05739555863617));
#9702=CARTESIAN_POINT('Ctrl Pts',(-2.71528969016249,-6.19834581953099,4.0656134497594));
#9703=CARTESIAN_POINT('Ctrl Pts',(-2.55536399152904,-6.26840396299939,4.07384415805193));
#9704=CARTESIAN_POINT('Ctrl Pts',(-2.39289299910971,-6.33219520177195,4.08207486634445));
#9705=CARTESIAN_POINT('Ctrl Pts',(-2.22841381171218,-6.38955873936302,4.09030557463697));
#9706=CARTESIAN_POINT('Ctrl Pts',(-2.07735383705311,-6.44224221057887,4.0978647716744));
#9707=CARTESIAN_POINT('Ctrl Pts',(-1.92460035350539,-6.48950454530975,4.10542396871184));
#9708=CARTESIAN_POINT('Ctrl Pts',(-1.77057662546198,-6.53125925173452,4.11298316574927));
#9709=CARTESIAN_POINT('Ctrl Pts',(-1.60443543898398,-6.57629891253597,4.12113706502553));
#9710=CARTESIAN_POINT('Ctrl Pts',(-1.43630241505965,-6.61506879967032,4.12929096430179));
#9711=CARTESIAN_POINT('Ctrl Pts',(-1.26669608406012,-6.647388211217,4.13744486357804));
#9712=CARTESIAN_POINT('Ctrl Pts',(-1.09729671869426,-6.67966818433323,4.14558881289005));
#9713=CARTESIAN_POINT('Ctrl Pts',(-0.926427980106585,-6.705513282256,4.15373276220206));
#9714=CARTESIAN_POINT('Ctrl Pts',(-0.754624309461781,-6.72479227571896,
4.16187671151406));
#9715=CARTESIAN_POINT('Ctrl Pts',(-0.58299412470652,-6.74405180141782,4.17001243713512));
#9716=CARTESIAN_POINT('Ctrl Pts',(-0.410431248022078,-6.75675838200398,
4.17814816275618));
#9717=CARTESIAN_POINT('Ctrl Pts',(-0.237481088370139,-6.7628316356883,4.18628388837724));
#9718=CARTESIAN_POINT('Ctrl Pts',(-0.0646691923669045,-6.76890003415761,
4.19441310995626));
#9719=CARTESIAN_POINT('Ctrl Pts',(0.108529006420706,-6.76834565170371,4.20254233153528));
#9720=CARTESIAN_POINT('Ctrl Pts',(0.281562188883845,-6.76113982504363,4.2106715531143));
#9721=CARTESIAN_POINT('Ctrl Pts',(0.454493423549635,-6.75393824391694,4.21879598511352));
#9722=CARTESIAN_POINT('Ctrl Pts',(0.627259471093833,-6.74009303809521,4.22692041711275));
#9723=CARTESIAN_POINT('Ctrl Pts',(0.799308222788764,-6.71962762100567,4.23504484911198));
#9724=CARTESIAN_POINT('Ctrl Pts',(0.972401168918694,-6.69903799566454,4.24321858973215));
#9725=CARTESIAN_POINT('Ctrl Pts',(1.14476770881433,-6.67174752452259,4.25139233035232));
#9726=CARTESIAN_POINT('Ctrl Pts',(1.31584942939305,-6.63783317650918,4.25956607097249));
#9727=CARTESIAN_POINT('Ctrl Pts',(1.48583584150506,-6.60413595673365,4.26768748123687));
#9728=CARTESIAN_POINT('Ctrl Pts',(1.65455347901243,-6.56389952228322,4.27580889150126));
#9729=CARTESIAN_POINT('Ctrl Pts',(1.82146379873784,-6.51725084908411,4.28393030176565));
#9730=CARTESIAN_POINT('Ctrl Pts',(1.98838702354686,-6.47059856912761,4.29205233995692));
#9731=CARTESIAN_POINT('Ctrl Pts',(2.15350229973429,-6.41753316134611,4.3001743781482));
#9732=CARTESIAN_POINT('Ctrl Pts',(2.31628549880373,-6.35823171078497,4.30829641633948));
#9733=CARTESIAN_POINT('Ctrl Pts',(2.47911228141139,-6.29891438286639,4.3164206291235));
#9734=CARTESIAN_POINT('Ctrl Pts',(2.63960539989487,-6.23335781284451,4.32454484190751));
#9735=CARTESIAN_POINT('Ctrl Pts',(2.79726002877108,-6.16178751105875,4.33266905469152));
#9736=CARTESIAN_POINT('Ctrl Pts',(2.95662075258456,-6.08944269519494,4.3408811854669));
#9737=CARTESIAN_POINT('Ctrl Pts',(3.11308084356436,-6.0109533872662,4.34909331624228));
#9738=CARTESIAN_POINT('Ctrl Pts',(3.26614451899616,-5.92660011988588,4.35730544701766));
#9739=CARTESIAN_POINT('Ctrl Pts',(3.41781127900701,-5.84301669146101,4.36544263086597));
#9740=CARTESIAN_POINT('Ctrl Pts',(3.5661430787814,-5.75367613426408,4.37357981471428));
#9741=CARTESIAN_POINT('Ctrl Pts',(3.71068719452792,-5.6588947281573,4.3817169985626));
#9742=CARTESIAN_POINT('Ctrl Pts',(3.85722827952742,-5.56280385640558,4.38996660280151));
#9743=CARTESIAN_POINT('Ctrl Pts',(3.99987593618909,-5.46112092530692,4.39821620704042));
#9744=CARTESIAN_POINT('Ctrl Pts',(4.13819382896349,-5.35421710747038,4.40646581127933));
#9745=CARTESIAN_POINT('Ctrl Pts',(4.27651172173791,-5.24731328963384,4.41471541551824));
#9746=CARTESIAN_POINT('Ctrl Pts',(4.41049959614208,-5.13518888050348,4.42296501975715));
#9747=CARTESIAN_POINT('Ctrl Pts',(4.5397608289452,-5.01825274532629,4.43121462399606));
#9748=CARTESIAN_POINT('Ctrl Pts',(4.6686344797541,-4.90166723608299,4.43943949229526));
#9749=CARTESIAN_POINT('Ctrl Pts',(4.79319512442212,-4.77995045954151,4.44766436059445));
#9750=CARTESIAN_POINT('Ctrl Pts',(4.91300921252629,-4.65345350010418,4.45588922889364));
#9751=CARTESIAN_POINT('Ctrl Pts',(5.03268831700465,-4.5270990532754,4.46410483098248));
#9752=CARTESIAN_POINT('Ctrl Pts',(5.14763126871457,-4.3959754053497,4.47232043307131));
#9753=CARTESIAN_POINT('Ctrl Pts',(5.25743829939608,-4.26047315776585,4.48053603516014));
#9754=CARTESIAN_POINT('Ctrl Pts',(5.36714368291744,-4.12509634312172,4.48874403215651));
#9755=CARTESIAN_POINT('Ctrl Pts',(5.47172238916977,-3.98534927787293,4.49695202915288));
#9756=CARTESIAN_POINT('Ctrl Pts',(5.57081212771845,-3.84165865709917,4.50516002614925));
#9757=CARTESIAN_POINT('Ctrl Pts',(5.66983004266583,-3.69807218815797,4.51336207371117));
#9758=CARTESIAN_POINT('Ctrl Pts',(5.76336671165853,-3.55054815128399,4.5215641212731));
#9759=CARTESIAN_POINT('Ctrl Pts',(5.85110066242351,-3.39954556348157,4.52976616883502));
#9760=CARTESIAN_POINT('Ctrl Pts',(5.93878863840104,-3.24862210481691,4.53796391831861));
#9761=CARTESIAN_POINT('Ctrl Pts',(6.02067977404064,-3.0942240361053,4.54616166780219));
#9762=CARTESIAN_POINT('Ctrl Pts',(6.0964963675306,-2.9368386133198,4.55435941728578));
#9763=CARTESIAN_POINT('Ctrl Pts',(6.17229850081262,-2.77948320805207,4.56255560324406));
#9764=CARTESIAN_POINT('Ctrl Pts',(6.2420282385286,-2.61914190380967,4.57075178920234));
#9765=CARTESIAN_POINT('Ctrl Pts',(6.30545409585691,-2.45632604615946,4.57894797516063));
#9766=CARTESIAN_POINT('Ctrl Pts',(6.36887526122796,-2.29352223288794,4.58714355480225));
#9767=CARTESIAN_POINT('Ctrl Pts',(6.42599334384335,-2.1282445647956,4.59533913444387));
#9768=CARTESIAN_POINT('Ctrl Pts',(6.47662525903511,-1.96102377701762,4.60353471408549));
#9769=CARTESIAN_POINT('Ctrl Pts',(6.52726264058033,-1.79378493564775,4.61173117854324));
#9770=CARTESIAN_POINT('Ctrl Pts',(6.57141235555588,-1.62460290014048,4.61992764300099));
#9771=CARTESIAN_POINT('Ctrl Pts',(6.60894137641023,-1.45402299953366,4.62812410745874));
#9772=CARTESIAN_POINT('Ctrl Pts',(6.64648127698161,-1.28339364756873,4.6363229480833));
#9773=CARTESIAN_POINT('Ctrl Pts',(6.67739658325312,-1.11136597367322,4.64452178870787));
#9774=CARTESIAN_POINT('Ctrl Pts',(6.7016054944437,-0.938494963674312,4.65272062933243));
#9775=CARTESIAN_POINT('Ctrl Pts',(6.72583969259791,-0.765443384507747,4.66092803390203));
#9776=CARTESIAN_POINT('Ctrl Pts',(6.74335345068524,-0.591547065171197,4.66913543847162));
#9777=CARTESIAN_POINT('Ctrl Pts',(6.75411682876472,-0.417366581552912,4.67734284304122));
#9778=CARTESIAN_POINT('Ctrl Pts',(6.764885972297,-0.243092797360377,4.68555464394468));
#9779=CARTESIAN_POINT('Ctrl Pts',(6.76889751925103,-0.0685349038397829,
4.69376644484815));
#9780=CARTESIAN_POINT('Ctrl Pts',(6.7661736998704,0.105747166308009,4.70197824575162));
#9781=CARTESIAN_POINT('Ctrl Pts',(6.76344587064204,0.280285804335476,4.71020213558852));
#9782=CARTESIAN_POINT('Ctrl Pts',(6.75396287890137,0.454547449203377,4.71842602542543));
#9783=CARTESIAN_POINT('Ctrl Pts',(6.73779892515249,0.627976627123945,4.72664991526234));
#9784=CARTESIAN_POINT('Ctrl Pts',(6.7228637304116,0.788221984555494,4.73424863758919));
#9785=CARTESIAN_POINT('Ctrl Pts',(6.70222532253822,0.947756493134326,4.74184735991604));
#9786=CARTESIAN_POINT('Ctrl Pts',(6.67598072542722,1.10615114415903,4.7494460822429));
#9787=CARTESIAN_POINT('Ctrl Pts',(6.64757229195141,1.27760524907543,4.75767131034644));
#9788=CARTESIAN_POINT('Ctrl Pts',(6.61251475319008,1.44820490932618,4.76589653844998));
#9789=CARTESIAN_POINT('Ctrl Pts',(6.57086910197774,1.61739551275323,4.77412176655352));
#9790=CARTESIAN_POINT('Ctrl Pts',(6.52927076183557,1.78639390911235,4.78233765047987));
#9791=CARTESIAN_POINT('Ctrl Pts',(6.48109929797756,1.953986090966,4.79055353440623));
#9792=CARTESIAN_POINT('Ctrl Pts',(6.42646721677411,2.11962452140175,4.79876941833258));
#9793=CARTESIAN_POINT('Ctrl Pts',(6.37188622260497,2.28510806159735,4.80697761949938));
#9794=CARTESIAN_POINT('Ctrl Pts',(6.31085675483196,2.44864115035205,4.81518582066617));
#9795=CARTESIAN_POINT('Ctrl Pts',(6.24354194746007,2.60968828604232,4.82339402183297));
#9796=CARTESIAN_POINT('Ctrl Pts',(6.17627656594569,2.77061717296844,4.83159619613291));
#9797=CARTESIAN_POINT('Ctrl Pts',(6.10273517536377,2.92906341298115,4.83979837043286));
#9798=CARTESIAN_POINT('Ctrl Pts',(6.02313016636458,3.08450838854898,4.8480005447328));
#9799=CARTESIAN_POINT('Ctrl Pts',(5.94318809705292,3.24061154295122,4.85623744834774));
#9800=CARTESIAN_POINT('Ctrl Pts',(5.85713105593703,3.39368761115387,4.86447435196267));
#9801=CARTESIAN_POINT('Ctrl Pts',(5.76522269587831,3.54323246018796,4.87271125557761));
#9802=CARTESIAN_POINT('Ctrl Pts',(5.67377311696107,3.69203082265109,4.88090704284534));
#9803=CARTESIAN_POINT('Ctrl Pts',(5.57653070104813,3.83733283623083,4.88910283011308));
#9804=CARTESIAN_POINT('Ctrl Pts',(5.47380066331511,3.97866752799113,4.89729861738081));
#9805=CARTESIAN_POINT('Ctrl Pts',(5.37107953619944,4.11998996063635,4.90549369376081));
#9806=CARTESIAN_POINT('Ctrl Pts',(5.26287194613215,4.25734546662081,4.91368877014081));
#9807=CARTESIAN_POINT('Ctrl Pts',(5.14952554808702,4.39029334208992,4.92188384652081));
#9808=CARTESIAN_POINT('Ctrl Pts',(5.03616836004626,4.52325387351475,4.93007970303003));
#9809=CARTESIAN_POINT('Ctrl Pts',(4.91767162284475,4.65180566603528,4.93827555953926));
#9810=CARTESIAN_POINT('Ctrl Pts',(4.79442228751602,4.77554226543643,4.94647141604849));
#9811=CARTESIAN_POINT('Ctrl Pts',(4.67008954242387,4.90036655784238,4.95473931733539));
#9812=CARTESIAN_POINT('Ctrl Pts',(4.54092049909171,5.02029032542614,4.96300721862229));
#9813=CARTESIAN_POINT('Ctrl Pts',(4.40734890870411,5.1349356955024,4.97127511990918));
#9814=CARTESIAN_POINT('Ctrl Pts',(4.27479143544765,5.24871064220897,4.97948024871348));
#9815=CARTESIAN_POINT('Ctrl Pts',(4.1378983484203,5.35728687916309,4.98768537751777));
#9816=CARTESIAN_POINT('Ctrl Pts',(3.99712506123443,5.46033700835871,4.99589050632207));
#9817=CARTESIAN_POINT('Ctrl Pts',(3.85473631700978,5.56456969896128,5.00418979385027));
#9818=CARTESIAN_POINT('Ctrl Pts',(3.70837807988881,5.66314845353252,5.01248908137847));
#9819=CARTESIAN_POINT('Ctrl Pts',(3.55854948648691,5.75578096805497,5.02078836890666));
#9820=CARTESIAN_POINT('Ctrl Pts',(3.40872089308502,5.84841348257741,5.02908765643486));
#9821=CARTESIAN_POINT('Ctrl Pts',(3.25542229250714,5.93509961111655,5.03738694396306));
#9822=CARTESIAN_POINT('Ctrl Pts',(3.09917575053259,6.01559628526639,5.04568623149126));
#9823=CARTESIAN_POINT('Ctrl Pts',(3.09917575053259,6.01559628526639,3.04575158274221));
#9824=CARTESIAN_POINT('Ctrl Pts',(2.93382384459267,6.10078395293758,3.05450103065462));
#9825=CARTESIAN_POINT('Ctrl Pts',(2.76495772122989,6.17915010267047,3.06325047856702));
#9826=CARTESIAN_POINT('Ctrl Pts',(2.59315093316718,6.25042856433175,3.07199992647943));
#9827=CARTESIAN_POINT('Ctrl Pts',(2.42134553245621,6.3217064504145,3.08074930373944));
#9828=CARTESIAN_POINT('Ctrl Pts',(2.24659977927592,6.38589665313457,3.08949868099945));
#9829=CARTESIAN_POINT('Ctrl Pts',(2.06950718689917,6.44278115439076,3.09824805825945));
#9830=CARTESIAN_POINT('Ctrl Pts',(1.8924159657286,6.49966521519724,3.10699736777411));
#9831=CARTESIAN_POINT('Ctrl Pts',(1.71297821457198,6.54924360009546,3.11574667728876));
#9832=CARTESIAN_POINT('Ctrl Pts',(1.53180337335845,6.59134792173556,3.12449598680342));
#9833=CARTESIAN_POINT('Ctrl Pts',(1.3506298747778,6.63345193135305,3.13324523147954));
#9834=CARTESIAN_POINT('Ctrl Pts',(1.16771959102946,6.66808192368239,3.14199447615567));
#9835=CARTESIAN_POINT('Ctrl Pts',(0.983693746906757,6.6951202836317,3.15074372083179));
#9836=CARTESIAN_POINT('Ctrl Pts',(0.799669205419815,6.72215845218868,3.15949290357597));
#9837=CARTESIAN_POINT('Ctrl Pts',(0.614529402873452,6.74160505424579,3.16824208632015));
#9838=CARTESIAN_POINT('Ctrl Pts',(0.428903127363257,6.75339404354122,3.17699126906432));
#9839=CARTESIAN_POINT('Ctrl Pts',(0.243278104163808,6.76518295330331,3.18574039278293));
#9840=CARTESIAN_POINT('Ctrl Pts',(0.0571669005389651,6.76931433552276,3.19448951650154));
#9841=CARTESIAN_POINT('Ctrl Pts',(-0.128798404777745,6.76577415902472,3.20323864022016));
#9842=CARTESIAN_POINT('Ctrl Pts',(-0.314762517259277,6.7622340052344,3.21198770781936));
#9843=CARTESIAN_POINT('Ctrl Pts',(-0.500580446819634,6.75102239665088,3.22073677541857));
#9844=CARTESIAN_POINT('Ctrl Pts',(-0.685621118842681,6.73217741012497,3.22948584301777));
#9845=CARTESIAN_POINT('Ctrl Pts',(-0.870660665414701,6.71333253821769,3.23823485740356));
#9846=CARTESIAN_POINT('Ctrl Pts',(-1.05492267885522,6.68685441030607,3.24698387178934));
#9847=CARTESIAN_POINT('Ctrl Pts',(-1.23778137635301,6.65283295028168,3.25573288617513));
#9848=CARTESIAN_POINT('Ctrl Pts',(-1.42999922978895,6.61707018861855,3.26492969654252));
#9849=CARTESIAN_POINT('Ctrl Pts',(-1.62066601233743,6.57297172934401,3.27412650690992));
#9850=CARTESIAN_POINT('Ctrl Pts',(-1.80906628500433,6.52070304311281,3.28332331727731));
#9851=CARTESIAN_POINT('Ctrl Pts',(-1.98831342545571,6.47097374915017,3.29207331501507));
#9852=CARTESIAN_POINT('Ctrl Pts',(-2.16550875896742,6.41384933989515,3.30082331275283));
#9853=CARTESIAN_POINT('Ctrl Pts',(-2.34005036714047,6.34952386240462,3.30957331049059));
#9854=CARTESIAN_POINT('Ctrl Pts',(-2.51458843547124,6.28519968948582,3.31832313077146));
#9855=CARTESIAN_POINT('Ctrl Pts',(-2.6864726171809,6.21367483971084,3.32707295105232));
#9856=CARTESIAN_POINT('Ctrl Pts',(-2.85511905908764,6.13519226743828,3.33582277133319));
#9857=CARTESIAN_POINT('Ctrl Pts',(-3.02376230488918,6.0567111825292,3.34457242579172));
#9858=CARTESIAN_POINT('Ctrl Pts',(-3.18916767379939,5.97127275992615,3.35332208025025));
#9859=CARTESIAN_POINT('Ctrl Pts',(-3.35077334102822,5.87916720437977,3.36207173470879));
#9860=CARTESIAN_POINT('Ctrl Pts',(-3.51237616037398,5.78706327195624,3.37082123497723));
#9861=CARTESIAN_POINT('Ctrl Pts',(-3.67017916302325,5.68829258362281,3.37957073524567));
#9862=CARTESIAN_POINT('Ctrl Pts',(-3.82364636566484,5.58319061741027,3.38832023551411));
#9863=CARTESIAN_POINT('Ctrl Pts',(-3.9771110677882,5.47809036367686,3.39706959322255));
#9864=CARTESIAN_POINT('Ctrl Pts',(-4.12623987481949,5.36665920043208,3.40581895093099));
#9865=CARTESIAN_POINT('Ctrl Pts',(-4.27052628213952,5.24927559512316,3.41456830863943));
#9866=CARTESIAN_POINT('Ctrl Pts',(-4.41481053025008,5.13189374643011,3.42331753541595));
#9867=CARTESIAN_POINT('Ctrl Pts',(-4.55425230136567,5.0085598147732,3.43206676219247));
#9868=CARTESIAN_POINT('Ctrl Pts',(-4.68837800630591,4.87969268192035,3.44081598896899));
#9869=CARTESIAN_POINT('Ctrl Pts',(-4.82250188228962,4.75082730631742,3.44956509643985));
#9870=CARTESIAN_POINT('Ctrl Pts',(-4.95130963053056,4.61642907903431,3.45831420391071));
#9871=CARTESIAN_POINT('Ctrl Pts',(-5.07436379033477,4.47695444731565,3.46706331138157));
#9872=CARTESIAN_POINT('Ctrl Pts',(-5.19741643562917,4.33748153220453,3.47581231117132));
#9873=CARTESIAN_POINT('Ctrl Pts',(-5.31471544462885,4.19293255254448,3.48456131096107));
#9874=CARTESIAN_POINT('Ctrl Pts',(-5.42586245275739,4.04379841779453,3.49331031075082));
#9875=CARTESIAN_POINT('Ctrl Pts',(-5.53702160019253,3.89464799484199,3.50206026609297));
#9876=CARTESIAN_POINT('Ctrl Pts',(-5.64202723081342,3.74091164443713,3.51081022143512));
#9877=CARTESIAN_POINT('Ctrl Pts',(-5.74052265233048,3.58311159163103,3.51956017677727));
#9878=CARTESIAN_POINT('Ctrl Pts',(-5.83901427066995,3.42531763191653,3.52830979425972));
#9879=CARTESIAN_POINT('Ctrl Pts',(-5.93099603115812,3.26346052695481,3.53705941174217));
#9880=CARTESIAN_POINT('Ctrl Pts',(-6.01615550622822,3.09809004466944,3.54580902922461));
#9881=CARTESIAN_POINT('Ctrl Pts',(-6.10131214578869,2.93272506863683,3.55455835537571));
#9882=CARTESIAN_POINT('Ctrl Pts',(-6.17964682328819,2.76384720416736,3.56330768152681));
#9883=CARTESIAN_POINT('Ctrl Pts',(-6.25089348288635,2.59203002791423,3.57205700767791));
#9884=CARTESIAN_POINT('Ctrl Pts',(-6.32213814889406,2.42021765936833,3.58080608900949));
#9885=CARTESIAN_POINT('Ctrl Pts',(-6.38629508412663,2.24546640831697,3.58955517034107));
#9886=CARTESIAN_POINT('Ctrl Pts',(-6.44314639819891,2.06836976659795,3.59830425167265));
#9887=CARTESIAN_POINT('Ctrl Pts',(-6.50000285283774,1.89125711158024,3.60705412410705));
#9888=CARTESIAN_POINT('Ctrl Pts',(-6.54955227673317,1.71179891439998,3.61580399654145));
#9889=CARTESIAN_POINT('Ctrl Pts',(-6.59162635926446,1.53060476278169,3.62455386897585));
#9890=CARTESIAN_POINT('Ctrl Pts',(-6.63369752055247,1.34942319164445,3.63330313389834));
#9891=CARTESIAN_POINT('Ctrl Pts',(-6.66829431424295,1.16650618642466,3.64205239882084));
#9892=CARTESIAN_POINT('Ctrl Pts',(-6.6952992374545,0.982474997616297,3.65080166374333));
#9893=CARTESIAN_POINT('Ctrl Pts',(-6.72230554731469,0.798434359175536,3.65955137792303));
#9894=CARTESIAN_POINT('Ctrl Pts',(-6.74171916496722,0.613279706238185,3.66830109210272));
#9895=CARTESIAN_POINT('Ctrl Pts',(-6.75347414817288,0.427639953653287,3.67705080628242));
#9896=CARTESIAN_POINT('Ctrl Pts',(-6.76248837758749,0.285283364197234,3.68376046545829));
#9897=CARTESIAN_POINT('Ctrl Pts',(-6.76699999999996,0.142641701104535,3.69047012463415));
#9898=CARTESIAN_POINT('Ctrl Pts',(-6.767,1.74262956926013E-12,3.69717978381002));
#9899=CARTESIAN_POINT('',(-6.76699897167863,0.00373058981880235,3.30282021616294));
#9900=CARTESIAN_POINT('Ctrl Pts',(3.09917575053259,6.01559628526639,2.65160425626863));
#9901=CARTESIAN_POINT('Ctrl Pts',(2.94520675288169,6.09491959109098,2.65972997863448));
#9902=CARTESIAN_POINT('Ctrl Pts',(2.78810984876472,6.16836926240051,2.66785570100033));
#9903=CARTESIAN_POINT('Ctrl Pts',(2.62837909668337,6.23569661899277,2.67598142336617));
#9904=CARTESIAN_POINT('Ctrl Pts',(2.46866863440386,6.30301542332628,2.68410611356198));
#9905=CARTESIAN_POINT('Ctrl Pts',(2.30632532403241,6.36421331269895,2.69223080375779));
#9906=CARTESIAN_POINT('Ctrl Pts',(2.14186485538603,6.41908902736691,2.7003554939536));
#9907=CARTESIAN_POINT('Ctrl Pts',(1.97740802041331,6.47396352958277,2.70848000463836));
#9908=CARTESIAN_POINT('Ctrl Pts',(1.81083446692612,6.5225160187193,2.71660451532311));
#9909=CARTESIAN_POINT('Ctrl Pts',(1.64267658948007,6.56459462742172,2.72472902600786));
#9910=CARTESIAN_POINT('Ctrl Pts',(1.47449045949953,6.60668030583364,2.73285490170757));
#9911=CARTESIAN_POINT('Ctrl Pts',(1.30471983022654,6.6422898490823,2.74098077740728));
#9912=CARTESIAN_POINT('Ctrl Pts',(1.13390883005738,6.67132219017474,2.74910665310699));
#9913=CARTESIAN_POINT('Ctrl Pts',(0.963036657325268,6.70036492862281,2.75723543892749));
#9914=CARTESIAN_POINT('Ctrl Pts',(0.791123732014469,6.72282571346218,2.76536422474799));
#9915=CARTESIAN_POINT('Ctrl Pts',(0.618720828427367,6.7386551726936,2.77349301056849));
#9916=CARTESIAN_POINT('Ctrl Pts',(0.446129455341023,6.75450193656543,2.78163068271377));
#9917=CARTESIAN_POINT('Ctrl Pts',(0.273047398515536,6.7637028639598,2.78976835485904));
#9918=CARTESIAN_POINT('Ctrl Pts',(0.10002782907235,6.76626066844983,2.79790602700432));
#9919=CARTESIAN_POINT('Ctrl Pts',(-0.0730973733828469,6.76882003454697,
2.80604866741314));
#9920=CARTESIAN_POINT('Ctrl Pts',(-0.246159647961955,6.76472820531347,2.81419130782195));
#9921=CARTESIAN_POINT('Ctrl Pts',(-0.418609710536651,6.75403989551768,2.82233394823077));
#9922=CARTESIAN_POINT('Ctrl Pts',(-0.591303279505669,6.74333649340043,2.83048808637393));
#9923=CARTESIAN_POINT('Ctrl Pts',(-0.763382547419845,6.72601804475287,2.83864222451709));
#9924=CARTESIAN_POINT('Ctrl Pts',(-0.934306249721319,6.70219074868298,2.84679636266025));
#9925=CARTESIAN_POINT('Ctrl Pts',(-1.02815752174827,6.68910758926733,2.85127365999651));
#9926=CARTESIAN_POINT('Ctrl Pts',(-1.12166061344754,6.67406295807002,2.85575095733278));
#9927=CARTESIAN_POINT('Ctrl Pts',(-1.21472783458636,6.65708083831653,2.86022825466904));
#9928=CARTESIAN_POINT('Ctrl Pts',(-1.38571430848921,6.62588067202261,2.86845410771133));
#9929=CARTESIAN_POINT('Ctrl Pts',(-1.55573714104419,6.58804497094957,2.87667996075363));
#9930=CARTESIAN_POINT('Ctrl Pts',(-1.72424274715405,6.54364393506299,2.88490581379592));
#9931=CARTESIAN_POINT('Ctrl Pts',(-1.89255898443555,6.49929279764767,2.89312242251579));
#9932=CARTESIAN_POINT('Ctrl Pts',(-2.05936104686051,6.44839110797352,2.90133903123566));
#9933=CARTESIAN_POINT('Ctrl Pts',(-2.22410326461305,6.39106044943541,2.90955563995553));
#9934=CARTESIAN_POINT('Ctrl Pts',(-2.38869341676192,6.33378271006592,2.91776466431978));
#9935=CARTESIAN_POINT('Ctrl Pts',(-2.55122717421177,6.2700879372776,2.92597368868403));
#9936=CARTESIAN_POINT('Ctrl Pts',(-2.71117172540353,6.20014813334105,2.93418271304828));
#9937=CARTESIAN_POINT('Ctrl Pts',(-2.87100073986314,6.13025885076539,2.94238580758346));
#9938=CARTESIAN_POINT('Ctrl Pts',(-3.02824394613097,6.05413366553863,2.95058890211865));
#9939=CARTESIAN_POINT('Ctrl Pts',(-3.18238621523416,5.97199355132669,2.95879199665383));
#9940=CARTESIAN_POINT('Ctrl Pts',(-3.33644806769062,5.88989628994536,2.96699081160133));
#9941=CARTESIAN_POINT('Ctrl Pts',(-3.48741189008429,5.80179051932399,2.97518962654884));
#9942=CARTESIAN_POINT('Ctrl Pts',(-3.63478489442442,5.70794426840908,2.98338844149634));
#9943=CARTESIAN_POINT('Ctrl Pts',(-3.7821301124861,5.6141157116307,2.99158571060744));
#9944=CARTESIAN_POINT('Ctrl Pts',(-3.92588555548995,5.51454901765805,2.99978297971854));
#9945=CARTESIAN_POINT('Ctrl Pts',(-4.06558503985017,5.40955703211885,3.00798024882964));
#9946=CARTESIAN_POINT('Ctrl Pts',(-4.20527443122158,5.30457263202594,3.01617692570559));
#9947=CARTESIAN_POINT('Ctrl Pts',(-4.34090816025273,5.19416393579372,3.02437360258154));
#9948=CARTESIAN_POINT('Ctrl Pts',(-4.47205097788837,5.07868576023046,3.03257027945749));
#9949=CARTESIAN_POINT('Ctrl Pts',(-4.60320816200925,4.96319493421837,3.04076785426624));
#9950=CARTESIAN_POINT('Ctrl Pts',(-4.72987318530872,4.84263375956345,3.04896542907498));
#9951=CARTESIAN_POINT('Ctrl Pts',(-4.85164566609175,4.71739582086273,3.05716300388373));
#9952=CARTESIAN_POINT('Ctrl Pts',(-4.97345362471786,4.59212139467397,3.06536296701758));
#9953=CARTESIAN_POINT('Ctrl Pts',(-5.09036595156392,4.46216774752229,3.07356293015143));
#9954=CARTESIAN_POINT('Ctrl Pts',(-5.20202072554249,4.32796365176816,3.08176289328529));
#9955=CARTESIAN_POINT('Ctrl Pts',(-5.31379188115593,4.19361967044072,3.08997140352448));
#9956=CARTESIAN_POINT('Ctrl Pts',(-5.42029430570767,4.05501666538604,3.09817991376367));
#9957=CARTESIAN_POINT('Ctrl Pts',(-5.52120722161112,3.91261546999309,3.10638842400287));
#9958=CARTESIAN_POINT('Ctrl Pts',(-5.62217430664552,3.77013783493995,3.11460134049534));
#9959=CARTESIAN_POINT('Ctrl Pts',(-5.71754570592351,3.62385824527043,3.12281425698781));
#9960=CARTESIAN_POINT('Ctrl Pts',(-5.80704532664466,3.47426446522057,3.13102717348027));
#9961=CARTESIAN_POINT('Ctrl Pts',(-5.89667590943826,3.32445178914297,3.13925210768361));
#9962=CARTESIAN_POINT('Ctrl Pts',(-5.98041737103897,3.1713155458808,3.14747704188695));
#9963=CARTESIAN_POINT('Ctrl Pts',(-6.05804014883562,3.01536706805253,3.15570197609028));
#9964=CARTESIAN_POINT('Ctrl Pts',(-6.128284741187,2.8742417751448,3.1631451154191));
#9965=CARTESIAN_POINT('Ctrl Pts',(-6.19351909483421,2.73081390417555,3.17058825474792));
#9966=CARTESIAN_POINT('Ctrl Pts',(-6.25360800368249,2.58547402545033,3.17803139407673));
#9967=CARTESIAN_POINT('Ctrl Pts',(-6.32747811552127,2.40680090087797,3.18718159409184));
#9968=CARTESIAN_POINT('Ctrl Pts',(-6.39374764619014,2.22481332471955,3.19633179410695));
#9969=CARTESIAN_POINT('Ctrl Pts',(-6.45214081017707,2.04013920251721,3.20548199412205));
#9970=CARTESIAN_POINT('Ctrl Pts',(-6.510302139696,1.8561982796134,3.21459586571089));
#9971=CARTESIAN_POINT('Ctrl Pts',(-6.56064941685709,1.66959229364365,3.22370973729973));
#9972=CARTESIAN_POINT('Ctrl Pts',(-6.60295632276621,1.48096482052808,3.23282360888856));
#9973=CARTESIAN_POINT('Ctrl Pts',(-6.64515326820406,1.29282761171784,3.2419137924862));
#9974=CARTESIAN_POINT('Ctrl Pts',(-6.67935147609421,1.10267960418178,3.25100397608384));
#9975=CARTESIAN_POINT('Ctrl Pts',(-6.70537402831222,0.911179532494014,3.26009415968147));
#9976=CARTESIAN_POINT('Ctrl Pts',(-6.73128437064188,0.720505213848521,3.26914514618276));
#9977=CARTESIAN_POINT('Ctrl Pts',(-6.74908932618658,0.528490671122382,3.27819613268405));
#9978=CARTESIAN_POINT('Ctrl Pts',(-6.75866297586654,0.335803184396522,3.28724711918534));
#9979=CARTESIAN_POINT('Ctrl Pts',(-6.76415377236239,0.225290703548003,3.2924381515112));
#9980=CARTESIAN_POINT('Ctrl Pts',(-6.76693787391787,0.114557162636319,3.29762918383707));
#9981=CARTESIAN_POINT('Ctrl Pts',(-6.76699897167863,0.00373058981880468,
3.30282021616294));
#9982=CARTESIAN_POINT('Ctrl Pts',(-6.76699897167895,0.00373058924357801,
3.30282021618988));
#9983=CARTESIAN_POINT('Ctrl Pts',(-6.76709684169258,-0.173798009695901,
3.31113552065549));
#9984=CARTESIAN_POINT('Ctrl Pts',(-6.76020431043818,-0.351321971043665,
3.31945082512111));
#9985=CARTESIAN_POINT('Ctrl Pts',(-6.74634909808389,-0.528263993456603,
3.32776612958672));
#9986=CARTESIAN_POINT('Ctrl Pts',(-6.73249065934686,-0.705247219329472,
3.33608337038893));
#9987=CARTESIAN_POINT('Ctrl Pts',(-6.71166633374003,-0.88164789311043,3.34440061119115));
#9988=CARTESIAN_POINT('Ctrl Pts',(-6.68395576145156,-1.05689374061849,3.35271785199336));
#9989=CARTESIAN_POINT('Ctrl Pts',(-6.65623432495978,-1.23220829499037,3.3610383536519));
#9990=CARTESIAN_POINT('Ctrl Pts',(-6.62162131335795,-1.40636678086737,3.36935885531044));
#9991=CARTESIAN_POINT('Ctrl Pts',(-6.5802475750166,-1.57880678092292,3.37767935696899));
#9992=CARTESIAN_POINT('Ctrl Pts',(-6.53885102718628,-1.75134184776324,3.38600444574966));
#9993=CARTESIAN_POINT('Ctrl Pts',(-6.49068640260336,-1.92215620608231,3.39432953453034));
#9994=CARTESIAN_POINT('Ctrl Pts',(-6.4359345866935,-2.09070203419866,3.40265462331101));
#9995=CARTESIAN_POINT('Ctrl Pts',(-6.38110929144823,-2.25947405819964,3.41099088472552));
#9996=CARTESIAN_POINT('Ctrl Pts',(-6.31967924721766,-2.42597114142646,3.41932714614002));
#9997=CARTESIAN_POINT('Ctrl Pts',(-6.25187420606412,-2.58966366765071,3.42766340755453));
#9998=CARTESIAN_POINT('Ctrl Pts',(-6.18402023240115,-2.75347432500427,3.43600568495521));
#9999=CARTESIAN_POINT('Ctrl Pts',(-6.10978223002811,-2.91447607712649,3.44434796235589));
#10000=CARTESIAN_POINT('Ctrl Pts',(-6.02943630481958,-3.07216321931691,
3.45269023975658));
#10001=CARTESIAN_POINT('Ctrl Pts',(-5.94896154971195,-3.2301032034351,3.46104589350152));
#10002=CARTESIAN_POINT('Ctrl Pts',(-5.86235946643278,-3.38471765599889,
3.46940154724647));
#10003=CARTESIAN_POINT('Ctrl Pts',(-5.769950702733,-3.53552795039594,3.47775720099142));
#10004=CARTESIAN_POINT('Ctrl Pts',(-5.70330904118431,-3.64428655937289,
3.48378297848908));
#10005=CARTESIAN_POINT('Ctrl Pts',(-5.63364838875367,-3.75106733002901,
3.48980875598674));
#10006=CARTESIAN_POINT('Ctrl Pts',(-5.56110198131188,-3.85570146062284,
3.4958345334844));
#10007=CARTESIAN_POINT('Ctrl Pts',(-5.46294839384705,-3.99726898479401,
3.50398726908519));
#10008=CARTESIAN_POINT('Ctrl Pts',(-5.35923204261449,-4.13530739791128,
3.51214000468598));
#10009=CARTESIAN_POINT('Ctrl Pts',(-5.25023597555782,-4.2693455237259,3.52029274028678));
#10010=CARTESIAN_POINT('Ctrl Pts',(-5.14136615543722,-4.40322839712494,
3.5284360328139));
#10011=CARTESIAN_POINT('Ctrl Pts',(-5.02722902094046,-4.53311992577148,
3.53657932534103));
#10012=CARTESIAN_POINT('Ctrl Pts',(-4.90815148857804,-4.65857681756662,
3.54472261786816));
#10013=CARTESIAN_POINT('Ctrl Pts',(-4.78918684827596,-4.78391476931726,
3.55285819010539));
#10014=CARTESIAN_POINT('Ctrl Pts',(-4.66529138482328,-4.9048261910985,3.56099376234261));
#10015=CARTESIAN_POINT('Ctrl Pts',(-4.53683296001558,-5.02089988875662,
3.56912933457983));
#10016=CARTESIAN_POINT('Ctrl Pts',(-4.40846933145566,-5.13688792951043,
3.57725890314915));
#10017=CARTESIAN_POINT('Ctrl Pts',(-4.27554971641228,-5.24804511062683,
3.58538847171847));
#10018=CARTESIAN_POINT('Ctrl Pts',(-4.13847958908387,-5.35399623559227,
3.59351804028779));
#10019=CARTESIAN_POINT('Ctrl Pts',(-4.00148182471231,-5.45989142614784,
3.60164331704218));
#10020=CARTESIAN_POINT('Ctrl Pts',(-3.86033820042873,-5.560585811085,3.60976859379657));
#10021=CARTESIAN_POINT('Ctrl Pts',(-3.71548809435513,-5.65574373718482,
3.61789387055095));
#10022=CARTESIAN_POINT('Ctrl Pts',(-3.57009042878715,-5.75126137738712,
3.62604986231517));
#10023=CARTESIAN_POINT('Ctrl Pts',(-3.42095848583829,-5.84120037585115,
3.63420585407938));
#10024=CARTESIAN_POINT('Ctrl Pts',(-3.26856735302294,-5.92526425222982,
3.64236184584359));
#10025=CARTESIAN_POINT('Ctrl Pts',(-3.11678391566199,-6.00899290414622,
3.65048531367397));
#10026=CARTESIAN_POINT('Ctrl Pts',(-2.96176756699753,-6.08689304547798,
3.65860878150434));
#10027=CARTESIAN_POINT('Ctrl Pts',(-2.80401345750796,-6.15871719842,3.66673224933472));
#10028=CARTESIAN_POINT('Ctrl Pts',(-2.64623832554524,-6.23055092272172,
3.67485679970668));
#10029=CARTESIAN_POINT('Ctrl Pts',(-2.48572503902925,-6.29630689428214,
3.68298135007864));
#10030=CARTESIAN_POINT('Ctrl Pts',(-2.32298971280541,-6.35578537980951,
3.69110590045061));
#10031=CARTESIAN_POINT('Ctrl Pts',(-2.16020174222565,-6.4152831064361,3.69923307908855));
#10032=CARTESIAN_POINT('Ctrl Pts',(-1.99519064393342,-6.46849917765662,
3.70736025772649));
#10033=CARTESIAN_POINT('Ctrl Pts',(-1.82848866297087,-6.51528343277459,
3.71548743636443));
#10034=CARTESIAN_POINT('Ctrl Pts',(-1.66071991658294,-6.56236707141232,
3.72366662274174));
#10035=CARTESIAN_POINT('Ctrl Pts',(-1.49123893429748,-6.60293619267932,
3.73184580911904));
#10036=CARTESIAN_POINT('Ctrl Pts',(-1.32059876411721,-6.63688992708272,
3.74002499549634));
#10037=CARTESIAN_POINT('Ctrl Pts',(-1.15075111353853,-6.67068596708139,
3.74816619453736));
#10038=CARTESIAN_POINT('Ctrl Pts',(-0.979755390533758,-6.69792794448416,
3.75630739357837));
#10039=CARTESIAN_POINT('Ctrl Pts',(-0.808161859079969,-6.71856855360786,
3.76444859261939));
#10040=CARTESIAN_POINT('Ctrl Pts',(-0.635367328642229,-6.73935362826226,
3.77264677266483));
#10041=CARTESIAN_POINT('Ctrl Pts',(-0.46196696728385,-6.75344456246767,
3.78084495271028));
#10042=CARTESIAN_POINT('Ctrl Pts',(-0.288522019283917,-6.76084639999966,
3.78904313275573));
#10043=CARTESIAN_POINT('Ctrl Pts',(-0.115077071283985,-6.76824823753165,
3.79724131280118));
#10044=CARTESIAN_POINT('Ctrl Pts',(0.0584120919248692,-6.7689610416055,
3.80543949284662));
#10045=CARTESIAN_POINT('Ctrl Pts',(0.231390498827155,-6.76304276469198,
3.81363767289207));
#10046=CARTESIAN_POINT('Ctrl Pts',(0.405103527568918,-6.7570993534536,3.82187066978092));
#10047=CARTESIAN_POINT('Ctrl Pts',(0.578841395616977,-6.74445006384751,
3.83010366666977));
#10048=CARTESIAN_POINT('Ctrl Pts',(0.752046094964177,-6.72508109029543,
3.83833666355863));
#10049=CARTESIAN_POINT('Ctrl Pts',(0.925044525674072,-6.70573518316012,
3.84655985581137));
#10050=CARTESIAN_POINT('Ctrl Pts',(1.09751069954499,-6.67968556632619,3.85478304806411));
#10051=CARTESIAN_POINT('Ctrl Pts',(1.26888665828042,-6.64697041128046,3.86300624031686));
#10052=CARTESIAN_POINT('Ctrl Pts',(1.44009282883251,-6.61428766828823,3.87122128556413));
#10053=CARTESIAN_POINT('Ctrl Pts',(1.61021058589455,-6.57495260529816,3.8794363308114));
#10054=CARTESIAN_POINT('Ctrl Pts',(1.77868704744523,-6.52905516803546,3.88765137605867));
#10055=CARTESIAN_POINT('Ctrl Pts',(1.94703030351596,-6.4831940194632,3.89585992610159));
#10056=CARTESIAN_POINT('Ctrl Pts',(2.11373450476834,-6.43078092484251,3.90406847614452));
#10057=CARTESIAN_POINT('Ctrl Pts',(2.27825682815937,-6.37195690702199,3.91227702618745));
#10058=CARTESIAN_POINT('Ctrl Pts',(2.44268198274175,-6.31316763135447,3.9204807281647));
#10059=CARTESIAN_POINT('Ctrl Pts',(2.60492749024062,-6.24797509570972,3.92868443014195));
#10060=CARTESIAN_POINT('Ctrl Pts',(2.76446547667916,-6.17657021560098,3.93688813211921));
#10061=CARTESIAN_POINT('Ctrl Pts',(2.92395625777821,-6.10518646332317,3.94508940672135));
#10062=CARTESIAN_POINT('Ctrl Pts',(3.08074078552628,-6.02759417073968,3.9532906813235));
#10063=CARTESIAN_POINT('Ctrl Pts',(3.234310741282,-5.9440325561716,3.96149195592565));
#10064=CARTESIAN_POINT('Ctrl Pts',(3.38785951728152,-5.86048246608834,3.96969209944069));
#10065=CARTESIAN_POINT('Ctrl Pts',(3.53819428927971,-5.77096486415899,3.97789224295573));
#10066=CARTESIAN_POINT('Ctrl Pts',(3.68483093413852,-5.675765145495,3.98609238647077));
#10067=CARTESIAN_POINT('Ctrl Pts',(3.83147393003582,-5.58056130359784,3.99429288514552));
#10068=CARTESIAN_POINT('Ctrl Pts',(3.9744181791317,-5.47967504973398,4.00249338382026));
#10069=CARTESIAN_POINT('Ctrl Pts',(4.11320812387964,-5.37343539364255,4.01069388249501));
#10070=CARTESIAN_POINT('Ctrl Pts',(4.25202923225124,-5.26717188270585,4.01889622249374));
#10071=CARTESIAN_POINT('Ctrl Pts',(4.38669389395538,-5.15555279314839,4.02709856249247));
#10072=CARTESIAN_POINT('Ctrl Pts',(4.51677920984576,-5.03894776411753,4.0353009024912));
#10073=CARTESIAN_POINT('Ctrl Pts',(4.64698618487179,-4.92223368306227,4.04351091352941));
#10074=CARTESIAN_POINT('Ctrl Pts',(4.77260499042225,-4.80052458574869,4.05172092456763));
#10075=CARTESIAN_POINT('Ctrl Pts',(4.89324855634459,-4.67422801816852,4.05993093560584));
#10076=CARTESIAN_POINT('Ctrl Pts',(5.01394986229968,-4.54787100502797,4.06814487595685));
#10077=CARTESIAN_POINT('Ctrl Pts',(5.12967094387691,-4.41692241235564,4.07635881630785));
#10078=CARTESIAN_POINT('Ctrl Pts',(5.24006477789551,-4.28182322421874,4.08457275665885));
#10079=CARTESIAN_POINT('Ctrl Pts',(5.35060912579644,-4.1465398382642,4.09279789611407));
#10080=CARTESIAN_POINT('Ctrl Pts',(5.45581149447148,-4.00709483329603,4.10102303556928));
#10081=CARTESIAN_POINT('Ctrl Pts',(5.55536728286152,-3.86395954333269,4.1092481750245));
#10082=CARTESIAN_POINT('Ctrl Pts',(5.64490600790569,-3.7352261810702,4.11664572078291));
#10083=CARTESIAN_POINT('Ctrl Pts',(5.72987777030852,-3.60350832328702,4.12404326654133));
#10084=CARTESIAN_POINT('Ctrl Pts',(5.81009297579069,-3.46916540578101,4.13144081229974));
#10085=CARTESIAN_POINT('Ctrl Pts',(5.90384440396677,-3.31215227708771,4.14008668530699));
#10086=CARTESIAN_POINT('Ctrl Pts',(5.99131091009206,-3.15119672324539,4.14873255831424));
#10087=CARTESIAN_POINT('Ctrl Pts',(6.07216684534548,-2.98681750401446,4.15737843132149));
#10088=CARTESIAN_POINT('Ctrl Pts',(6.15291935100299,-2.82264855600438,4.16601324466876));
#10089=CARTESIAN_POINT('Ctrl Pts',(6.22707801385425,-2.65506494791864,4.17464805801603));
#10090=CARTESIAN_POINT('Ctrl Pts',(6.29436207283328,-2.48461165900789,4.1832828713633));
#10091=CARTESIAN_POINT('Ctrl Pts',(6.36388102804483,-2.30849662169808,4.19220449724999));
#10092=CARTESIAN_POINT('Ctrl Pts',(6.42606064646887,-2.12931824850697,4.20112612313668));
#10093=CARTESIAN_POINT('Ctrl Pts',(6.48064306107319,-1.9477049352928,4.21004774902337));
#10094=CARTESIAN_POINT('Ctrl Pts',(6.53332486058637,-1.77241558202708,4.21865871483903));
#10095=CARTESIAN_POINT('Ctrl Pts',(6.5789294816883,-1.59485832255998,4.2272696806547));
#10096=CARTESIAN_POINT('Ctrl Pts',(6.61727384809151,-1.41561852889973,4.23588064647036));
#10097=CARTESIAN_POINT('Ctrl Pts',(6.65558205665078,-1.23654775418788,4.24448349234593));
#10098=CARTESIAN_POINT('Ctrl Pts',(6.68664359655048,-1.05579790576891,4.2530863382215));
#10099=CARTESIAN_POINT('Ctrl Pts',(6.71032549532368,-0.87396839005139,4.26168918409707));
#10100=CARTESIAN_POINT('Ctrl Pts',(6.73398087924588,-0.692342455244416,
4.27028239800948));
#10101=CARTESIAN_POINT('Ctrl Pts',(6.75027306605747,-0.509639566479221,
4.27887561192189));
#10102=CARTESIAN_POINT('Ctrl Pts',(6.75912031192382,-0.326468388881435,
4.2874688258343));
#10103=CARTESIAN_POINT('Ctrl Pts',(6.76010647993188,-0.306051011759411,
4.28842667789073));
#10104=CARTESIAN_POINT('Ctrl Pts',(6.76100019942572,-0.28562782510727,4.28938452994716));
#10105=CARTESIAN_POINT('Ctrl Pts',(6.76180139687412,-0.26519967803756,4.29034238200358));
#10106=CARTESIAN_POINT('Ctrl Pts',(6.76899140555886,-0.0818758854607504,
4.29893822141634));
#10107=CARTESIAN_POINT('Ctrl Pts',(6.76871754992939,0.101632850524437,4.3075340608291));
#10108=CARTESIAN_POINT('Ctrl Pts',(6.76100790797412,0.284712255288441,4.31612990024186));
#10109=CARTESIAN_POINT('Ctrl Pts',(6.75329107009757,0.467962540229786,4.32473376272289));
#10110=CARTESIAN_POINT('Ctrl Pts',(6.73812460561502,0.650782389070587,4.33333762520391));
#10111=CARTESIAN_POINT('Ctrl Pts',(6.71558847263786,0.832562589943548,4.34194148768494));
#10112=CARTESIAN_POINT('Ctrl Pts',(6.69216698990923,1.02148416932313,4.35088335968682));
#10113=CARTESIAN_POINT('Ctrl Pts',(6.66078514618406,1.20928239056665,4.35982523168869));
#10114=CARTESIAN_POINT('Ctrl Pts',(6.62159082338148,1.39528633896783,4.36876710369056));
#10115=CARTESIAN_POINT('Ctrl Pts',(6.58377537545608,1.57474658018979,4.37739439639174));
#10116=CARTESIAN_POINT('Ctrl Pts',(6.53868789761558,1.75253636908757,4.38602168909292));
#10117=CARTESIAN_POINT('Ctrl Pts',(6.48651197892727,1.92806933154205,4.3946489817941));
#10118=CARTESIAN_POINT('Ctrl Pts',(6.43428636139952,2.10376949343908,4.40328449220271));
#10119=CARTESIAN_POINT('Ctrl Pts',(6.37495892132687,2.27720824858467,4.41192000261132));
#10120=CARTESIAN_POINT('Ctrl Pts',(6.30876192969389,2.44781778620163,4.42055551301993));
#10121=CARTESIAN_POINT('Ctrl Pts',(6.24246713047884,2.61867940334578,4.42920378259436));
#10122=CARTESIAN_POINT('Ctrl Pts',(6.16928261451574,2.78670316820374,4.43785205216879));
#10123=CARTESIAN_POINT('Ctrl Pts',(6.08948787542499,2.9513431544048,4.44650032174322));
#10124=CARTESIAN_POINT('Ctrl Pts',(6.0810496849766,2.96875361999207,4.44741486506461));
#10125=CARTESIAN_POINT('Ctrl Pts',(6.07253761502701,2.98612627013083,4.44832940838601));
#10126=CARTESIAN_POINT('Ctrl Pts',(6.06395202511095,3.00346047704191,4.44924395170741));
#10127=CARTESIAN_POINT('Ctrl Pts',(5.98492975694224,3.16300552408128,4.45766146154679));
#10128=CARTESIAN_POINT('Ctrl Pts',(5.89950056531221,3.31964412149655,4.46607897138617));
#10129=CARTESIAN_POINT('Ctrl Pts',(5.80790468167551,3.47282769635519,4.47449648122555));
#10130=CARTESIAN_POINT('Ctrl Pts',(5.71849559537438,3.62235410431883,4.48271302801552));
#10131=CARTESIAN_POINT('Ctrl Pts',(5.62321108275568,3.76858823202246,4.49092957480549));
#10132=CARTESIAN_POINT('Ctrl Pts',(5.52232284465145,3.91104070541854,4.49914612159546));
#10133=CARTESIAN_POINT('Ctrl Pts',(5.42151524506533,4.05337931860087,4.50735610101772));
#10134=CARTESIAN_POINT('Ctrl Pts',(5.31511304438239,4.19194200544041,4.51556608043998));
#10135=CARTESIAN_POINT('Ctrl Pts',(5.20343264862878,4.32626601946576,4.52377605986224));
#10136=CARTESIAN_POINT('Ctrl Pts',(5.09182127392538,4.46050701816461,4.53198096532862));
#10137=CARTESIAN_POINT('Ctrl Pts',(4.97493842906929,4.59051428673738,4.54018587079499));
#10138=CARTESIAN_POINT('Ctrl Pts',(4.85314245757157,4.7158559442074,4.54839077626136));
#10139=CARTESIAN_POINT('Ctrl Pts',(4.72588558709957,4.84681747662315,4.55696356056062));
#10140=CARTESIAN_POINT('Ctrl Pts',(4.59326508132317,4.9726850335613,4.56553634485988));
#10141=CARTESIAN_POINT('Ctrl Pts',(4.45573544088481,5.09300605544929,4.57410912915914));
#10142=CARTESIAN_POINT('Ctrl Pts',(4.32418742979502,5.20809390902911,4.58230905406606));
#10143=CARTESIAN_POINT('Ctrl Pts',(4.1881485802155,5.31810724398039,4.59050897897297));
#10144=CARTESIAN_POINT('Ctrl Pts',(4.0480528287496,5.42268912032142,4.59870890387989));
#10145=CARTESIAN_POINT('Ctrl Pts',(3.90796767698092,5.52726308395839,4.6069082083774));
#10146=CARTESIAN_POINT('Ctrl Pts',(3.76382652423189,5.62640619670433,4.61510751287492));
#10147=CARTESIAN_POINT('Ctrl Pts',(3.61609443087256,5.71980332415481,4.62330681737243));
#10148=CARTESIAN_POINT('Ctrl Pts',(3.46832615795948,5.81322332453911,4.63150812987763));
#10149=CARTESIAN_POINT('Ctrl Pts',(3.31696549318485,5.90089434166774,4.63970944238282));
#10150=CARTESIAN_POINT('Ctrl Pts',(3.16250461406014,5.98254574291315,4.64791075488801));
#10151=CARTESIAN_POINT('Ctrl Pts',(3.14145212181365,5.99367455107077,4.64902856587618));
#10152=CARTESIAN_POINT('Ctrl Pts',(3.12034207408623,6.00469160457064,4.65014637686434));
#10153=CARTESIAN_POINT('Ctrl Pts',(3.09917575053259,6.01559628526639,4.6512641878525));
#10154=CARTESIAN_POINT('Origin',(0.,0.,-3.69717978381041));
#10155=CARTESIAN_POINT('',(3.09917575053257,6.0155962852664,7.04594397030302));
#10156=CARTESIAN_POINT('',(3.0991757505326,6.01559628526638,6.65133473543275));
#10157=CARTESIAN_POINT('',(3.09917575053259,6.01559628526639,-3.69717978381041));
#10158=CARTESIAN_POINT('',(-6.76699981083753,-0.00160003901735913,5.69717978376657));
#10159=CARTESIAN_POINT('Ctrl Pts',(-6.76699981083731,-0.00160003993641796,
5.69717978381002));
#10160=CARTESIAN_POINT('Ctrl Pts',(-6.76698820601404,-0.0506799629623293,
5.69950000820113));
#10161=CARTESIAN_POINT('Ctrl Pts',(-6.76644265511029,-0.0997553428157312,
5.70182023259224));
#10162=CARTESIAN_POINT('Ctrl Pts',(-6.76536341443635,-0.148818246885836,
5.70414045698336));
#10163=CARTESIAN_POINT('Ctrl Pts',(-6.76134190307601,-0.331638474897428,
5.71278617333996));
#10164=CARTESIAN_POINT('Ctrl Pts',(-6.74990195841384,-0.514459101048899,
5.72143188969656));
#10165=CARTESIAN_POINT('Ctrl Pts',(-6.73104324404487,-0.69666767313971,
5.73007760605316));
#10166=CARTESIAN_POINT('Ctrl Pts',(-6.71220874041747,-0.878642326599372,
5.73871222307391));
#10167=CARTESIAN_POINT('Ctrl Pts',(-6.68597449005211,-1.06000619092076,
5.74734684009467));
#10168=CARTESIAN_POINT('Ctrl Pts',(-6.6523921143403,-1.24014844154358,5.75598145711543));
#10169=CARTESIAN_POINT('Ctrl Pts',(-6.61762372947053,-1.42665267086645,
5.76492101786471));
#10170=CARTESIAN_POINT('Ctrl Pts',(-6.57497870581106,-1.61184710402766,
5.77386057861398));
#10171=CARTESIAN_POINT('Ctrl Pts',(-6.52457313922218,-1.79505831407797,
5.78280013936326));
#10172=CARTESIAN_POINT('Ctrl Pts',(-6.47602212139883,-1.97152871857001,
5.79141079097663));
#10173=CARTESIAN_POINT('Ctrl Pts',(-6.42027148215713,-2.14615888479742,
5.80002144258999));
#10174=CARTESIAN_POINT('Ctrl Pts',(-6.35747716681006,-2.31835568312732,
5.80863209420336));
#10175=CARTESIAN_POINT('Ctrl Pts',(-6.29474229034639,-2.49038948604338,
5.81723459527771));
#10176=CARTESIAN_POINT('Ctrl Pts',(-6.22497713471703,-2.65999422771345,
5.82583709635205));
#10177=CARTESIAN_POINT('Ctrl Pts',(-6.14838754772299,-2.8265915097525,5.8344395974264));
#10178=CARTESIAN_POINT('Ctrl Pts',(-6.07188416047097,-2.99300129054892,
5.84303241659225));
#10179=CARTESIAN_POINT('Ctrl Pts',(-5.98857179181415,-3.156410087815,5.8516252357581));
#10180=CARTESIAN_POINT('Ctrl Pts',(-5.89870460580497,-3.31625888215248,
5.86021805492395));
#10181=CARTESIAN_POINT('Ctrl Pts',(-5.88811326999088,-3.33509793048024,
5.86123076531822));
#10182=CARTESIAN_POINT('Ctrl Pts',(-5.87743094336133,-3.3538875535566,5.86224347571249));
#10183=CARTESIAN_POINT('Ctrl Pts',(-5.86665808582902,-3.37262685513488,
5.86325618610676));
#10184=CARTESIAN_POINT('Ctrl Pts',(-5.77522474126469,-3.5316744442229,5.8718514448991));
#10185=CARTESIAN_POINT('Ctrl Pts',(-5.677373755905,-3.68690796342183,5.88044670369145));
#10186=CARTESIAN_POINT('Ctrl Pts',(-5.57345574042497,-3.83782231343818,
5.88904196248379));
#10187=CARTESIAN_POINT('Ctrl Pts',(-5.46944040975675,-3.98887798888597,
5.89764527040239));
#10188=CARTESIAN_POINT('Ctrl Pts',(-5.35934688157355,-4.13560617021424,
5.90624857832099));
#10189=CARTESIAN_POINT('Ctrl Pts',(-5.24356699655792,-4.27753365300714,
5.91485188623959));
#10190=CARTESIAN_POINT('Ctrl Pts',(-5.12298685932865,-4.42534547152348,
5.92381188865547));
#10191=CARTESIAN_POINT('Ctrl Pts',(-4.99623905480765,-4.56794974683564,
5.93277189107135));
#10192=CARTESIAN_POINT('Ctrl Pts',(-4.86380883061562,-4.70485415918767,
5.94173189348723));
#10193=CARTESIAN_POINT('Ctrl Pts',(-4.73630273460883,-4.83666808045537,
5.95035873781398));
#10194=CARTESIAN_POINT('Ctrl Pts',(-4.60352942197209,-4.9631981987936,5.95898558214072));
#10195=CARTESIAN_POINT('Ctrl Pts',(-4.46595639412251,-5.08404587762505,
5.96761242646746));
#10196=CARTESIAN_POINT('Ctrl Pts',(-4.32825188099425,-5.20500905650021,
5.97624751589172));
#10197=CARTESIAN_POINT('Ctrl Pts',(-4.18573873102094,-5.32027876107326,
5.98488260531599));
#10198=CARTESIAN_POINT('Ctrl Pts',(-4.03891577337752,-5.42949798559336,
5.99351769474025));
#10199=CARTESIAN_POINT('Ctrl Pts',(-3.89187475396772,-5.53887942273608,
6.00216560901754));
#10200=CARTESIAN_POINT('Ctrl Pts',(-3.74051138500744,-5.64219224681083,
6.01081352329483));
#10201=CARTESIAN_POINT('Ctrl Pts',(-3.58535282606466,-5.73912311356275,
6.01946143757212));
#10202=CARTESIAN_POINT('Ctrl Pts',(-3.56794648950848,-5.74999722389777,
6.02043159679147));
#10203=CARTESIAN_POINT('Ctrl Pts',(-3.55049241386118,-5.7607910635445,6.02140175601082));
#10204=CARTESIAN_POINT('Ctrl Pts',(-3.53299136149909,-5.77150422676557,
6.02237191523017));
#10205=CARTESIAN_POINT('Ctrl Pts',(-3.38462340153565,-5.86232677497461,
6.03059659459439));
#10206=CARTESIAN_POINT('Ctrl Pts',(-3.23255550819682,-5.94754419851678,
6.03882127395862));
#10207=CARTESIAN_POINT('Ctrl Pts',(-3.07724947677291,-6.02684201366693,
6.04704595332284));
#10208=CARTESIAN_POINT('Ctrl Pts',(-2.92210668960703,-6.10605647781726,
6.05526198761599));
#10209=CARTESIAN_POINT('Ctrl Pts',(-2.7637328588157,-6.17936356249282,6.06347802190914));
#10210=CARTESIAN_POINT('Ctrl Pts',(-2.60261784015299,-6.24649256608198,
6.07169405620228));
#10211=CARTESIAN_POINT('Ctrl Pts',(-2.44163990002671,-6.31356445553218,
6.07990310019766));
#10212=CARTESIAN_POINT('Ctrl Pts',(-2.27792574593822,-6.37446859553087,
6.08811214419304));
#10213=CARTESIAN_POINT('Ctrl Pts',(-2.11198895129626,-6.42898060889925,
6.09632118818841));
#10214=CARTESIAN_POINT('Ctrl Pts',(-1.94616010956576,-6.48345715858059,
6.10452489165518));
#10215=CARTESIAN_POINT('Ctrl Pts',(-1.77811184683441,-6.53154975353674,
6.11272859512194));
#10216=CARTESIAN_POINT('Ctrl Pts',(-1.60837688150384,-6.57308244334757,
6.12093229858871));
#10217=CARTESIAN_POINT('Ctrl Pts',(-1.43871835834537,-6.6145964284147,6.12913230741948));
#10218=CARTESIAN_POINT('Ctrl Pts',(-1.26737499339819,-6.64955630916641,
6.13733231625025));
#10219=CARTESIAN_POINT('Ctrl Pts',(-1.09489389232812,-6.67783620378207,
6.14553232508102));
#10220=CARTESIAN_POINT('Ctrl Pts',(-0.922426583258931,-6.70611383706981,
6.15373167821949));
#10221=CARTESIAN_POINT('Ctrl Pts',(-0.748822071284916,-6.72771248159113,
6.16193103135797));
#10222=CARTESIAN_POINT('Ctrl Pts',(-0.574637238014458,-6.74255745579429,
6.17013038449645));
#10223=CARTESIAN_POINT('Ctrl Pts',(-0.400453540407016,-6.75740233321009,
6.17832968417618));
#10224=CARTESIAN_POINT('Ctrl Pts',(-0.225689886167997,-6.76549359648846,
6.18652898385591));
#10225=CARTESIAN_POINT('Ctrl Pts',(-0.0509077364817006,-6.76680850936143,
6.19472828353565));
#10226=CARTESIAN_POINT('Ctrl Pts',(0.12390498084826,-6.76812365219948,6.2029290171906));
#10227=CARTESIAN_POINT('Ctrl Pts',(0.298735841557815,-6.76266008079018,
6.21112975084555));
#10228=CARTESIAN_POINT('Ctrl Pts',(0.473023870177445,-6.7504472013521,6.2193304845005));
#10229=CARTESIAN_POINT('Ctrl Pts',(0.647373997929306,-6.73822997044351,
6.22753414009133));
#10230=CARTESIAN_POINT('Ctrl Pts',(0.821180550889936,-6.71925866608624,
6.23573779568215));
#10231=CARTESIAN_POINT('Ctrl Pts',(0.993888098807123,-6.69361452782049,
6.24394145127298));
#10232=CARTESIAN_POINT('Ctrl Pts',(1.16679349431086,-6.66794101254762,6.25215450467808));
#10233=CARTESIAN_POINT('Ctrl Pts',(1.33859701452745,-6.6355794442417,6.26036755808319));
#10234=CARTESIAN_POINT('Ctrl Pts',(1.50875278765621,-6.59666233983062,6.26858061148829));
#10235=CARTESIAN_POINT('Ctrl Pts',(1.67900924576156,-6.55772220729846,6.27679852474078));
#10236=CARTESIAN_POINT('Ctrl Pts',(1.84761566766184,-6.51221889950933,6.28501643799327));
#10237=CARTESIAN_POINT('Ctrl Pts',(2.01404186673779,-6.46033469404081,6.29323435124576));
#10238=CARTESIAN_POINT('Ctrl Pts',(2.1807276345616,-6.4083695667083,6.30146508167166));
#10239=CARTESIAN_POINT('Ctrl Pts',(2.34522604641402,-6.35000377306232,6.30969581209757));
#10240=CARTESIAN_POINT('Ctrl Pts',(2.50702614051678,-6.28546807570968,6.31792654252347));
#10241=CARTESIAN_POINT('Ctrl Pts',(2.65562021793037,-6.22619973930026,6.32548548617464));
#10242=CARTESIAN_POINT('Ctrl Pts',(2.80193853728015,-6.16172820601175,6.33304442982581));
#10243=CARTESIAN_POINT('Ctrl Pts',(2.94560484711739,-6.09226567745027,6.34060337347697));
#10244=CARTESIAN_POINT('Ctrl Pts',(3.10057882950525,-6.01733589961927,6.34875726565667));
#10245=CARTESIAN_POINT('Ctrl Pts',(3.25294572789472,-5.93636621911992,6.35691115783636));
#10246=CARTESIAN_POINT('Ctrl Pts',(3.40219555097585,-5.84956019140928,6.36506505001605));
#10247=CARTESIAN_POINT('Ctrl Pts',(3.55126324757393,-5.76286009130517,6.37320899216917));
#10248=CARTESIAN_POINT('Ctrl Pts',(3.69722112764911,-5.67033800227159,6.38135293432229));
#10249=CARTESIAN_POINT('Ctrl Pts',(3.83957962510095,-5.57224526582505,6.3894968764754));
#10250=CARTESIAN_POINT('Ctrl Pts',(3.98179436903647,-5.47425158335871,6.39763259488114));
#10251=CARTESIAN_POINT('Ctrl Pts',(4.12041666740123,-5.37069865812758,6.40576831328687));
#10252=CARTESIAN_POINT('Ctrl Pts',(4.25498201289986,-5.26188341470035,6.4139040316926));
#10253=CARTESIAN_POINT('Ctrl Pts',(4.38943978025423,-5.15315516352148,6.42203324600558));
#10254=CARTESIAN_POINT('Ctrl Pts',(4.5198467695529,-5.03917319947558,6.43016246031856));
#10255=CARTESIAN_POINT('Ctrl Pts',(4.64576792213785,-4.92027737161585,6.43829167463154));
#10256=CARTESIAN_POINT('Ctrl Pts',(4.77161488365571,-4.80145159559538,6.44641609931964));
#10257=CARTESIAN_POINT('Ctrl Pts',(4.89298100668191,-4.677717971802,6.45454052400775));
#10258=CARTESIAN_POINT('Ctrl Pts',(5.00946478225142,-4.54945618677471,6.46266494869586));
#10259=CARTESIAN_POINT('Ctrl Pts',(5.12665568860967,-4.42041577093153,6.47083869382202));
#10260=CARTESIAN_POINT('Ctrl Pts',(5.23890448375643,-4.28679227231257,6.47901243894818));
#10261=CARTESIAN_POINT('Ctrl Pts',(5.34584001264921,-4.14900994927208,6.48718618407435));
#10262=CARTESIAN_POINT('Ctrl Pts',(5.45209075797299,-4.01210994356703,6.4953075869489));
#10263=CARTESIAN_POINT('Ctrl Pts',(5.55309587850924,-3.87110452812187,6.50342898982345));
#10264=CARTESIAN_POINT('Ctrl Pts',(5.64853201215003,-3.726442688103,6.511550392698));
#10265=CARTESIAN_POINT('Ctrl Pts',(5.74397552440886,-3.58176966359435,6.51967242347655));
#10266=CARTESIAN_POINT('Ctrl Pts',(5.83384899054407,-3.43343995688232,6.5277944542551));
#10267=CARTESIAN_POINT('Ctrl Pts',(5.91787278782245,-3.28193093576793,6.53591648503365));
#10268=CARTESIAN_POINT('Ctrl Pts',(6.00191908144825,-3.13038134996012,6.54404069038692));
#10269=CARTESIAN_POINT('Ctrl Pts',(6.08011241025209,-2.97565107474226,6.5521648957402));
#10270=CARTESIAN_POINT('Ctrl Pts',(6.15221947768191,-2.81824138398956,6.56028910109348));
#10271=CARTESIAN_POINT('Ctrl Pts',(6.22510705390718,-2.65912784294172,6.56850124531267));
#10272=CARTESIAN_POINT('Ctrl Pts',(6.29177567936625,-2.49727689032067,6.57671338953187));
#10273=CARTESIAN_POINT('Ctrl Pts',(6.35203496101377,-2.33322541861237,6.58492553375106));
#10274=CARTESIAN_POINT('Ctrl Pts',(6.41174414208941,-2.17067155533774,6.59306271017927));
#10275=CARTESIAN_POINT('Ctrl Pts',(6.46516046002134,-2.00595754963186,6.60119988660748));
#10276=CARTESIAN_POINT('Ctrl Pts',(6.51214947318962,-1.83961904720411,6.60933706303569));
#10277=CARTESIAN_POINT('Ctrl Pts',(6.55978785089153,-1.67098183031588,6.61758669115038));
#10278=CARTESIAN_POINT('Ctrl Pts',(6.60081988677828,-1.50067526997758,6.62583631926506));
#10279=CARTESIAN_POINT('Ctrl Pts',(6.63515950442006,-1.32926571869741,6.63408594737974));
#10280=CARTESIAN_POINT('Ctrl Pts',(6.66949912206185,-1.15785616741723,6.64233557549442));
#10281=CARTESIAN_POINT('Ctrl Pts',(6.69714632303405,-0.985344015134451,
6.65058520360911));
#10282=CARTESIAN_POINT('Ctrl Pts',(6.71806973041192,-0.812298034789663,
6.65883483172379));
#10283=CARTESIAN_POINT('Ctrl Pts',(6.73893033832974,-0.639771434196579,
6.66705969942628));
#10284=CARTESIAN_POINT('Ctrl Pts',(6.7531699834837,-0.466198525443087,6.67528456712877));
#10285=CARTESIAN_POINT('Ctrl Pts',(6.76069152120858,-0.292128661822798,
6.68350943483126));
#10286=CARTESIAN_POINT('Ctrl Pts',(6.76820458507971,-0.118254907378856,
6.69172503630008));
#10287=CARTESIAN_POINT('Ctrl Pts',(6.76901459738444,0.0561143319093995,
6.69994063776891));
#10288=CARTESIAN_POINT('Ctrl Pts',(6.76307583088638,0.230422016483844,6.70815623923773));
#10289=CARTESIAN_POINT('Ctrl Pts',(6.75714256185588,0.404568345860861,6.71636423559149));
#10290=CARTESIAN_POINT('Ctrl Pts',(6.74447296776536,0.578652877699234,6.72457223194525));
#10291=CARTESIAN_POINT('Ctrl Pts',(6.72507328449049,0.752115894149552,6.73278022829902));
#10292=CARTESIAN_POINT('Ctrl Pts',(6.70568766281652,0.925453178252891,6.74098227519642));
#10293=CARTESIAN_POINT('Ctrl Pts',(6.67958170815466,1.09816948917078,6.74918432209383));
#10294=CARTESIAN_POINT('Ctrl Pts',(6.64681366850358,1.2697074687478,6.75738636899124));
#10295=CARTESIAN_POINT('Ctrl Pts',(6.61406280021216,1.44115555767607,6.76558411778908));
#10296=CARTESIAN_POINT('Ctrl Pts',(6.57465686895185,1.61142619381439,6.77378186658691));
#10297=CARTESIAN_POINT('Ctrl Pts',(6.52870568679892,1.77996939725364,6.78197961538475));
#10298=CARTESIAN_POINT('Ctrl Pts',(6.48276326890898,1.94848045446964,6.79017580062702));
#10299=CARTESIAN_POINT('Ctrl Pts',(6.43027817500591,2.1152643878326,6.7983719858693));
#10300=CARTESIAN_POINT('Ctrl Pts',(6.37141090777295,2.27978333275597,6.80656817111157));
#10301=CARTESIAN_POINT('Ctrl Pts',(6.31254799540589,2.44429010694374,6.81476375001879));
#10302=CARTESIAN_POINT('Ctrl Pts',(6.2473039700302,2.60653188824039,6.82295932892601));
#10303=CARTESIAN_POINT('Ctrl Pts',(6.1758885915632,2.76598790752952,6.83115490783323));
#10304=CARTESIAN_POINT('Ctrl Pts',(6.10446550306057,2.92546114176053,6.83935137153874));
#10305=CARTESIAN_POINT('Ctrl Pts',(6.02686988076987,3.08214768724175,6.84754783524426));
#10306=CARTESIAN_POINT('Ctrl Pts',(5.94335884845949,3.23554857766629,6.85574429894977));
#10307=CARTESIAN_POINT('Ctrl Pts',(5.85982360635481,3.38899393890983,6.86394313880482));
#10308=CARTESIAN_POINT('Ctrl Pts',(5.7703697099494,3.53915143274394,6.87214197865987));
#10309=CARTESIAN_POINT('Ctrl Pts',(5.67529929279949,3.68554839028735,6.88034081851492));
#10310=CARTESIAN_POINT('Ctrl Pts',(5.58012957189289,3.83209826361977,6.88854822229156));
#10311=CARTESIAN_POINT('Ctrl Pts',(5.47933180520223,3.97487945171123,6.8967556260682));
#10312=CARTESIAN_POINT('Ctrl Pts',(5.37325094832126,4.11344906937775,6.90496302984484));
#10313=CARTESIAN_POINT('Ctrl Pts',(5.26711326891827,4.25209291226628,6.91317482994137));
#10314=CARTESIAN_POINT('Ctrl Pts',(5.15568708661717,4.38652041145342,6.92138663003791));
#10315=CARTESIAN_POINT('Ctrl Pts',(5.03935632556689,4.51632337460118,6.92959843013445));
#10316=CARTESIAN_POINT('Ctrl Pts',(4.92285430938292,4.64631742584642,6.93782231914806));
#10317=CARTESIAN_POINT('Ctrl Pts',(4.80143353468832,4.77167307777975,6.94604620816167));
#10318=CARTESIAN_POINT('Ctrl Pts',(4.67551424132182,4.89201958082721,6.95427009717528));
#10319=CARTESIAN_POINT('Ctrl Pts',(4.55916699638352,5.003217664085,6.96186882810706));
#10320=CARTESIAN_POINT('Ctrl Pts',(4.43897971397702,5.11013950919111,6.96946755903884));
#10321=CARTESIAN_POINT('Ctrl Pts',(4.31530694643228,5.21252481606307,6.97706628997062));
#10322=CARTESIAN_POINT('Ctrl Pts',(4.18143145231705,5.32335668163658,6.98529189920001));
#10323=CARTESIAN_POINT('Ctrl Pts',(4.04309549009467,5.4291832258518,6.99351750842941));
#10324=CARTESIAN_POINT('Ctrl Pts',(3.90070882041701,5.52962563817126,7.0017431176588));
#10325=CARTESIAN_POINT('Ctrl Pts',(3.75850810645129,5.62993687360223,7.00995798431641));
#10326=CARTESIAN_POINT('Ctrl Pts',(3.61226751526927,5.72487778127523,7.01817285097402));
#10327=CARTESIAN_POINT('Ctrl Pts',(3.46243083959908,5.81410884667575,7.02638771763162));
#10328=CARTESIAN_POINT('Ctrl Pts',(3.3435308009667,5.88491645820261,7.03290646852209));
#10329=CARTESIAN_POINT('Ctrl Pts',(3.22236708440406,5.95212932762741,7.03942521941255));
#10330=CARTESIAN_POINT('Ctrl Pts',(3.09917575053257,6.0155962852664,7.04594397030302));
#10331=CARTESIAN_POINT('Ctrl Pts',(3.09917575053259,6.01559628526639,5.04568623149126));
#10332=CARTESIAN_POINT('Ctrl Pts',(2.96116928620942,6.08669585168754,5.05301666782408));
#10333=CARTESIAN_POINT('Ctrl Pts',(2.82086347532898,6.15296737661428,5.0603471041569));
#10334=CARTESIAN_POINT('Ctrl Pts',(2.6786296007288,6.21427650351185,5.06767754048972));
#10335=CARTESIAN_POINT('Ctrl Pts',(2.52047449629172,6.28244838868821,5.07582852369992));
#10336=CARTESIAN_POINT('Ctrl Pts',(2.35946675698987,6.34468578280044,5.08397950691011));
#10337=CARTESIAN_POINT('Ctrl Pts',(2.19609554583758,6.40073850063822,5.0921304901203));
#10338=CARTESIAN_POINT('Ctrl Pts',(2.03291410529744,6.45672610811473,5.10027200521759));
#10339=CARTESIAN_POINT('Ctrl Pts',(1.86737500017405,6.50654322228651,5.10841352031487));
#10340=CARTESIAN_POINT('Ctrl Pts',(1.69998989059556,6.54998651692299,5.11655503541215));
#10341=CARTESIAN_POINT('Ctrl Pts',(1.53276399019445,6.59338849025425,5.12468880666696));
#10342=CARTESIAN_POINT('Ctrl Pts',(1.36369593248479,6.63042862233689,5.13282257792177));
#10343=CARTESIAN_POINT('Ctrl Pts',(1.19331516365316,6.66095247845197,5.14095634917658));
#10344=CARTESIAN_POINT('Ctrl Pts',(1.02306061877344,6.69145372144133,5.14908409465302));
#10345=CARTESIAN_POINT('Ctrl Pts',(0.851495657629336,6.71544823651412,5.15721184012945));
#10346=CARTESIAN_POINT('Ctrl Pts',(0.679162619569531,6.73283202940482,5.16533958560589));
#10347=CARTESIAN_POINT('Ctrl Pts',(0.506921020068551,6.75020659859132,5.1734630185643));
#10348=CARTESIAN_POINT('Ctrl Pts',(0.333912518318684,6.76097739442739,5.18158645152271));
#10349=CARTESIAN_POINT('Ctrl Pts',(0.160687322145687,6.76509191249473,5.18970988448112));
#10350=CARTESIAN_POINT('Ctrl Pts',(-0.0136367096904394,6.76923253057113,
5.1978848475751));
#10351=CARTESIAN_POINT('Ctrl Pts',(-0.188179824193343,6.76663207214025,
5.20605981066907));
#10352=CARTESIAN_POINT('Ctrl Pts',(-0.362377918111779,6.7572902294089,5.21423477376305));
#10353=CARTESIAN_POINT('Ctrl Pts',(-0.53543870436596,6.74800937786923,5.22235636401021));
#10354=CARTESIAN_POINT('Ctrl Pts',(-0.708158593633639,6.7320749528716,5.23047795425738));
#10355=CARTESIAN_POINT('Ctrl Pts',(-0.879986681490872,6.70953891414296,
5.23859954450454));
#10356=CARTESIAN_POINT('Ctrl Pts',(-1.05183745423552,6.6869999001877,5.24672220697082));
#10357=CARTESIAN_POINT('Ctrl Pts',(-1.22279582814528,6.65785758412463,5.2548448694371));
#10358=CARTESIAN_POINT('Ctrl Pts',(-1.39231836932743,6.62221553246596,5.26296753190337));
#10359=CARTESIAN_POINT('Ctrl Pts',(-1.56189557310442,6.58656198801692,5.27109281352463));
#10360=CARTESIAN_POINT('Ctrl Pts',(-1.73003566423887,6.54440460977088,5.27921809514588));
#10361=CARTESIAN_POINT('Ctrl Pts',(-1.89620775112108,6.49589756420068,5.28734337676714));
#10362=CARTESIAN_POINT('Ctrl Pts',(-2.0641901860791,6.44686206262888,5.29555717859792));
#10363=CARTESIAN_POINT('Ctrl Pts',(-2.2301611163303,6.39133783897611,5.3037709804287));
#10364=CARTESIAN_POINT('Ctrl Pts',(-2.39359110047914,6.32953478888513,5.31198478225949));
#10365=CARTESIAN_POINT('Ctrl Pts',(-2.555539556285,6.26829199688184,5.32012412419064));
#10366=CARTESIAN_POINT('Ctrl Pts',(-2.7149926340114,6.20088394956441,5.3282634661218));
#10367=CARTESIAN_POINT('Ctrl Pts',(-2.87145868722545,6.12756183221006,5.33640280805295));
#10368=CARTESIAN_POINT('Ctrl Pts',(-3.03007180221354,6.05323357255117,5.34465383983355));
#10369=CARTESIAN_POINT('Ctrl Pts',(-3.1856149723243,5.97282793781744,5.35290487161414));
#10370=CARTESIAN_POINT('Ctrl Pts',(-3.3376055319347,5.88665255584181,5.36115590339474));
#10371=CARTESIAN_POINT('Ctrl Pts',(-3.4895960915451,5.80047717386617,5.36940693517534));
#10372=CARTESIAN_POINT('Ctrl Pts',(-3.63803374962661,5.70853230380453,5.37765796695593));
#10373=CARTESIAN_POINT('Ctrl Pts',(-3.78247011302279,5.61116822454018,5.38590899873653));
#10374=CARTESIAN_POINT('Ctrl Pts',(-3.92610605910102,5.51434370396698,5.39411430609861));
#10375=CARTESIAN_POINT('Ctrl Pts',(-4.06623930133962,5.41185376680362,5.4023196134607));
#10376=CARTESIAN_POINT('Ctrl Pts',(-4.20239125627052,5.30397932963743,5.41052492082279));
#10377=CARTESIAN_POINT('Ctrl Pts',(-4.33838048651541,5.19623382072589,5.41872042145044));
#10378=CARTESIAN_POINT('Ctrl Pts',(-4.4703976232599,5.08311684669612,5.4269159220781));
#10379=CARTESIAN_POINT('Ctrl Pts',(-4.59799152353825,4.96495346901362,5.43511142270575));
#10380=CARTESIAN_POINT('Ctrl Pts',(-4.72545897646506,4.84690719290202,5.4432988014769));
#10381=CARTESIAN_POINT('Ctrl Pts',(-4.84851165873501,4.72382471526246,5.45148618024805));
#10382=CARTESIAN_POINT('Ctrl Pts',(-4.96673006214933,4.59607239822679,5.4596735590192));
#10383=CARTESIAN_POINT('Ctrl Pts',(-5.0848554348888,4.46842061447463,5.46785449482251));
#10384=CARTESIAN_POINT('Ctrl Pts',(-5.1981538612819,4.33610657394146,5.47603543062581));
#10385=CARTESIAN_POINT('Ctrl Pts',(-5.30624135968965,4.19953469240568,5.48421636642911));
#10386=CARTESIAN_POINT('Ctrl Pts',(-5.41426585178197,4.06304242128902,5.49239253340504));
#10387=CARTESIAN_POINT('Ctrl Pts',(-5.51708524309896,3.92229753546664,5.50056870038096));
#10388=CARTESIAN_POINT('Ctrl Pts',(-5.61435462919919,3.7777388868991,5.50874486735688));
#10389=CARTESIAN_POINT('Ctrl Pts',(-5.71159650740211,3.63322111968817,5.51691872210312));
#10390=CARTESIAN_POINT('Ctrl Pts',(-5.80329130197457,3.4848920348556,5.52509257684936));
#10391=CARTESIAN_POINT('Ctrl Pts',(-5.88913627471908,3.33322110544558,5.53326643159561));
#10392=CARTESIAN_POINT('Ctrl Pts',(-5.97497064196954,3.18156891382636,5.54143927652421));
#10393=CARTESIAN_POINT('Ctrl Pts',(-6.05495644819303,3.02657601364368,5.54961212145281));
#10394=CARTESIAN_POINT('Ctrl Pts',(-6.12883595213694,2.86873820203128,5.55778496638141));
#10395=CARTESIAN_POINT('Ctrl Pts',(-6.20271998252309,2.71089072002725,5.56595831204307));
#10396=CARTESIAN_POINT('Ctrl Pts',(-6.27049681243584,2.55019830651772,5.57413165770474));
#10397=CARTESIAN_POINT('Ctrl Pts',(-6.33195605887713,2.38717855814122,5.5823050033664));
#10398=CARTESIAN_POINT('Ctrl Pts',(-6.39343042916145,2.22411869399324,5.59048036031854));
#10399=CARTESIAN_POINT('Ctrl Pts',(-6.44858399277493,2.05873069227569,5.59865571727068));
#10400=CARTESIAN_POINT('Ctrl Pts',(-6.49725561951404,1.89154921022246,5.60683107422282));
#10401=CARTESIAN_POINT('Ctrl Pts',(-6.54597272310192,1.72421152038486,5.61501406990611));
#10402=CARTESIAN_POINT('Ctrl Pts',(-6.58819569097599,1.55507734991728,5.62319706558941));
#10403=CARTESIAN_POINT('Ctrl Pts',(-6.62381390017596,1.38469434021946,5.63138006127271));
#10404=CARTESIAN_POINT('Ctrl Pts',(-6.65945008661356,1.21422533473683,5.63956718708105));
#10405=CARTESIAN_POINT('Ctrl Pts',(-6.68847480924185,1.04250658917657,5.64775431288939));
#10406=CARTESIAN_POINT('Ctrl Pts',(-6.71082913503712,0.870092707897813,
5.65594143869773));
#10407=CARTESIAN_POINT('Ctrl Pts',(-6.73321254946114,0.69745447257546,5.66413921802636));
#10408=CARTESIAN_POINT('Ctrl Pts',(-6.74890819351579,0.524119653610915,
5.67233699735498));
#10409=CARTESIAN_POINT('Ctrl Pts',(-6.75790918579735,0.350645742189842,
5.6805347766836));
#10410=CARTESIAN_POINT('Ctrl Pts',(-6.76400114372378,0.233236934732492,
5.68608311237792));
#10411=CARTESIAN_POINT('Ctrl Pts',(-6.767027561351,0.115764423594308,5.69163144807225));
#10412=CARTESIAN_POINT('Ctrl Pts',(-6.76699981083753,-0.0016000390173538,
5.69717978376658));
#10413=CARTESIAN_POINT('',(-6.76699775674603,-0.00551000855003846,5.30282021621645));
#10414=CARTESIAN_POINT('Ctrl Pts',(3.09917575053259,6.01559628526639,4.6512641878525));
#10415=CARTESIAN_POINT('Ctrl Pts',(2.94379378017301,6.09564754066526,4.65947003774372));
#10416=CARTESIAN_POINT('Ctrl Pts',(2.78537750733939,6.16963903341803,4.66767588763494));
#10417=CARTESIAN_POINT('Ctrl Pts',(2.62444459443469,6.23735357108626,4.67588173752615));
#10418=CARTESIAN_POINT('Ctrl Pts',(2.46332583431231,6.30514630629777,4.68409706362919));
#10419=CARTESIAN_POINT('Ctrl Pts',(2.29968495923358,6.36664746761495,4.69231238973223));
#10420=CARTESIAN_POINT('Ctrl Pts',(2.13405782503788,6.42168873423453,4.70052771583526));
#10421=CARTESIAN_POINT('Ctrl Pts',(1.96832706039393,6.47676443936057,4.70874818214633));
#10422=CARTESIAN_POINT('Ctrl Pts',(1.8006079028474,6.52537209375087,4.71696864845741));
#10423=CARTESIAN_POINT('Ctrl Pts',(1.63144841051177,6.56739408622923,4.72518911476848));
#10424=CARTESIAN_POINT('Ctrl Pts',(1.46203675112782,6.60947872113848,4.73342183537694));
#10425=CARTESIAN_POINT('Ctrl Pts',(1.29118081740452,6.64495800742516,4.74165455598541));
#10426=CARTESIAN_POINT('Ctrl Pts',(1.11943700963936,6.67376578712871,4.74988727659387));
#10427=CARTESIAN_POINT('Ctrl Pts',(1.00011266853046,6.693780886227,4.7556072147676));
#10428=CARTESIAN_POINT('Ctrl Pts',(0.880359858345819,6.71057659890094,4.76132715294134));
#10429=CARTESIAN_POINT('Ctrl Pts',(0.760365468820596,6.72414554823327,4.76704709111507));
#10430=CARTESIAN_POINT('Ctrl Pts',(0.589277934671798,6.74349210344675,4.77520255672892));
#10431=CARTESIAN_POINT('Ctrl Pts',(0.417172491072261,6.75633628735233,4.78335802234277));
#10432=CARTESIAN_POINT('Ctrl Pts',(0.244589315295944,6.76257828545024,4.79151348795662));
#10433=CARTESIAN_POINT('Ctrl Pts',(0.0722161943895885,6.76881268627169,
4.7996590273696));
#10434=CARTESIAN_POINT('Ctrl Pts',(-0.100633140023653,6.7684608835869,4.80780456678259));
#10435=CARTESIAN_POINT('Ctrl Pts',(-0.27341030951152,6.7614743808324,4.81595010619557));
#10436=CARTESIAN_POINT('Ctrl Pts',(-0.44601351943161,6.75449491239269,4.82408744432525));
#10437=CARTESIAN_POINT('Ctrl Pts',(-0.618544346604936,6.7408940574451,4.83222478245492));
#10438=CARTESIAN_POINT('Ctrl Pts',(-0.790451303999063,6.72067524405146,
4.8403621205846));
#10439=CARTESIAN_POINT('Ctrl Pts',(-0.962221304617605,6.70047253881035,
4.84849297576787));
#10440=CARTESIAN_POINT('Ctrl Pts',(-1.13336806379849,6.67366241576214,4.85662383095114));
#10441=CARTESIAN_POINT('Ctrl Pts',(-1.30334211510246,6.640300319338,4.86475468613441));
#10442=CARTESIAN_POINT('Ctrl Pts',(-1.47321645540309,6.60695779394885,4.87288077155593));
#10443=CARTESIAN_POINT('Ctrl Pts',(-1.64191910008596,6.56707101975891,4.88100685697745));
#10444=CARTESIAN_POINT('Ctrl Pts',(-1.80890771665984,6.52074703332437,4.88913294239897));
#10445=CARTESIAN_POINT('Ctrl Pts',(-1.97648819713343,6.47425885907975,4.89728782940413));
#10446=CARTESIAN_POINT('Ctrl Pts',(-2.1423421084596,6.42128780712883,4.90544271640928));
#10447=CARTESIAN_POINT('Ctrl Pts',(-2.30593306370863,6.36199353235252,4.91359760341444));
#10448=CARTESIAN_POINT('Ctrl Pts',(-2.46888631352175,6.302930396769,4.92172070127964));
#10449=CARTESIAN_POINT('Ctrl Pts',(-2.62959387792738,6.23759338951028,4.92984379914484));
#10450=CARTESIAN_POINT('Ctrl Pts',(-2.78754251622039,6.16618972464063,4.93796689701004));
#10451=CARTESIAN_POINT('Ctrl Pts',(-2.94550355781162,6.09478045262579,4.94609063276112));
#10452=CARTESIAN_POINT('Ctrl Pts',(-3.10070490837661,6.01730372472583,4.95421436851219));
#10453=CARTESIAN_POINT('Ctrl Pts',(-3.25265517233035,5.9340140992344,4.96233810426327));
#10454=CARTESIAN_POINT('Ctrl Pts',(-3.40464627678165,5.85070208753805,4.97046402347491));
#10455=CARTESIAN_POINT('Ctrl Pts',(-3.55338423403857,5.76157424305647,4.97858994268655));
#10456=CARTESIAN_POINT('Ctrl Pts',(-3.69840406820863,5.66693006382273,4.9867158618982));
#10457=CARTESIAN_POINT('Ctrl Pts',(-3.84435093991683,5.57168087281651,4.99489372595025));
#10458=CARTESIAN_POINT('Ctrl Pts',(-3.98653167296087,5.47084478143509,5.0030715900023));
#10459=CARTESIAN_POINT('Ctrl Pts',(-4.12450434650044,5.36476960322612,5.01124945405434));
#10460=CARTESIAN_POINT('Ctrl Pts',(-4.26181886296236,5.25920042470181,5.01938830806935));
#10461=CARTESIAN_POINT('Ctrl Pts',(-4.39496513663363,5.14844231410795,5.02752716208435));
#10462=CARTESIAN_POINT('Ctrl Pts',(-4.52354328470869,5.03287642917715,5.03566601609935));
#10463=CARTESIAN_POINT('Ctrl Pts',(-4.65304585745895,4.91647967245949,5.04386338516992));
#10464=CARTESIAN_POINT('Ctrl Pts',(-4.77791410018989,4.79520601220695,5.05206075424049));
#10465=CARTESIAN_POINT('Ctrl Pts',(-4.89777978688905,4.66947985959261,5.06025812331106));
#10466=CARTESIAN_POINT('Ctrl Pts',(-5.01764547358821,4.54375370697827,5.06845549238163));
#10467=CARTESIAN_POINT('Ctrl Pts',(-5.13250840380614,4.41357538154202,5.0766528614522));
#10468=CARTESIAN_POINT('Ctrl Pts',(-5.24204411540993,4.27939978175633,5.08485023052277));
#10469=CARTESIAN_POINT('Ctrl Pts',(-5.35181758225108,4.14493294406195,5.09306539257976));
#10470=CARTESIAN_POINT('Ctrl Pts',(-5.45657409523093,4.00604321012243,5.10128055463675));
#10471=CARTESIAN_POINT('Ctrl Pts',(-5.55593672498614,3.86314070517116,5.10949571669374));
#10472=CARTESIAN_POINT('Ctrl Pts',(-5.65514609786602,3.72045861297909,5.11769820768848));
#10473=CARTESIAN_POINT('Ctrl Pts',(-5.74897796451272,3.57377637754121,5.12590069868322));
#10474=CARTESIAN_POINT('Ctrl Pts',(-5.83709498010553,3.42353781828488,5.13410318967796));
#10475=CARTESIAN_POINT('Ctrl Pts',(-5.92513272842456,3.27343440887366,5.14229830197183));
#10476=CARTESIAN_POINT('Ctrl Pts',(-6.00746567983744,3.11978135266527,5.15049341426569));
#10477=CARTESIAN_POINT('Ctrl Pts',(-6.08379874921153,2.96305278034196,5.15868852655956));
#10478=CARTESIAN_POINT('Ctrl Pts',(-6.16007713347613,2.80643648857032,5.1668777678644));
#10479=CARTESIAN_POINT('Ctrl Pts',(-6.23036403780076,2.64674938977569,5.17506700916924));
#10480=CARTESIAN_POINT('Ctrl Pts',(-6.29440943045395,2.48449168278189,5.18325625047408));
#10481=CARTESIAN_POINT('Ctrl Pts',(-6.35842067059958,2.32232050047526,5.19144112482738));
#10482=CARTESIAN_POINT('Ctrl Pts',(-6.41619689627616,2.15758177379574,5.19962599918069));
#10483=CARTESIAN_POINT('Ctrl Pts',(-6.4675354844331,1.99079726682521,5.207810873534));
#10484=CARTESIAN_POINT('Ctrl Pts',(-6.51886159240832,1.82405330442417,5.21599375818087));
#10485=CARTESIAN_POINT('Ctrl Pts',(-6.56375306949973,1.65526489418047,5.22417664282774));
#10486=CARTESIAN_POINT('Ctrl Pts',(-6.60205654749343,1.48497082250767,5.23235952747461));
#10487=CARTESIAN_POINT('Ctrl Pts',(-6.6403536107168,1.31470527036933,5.24054104171522));
#10488=CARTESIAN_POINT('Ctrl Pts',(-6.67206479634895,1.14293491054509,5.24872255595584));
#10489=CARTESIAN_POINT('Ctrl Pts',(-6.69708747044849,0.970210499408155,
5.25690407019646));
#10490=CARTESIAN_POINT('Ctrl Pts',(-6.72211774241653,0.797433642343305,
5.26508806866674));
#10491=CARTESIAN_POINT('Ctrl Pts',(-6.74045539111042,0.623702511082844,
5.27327206713702));
#10492=CARTESIAN_POINT('Ctrl Pts',(-6.75204939536963,0.449575313477734,
5.28145606560731));
#10493=CARTESIAN_POINT('Ctrl Pts',(-6.76213802762554,0.298056888685469,
5.28857744913483));
#10494=CARTESIAN_POINT('Ctrl Pts',(-6.76712131778368,0.146238821399111,
5.29569883266236));
#10495=CARTESIAN_POINT('Ctrl Pts',(-6.76699775674649,-0.005510007984206,
5.30282021618989));
#10496=CARTESIAN_POINT('Ctrl Pts',(-6.76699775674603,-0.00551000855004313,
5.30282021621645));
#10497=CARTESIAN_POINT('Ctrl Pts',(-6.76683015283113,-0.211349129456567,
5.31247998974423));
#10498=CARTESIAN_POINT('Ctrl Pts',(-6.7572668966955,-0.416798432664565,
5.32213976327201));
#10499=CARTESIAN_POINT('Ctrl Pts',(-6.73843761571402,-0.621085742172807,
5.3317995367998));
#10500=CARTESIAN_POINT('Ctrl Pts',(-6.71949010387446,-0.826655791256934,
5.34151996497044));
#10501=CARTESIAN_POINT('Ctrl Pts',(-6.69115993265996,-1.03104915348694,
5.35124039314108));
#10502=CARTESIAN_POINT('Ctrl Pts',(-6.65362825886052,-1.23349908507983,
5.36096082131172));
#10503=CARTESIAN_POINT('Ctrl Pts',(-6.61582629362638,-1.4374069980768,5.37075125298101));
#10504=CARTESIAN_POINT('Ctrl Pts',(-6.56868987512742,-1.63934333522378,
5.3805416846503));
#10505=CARTESIAN_POINT('Ctrl Pts',(-6.51245256702596,-1.83854577376713,
5.39033211631959));
#10506=CARTESIAN_POINT('Ctrl Pts',(-6.48886102517112,-1.92211116523296,
5.39443920085654));
#10507=CARTESIAN_POINT('Ctrl Pts',(-6.4636684854269,-2.00519570320228,5.39854628539348));
#10508=CARTESIAN_POINT('Ctrl Pts',(-6.43689467054598,-2.08774423728021,
5.40265336993043));
#10509=CARTESIAN_POINT('Ctrl Pts',(-6.38326861970604,-2.25308309186314,
5.41087956874304));
#10510=CARTESIAN_POINT('Ctrl Pts',(-6.32319315124855,-2.41658554801291,
5.41910576755564));
#10511=CARTESIAN_POINT('Ctrl Pts',(-6.25681139010063,-2.57771220827832,
5.42733196636825));
#10512=CARTESIAN_POINT('Ctrl Pts',(-6.19050419513153,-2.73865787606696,
5.43554892474792));
#10513=CARTESIAN_POINT('Ctrl Pts',(-6.11790494864706,-2.8972327335221,5.4437658831276));
#10514=CARTESIAN_POINT('Ctrl Pts',(-6.03920665213129,-3.05291205455598,
5.45198284150727));
#10515=CARTESIAN_POINT('Ctrl Pts',(-5.96058096147473,-3.20844774820064,
5.46019221904531));
#10516=CARTESIAN_POINT('Ctrl Pts',(-5.87586758773257,-3.36109290751923,
5.46840159658335));
#10517=CARTESIAN_POINT('Ctrl Pts',(-5.78530779642657,-3.51034224835785,
5.47661097412138));
#10518=CARTESIAN_POINT('Ctrl Pts',(-5.69481338394813,-3.659483839976,5.48481442497307));
#10519=CARTESIAN_POINT('Ctrl Pts',(-5.59848114623985,-3.80523419087512,
5.49301787582476));
#10520=CARTESIAN_POINT('Ctrl Pts',(-5.49659853754853,-3.94711204768998,
5.50122132667646));
#10521=CARTESIAN_POINT('Ctrl Pts',(-5.39476904465944,-4.08891593745314,
5.50942050071507));
#10522=CARTESIAN_POINT('Ctrl Pts',(-5.28739515414085,-4.22685106452199,
5.51761967475368));
#10523=CARTESIAN_POINT('Ctrl Pts',(-5.17480799130005,-4.36046456850381,
5.5258188487923));
#10524=CARTESIAN_POINT('Ctrl Pts',(-5.06224201381201,-4.49405293063869,
5.53401648000498));
#10525=CARTESIAN_POINT('Ctrl Pts',(-4.9444649440962,-4.62332101150091,5.54221411121767));
#10526=CARTESIAN_POINT('Ctrl Pts',(-4.82184879385737,-4.74784827149902,
5.55041174243035));
#10527=CARTESIAN_POINT('Ctrl Pts',(-4.69924147523692,-4.8723665622281,5.55860878319593));
#10528=CARTESIAN_POINT('Ctrl Pts',(-4.57179602126017,-4.99214445594116,
5.56680582396151));
#10529=CARTESIAN_POINT('Ctrl Pts',(-4.43992193486087,-5.10679764748333,
5.57500286472709));
#10530=CARTESIAN_POINT('Ctrl Pts',(-4.3080333789626,-5.22146341901208,5.58320080488903));
#10531=CARTESIAN_POINT('Ctrl Pts',(-4.17171549328966,-5.33100313273541,
5.59139874505098));
#10532=CARTESIAN_POINT('Ctrl Pts',(-4.03141157506078,-5.43507219017981,
5.59959668521292));
#10533=CARTESIAN_POINT('Ctrl Pts',(-3.89106676225446,-5.53917158077658,
5.60779701483983));
#10534=CARTESIAN_POINT('Ctrl Pts',(-3.74673389070807,-5.63779692533518,
5.61599734446675));
#10535=CARTESIAN_POINT('Ctrl Pts',(-3.5988860268442,-5.7306464177949,5.62419767409366));
#10536=CARTESIAN_POINT('Ctrl Pts',(-3.45088406562515,-5.82359268447135,
5.63240655067604));
#10537=CARTESIAN_POINT('Ctrl Pts',(-3.29936009697943,-5.91075088099942,
5.64061542725841));
#10538=CARTESIAN_POINT('Ctrl Pts',(-3.14481350150923,-5.99186423750783,
5.64882430384079));
#10539=CARTESIAN_POINT('Ctrl Pts',(-2.99018394195464,-6.07302113748825,
5.65703758713253));
#10540=CARTESIAN_POINT('Ctrl Pts',(-2.83252884433751,-6.14812657430631,
5.66525087042427));
#10541=CARTESIAN_POINT('Ctrl Pts',(-2.67236834906832,-6.21697164276128,
5.67346415371601));
#10542=CARTESIAN_POINT('Ctrl Pts',(-2.51197355847061,-6.2859174231796,5.68168945204244));
#10543=CARTESIAN_POINT('Ctrl Pts',(-2.34906638051688,-6.3485844044854,5.68991475036888));
#10544=CARTESIAN_POINT('Ctrl Pts',(-2.18418413767397,-6.40481292878515,
5.69814004869531));
#10545=CARTESIAN_POINT('Ctrl Pts',(-2.03506743547588,-6.45566505190331,
5.70557886890958));
#10546=CARTESIAN_POINT('Ctrl Pts',(-1.88433568322539,-6.50125170540708,
5.71301768912384));
#10547=CARTESIAN_POINT('Ctrl Pts',(-1.73239321362362,-6.54149086626213,
5.72045650933811));
#10548=CARTESIAN_POINT('Ctrl Pts',(-1.56587222656749,-6.58559087859873,
5.72860906660441));
#10549=CARTESIAN_POINT('Ctrl Pts',(-1.39740575776914,-6.62339724995082,
5.73676162387072));
#10550=CARTESIAN_POINT('Ctrl Pts',(-1.22751480718071,-6.65473488563986,
5.74491418113703));
#10551=CARTESIAN_POINT('Ctrl Pts',(-1.05782067914945,-6.68603621596024,
5.75305729347903));
#10552=CARTESIAN_POINT('Ctrl Pts',(-0.886705710220385,-6.71088366286189,
5.76120040582103));
#10553=CARTESIAN_POINT('Ctrl Pts',(-0.714706210401798,-6.72915180634329,
5.76934351816303));
#10554=CARTESIAN_POINT('Ctrl Pts',(-0.542869815212691,-6.74740262640934,
5.77747890850978));
#10555=CARTESIAN_POINT('Ctrl Pts',(-0.370150920070342,-6.75908652587784,
5.78561429885652));
#10556=CARTESIAN_POINT('Ctrl Pts',(-0.197096186913418,-6.76412907129249,
5.79374968920327));
#10557=CARTESIAN_POINT('Ctrl Pts',(-0.0241691960950483,-6.76916789449434,
5.80187907431821));
#10558=CARTESIAN_POINT('Ctrl Pts',(0.149092775254158,-6.7675751145626,5.81000845943315));
#10559=CARTESIAN_POINT('Ctrl Pts',(0.322137779497406,-6.75932809168341,
5.81813784454809));
#10560=CARTESIAN_POINT('Ctrl Pts',(0.495091396288253,-6.7510854241707,5.82626293642267));
#10561=CARTESIAN_POINT('Ctrl Pts',(0.667827909838346,-6.73619552974571,
5.83438802829725));
#10562=CARTESIAN_POINT('Ctrl Pts',(0.839795209358442,-6.71468785621034,
5.84251312017184));
#10563=CARTESIAN_POINT('Ctrl Pts',(1.01241890820848,-6.69309808786662,5.85066922552909));
#10564=CARTESIAN_POINT('Ctrl Pts',(1.18426713698976,-6.66483991755443,5.85882533088633));
#10565=CARTESIAN_POINT('Ctrl Pts',(1.35478594662076,-6.62999577969993,5.86698143624358));
#10566=CARTESIAN_POINT('Ctrl Pts',(1.52461848563241,-6.59529187568895,5.87510471650964));
#10567=CARTESIAN_POINT('Ctrl Pts',(1.69313192983739,-6.55405501238566,5.8832279967757));
#10568=CARTESIAN_POINT('Ctrl Pts',(1.85978889903861,-6.50641792778582,5.89135127704177));
#10569=CARTESIAN_POINT('Ctrl Pts',(2.02646806008045,-6.45877449988937,5.89947563899401));
#10570=CARTESIAN_POINT('Ctrl Pts',(2.19128990195624,-6.40472925373183,5.90760000094626));
#10571=CARTESIAN_POINT('Ctrl Pts',(2.35373205038518,-6.34446486592759,5.9157243628985));
#10572=CARTESIAN_POINT('Ctrl Pts',(2.51622673485063,-6.2841809877872,5.92385135238172));
#10573=CARTESIAN_POINT('Ctrl Pts',(2.67633985049586,-6.21767408993008,5.93197834186494));
#10574=CARTESIAN_POINT('Ctrl Pts',(2.83356889446269,-6.14517504391319,5.94010533134816));
#10575=CARTESIAN_POINT('Ctrl Pts',(2.99181434641751,-6.0722073274291,5.94828485779796));
#10576=CARTESIAN_POINT('Ctrl Pts',(3.14713796794377,-5.99316987903029,5.95646438424776));
#10577=CARTESIAN_POINT('Ctrl Pts',(3.29905329503049,-5.90834463759084,5.96464391069756));
#10578=CARTESIAN_POINT('Ctrl Pts',(3.4502532609927,-5.82391883366219,5.97278492019617));
#10579=CARTESIAN_POINT('Ctrl Pts',(3.59807668396,-5.73375987335539,5.98092592969477));
#10580=CARTESIAN_POINT('Ctrl Pts',(3.74207405287236,-5.63818860830493,5.98906693919338));
#10581=CARTESIAN_POINT('Ctrl Pts',(3.88709334780595,-5.54193908945458,5.99726572411878));
#10582=CARTESIAN_POINT('Ctrl Pts',(4.02823177706549,-5.44020038376709,6.00546450904418));
#10583=CARTESIAN_POINT('Ctrl Pts',(4.16506530151591,-5.3333404198596,6.01366329396958));
#10584=CARTESIAN_POINT('Ctrl Pts',(4.30189882596633,-5.22648045595211,6.02186207889498));
#10585=CARTESIAN_POINT('Ctrl Pts',(4.43442720375673,-5.11449952299128,6.03006086382038));
#10586=CARTESIAN_POINT('Ctrl Pts',(4.56226549995563,-4.99780176756888,6.03825964874578));
#10587=CARTESIAN_POINT('Ctrl Pts',(4.69063807453216,-4.88061629376089,6.04649269909585));
#10588=CARTESIAN_POINT('Ctrl Pts',(4.81468041406076,-4.75831030239312,6.05472574944592));
#10589=CARTESIAN_POINT('Ctrl Pts',(4.93395882092062,-4.63123518658464,6.06295879979599));
#10590=CARTESIAN_POINT('Ctrl Pts',(5.053095185574,-4.50431139766183,6.07118204585148));
#10591=CARTESIAN_POINT('Ctrl Pts',(5.16747867139335,-4.37263005177017,6.07940529190697));
#10592=CARTESIAN_POINT('Ctrl Pts',(5.27670932851735,-4.23658207312664,6.08762853796247));
#10593=CARTESIAN_POINT('Ctrl Pts',(5.38583177150484,-4.10066887637421,6.09584363729894));
#10594=CARTESIAN_POINT('Ctrl Pts',(5.48981132951567,-3.96039793952431,6.10405873663542));
#10595=CARTESIAN_POINT('Ctrl Pts',(5.58828549491801,-3.81619630355791,6.1122738359719));
#10596=CARTESIAN_POINT('Ctrl Pts',(5.68668180526696,-3.67210867542309,6.12048244033587));
#10597=CARTESIAN_POINT('Ctrl Pts',(5.77958119151103,-3.52409683248066,6.12869104469984));
#10598=CARTESIAN_POINT('Ctrl Pts',(5.86666192876941,-3.37262017036127,6.1368996490638));
#10599=CARTESIAN_POINT('Ctrl Pts',(5.95369123735051,-3.22123296826042,6.14510340553973));
#10600=CARTESIAN_POINT('Ctrl Pts',(6.03490856471226,-3.06638533313291,6.15330716201566));
#10601=CARTESIAN_POINT('Ctrl Pts',(6.11003592269379,-2.90856494226816,6.16151091849158));
#10602=CARTESIAN_POINT('Ctrl Pts',(6.18514105240366,-2.75079124643726,6.16971224768493));
#10603=CARTESIAN_POINT('Ctrl Pts',(6.25415964474432,-2.5900468682646,6.17791357687827));
#10604=CARTESIAN_POINT('Ctrl Pts',(6.31685992330173,-2.42684356920353,6.18611490607161));
#10605=CARTESIAN_POINT('Ctrl Pts',(6.37955155490192,-2.26366277741001,6.19431510422464));
#10606=CARTESIAN_POINT('Ctrl Pts',(6.43592647895956,-2.09802407416045,6.20251530237767));
#10607=CARTESIAN_POINT('Ctrl Pts',(6.48580128391907,-1.93045867749449,6.2107155005307));
#10608=CARTESIAN_POINT('Ctrl Pts',(6.53567824900255,-1.76288602341608,6.2189160538419));
#10609=CARTESIAN_POINT('Ctrl Pts',(6.5790544318461,-1.59338685307305,6.22711660715311));
#10610=CARTESIAN_POINT('Ctrl Pts',(6.61579645043946,-1.42250705669696,6.23531716046431));
#10611=CARTESIAN_POINT('Ctrl Pts',(6.65254671873605,-1.25158889259744,6.24351955504972));
#10612=CARTESIAN_POINT('Ctrl Pts',(6.68265978067487,-1.0792898352538,6.25172194963513));
#10613=CARTESIAN_POINT('Ctrl Pts',(6.7060534630617,-0.906165520508382,6.25992434422054));
#10614=CARTESIAN_POINT('Ctrl Pts',(6.72946902265369,-0.732879304096949,
6.2681344094867));
#10615=CARTESIAN_POINT('Ctrl Pts',(6.74615260014355,-0.558766643887226,
6.27634447475286));
#10616=CARTESIAN_POINT('Ctrl Pts',(6.75607387881625,-0.384388792730363,
6.28455454001902));
#10617=CARTESIAN_POINT('Ctrl Pts',(6.76599990563727,-0.209927487421393,
6.29276853447705));
#10618=CARTESIAN_POINT('Ctrl Pts',(6.76915717448567,-0.0352010961438072,
6.30098252893508));
#10619=CARTESIAN_POINT('Ctrl Pts',(6.76556753754379,0.139229648185006,6.30919652339312));
#10620=CARTESIAN_POINT('Ctrl Pts',(6.76197300673196,0.313898199676781,6.31742171625958));
#10621=CARTESIAN_POINT('Ctrl Pts',(6.75161320850349,0.48826994093554,6.32564690912605));
#10622=CARTESIAN_POINT('Ctrl Pts',(6.734561969058,0.661788550004968,6.33387210199252));
#10623=CARTESIAN_POINT('Ctrl Pts',(6.7192278320421,0.81783340145307,6.3412689973795));
#10624=CARTESIAN_POINT('Ctrl Pts',(6.69848280746823,0.973188206981381,6.34866589276647));
#10625=CARTESIAN_POINT('Ctrl Pts',(6.67241566428336,1.12745651935055,6.35606278815344));
#10626=CARTESIAN_POINT('Ctrl Pts',(6.64194671870187,1.30777519797171,6.36470875297664));
#10627=CARTESIAN_POINT('Ctrl Pts',(6.60413684375698,1.48701865212884,6.37335471779985));
#10628=CARTESIAN_POINT('Ctrl Pts',(6.55907461042364,1.66458080455592,6.38200068262305));
#10629=CARTESIAN_POINT('Ctrl Pts',(6.51407001780353,1.84191583088753,6.39063558808362));
#10630=CARTESIAN_POINT('Ctrl Pts',(6.4618316398377,2.01757354977261,6.3992704935442));
#10631=CARTESIAN_POINT('Ctrl Pts',(6.40249921940896,2.19095703870881,6.40790539900478));
#10632=CARTESIAN_POINT('Ctrl Pts',(6.34119699297558,2.37009677077723,6.41682697890915));
#10633=CARTESIAN_POINT('Ctrl Pts',(6.27232161673629,2.54680835028713,6.42574855881353));
#10634=CARTESIAN_POINT('Ctrl Pts',(6.19608434960343,2.72044623777047,6.4346701387179));
#10635=CARTESIAN_POINT('Ctrl Pts',(6.12250058011828,2.88804052291443,6.44328119606316));
#10636=CARTESIAN_POINT('Ctrl Pts',(6.04205885699316,3.0527711420892,6.45189225340842));
#10637=CARTESIAN_POINT('Ctrl Pts',(5.95499947385894,3.21407378047546,6.46050331075368));
#10638=CARTESIAN_POINT('Ctrl Pts',(5.86802219155686,3.37522430337039,6.46910624749265));
#10639=CARTESIAN_POINT('Ctrl Pts',(5.7744398360222,3.53295302322623,6.47770918423163));
#10640=CARTESIAN_POINT('Ctrl Pts',(5.67453994056898,3.68671743735364,6.4863121209706));
#10641=CARTESIAN_POINT('Ctrl Pts',(5.57475190951144,3.84030967148841,6.49490542444305));
#10642=CARTESIAN_POINT('Ctrl Pts',(5.46866061707592,3.989946200575,6.50349872791549));
#10643=CARTESIAN_POINT('Ctrl Pts',(5.3565985952027,4.13511069862373,6.51209203138793));
#10644=CARTESIAN_POINT('Ctrl Pts',(5.34411295400281,4.15128452636039,6.51304947354438));
#10645=CARTESIAN_POINT('Ctrl Pts',(5.33155323905529,4.16740286656107,6.51400691570084));
#10646=CARTESIAN_POINT('Ctrl Pts',(5.31891994443521,4.18346502611046,6.51496435785729));
#10647=CARTESIAN_POINT('Ctrl Pts',(5.20551707715331,4.32764712606281,6.52355884481129));
#10648=CARTESIAN_POINT('Ctrl Pts',(5.08631475608562,4.46713086329329,6.53215333176528));
#10649=CARTESIAN_POINT('Ctrl Pts',(4.96173253515189,4.6014670757939,6.54074781871927));
#10650=CARTESIAN_POINT('Ctrl Pts',(4.83703437850644,4.73592830103138,6.54935030366812));
#10651=CARTESIAN_POINT('Ctrl Pts',(4.70694653633858,4.8652322163818,6.55795278861697));
#10652=CARTESIAN_POINT('Ctrl Pts',(4.57192474548497,4.98896713976172,6.56655527356581));
#10653=CARTESIAN_POINT('Ctrl Pts',(4.43668617461203,5.11290072188339,6.5751715699657));
#10654=CARTESIAN_POINT('Ctrl Pts',(4.29649804557332,5.23124723238171,6.58378786636558));
#10655=CARTESIAN_POINT('Ctrl Pts',(4.15184981072849,5.34363473201096,6.59240416276547));
#10656=CARTESIAN_POINT('Ctrl Pts',(4.00707356132342,5.45612169525521,6.60102808463963));
#10657=CARTESIAN_POINT('Ctrl Pts',(3.85782957356289,5.56263894109501,6.6096520065138));
#10658=CARTESIAN_POINT('Ctrl Pts',(3.7046362967204,5.66285783937949,6.61827592838796));
#10659=CARTESIAN_POINT('Ctrl Pts',(3.55121921613449,5.76322314986338,6.62691244915705));
#10660=CARTESIAN_POINT('Ctrl Pts',(3.39384157512814,5.85727156267731,6.63554896992614));
#10661=CARTESIAN_POINT('Ctrl Pts',(3.23304779615372,5.94471958529463,6.64418549069524));
#10662=CARTESIAN_POINT('Ctrl Pts',(3.18867984950435,5.96884918301181,6.64656857227441));
#10663=CARTESIAN_POINT('Ctrl Pts',(3.14405193078544,5.99247652073751,6.64895165385358));
#10664=CARTESIAN_POINT('Ctrl Pts',(3.0991757505326,6.01559628526638,6.65133473543275));
#10665=CARTESIAN_POINT('Origin',(0.,0.,-3.69717978381041));
#10666=CARTESIAN_POINT('',(3.09917575053258,6.01559628526639,9.04575158274221));
#10667=CARTESIAN_POINT('',(3.09917575053261,6.01559628526638,8.65154848238438));
#10668=CARTESIAN_POINT('',(3.09917575053259,6.01559628526639,-3.69717978381041));
#10669=CARTESIAN_POINT('',(-6.767,1.71993712674845E-12,7.69717978381002));
#10670=CARTESIAN_POINT('Ctrl Pts',(-6.767,1.71993607050078E-12,7.69717978381002));
#10671=CARTESIAN_POINT('Ctrl Pts',(-6.76700000000005,-0.186007249414041,
7.70592929561598));
#10672=CARTESIAN_POINT('Ctrl Pts',(-6.75932637295447,-0.37201435552598,
7.71467880742193));
#10673=CARTESIAN_POINT('Ctrl Pts',(-6.7440051826694,-0.557389537153581,
7.72342831922788));
#10674=CARTESIAN_POINT('Ctrl Pts',(-6.7286840570966,-0.742763935810137,
7.73217779407844));
#10675=CARTESIAN_POINT('Ctrl Pts',(-6.70571545653006,-0.927506129693983,
7.74092726892899));
#10676=CARTESIAN_POINT('Ctrl Pts',(-6.67517739415664,-1.11098863924891,
7.74967674377954));
#10677=CARTESIAN_POINT('Ctrl Pts',(-6.64463945823084,-1.29447038906586,
7.75842618240152));
#10678=CARTESIAN_POINT('Ctrl Pts',(-6.60653217027137,-1.47669218228306,
7.76717562102351));
#10679=CARTESIAN_POINT('Ctrl Pts',(-6.56098496116688,-1.65703510504215,
7.77592505964549));
#10680=CARTESIAN_POINT('Ctrl Pts',(-6.51543793687484,-1.83737729604139,
7.78467446276574));
#10681=CARTESIAN_POINT('Ctrl Pts',(-6.46245112202596,-2.01584035397194,
7.79342386588598));
#10682=CARTESIAN_POINT('Ctrl Pts',(-6.40220448416187,-2.19181813638306,
7.80217326900622));
#10683=CARTESIAN_POINT('Ctrl Pts',(-6.34195808575123,-2.36779521936116,
7.8109226373515));
#10684=CARTESIAN_POINT('Ctrl Pts',(-6.27445201489161,-2.54128677545009,
7.81967200569678));
#10685=CARTESIAN_POINT('Ctrl Pts',(-6.199915551361,-2.71170355238031,7.82842137404205));
#10686=CARTESIAN_POINT('Ctrl Pts',(-6.12537937788953,-2.88211966613253,
7.83717070833911));
#10687=CARTESIAN_POINT('Ctrl Pts',(-6.0438129813353,-3.04946076210617,7.84592004263616));
#10688=CARTESIAN_POINT('Ctrl Pts',(-5.95549339426218,-3.21315848207018,
7.85466937693321));
#10689=CARTESIAN_POINT('Ctrl Pts',(-5.86717414355068,-3.37685557859797,
7.86341867790878));
#10690=CARTESIAN_POINT('Ctrl Pts',(-5.77210188986141,-3.5369090746747,7.87216797888434));
#10691=CARTESIAN_POINT('Ctrl Pts',(-5.67059953466966,-3.69277536785061,
7.8809172798599));
#10692=CARTESIAN_POINT('Ctrl Pts',(-5.56909755761657,-3.8486410803595,7.88966654824066));
#10693=CARTESIAN_POINT('Ctrl Pts',(-5.46116568337954,-4.00031938104437,
7.89841581662143));
#10694=CARTESIAN_POINT('Ctrl Pts',(-5.34717048685992,-4.14729511663377,
7.90716508500219));
#10695=CARTESIAN_POINT('Ctrl Pts',(-5.23317570555387,-4.294270316882,7.91591432151482));
#10696=CARTESIAN_POINT('Ctrl Pts',(-5.11311782178666,-4.4365427598729,7.92466355802744));
#10697=CARTESIAN_POINT('Ctrl Pts',(-4.98740459171866,-4.57362924147811,
7.93341279454006));
#10698=CARTESIAN_POINT('Ctrl Pts',(-4.86169180910669,-4.71071523514602,
7.94216199991119));
#10699=CARTESIAN_POINT('Ctrl Pts',(-4.73032391415257,-4.84261509316694,
7.95091120528231));
#10700=CARTESIAN_POINT('Ctrl Pts',(-4.59374707237105,-4.96888084331697,
7.95966041065343));
#10701=CARTESIAN_POINT('Ctrl Pts',(-4.45717070537202,-5.095146154529,7.96840958560966));
#10702=CARTESIAN_POINT('Ctrl Pts',(-4.31538563819296,-5.21577720253809,
7.9771587605659));
#10703=CARTESIAN_POINT('Ctrl Pts',(-4.16887341290422,-5.33036429028827,
7.98590793552213));
#10704=CARTESIAN_POINT('Ctrl Pts',(-4.02236168477122,-5.44495098921336,
7.99465708079004));
#10705=CARTESIAN_POINT('Ctrl Pts',(-3.87112305634232,-5.55349359238902,
8.00340622605795));
#10706=CARTESIAN_POINT('Ctrl Pts',(-3.71567117316537,-5.65562346102602,
8.01215537132586));
#10707=CARTESIAN_POINT('Ctrl Pts',(-3.5602198045709,-5.757752991589,8.02090448763203));
#10708=CARTESIAN_POINT('Ctrl Pts',(-3.40055544862162,-5.85346967275485,
8.0296536039382));
#10709=CARTESIAN_POINT('Ctrl Pts',(-3.23722036323162,-5.94244842803693,
8.03840272024437));
#10710=CARTESIAN_POINT('Ctrl Pts',(-3.07388580495802,-6.031426896166,8.04715180831531));
#10711=CARTESIAN_POINT('Ctrl Pts',(-2.90688079257459,-6.1136673448494,8.05590089638626));
#10712=CARTESIAN_POINT('Ctrl Pts',(-2.73677251094364,-6.18889046787413,
8.0646499844572));
#10713=CARTESIAN_POINT('Ctrl Pts',(-2.56666476416375,-6.26411335438381,
8.07339904501944));
#10714=CARTESIAN_POINT('Ctrl Pts',(-2.39345402971805,-6.332318843504,8.08214810558168));
#10715=CARTESIAN_POINT('Ctrl Pts',(-2.21772856473731,-6.3932752962115,8.09089716614392));
#10716=CARTESIAN_POINT('Ctrl Pts',(-2.04200363767987,-6.4542315623217,8.09964619992391));
#10717=CARTESIAN_POINT('Ctrl Pts',(-1.86376426619836,-6.50793874252129,
8.10839523370389));
#10718=CARTESIAN_POINT('Ctrl Pts',(-1.68361578194457,-6.55421443796182,
8.11714426748388));
#10719=CARTESIAN_POINT('Ctrl Pts',(-1.50346783419658,-6.60048999558727,
8.1258932752081));
#10720=CARTESIAN_POINT('Ctrl Pts',(-1.32141106257057,-6.63933404145532,
8.13464228293232));
#10721=CARTESIAN_POINT('Ctrl Pts',(-1.13806375958877,-6.67061465527058,
8.14339129065653));
#10722=CARTESIAN_POINT('Ctrl Pts',(-0.954716987417111,-6.70189517852511,
8.15214027305143));
#10723=CARTESIAN_POINT('Ctrl Pts',(-0.77007997380747,-6.72561226535856,
8.16088925544634));
#10724=CARTESIAN_POINT('Ctrl Pts',(-0.584779770549684,-6.74168536939806,
8.16963823784124));
#10725=CARTESIAN_POINT('Ctrl Pts',(-0.391490647551172,-6.7584514394241,
8.17876441851729));
#10726=CARTESIAN_POINT('Ctrl Pts',(-0.197480213101632,-6.76689975924034,
8.18789059919334));
#10727=CARTESIAN_POINT('Ctrl Pts',(-0.00346532629513419,-6.76699911271708,
8.19701677986939));
#10728=CARTESIAN_POINT('Ctrl Pts',(0.184486595298659,-6.76709536139766,
8.20585776739931));
#10729=CARTESIAN_POINT('Ctrl Pts',(0.37244237818777,-6.75935659726756,8.21469875492924));
#10730=CARTESIAN_POINT('Ctrl Pts',(0.559750217724562,-6.74380965728996,
8.22353974245916));
#10731=CARTESIAN_POINT('Ctrl Pts',(0.745129914460219,-6.72842275717226,
8.23228972105693));
#10732=CARTESIAN_POINT('Ctrl Pts',(0.929874656316636,-6.70538772273439,
8.2410396996547));
#10733=CARTESIAN_POINT('Ctrl Pts',(1.11335688290021,-6.67478280180702,8.24978967825247));
#10734=CARTESIAN_POINT('Ctrl Pts',(1.29683723119098,-6.64417819417976,8.25853956727741));
#10735=CARTESIAN_POINT('Ctrl Pts',(1.47905480730475,-6.60600390230022,8.26728945630235));
#10736=CARTESIAN_POINT('Ctrl Pts',(1.65939064805045,-6.56038959797074,8.27603934532729));
#10737=CARTESIAN_POINT('Ctrl Pts',(1.83972470264504,-6.51477574543189,8.28478914768824));
#10738=CARTESIAN_POINT('Ctrl Pts',(2.01817678126087,-6.46172209820025,8.29353895004919));
#10739=CARTESIAN_POINT('Ctrl Pts',(2.1941407234792,-6.40140886723932,8.30228875241014));
#10740=CARTESIAN_POINT('Ctrl Pts',(2.37010298132331,-6.34109621361287,8.31103847101562));
#10741=CARTESIAN_POINT('Ctrl Pts',(2.54357687927141,-6.27352420825878,8.31978818962111));
#10742=CARTESIAN_POINT('Ctrl Pts',(2.71397317790192,-6.198922373254,8.3285379082266));
#10743=CARTESIAN_POINT('Ctrl Pts',(2.88436790207417,-6.12432122756862,8.33728754598486));
#10744=CARTESIAN_POINT('Ctrl Pts',(3.05168482126466,-6.04269049717311,8.34603718374313));
#10745=CARTESIAN_POINT('Ctrl Pts',(3.21535561997593,-5.95430745234819,8.35478682150139));
#10746=CARTESIAN_POINT('Ctrl Pts',(3.37902496075477,-5.86592519481403,8.3635363813204));
#10747=CARTESIAN_POINT('Ctrl Pts',(3.53904799385064,-5.77079087940116,8.37228594113941));
#10748=CARTESIAN_POINT('Ctrl Pts',(3.69488118815166,-5.66922763746906,8.38103550095842));
#10749=CARTESIAN_POINT('Ctrl Pts',(3.85071304611015,-5.56766526648926,8.38978498574586));
#10750=CARTESIAN_POINT('Ctrl Pts',(4.00235489706149,-5.45967423580581,8.3985344705333));
#10751=CARTESIAN_POINT('Ctrl Pts',(4.14929168607834,-5.34562133936189,8.40728395532074));
#10752=CARTESIAN_POINT('Ctrl Pts',(4.29622726385922,-5.23156938308395,8.41603336798403));
#10753=CARTESIAN_POINT('Ctrl Pts',(4.43845763092217,-5.11145583677071,8.42478278064733));
#10754=CARTESIAN_POINT('Ctrl Pts',(4.57549970661098,-4.98568866204087,8.43353219331062));
#10755=CARTESIAN_POINT('Ctrl Pts',(4.71254069815435,-4.85992248226026,8.44228153675695));
#10756=CARTESIAN_POINT('Ctrl Pts',(4.84439326931456,-4.72850295733857,8.45103088020328));
#10757=CARTESIAN_POINT('Ctrl Pts',(4.97060959434843,-4.59187644221525,8.45978022364961));
#10758=CARTESIAN_POINT('Ctrl Pts',(5.09682496280651,-4.45525096256508,8.4685295007859));
#10759=CARTESIAN_POINT('Ctrl Pts',(5.21740397615967,-4.31341878218171,8.4772787779222));
#10760=CARTESIAN_POINT('Ctrl Pts',(5.33193710452054,-4.16686161438524,8.48602805505849));
#10761=CARTESIAN_POINT('Ctrl Pts',(5.44646940289505,-4.02030550864349,8.49477726879145));
#10762=CARTESIAN_POINT('Ctrl Pts',(5.55495572749788,-3.86902470979958,8.50352648252442));
#10763=CARTESIAN_POINT('Ctrl Pts',(5.65702762491579,-3.71353301465594,8.51227569625739));
#10764=CARTESIAN_POINT('Ctrl Pts',(5.75909881655262,-3.55804239466717,8.5210248494935));
#10765=CARTESIAN_POINT('Ctrl Pts',(5.85475551250876,-3.3983411761939,8.5297740027296));
#10766=CARTESIAN_POINT('Ctrl Pts',(5.94367283728176,-3.2349717469182,8.53852315596571));
#10767=CARTESIAN_POINT('Ctrl Pts',(6.03258957676395,-3.07160339300803,8.54727225161125));
#10768=CARTESIAN_POINT('Ctrl Pts',(6.11476689685369,-2.90456712829327,8.55602134725679));
#10769=CARTESIAN_POINT('Ctrl Pts',(6.18992570525345,-2.73443024475713,8.56477044290233));
#10770=CARTESIAN_POINT('Ctrl Pts',(6.26508404388786,-2.56429442462816,8.57351948386337));
#10771=CARTESIAN_POINT('Ctrl Pts',(6.33322384283405,-2.39105828655755,8.5822685248244));
#10772=CARTESIAN_POINT('Ctrl Pts',(6.39411368720123,-2.2153101713182,8.59101756578544));
#10773=CARTESIAN_POINT('Ctrl Pts',(6.4550031712098,-2.03956309619233,8.59976655496786));
#10774=CARTESIAN_POINT('Ctrl Pts',(6.50864269270161,-1.86130434438329,8.60851554415027));
#10775=CARTESIAN_POINT('Ctrl Pts',(6.55485008446417,-1.68113930719619,8.61726453333269));
#10776=CARTESIAN_POINT('Ctrl Pts',(6.60199664749477,-1.49731239211518,8.62619134686205));
#10777=CARTESIAN_POINT('Ctrl Pts',(6.64140563640969,-1.31150116499353,8.63511816039141));
#10778=CARTESIAN_POINT('Ctrl Pts',(6.67293772282225,-1.12436255155346,8.64404497392078));
#10779=CARTESIAN_POINT('Ctrl Pts',(6.70384494949915,-0.940932395048195,
8.65279488807631));
#10780=CARTESIAN_POINT('Ctrl Pts',(6.72718449348966,-0.756227260503556,
8.66154480223183));
#10781=CARTESIAN_POINT('Ctrl Pts',(6.74287707373959,-0.570874564538526,
8.67029471638736));
#10782=CARTESIAN_POINT('Ctrl Pts',(6.75856934538688,-0.385525513629339,
8.67904445847133));
#10783=CARTESIAN_POINT('Ctrl Pts',(6.76661493004112,-0.199529212415126,
8.68779420055531));
#10784=CARTESIAN_POINT('Ctrl Pts',(6.76698649908907,-0.0135174385973606,
8.69654394263929));
#10785=CARTESIAN_POINT('Ctrl Pts',(6.76735806132382,0.172490924448839,8.70529352428518));
#10786=CARTESIAN_POINT('Ctrl Pts',(6.76005588896273,0.358514472904459,8.71404310593108));
#10787=CARTESIAN_POINT('Ctrl Pts',(6.7451047845456,0.543921359665251,8.72279268757698));
#10788=CARTESIAN_POINT('Ctrl Pts',(6.73015393440655,0.729325093153482,8.73154212041602));
#10789=CARTESIAN_POINT('Ctrl Pts',(6.70755443556856,0.914111900259384,8.74029155325507));
#10790=CARTESIAN_POINT('Ctrl Pts',(6.67738304682269,1.0976541559184,8.74904098609411));
#10791=CARTESIAN_POINT('Ctrl Pts',(6.64721213111802,1.28119353391578,8.75779028175544));
#10792=CARTESIAN_POINT('Ctrl Pts',(6.60946960955426,1.46348811672961,8.76653957741676));
#10793=CARTESIAN_POINT('Ctrl Pts',(6.56428366991105,1.64391876348532,8.77528887307809));
#10794=CARTESIAN_POINT('Ctrl Pts',(6.51909837867631,1.82434682110027,8.78403804318892));
#10795=CARTESIAN_POINT('Ctrl Pts',(6.46646995271825,2.00291071820757,8.79278721329975));
#10796=CARTESIAN_POINT('Ctrl Pts',(6.40657713281443,2.17900400213016,8.80153638341057));
#10797=CARTESIAN_POINT('Ctrl Pts',(6.34668509278943,2.35509499309974,8.81028543959635));
#10798=CARTESIAN_POINT('Ctrl Pts',(6.27952894037398,2.52871516398441,8.81903449578213));
#10799=CARTESIAN_POINT('Ctrl Pts',(6.20533675061307,2.69927486771741,8.82778355196791));
#10800=CARTESIAN_POINT('Ctrl Pts',(6.12832117907775,2.87632521636224,8.83686555325017));
#10801=CARTESIAN_POINT('Ctrl Pts',(6.04372366625938,3.05007728920277,8.84594755453243));
#10802=CARTESIAN_POINT('Ctrl Pts',(5.95185378007727,3.21989527478455,8.8550295558147));
#10803=CARTESIAN_POINT('Ctrl Pts',(5.86334450817224,3.38350129287006,8.86377933612182));
#10804=CARTESIAN_POINT('Ctrl Pts',(5.76808562057103,3.5434556712521,8.87252911642894));
#10805=CARTESIAN_POINT('Ctrl Pts',(5.66640068804326,3.69921508465552,8.88127889673606));
#10806=CARTESIAN_POINT('Ctrl Pts',(5.56471941107758,3.85496889852522,8.89002836248954));
#10807=CARTESIAN_POINT('Ctrl Pts',(5.45661270814941,4.00652780919872,8.89877782824303));
#10808=CARTESIAN_POINT('Ctrl Pts',(5.34244776448935,4.1533770456946,8.90752729399651));
#10809=CARTESIAN_POINT('Ctrl Pts',(5.22828631819409,4.30022178356475,8.91627649171611));
#10810=CARTESIAN_POINT('Ctrl Pts',(5.10806717843877,4.442356909729,8.92502568943571));
#10811=CARTESIAN_POINT('Ctrl Pts',(4.98219864544521,4.5792996907086,8.9337748871553));
#10812=CARTESIAN_POINT('Ctrl Pts',(4.85633329943815,4.71623900430217,8.94252386334555));
#10813=CARTESIAN_POINT('Ctrl Pts',(4.72481904033426,4.84798602483834,8.95127283953579));
#10814=CARTESIAN_POINT('Ctrl Pts',(4.58810250736964,4.97409332259342,8.96002181572603));
#10815=CARTESIAN_POINT('Ctrl Pts',(4.451377086854,5.10020881822347,8.9687713606622));
#10816=CARTESIAN_POINT('Ctrl Pts',(4.30944892635802,5.22068366308139,8.97752090559838));
#10817=CARTESIAN_POINT('Ctrl Pts',(4.16280009466404,5.33510865605051,8.98627045053456));
#10818=CARTESIAN_POINT('Ctrl Pts',(4.01615988348527,5.44952692273084,8.99501948114284));
#10819=CARTESIAN_POINT('Ctrl Pts',(3.86479978231965,5.55789587288811,9.00376851175112));
#10820=CARTESIAN_POINT('Ctrl Pts',(3.70923383580798,5.65984746714055,9.0125175423594));
#10821=CARTESIAN_POINT('Ctrl Pts',(3.55366577799268,5.76180044505551,9.02126669170742));
#10822=CARTESIAN_POINT('Ctrl Pts',(3.39389200026565,5.85733573571219,9.03001584105543));
#10823=CARTESIAN_POINT('Ctrl Pts',(3.23045513625763,5.94612887622079,9.03876499040345));
#10824=CARTESIAN_POINT('Ctrl Pts',(3.18695122151392,5.96976399206787,9.04109385451637));
#10825=CARTESIAN_POINT('Ctrl Pts',(3.1431879126257,5.99292165435381,9.04342271862929));
#10826=CARTESIAN_POINT('Ctrl Pts',(3.09917575053258,6.01559628526639,9.04575158274221));
#10827=CARTESIAN_POINT('Ctrl Pts',(3.09917575053257,6.0155962852664,7.04594397030302));
#10828=CARTESIAN_POINT('Ctrl Pts',(2.94415309791935,6.09546242371369,7.05414709647275));
#10829=CARTESIAN_POINT('Ctrl Pts',(2.78591898524294,6.16939525231196,7.06235022264247));
#10830=CARTESIAN_POINT('Ctrl Pts',(2.62496877406909,6.23713299001731,7.0705533488122));
#10831=CARTESIAN_POINT('Ctrl Pts',(2.46410949560556,6.30483245765121,7.07875184042761));
#10832=CARTESIAN_POINT('Ctrl Pts',(2.30053750533951,6.36634366800712,7.08695033204302));
#10833=CARTESIAN_POINT('Ctrl Pts',(2.13477077043363,6.42145176402519,7.09514882365843));
#10834=CARTESIAN_POINT('Ctrl Pts',(1.96615218344512,6.47750794011788,7.10348836218172));
#10835=CARTESIAN_POINT('Ctrl Pts',(1.79526298420467,6.52693850177259,7.11182790070501));
#10836=CARTESIAN_POINT('Ctrl Pts',(1.6226680115254,6.56956905164808,7.12016743922831));
#10837=CARTESIAN_POINT('Ctrl Pts',(1.45305240438134,6.61146370528584,7.12836301913409));
#10838=CARTESIAN_POINT('Ctrl Pts',(1.28178980116446,6.64679113915501,7.13655859903987));
#10839=CARTESIAN_POINT('Ctrl Pts',(1.10942978191014,6.67543665680462,7.14475417894565));
#10840=CARTESIAN_POINT('Ctrl Pts',(0.937056999630132,6.70408429561597,7.15295036572302));
#10841=CARTESIAN_POINT('Ctrl Pts',(0.763586993430932,6.72604897339413,7.16114655250038));
#10842=CARTESIAN_POINT('Ctrl Pts',(0.589577551380603,6.74126748548877,7.16934273927774));
#10843=CARTESIAN_POINT('Ctrl Pts',(0.415523565114005,6.75648989333002,7.17754102417525));
#10844=CARTESIAN_POINT('Ctrl Pts',(0.240930225363941,6.76496266437051,7.18573930907276));
#10845=CARTESIAN_POINT('Ctrl Pts',(0.0663584836826785,6.76667463024811,
7.19393759397027));
#10846=CARTESIAN_POINT('Ctrl Pts',(-0.113502496237864,6.76843846589167,
7.20238427349086));
#10847=CARTESIAN_POINT('Ctrl Pts',(-0.293340137794372,6.76302535317051,
7.21083095301146));
#10848=CARTESIAN_POINT('Ctrl Pts',(-0.472543928585516,6.7504808151388,7.21927763253206));
#10849=CARTESIAN_POINT('Ctrl Pts',(-0.646748104996574,6.7382862577211,7.22748865777208));
#10850=CARTESIAN_POINT('Ctrl Pts',(-0.820352974813139,6.71935296395488,
7.2356996830121));
#10851=CARTESIAN_POINT('Ctrl Pts',(-0.992805957653864,6.6937751180068,7.24391070825212));
#10852=CARTESIAN_POINT('Ctrl Pts',(-1.17268297386735,6.66709615580783,7.252475214913));
#10853=CARTESIAN_POINT('Ctrl Pts',(-1.3513062867024,6.63318795858461,7.26103972157388));
#10854=CARTESIAN_POINT('Ctrl Pts',(-1.52806445370092,6.59221571441164,7.26960422823477));
#10855=CARTESIAN_POINT('Ctrl Pts',(-1.70482262069945,6.55124347023866,7.27816873489565));
#10856=CARTESIAN_POINT('Ctrl Pts',(-1.87971523837467,6.50320735711522,7.28673324155653));
#10857=CARTESIAN_POINT('Ctrl Pts',(-2.05215294173931,6.44832980729977,7.29529774821742));
#10858=CARTESIAN_POINT('Ctrl Pts',(-2.21626474669054,6.3961019384765,7.30344873039364));
#10859=CARTESIAN_POINT('Ctrl Pts',(-2.378639230899,6.3375228963036,7.31159971256987));
#10860=CARTESIAN_POINT('Ctrl Pts',(-2.53874301684855,6.27272451925021,7.31975069474609));
#10861=CARTESIAN_POINT('Ctrl Pts',(-2.69866082741191,6.20800141151743,7.32789220880107));
#10862=CARTESIAN_POINT('Ctrl Pts',(-2.85631285459867,6.13707348528331,7.33603372285604));
#10863=CARTESIAN_POINT('Ctrl Pts',(-3.01117945953484,6.06012271018298,7.34417523691102));
#10864=CARTESIAN_POINT('Ctrl Pts',(-3.16589876216972,5.98324512727449,7.35230900711601));
#10865=CARTESIAN_POINT('Ctrl Pts',(-3.31783759181699,5.90035626204422,7.360442777321));
#10866=CARTESIAN_POINT('Ctrl Pts',(-3.466494937956,5.81168666095527,7.36857654752598));
#10867=CARTESIAN_POINT('Ctrl Pts',(-3.61504215346738,5.72308274944759,7.3767042919459));
#10868=CARTESIAN_POINT('Ctrl Pts',(-3.76031241329552,5.62870681590016,7.38483203636581));
#10869=CARTESIAN_POINT('Ctrl Pts',(-3.90182804519759,5.52883594490825,7.39295978078573));
#10870=CARTESIAN_POINT('Ctrl Pts',(-4.04326858990214,5.42901806469706,7.4010832126817));
#10871=CARTESIAN_POINT('Ctrl Pts',(-4.18095817601844,5.32371126386678,7.40920664457768));
#10872=CARTESIAN_POINT('Ctrl Pts',(-4.31444695146456,5.213236662861,7.41733007647365));
#10873=CARTESIAN_POINT('Ctrl Pts',(-4.44878252714567,5.10206125448188,7.42550504022326));
#10874=CARTESIAN_POINT('Ctrl Pts',(-4.57886349229339,4.98565245184027,7.43368000397286));
#10875=CARTESIAN_POINT('Ctrl Pts',(-4.70426372759376,4.86437989688775,7.44185496772247));
#10876=CARTESIAN_POINT('Ctrl Pts',(-4.82884522113193,4.74389913395309,7.44997655689738));
#10877=CARTESIAN_POINT('Ctrl Pts',(-4.94880667653275,4.61861821717317,7.45809814607229));
#10878=CARTESIAN_POINT('Ctrl Pts',(-5.06376621136556,4.48893759776548,7.4662197352472));
#10879=CARTESIAN_POINT('Ctrl Pts',(-5.17874092321446,4.35923985785665,7.47434239663843));
#10880=CARTESIAN_POINT('Ctrl Pts',(-5.28871215637903,4.22514153226331,7.48246505802966));
#10881=CARTESIAN_POINT('Ctrl Pts',(-5.39333750674595,4.08707713877869,7.49058771942089));
#10882=CARTESIAN_POINT('Ctrl Pts',(-5.49799659356594,3.94896822641872,7.49871299996498));
#10883=CARTESIAN_POINT('Ctrl Pts',(-5.59730614408126,3.80689099110871,7.50683828050906));
#10884=CARTESIAN_POINT('Ctrl Pts',(-5.69096640168317,3.66130993155637,7.51496356105314));
#10885=CARTESIAN_POINT('Ctrl Pts',(-5.78564706829542,3.51414279666423,7.5231773648374));
#10886=CARTESIAN_POINT('Ctrl Pts',(-5.8745544172481,3.36339536639403,7.53139116862166));
#10887=CARTESIAN_POINT('Ctrl Pts',(-5.9574263274126,3.20957326656539,7.53960497240592));
#10888=CARTESIAN_POINT('Ctrl Pts',(-6.03954695532302,3.05714565388755,7.54774431326288));
#10889=CARTESIAN_POINT('Ctrl Pts',(-6.11574102122482,2.90169924571963,7.55588365411985));
#10890=CARTESIAN_POINT('Ctrl Pts',(-6.18580201378812,2.74374606081081,7.56402299497681));
#10891=CARTESIAN_POINT('Ctrl Pts',(-6.25682443799939,2.58362531895894,7.57227403022472));
#10892=CARTESIAN_POINT('Ctrl Pts',(-6.32154409751292,2.42092886630554,7.58052506547263));
#10893=CARTESIAN_POINT('Ctrl Pts',(-6.37979827012356,2.25620544998198,7.58877610072053));
#10894=CARTESIAN_POINT('Ctrl Pts',(-6.43805244273421,2.09148203365842,7.59702713596844));
#10895=CARTESIAN_POINT('Ctrl Pts',(-6.48984107863011,1.9247320401606,7.60527817121635));
#10896=CARTESIAN_POINT('Ctrl Pts',(-6.53505529828139,1.75651394768285,7.61352920646426));
#10897=CARTESIAN_POINT('Ctrl Pts',(-6.59561712467624,1.53119556351781,7.62458098991017));
#10898=CARTESIAN_POINT('Ctrl Pts',(-6.64454081796998,1.30267368207627,7.63563277335607));
#10899=CARTESIAN_POINT('Ctrl Pts',(-6.68155380170293,1.07197378463705,7.64668455680198));
#10900=CARTESIAN_POINT('Ctrl Pts',(-6.71759850281841,0.847309139642104,
7.65744721873637));
#10901=CARTESIAN_POINT('Ctrl Pts',(-6.74234764100618,0.620578598254374,
7.66820988067075));
#10902=CARTESIAN_POINT('Ctrl Pts',(-6.75559287276856,0.392751750344489,
7.67897254260514));
#10903=CARTESIAN_POINT('Ctrl Pts',(-6.76306187783386,0.264279866154085,
7.68504162300676));
#10904=CARTESIAN_POINT('Ctrl Pts',(-6.76687359068,0.135459811375129,7.69111070340839));
#10905=CARTESIAN_POINT('Ctrl Pts',(-6.76699690759725,0.00646935617321545,
7.69717978381002));
#10906=CARTESIAN_POINT('',(-6.76699976915238,-0.00176756656877366,7.30282021615314));
#10907=CARTESIAN_POINT('Ctrl Pts',(3.0991757505326,6.01559628526638,6.65133473543275));
#10908=CARTESIAN_POINT('Ctrl Pts',(2.9577462882066,6.08845934642711,6.65884513280887));
#10909=CARTESIAN_POINT('Ctrl Pts',(2.81385032318343,6.15627895275546,6.66635553018499));
#10910=CARTESIAN_POINT('Ctrl Pts',(2.66786098159252,6.21890720166302,6.67386592756111));
#10911=CARTESIAN_POINT('Ctrl Pts',(2.50796169101893,6.28750270638314,6.68209191994713));
#10912=CARTESIAN_POINT('Ctrl Pts',(2.34520526418079,6.35001733527718,6.69031791233315));
#10913=CARTESIAN_POINT('Ctrl Pts',(2.18009410799565,6.40620626270203,6.69854390471918));
#10914=CARTESIAN_POINT('Ctrl Pts',(2.01515604956891,6.46233628328128,6.70676127321281));
#10915=CARTESIAN_POINT('Ctrl Pts',(1.84786851415233,6.51215369404529,6.71497864170645));
#10916=CARTESIAN_POINT('Ctrl Pts',(1.67875537281941,6.55546103628341,6.72319601020009));
#10917=CARTESIAN_POINT('Ctrl Pts',(1.50978568599895,6.59873164196979,6.73140640810243));
#10918=CARTESIAN_POINT('Ctrl Pts',(1.33899382267921,6.63550308920923,6.73961680600477));
#10919=CARTESIAN_POINT('Ctrl Pts',(1.1669204561316,6.66562717597239,6.74782720390712));
#10920=CARTESIAN_POINT('Ctrl Pts',(0.994958633739034,6.6957317352173,6.75603227953376));
#10921=CARTESIAN_POINT('Ctrl Pts',(0.821717314504548,6.71919745575553,6.76423735516041));
#10922=CARTESIAN_POINT('Ctrl Pts',(0.647749147972829,6.73592681383197,6.77244243078706));
#10923=CARTESIAN_POINT('Ctrl Pts',(0.47385896046791,6.75264867318558,6.7806438285925));
#10924=CARTESIAN_POINT('Ctrl Pts',(0.299242930652763,6.76264015156045,6.78884522639794));
#10925=CARTESIAN_POINT('Ctrl Pts',(0.124460741667302,6.76585534310213,6.79704662420338));
#10926=CARTESIAN_POINT('Ctrl Pts',(-0.0503077568719296,6.76907028280232,
6.80524737960472));
#10927=CARTESIAN_POINT('Ctrl Pts',(-0.225242030875551,6.76550997761102,
6.81344813500605));
#10928=CARTESIAN_POINT('Ctrl Pts',(-0.399780088322315,6.75518059573399,
6.82164889040739));
#10929=CARTESIAN_POINT('Ctrl Pts',(-0.57431725916889,6.74485126632707,6.82984960415138));
#10930=CARTESIAN_POINT('Ctrl Pts',(-0.748457859656909,6.72775294883227,
6.83805031789538));
#10931=CARTESIAN_POINT('Ctrl Pts',(-0.921642836535204,6.70394387520237,
6.84625103163937));
#10932=CARTESIAN_POINT('Ctrl Pts',(-1.09485831912054,6.6801306077178,6.85445318989995));
#10933=CARTESIAN_POINT('Ctrl Pts',(-1.2671174876918,6.64960427784065,6.86265534816053));
#10934=CARTESIAN_POINT('Ctrl Pts',(-1.43786926684679,6.61247464807673,6.87085750642111));
#10935=CARTESIAN_POINT('Ctrl Pts',(-1.60868206791768,6.57533174922036,6.87906259590392));
#10936=CARTESIAN_POINT('Ctrl Pts',(-1.77798605648574,6.53158092564861,6.88726768538673));
#10937=CARTESIAN_POINT('Ctrl Pts',(-1.94524309557896,6.48138243734332,6.89547277486954));
#10938=CARTESIAN_POINT('Ctrl Pts',(-2.1126912060525,6.43112660320373,6.90368723769641));
#10939=CARTESIAN_POINT('Ctrl Pts',(-2.27808735174958,6.37440849209118,6.91190170052328));
#10940=CARTESIAN_POINT('Ctrl Pts',(-2.44091022994374,6.31143773235196,6.92011616335015));
#10941=CARTESIAN_POINT('Ctrl Pts',(-2.60382957553541,6.24842966443234,6.92833549298602));
#10942=CARTESIAN_POINT('Ctrl Pts',(-2.7641722861174,6.1791617052847,6.9365548226219));
#10943=CARTESIAN_POINT('Ctrl Pts',(-2.92143973013384,6.10389047273913,6.94477415225778));
#10944=CARTESIAN_POINT('Ctrl Pts',(-3.07895085053445,6.02850261197535,6.95300621724736));
#10945=CARTESIAN_POINT('Ctrl Pts',(-3.23337686536588,5.9470930563785,6.96123828223694));
#10946=CARTESIAN_POINT('Ctrl Pts',(-3.38424514690154,5.85996363347704,6.96947034722653));
#10947=CARTESIAN_POINT('Ctrl Pts',(-3.519856430504,5.78164542928634,6.97686992047395));
#10948=CARTESIAN_POINT('Ctrl Pts',(-3.65259340203968,5.69870643024907,6.98426949372138));
#10949=CARTESIAN_POINT('Ctrl Pts',(-3.7821351902108,5.61139398037325,6.9916690669688));
#10950=CARTESIAN_POINT('Ctrl Pts',(-3.92441161092521,5.51549826187561,6.99979605680985));
#10951=CARTESIAN_POINT('Ctrl Pts',(-4.06327781887667,5.41402657110997,7.0079230466509));
#10952=CARTESIAN_POINT('Ctrl Pts',(-4.19825979227066,5.30725010872896,7.01605003649194));
#10953=CARTESIAN_POINT('Ctrl Pts',(-4.33307753009959,5.20060356364129,7.02416713804395));
#10954=CARTESIAN_POINT('Ctrl Pts',(-4.46402015411438,5.08866531908903,7.03228423959595));
#10955=CARTESIAN_POINT('Ctrl Pts',(-4.59064053134282,4.97175105088666,7.04040134114795));
#10956=CARTESIAN_POINT('Ctrl Pts',(-4.71713389446909,4.85495406049637,7.04851030035834));
#10957=CARTESIAN_POINT('Ctrl Pts',(-4.83931337293362,4.73319123036887,7.05661925956874));
#10958=CARTESIAN_POINT('Ctrl Pts',(-4.95676303128499,4.60681986316879,7.06472821877914));
#10959=CARTESIAN_POINT('Ctrl Pts',(-5.07411994308032,4.48054828773697,7.07283077458189));
#10960=CARTESIAN_POINT('Ctrl Pts',(-5.18675422130604,4.34967568903663,7.08093333038464));
#10961=CARTESIAN_POINT('Ctrl Pts',(-5.29428512757639,4.21459772551586,7.08903588618739));
#10962=CARTESIAN_POINT('Ctrl Pts',(-5.40175405835308,4.07959761424951,7.0971337720779));
#10963=CARTESIAN_POINT('Ctrl Pts',(-5.50412524544081,3.94039725193013,7.10523165796841));
#10964=CARTESIAN_POINT('Ctrl Pts',(-5.60105679618804,3.79742699283025,7.11332954385892));
#10965=CARTESIAN_POINT('Ctrl Pts',(-5.69796499854406,3.65449117169732,7.12142547917084));
#10966=CARTESIAN_POINT('Ctrl Pts',(-5.78943596202585,3.50778756300871,7.12952141448275));
#10967=CARTESIAN_POINT('Ctrl Pts',(-5.87516979223443,3.35777737683964,7.13761734979467));
#10968=CARTESIAN_POINT('Ctrl Pts',(-5.96089526601023,3.20778181208704,7.14571249599989));
#10969=CARTESIAN_POINT('Ctrl Pts',(-6.04088453607234,3.05448063083582,7.15380764220512));
#10970=CARTESIAN_POINT('Ctrl Pts',(-6.1148826341711,2.89836149752109,7.16190278841034));
#10971=CARTESIAN_POINT('Ctrl Pts',(-6.18888781242569,2.74222742669011,7.16999870916111));
#10972=CARTESIAN_POINT('Ctrl Pts',(-6.25690051941951,2.58327519992421,7.17809462991187));
#10973=CARTESIAN_POINT('Ctrl Pts',(-6.31871312917002,2.42201432515468,7.18619055066263));
#10974=CARTESIAN_POINT('Ctrl Pts',(-6.38054359334956,2.26070687055528,7.19428880990133));
#10975=CARTESIAN_POINT('Ctrl Pts',(-6.43617026313767,2.09708978429863,7.20238706914003));
#10976=CARTESIAN_POINT('Ctrl Pts',(-6.48543478515187,1.93168958363971,7.21048532837874));
#10977=CARTESIAN_POINT('Ctrl Pts',(-6.53475099061234,1.76611586150863,7.21859208350716));
#10978=CARTESIAN_POINT('Ctrl Pts',(-6.57769161173451,1.59875564208336,7.2266988386356));
#10979=CARTESIAN_POINT('Ctrl Pts',(-6.61414882311636,1.43014836491482,7.23480559376402));
#10980=CARTESIAN_POINT('Ctrl Pts',(-6.65062624168162,1.26144763358326,7.24291684223359));
#10981=CARTESIAN_POINT('Ctrl Pts',(-6.68061302708018,1.09149882952185,7.25102809070316));
#10982=CARTESIAN_POINT('Ctrl Pts',(-6.70405308758127,0.920848086761328,
7.25913933917273));
#10983=CARTESIAN_POINT('Ctrl Pts',(-6.72752745630857,0.749947569718673,
7.26726245973398));
#10984=CARTESIAN_POINT('Ctrl Pts',(-6.74443592206768,0.578343427576287,
7.27538558029523));
#10985=CARTESIAN_POINT('Ctrl Pts',(-6.75477446505585,0.406584463831959,
7.28350870085649));
#10986=CARTESIAN_POINT('Ctrl Pts',(-6.76296724965365,0.270473969895757,
7.28994587262204));
#10987=CARTESIAN_POINT('Ctrl Pts',(-6.76703530173109,0.134266321004993,
7.29638304438759));
#10988=CARTESIAN_POINT('Ctrl Pts',(-6.76699976915239,-0.00176756656875029,
7.30282021615314));
#10989=CARTESIAN_POINT('Ctrl Pts',(-6.76699976915218,-0.00176756734519897,
7.30282021618988));
#10990=CARTESIAN_POINT('Ctrl Pts',(-6.76698752969479,-0.0486254172486542,
7.30503754625208));
#10991=CARTESIAN_POINT('Ctrl Pts',(-6.76648859969451,-0.0954783083698461,
7.30725487631427));
#10992=CARTESIAN_POINT('Ctrl Pts',(-6.76550324311227,-0.142319596111774,
7.30947220637647));
#10993=CARTESIAN_POINT('Ctrl Pts',(-6.76184760804056,-0.316098974419329,
7.3176984157376));
#10994=CARTESIAN_POINT('Ctrl Pts',(-6.75148698982309,-0.489980337408581,
7.32592462509874));
#10995=CARTESIAN_POINT('Ctrl Pts',(-6.73440283697741,-0.663405931018561,
7.33415083445988));
#10996=CARTESIAN_POINT('Ctrl Pts',(-6.71733787744475,-0.836636688412039,
7.34236780202761));
#10997=CARTESIAN_POINT('Ctrl Pts',(-6.69356445939919,-1.00941234236451,
7.35058476959534));
#10998=CARTESIAN_POINT('Ctrl Pts',(-6.66311601983172,-1.1811747991986,7.35880173716306));
#10999=CARTESIAN_POINT('Ctrl Pts',(-6.63269567653462,-1.35277876237934,
7.36701112253132));
#11000=CARTESIAN_POINT('Ctrl Pts',(-6.59561264053686,-1.52337103947165,
7.37522050789958));
#11001=CARTESIAN_POINT('Ctrl Pts',(-6.55195216944722,-1.69239823010894,
7.38342989326784));
#11002=CARTESIAN_POINT('Ctrl Pts',(-6.50832322582457,-1.8613033652796,7.39163335059364));
#11003=CARTESIAN_POINT('Ctrl Pts',(-6.45812639683201,-2.02864531924276,
7.39983680791945));
#11004=CARTESIAN_POINT('Ctrl Pts',(-6.40149809730226,-2.19388037737602,
7.40804026524525));
#11005=CARTESIAN_POINT('Ctrl Pts',(-6.34489932988242,-2.35902926410844,
7.41623944440262));
#11006=CARTESIAN_POINT('Ctrl Pts',(-6.2818758898107,-2.52207310548398,7.42443862356));
#11007=CARTESIAN_POINT('Ctrl Pts',(-6.21261419681645,-2.68248277562312,
7.43263780271737));
#11008=CARTESIAN_POINT('Ctrl Pts',(-6.14336555421465,-2.84286222113075,
7.44083543697307));
#11009=CARTESIAN_POINT('Ctrl Pts',(-6.06788113631693,-3.00060815266827,
7.44903307122876));
#11010=CARTESIAN_POINT('Ctrl Pts',(-5.98639583441627,-3.15521059735853,
7.45723070548445));
#11011=CARTESIAN_POINT('Ctrl Pts',(-5.90491641421171,-3.30980188267925,
7.46542774802615));
#11012=CARTESIAN_POINT('Ctrl Pts',(-5.81743713910388,-3.46124981532172,
7.47362479056785));
#11013=CARTESIAN_POINT('Ctrl Pts',(-5.72423925008868,-3.60906830189513,
7.48182183310955));
#11014=CARTESIAN_POINT('Ctrl Pts',(-5.6310311496367,-3.75690298453421,7.4900197737787));
#11015=CARTESIAN_POINT('Ctrl Pts',(-5.53210337829873,-3.90110712536116,
7.49821771444784));
#11016=CARTESIAN_POINT('Ctrl Pts',(-5.42778098858982,-4.04122290153649,
7.50641565511699));
#11017=CARTESIAN_POINT('Ctrl Pts',(-5.32342820807334,-4.18137949571457,
7.51461598397948));
#11018=CARTESIAN_POINT('Ctrl Pts',(-5.21367789301692,-4.31744506527575,
7.52281631284197));
#11019=CARTESIAN_POINT('Ctrl Pts',(-5.09889594358894,-4.44899417356916,
7.53101664170447));
#11020=CARTESIAN_POINT('Ctrl Pts',(-4.9839943883899,-4.58068035944843,7.53922551552252));
#11021=CARTESIAN_POINT('Ctrl Pts',(-4.8640509600376,-4.70784041102398,7.54743438934057));
#11022=CARTESIAN_POINT('Ctrl Pts',(-4.73946974533751,-4.83008442297134,
7.55564326315862));
#11023=CARTESIAN_POINT('Ctrl Pts',(-4.6148216692723,-4.95239404193286,7.56385654258879));
#11024=CARTESIAN_POINT('Ctrl Pts',(-4.4855311101498,-5.0697821206818,7.57206982201896));
#11025=CARTESIAN_POINT('Ctrl Pts',(-4.35203583918027,-5.181898595543,7.58028310144913));
#11026=CARTESIAN_POINT('Ctrl Pts',(-4.21834531039661,-5.29417905836909,
7.58850839409128));
#11027=CARTESIAN_POINT('Ctrl Pts',(-4.08043806266068,-5.40117228842603,
7.59673368673343));
#11028=CARTESIAN_POINT('Ctrl Pts',(-3.9387825246479,-5.50257041967919,7.60495897937558));
#11029=CARTESIAN_POINT('Ctrl Pts',(-3.8106721125475,-5.5942728448952,7.61239776817843));
#11030=CARTESIAN_POINT('Ctrl Pts',(-3.67949649292701,-5.68139948981056,
7.61983655698129));
#11031=CARTESIAN_POINT('Ctrl Pts',(-3.54561914823371,-5.76375518700079,
7.62727534578415));
#11032=CARTESIAN_POINT('Ctrl Pts',(-3.39757059137176,-5.85482841635341,
7.63550154678617));
#11033=CARTESIAN_POINT('Ctrl Pts',(-3.24580387325173,-5.94032108328819,
7.64372774778819));
#11034=CARTESIAN_POINT('Ctrl Pts',(-3.09077776091241,-6.01991543401145,
7.65195394879021));
#11035=CARTESIAN_POINT('Ctrl Pts',(-2.93592578774073,-6.09942037725506,
7.66017090938896));
#11036=CARTESIAN_POINT('Ctrl Pts',(-2.77782202702455,-6.17304003517207,
7.6683878699877));
#11037=CARTESIAN_POINT('Ctrl Pts',(-2.61695369561579,-6.24050016865658,
7.67660483058645));
#11038=CARTESIAN_POINT('Ctrl Pts',(-2.45623377832424,-6.30789806468224,
7.68481421037086));
#11039=CARTESIAN_POINT('Ctrl Pts',(-2.29275469849348,-6.36914761568798,
7.69302359015528));
#11040=CARTESIAN_POINT('Ctrl Pts',(-2.12702780144999,-6.4240206827079,7.70123296993969));
#11041=CARTESIAN_POINT('Ctrl Pts',(-1.96142054891306,-6.47885413478815,
7.70943642306276));
#11042=CARTESIAN_POINT('Ctrl Pts',(-1.79356905055117,-6.52732015984342,
7.71763987618583));
#11043=CARTESIAN_POINT('Ctrl Pts',(-1.62400422441038,-6.56923886604051,
7.7258433293089));
#11044=CARTESIAN_POINT('Ctrl Pts',(-1.45452779923989,-6.61113571832848,
7.7340425056416));
#11045=CARTESIAN_POINT('Ctrl Pts',(-1.28334017308492,-6.64649196595729,
7.7422416819743));
#11046=CARTESIAN_POINT('Ctrl Pts',(-1.11098709125494,-6.67517765179811,
7.750440858307));
#11047=CARTESIAN_POINT('Ctrl Pts',(-0.938666440261681,-6.70385793999367,
7.75863849184078));
#11048=CARTESIAN_POINT('Ctrl Pts',(-0.765181122795862,-6.72587010160438,
7.76683612537456));
#11049=CARTESIAN_POINT('Ctrl Pts',(-0.591087044441642,-6.74113529799642,
7.77503375890834));
#11050=CARTESIAN_POINT('Ctrl Pts',(-0.417005505135572,-6.75639939491951,
7.78323080201123));
#11051=CARTESIAN_POINT('Ctrl Pts',(-0.242315649492823,-6.76491746220367,
7.79142784511412));
#11052=CARTESIAN_POINT('Ctrl Pts',(-0.0675784208831055,-6.76666255675802,
7.79962488821701));
#11053=CARTESIAN_POINT('Ctrl Pts',(0.107177980555809,-6.76840784279074,
7.80782283073045));
#11054=CARTESIAN_POINT('Ctrl Pts',(0.281981406580633,-6.76337867192868,
7.81602077324388));
#11055=CARTESIAN_POINT('Ctrl Pts',(0.456270941966133,-6.75160024198096,
7.82421871575733));
#11056=CARTESIAN_POINT('Ctrl Pts',(0.630611278008756,-6.7398183789414,7.83241904774794));
#11057=CARTESIAN_POINT('Ctrl Pts',(0.804437067284309,-6.72128336251896,
7.84061937973855));
#11058=CARTESIAN_POINT('Ctrl Pts',(0.9771924877412,-6.69607226976398,7.84881971172917));
#11059=CARTESIAN_POINT('Ctrl Pts',(1.15012796603896,-6.67083490023624,7.85702859068213));
#11060=CARTESIAN_POINT('Ctrl Pts',(1.32199049130191,-6.63890760465673,7.86523746963509));
#11061=CARTESIAN_POINT('Ctrl Pts',(1.49223341972256,-6.60041880648972,7.87344634858804));
#11062=CARTESIAN_POINT('Ctrl Pts',(1.66256773849562,-6.56190934664318,7.88165963425761));
#11063=CARTESIAN_POINT('Ctrl Pts',(1.83128038098567,-6.51683145474681,7.88987291992717));
#11064=CARTESIAN_POINT('Ctrl Pts',(1.99783994387982,-6.46536345139531,7.89808620559674));
#11065=CARTESIAN_POINT('Ctrl Pts',(2.16464316288966,-6.41382015669721,7.90631150629113));
#11066=CARTESIAN_POINT('Ctrl Pts',(2.32928666954229,-6.3558681883647,7.91453680698553));
#11067=CARTESIAN_POINT('Ctrl Pts',(2.49125792102187,-6.29173449622168,7.92276210767992));
#11068=CARTESIAN_POINT('Ctrl Pts',(2.63774138419605,-6.23373330622382,7.93020090018388));
#11069=CARTESIAN_POINT('Ctrl Pts',(2.78203930985302,-6.17067676984828,7.93763969268784));
#11070=CARTESIAN_POINT('Ctrl Pts',(2.92379073791715,-6.10276467847728,7.94507848519181));
#11071=CARTESIAN_POINT('Ctrl Pts',(3.07914343599351,-6.02833631630432,7.95323104140731));
#11072=CARTESIAN_POINT('Ctrl Pts',(3.23189528432432,-5.94785565104467,7.96138359762281));
#11073=CARTESIAN_POINT('Ctrl Pts',(3.38153615325296,-5.86152729621241,7.96953615383832));
#11074=CARTESIAN_POINT('Ctrl Pts',(3.53100365962748,-5.77529895486039,7.97767926512091));
#11075=CARTESIAN_POINT('Ctrl Pts',(3.67736704758343,-5.68323659041015,7.9858223764035));
#11076=CARTESIAN_POINT('Ctrl Pts',(3.82013675003357,-5.58559255684149,7.99396548768609));
#11077=CARTESIAN_POINT('Ctrl Pts',(3.96277106589319,-5.48804111779786,8.00210087696567));
#11078=CARTESIAN_POINT('Ctrl Pts',(4.10181818116243,-5.38491875231458,8.01023626624525));
#11079=CARTESIAN_POINT('Ctrl Pts',(4.23681371614003,-5.27652333783598,8.01837165552482));
#11080=CARTESIAN_POINT('Ctrl Pts',(4.37170960248498,-5.16820793678033,8.02650103956565));
#11081=CARTESIAN_POINT('Ctrl Pts',(4.50255957975303,-5.05462746502777,8.03463042360648));
#11082=CARTESIAN_POINT('Ctrl Pts',(4.62892883536721,-4.93612265215381,8.0427598076473));
#11083=CARTESIAN_POINT('Ctrl Pts',(4.75523135353173,-4.81768042340244,8.05088489844168));
#11084=CARTESIAN_POINT('Ctrl Pts',(4.87705759663659,-4.69431928226894,8.05900998923605));
#11085=CARTESIAN_POINT('Ctrl Pts',(4.99400640904814,-4.56641971202672,8.06713508003043));
#11086=CARTESIAN_POINT('Ctrl Pts',(5.11140164037723,-4.43803192145523,8.07529118605414));
#11087=CARTESIAN_POINT('Ctrl Pts',(5.22388184578451,-4.30507122419482,8.08344729207785));
#11088=CARTESIAN_POINT('Ctrl Pts',(5.3310788343176,-4.16795962819831,8.09160339810156));
#11089=CARTESIAN_POINT('Ctrl Pts',(5.4378443744059,-4.0313998815183,8.09972667727717));
#11090=CARTESIAN_POINT('Ctrl Pts',(5.53936893675134,-3.89072289073989,8.10784995645278));
#11091=CARTESIAN_POINT('Ctrl Pts',(5.63532956659387,-3.74637820779923,8.11597323562839));
#11092=CARTESIAN_POINT('Ctrl Pts',(5.73130297440501,-3.6020143041445,8.12409759648726));
#11093=CARTESIAN_POINT('Ctrl Pts',(5.82171077145809,-3.45398204023489,8.13222195734612));
#11094=CARTESIAN_POINT('Ctrl Pts',(5.90627381256288,-3.30275924811875,8.14034631820498));
#11095=CARTESIAN_POINT('Ctrl Pts',(5.99086420250468,-3.15148754849598,8.14847330659259));
#11096=CARTESIAN_POINT('Ctrl Pts',(6.06960589391021,-2.99702358503507,8.1566002949802));
#11097=CARTESIAN_POINT('Ctrl Pts',(6.1422661238186,-2.83986898715247,8.1647272833678));
#11098=CARTESIAN_POINT('Ctrl Pts',(6.21539609378466,-2.68169840280844,8.17290681180378));
#11099=CARTESIAN_POINT('Ctrl Pts',(6.28236554001722,-2.52080261527084,8.18108634023975));
#11100=CARTESIAN_POINT('Ctrl Pts',(6.34298702717897,-2.35771172390504,8.18926586867573));
#11101=CARTESIAN_POINT('Ctrl Pts',(6.40332302826017,-2.19538888000113,8.19740687708154));
#11102=CARTESIAN_POINT('Ctrl Pts',(6.45737067781465,-2.03089192985121,8.20554788548735));
#11103=CARTESIAN_POINT('Ctrl Pts',(6.50499590511038,-1.86475662607675,8.21368889389316));
#11104=CARTESIAN_POINT('Ctrl Pts',(6.55295914799961,-1.69744219253233,8.22188768234421));
#11105=CARTESIAN_POINT('Ctrl Pts',(6.59440837850788,-1.52846643040878,8.23008647079526));
#11106=CARTESIAN_POINT('Ctrl Pts',(6.62925944593312,-1.35838440748798,8.23828525924632));
#11107=CARTESIAN_POINT('Ctrl Pts',(6.66411051335837,-1.18830238456717,8.24648404769737));
#11108=CARTESIAN_POINT('Ctrl Pts',(6.69236342114684,-1.01711447780827,8.25468283614843));
#11109=CARTESIAN_POINT('Ctrl Pts',(6.7139872728954,-0.845377962451505,8.26288162459949));
#11110=CARTESIAN_POINT('Ctrl Pts',(6.73570148794889,-0.672923782208495,
8.27111467473664));
#11111=CARTESIAN_POINT('Ctrl Pts',(6.75079874565138,-0.499380333445228,
8.27934772487379));
#11112=CARTESIAN_POINT('Ctrl Pts',(6.75917681953755,-0.325296360610221,
8.28758077501095));
#11113=CARTESIAN_POINT('Ctrl Pts',(6.76754491642563,-0.151419695026239,
8.295804020851));
#11114=CARTESIAN_POINT('Ctrl Pts',(6.76920974544321,0.0229958586427361,
8.30402726669104));
#11115=CARTESIAN_POINT('Ctrl Pts',(6.76412040581053,0.197393352718985,8.31225051253109));
#11116=CARTESIAN_POINT('Ctrl Pts',(6.7590361081567,0.371618072223139,8.32046561164983));
#11117=CARTESIAN_POINT('Ctrl Pts',(6.74721097806552,0.545824412197253,8.32868071076857));
#11118=CARTESIAN_POINT('Ctrl Pts',(6.72864603823996,0.719452216674408,8.3368958098873));
#11119=CARTESIAN_POINT('Ctrl Pts',(6.71009577612072,0.892942748531908,8.34510441403146));
#11120=CARTESIAN_POINT('Ctrl Pts',(6.68481635566108,1.06585530138931,8.35331301817561));
#11121=CARTESIAN_POINT('Ctrl Pts',(6.65286082587563,1.23763154110155,8.36152162231977));
#11122=CARTESIAN_POINT('Ctrl Pts',(6.62092416859118,1.40930633210439,8.36972537857403));
#11123=CARTESIAN_POINT('Ctrl Pts',(6.58231932194603,1.57984579567035,8.3779291348283));
#11124=CARTESIAN_POINT('Ctrl Pts',(6.53715096824298,1.74869843552281,8.38613289108256));
#11125=CARTESIAN_POINT('Ctrl Pts',(6.49199597871709,1.91750111613588,8.39433422005217));
#11126=CARTESIAN_POINT('Ctrl Pts',(6.44028143919269,2.08461762062783,8.40253554902176));
#11127=CARTESIAN_POINT('Ctrl Pts',(6.38216282693135,2.24950809079134,8.41073687799137));
#11128=CARTESIAN_POINT('Ctrl Pts',(6.32405222978137,2.41437582098516,8.41893707591942));
#11129=CARTESIAN_POINT('Ctrl Pts',(6.25953943719118,2.57701779021335,8.42713727384749));
#11130=CARTESIAN_POINT('Ctrl Pts',(6.18882935908951,2.73691069713129,8.43533747177554));
#11131=CARTESIAN_POINT('Ctrl Pts',(6.11811621847773,2.89681052913908,8.44353802486074));
#11132=CARTESIAN_POINT('Ctrl Pts',(6.04120540247875,3.05396073391649,8.45173857794594));
#11133=CARTESIAN_POINT('Ctrl Pts',(5.95834941791655,3.20785928837497,8.45993913103113));
#11134=CARTESIAN_POINT('Ctrl Pts',(5.87547482966789,3.36179239773577,8.4681415253897));
#11135=CARTESIAN_POINT('Ctrl Pts',(5.78665258397753,3.51247208723095,8.47634391974827));
#11136=CARTESIAN_POINT('Ctrl Pts',(5.69218048709079,3.65942212683681,8.48454631410685));
#11137=CARTESIAN_POINT('Ctrl Pts',(5.59762004218647,3.80650959056166,8.49275637914602));
#11138=CARTESIAN_POINT('Ctrl Pts',(5.49739938388745,3.94986013414001,8.50096644418519));
#11139=CARTESIAN_POINT('Ctrl Pts',(5.39185943326424,4.08902688324734,8.50917650922437));
#11140=CARTESIAN_POINT('Ctrl Pts',(5.28626897309297,4.22826023509192,8.51739050345502));
#11141=CARTESIAN_POINT('Ctrl Pts',(5.17535437212263,4.36330552350885,8.52560449768567));
#11142=CARTESIAN_POINT('Ctrl Pts',(5.05949592397364,4.49375010378795,8.53381849191632));
#11143=CARTESIAN_POINT('Ctrl Pts',(4.94347952217289,4.62437252347483,8.5420436845568));
#11144=CARTESIAN_POINT('Ctrl Pts',(4.82250605119118,4.7503814412255,8.55026887719728));
#11145=CARTESIAN_POINT('Ctrl Pts',(4.69699250535623,4.87140127731513,8.55849406983776));
#11146=CARTESIAN_POINT('Ctrl Pts',(4.58411844345555,4.98023415570383,8.56589096789422));
#11147=CARTESIAN_POINT('Ctrl Pts',(4.46757326273479,5.08503258278129,8.57328786595068));
#11148=CARTESIAN_POINT('Ctrl Pts',(4.34768164610651,5.18555236248836,8.58068476400715));
#11149=CARTESIAN_POINT('Ctrl Pts',(4.20753111020087,5.3030576676236,8.58933156731006));
#11150=CARTESIAN_POINT('Ctrl Pts',(4.06248921193366,5.41498253421157,8.59797837061297));
#11151=CARTESIAN_POINT('Ctrl Pts',(3.91301657326871,5.52092295701764,8.60662517391588));
#11152=CARTESIAN_POINT('Ctrl Pts',(3.76378560526331,5.62669209301107,8.61525799687647));
#11153=CARTESIAN_POINT('Ctrl Pts',(3.61013843570947,5.72649591228951,8.62389081983705));
#11154=CARTESIAN_POINT('Ctrl Pts',(3.45256820668289,5.81997094307201,8.63252364279763));
#11155=CARTESIAN_POINT('Ctrl Pts',(3.33681818514436,5.88863706669974,8.63886525599322));
#11156=CARTESIAN_POINT('Ctrl Pts',(3.21895191095766,5.95388879123284,8.6452068691888));
#11157=CARTESIAN_POINT('Ctrl Pts',(3.09917575053261,6.01559628526638,8.65154848238438));
#11158=CARTESIAN_POINT('Origin',(0.,0.,-3.69717978381041));
#11159=CARTESIAN_POINT('',(3.0991757505326,6.01559628526639,11.0455440641533));
#11160=CARTESIAN_POINT('',(3.09917575053259,6.01559628526639,10.6513920151221));
#11161=CARTESIAN_POINT('',(3.09917575053259,6.01559628526639,-3.69717978381041));
#11162=CARTESIAN_POINT('',(-6.767,1.72459919609014E-12,9.69717978381002));
#11163=CARTESIAN_POINT('Ctrl Pts',(-6.76699931536137,-0.00304399388113017,
9.69717978381003));
#11164=CARTESIAN_POINT('Ctrl Pts',(-6.76691563275954,-0.189075941186378,
9.70587829366268));
#11165=CARTESIAN_POINT('Ctrl Pts',(-6.75915646223125,-0.374883524766316,
9.71457680351534));
#11166=CARTESIAN_POINT('Ctrl Pts',(-6.74380218515861,-0.559840233861357,
9.72327531336799));
#11167=CARTESIAN_POINT('Ctrl Pts',(-6.72841643646549,-0.74517604822634,
9.73199165253293));
#11168=CARTESIAN_POINT('Ctrl Pts',(-6.70540450111108,-0.929657222362386,
9.74070799169786));
#11169=CARTESIAN_POINT('Ctrl Pts',(-6.67489790911547,-1.11266657309634,
9.7494243308628));
#11170=CARTESIAN_POINT('Ctrl Pts',(-6.64429394823896,-1.29626004072139,
9.75816849025067));
#11171=CARTESIAN_POINT('Ctrl Pts',(-6.60614751276337,-1.47837200472053,
9.76691264963853));
#11172=CARTESIAN_POINT('Ctrl Pts',(-6.5606409249368,-1.6583967119011,9.7756568090264));
#11173=CARTESIAN_POINT('Ctrl Pts',(-6.51505618434852,-1.83873059251602,
9.78441598558513));
#11174=CARTESIAN_POINT('Ctrl Pts',(-6.46208612285544,-2.01696978566612,
9.79317516214386));
#11175=CARTESIAN_POINT('Ctrl Pts',(-6.4019618448933,-2.19252674705018,9.8019343387026));
#11176=CARTESIAN_POINT('Ctrl Pts',(-6.34167561950224,-2.36855657895322,
9.81071710849473));
#11177=CARTESIAN_POINT('Ctrl Pts',(-6.27419673216841,-2.54188946277467,
9.81949987828687));
#11178=CARTESIAN_POINT('Ctrl Pts',(-6.19980411841009,-2.71195831334946,
9.828282648079));
#11179=CARTESIAN_POINT('Ctrl Pts',(-6.16347570173305,-2.79500865605606,
9.83257157011666));
#11180=CARTESIAN_POINT('Ctrl Pts',(-6.12549925121098,-2.87728103007024,
9.83686049215433));
#11181=CARTESIAN_POINT('Ctrl Pts',(-6.08591104570938,-2.9587118385731,9.84114941419199));
#11182=CARTESIAN_POINT('Ctrl Pts',(-6.00992899708752,-3.11500282404684,
9.84938118622287));
#11183=CARTESIAN_POINT('Ctrl Pts',(-5.9278110264455,-3.26859445189463,9.85761295825376));
#11184=CARTESIAN_POINT('Ctrl Pts',(-5.83977091139031,-3.41897129301777,
9.86584473028464));
#11185=CARTESIAN_POINT('Ctrl Pts',(-5.75183592503064,-3.56916856916496,
9.87406667275709));
#11186=CARTESIAN_POINT('Ctrl Pts',(-5.6579930547608,-3.71615839630879,9.88228861522954));
#11187=CARTESIAN_POINT('Ctrl Pts',(-5.55850356303743,-3.85944648099961,
9.89051055770199));
#11188=CARTESIAN_POINT('Ctrl Pts',(-5.4591129381152,-4.00259217442547,9.89872432969194));
#11189=CARTESIAN_POINT('Ctrl Pts',(-5.35408706952809,-4.14204315897073,
9.90693810168188));
#11190=CARTESIAN_POINT('Ctrl Pts',(-5.24373247890332,-4.27733079030538,
9.91515187367183));
#11191=CARTESIAN_POINT('Ctrl Pts',(-5.13346544969492,-4.41251107697453,
9.92335912840223));
#11192=CARTESIAN_POINT('Ctrl Pts',(-5.01787834537423,-4.54353431375377,
9.93156638313264));
#11193=CARTESIAN_POINT('Ctrl Pts',(-4.89732028676702,-4.66996177808986,
9.93977363786304));
#11194=CARTESIAN_POINT('Ctrl Pts',(-4.77683374576919,-4.79631424296002,
9.94797602387504));
#11195=CARTESIAN_POINT('Ctrl Pts',(-4.65138237160784,-4.91807610790113,
9.95617840988704));
#11196=CARTESIAN_POINT('Ctrl Pts',(-4.52135481620011,-5.03484256218842,
9.96438079589904));
#11197=CARTESIAN_POINT('Ctrl Pts',(-4.39136607086359,-5.15157416452151,
9.97258073369779));
#11198=CARTESIAN_POINT('Ctrl Pts',(-4.25680412872402,-5.26331308423868,
9.98078067149653));
#11199=CARTESIAN_POINT('Ctrl Pts',(-4.11809384882402,-5.36969198858536,
9.98898060929528));
#11200=CARTESIAN_POINT('Ctrl Pts',(-3.97940296420127,-5.47605601841556,
9.99717940053108));
#11201=CARTESIAN_POINT('Ctrl Pts',(-3.83656518087139,-5.57706130684962,
10.0053781917669));
#11202=CARTESIAN_POINT('Ctrl Pts',(-3.69003773789161,-5.67238137759934,
10.0135769830027));
#11203=CARTESIAN_POINT('Ctrl Pts',(-3.54350420239129,-5.7677054116987,10.0217761151391));
#11204=CARTESIAN_POINT('Ctrl Pts',(-3.39328100202644,-5.85734356164554,
10.0299752472756));
#11205=CARTESIAN_POINT('Ctrl Pts',(-3.23985363895098,-5.94101316259913,
10.0381743794121));
#11206=CARTESIAN_POINT('Ctrl Pts',(-3.0863920640432,-6.02470142052694,10.0463753398231));
#11207=CARTESIAN_POINT('Ctrl Pts',(-2.92972521800756,-6.10241830714088,
10.054576300234));
#11208=CARTESIAN_POINT('Ctrl Pts',(-2.77036247488132,-6.17392749858382,
10.062777260645));
#11209=CARTESIAN_POINT('Ctrl Pts',(-2.61085037050137,-6.24550371135356,
10.0709859073301));
#11210=CARTESIAN_POINT('Ctrl Pts',(-2.44863764827458,-6.31086045780384,
10.0791945540152));
#11211=CARTESIAN_POINT('Ctrl Pts',(-2.28425378236797,-6.36980954642583,
10.0874032007002));
#11212=CARTESIAN_POINT('Ctrl Pts',(-2.11979143498689,-6.42878677899837,
10.0956157664238));
#11213=CARTESIAN_POINT('Ctrl Pts',(-1.9531562188367,-6.48135014645744,10.1038283321474));
#11214=CARTESIAN_POINT('Ctrl Pts',(-1.7848919051021,-6.52736163293417,10.1120408978709));
#11215=CARTESIAN_POINT('Ctrl Pts',(-1.61639670844841,-6.57343625380983,
10.1202647324197));
#11216=CARTESIAN_POINT('Ctrl Pts',(-1.44626829600009,-6.6129409453816,10.1284885669685));
#11217=CARTESIAN_POINT('Ctrl Pts',(-1.27506096342839,-6.64578878234488,
10.1367124015174));
#11218=CARTESIAN_POINT('Ctrl Pts',(-1.11775363041975,-6.67596976554333,
10.1442685584912));
#11219=CARTESIAN_POINT('Ctrl Pts',(-0.959535757706112,-6.70053149720022,
10.151824715465));
#11220=CARTESIAN_POINT('Ctrl Pts',(-0.800839558192604,-6.71944528975673,
10.1593808724388));
#11221=CARTESIAN_POINT('Ctrl Pts',(-0.619260138690586,-6.7410863591933,
10.1680265904911));
#11222=CARTESIAN_POINT('Ctrl Pts',(-0.436640606077396,-6.75538226963625,
10.1766723085434));
#11223=CARTESIAN_POINT('Ctrl Pts',(-0.253587320618503,-6.76224685077538,
10.1853180265958));
#11224=CARTESIAN_POINT('Ctrl Pts',(-0.0707690382729579,-6.76910261919128,
10.1939526453081));
#11225=CARTESIAN_POINT('Ctrl Pts',(0.112481583221877,-6.76854607080577,
10.2025872640203));
#11226=CARTESIAN_POINT('Ctrl Pts',(0.295552513121757,-6.76054270839164,
10.2112218827326));
#11227=CARTESIAN_POINT('Ctrl Pts',(0.485088797093329,-6.75225669830757,
10.2201614426351));
#11228=CARTESIAN_POINT('Ctrl Pts',(0.674432150438052,-6.73598822265197,
10.2291010025376));
#11229=CARTESIAN_POINT('Ctrl Pts',(0.862899522178615,-6.71175784833034,
10.23804056244));
#11230=CARTESIAN_POINT('Ctrl Pts',(1.04443275295916,-6.68841896429431,10.2466512157105));
#11231=CARTESIAN_POINT('Ctrl Pts',(1.2251529601535,-6.65769360214627,10.2552618689809));
#11232=CARTESIAN_POINT('Ctrl Pts',(1.40445101194971,-6.61965303887095,10.2638725222514));
#11233=CARTESIAN_POINT('Ctrl Pts',(1.58357934614409,-6.58164848353386,10.2724750249624));
#11234=CARTESIAN_POINT('Ctrl Pts',(1.76128791146506,-6.53634259540759,10.2810775276734));
#11235=CARTESIAN_POINT('Ctrl Pts',(1.93697516794393,-6.48385812605185,10.2896800303845));
#11236=CARTESIAN_POINT('Ctrl Pts',(2.11246469195233,-6.43143272690982,10.2982728511519));
#11237=CARTESIAN_POINT('Ctrl Pts',(2.2859371539519,-6.3718449517129,10.3068656719193));
#11238=CARTESIAN_POINT('Ctrl Pts',(2.45680342999803,-6.30526810741224,10.3154584926867));
#11239=CARTESIAN_POINT('Ctrl Pts',(2.47694079675369,-6.29742172390029,10.3164711956452));
#11240=CARTESIAN_POINT('Ctrl Pts',(2.49704197929952,-6.28947832197825,10.3174838986037));
#11241=CARTESIAN_POINT('Ctrl Pts',(2.51710602579774,-6.28143823139993,10.3184966015622));
#11242=CARTESIAN_POINT('Ctrl Pts',(2.68739845944339,-6.21319842785709,10.3270918593223));
#11243=CARTESIAN_POINT('Ctrl Pts',(2.85481392433213,-6.13806977349865,10.3356871170823));
#11244=CARTESIAN_POINT('Ctrl Pts',(3.01880316740535,-6.05632862685501,10.3442823748424));
#11245=CARTESIAN_POINT('Ctrl Pts',(3.18294597945007,-5.9745109330941,10.3528856816969));
#11246=CARTESIAN_POINT('Ctrl Pts',(3.34365589208657,-5.88606852315955,10.3614889885513));
#11247=CARTESIAN_POINT('Ctrl Pts',(3.50040945379159,-5.79132304882109,10.3700922954058));
#11248=CARTESIAN_POINT('Ctrl Pts',(3.66366207252199,-5.69264939426189,10.3790522983458));
#11249=CARTESIAN_POINT('Ctrl Pts',(3.82262296714999,-5.58713909241298,10.3880123012858));
#11250=CARTESIAN_POINT('Ctrl Pts',(3.97673666788187,-5.47520360117537,10.3969723042257));
#11251=CARTESIAN_POINT('Ctrl Pts',(4.12511995980998,-5.3674302066326,10.4055991474305));
#11252=CARTESIAN_POINT('Ctrl Pts',(4.26900982086606,-5.25370104216551,10.4142259906353));
#11253=CARTESIAN_POINT('Ctrl Pts',(4.40794602725427,-5.13442312444283,10.4228528338401));
#11254=CARTESIAN_POINT('Ctrl Pts',(4.54701502153511,-5.01503120718222,10.4314879221262));
#11255=CARTESIAN_POINT('Ctrl Pts',(4.68112068568571,-4.89008015654943,10.4401230104124));
#11256=CARTESIAN_POINT('Ctrl Pts',(4.80983962513759,-4.76001384246477,10.4487580986985));
#11257=CARTESIAN_POINT('Ctrl Pts',(4.9387497380463,-4.62975435380156,10.4574060118237));
#11258=CARTESIAN_POINT('Ctrl Pts',(5.06225693002524,-4.49436464221067,10.4660539249489));
#11259=CARTESIAN_POINT('Ctrl Pts',(5.17997706645217,-4.35432274768759,10.4747018380741));
#11260=CARTESIAN_POINT('Ctrl Pts',(5.19318347368377,-4.33861217900587,10.4756720022779));
#11261=CARTESIAN_POINT('Ctrl Pts',(5.20631709256602,-4.32284309161049,10.4766421664818));
#11262=CARTESIAN_POINT('Ctrl Pts',(5.21937741450869,-4.30701618349833,10.4776123306856));
#11263=CARTESIAN_POINT('Ctrl Pts',(5.33009780798819,-4.17284173500972,10.4858370102044));
#11264=CARTESIAN_POINT('Ctrl Pts',(5.43578695861546,-4.03421829462914,10.4940616897232));
#11265=CARTESIAN_POINT('Ctrl Pts',(5.53606876448858,-3.89155902368882,10.502286369242));
#11266=CARTESIAN_POINT('Ctrl Pts',(5.63624516283858,-3.74904970378168,10.5105024036921));
#11267=CARTESIAN_POINT('Ctrl Pts',(5.73102533033411,-3.60251329167313,10.5187184381423));
#11268=CARTESIAN_POINT('Ctrl Pts',(5.82007258227959,-3.45239686840858,10.5269344725924));
#11269=CARTESIAN_POINT('Ctrl Pts',(5.90904407181046,-3.30240816590409,10.535143516747));
#11270=CARTESIAN_POINT('Ctrl Pts',(5.99229217833759,-3.14884582507148,10.5433525609016));
#11271=CARTESIAN_POINT('Ctrl Pts',(6.06952276025712,-2.99218690303945,10.5515616050562));
#11272=CARTESIAN_POINT('Ctrl Pts',(6.14670309857145,-2.835629898005,10.5597653086843));
#11273=CARTESIAN_POINT('Ctrl Pts',(6.21787355229081,-2.67598064486513,10.5679690123123));
#11274=CARTESIAN_POINT('Ctrl Pts',(6.28278524535251,-2.51374194395146,10.5761727159403));
#11275=CARTESIAN_POINT('Ctrl Pts',(6.34766770467248,-2.35157630913816,10.5843727249343));
#11276=CARTESIAN_POINT('Ctrl Pts',(6.40629688610756,-2.18682388199999,10.5925727339283));
#11277=CARTESIAN_POINT('Ctrl Pts',(6.45847147158352,-2.02000872541228,10.6007727429222));
#11278=CARTESIAN_POINT('Ctrl Pts',(6.51064188506953,-1.85320690771652,10.6089720962262));
#11279=CARTESIAN_POINT('Ctrl Pts',(6.55635861538592,-1.68434302830992,10.6171714495301));
#11280=CARTESIAN_POINT('Ctrl Pts',(6.59546966923875,-1.51395800541219,10.6253708028341));
#11281=CARTESIAN_POINT('Ctrl Pts',(6.63458046809908,-1.34357409337446,10.6335701026807));
#11282=CARTESIAN_POINT('Ctrl Pts',(6.66708559501083,-1.17166940678454,10.6417694025272));
#11283=CARTESIAN_POINT('Ctrl Pts',(6.69288384741036,-0.998796678545469,
10.6499687023738));
#11284=CARTESIAN_POINT('Ctrl Pts',(6.71868661166906,-0.825893716576185,
10.6581694361968));
#11285=CARTESIAN_POINT('Ctrl Pts',(6.73778011155967,-0.652022730249603,
10.6663701700199));
#11286=CARTESIAN_POINT('Ctrl Pts',(6.75011484042284,-0.477743279495723,
10.6745709038429));
#11287=CARTESIAN_POINT('Ctrl Pts',(6.76245396417321,-0.303401732644257,
10.6827745596029));
#11288=CARTESIAN_POINT('Ctrl Pts',(6.76802949441791,-0.128651788846136,
10.6909782153628));
#11289=CARTESIAN_POINT('Ctrl Pts',(6.7668440233951,0.0459452178362025,10.6991818711228));
#11290=CARTESIAN_POINT('Ctrl Pts',(6.76565719433903,0.220742236613633,10.7073949246978));
#11291=CARTESIAN_POINT('Ctrl Pts',(6.7576938928307,0.395385609373892,10.7156079782729));
#11292=CARTESIAN_POINT('Ctrl Pts',(6.74300882202752,0.569316279460716,10.7238210318479));
#11293=CARTESIAN_POINT('Ctrl Pts',(6.72831506173848,0.743349868227267,10.732038945271));
#11294=CARTESIAN_POINT('Ctrl Pts',(6.70689164757387,0.916669558450377,10.7402568586941));
#11295=CARTESIAN_POINT('Ctrl Pts',(6.67884475052505,1.08872484971362,10.7484747721172));
#11296=CARTESIAN_POINT('Ctrl Pts',(6.65075410977755,1.261048489194,10.7567055027131));
#11297=CARTESIAN_POINT('Ctrl Pts',(6.61601941289762,1.43210343761496,10.7649362333091));
#11298=CARTESIAN_POINT('Ctrl Pts',(6.57479753177616,1.60135143430484,10.7731669639051));
#11299=CARTESIAN_POINT('Ctrl Pts',(6.53694016400921,1.75678547758949,10.7807259055809));
#11300=CARTESIAN_POINT('Ctrl Pts',(6.49361200355109,1.91069547167616,10.7882848472566));
#11301=CARTESIAN_POINT('Ctrl Pts',(6.44497042446897,2.06267913833449,10.7958437889324));
#11302=CARTESIAN_POINT('Ctrl Pts',(6.39249147917856,2.2266528965493,10.8039990604952));
#11303=CARTESIAN_POINT('Ctrl Pts',(6.33366470589249,2.38889122907565,10.8121543320579));
#11304=CARTESIAN_POINT('Ctrl Pts',(6.26862024425497,2.5488603793297,10.8203096036207));
#11305=CARTESIAN_POINT('Ctrl Pts',(6.20365726218112,2.70862914024645,10.8284546592796));
#11306=CARTESIAN_POINT('Ctrl Pts',(6.13249223341637,2.86613404240104,10.8365997149385));
#11307=CARTESIAN_POINT('Ctrl Pts',(6.05530549016273,3.02085491555042,10.8447447705973));
#11308=CARTESIAN_POINT('Ctrl Pts',(5.97601892578176,3.17978488140902,10.8531114078288));
#11309=CARTESIAN_POINT('Ctrl Pts',(5.89037843145591,3.33577681303247,10.8614780450603));
#11310=CARTESIAN_POINT('Ctrl Pts',(5.79863370633216,3.48828555880802,10.8698446822918));
#11311=CARTESIAN_POINT('Ctrl Pts',(5.70949954984256,3.63645471396822,10.8779732493705));
#11312=CARTESIAN_POINT('Ctrl Pts',(5.61460399167447,3.78133584760525,10.8861018164492));
#11313=CARTESIAN_POINT('Ctrl Pts',(5.51422380440614,3.92245138082305,10.8942303835279));
#11314=CARTESIAN_POINT('Ctrl Pts',(5.41389742076104,4.06349127633597,10.9023545937074));
#11315=CARTESIAN_POINT('Ctrl Pts',(5.30809247157963,4.20076929221523,10.9104788038868));
#11316=CARTESIAN_POINT('Ctrl Pts',(5.19712983400608,4.3338355400827,10.9186030140663));
#11317=CARTESIAN_POINT('Ctrl Pts',(5.08620554266485,4.46685580319922,10.9267244166985));
#11318=CARTESIAN_POINT('Ctrl Pts',(4.97012734613717,4.59566691608216,10.9348458193306));
#11319=CARTESIAN_POINT('Ctrl Pts',(4.84925728527732,4.71985092785618,10.9429672219628));
#11320=CARTESIAN_POINT('Ctrl Pts',(4.72840597956668,4.84401567026232,10.9510873644143));
#11321=CARTESIAN_POINT('Ctrl Pts',(4.60276454632192,4.96355448040034,10.9592075068658));
#11322=CARTESIAN_POINT('Ctrl Pts',(4.47273283158707,5.07808527077314,10.9673276493173));
#11323=CARTESIAN_POINT('Ctrl Pts',(4.34266559527193,5.19264734824135,10.9754500099991));
#11324=CARTESIAN_POINT('Ctrl Pts',(4.20820595494758,5.30219842961339,10.9835723706809));
#11325=CARTESIAN_POINT('Ctrl Pts',(4.06978813473268,5.40639561430618,10.9916947313627));
#11326=CARTESIAN_POINT('Ctrl Pts',(3.93134630479885,5.51061087286485,10.9998185009353));
#11327=CARTESIAN_POINT('Ctrl Pts',(3.78894522419705,5.60947017119006,11.0079422705079));
#11328=CARTESIAN_POINT('Ctrl Pts',(3.64304905248789,5.70267328550103,11.0160660400805));
#11329=CARTESIAN_POINT('Ctrl Pts',(3.49706115350793,5.79593499810972,11.0241949171978));
#11330=CARTESIAN_POINT('Ctrl Pts',(3.34757408948374,5.88353323843629,11.0323237943151));
#11331=CARTESIAN_POINT('Ctrl Pts',(3.19507795083086,5.9652129792753,11.0404526714324));
#11332=CARTESIAN_POINT('Ctrl Pts',(3.16324010823984,5.98226591421962,11.0421498023394));
#11333=CARTESIAN_POINT('Ctrl Pts',(3.13127118247908,5.99906103594538,11.0438469332463));
#11334=CARTESIAN_POINT('Ctrl Pts',(3.0991757505326,6.01559628526638,11.0455440641533));
#11335=CARTESIAN_POINT('Ctrl Pts',(3.09917575053258,6.01559628526639,9.04575158274221));
#11336=CARTESIAN_POINT('Ctrl Pts',(2.9338238445926,6.10078395293762,9.05450103065462));
#11337=CARTESIAN_POINT('Ctrl Pts',(2.76495772122974,6.17915010267054,9.06325047856703));
#11338=CARTESIAN_POINT('Ctrl Pts',(2.59315093316697,6.25042856433183,9.07199992647944));
#11339=CARTESIAN_POINT('Ctrl Pts',(2.42134553245612,6.32170645041453,9.08074930373944));
#11340=CARTESIAN_POINT('Ctrl Pts',(2.24659977927594,6.38589665313456,9.08949868099944));
#11341=CARTESIAN_POINT('Ctrl Pts',(2.06950718689932,6.44278115439071,9.09824805825945));
#11342=CARTESIAN_POINT('Ctrl Pts',(1.89241596572878,6.49966521519719,9.1069973677741));
#11343=CARTESIAN_POINT('Ctrl Pts',(1.71297821457217,6.54924360009541,9.11574667728875));
#11344=CARTESIAN_POINT('Ctrl Pts',(1.53180337335867,6.59134792173551,9.12449598680341));
#11345=CARTESIAN_POINT('Ctrl Pts',(1.35062987477799,6.63345193135302,9.13324523147953));
#11346=CARTESIAN_POINT('Ctrl Pts',(1.16771959102961,6.66808192368236,9.14199447615566));
#11347=CARTESIAN_POINT('Ctrl Pts',(0.983693746906862,6.69512028363168,9.15074372083179));
#11348=CARTESIAN_POINT('Ctrl Pts',(0.799669205419905,6.72215845218867,9.15949290357596));
#11349=CARTESIAN_POINT('Ctrl Pts',(0.614529402873525,6.74160505424579,9.16824208632014));
#11350=CARTESIAN_POINT('Ctrl Pts',(0.428903127363314,6.75339404354122,9.17699126906432));
#11351=CARTESIAN_POINT('Ctrl Pts',(0.243278104163857,6.7651829533033,9.18574039278293));
#11352=CARTESIAN_POINT('Ctrl Pts',(0.0571669005390063,6.76931433552276,
9.19448951650154));
#11353=CARTESIAN_POINT('Ctrl Pts',(-0.128798404777712,6.76577415902473,
9.20323864022015));
#11354=CARTESIAN_POINT('Ctrl Pts',(-0.314762517259244,6.76223400523441,
9.21198770781936));
#11355=CARTESIAN_POINT('Ctrl Pts',(-0.500580446819601,6.75102239665088,
9.22073677541857));
#11356=CARTESIAN_POINT('Ctrl Pts',(-0.685621118842648,6.73217741012497,
9.22948584301777));
#11357=CARTESIAN_POINT('Ctrl Pts',(-0.8706606654147,6.71333253821769,9.23823485740356));
#11358=CARTESIAN_POINT('Ctrl Pts',(-1.05492267885525,6.68685441030606,9.24698387178934));
#11359=CARTESIAN_POINT('Ctrl Pts',(-1.23778137635307,6.65283295028167,9.25573288617513));
#11360=CARTESIAN_POINT('Ctrl Pts',(-1.42999922978902,6.61707018861853,9.26492969654252));
#11361=CARTESIAN_POINT('Ctrl Pts',(-1.62066601233751,6.57297172934399,9.27412650690992));
#11362=CARTESIAN_POINT('Ctrl Pts',(-1.80906628500441,6.52070304311279,9.28332331727731));
#11363=CARTESIAN_POINT('Ctrl Pts',(-1.98831342545581,6.47097374915014,9.29207331501507));
#11364=CARTESIAN_POINT('Ctrl Pts',(-2.16550875896753,6.41384933989511,9.30082331275284));
#11365=CARTESIAN_POINT('Ctrl Pts',(-2.3400503671406,6.34952386240458,9.3095733104906));
#11366=CARTESIAN_POINT('Ctrl Pts',(-2.51458843547144,6.28519968948574,9.31832313077147));
#11367=CARTESIAN_POINT('Ctrl Pts',(-2.68647261718115,6.21367483971073,9.32707295105234));
#11368=CARTESIAN_POINT('Ctrl Pts',(-2.85511905908796,6.13519226743814,9.33582277133321));
#11369=CARTESIAN_POINT('Ctrl Pts',(-3.02376230488947,6.05671118252905,9.34457242579174));
#11370=CARTESIAN_POINT('Ctrl Pts',(-3.18916767379966,5.971272759926,9.35332208025027));
#11371=CARTESIAN_POINT('Ctrl Pts',(-3.35077334102847,5.87916720437963,9.3620717347088));
#11372=CARTESIAN_POINT('Ctrl Pts',(-3.51237616037431,5.78706327195605,9.37082123497725));
#11373=CARTESIAN_POINT('Ctrl Pts',(-3.67017916302367,5.68829258362255,9.37957073524569));
#11374=CARTESIAN_POINT('Ctrl Pts',(-3.82364636566533,5.58319061740994,9.38832023551414));
#11375=CARTESIAN_POINT('Ctrl Pts',(-3.97711106778862,5.47809036367655,9.39706959322257));
#11376=CARTESIAN_POINT('Ctrl Pts',(-4.12623987481985,5.3666592004318,9.40581895093101));
#11377=CARTESIAN_POINT('Ctrl Pts',(-4.27052628213981,5.24927559512293,9.41456830863944));
#11378=CARTESIAN_POINT('Ctrl Pts',(-4.41481053025038,5.13189374642985,9.42331753541596));
#11379=CARTESIAN_POINT('Ctrl Pts',(-4.55425230136597,5.00855981477292,9.43206676219249));
#11380=CARTESIAN_POINT('Ctrl Pts',(-4.68837800630622,4.87969268192005,9.44081598896901));
#11381=CARTESIAN_POINT('Ctrl Pts',(-4.82250188228976,4.75082730631727,9.44956509643986));
#11382=CARTESIAN_POINT('Ctrl Pts',(-4.95130963053055,4.61642907903431,9.45831420391071));
#11383=CARTESIAN_POINT('Ctrl Pts',(-5.07436379033463,4.47695444731581,9.46706331138156));
#11384=CARTESIAN_POINT('Ctrl Pts',(-5.19741643562904,4.33748153220469,9.47581231117131));
#11385=CARTESIAN_POINT('Ctrl Pts',(-5.31471544462873,4.19293255254462,9.48456131096106));
#11386=CARTESIAN_POINT('Ctrl Pts',(-5.42586245275729,4.04379841779467,9.49331031075081));
#11387=CARTESIAN_POINT('Ctrl Pts',(-5.53702160019251,3.89464799484203,9.50206026609297));
#11388=CARTESIAN_POINT('Ctrl Pts',(-5.64202723081347,3.74091164443706,9.51081022143512));
#11389=CARTESIAN_POINT('Ctrl Pts',(-5.74052265233059,3.58311159163086,9.51956017677728));
#11390=CARTESIAN_POINT('Ctrl Pts',(-5.83901427067006,3.42531763191634,9.52830979425973));
#11391=CARTESIAN_POINT('Ctrl Pts',(-5.93099603115823,3.26346052695461,9.53705941174218));
#11392=CARTESIAN_POINT('Ctrl Pts',(-6.01615550622833,3.09809004466923,9.54580902922462));
#11393=CARTESIAN_POINT('Ctrl Pts',(-6.1013121457888,2.93272506863661,9.55455835537572));
#11394=CARTESIAN_POINT('Ctrl Pts',(-6.17964682328829,2.76384720416714,9.56330768152682));
#11395=CARTESIAN_POINT('Ctrl Pts',(-6.25089348288644,2.59203002791399,9.57205700767793));
#11396=CARTESIAN_POINT('Ctrl Pts',(-6.32213814889404,2.42021765936835,9.58080608900949));
#11397=CARTESIAN_POINT('Ctrl Pts',(-6.38629508412653,2.24546640831724,9.58955517034106));
#11398=CARTESIAN_POINT('Ctrl Pts',(-6.44314639819874,2.06836976659848,9.59830425167263));
#11399=CARTESIAN_POINT('Ctrl Pts',(-6.50000285283759,1.89125711158074,9.60705412410703));
#11400=CARTESIAN_POINT('Ctrl Pts',(-6.54955227673304,1.71179891440046,9.61580399654143));
#11401=CARTESIAN_POINT('Ctrl Pts',(-6.59162635926435,1.53060476278214,9.62455386897583));
#11402=CARTESIAN_POINT('Ctrl Pts',(-6.63369752055242,1.34942319164472,9.63330313389833));
#11403=CARTESIAN_POINT('Ctrl Pts',(-6.66829431424295,1.16650618642473,9.64205239882083));
#11404=CARTESIAN_POINT('Ctrl Pts',(-6.69529923745452,0.982474997616181,
9.65080166374333));
#11405=CARTESIAN_POINT('Ctrl Pts',(-6.72230554731472,0.798434359175324,
9.65955137792304));
#11406=CARTESIAN_POINT('Ctrl Pts',(-6.74171916496725,0.61327970623788,9.66830109210274));
#11407=CARTESIAN_POINT('Ctrl Pts',(-6.75347414817291,0.427639953652885,
9.67705080628244));
#11408=CARTESIAN_POINT('Ctrl Pts',(-6.76248837758749,0.285283364196959,
9.6837604654583));
#11409=CARTESIAN_POINT('Ctrl Pts',(-6.76699999999996,0.142641701104389,
9.69047012463416));
#11410=CARTESIAN_POINT('Ctrl Pts',(-6.767,1.7245986591618E-12,9.69717978381002));
#11411=CARTESIAN_POINT('',(-6.76699881632875,0.00201345172301315,9.30282021618989));
#11412=CARTESIAN_POINT('Ctrl Pts',(3.09917575053261,6.01559628526638,8.65154848238438));
#11413=CARTESIAN_POINT('Ctrl Pts',(2.93648754800763,6.09941163926513,8.66016209671495));
#11414=CARTESIAN_POINT('Ctrl Pts',(2.77027489456604,6.17668648178732,8.66877571104552));
#11415=CARTESIAN_POINT('Ctrl Pts',(2.60107937308078,6.2471333501802,8.67738932537608));
#11416=CARTESIAN_POINT('Ctrl Pts',(2.43204707156897,6.31751225970581,8.6859946303029));
#11417=CARTESIAN_POINT('Ctrl Pts',(2.2600379194756,6.38107621066294,8.6945999352297));
#11418=CARTESIAN_POINT('Ctrl Pts',(2.08561650640442,6.4375843907644,8.70320524015651));
#11419=CARTESIAN_POINT('Ctrl Pts',(1.91140403447069,6.49402487915749,8.71180023670336));
#11420=CARTESIAN_POINT('Ctrl Pts',(1.73478535613973,6.54342636604349,8.72039523325021));
#11421=CARTESIAN_POINT('Ctrl Pts',(1.5563434826823,6.58559670522819,8.72899022979705));
#11422=CARTESIAN_POINT('Ctrl Pts',(1.4830144389203,6.60292621756527,8.73252226443504));
#11423=CARTESIAN_POINT('Ctrl Pts',(1.40937772352134,6.61903515919354,8.73605429907302));
#11424=CARTESIAN_POINT('Ctrl Pts',(1.3354746271782,6.6339126102296,8.739586333711));
#11425=CARTESIAN_POINT('Ctrl Pts',(1.15561990778682,6.67011920932695,8.74818209126553));
#11426=CARTESIAN_POINT('Ctrl Pts',(0.974397471948755,6.69898614923061,8.75677784882006));
#11427=CARTESIAN_POINT('Ctrl Pts',(0.792418247089899,6.72044361048279,8.76537360637459));
#11428=CARTESIAN_POINT('Ctrl Pts',(0.610269229423072,6.74192109227634,8.77397738406336));
#11429=CARTESIAN_POINT('Ctrl Pts',(0.4273623165183,6.75597526047728,8.78258116175212));
#11430=CARTESIAN_POINT('Ctrl Pts',(0.244311675476918,6.76258832143623,8.79118493944089));
#11431=CARTESIAN_POINT('Ctrl Pts',(0.0540669844083164,6.76946128146519,
8.80012685310539));
#11432=CARTESIAN_POINT('Ctrl Pts',(-0.136332583699432,6.76829642190302,
8.80906876676989));
#11433=CARTESIAN_POINT('Ctrl Pts',(-0.326201127095777,6.75913321548566,
8.81801068043438));
#11434=CARTESIAN_POINT('Ctrl Pts',(-0.509387232777708,6.75029250880971,
8.8266378827726));
#11435=CARTESIAN_POINT('Ctrl Pts',(-0.692078764494619,6.73400693969177,
8.83526508511082));
#11436=CARTESIAN_POINT('Ctrl Pts',(-0.873667647935661,6.7103646578223,8.84389228744904));
#11437=CARTESIAN_POINT('Ctrl Pts',(-1.0554294669953,6.68669986029789,8.85252770587705));
#11438=CARTESIAN_POINT('Ctrl Pts',(-1.23608624078694,6.65566441370846,8.86116312430507));
#11439=CARTESIAN_POINT('Ctrl Pts',(-1.41504049283352,6.61739747964723,8.86979854273309));
#11440=CARTESIAN_POINT('Ctrl Pts',(-1.59425912429878,6.57907401164133,8.87844671876188));
#11441=CARTESIAN_POINT('Ctrl Pts',(-1.77176991134944,6.53349777857669,8.88709489479067));
#11442=CARTESIAN_POINT('Ctrl Pts',(-1.94698948617415,6.48085804047021,8.89574307081946));
#11443=CARTESIAN_POINT('Ctrl Pts',(-1.96552705211969,6.47528895598018,8.89665801501792));
#11444=CARTESIAN_POINT('Ctrl Pts',(-1.98403899069124,6.4696408554876,8.89757295921638));
#11445=CARTESIAN_POINT('Ctrl Pts',(-2.00252462408755,6.46391399462609,8.89848790341484));
#11446=CARTESIAN_POINT('Ctrl Pts',(-2.1687234837376,6.4124254832967,8.90671389595549));
#11447=CARTESIAN_POINT('Ctrl Pts',(-2.33315341001072,6.35445537053403,8.91493988849615));
#11448=CARTESIAN_POINT('Ctrl Pts',(-2.49527320211393,6.29014313404807,8.9231658810368));
#11449=CARTESIAN_POINT('Ctrl Pts',(-2.65722303256971,6.22589832062947,8.93138324968752));
#11450=CARTESIAN_POINT('Ctrl Pts',(-2.81686722140321,6.15532475493372,8.93960061833823));
#11451=CARTESIAN_POINT('Ctrl Pts',(-2.97367894937343,6.07861188973711,8.94781798698894));
#11452=CARTESIAN_POINT('Ctrl Pts',(-3.13035765786271,6.00196409815229,8.95602838505062));
#11453=CARTESIAN_POINT('Ctrl Pts',(-3.28420837076711,5.91918753569112,8.96423878311229));
#11454=CARTESIAN_POINT('Ctrl Pts',(-3.43472342455742,5.83052004514147,8.97244918117397));
#11455=CARTESIAN_POINT('Ctrl Pts',(-3.58514090910781,5.74191003202974,8.98065425696203));
#11456=CARTESIAN_POINT('Ctrl Pts',(-3.73222673407548,5.64741687862983,8.9888593327501));
#11457=CARTESIAN_POINT('Ctrl Pts',(-3.87549698699058,5.54732476999742,8.99706440853817));
#11458=CARTESIAN_POINT('Ctrl Pts',(-4.01870302086423,5.44727752636066,9.00526580650692));
#11459=CARTESIAN_POINT('Ctrl Pts',(-4.15809659696912,5.34163653223326,9.01346720447568));
#11460=CARTESIAN_POINT('Ctrl Pts',(-4.29322192553541,5.23072982461358,9.02166860244444));
#11461=CARTESIAN_POINT('Ctrl Pts',(-4.42833666996081,5.11983180413074,9.02986935801142));
#11462=CARTESIAN_POINT('Ctrl Pts',(-4.55918355052281,5.00366911210476,9.0380701135784));
#11463=CARTESIAN_POINT('Ctrl Pts',(-4.68533879233318,4.88261092050738,9.04627086914538));
#11464=CARTESIAN_POINT('Ctrl Pts',(-4.81149339333496,4.76155334382798,9.05447158305643));
#11465=CARTESIAN_POINT('Ctrl Pts',(-4.93295614373756,4.63560056447028,9.06267229696747));
#11466=CARTESIAN_POINT('Ctrl Pts',(-5.0493392712357,4.50515947819352,9.07087301087851));
#11467=CARTESIAN_POINT('Ctrl Pts',(-5.16574289908355,4.37469541532263,9.07907516930739));
#11468=CARTESIAN_POINT('Ctrl Pts',(-5.27706488279496,4.23974173781979,9.08727732773627));
#11469=CARTESIAN_POINT('Ctrl Pts',(-5.38295694247679,4.10073939130993,9.09547948616514));
#11470=CARTESIAN_POINT('Ctrl Pts',(-5.48888684503592,3.96168736922706,9.10368457581734));
#11471=CARTESIAN_POINT('Ctrl Pts',(-5.58938274093627,3.81858408075926,9.11188966546954));
#11472=CARTESIAN_POINT('Ctrl Pts',(-5.6841389485791,3.67190051788526,9.12009475512174));
#11473=CARTESIAN_POINT('Ctrl Pts',(-5.77900340398618,3.52504938638302,9.12830921811878));
#11474=CARTESIAN_POINT('Ctrl Pts',(-5.8681148769155,3.37461011062403,9.13652368111582));
#11475=CARTESIAN_POINT('Ctrl Pts',(-5.9512125171873,3.22108034287772,9.14473814411286));
#11476=CARTESIAN_POINT('Ctrl Pts',(-6.03435939018455,3.06745961359652,9.1529574739196));
#11477=CARTESIAN_POINT('Ctrl Pts',(-6.11148517010585,2.91074506340614,9.16117680372633));
#11478=CARTESIAN_POINT('Ctrl Pts',(-6.18237673831163,2.75145540861254,9.16939613353307));
#11479=CARTESIAN_POINT('Ctrl Pts',(-6.25337814870437,2.59191894415619,9.17762819869303));
#11480=CARTESIAN_POINT('Ctrl Pts',(-6.31812591104038,2.42979973416161,9.18586026385298));
#11481=CARTESIAN_POINT('Ctrl Pts',(-6.37645602069225,2.26563404286252,9.19409232901294));
#11482=CARTESIAN_POINT('Ctrl Pts',(-6.42888731164545,2.11807013159255,9.20149190028279));
#11483=CARTESIAN_POINT('Ctrl Pts',(-6.47613395471416,1.96885309922747,9.20889147155265));
#11484=CARTESIAN_POINT('Ctrl Pts',(-6.51811212380928,1.81837931726316,9.2162910428225));
#11485=CARTESIAN_POINT('Ctrl Pts',(-6.57652369905974,1.60899880286983,9.22658736167982));
#11486=CARTESIAN_POINT('Ctrl Pts',(-6.62488316915981,1.39665633020682,9.23688368053714));
#11487=CARTESIAN_POINT('Ctrl Pts',(-6.66293320233366,1.18220562561667,9.24717999939447));
#11488=CARTESIAN_POINT('Ctrl Pts',(-6.7003504764938,0.971321162761626,9.25730509399726));
#11489=CARTESIAN_POINT('Ctrl Pts',(-6.72779836156197,0.758397917147425,
9.26743018860006));
#11490=CARTESIAN_POINT('Ctrl Pts',(-6.74507664073389,0.544270255136271,
9.27755528320285));
#11491=CARTESIAN_POINT('Ctrl Pts',(-6.7594480147814,0.366167523141684,9.28597692753186));
#11492=CARTESIAN_POINT('Ctrl Pts',(-6.7667845369513,0.187231905133603,9.29439857186088));
#11493=CARTESIAN_POINT('Ctrl Pts',(-6.76699532258635,0.00795638702641748,
9.30282021618989));
#11494=CARTESIAN_POINT('Ctrl Pts',(-6.767,1.50055999763773E-12,9.30282021618989));
#11495=CARTESIAN_POINT('Ctrl Pts',(-6.76700000000004,-0.186007249414152,
9.31156972799584));
#11496=CARTESIAN_POINT('Ctrl Pts',(-6.75932637295447,-0.372014355525981,
9.32031923980179));
#11497=CARTESIAN_POINT('Ctrl Pts',(-6.74400518266941,-0.557389537153473,
9.32906875160774));
#11498=CARTESIAN_POINT('Ctrl Pts',(-6.72868405709661,-0.742763935810001,
9.33781822645829));
#11499=CARTESIAN_POINT('Ctrl Pts',(-6.70571545653009,-0.927506129693821,
9.34656770130884));
#11500=CARTESIAN_POINT('Ctrl Pts',(-6.67517739415667,-1.11098863924872,
9.35531717615939));
#11501=CARTESIAN_POINT('Ctrl Pts',(-6.64463945823084,-1.29447038906588,
9.36406661478138));
#11502=CARTESIAN_POINT('Ctrl Pts',(-6.60653217027133,-1.47669218228329,
9.37281605340338));
#11503=CARTESIAN_POINT('Ctrl Pts',(-6.56098496116677,-1.65703510504258,
9.38156549202537));
#11504=CARTESIAN_POINT('Ctrl Pts',(-6.5154379368747,-1.83737729604189,9.39031489514562));
#11505=CARTESIAN_POINT('Ctrl Pts',(-6.46245112202578,-2.01584035397252,
9.39906429826587));
#11506=CARTESIAN_POINT('Ctrl Pts',(-6.40220448416164,-2.19181813638371,
9.40781370138612));
#11507=CARTESIAN_POINT('Ctrl Pts',(-6.34195808575096,-2.36779521936189,
9.4165630697314));
#11508=CARTESIAN_POINT('Ctrl Pts',(-6.27445201489129,-2.54128677545089,
9.42531243807668));
#11509=CARTESIAN_POINT('Ctrl Pts',(-6.19991555136063,-2.71170355238117,
9.43406180642196));
#11510=CARTESIAN_POINT('Ctrl Pts',(-6.1253793778891,-2.88211966613345,9.44281114071902));
#11511=CARTESIAN_POINT('Ctrl Pts',(-6.04381298133482,-3.04946076210713,
9.45156047501607));
#11512=CARTESIAN_POINT('Ctrl Pts',(-5.95549339426164,-3.21315848207118,
9.46030980931313));
#11513=CARTESIAN_POINT('Ctrl Pts',(-5.86717414355014,-3.37685557859891,
9.46905911028869));
#11514=CARTESIAN_POINT('Ctrl Pts',(-5.77210188986087,-3.53690907467557,
9.47780841126425));
#11515=CARTESIAN_POINT('Ctrl Pts',(-5.67059953466914,-3.69277536785142,
9.48655771223981));
#11516=CARTESIAN_POINT('Ctrl Pts',(-5.56909755761611,-3.84864108036016,
9.49530698062057));
#11517=CARTESIAN_POINT('Ctrl Pts',(-5.46116568337916,-4.00031938104489,
9.50405624900132));
#11518=CARTESIAN_POINT('Ctrl Pts',(-5.34717048685962,-4.14729511663415,
9.51280551738208));
#11519=CARTESIAN_POINT('Ctrl Pts',(-5.23317570555364,-4.29427031688228,
9.5215547538947));
#11520=CARTESIAN_POINT('Ctrl Pts',(-5.1131178217865,-4.43654275987308,9.53030399040731));
#11521=CARTESIAN_POINT('Ctrl Pts',(-4.98740459171859,-4.57362924147819,
9.53905322691993));
#11522=CARTESIAN_POINT('Ctrl Pts',(-4.86169180910671,-4.710715235146,9.54780243229105));
#11523=CARTESIAN_POINT('Ctrl Pts',(-4.73032391415269,-4.84261509316682,
9.55655163766216));
#11524=CARTESIAN_POINT('Ctrl Pts',(-4.59374707237128,-4.96888084331676,
9.56530084303328));
#11525=CARTESIAN_POINT('Ctrl Pts',(-4.45717070537247,-5.09514615452859,
9.5740500179895));
#11526=CARTESIAN_POINT('Ctrl Pts',(-4.31538563819366,-5.2157772025375,9.58279919294572));
#11527=CARTESIAN_POINT('Ctrl Pts',(-4.16887341290518,-5.33036429028752,
9.59154836790194));
#11528=CARTESIAN_POINT('Ctrl Pts',(-4.0223616847722,-5.44495098921263,9.60029751316984));
#11529=CARTESIAN_POINT('Ctrl Pts',(-3.87112305634334,-5.55349359238831,
9.60904665843776));
#11530=CARTESIAN_POINT('Ctrl Pts',(-3.71567117316642,-5.65562346102533,
9.61779580370566));
#11531=CARTESIAN_POINT('Ctrl Pts',(-3.56021980457225,-5.75775299158815,
9.62654492001182));
#11532=CARTESIAN_POINT('Ctrl Pts',(-3.40055544862328,-5.85346967275388,
9.63529403631797));
#11533=CARTESIAN_POINT('Ctrl Pts',(-3.23722036323359,-5.94244842803585,
9.64404315262413));
#11534=CARTESIAN_POINT('Ctrl Pts',(-3.07388580495981,-6.03142689616509,
9.65279224069508));
#11535=CARTESIAN_POINT('Ctrl Pts',(-2.90688079257619,-6.11366734484865,
9.66154132876604));
#11536=CARTESIAN_POINT('Ctrl Pts',(-2.73677251094504,-6.18889046787351,
9.670290416837));
#11537=CARTESIAN_POINT('Ctrl Pts',(-2.56666476416553,-6.26411335438307,
9.67903947739921));
#11538=CARTESIAN_POINT('Ctrl Pts',(-2.39345402972021,-6.33231884350317,
9.68778853796143));
#11539=CARTESIAN_POINT('Ctrl Pts',(-2.21772856473987,-6.39327529621061,
9.69653759852365));
#11540=CARTESIAN_POINT('Ctrl Pts',(-2.04200363768245,-6.45423156232089,
9.70528663230364));
#11541=CARTESIAN_POINT('Ctrl Pts',(-1.86376426620097,-6.50793874252054,
9.71403566608363));
#11542=CARTESIAN_POINT('Ctrl Pts',(-1.68361578194719,-6.55421443796115,
9.72278469986361));
#11543=CARTESIAN_POINT('Ctrl Pts',(-1.50346783419942,-6.60048999558662,
9.73153370758782));
#11544=CARTESIAN_POINT('Ctrl Pts',(-1.32141106257363,-6.63933404145471,
9.74028271531203));
#11545=CARTESIAN_POINT('Ctrl Pts',(-1.13806375959204,-6.67061465527003,
9.74903172303624));
#11546=CARTESIAN_POINT('Ctrl Pts',(-0.954716987420288,-6.70189517852466,
9.75778070543114));
#11547=CARTESIAN_POINT('Ctrl Pts',(-0.770079973810545,-6.72561226535821,
9.76652968782605));
#11548=CARTESIAN_POINT('Ctrl Pts',(-0.584779770552651,-6.7416853693978,
9.77527867022096));
#11549=CARTESIAN_POINT('Ctrl Pts',(-0.391490647554111,-6.75845143942393,
9.78440485089701));
#11550=CARTESIAN_POINT('Ctrl Pts',(-0.197480213104537,-6.76689975924026,
9.79353103157306));
#11551=CARTESIAN_POINT('Ctrl Pts',(-0.00346532629800411,-6.76699911271707,
9.80265721224912));
#11552=CARTESIAN_POINT('Ctrl Pts',(0.184486595295824,-6.76709536139774,
9.81149819977905));
#11553=CARTESIAN_POINT('Ctrl Pts',(0.372442378184971,-6.75935659726771,
9.82033918730897));
#11554=CARTESIAN_POINT('Ctrl Pts',(0.559750217721805,-6.74380965729019,
9.8291801748389));
#11555=CARTESIAN_POINT('Ctrl Pts',(0.745129914457424,-6.72842275717257,
9.83793015343666));
#11556=CARTESIAN_POINT('Ctrl Pts',(0.929874656313808,-6.70538772273478,
9.84668013203443));
#11557=CARTESIAN_POINT('Ctrl Pts',(1.11335688289735,-6.67478280180749,9.8554301106322));
#11558=CARTESIAN_POINT('Ctrl Pts',(1.29683723118809,-6.64417819418033,9.86417999965714));
#11559=CARTESIAN_POINT('Ctrl Pts',(1.47905480730182,-6.60600390230087,9.87292988868207));
#11560=CARTESIAN_POINT('Ctrl Pts',(1.6593906480475,-6.56038959797149,9.88167977770701));
#11561=CARTESIAN_POINT('Ctrl Pts',(1.83972470264205,-6.51477574543273,9.89042958006796));
#11562=CARTESIAN_POINT('Ctrl Pts',(2.01817678125786,-6.46172209820119,9.89917938242891));
#11563=CARTESIAN_POINT('Ctrl Pts',(2.19414072347616,-6.40140886724036,9.90792918478985));
#11564=CARTESIAN_POINT('Ctrl Pts',(2.37010298132039,-6.34109621361396,9.91667890339534));
#11565=CARTESIAN_POINT('Ctrl Pts',(2.54357687926861,-6.27352420825992,9.92542862200083));
#11566=CARTESIAN_POINT('Ctrl Pts',(2.71397317789925,-6.19892237325517,9.93417834060632));
#11567=CARTESIAN_POINT('Ctrl Pts',(2.88436790207162,-6.12432122756982,9.94292797836459));
#11568=CARTESIAN_POINT('Ctrl Pts',(3.05168482126224,-6.04269049717434,9.95167761612286));
#11569=CARTESIAN_POINT('Ctrl Pts',(3.21535561997362,-5.95430745234944,9.96042725388113));
#11570=CARTESIAN_POINT('Ctrl Pts',(3.37902496075256,-5.86592519481531,9.96917681370014));
#11571=CARTESIAN_POINT('Ctrl Pts',(3.53904799384852,-5.77079087940246,9.97792637351916));
#11572=CARTESIAN_POINT('Ctrl Pts',(3.69488118814964,-5.66922763747038,9.98667593333817));
#11573=CARTESIAN_POINT('Ctrl Pts',(3.85071304610807,-5.5676652664907,9.99542541812561));
#11574=CARTESIAN_POINT('Ctrl Pts',(4.00235489705936,-5.45967423580737,10.004174902913));
#11575=CARTESIAN_POINT('Ctrl Pts',(4.14929168607617,-5.34562133936357,10.0129243877005));
#11576=CARTESIAN_POINT('Ctrl Pts',(4.29622726385719,-5.23156938308562,10.0216738003638));
#11577=CARTESIAN_POINT('Ctrl Pts',(4.43845763092027,-5.11145583677237,10.0304232130271));
#11578=CARTESIAN_POINT('Ctrl Pts',(4.57549970660921,-4.98568866204249,10.0391726256904));
#11579=CARTESIAN_POINT('Ctrl Pts',(4.71254069815249,-4.85992248226205,10.0479219691367));
#11580=CARTESIAN_POINT('Ctrl Pts',(4.84439326931264,-4.72850295734053,10.056671312583));
#11581=CARTESIAN_POINT('Ctrl Pts',(4.97060959434645,-4.59187644221739,10.0654206560293));
#11582=CARTESIAN_POINT('Ctrl Pts',(5.09682496280464,-4.45525096256723,10.0741699331656));
#11583=CARTESIAN_POINT('Ctrl Pts',(5.21740397615789,-4.31341878218386,10.0829192103019));
#11584=CARTESIAN_POINT('Ctrl Pts',(5.33193710451886,-4.16686161438738,10.0916684874382));
#11585=CARTESIAN_POINT('Ctrl Pts',(5.44646940289332,-4.02030550864583,10.1004177011712));
#11586=CARTESIAN_POINT('Ctrl Pts',(5.5549557274961,-3.86902470980211,10.1091669149041));
#11587=CARTESIAN_POINT('Ctrl Pts',(5.65702762491399,-3.71353301465869,10.1179161286371));
#11588=CARTESIAN_POINT('Ctrl Pts',(5.75909881655102,-3.55804239466978,10.1266652818732));
#11589=CARTESIAN_POINT('Ctrl Pts',(5.85475551250734,-3.39834117619635,10.1354144351093));
#11590=CARTESIAN_POINT('Ctrl Pts',(5.94367283728051,-3.23497174692049,10.1441635883455));
#11591=CARTESIAN_POINT('Ctrl Pts',(6.03258957676271,-3.07160339301045,10.152912683991));
#11592=CARTESIAN_POINT('Ctrl Pts',(6.11476689685247,-2.90456712829582,10.1616617796365));
#11593=CARTESIAN_POINT('Ctrl Pts',(6.18992570525227,-2.73443024475981,10.1704108752821));
#11594=CARTESIAN_POINT('Ctrl Pts',(6.26508404388674,-2.56429442463088,10.1791599162431));
#11595=CARTESIAN_POINT('Ctrl Pts',(6.33322384283301,-2.39105828656032,10.1879089572041));
#11596=CARTESIAN_POINT('Ctrl Pts',(6.39411368720026,-2.21531017132101,10.1966579981652));
#11597=CARTESIAN_POINT('Ctrl Pts',(6.45500317120884,-2.03956309619534,10.2054069873476));
#11598=CARTESIAN_POINT('Ctrl Pts',(6.50864269270068,-1.86130434438651,10.21415597653));
#11599=CARTESIAN_POINT('Ctrl Pts',(6.55485008446329,-1.68113930719961,10.2229049657124));
#11600=CARTESIAN_POINT('Ctrl Pts',(6.60199664749401,-1.49731239211854,10.2318317792418));
#11601=CARTESIAN_POINT('Ctrl Pts',(6.64140563640904,-1.31150116499684,10.2407585927711));
#11602=CARTESIAN_POINT('Ctrl Pts',(6.6729377228217,-1.1243625515567,10.2496854063005));
#11603=CARTESIAN_POINT('Ctrl Pts',(6.7038449494987,-0.94093239505143,10.258435320456));
#11604=CARTESIAN_POINT('Ctrl Pts',(6.7271844934893,-0.756227260506783,10.2671852346115));
#11605=CARTESIAN_POINT('Ctrl Pts',(6.74287707373932,-0.570874564541741,
10.2759351487671));
#11606=CARTESIAN_POINT('Ctrl Pts',(6.7585693453867,-0.385525513632511,10.2846848908511));
#11607=CARTESIAN_POINT('Ctrl Pts',(6.76661493004103,-0.199529212418251,
10.293434632935));
#11608=CARTESIAN_POINT('Ctrl Pts',(6.76698649908907,-0.0135174386004342,
10.302184375019));
#11609=CARTESIAN_POINT('Ctrl Pts',(6.76735806132389,0.172490924445833,10.3109339566649));
#11610=CARTESIAN_POINT('Ctrl Pts',(6.76005588896289,0.358514472901523,10.3196835383108));
#11611=CARTESIAN_POINT('Ctrl Pts',(6.74510478454583,0.543921359662389,10.3284331199567));
#11612=CARTESIAN_POINT('Ctrl Pts',(6.73015393440686,0.729325093150645,10.3371825527958));
#11613=CARTESIAN_POINT('Ctrl Pts',(6.70755443556894,0.914111900256575,10.3459319856348));
#11614=CARTESIAN_POINT('Ctrl Pts',(6.67738304682315,1.09765415591563,10.3546814184738));
#11615=CARTESIAN_POINT('Ctrl Pts',(6.64721213111854,1.28119353391307,10.3634307141352));
#11616=CARTESIAN_POINT('Ctrl Pts',(6.60946960955485,1.46348811672696,10.3721800097965));
#11617=CARTESIAN_POINT('Ctrl Pts',(6.5642836699117,1.64391876348274,10.3809293054578));
#11618=CARTESIAN_POINT('Ctrl Pts',(6.51909837867704,1.82434682109763,10.3896784755687));
#11619=CARTESIAN_POINT('Ctrl Pts',(6.46646995271908,2.00291071820488,10.3984276456795));
#11620=CARTESIAN_POINT('Ctrl Pts',(6.40657713281536,2.17900400212742,10.4071768157903));
#11621=CARTESIAN_POINT('Ctrl Pts',(6.34668509279043,2.35509499309703,10.4159258719761));
#11622=CARTESIAN_POINT('Ctrl Pts',(6.27952894037506,2.52871516398173,10.4246749281619));
#11623=CARTESIAN_POINT('Ctrl Pts',(6.20533675061422,2.69927486771476,10.4334239843476));
#11624=CARTESIAN_POINT('Ctrl Pts',(6.12832117907892,2.87632521635975,10.4425059856299));
#11625=CARTESIAN_POINT('Ctrl Pts',(6.04372366626056,3.05007728920043,10.4515879869122));
#11626=CARTESIAN_POINT('Ctrl Pts',(5.95185378007846,3.21989527478237,10.4606699881944));
#11627=CARTESIAN_POINT('Ctrl Pts',(5.86334450817348,3.38350129286792,10.4694197685016));
#11628=CARTESIAN_POINT('Ctrl Pts',(5.76808562057231,3.54345567125002,10.4781695488087));
#11629=CARTESIAN_POINT('Ctrl Pts',(5.66640068804458,3.69921508465348,10.4869193291158));
#11630=CARTESIAN_POINT('Ctrl Pts',(5.56471941107895,3.85496889852324,10.4956687948693));
#11631=CARTESIAN_POINT('Ctrl Pts',(5.45661270815083,4.00652780919679,10.5044182606228));
#11632=CARTESIAN_POINT('Ctrl Pts',(5.3424477644908,4.15337704569273,10.5131677263763));
#11633=CARTESIAN_POINT('Ctrl Pts',(5.22828631819558,4.30022178356295,10.5219169240959));
#11634=CARTESIAN_POINT('Ctrl Pts',(5.10806717844028,4.44235690972726,10.5306661218155));
#11635=CARTESIAN_POINT('Ctrl Pts',(4.98219864544675,4.57929969070693,10.5394153195351));
#11636=CARTESIAN_POINT('Ctrl Pts',(4.8563332994399,4.71623900430036,10.5481642957253));
#11637=CARTESIAN_POINT('Ctrl Pts',(4.72481904033624,4.84798602483639,10.5569132719155));
#11638=CARTESIAN_POINT('Ctrl Pts',(4.58810250737186,4.97409332259137,10.5656622481058));
#11639=CARTESIAN_POINT('Ctrl Pts',(4.45137708685627,5.10020881822149,10.5744117930419));
#11640=CARTESIAN_POINT('Ctrl Pts',(4.30944892636032,5.22068366307949,10.5831613379781));
#11641=CARTESIAN_POINT('Ctrl Pts',(4.16280009466638,5.33510865604868,10.5919108829143));
#11642=CARTESIAN_POINT('Ctrl Pts',(4.01615988348775,5.44952692272901,10.6006599135226));
#11643=CARTESIAN_POINT('Ctrl Pts',(3.86479978232227,5.55789587288629,10.6094089441308));
#11644=CARTESIAN_POINT('Ctrl Pts',(3.70923383581073,5.65984746713874,10.6181579747391));
#11645=CARTESIAN_POINT('Ctrl Pts',(3.55366577799543,5.76180044505382,10.6269071240871));
#11646=CARTESIAN_POINT('Ctrl Pts',(3.39389200026838,5.8573357357106,10.6356562734352));
#11647=CARTESIAN_POINT('Ctrl Pts',(3.23045513626035,5.94612887621931,10.6444054227832));
#11648=CARTESIAN_POINT('Ctrl Pts',(3.18695122151575,5.9697639920669,10.6467342868961));
#11649=CARTESIAN_POINT('Ctrl Pts',(3.14318791262663,5.99292165435333,10.6490631510091));
#11650=CARTESIAN_POINT('Ctrl Pts',(3.09917575053259,6.01559628526639,10.6513920151221));
#11651=CARTESIAN_POINT('Origin',(0.,0.,-3.69717978381041));
#11652=CARTESIAN_POINT('',(3.09917575053261,6.01559628526638,13.045945719425));
#11653=CARTESIAN_POINT('',(3.09917575053257,6.0155962852664,12.6511155556306));
#11654=CARTESIAN_POINT('',(3.09917575053259,6.01559628526639,-3.69717978381041));
#11655=CARTESIAN_POINT('',(-6.76699833437543,-0.00474790060590539,11.6971797837751));
#11656=CARTESIAN_POINT('Ctrl Pts',(-6.76699833437491,-0.00474790134657525,
11.69717978381));
#11657=CARTESIAN_POINT('Ctrl Pts',(-6.76679660725303,-0.292261688620453,
11.7107429284341));
#11658=CARTESIAN_POINT('Ctrl Pts',(-6.74826864779524,-0.579070480480221,
11.7243060730581));
#11659=CARTESIAN_POINT('Ctrl Pts',(-6.71169741404573,-0.863369458743955,
11.7378692176821));
#11660=CARTESIAN_POINT('Ctrl Pts',(-6.70031069909056,-0.951887977143168,
11.7420921996791));
#11661=CARTESIAN_POINT('Ctrl Pts',(-6.6871750701465,-1.04016349819088,11.746315181676));
#11662=CARTESIAN_POINT('Ctrl Pts',(-6.67229977123769,-1.12814217310653,
11.7505381636729));
#11663=CARTESIAN_POINT('Ctrl Pts',(-6.64358823604027,-1.29795407651414,
11.7586891458472));
#11664=CARTESIAN_POINT('Ctrl Pts',(-6.60834472339372,-1.46693594567893,
11.7668401280215));
#11665=CARTESIAN_POINT('Ctrl Pts',(-6.5666250158011,-1.63454119001485,11.7749911101958));
#11666=CARTESIAN_POINT('Ctrl Pts',(-6.52495376951554,-1.80195174532542,
11.7831326242488));
#11667=CARTESIAN_POINT('Ctrl Pts',(-6.47682139022109,-1.96798850765806,
11.7912741383018));
#11668=CARTESIAN_POINT('Ctrl Pts',(-6.42233522229994,-2.13211146341031,
11.7994156523549));
#11669=CARTESIAN_POINT('Ctrl Pts',(-6.36790087922451,-2.29607831262788,
11.8075494225579));
#11670=CARTESIAN_POINT('Ctrl Pts',(-6.30712489355887,-2.45813463458681,
11.815683192761));
#11671=CARTESIAN_POINT('Ctrl Pts',(-6.24016531787777,-2.61775205196281,
11.8238169629641));
#11672=CARTESIAN_POINT('Ctrl Pts',(-6.17325534822217,-2.77725121910204,
11.831944707382));
#11673=CARTESIAN_POINT('Ctrl Pts',(-6.10017105095313,-2.93431474352113,
11.8400724518));
#11674=CARTESIAN_POINT('Ctrl Pts',(-6.02111982837664,-3.08843083334072,
11.848200196218));
#11675=CARTESIAN_POINT('Ctrl Pts',(-5.94211054982195,-3.24246515024876,
11.8563236281121));
#11676=CARTESIAN_POINT('Ctrl Pts',(-5.85714081766822,-3.39355482239924,
11.8644470600061));
#11677=CARTESIAN_POINT('Ctrl Pts',(-5.76646553451817,-3.54120943170749,
11.8725704919002));
#11678=CARTESIAN_POINT('Ctrl Pts',(-5.67521504303697,-3.68980070378044,
11.880745455651));
#11679=CARTESIAN_POINT('Ctrl Pts',(-5.57818651365921,-3.8349128373978,11.8889204194018));
#11680=CARTESIAN_POINT('Ctrl Pts',(-5.47568621780785,-3.97607211253885,
11.8970953831526));
#11681=CARTESIAN_POINT('Ctrl Pts',(-5.37385514939057,-4.11630975463763,
11.9052169723256));
#11682=CARTESIAN_POINT('Ctrl Pts',(-5.26662379139155,-4.25264571738984,
11.9133385614987));
#11683=CARTESIAN_POINT('Ctrl Pts',(-5.15433512035698,-4.38464576300693,
11.9214601506717));
#11684=CARTESIAN_POINT('Ctrl Pts',(-5.04203162491482,-4.51666323533733,
11.929582812061));
#11685=CARTESIAN_POINT('Ctrl Pts',(-4.92466972372092,-4.64434337155865,
11.9377054734504));
#11686=CARTESIAN_POINT('Ctrl Pts',(-4.8026316566751,-4.7672862479929,11.9458281348398));
#11687=CARTESIAN_POINT('Ctrl Pts',(-4.6805542384438,-4.8902687673685,11.953953415382));
#11688=CARTESIAN_POINT('Ctrl Pts',(-4.5537979095081,-5.00851072556508,11.9620786959243));
#11689=CARTESIAN_POINT('Ctrl Pts',(-4.42278057195902,-5.12165022354142,
11.9702039764665));
#11690=CARTESIAN_POINT('Ctrl Pts',(-4.29033582770329,-5.2360223528719,11.9784177802543));
#11691=CARTESIAN_POINT('Ctrl Pts',(-4.15353697598372,-5.34517993907141,
11.986631584042));
#11692=CARTESIAN_POINT('Ctrl Pts',(-4.01284791481315,-5.4487925830022,11.9948453878298));
#11693=CARTESIAN_POINT('Ctrl Pts',(-3.87343428221996,-5.5514659177504,12.002984728685));
#11694=CARTESIAN_POINT('Ctrl Pts',(-3.73020102221582,-5.64869428143773,
12.0111240695401));
#11695=CARTESIAN_POINT('Ctrl Pts',(-3.58362615654727,-5.74020143985473,
12.0192634103953));
#11696=CARTESIAN_POINT('Ctrl Pts',(-3.43503987597343,-5.83296433104378,
12.0275144456494));
#11697=CARTESIAN_POINT('Ctrl Pts',(-3.28301995323354,-5.91984766182591,
12.0357654809034));
#11698=CARTESIAN_POINT('Ctrl Pts',(-3.12808691313762,-6.00061340729906,
12.0440165161575));
#11699=CARTESIAN_POINT('Ctrl Pts',(-2.97315387304169,-6.08137915277221,
12.0522675514116));
#11700=CARTESIAN_POINT('Ctrl Pts',(-2.81530809128953,-6.15602720944744,
12.0605185866656));
#11701=CARTESIAN_POINT('Ctrl Pts',(-2.65508727394273,-6.22437149981807,
12.0687696219197));
#11702=CARTESIAN_POINT('Ctrl Pts',(-2.49524051503537,-6.29255623065688,
12.0770013939505));
#11703=CARTESIAN_POINT('Ctrl Pts',(-2.33253085409738,-6.35467961984619,
12.0852331659814));
#11704=CARTESIAN_POINT('Ctrl Pts',(-2.16745765985384,-6.41049267160808,
12.0934649380122));
#11705=CARTESIAN_POINT('Ctrl Pts',(-2.00258157950071,-6.46623907700853,
12.1016868804846));
#11706=CARTESIAN_POINT('Ctrl Pts',(-1.83534792177387,-6.51569003561539,
12.109908822957));
#11707=CARTESIAN_POINT('Ctrl Pts',(-1.66627804975084,-6.55864364491002,
12.1181307654294));
#11708=CARTESIAN_POINT('Ctrl Pts',(-1.49737618941545,-6.60155456943591,
12.1263445374193));
#11709=CARTESIAN_POINT('Ctrl Pts',(-1.32664209359358,-6.63798091548698,
12.1345583094092));
#11710=CARTESIAN_POINT('Ctrl Pts',(-1.15461447983466,-6.66776982228362,
12.1427720813991));
#11711=CARTESIAN_POINT('Ctrl Pts',(-0.982723362268644,-6.6975350929193,
12.1509793361294));
#11712=CARTESIAN_POINT('Ctrl Pts',(-0.809541122495328,-6.72067335318585,
12.1591865908598));
#11713=CARTESIAN_POINT('Ctrl Pts',(-0.635619022647368,-6.73708226594041,
12.1673938455901));
#11714=CARTESIAN_POINT('Ctrl Pts',(-0.461800097095261,-6.75348144457826,
12.1755962316021));
#11715=CARTESIAN_POINT('Ctrl Pts',(-0.287242541584296,-6.76315919466014,
12.183798617614));
#11716=CARTESIAN_POINT('Ctrl Pts',(-0.112505230085923,-6.76606470359273,
12.192001003626));
#11717=CARTESIAN_POINT('Ctrl Pts',(0.0621799265634823,-6.76896934530137,
12.2002009414247));
#11718=CARTESIAN_POINT('Ctrl Pts',(0.23704437457786,-6.76510576247856,12.2084008792234));
#11719=CARTESIAN_POINT('Ctrl Pts',(0.411526476122003,-6.75447518016393,
12.2166008170221));
#11720=CARTESIAN_POINT('Ctrl Pts',(0.585984180564948,-6.74384608427909,
12.2247996082578));
#11721=CARTESIAN_POINT('Ctrl Pts',(0.760059287329435,-6.72645189436287,
12.2329983994936));
#11722=CARTESIAN_POINT('Ctrl Pts',(0.933192499546701,-6.70234591458765,
12.2411971907293));
#11723=CARTESIAN_POINT('Ctrl Pts',(1.10633291053602,-6.67823893250068,12.2493963228658));
#11724=CARTESIAN_POINT('Ctrl Pts',(1.27853099392193,-6.64741965392924,12.2575954550022));
#11725=CARTESIAN_POINT('Ctrl Pts',(1.44923483975395,-6.60999299388762,12.2657945871386));
#11726=CARTESIAN_POINT('Ctrl Pts',(1.61997674979563,-6.57255798830329,12.2739955475495));
#11727=CARTESIAN_POINT('Ctrl Pts',(1.78922340862214,-6.5285127435271,12.2821965079604));
#11728=CARTESIAN_POINT('Ctrl Pts',(1.95643526729759,-6.47801281604739,12.2903974683713));
#11729=CARTESIAN_POINT('Ctrl Pts',(2.12380384373775,-6.42746555797872,12.2986061150564));
#11730=CARTESIAN_POINT('Ctrl Pts',(2.28913346618986,-6.37045163425554,12.3068147617414));
#11731=CARTESIAN_POINT('Ctrl Pts',(2.45190096910737,-6.30717612229834,12.3150234084265));
#11732=CARTESIAN_POINT('Ctrl Pts',(2.61474618180225,-6.24387040083458,12.32323597415));
#11733=CARTESIAN_POINT('Ctrl Pts',(2.77502650743805,-6.17429727330813,12.3314485398735));
#11734=CARTESIAN_POINT('Ctrl Pts',(2.93224088516228,-6.09870907581127,12.339661105597));
#11735=CARTESIAN_POINT('Ctrl Pts',(3.08967098369889,-6.02301716040001,12.3478849401458));
#11736=CARTESIAN_POINT('Ctrl Pts',(3.24402640969365,-5.9412938476673,12.3561087746945));
#11737=CARTESIAN_POINT('Ctrl Pts',(3.39483165528085,-5.85383694958299,12.3643326092433));
#11738=CARTESIAN_POINT('Ctrl Pts',(3.53339330817677,-5.77348051165853,12.3718887662177));
#11739=CARTESIAN_POINT('Ctrl Pts',(3.66895798881336,-5.68828431880963,12.3794449231921));
#11740=CARTESIAN_POINT('Ctrl Pts',(3.80118055163148,-5.59851010661753,12.3870010801665));
#11741=CARTESIAN_POINT('Ctrl Pts',(3.95246896479744,-5.4957908897434,12.3956467982189));
#11742=CARTESIAN_POINT('Ctrl Pts',(4.09972658582958,-5.38684383932133,12.4042925162713));
#11743=CARTESIAN_POINT('Ctrl Pts',(4.24243909134905,-5.27200147535957,12.4129382343236));
#11744=CARTESIAN_POINT('Ctrl Pts',(4.38496838309539,-5.15730654558895,12.421572853036));
#11745=CARTESIAN_POINT('Ctrl Pts',(4.52296395815918,-5.0367315843092,12.4302074717483));
#11746=CARTESIAN_POINT('Ctrl Pts',(4.6559410930395,-4.91065184452596,12.4388420904607));
#11747=CARTESIAN_POINT('Ctrl Pts',(4.79361446374846,-4.78011945811464,12.4477816503631));
#11748=CARTESIAN_POINT('Ctrl Pts',(4.92590817948129,-4.6436865385779,12.4567212102656));
#11749=CARTESIAN_POINT('Ctrl Pts',(5.05231999877382,-4.50181648115404,12.465660770168));
#11750=CARTESIAN_POINT('Ctrl Pts',(5.17408084126512,-4.36516614408195,12.4742714234385));
#11751=CARTESIAN_POINT('Ctrl Pts',(5.2903846176042,-4.22347185069932,12.482882076709));
#11752=CARTESIAN_POINT('Ctrl Pts',(5.40081814768467,-4.07718681637719,12.4914927299795));
#11753=CARTESIAN_POINT('Ctrl Pts',(5.51114714504044,-3.93104025062714,12.5000952326906));
#11754=CARTESIAN_POINT('Ctrl Pts',(5.61561679131165,-3.78031185019857,12.5086977354017));
#11755=CARTESIAN_POINT('Ctrl Pts',(5.71385338961835,-3.62548871766923,12.5173002381128));
#11756=CARTESIAN_POINT('Ctrl Pts',(5.81197942461125,-3.47083983545883,12.5258930588803));
#11757=CARTESIAN_POINT('Ctrl Pts',(5.90388624363981,-3.31210567202316,12.5344858796478));
#11758=CARTESIAN_POINT('Ctrl Pts',(5.98924267277715,-3.14980335998697,12.5430787004152));
#11759=CARTESIAN_POINT('Ctrl Pts',(5.99930231566164,-3.13067529529504,12.5440914033734));
#11760=CARTESIAN_POINT('Ctrl Pts',(6.00927102467809,-3.11149770383693,12.5451041063317));
#11761=CARTESIAN_POINT('Ctrl Pts',(6.01914829737112,-3.09227145869413,12.5461168092899));
#11762=CARTESIAN_POINT('Ctrl Pts',(6.10298107782584,-2.92908981553044,12.55471206705));
#11763=CARTESIAN_POINT('Ctrl Pts',(6.18012472976184,-2.76259324032409,12.56330732481));
#11764=CARTESIAN_POINT('Ctrl Pts',(6.25034575254777,-2.59335053041583,12.5719025825701));
#11765=CARTESIAN_POINT('Ctrl Pts',(6.32063253434351,-2.42394933188722,12.5805058894245));
#11766=CARTESIAN_POINT('Ctrl Pts',(6.38398363015338,-2.25179714760198,12.5891091962789));
#11767=CARTESIAN_POINT('Ctrl Pts',(6.44021471850249,-2.07748005515912,12.5977125031334));
#11768=CARTESIAN_POINT('Ctrl Pts',(6.49877716727391,-1.89593571561534,12.6066725060734));
#11769=CARTESIAN_POINT('Ctrl Pts',(6.54961652787162,-1.71204349383505,12.6156325090134));
#11770=CARTESIAN_POINT('Ctrl Pts',(6.59258318849465,-1.52647826803324,12.6245925119534));
#11771=CARTESIAN_POINT('Ctrl Pts',(6.63395222003498,-1.34781291290278,12.6332193551581));
#11772=CARTESIAN_POINT('Ctrl Pts',(6.66802344626706,-1.16759702429153,12.6418461983628));
#11773=CARTESIAN_POINT('Ctrl Pts',(6.69471625732958,-0.986439675726336,
12.6504730415676));
#11774=CARTESIAN_POINT('Ctrl Pts',(6.72143457997201,-0.805109186529252,
12.6591081298537));
#11775=CARTESIAN_POINT('Ctrl Pts',(6.74076037604901,-0.622835744093636,
12.6677432181398));
#11776=CARTESIAN_POINT('Ctrl Pts',(6.75266500716457,-0.440232099028653,
12.676378306426));
#11777=CARTESIAN_POINT('Ctrl Pts',(6.76458731904638,-0.257357250905425,
12.6850262195511));
#11778=CARTESIAN_POINT('Ctrl Pts',(6.76906642854844,-0.0741515248676813,
12.6936741326763));
#11779=CARTESIAN_POINT('Ctrl Pts',(6.76612574469661,0.10877227106996,12.7023220458014));
#11780=CARTESIAN_POINT('Ctrl Pts',(6.76579584473498,0.12929353629372,12.7032922100054));
#11781=CARTESIAN_POINT('Ctrl Pts',(6.76537261721316,0.149811258896166,12.7042623742094));
#11782=CARTESIAN_POINT('Ctrl Pts',(6.76485613579447,0.17032457839058,12.7052325384133));
#11783=CARTESIAN_POINT('Ctrl Pts',(6.76047760468728,0.344228622693202,12.7134572179321));
#11784=CARTESIAN_POINT('Ctrl Pts',(6.74938317409022,0.518192896016715,12.7216818974509));
#11785=CARTESIAN_POINT('Ctrl Pts',(6.731559778019,0.691658842896419,12.7299065769697));
#11786=CARTESIAN_POINT('Ctrl Pts',(6.71375511635345,0.864942457441293,12.7381226114198));
#11787=CARTESIAN_POINT('Ctrl Pts',(6.68923561020222,1.03772843500376,12.74633864587));
#11788=CARTESIAN_POINT('Ctrl Pts',(6.65804019558089,1.20945845485869,12.7545546803201));
#11789=CARTESIAN_POINT('Ctrl Pts',(6.62687132237308,1.38104236485982,12.7627637244747));
#11790=CARTESIAN_POINT('Ctrl Pts',(6.58903791666403,1.55157175580109,12.7709727686293));
#11791=CARTESIAN_POINT('Ctrl Pts',(6.54463069083944,1.72049356886983,12.7791818127839));
#11792=CARTESIAN_POINT('Ctrl Pts',(6.50025235485443,1.88930548711878,12.787385516412));
#11793=CARTESIAN_POINT('Ctrl Pts',(6.44930880837135,2.05651156530519,12.79558922004));
#11794=CARTESIAN_POINT('Ctrl Pts',(6.39194182025092,2.22156898756877,12.803792923668));
#11795=CARTESIAN_POINT('Ctrl Pts',(6.33460066802595,2.38655207428771,12.811992932662));
#11796=CARTESIAN_POINT('Ctrl Pts',(6.27084195498384,2.54938809510271,12.820192941656));
#11797=CARTESIAN_POINT('Ctrl Pts',(6.20085729943392,2.70954936328111,12.8283929506499));
#11798=CARTESIAN_POINT('Ctrl Pts',(6.13087824000474,2.86969782462654,12.8365923039539));
#11799=CARTESIAN_POINT('Ctrl Pts',(6.05467436508159,3.02717162767248,12.8447916572578));
#11800=CARTESIAN_POINT('Ctrl Pts',(5.97248558667473,3.18146270085988,12.8529910105618));
#11801=CARTESIAN_POINT('Ctrl Pts',(5.89029734411442,3.33575276811507,12.8611903104083));
#11802=CARTESIAN_POINT('Ctrl Pts',(5.80212444338723,3.48685982991059,12.8693896102549));
#11803=CARTESIAN_POINT('Ctrl Pts',(5.70825289195924,3.63430019693462,12.8775889101015));
#11804=CARTESIAN_POINT('Ctrl Pts',(5.6143649233254,3.78176634982049,12.8857896439245));
#11805=CARTESIAN_POINT('Ctrl Pts',(5.51477651090571,3.92556422788545,12.8939903777476));
#11806=CARTESIAN_POINT('Ctrl Pts',(5.40981717072618,4.0652388834257,12.9021911115706));
#11807=CARTESIAN_POINT('Ctrl Pts',(5.30482043333558,4.20496330530943,12.9103947673306));
#11808=CARTESIAN_POINT('Ctrl Pts',(5.19444917129497,4.34056129168992,12.9185984230905));
#11809=CARTESIAN_POINT('Ctrl Pts',(5.07907340035507,4.47161071581657,12.9268020788505));
#11810=CARTESIAN_POINT('Ctrl Pts',(4.9635654590525,4.60281026548321,12.9350151324255));
#11811=CARTESIAN_POINT('Ctrl Pts',(4.84304179239248,4.72945057342195,12.9432281860005));
#11812=CARTESIAN_POINT('Ctrl Pts',(4.7179102683927,4.85114540076823,12.9514412395756));
#11813=CARTESIAN_POINT('Ctrl Pts',(4.59270470126281,4.9729122376741,12.9596591529986));
#11814=CARTESIAN_POINT('Ctrl Pts',(4.46288610777912,5.08972752126063,12.9678770664217));
#11815=CARTESIAN_POINT('Ctrl Pts',(4.32889560573564,5.20124521962219,12.9760949798448));
#11816=CARTESIAN_POINT('Ctrl Pts',(4.19469612370625,5.31293684797637,12.9843257104408));
#11817=CARTESIAN_POINT('Ctrl Pts',(4.05631201387683,5.41931416084593,12.9925564410368));
#11818=CARTESIAN_POINT('Ctrl Pts',(3.91421464953569,5.52007361158891,13.0007871716328));
#11819=CARTESIAN_POINT('Ctrl Pts',(3.78371521490937,5.61260911649559,13.0083461133085));
#11820=CARTESIAN_POINT('Ctrl Pts',(3.65008444115707,5.70040679342884,13.0159050549843));
#11821=CARTESIAN_POINT('Ctrl Pts',(3.5137049190326,5.78326609641698,13.0234639966601));
#11822=CARTESIAN_POINT('Ctrl Pts',(3.37849875134788,5.86541251135917,13.0309579042484));
#11823=CARTESIAN_POINT('Ctrl Pts',(3.24020677386849,5.94293849593535,13.0384518118367));
#11824=CARTESIAN_POINT('Ctrl Pts',(3.09917575053261,6.01559628526638,13.045945719425));
#11825=CARTESIAN_POINT('Ctrl Pts',(3.0991757505326,6.01559628526638,11.0455440641533));
#11826=CARTESIAN_POINT('Ctrl Pts',(2.94526730765652,6.09488839386949,11.0536823803998));
#11827=CARTESIAN_POINT('Ctrl Pts',(2.78844847615828,6.16820072942692,11.0618206966463));
#11828=CARTESIAN_POINT('Ctrl Pts',(2.62923474293037,6.23533589043669,11.0699590128928));
#11829=CARTESIAN_POINT('Ctrl Pts',(2.46978442865988,6.30257080984081,11.0781094221373));
#11830=CARTESIAN_POINT('Ctrl Pts',(2.30793244489111,6.36361008803655,11.0862598313817));
#11831=CARTESIAN_POINT('Ctrl Pts',(2.14421045009698,6.41830589374602,11.0944102406261));
#11832=CARTESIAN_POINT('Ctrl Pts',(2.01253632167944,6.46229523405394,11.1009652428105));
#11833=CARTESIAN_POINT('Ctrl Pts',(1.8796529631955,6.50218241470288,11.1075202449948));
#11834=CARTESIAN_POINT('Ctrl Pts',(1.74584106724889,6.5379146497876,11.1140752471792));
#11835=CARTESIAN_POINT('Ctrl Pts',(1.57794102589216,6.58274955557868,11.1223001148568));
#11836=CARTESIAN_POINT('Ctrl Pts',(1.40807705294203,6.62117549259409,11.1305249825344));
#11837=CARTESIAN_POINT('Ctrl Pts',(1.23677946429998,6.65301928125012,11.138749850212));
#11838=CARTESIAN_POINT('Ctrl Pts',(1.06567486156505,6.68482719431392,11.1469654516555));
#11839=CARTESIAN_POINT('Ctrl Pts',(0.893140208782343,6.71006766024843,11.1551810530991));
#11840=CARTESIAN_POINT('Ctrl Pts',(0.719720638582738,6.72861733214173,11.1633966545426));
#11841=CARTESIAN_POINT('Ctrl Pts',(0.546461601468275,6.74714983275468,11.1716046508707));
#11842=CARTESIAN_POINT('Ctrl Pts',(0.372319632799995,6.75900383611599,11.1798126471989));
#11843=CARTESIAN_POINT('Ctrl Pts',(0.197849799874018,6.76410707016749,11.188020643527));
#11844=CARTESIAN_POINT('Ctrl Pts',(0.0235064290797352,6.76920660520784,
11.1962226903985));
#11845=CARTESIAN_POINT('Ctrl Pts',(-0.151163975458657,6.76756510683125,
11.2044247372699));
#11846=CARTESIAN_POINT('Ctrl Pts',(-0.325601393170112,6.75916213245146,
11.2126267841414));
#11847=CARTESIAN_POINT('Ctrl Pts',(-0.499947400840036,6.75076356146313,
11.2208245329129));
#11848=CARTESIAN_POINT('Ctrl Pts',(-0.674060307402147,6.73561059031559,
11.2290222816845));
#11849=CARTESIAN_POINT('Ctrl Pts',(-0.847380170823765,6.71373486563885,
11.237220030456));
#11850=CARTESIAN_POINT('Ctrl Pts',(-1.02066697696245,6.69186331331723,11.2454162156717));
#11851=CARTESIAN_POINT('Ctrl Pts',(-1.19316068488015,6.66327160021774,11.2536124008873));
#11852=CARTESIAN_POINT('Ctrl Pts',(-1.36430624382287,6.62804326125486,11.2618085861029));
#11853=CARTESIAN_POINT('Ctrl Pts',(-1.53543914180346,6.59281752840498,11.2700041649833));
#11854=CARTESIAN_POINT('Ctrl Pts',(-1.70522373779388,6.55095621892385,11.2781997438636));
#11855=CARTESIAN_POINT('Ctrl Pts',(-1.87311500420352,6.5025940347701,11.286395322744));
#11856=CARTESIAN_POINT('Ctrl Pts',(-2.04102439622373,6.45422662941494,11.2945917864224));
#11857=CARTESIAN_POINT('Ctrl Pts',(-2.20703970654683,6.39935705045834,11.3027882501009));
#11858=CARTESIAN_POINT('Ctrl Pts',(-2.3706308569867,6.33816995195794,11.3109847137793));
#11859=CARTESIAN_POINT('Ctrl Pts',(-2.53426943239221,6.27696511535841,11.3191835536071));
#11860=CARTESIAN_POINT('Ctrl Pts',(-2.69548211209535,6.20943923688715,11.3273823934349));
#11861=CARTESIAN_POINT('Ctrl Pts',(-2.85375854749797,6.13582522180858,11.3355812332627));
#11862=CARTESIAN_POINT('Ctrl Pts',(-3.01220030714001,6.06213431479708,11.343788637012));
#11863=CARTESIAN_POINT('Ctrl Pts',(-3.16769936923715,5.98234271779002,11.3519960407612));
#11864=CARTESIAN_POINT('Ctrl Pts',(-3.31976887326136,5.89672990971479,11.3602034445105));
#11865=CARTESIAN_POINT('Ctrl Pts',(-3.4719198337594,5.81107124288895,11.3684152445795));
#11866=CARTESIAN_POINT('Ctrl Pts',(-3.62063726863101,5.71958533672074,11.3766270446485));
#11867=CARTESIAN_POINT('Ctrl Pts',(-3.76546320619158,5.62259511638687,11.3848388447175));
#11868=CARTESIAN_POINT('Ctrl Pts',(-3.91050234776854,5.52546211289637,11.3930627337037));
#11869=CARTESIAN_POINT('Ctrl Pts',(-4.05163825293761,5.42280881245052,11.4012866226898));
#11870=CARTESIAN_POINT('Ctrl Pts',(-4.18844493344157,5.31499934520482,11.409510511676));
#11871=CARTESIAN_POINT('Ctrl Pts',(-4.31485194113688,5.21538526126131,11.417109242926));
#11872=CARTESIAN_POINT('Ctrl Pts',(-4.43756311217769,5.11136971193684,11.424707974176));
#11873=CARTESIAN_POINT('Ctrl Pts',(-4.55627102392818,5.00326726814714,11.432306705426));
#11874=CARTESIAN_POINT('Ctrl Pts',(-4.68269534251505,4.88813780801127,11.4403993793367));
#11875=CARTESIAN_POINT('Ctrl Pts',(-4.80495912097062,4.76802573065788,11.4484920532473));
#11876=CARTESIAN_POINT('Ctrl Pts',(-4.92263669390666,4.64326792031256,11.4565847271579));
#11877=CARTESIAN_POINT('Ctrl Pts',(-5.04018015380373,4.51865229210666,11.4646681781294));
#11878=CARTESIAN_POINT('Ctrl Pts',(-5.15314755820498,4.38940173596641,11.472751629101));
#11879=CARTESIAN_POINT('Ctrl Pts',(-5.26114657768875,4.25589305411614,11.4808350800725));
#11880=CARTESIAN_POINT('Ctrl Pts',(-5.36904598642814,4.1225075113392,11.488911075434));
#11881=CARTESIAN_POINT('Ctrl Pts',(-5.47198589985088,3.98487194762242,11.4969870707955));
#11882=CARTESIAN_POINT('Ctrl Pts',(-5.56961117993759,3.84339957645757,11.505063066157));
#11883=CARTESIAN_POINT('Ctrl Pts',(-5.66716307474747,3.70203355058679,11.5131329907636));
#11884=CARTESIAN_POINT('Ctrl Pts',(-5.75940808218336,3.55683676572979,11.5212029153701));
#11885=CARTESIAN_POINT('Ctrl Pts',(-5.84603177669574,3.40825490036524,11.5292728399766));
#11886=CARTESIAN_POINT('Ctrl Pts',(-5.93261980712226,3.25973420806001,11.5373394420917));
#11887=CARTESIAN_POINT('Ctrl Pts',(-6.01359094311208,3.10783152885777,11.5454060442068));
#11888=CARTESIAN_POINT('Ctrl Pts',(-6.08867442380893,2.95302095503147,11.5534726463219));
#11889=CARTESIAN_POINT('Ctrl Pts',(-6.16374173956836,2.79824371081665,11.5615375117552));
#11890=CARTESIAN_POINT('Ctrl Pts',(-6.2329237609722,2.64056015226075,11.5696023771884));
#11891=CARTESIAN_POINT('Ctrl Pts',(-6.29599604673013,2.48046825812358,11.5776672426217));
#11892=CARTESIAN_POINT('Ctrl Pts',(-6.35906714163235,2.3203793866507,11.5857319557837));
#11893=CARTESIAN_POINT('Ctrl Pts',(-6.41602859524056,2.15788261623926,11.5937966689458));
#11894=CARTESIAN_POINT('Ctrl Pts',(-6.46670445829191,1.99349503363001,11.6018613821078));
#11895=CARTESIAN_POINT('Ctrl Pts',(-6.51741120481266,1.8290072680427,11.6099310101605));
#11896=CARTESIAN_POINT('Ctrl Pts',(-6.56182459634185,1.66262674320034,11.6180006382131));
#11897=CARTESIAN_POINT('Ctrl Pts',(-6.59981868985138,1.49488536720662,11.6260702662658));
#11898=CARTESIAN_POINT('Ctrl Pts',(-6.63782396935663,1.3270946057916,11.6341422701305));
#11899=CARTESIAN_POINT('Ctrl Pts',(-6.66940611446372,1.15794255987394,11.6422142739952));
#11900=CARTESIAN_POINT('Ctrl Pts',(-6.6944905870027,0.987970030179167,11.6502862778599));
#11901=CARTESIAN_POINT('Ctrl Pts',(-6.71960330689822,0.817806096234619,
11.6583673715219));
#11902=CARTESIAN_POINT('Ctrl Pts',(-6.73820369187974,0.646820201885291,
11.6664484651839));
#11903=CARTESIAN_POINT('Ctrl Pts',(-6.75026915953388,0.475557855413853,
11.6745295588459));
#11904=CARTESIAN_POINT('Ctrl Pts',(-6.7615417903465,0.315549370105564,11.6820796338223));
#11905=CARTESIAN_POINT('Ctrl Pts',(-6.76711062799904,0.15529983985892,11.6896297087987));
#11906=CARTESIAN_POINT('Ctrl Pts',(-6.76699833437543,-0.0047479006059271,
11.6971797837751));
#11907=CARTESIAN_POINT('',(-6.76751319450492,-0.0015787245738949,11.3037082475646));
#11908=CARTESIAN_POINT('Ctrl Pts',(3.09917575053259,6.01559628526639,10.6513920151221));
#11909=CARTESIAN_POINT('Ctrl Pts',(2.93382384459261,6.10078395293761,10.6601414630345));
#11910=CARTESIAN_POINT('Ctrl Pts',(2.76495772122975,6.17915010267053,10.6688909109469));
#11911=CARTESIAN_POINT('Ctrl Pts',(2.59315093316697,6.25042856433183,10.6776403588593));
#11912=CARTESIAN_POINT('Ctrl Pts',(2.42134553245603,6.32170645041457,10.6863897361193));
#11913=CARTESIAN_POINT('Ctrl Pts',(2.24659977927576,6.38589665313462,10.6951391133793));
#11914=CARTESIAN_POINT('Ctrl Pts',(2.06950718689904,6.4427811543908,10.7038884906393));
#11915=CARTESIAN_POINT('Ctrl Pts',(1.89241596572852,6.49966521519726,10.712637800154));
#11916=CARTESIAN_POINT('Ctrl Pts',(1.71297821457194,6.54924360009547,10.7213871096686));
#11917=CARTESIAN_POINT('Ctrl Pts',(1.53180337335847,6.59134792173556,10.7301364191833));
#11918=CARTESIAN_POINT('Ctrl Pts',(1.35062987477783,6.63345193135305,10.7388856638594));
#11919=CARTESIAN_POINT('Ctrl Pts',(1.16771959102949,6.66808192368238,10.7476349085355));
#11920=CARTESIAN_POINT('Ctrl Pts',(0.983693746906791,6.69512028363169,10.7563841532117));
#11921=CARTESIAN_POINT('Ctrl Pts',(0.799669205419814,6.72215845218868,10.7651333359558));
#11922=CARTESIAN_POINT('Ctrl Pts',(0.614529402873416,6.7416050542458,10.7738825187));
#11923=CARTESIAN_POINT('Ctrl Pts',(0.428903127363185,6.75339404354122,10.7826317014442));
#11924=CARTESIAN_POINT('Ctrl Pts',(0.243278104163724,6.76518295330331,10.7913808251628));
#11925=CARTESIAN_POINT('Ctrl Pts',(0.0571669005388728,6.76931433552276,
10.8001299488814));
#11926=CARTESIAN_POINT('Ctrl Pts',(-0.128798404777849,6.76577415902472,
10.8088790726));
#11927=CARTESIAN_POINT('Ctrl Pts',(-0.314762517259335,6.7622340052344,10.8176281401992));
#11928=CARTESIAN_POINT('Ctrl Pts',(-0.500580446819649,6.75102239665088,
10.8263772077984));
#11929=CARTESIAN_POINT('Ctrl Pts',(-0.685621118842651,6.73217741012497,
10.8351262753976));
#11930=CARTESIAN_POINT('Ctrl Pts',(-0.870660665414531,6.71333253821771,
10.8438752897834));
#11931=CARTESIAN_POINT('Ctrl Pts',(-1.05492267885491,6.68685441030611,10.8526243041692));
#11932=CARTESIAN_POINT('Ctrl Pts',(-1.23778137635257,6.65283295028176,10.861373318555));
#11933=CARTESIAN_POINT('Ctrl Pts',(-1.42999922978852,6.61707018861864,10.8705701289224));
#11934=CARTESIAN_POINT('Ctrl Pts',(-1.62066601233702,6.57297172934411,10.8797669392898));
#11935=CARTESIAN_POINT('Ctrl Pts',(-1.80906628500392,6.52070304311292,10.8889637496572));
#11936=CARTESIAN_POINT('Ctrl Pts',(-1.98831342545534,6.47097374915028,10.8977137473949));
#11937=CARTESIAN_POINT('Ctrl Pts',(-2.16550875896709,6.41384933989526,10.9064637451327));
#11938=CARTESIAN_POINT('Ctrl Pts',(-2.34005036714018,6.34952386240473,10.9152137428704));
#11939=CARTESIAN_POINT('Ctrl Pts',(-2.51458843547101,6.28519968948591,10.9239635631513));
#11940=CARTESIAN_POINT('Ctrl Pts',(-2.68647261718072,6.21367483971092,10.9327133834322));
#11941=CARTESIAN_POINT('Ctrl Pts',(-2.85511905908752,6.13519226743834,10.9414632037131));
#11942=CARTESIAN_POINT('Ctrl Pts',(-3.02376230488894,6.05671118252932,10.9502128581716));
#11943=CARTESIAN_POINT('Ctrl Pts',(-3.18916767379903,5.97127275992633,10.9589625126301));
#11944=CARTESIAN_POINT('Ctrl Pts',(-3.35077334102776,5.87916720438003,10.9677121670886));
#11945=CARTESIAN_POINT('Ctrl Pts',(-3.51237616037357,5.7870632719565,10.9764616673571));
#11946=CARTESIAN_POINT('Ctrl Pts',(-3.67017916302288,5.68829258362306,10.9852111676255));
#11947=CARTESIAN_POINT('Ctrl Pts',(-3.82364636566451,5.5831906174105,10.993960667894));
#11948=CARTESIAN_POINT('Ctrl Pts',(-3.9771110677879,5.47809036367708,11.0027100256024));
#11949=CARTESIAN_POINT('Ctrl Pts',(-4.12623987481921,5.36665920043229,11.0114593833108));
#11950=CARTESIAN_POINT('Ctrl Pts',(-4.27052628213927,5.24927559512337,11.0202087410193));
#11951=CARTESIAN_POINT('Ctrl Pts',(-4.41481053024971,5.13189374643042,11.0289579677958));
#11952=CARTESIAN_POINT('Ctrl Pts',(-4.5542523013652,5.00855981477362,11.0377071945723));
#11953=CARTESIAN_POINT('Ctrl Pts',(-4.68837800630534,4.8796926819209,11.0464564213488));
#11954=CARTESIAN_POINT('Ctrl Pts',(-4.82250188228878,4.75082730631826,11.0552055288197));
#11955=CARTESIAN_POINT('Ctrl Pts',(-4.95130963052948,4.61642907903545,11.0639546362905));
#11956=CARTESIAN_POINT('Ctrl Pts',(-5.07436379033348,4.47695444731711,11.0727037437614));
#11957=CARTESIAN_POINT('Ctrl Pts',(-5.19741643562762,4.33748153220637,11.0814527435511));
#11958=CARTESIAN_POINT('Ctrl Pts',(-5.31471544462707,4.19293255254671,11.0902017433408));
#11959=CARTESIAN_POINT('Ctrl Pts',(-5.42586245275542,4.04379841779717,11.0989507431305));
#11960=CARTESIAN_POINT('Ctrl Pts',(-5.53702160019068,3.89464799484463,11.1077006984727));
#11961=CARTESIAN_POINT('Ctrl Pts',(-5.64202723081167,3.74091164443977,11.1164506538148));
#11962=CARTESIAN_POINT('Ctrl Pts',(-5.74052265232884,3.58311159163366,11.125200609157));
#11963=CARTESIAN_POINT('Ctrl Pts',(-5.83901427066841,3.42531763191915,11.1339502266394));
#11964=CARTESIAN_POINT('Ctrl Pts',(-5.93099603115669,3.26346052695742,11.1426998441219));
#11965=CARTESIAN_POINT('Ctrl Pts',(-6.01615550622689,3.09809004467203,11.1514494616043));
#11966=CARTESIAN_POINT('Ctrl Pts',(-6.1013121457874,2.93272506863952,11.1601987877554));
#11967=CARTESIAN_POINT('Ctrl Pts',(-6.17964682328694,2.76384720417015,11.1689481139065));
#11968=CARTESIAN_POINT('Ctrl Pts',(-6.25089348288515,2.59203002791711,11.1776974400576));
#11969=CARTESIAN_POINT('Ctrl Pts',(-6.32213814889292,2.42021765937131,11.1864465213892));
#11970=CARTESIAN_POINT('Ctrl Pts',(-6.38629508412556,2.24546640832003,11.1951956027208));
#11971=CARTESIAN_POINT('Ctrl Pts',(-6.4431463981979,2.0683697666011,11.2039446840524));
#11972=CARTESIAN_POINT('Ctrl Pts',(-6.50000285283682,1.89125711158338,11.2126945564868));
#11973=CARTESIAN_POINT('Ctrl Pts',(-6.54955227673235,1.71179891440311,11.2214444289212));
#11974=CARTESIAN_POINT('Ctrl Pts',(-6.59162635926374,1.5306047627848,11.2301943013556));
#11975=CARTESIAN_POINT('Ctrl Pts',(-6.63369752055189,1.34942319164735,11.2389435662781));
#11976=CARTESIAN_POINT('Ctrl Pts',(-6.66829431424249,1.16650618642733,11.2476928312006));
#11977=CARTESIAN_POINT('Ctrl Pts',(-6.69529923745415,0.982474997618738,
11.2564420961231));
#11978=CARTESIAN_POINT('Ctrl Pts',(-6.72230554731441,0.79843435917792,11.2651918103028));
#11979=CARTESIAN_POINT('Ctrl Pts',(-6.74171916496701,0.613279706240516,
11.2739415244825));
#11980=CARTESIAN_POINT('Ctrl Pts',(-6.75347414817274,0.427639953655554,
11.2826912386622));
#11981=CARTESIAN_POINT('Ctrl Pts',(-6.76248837758744,0.285283364198654,
11.2894008978381));
#11982=CARTESIAN_POINT('Ctrl Pts',(-6.76699999999997,0.142641701105099,
11.296110557014));
#11983=CARTESIAN_POINT('Ctrl Pts',(-6.767,1.45413500768681E-12,11.3028202161899));
#11984=CARTESIAN_POINT('Ctrl Pts',(-6.76699905057905,-0.0035846146663836,
11.3028202161899));
#11985=CARTESIAN_POINT('Ctrl Pts',(-6.76689717948375,-0.195895830608512,
11.3118251661962));
#11986=CARTESIAN_POINT('Ctrl Pts',(-6.75859330496265,-0.387925714519049,
11.3208301162025));
#11987=CARTESIAN_POINT('Ctrl Pts',(-6.74218372926967,-0.579005665577984,
11.3298350662088));
#11988=CARTESIAN_POINT('Ctrl Pts',(-6.72531576528353,-0.775423281318799,
11.3390915622477));
#11989=CARTESIAN_POINT('Ctrl Pts',(-6.69988280524364,-0.970836849582827,
11.3483480582867));
#11990=CARTESIAN_POINT('Ctrl Pts',(-6.66604400647577,-1.1645369482024,11.3576045543256));
#11991=CARTESIAN_POINT('Ctrl Pts',(-6.63287135500348,-1.35442388555294,
11.3666788278854));
#11992=CARTESIAN_POINT('Ctrl Pts',(-6.59162085975679,-1.54266400819156,
11.3757531014452));
#11993=CARTESIAN_POINT('Ctrl Pts',(-6.5424921374319,-1.72860800404308,11.384827375005));
#11994=CARTESIAN_POINT('Ctrl Pts',(-6.4918835681219,-1.92015297318757,11.3941749822836));
#11995=CARTESIAN_POINT('Ctrl Pts',(-6.43291490559951,-2.10926107711814,
11.4035225895621));
#11996=CARTESIAN_POINT('Ctrl Pts',(-6.36585668772188,-2.29524674738613,
11.4128701968406));
#11997=CARTESIAN_POINT('Ctrl Pts',(-6.29879846984425,-2.48123241765411,
11.4222178041192));
#11998=CARTESIAN_POINT('Ctrl Pts',(-6.22365085991296,-2.66409544755373,
11.4315654113977));
#11999=CARTESIAN_POINT('Ctrl Pts',(-6.1407351238976,-2.84317799972677,11.4409130186762));
#12000=CARTESIAN_POINT('Ctrl Pts',(-6.06839406204169,-2.99942122455524,
11.449068477083));
#12001=CARTESIAN_POINT('Ctrl Pts',(-5.98996799741044,-3.15315655311691,
11.4572239354898));
#12002=CARTESIAN_POINT('Ctrl Pts',(-5.90565223682026,-3.30387055704969,
11.4653793938966));
#12003=CARTESIAN_POINT('Ctrl Pts',(-5.82143909959385,-3.45440112222866,
11.4735249260385));
#12004=CARTESIAN_POINT('Ctrl Pts',(-5.7313507121931,-3.60191736723609,11.4816704581804));
#12005=CARTESIAN_POINT('Ctrl Pts',(-5.63563049261017,-3.74592551324269,
11.4898159903223));
#12006=CARTESIAN_POINT('Ctrl Pts',(-5.54000664907487,-3.88978866443002,
11.4979533211228));
#12007=CARTESIAN_POINT('Ctrl Pts',(-5.43876246296973,-4.03015044635292,
11.5060906519234));
#12008=CARTESIAN_POINT('Ctrl Pts',(-5.33218733651383,-4.16654139644881,
11.5142279827239));
#12009=CARTESIAN_POINT('Ctrl Pts',(-5.22569711829203,-4.30282368409123,
11.5223588305259));
#12010=CARTESIAN_POINT('Ctrl Pts',(-5.11388464032455,-4.43514115227457,
11.5304896783279));
#12011=CARTESIAN_POINT('Ctrl Pts',(-4.99708270305726,-4.56305308524961,
11.5386205261299));
#12012=CARTESIAN_POINT('Ctrl Pts',(-4.88034928543937,-4.69088998110619,
11.5467466041237));
#12013=CARTESIAN_POINT('Ctrl Pts',(-4.7586324833724,-4.81432621935578,11.5548726821175));
#12014=CARTESIAN_POINT('Ctrl Pts',(-4.63230547684412,-4.93295398004076,
11.5629987601113));
#12015=CARTESIAN_POINT('Ctrl Pts',(-4.50553053782335,-5.05200237309867,
11.5711536516935));
#12016=CARTESIAN_POINT('Ctrl Pts',(-4.37411287423625,-5.16620783683439,
11.5793085432757));
#12017=CARTESIAN_POINT('Ctrl Pts',(-4.23846754166975,-5.27519496305227,
11.5874634348579));
#12018=CARTESIAN_POINT('Ctrl Pts',(-4.10335117847325,-5.38375707758414,
11.5955865252142));
#12019=CARTESIAN_POINT('Ctrl Pts',(-3.96404035782896,-5.48714126357408,
11.6037096155705));
#12020=CARTESIAN_POINT('Ctrl Pts',(-3.82097874921737,-5.58501659782934,
11.6118327059268));
#12021=CARTESIAN_POINT('Ctrl Pts',(-3.67790590675518,-5.68289961770267,
11.6199564341452));
#12022=CARTESIAN_POINT('Ctrl Pts',(-3.53108199156581,-5.77527271758845,
11.6280801623636));
#12023=CARTESIAN_POINT('Ctrl Pts',(-3.38097978101672,-5.86184823416268,
11.6362038905821));
#12024=CARTESIAN_POINT('Ctrl Pts',(-3.23083722698936,-5.94844701993101,
11.6443298022424));
#12025=CARTESIAN_POINT('Ctrl Pts',(-3.07741493989091,-6.02924493694812,
11.6524557139027));
#12026=CARTESIAN_POINT('Ctrl Pts',(-2.9212103740452,-6.10400024169157,11.660581625563));
#12027=CARTESIAN_POINT('Ctrl Pts',(-2.76400686376333,-6.17923361437971,
11.6687595032731));
#12028=CARTESIAN_POINT('Ctrl Pts',(-2.60398570409236,-6.24834665812697,
11.6769373809832));
#12029=CARTESIAN_POINT('Ctrl Pts',(-2.4416736627962,-6.31114242624958,11.6851152586932));
#12030=CARTESIAN_POINT('Ctrl Pts',(-2.28013630166992,-6.37363848379047,
11.6932541051667));
#12031=CARTESIAN_POINT('Ctrl Pts',(-2.11633024476488,-6.42987737492793,
11.7013929516401));
#12032=CARTESIAN_POINT('Ctrl Pts',(-1.95078891128069,-6.47971539680751,
11.7095317981135));
#12033=CARTESIAN_POINT('Ctrl Pts',(-1.78405675493559,-6.52991192888239,
11.7177291914419));
#12034=CARTESIAN_POINT('Ctrl Pts',(-1.61556462809543,-6.57361506025311,
11.7259265847703));
#12035=CARTESIAN_POINT('Ctrl Pts',(-1.44586647194078,-6.61073060601607,
11.7341239780987));
#12036=CARTESIAN_POINT('Ctrl Pts',(-1.27616831578612,-6.64784615177903,
11.7423213714271));
#12037=CARTESIAN_POINT('Ctrl Pts',(-1.10526450749564,-6.67837410663854,
11.7505187647555));
#12038=CARTESIAN_POINT('Ctrl Pts',(-0.933712306061313,-6.70227351944918,
11.7587161580839));
#12039=CARTESIAN_POINT('Ctrl Pts',(-0.761557053204323,-6.72625694502547,
11.7669423674209));
#12040=CARTESIAN_POINT('Ctrl Pts',(-0.588236492379632,-6.74363664009532,
11.7751685767579));
#12041=CARTESIAN_POINT('Ctrl Pts',(-0.414298356368247,-6.75430572834178,
11.7833947860948));
#12042=CARTESIAN_POINT('Ctrl Pts',(-0.240555632401363,-6.76496283032465,
11.791611753638));
#12043=CARTESIAN_POINT('Ctrl Pts',(-0.0661970695429192,-6.76892431608196,
11.7998287211812));
#12044=CARTESIAN_POINT('Ctrl Pts',(0.108221009389168,-6.76613458431968,
11.8080456887244));
#12045=CARTESIAN_POINT('Ctrl Pts',(0.282478144187115,-6.76334742678001,
11.8162550740678));
#12046=CARTESIAN_POINT('Ctrl Pts',(0.456794329349758,-6.7538214640603,11.8244644594112));
#12047=CARTESIAN_POINT('Ctrl Pts',(0.63060964775381,-6.73755300329132,11.8326738447545));
#12048=CARTESIAN_POINT('Ctrl Pts',(0.804299453150475,-6.72129629006826,
11.8408773020551));
#12049=CARTESIAN_POINT('Ctrl Pts',(0.977488756561493,-6.69830680988572,
11.8490807593557));
#12050=CARTESIAN_POINT('Ctrl Pts',(1.1496190809913,-6.66863291601965,11.8572842166563));
#12051=CARTESIAN_POINT('Ctrl Pts',(1.32165963807766,-6.63897449732701,11.8654833957882));
#12052=CARTESIAN_POINT('Ctrl Pts',(1.49264196381272,-6.60263867041663,11.8736825749201));
#12053=CARTESIAN_POINT('Ctrl Pts',(1.66201404509435,-6.55972547549889,11.8818817540519));
#12054=CARTESIAN_POINT('Ctrl Pts',(1.83135421302534,-6.516820366352,11.8900793882817));
#12055=CARTESIAN_POINT('Ctrl Pts',(1.99908439203378,-6.46734043975449,11.8982770225116));
#12056=CARTESIAN_POINT('Ctrl Pts',(2.16466378273087,-6.41143663368307,11.9064746567414));
#12057=CARTESIAN_POINT('Ctrl Pts',(2.3302312217262,-6.35553686280959,11.914671699257));
#12058=CARTESIAN_POINT('Ctrl Pts',(2.49364784147683,-6.29321424981038,11.9228687417725));
#12059=CARTESIAN_POINT('Ctrl Pts',(2.65438905974009,-6.22466928595666,11.9310657842881));
#12060=CARTESIAN_POINT('Ctrl Pts',(2.81514788997328,-6.15611681182116,11.939263724931));
#12061=CARTESIAN_POINT('Ctrl Pts',(2.97323040470381,-6.08134076927961,11.9474616655738));
#12062=CARTESIAN_POINT('Ctrl Pts',(3.12813297720783,-6.00058939412662,11.9556596062166));
#12063=CARTESIAN_POINT('Ctrl Pts',(3.283080675345,-5.91981449478761,11.9638599350526));
#12064=CARTESIAN_POINT('Ctrl Pts',(3.43484626806414,-5.83306096131377,11.9720602638886));
#12065=CARTESIAN_POINT('Ctrl Pts',(3.58295161818903,-5.7406225012377,11.9802605927246));
#12066=CARTESIAN_POINT('Ctrl Pts',(3.73121129793195,-5.64808771788755,11.988469466516));
#12067=CARTESIAN_POINT('Ctrl Pts',(3.87580281047055,-5.54985636315848,11.9966783403074));
#12068=CARTESIAN_POINT('Ctrl Pts',(4.016277035931,-5.44626548844741,12.0048872140988));
#12069=CARTESIAN_POINT('Ctrl Pts',(4.15682665235861,-5.34261901765664,12.0131004935022));
#12070=CARTESIAN_POINT('Ctrl Pts',(4.29325429664768,-5.23360751637436,12.0213137729056));
#12071=CARTESIAN_POINT('Ctrl Pts',(4.42514483673317,-5.11960761913779,12.0295270523091));
#12072=CARTESIAN_POINT('Ctrl Pts',(4.557228287463,-5.00544097913396,12.0377523449245));
#12073=CARTESIAN_POINT('Ctrl Pts',(4.68476110986385,-4.88627160683936,12.04597763754));
#12074=CARTESIAN_POINT('Ctrl Pts',(4.80736496639999,-4.76251310547594,12.0542029301554));
#12075=CARTESIAN_POINT('Ctrl Pts',(4.91824542691824,-4.65058840741246,12.0616417192675));
#12076=CARTESIAN_POINT('Ctrl Pts',(5.02509484876144,-4.53491084447065,12.0690805083795));
#12077=CARTESIAN_POINT('Ctrl Pts',(5.12766282663466,-4.41580829932064,12.0765192974916));
#12078=CARTESIAN_POINT('Ctrl Pts',(5.24108784667101,-4.28409849232106,12.0847454985104));
#12079=CARTESIAN_POINT('Ctrl Pts',(5.34959346886797,-4.14783161111323,12.0929716995293));
#12080=CARTESIAN_POINT('Ctrl Pts',(5.45279312744014,-4.00741014987755,12.1011979005481));
#12081=CARTESIAN_POINT('Ctrl Pts',(5.55587686294633,-3.86714642255825,12.1094148611639));
#12082=CARTESIAN_POINT('Ctrl Pts',(5.65366629261492,-3.72273769443094,12.1176318217797));
#12083=CARTESIAN_POINT('Ctrl Pts',(5.74581329606023,-3.57462145783542,12.1258487823954));
#12084=CARTESIAN_POINT('Ctrl Pts',(5.83787528640367,-3.42664187050944,12.134058162197));
#12085=CARTESIAN_POINT('Ctrl Pts',(5.92430502940764,-3.27496188932745,12.1422675419986));
#12086=CARTESIAN_POINT('Ctrl Pts',(6.00479608888126,-3.12005014878869,12.1504769218002));
#12087=CARTESIAN_POINT('Ctrl Pts',(6.08522903882042,-2.96525024488351,12.1586803749406));
#12088=CARTESIAN_POINT('Ctrl Pts',(6.15973168022834,-2.80722354576659,12.166883828081));
#12089=CARTESIAN_POINT('Ctrl Pts',(6.22804210422755,-2.64646567103542,12.1750872812214));
#12090=CARTESIAN_POINT('Ctrl Pts',(6.29631691525374,-2.48579160585363,12.1832864575715));
#12091=CARTESIAN_POINT('Ctrl Pts',(6.35840580020133,-2.32238953095174,12.1914856339217));
#12092=CARTESIAN_POINT('Ctrl Pts',(6.41409379715271,-2.15677763372287,12.1996848102718));
#12093=CARTESIAN_POINT('Ctrl Pts',(6.46977131556704,-1.99119689887178,12.2078824438232));
#12094=CARTESIAN_POINT('Ctrl Pts',(6.51905022498551,-1.82340750754573,12.2160800773745));
#12095=CARTESIAN_POINT('Ctrl Pts',(6.56176442024781,-1.65394579511239,12.2242777109259));
#12096=CARTESIAN_POINT('Ctrl Pts',(6.60447553903973,-1.48449628808137,12.2324747540465));
#12097=CARTESIAN_POINT('Ctrl Pts',(6.64062279680041,-1.3133750474065,12.2406717971671));
#12098=CARTESIAN_POINT('Ctrl Pts',(6.6700905256658,-1.1411316223045,12.2488688402876));
#12099=CARTESIAN_POINT('Ctrl Pts',(6.69956148784204,-0.968869298001379,
12.2570667828188));
#12100=CARTESIAN_POINT('Ctrl Pts',(6.72235140047008,-0.795484897576925,
12.26526472535));
#12101=CARTESIAN_POINT('Ctrl Pts',(6.73839607959482,-0.621536221391113,
12.2734626678812));
#12102=CARTESIAN_POINT('Ctrl Pts',(6.75444543530706,-0.447536843898206,
12.2816629998897));
#12103=CARTESIAN_POINT('Ctrl Pts',(6.7637456084418,-0.272973220111627,12.2898633318981));
#12104=CARTESIAN_POINT('Ctrl Pts',(6.7662844448387,-0.0984063592142831,
12.2980636639065));
#12105=CARTESIAN_POINT('Ctrl Pts',(6.76882592738933,0.0763424475338137,
12.3062725428773));
#12106=CARTESIAN_POINT('Ctrl Pts',(6.76459198885875,0.251094139017972,12.314481421848));
#12107=CARTESIAN_POINT('Ctrl Pts',(6.7536226274409,0.425288615081848,12.3226903008188));
#12108=CARTESIAN_POINT('Ctrl Pts',(6.74264737741542,0.599576602780875,12.3309035865062));
#12109=CARTESIAN_POINT('Ctrl Pts',(6.72492953277396,0.773306422258561,12.3391168721936));
#12110=CARTESIAN_POINT('Ctrl Pts',(6.70056077573087,0.945925097847058,12.347330157881));
#12111=CARTESIAN_POINT('Ctrl Pts',(6.67615637019961,1.11879629328312,12.3555554585931));
#12112=CARTESIAN_POINT('Ctrl Pts',(6.64508167241789,1.29055274351432,12.3637807593051));
#12113=CARTESIAN_POINT('Ctrl Pts',(6.60747937158772,1.4606523727577,12.3720060600172));
#12114=CARTESIAN_POINT('Ctrl Pts',(6.57347262637041,1.61448696866093,12.3794448523112));
#12115=CARTESIAN_POINT('Ctrl Pts',(6.5341276476508,1.76696644063304,12.3868836446052));
#12116=CARTESIAN_POINT('Ctrl Pts',(6.4895843790117,1.91770268490382,12.3943224368992));
#12117=CARTESIAN_POINT('Ctrl Pts',(6.4407603161478,2.08292531204811,12.4024761282131));
#12118=CARTESIAN_POINT('Ctrl Pts',(6.38554598662076,2.24654062068834,12.4106298195269));
#12119=CARTESIAN_POINT('Ctrl Pts',(6.32406246397546,2.40801224077799,12.4187835108408));
#12120=CARTESIAN_POINT('Ctrl Pts',(6.26265194244936,2.56929214106243,12.4269275210471));
#12121=CARTESIAN_POINT('Ctrl Pts',(6.1949871753131,2.72843308152131,12.4350715312535));
#12122=CARTESIAN_POINT('Ctrl Pts',(6.12123964829143,2.88491146626461,12.4432155414599));
#12123=CARTESIAN_POINT('Ctrl Pts',(6.04756417639992,3.04123696357107,12.4513515945491));
#12124=CARTESIAN_POINT('Ctrl Pts',(5.96781793304699,3.194904756398,12.4594876476382));
#12125=CARTESIAN_POINT('Ctrl Pts',(5.8822213506837,3.34540894085623,12.4676237007274));
#12126=CARTESIAN_POINT('Ctrl Pts',(5.79669876936719,3.49578300952146,12.4757527199324));
#12127=CARTESIAN_POINT('Ctrl Pts',(5.70533610633201,3.64299860269472,12.4838817391374));
#12128=CARTESIAN_POINT('Ctrl Pts',(5.60840070748488,3.78657239522541,12.4920107583424));
#12129=CARTESIAN_POINT('Ctrl Pts',(5.51151178316446,3.93007735300498,12.5001358801856));
#12130=CARTESIAN_POINT('Ctrl Pts',(5.40905564570289,4.0699436835985,12.5082610020288));
#12131=CARTESIAN_POINT('Ctrl Pts',(5.30134427226658,4.20571491032218,12.516386123872));
#12132=CARTESIAN_POINT('Ctrl Pts',(5.19366404882027,4.34144687218257,12.5245088959405));
#12133=CARTESIAN_POINT('Ctrl Pts',(5.08073184271923,4.47308580225137,12.532631668009));
#12134=CARTESIAN_POINT('Ctrl Pts',(4.96290140266499,4.60020637226482,12.5407544400775));
#12135=CARTESIAN_POINT('Ctrl Pts',(4.84508262376716,4.72731436171888,12.5488764082712));
#12136=CARTESIAN_POINT('Ctrl Pts',(4.72236682569628,4.84990461439186,12.5569983764649));
#12137=CARTESIAN_POINT('Ctrl Pts',(4.5951462456726,4.96758693742556,12.5651203446587));
#12138=CARTESIAN_POINT('Ctrl Pts',(4.46787474726667,5.08531636127823,12.5732455635645));
#12139=CARTESIAN_POINT('Ctrl Pts',(4.33609513224914,5.19813368123317,12.5813707824703));
#12140=CARTESIAN_POINT('Ctrl Pts',(4.2002348556424,5.3056871522402,12.5894960013762));
#12141=CARTESIAN_POINT('Ctrl Pts',(4.06434482499791,5.41326417796179,12.5976229997431));
#12142=CARTESIAN_POINT('Ctrl Pts',(3.92437264431104,5.51557483790704,12.60574999811));
#12143=CARTESIAN_POINT('Ctrl Pts',(3.7807765139826,5.61230950245241,12.6138769964769));
#12144=CARTESIAN_POINT('Ctrl Pts',(3.6370642353945,5.709122411188,12.6220105683964));
#12145=CARTESIAN_POINT('Ctrl Pts',(3.48972246127582,5.80035012042969,12.6301441403159));
#12146=CARTESIAN_POINT('Ctrl Pts',(3.33923637653553,5.88572760341675,12.6382777122353));
#12147=CARTESIAN_POINT('Ctrl Pts',(3.26006178148752,5.93064689049492,12.6425569933671));
#12148=CARTESIAN_POINT('Ctrl Pts',(3.18001721780825,5.9739475603292,12.6468362744988));
#12149=CARTESIAN_POINT('Ctrl Pts',(3.09917575053257,6.0155962852664,12.6511155556306));
#12150=CARTESIAN_POINT('Origin',(0.,0.,-3.69717978381041));
#12151=CARTESIAN_POINT('',(3.09917575053257,6.0155962852664,15.0458593505058));
#12152=CARTESIAN_POINT('',(3.09917575053259,6.01559628526639,14.6513920151221));
#12153=CARTESIAN_POINT('',(3.09917575053259,6.01559628526639,-3.69717978381041));
#12154=CARTESIAN_POINT('',(-6.76699862985715,0.00430621776387394,13.697179783847));
#12155=CARTESIAN_POINT('Ctrl Pts',(-6.76699862985715,0.00430621776387394,
13.697179783847));
#12156=CARTESIAN_POINT('Ctrl Pts',(-6.76710791901341,-0.167436042203893,
13.7052923628463));
#12157=CARTESIAN_POINT('Ctrl Pts',(-6.76067498570166,-0.339425333033403,
13.7134049418455));
#12158=CARTESIAN_POINT('Ctrl Pts',(-6.74766992581323,-0.51111600667133,
13.7215175208448));
#12159=CARTESIAN_POINT('Ctrl Pts',(-6.73467774622239,-0.68263663672721,
13.729622065092));
#12160=CARTESIAN_POINT('Ctrl Pts',(-6.71512642437169,-0.853858873096928,
13.7377266093393));
#12161=CARTESIAN_POINT('Ctrl Pts',(-6.68903806257846,-1.02423571377715,
13.7458311535865));
#12162=CARTESIAN_POINT('Ctrl Pts',(-6.6629699464566,-1.19448033482812,13.7539294083648));
#12163=CARTESIAN_POINT('Ctrl Pts',(-6.63037494574035,-1.36388050322722,
13.7620276631432));
#12164=CARTESIAN_POINT('Ctrl Pts',(-6.59132708286434,-1.53189304022805,
13.7701259179215));
#12165=CARTESIAN_POINT('Ctrl Pts',(-6.55230115731951,-1.6998111867451,13.7782196230502));
#12166=CARTESIAN_POINT('Ctrl Pts',(-6.50682967182941,-1.86634289563401,
13.7863133281788));
#12167=CARTESIAN_POINT('Ctrl Pts',(-6.45503795771554,-2.03095395429135,
13.7944070333075));
#12168=CARTESIAN_POINT('Ctrl Pts',(-6.40325802058797,-2.19552758182253,
13.8024988979979));
#12169=CARTESIAN_POINT('Ctrl Pts',(-6.34516082144924,-2.35818107520942,
13.8105907626882));
#12170=CARTESIAN_POINT('Ctrl Pts',(-6.28092193695672,-2.51839405611112,
13.8186826273786));
#12171=CARTESIAN_POINT('Ctrl Pts',(-6.21668840886093,-2.67859367805907,
13.8267738173493));
#12172=CARTESIAN_POINT('Ctrl Pts',(-6.14631435157219,-2.83635284963488,
13.83486500732));
#12173=CARTESIAN_POINT('Ctrl Pts',(-6.0700239420726,-2.99117006247813,13.8429561972907));
#12174=CARTESIAN_POINT('Ctrl Pts',(-5.9937250956006,-3.14600439658946,13.8510482820678));
#12175=CARTESIAN_POINT('Ctrl Pts',(-5.91150875758756,-3.29789579299366,
13.8591403668449));
#12176=CARTESIAN_POINT('Ctrl Pts',(-5.82364557679827,-3.44636637574097,
13.867232451622));
#12177=CARTESIAN_POINT('Ctrl Pts',(-5.73575563432666,-3.59488218019017,
13.8753270011153));
#12178=CARTESIAN_POINT('Ctrl Pts',(-5.6422156132573,-3.73997477928341,13.8834215506086));
#12179=CARTESIAN_POINT('Ctrl Pts',(-5.54334002749553,-3.88119444753363,
13.8915161001018));
#12180=CARTESIAN_POINT('Ctrl Pts',(-5.44436299263744,-4.0225590110845,13.8996189548276));
#12181=CARTESIAN_POINT('Ctrl Pts',(-5.34003967278028,-4.16004240580135,
13.9077218095534));
#12182=CARTESIAN_POINT('Ctrl Pts',(-5.23072596280807,-4.29322663063641,
13.9158246642792));
#12183=CARTESIAN_POINT('Ctrl Pts',(-5.12134985217798,-4.42648688237833,
13.9239321444401));
#12184=CARTESIAN_POINT('Ctrl Pts',(-5.00697792077875,-4.5554427997631,13.9320396246009));
#12185=CARTESIAN_POINT('Ctrl Pts',(-4.88800332975851,-4.67971285959616,
13.9401471047618));
#12186=CARTESIAN_POINT('Ctrl Pts',(-4.76886601445183,-4.80415288645025,
13.9482656737098));
#12187=CARTESIAN_POINT('Ctrl Pts',(-4.64511373259073,-4.92389400117209,
13.9563842426579));
#12188=CARTESIAN_POINT('Ctrl Pts',(-4.51717380191012,-5.03859403438468,
13.964502811606));
#12189=CARTESIAN_POINT('Ctrl Pts',(-4.44544148123866,-5.10290311693352,
13.9690546648709));
#12190=CARTESIAN_POINT('Ctrl Pts',(-4.37239332102361,-5.16562827586466,
13.9736065181357));
#12191=CARTESIAN_POINT('Ctrl Pts',(-4.29810856065524,-5.22671520180908,
13.9781583714006));
#12192=CARTESIAN_POINT('Ctrl Pts',(-4.16508719060017,-5.33610327200389,
13.9863093535749));
#12193=CARTESIAN_POINT('Ctrl Pts',(-4.02767819514069,-5.44058171598578,
13.9944603357492));
#12194=CARTESIAN_POINT('Ctrl Pts',(-3.88628208341779,-5.5397744149113,14.0026113179234));
#12195=CARTESIAN_POINT('Ctrl Pts',(-3.74505021638349,-5.63885189232368,
14.0107528319765));
#12196=CARTESIAN_POINT('Ctrl Pts',(-3.59984074856104,-5.73265563871572,
14.0188943460295));
#12197=CARTESIAN_POINT('Ctrl Pts',(-3.45108880764441,-5.8208483094607,14.0270358600825));
#12198=CARTESIAN_POINT('Ctrl Pts',(-3.30247835302977,-5.90895709521723,
14.0351696302856));
#12199=CARTESIAN_POINT('Ctrl Pts',(-3.15033244579128,-5.99146524530517,
14.0433034004886));
#12200=CARTESIAN_POINT('Ctrl Pts',(-2.99511687030795,-6.06807744950546,
14.0514371706917));
#12201=CARTESIAN_POINT('Ctrl Pts',(-2.84001628402086,-6.14463289667118,
14.0595649151097));
#12202=CARTESIAN_POINT('Ctrl Pts',(-2.68185088416405,-6.21530093398868,
14.0676926595276));
#12203=CARTESIAN_POINT('Ctrl Pts',(-2.52111284102055,-6.27983113171376,
14.0758204039456));
#12204=CARTESIAN_POINT('Ctrl Pts',(-2.36046008435082,-6.34432709017035,
14.0839438358396));
#12205=CARTESIAN_POINT('Ctrl Pts',(-2.19723774149744,-6.40269155886517,
14.0920672677336));
#12206=CARTESIAN_POINT('Ctrl Pts',(-2.03195983261033,-6.45472139124984,
14.1001906996277));
#12207=CARTESIAN_POINT('Ctrl Pts',(-1.86563346567688,-6.50708128042661,
14.1083656633785));
#12208=CARTESIAN_POINT('Ctrl Pts',(-1.6972257023513,-6.55302572609678,14.1165406271293));
#12209=CARTESIAN_POINT('Ctrl Pts',(-1.5272783993263,-6.59239787110512,14.1247155908801));
#12210=CARTESIAN_POINT('Ctrl Pts',(-1.35844068722097,-6.63151295422539,
14.1328371800532));
#12211=CARTESIAN_POINT('Ctrl Pts',(-1.18808384551203,-6.66414124503068,
14.1409587692262));
#12212=CARTESIAN_POINT('Ctrl Pts',(-1.01675155659607,-6.69017976381498,
14.1490803583992));
#12213=CARTESIAN_POINT('Ctrl Pts',(-0.84539664830377,-6.71622172021784,
14.1572030197886));
#12214=CARTESIAN_POINT('Ctrl Pts',(-0.673066398166757,-6.73567211674775,
14.165325681178));
#12215=CARTESIAN_POINT('Ctrl Pts',(-0.500311634498783,-6.74847962643329,
14.1734483425673));
#12216=CARTESIAN_POINT('Ctrl Pts',(-0.32750116604283,-6.76129126590139,
14.1815736231096));
#12217=CARTESIAN_POINT('Ctrl Pts',(-0.15426627627263,-6.76745572610162,
14.1896989036518));
#12218=CARTESIAN_POINT('Ctrl Pts',(0.018840212519595,-6.76697377314204,
14.197824184194));
#12219=CARTESIAN_POINT('Ctrl Pts',(0.193832660588631,-6.76648656940497,
14.2060379879818));
#12220=CARTESIAN_POINT('Ctrl Pts',(0.36869350937776,-6.75920728251903,14.2142517917696));
#12221=CARTESIAN_POINT('Ctrl Pts',(0.542855862123635,-6.74519062095046,
14.2224655955574));
#12222=CARTESIAN_POINT('Ctrl Pts',(0.715439331337447,-6.73130102861227,
14.2306049364125));
#12223=CARTESIAN_POINT('Ctrl Pts',(0.887336562306852,-6.71079582288724,
14.2387442772677));
#12224=CARTESIAN_POINT('Ctrl Pts',(1.05800550951591,-6.68377986934294,14.2468836181229));
#12225=CARTESIAN_POINT('Ctrl Pts',(1.23101650945525,-6.65639318176182,14.255134653377));
#12226=CARTESIAN_POINT('Ctrl Pts',(1.40276488520187,-6.62231583582359,14.263385688631));
#12227=CARTESIAN_POINT('Ctrl Pts',(1.57270155325428,-6.58170941506776,14.2716367238851));
#12228=CARTESIAN_POINT('Ctrl Pts',(1.74263822130669,-6.54110299431192,14.2798877591392));
#12229=CARTESIAN_POINT('Ctrl Pts',(1.91076283014249,-6.49396766694165,14.2881387943933));
#12230=CARTESIAN_POINT('Ctrl Pts',(2.07654738497298,-6.44051550405415,14.2963898296474));
#12231=CARTESIAN_POINT('Ctrl Pts',(2.24194489202171,-6.38718813289467,14.3046216016782));
#12232=CARTESIAN_POINT('Ctrl Pts',(2.40552965522928,-6.3274070782602,14.3128533737091));
#12233=CARTESIAN_POINT('Ctrl Pts',(2.56676137122036,-6.26131176856823,14.3210851457399));
#12234=CARTESIAN_POINT('Ctrl Pts',(2.72780056043021,-6.19529538328112,14.3293070882123));
#12235=CARTESIAN_POINT('Ctrl Pts',(2.88649196906151,-6.12297989109231,14.3375290306847));
#12236=CARTESIAN_POINT('Ctrl Pts',(3.04230956560976,-6.04455469881772,14.3457509731571));
#12237=CARTESIAN_POINT('Ctrl Pts',(3.19797231980186,-5.96620744088317,14.353964745147));
#12238=CARTESIAN_POINT('Ctrl Pts',(3.35076663142432,-5.88176273412973,14.3621785171369));
#12239=CARTESIAN_POINT('Ctrl Pts',(3.50018552170184,-5.79145839263901,14.3703922891268));
#12240=CARTESIAN_POINT('Ctrl Pts',(3.64948585479403,-5.70122570359151,14.3785995438572));
#12241=CARTESIAN_POINT('Ctrl Pts',(3.79541579575059,-5.60514282481725,14.3868067985876));
#12242=CARTESIAN_POINT('Ctrl Pts',(3.93749202181478,-5.50349394277353,14.3950140533179));
#12243=CARTESIAN_POINT('Ctrl Pts',(4.07948396523469,-5.4019053610123,14.4032164393299));
#12244=CARTESIAN_POINT('Ctrl Pts',(4.21762645732611,-5.29475756163349,14.4114188253419));
#12245=CARTESIAN_POINT('Ctrl Pts',(4.35146421202563,-5.18237862486524,14.4196212113539));
#12246=CARTESIAN_POINT('Ctrl Pts',(4.48526201940106,-5.07003323048434,14.4278211491526));
#12247=CARTESIAN_POINT('Ctrl Pts',(4.61475737221627,-4.95246003604422,14.4360210869513));
#12248=CARTESIAN_POINT('Ctrl Pts',(4.73952701790977,-4.83002822419324,14.44422102475));
#12249=CARTESIAN_POINT('Ctrl Pts',(4.86427921758664,-4.70761353146938,14.4524198159858));
#12250=CARTESIAN_POINT('Ctrl Pts',(4.98430676985345,-4.58034182473609,14.4606186072215));
#12251=CARTESIAN_POINT('Ctrl Pts',(5.09922233718302,-4.44862007323325,14.4688173984573));
#12252=CARTESIAN_POINT('Ctrl Pts',(5.21414268263058,-4.31689284482169,14.4770165305937));
#12253=CARTESIAN_POINT('Ctrl Pts',(5.32395038398178,-4.18071547306964,14.4852156627301));
#12254=CARTESIAN_POINT('Ctrl Pts',(5.42829752155873,-4.04052905167621,14.4934147948665));
#12255=CARTESIAN_POINT('Ctrl Pts',(5.53266792686751,-3.90031137096761,14.5016157552774));
#12256=CARTESIAN_POINT('Ctrl Pts',(5.63157512928682,-3.75608314758275,14.5098167156883));
#12257=CARTESIAN_POINT('Ctrl Pts',(5.7247137470009,-3.60831560633198,14.5180176760992));
#12258=CARTESIAN_POINT('Ctrl Pts',(5.81793965802138,-3.46040957132243,14.5262263227842));
#12259=CARTESIAN_POINT('Ctrl Pts',(5.90538599100199,-3.30895789451858,14.5344349694692));
#12260=CARTESIAN_POINT('Ctrl Pts',(5.98679220429685,-3.15445844838231,14.5426436161543));
#12261=CARTESIAN_POINT('Ctrl Pts',(6.06823728320451,-2.99988523987078,14.5508561818778));
#12262=CARTESIAN_POINT('Ctrl Pts',(6.14363633818558,-2.84226168399215,14.5590687476013));
#12263=CARTESIAN_POINT('Ctrl Pts',(6.21277650421415,-2.6821068414,14.5672813133249));
#12264=CARTESIAN_POINT('Ctrl Pts',(6.2820115405274,-2.52173224325353,14.5755051478736));
#12265=CARTESIAN_POINT('Ctrl Pts',(6.34497039488857,-2.35881975129657,14.5837289824224));
#12266=CARTESIAN_POINT('Ctrl Pts',(6.40148931351874,-2.19390600730873,14.5919528169712));
#12267=CARTESIAN_POINT('Ctrl Pts',(6.45341956803154,-2.04238129831731,14.5995089739455));
#12268=CARTESIAN_POINT('Ctrl Pts',(6.49991364943102,-1.8891674794027,14.6070651309199));
#12269=CARTESIAN_POINT('Ctrl Pts',(6.54088257718518,-1.73468847678058,14.6146212878942));
#12270=CARTESIAN_POINT('Ctrl Pts',(6.58775902502417,-1.55793435345847,14.6232670059466));
#12271=CARTESIAN_POINT('Ctrl Pts',(6.62750858751518,-1.37912093385762,14.6319127239989));
#12272=CARTESIAN_POINT('Ctrl Pts',(6.65996096138983,-1.19883651627882,14.6405584420513));
#12273=CARTESIAN_POINT('Ctrl Pts',(6.69237167303007,-1.01878354715095,14.6491930607636));
#12274=CARTESIAN_POINT('Ctrl Pts',(6.71750382276465,-0.837263644455639,
14.657827679476));
#12275=CARTESIAN_POINT('Ctrl Pts',(6.73523747564718,-0.654877963163986,
14.6664622981884));
#12276=CARTESIAN_POINT('Ctrl Pts',(6.75359741225974,-0.466051128121339,
14.6754018580908));
#12277=CARTESIAN_POINT('Ctrl Pts',(6.76402663197152,-0.276296549436255,
14.6843414179932));
#12278=CARTESIAN_POINT('Ctrl Pts',(6.7664497667447,-0.0862934187562398,
14.6932809778957));
#12279=CARTESIAN_POINT('Ctrl Pts',(6.76878374890793,0.09671906691934,14.7018916311661));
#12280=CARTESIAN_POINT('Ctrl Pts',(6.76369021095113,0.279961794029591,14.7105022844366));
#12281=CARTESIAN_POINT('Ctrl Pts',(6.7511543544222,0.462821653303111,14.7191129377071));
#12282=CARTESIAN_POINT('Ctrl Pts',(6.73863036392011,0.645508423486494,14.7277154404182));
#12283=CARTESIAN_POINT('Ctrl Pts',(6.71867812078026,0.827812745107107,14.7363179431293));
#12284=CARTESIAN_POINT('Ctrl Pts',(6.69133485708387,1.009121811465,14.7449204458404));
#12285=CARTESIAN_POINT('Ctrl Pts',(6.66402236768029,1.19022681811882,14.7535132666079));
#12286=CARTESIAN_POINT('Ctrl Pts',(6.62933549815467,1.37033850321513,14.7621060873754));
#12287=CARTESIAN_POINT('Ctrl Pts',(6.58736327713615,1.54884926801741,14.7706989081429));
#12288=CARTESIAN_POINT('Ctrl Pts',(6.58241666024053,1.56988757249101,14.7717116111011));
#12289=CARTESIAN_POINT('Ctrl Pts',(6.57736891118489,1.59090364736417,14.7727243140594));
#12290=CARTESIAN_POINT('Ctrl Pts',(6.57222022306497,1.61189650397781,14.7737370170176));
#12291=CARTESIAN_POINT('Ctrl Pts',(6.52852103056551,1.79007215977691,14.7823322747777));
#12292=CARTESIAN_POINT('Ctrl Pts',(6.47759776454528,1.9663647392222,14.7909275325378));
#12293=CARTESIAN_POINT('Ctrl Pts',(6.4196470761144,2.14019167789614,14.7995227902978));
#12294=CARTESIAN_POINT('Ctrl Pts',(6.36164211932129,2.31418139812675,14.8081260971523));
#12295=CARTESIAN_POINT('Ctrl Pts',(6.29659670099373,2.4857005791225,14.8167294040068));
#12296=CARTESIAN_POINT('Ctrl Pts',(6.22475593460164,2.65418585533148,14.8253327108613));
#12297=CARTESIAN_POINT('Ctrl Pts',(6.14993662512315,2.82965658951669,14.8342927138013));
#12298=CARTESIAN_POINT('Ctrl Pts',(6.06774664756277,3.00183613942243,14.8432527167412));
#12299=CARTESIAN_POINT('Ctrl Pts',(5.97851554764615,3.17011685061502,14.8522127196812));
#12300=CARTESIAN_POINT('Ctrl Pts',(5.89260232717896,3.33214038113938,14.860839562886));
#12301=CARTESIAN_POINT('Ctrl Pts',(5.80016235165871,3.49054955350911,14.8694664060907));
#12302=CARTESIAN_POINT('Ctrl Pts',(5.70153411846878,3.64483164164498,14.8780932492955));
#12303=CARTESIAN_POINT('Ctrl Pts',(5.60281162161947,3.79926118445721,14.8867283375816));
#12304=CARTESIAN_POINT('Ctrl Pts',(5.49788923338844,3.94955551788104,14.8953634258678));
#12305=CARTESIAN_POINT('Ctrl Pts',(5.38714710240445,4.09523321644267,14.9039985141539));
#12306=CARTESIAN_POINT('Ctrl Pts',(5.27624049713202,4.24112727562152,14.9126464272791));
#12307=CARTESIAN_POINT('Ctrl Pts',(5.15949706732643,4.38239076018922,14.9212943404042));
#12308=CARTESIAN_POINT('Ctrl Pts',(5.0373362968425,4.51857632806099,14.9299422535294));
#12309=CARTESIAN_POINT('Ctrl Pts',(5.02363171806996,4.53385427559839,14.9309124177333));
#12310=CARTESIAN_POINT('Ctrl Pts',(5.00985899663787,4.54906835482126,14.9318825819371));
#12311=CARTESIAN_POINT('Ctrl Pts',(4.99601875237309,4.56421796433261,14.932852746141));
#12312=CARTESIAN_POINT('Ctrl Pts',(4.87866384123369,4.69267531262694,14.9410790123657));
#12313=CARTESIAN_POINT('Ctrl Pts',(4.7561967314082,4.81677293629984,14.9493052785904));
#12314=CARTESIAN_POINT('Ctrl Pts',(4.62897400458076,4.93608029360499,14.9575315448151));
#12315=CARTESIAN_POINT('Ctrl Pts',(4.50191908125205,5.05523028757988,14.9657469608065));
#12316=CARTESIAN_POINT('Ctrl Pts',(4.37012130086407,5.16960236340963,14.973962376798));
#12317=CARTESIAN_POINT('Ctrl Pts',(4.23397606086872,5.27880059445236,14.9821777927895));
#12318=CARTESIAN_POINT('Ctrl Pts',(4.09793449084457,5.38791567475499,14.990386953021));
#12319=CARTESIAN_POINT('Ctrl Pts',(3.95755232917933,5.4918645300023,14.9985961132526));
#12320=CARTESIAN_POINT('Ctrl Pts',(3.81326072202526,5.590289050296,15.0068052734841));
#12321=CARTESIAN_POINT('Ctrl Pts',(3.66906843414041,5.68864582270318,15.0150087831597));
#12322=CARTESIAN_POINT('Ctrl Pts',(3.52097235714589,5.78148563488334,15.0232122928354));
#12323=CARTESIAN_POINT('Ctrl Pts',(3.36943541864658,5.86849162558574,15.031415802511));
#12324=CARTESIAN_POINT('Ctrl Pts',(3.28050067686138,5.9195541281908,15.0362303185093));
#12325=CARTESIAN_POINT('Ctrl Pts',(3.19038138094769,5.96860804591482,15.0410448345075));
#12326=CARTESIAN_POINT('Ctrl Pts',(3.09917575053257,6.0155962852664,15.0458593505058));
#12327=CARTESIAN_POINT('Ctrl Pts',(3.09917575053261,6.01559628526638,13.045945719425));
#12328=CARTESIAN_POINT('Ctrl Pts',(2.94589749677957,6.09456372666182,13.054090403068));
#12329=CARTESIAN_POINT('Ctrl Pts',(2.7893836746281,6.16778000659029,13.062235086711));
#12330=CARTESIAN_POINT('Ctrl Pts',(2.63010911547121,6.234967124269,13.070379770354));
#12331=CARTESIAN_POINT('Ctrl Pts',(2.47099810587648,6.30208525149666,13.0785160907062));
#12332=CARTESIAN_POINT('Ctrl Pts',(2.30913233709464,6.3631864003597,13.0866524110585));
#12333=CARTESIAN_POINT('Ctrl Pts',(2.1450116533509,6.41803817431689,13.0947887314108));
#12334=CARTESIAN_POINT('Ctrl Pts',(1.98102497110466,6.47284516281692,13.1029184086082));
#12335=CARTESIAN_POINT('Ctrl Pts',(1.81478738476683,6.52141282054947,13.1110480858057));
#12336=CARTESIAN_POINT('Ctrl Pts',(1.64681915269871,6.56355663328235,13.1191777630031));
#12337=CARTESIAN_POINT('Ctrl Pts',(1.47895274518715,6.60567489788038,13.1273025118831));
#12338=CARTESIAN_POINT('Ctrl Pts',(1.30935813494568,6.64137698378639,13.135427260763));
#12339=CARTESIAN_POINT('Ctrl Pts',(1.13857118912809,6.67052806360092,13.143552009643));
#12340=CARTESIAN_POINT('Ctrl Pts',(0.965025754317399,6.70014998111572,13.151807986529));
#12341=CARTESIAN_POINT('Ctrl Pts',(0.790249501735948,6.72300733236068,13.160063963415));
#12342=CARTESIAN_POINT('Ctrl Pts',(0.614816607369404,6.73901250475934,13.168319940301));
#12343=CARTESIAN_POINT('Ctrl Pts',(0.442243001821795,6.75475681723975,13.1764413573458));
#12344=CARTESIAN_POINT('Ctrl Pts',(0.269034373158783,6.7638705907001,13.1845627743907));
#12345=CARTESIAN_POINT('Ctrl Pts',(0.0957431469898265,6.76632265339191,
13.1926841914355));
#12346=CARTESIAN_POINT('Ctrl Pts',(-0.0775591384366407,6.76877487257169,
13.2008061267804));
#12347=CARTESIAN_POINT('Ctrl Pts',(-0.250943665915966,6.76456452879857,
13.2089280621252));
#12348=CARTESIAN_POINT('Ctrl Pts',(-0.42385758428952,6.75371258999376,13.21704999747));
#12349=CARTESIAN_POINT('Ctrl Pts',(-0.596815464492231,6.74285789217983,
13.2251739977449));
#12350=CARTESIAN_POINT('Ctrl Pts',(-0.769302132211122,6.7253582599974,13.2332979980197));
#12351=CARTESIAN_POINT('Ctrl Pts',(-0.940769476151189,6.70128657742244,
13.2414219982945));
#12352=CARTESIAN_POINT('Ctrl Pts',(-1.11713603092092,6.67652711229222,13.2497781196789));
#12353=CARTESIAN_POINT('Ctrl Pts',(-1.29242373346546,6.64481450465825,13.2581342410633));
#12354=CARTESIAN_POINT('Ctrl Pts',(-1.46604785067862,6.60628433383855,13.2664903624476));
#12355=CARTESIAN_POINT('Ctrl Pts',(-1.63511721627612,6.56876494055718,13.2746272743236));
#12356=CARTESIAN_POINT('Ctrl Pts',(-1.80260884726462,6.52478134245833,13.2827641861996));
#12357=CARTESIAN_POINT('Ctrl Pts',(-1.96799907955178,6.47450914146265,13.2909010980756));
#12358=CARTESIAN_POINT('Ctrl Pts',(-2.14007276473768,6.42220543060798,13.2993668242142));
#12359=CARTESIAN_POINT('Ctrl Pts',(-2.309871248914,6.36309443250584,13.3078325503527));
#12360=CARTESIAN_POINT('Ctrl Pts',(-2.47682913674139,6.29742855675147,13.3162982764913));
#12361=CARTESIAN_POINT('Ctrl Pts',(-2.64378702456875,6.23176268099711,13.3247640026299));
#12362=CARTESIAN_POINT('Ctrl Pts',(-2.80790394372058,6.15954216912804,13.3332297287684));
#12363=CARTESIAN_POINT('Ctrl Pts',(-2.968645063856,6.08107190262074,13.341695454907));
#12364=CARTESIAN_POINT('Ctrl Pts',(-3.12481293673833,6.00483419446846,13.3499203225846));
#12365=CARTESIAN_POINT('Ctrl Pts',(-3.27826137829459,5.92246977420169,13.3581451902622));
#12366=CARTESIAN_POINT('Ctrl Pts',(-3.42847643053927,5.8341956056715,13.3663700579398));
#12367=CARTESIAN_POINT('Ctrl Pts',(-3.57852224871382,5.74602088787282,13.3745856593833));
#12368=CARTESIAN_POINT('Ctrl Pts',(-3.72534162477454,5.65194985968362,13.3828012608268));
#12369=CARTESIAN_POINT('Ctrl Pts',(-3.86844208815066,5.55224682544144,13.3910168622704));
#12370=CARTESIAN_POINT('Ctrl Pts',(-4.01141008459231,5.45263608548672,13.3992248585985));
#12371=CARTESIAN_POINT('Ctrl Pts',(-4.1506657317795,5.34740392607763,13.4074328549267));
#12372=CARTESIAN_POINT('Ctrl Pts',(-4.28574254716233,5.23685972883011,13.4156408512548));
#12373=CARTESIAN_POINT('Ctrl Pts',(-4.4207214539168,5.12639565806984,13.4238428981262));
#12374=CARTESIAN_POINT('Ctrl Pts',(-4.55152728548307,5.01062744495931,13.4320449449977));
#12375=CARTESIAN_POINT('Ctrl Pts',(-4.67772380324455,4.88990685193076,13.4402469918691));
#12376=CARTESIAN_POINT('Ctrl Pts',(-4.80385419053292,4.76924951983898,13.4484447406407));
#12377=CARTESIAN_POINT('Ctrl Pts',(-4.92537981725779,4.64364522526605,13.4566424894123));
#12378=CARTESIAN_POINT('Ctrl Pts',(-5.04189865823783,4.51348500829011,13.4648402381838));
#12379=CARTESIAN_POINT('Ctrl Pts',(-5.15839527558922,4.38334961676131,13.4730364233994));
#12380=CARTESIAN_POINT('Ctrl Pts',(-5.26988676563717,4.24866029656104,13.4812326086151));
#12381=CARTESIAN_POINT('Ctrl Pts',(-5.37600881867134,4.10984405805963,13.4894287938307));
#12382=CARTESIAN_POINT('Ctrl Pts',(-5.48212302103556,3.9710380888702,13.497624372711));
#12383=CARTESIAN_POINT('Ctrl Pts',(-5.58286835882044,3.82810609391566,13.5058199515914));
#12384=CARTESIAN_POINT('Ctrl Pts',(-5.67792163962859,3.68150714439581,13.5140155304717));
#12385=CARTESIAN_POINT('Ctrl Pts',(-5.77298518242844,3.53489236799243,13.5222119941502));
#12386=CARTESIAN_POINT('Ctrl Pts',(-5.86235524868935,3.38461014943962,13.5304084578286));
#12387=CARTESIAN_POINT('Ctrl Pts',(-5.94575268618598,3.23114747337726,13.5386049215071));
#12388=CARTESIAN_POINT('Ctrl Pts',(-6.02917430054413,3.07764030858743,13.5468037613349));
#12389=CARTESIAN_POINT('Ctrl Pts',(-6.10661966599629,2.92095116496101,13.5550026011627));
#12390=CARTESIAN_POINT('Ctrl Pts',(-6.17785616444124,2.76159052204982,13.5632014409905));
#12391=CARTESIAN_POINT('Ctrl Pts',(-6.24916707143531,2.60206342241369,13.5714088447397));
#12392=CARTESIAN_POINT('Ctrl Pts',(-6.31425600792885,2.43985957655252,13.5796162484889));
#12393=CARTESIAN_POINT('Ctrl Pts',(-6.37293862778668,2.27550922794534,13.5878236522382));
#12394=CARTESIAN_POINT('Ctrl Pts',(-6.43165268116115,2.11107084459415,13.5960354523072));
#12395=CARTESIAN_POINT('Ctrl Pts',(-6.48395346961002,1.94448400841016,13.6042472523762));
#12396=CARTESIAN_POINT('Ctrl Pts',(-6.52970694613362,1.77629282428724,13.6124590524452));
#12397=CARTESIAN_POINT('Ctrl Pts',(-6.57552777816776,1.60785403924009,13.6206829414314));
#12398=CARTESIAN_POINT('Ctrl Pts',(-6.61478195517534,1.43780653585421,13.6289068304175));
#12399=CARTESIAN_POINT('Ctrl Pts',(-6.64738659624081,1.26670455912892,13.6371307194037));
#12400=CARTESIAN_POINT('Ctrl Pts',(-6.67751272092189,1.10860929061629,13.6447294506537));
#12401=CARTESIAN_POINT('Ctrl Pts',(-6.70196238596804,0.949614070944114,
13.6523281819037));
#12402=CARTESIAN_POINT('Ctrl Pts',(-6.72070973630126,0.790157984447094,
13.6599269131537));
#12403=CARTESIAN_POINT('Ctrl Pts',(-6.75134610589733,0.529579528642073,
13.6723445367058));
#12404=CARTESIAN_POINT('Ctrl Pts',(-6.76683134497133,0.267185721162299,
13.6847621602579));
#12405=CARTESIAN_POINT('Ctrl Pts',(-6.76699862985665,0.00430621854705538,
13.69717978381));
#12406=CARTESIAN_POINT('',(-6.767,1.40740026512327E-12,13.3028202161899));
#12407=CARTESIAN_POINT('Ctrl Pts',(3.09917575053257,6.0155962852664,12.6511155556306));
#12408=CARTESIAN_POINT('Ctrl Pts',(2.94532479176222,6.09485877862638,12.6592595382568));
#12409=CARTESIAN_POINT('Ctrl Pts',(2.78858665361273,6.16813513728891,12.6674035208829));
#12410=CARTESIAN_POINT('Ctrl Pts',(2.62947835233266,6.23523316281067,12.6755475035091));
#12411=CARTESIAN_POINT('Ctrl Pts',(2.47013644809179,6.30242970171796,12.6837034431384));
#12412=CARTESIAN_POINT('Ctrl Pts',(2.30841777229537,6.36342966448213,12.6918593827677));
#12413=CARTESIAN_POINT('Ctrl Pts',(2.14485468170803,6.41809063463232,12.700015322397));
#12414=CARTESIAN_POINT('Ctrl Pts',(2.06389975203557,6.44514487393807,12.7040520737003));
#12415=CARTESIAN_POINT('Ctrl Pts',(1.98249316051284,6.47064702757832,12.7080888250036));
#12416=CARTESIAN_POINT('Ctrl Pts',(1.90070022083335,6.49458448790406,12.7121255763069));
#12417=CARTESIAN_POINT('Ctrl Pts',(1.73388157825965,6.54340550661118,12.7203586264389));
#12418=CARTESIAN_POINT('Ctrl Pts',(1.56493684531338,6.58586646477601,12.7285916765709));
#12419=CARTESIAN_POINT('Ctrl Pts',(1.39439157355043,6.62177930314893,12.7368247267029));
#12420=CARTESIAN_POINT('Ctrl Pts',(1.2240493949906,6.65764937485173,12.7450479725378));
#12421=CARTESIAN_POINT('Ctrl Pts',(1.0521108199802,6.68698678103675,12.7532712183727));
#12422=CARTESIAN_POINT('Ctrl Pts',(0.879117648729215,6.70965283451334,12.7614944642075));
#12423=CARTESIAN_POINT('Ctrl Pts',(0.706295860796889,6.73229643286387,12.769709563321));
#12424=CARTESIAN_POINT('Ctrl Pts',(0.532421910026123,6.74828179473598,12.7779246624345));
#12425=CARTESIAN_POINT('Ctrl Pts',(0.358049008625063,6.75752098830796,12.786139761548));
#12426=CARTESIAN_POINT('Ctrl Pts',(0.183813968928741,6.76675287724164,12.7943483656869));
#12427=CARTESIAN_POINT('Ctrl Pts',(0.009081120393062,6.76924920250609,12.8025569698258));
#12428=CARTESIAN_POINT('Ctrl Pts',(-0.165589862747555,6.76497368785387,
12.8107655739647));
#12429=CARTESIAN_POINT('Ctrl Pts',(-0.340157687582229,6.76070069826244,
12.8189693302137));
#12430=CARTESIAN_POINT('Ctrl Pts',(-0.514663362693545,6.74966384475748,
12.8271730864627));
#12431=CARTESIAN_POINT('Ctrl Pts',(-0.688545766638032,6.731878915076,12.8353768427117));
#12432=CARTESIAN_POINT('Ctrl Pts',(-0.862376723161842,6.71409924750696,
12.8435781716759));
#12433=CARTESIAN_POINT('Ctrl Pts',(-1.03558441959404,6.68957551344629,12.8517795006402));
#12434=CARTESIAN_POINT('Ctrl Pts',(-1.20761115969753,6.65837549909691,12.8599808296045));
#12435=CARTESIAN_POINT('Ctrl Pts',(-1.3796141756712,6.62717978752738,12.8681810275272));
#12436=CARTESIAN_POINT('Ctrl Pts',(-1.55043620713395,6.58930969255507,12.8763812254499));
#12437=CARTESIAN_POINT('Ctrl Pts',(-1.71952805575321,6.5448844348451,12.8845814233727));
#12438=CARTESIAN_POINT('Ctrl Pts',(-1.8886272278758,6.50045725304164,12.8927819764525));
#12439=CARTESIAN_POINT('Ctrl Pts',(-2.05599572130581,6.44947443387279,12.9009825295324));
#12440=CARTESIAN_POINT('Ctrl Pts',(-2.22109778859676,6.39210556964531,12.9091830826122));
#12441=CARTESIAN_POINT('Ctrl Pts',(-2.38623692631856,6.33472382436462,12.9173854769654));
#12442=CARTESIAN_POINT('Ctrl Pts',(-2.54910828598719,6.27095329575223,12.9255878713186));
#12443=CARTESIAN_POINT('Ctrl Pts',(-2.70919439336898,6.20101239628966,12.9337902656718));
#12444=CARTESIAN_POINT('Ctrl Pts',(-2.86943020940303,6.13100608979105,12.9420003307056));
#12445=CARTESIAN_POINT('Ctrl Pts',(-3.0268752404332,6.05481802732757,12.9502103957395));
#12446=CARTESIAN_POINT('Ctrl Pts',(-3.18103414974751,5.97271385034811,12.9584204607733));
#12447=CARTESIAN_POINT('Ctrl Pts',(-3.33526683678104,5.89057037976607,12.9666344549986));
#12448=CARTESIAN_POINT('Ctrl Pts',(-3.48620995713884,5.80250532987613,12.9748484492239));
#12449=CARTESIAN_POINT('Ctrl Pts',(-3.63339571791366,5.70882865017393,12.9830624434493));
#12450=CARTESIAN_POINT('Ctrl Pts',(-3.78078214190203,5.61502425795739,12.9912876360844));
#12451=CARTESIAN_POINT('Ctrl Pts',(-3.92440067420043,5.51559315026165,12.9995128287196));
#12452=CARTESIAN_POINT('Ctrl Pts',(-4.0638142893429,5.41088739688163,13.0077380213548));
#12453=CARTESIAN_POINT('Ctrl Pts',(-4.18918865484122,5.31672573712818,13.0151349194747));
#12454=CARTESIAN_POINT('Ctrl Pts',(-4.31116265020452,5.21829894024396,13.0225318175947));
#12455=CARTESIAN_POINT('Ctrl Pts',(-4.4294436240944,5.11588879677515,13.0299287157146));
#12456=CARTESIAN_POINT('Ctrl Pts',(-4.56769797344227,4.9961852866816,13.0385746822055));
#12457=CARTESIAN_POINT('Ctrl Pts',(-4.70122024466824,4.87076751104999,13.0472206486964));
#12458=CARTESIAN_POINT('Ctrl Pts',(-4.82953855572552,4.74002598503011,13.0558666151873));
#12459=CARTESIAN_POINT('Ctrl Pts',(-4.95769273021877,4.60945169519562,13.0645015223116));
#12460=CARTESIAN_POINT('Ctrl Pts',(-5.08065600555787,4.47356745071522,13.073136429436));
#12461=CARTESIAN_POINT('Ctrl Pts',(-5.19799090404531,4.33280273742785,13.0817713365604));
#12462=CARTESIAN_POINT('Ctrl Pts',(-5.31922122645921,4.18736474927332,13.0906929156319));
#12463=CARTESIAN_POINT('Ctrl Pts',(-5.43444277310879,4.03671685598993,13.0996144947034));
#12464=CARTESIAN_POINT('Ctrl Pts',(-5.54321367318089,3.88137490761462,13.1085360737749));
#12465=CARTESIAN_POINT('Ctrl Pts',(-5.64819874677098,3.73143971473676,13.1171471327506));
#12466=CARTESIAN_POINT('Ctrl Pts',(-5.7471744107683,3.57713197712779,13.1257581917263));
#12467=CARTESIAN_POINT('Ctrl Pts',(-5.83978328245506,3.41895016254383,13.134369250702));
#12468=CARTESIAN_POINT('Ctrl Pts',(-5.93230481970014,3.26091752071413,13.1429721890515));
#12469=CARTESIAN_POINT('Ctrl Pts',(-6.01847138182566,3.09901834820389,13.151575127401));
#12470=CARTESIAN_POINT('Ctrl Pts',(-6.09796876350521,2.93378014842878,13.1601780657506));
#12471=CARTESIAN_POINT('Ctrl Pts',(-6.17737712650779,2.76872697721207,13.1687713707993));
#12472=CARTESIAN_POINT('Ctrl Pts',(-6.25013107546449,2.60034251203016,13.177364675848));
#12473=CARTESIAN_POINT('Ctrl Pts',(-6.31596214781488,2.42917910977548,13.1859579808968));
#12474=CARTESIAN_POINT('Ctrl Pts',(-6.32329680681988,2.41010870510411,13.1869154157373));
#12475=CARTESIAN_POINT('Ctrl Pts',(-6.33054557508072,2.39100382863419,13.1878728505779));
#12476=CARTESIAN_POINT('Ctrl Pts',(-6.3377081169916,2.37186526257686,13.1888302854184));
#12477=CARTESIAN_POINT('Ctrl Pts',(-6.39853439478797,2.20933529066032,13.1969610856716));
#12478=CARTESIAN_POINT('Ctrl Pts',(-6.45309310219485,2.04449445500953,13.2050918859248));
#12479=CARTESIAN_POINT('Ctrl Pts',(-6.50122165943161,1.87787271531842,13.213222686178));
#12480=CARTESIAN_POINT('Ctrl Pts',(-6.5493880577674,1.71111996921211,13.2213598792764));
#12481=CARTESIAN_POINT('Ctrl Pts',(-6.59111410585841,1.54258387283326,13.2294970723749));
#12482=CARTESIAN_POINT('Ctrl Pts',(-6.62628766982595,1.3728076036767,13.2376342654733));
#12483=CARTESIAN_POINT('Ctrl Pts',(-6.66147613186161,1.20295942430871,13.2457749051505));
#12484=CARTESIAN_POINT('Ctrl Pts',(-6.69010651725162,1.03187038450069,13.2539155448276));
#12485=CARTESIAN_POINT('Ctrl Pts',(-6.7121183391382,0.86009092624247,13.2620561845048));
#12486=CARTESIAN_POINT('Ctrl Pts',(-6.73415609503676,0.688109079897025,
13.2702064153665));
#12487=CARTESIAN_POINT('Ctrl Pts',(-6.74955967681732,0.515435553012798,
13.2783566462283));
#12488=CARTESIAN_POINT('Ctrl Pts',(-6.75832064195188,0.342623847049734,
13.28650687709));
#12489=CARTESIAN_POINT('Ctrl Pts',(-6.76411034278237,0.228420895415216,
13.2918929729897));
#12490=CARTESIAN_POINT('Ctrl Pts',(-6.76700012102719,0.114157610253499,
13.2972790688895));
#12491=CARTESIAN_POINT('Ctrl Pts',(-6.7669999999962,-7.17398757052791E-6,
13.3026651647892));
#12492=CARTESIAN_POINT('Ctrl Pts',(-6.767,1.4554827223919E-12,13.3028202161899));
#12493=CARTESIAN_POINT('Ctrl Pts',(-6.76700000000004,-0.186007249414258,
13.3115697279959));
#12494=CARTESIAN_POINT('Ctrl Pts',(-6.75932637295446,-0.372014355526148,
13.3203192398018));
#12495=CARTESIAN_POINT('Ctrl Pts',(-6.74400518266939,-0.557389537153701,
13.3290687516078));
#12496=CARTESIAN_POINT('Ctrl Pts',(-6.72868405709659,-0.742763935810194,
13.3378182264583));
#12497=CARTESIAN_POINT('Ctrl Pts',(-6.70571545653006,-0.927506129693977,
13.3465677013089));
#12498=CARTESIAN_POINT('Ctrl Pts',(-6.67517739415665,-1.11098863924884,
13.3553171761594));
#12499=CARTESIAN_POINT('Ctrl Pts',(-6.64463945823081,-1.294470389066,13.3640666147814));
#12500=CARTESIAN_POINT('Ctrl Pts',(-6.6065321702713,-1.4766921822834,13.3728160534034));
#12501=CARTESIAN_POINT('Ctrl Pts',(-6.56098496116674,-1.65703510504269,
13.3815654920254));
#12502=CARTESIAN_POINT('Ctrl Pts',(-6.51543793687471,-1.83737729604186,
13.3903148951456));
#12503=CARTESIAN_POINT('Ctrl Pts',(-6.46245112202583,-2.01584035397235,
13.3990642982659));
#12504=CARTESIAN_POINT('Ctrl Pts',(-6.40220448416175,-2.19181813638341,
13.4078137013861));
#12505=CARTESIAN_POINT('Ctrl Pts',(-6.34195808575111,-2.36779521936147,
13.4165630697314));
#12506=CARTESIAN_POINT('Ctrl Pts',(-6.2744520148915,-2.54128677545037,13.4253124380767));
#12507=CARTESIAN_POINT('Ctrl Pts',(-6.19991555136089,-2.71170355238056,
13.4340618064219));
#12508=CARTESIAN_POINT('Ctrl Pts',(-6.12537937788937,-2.88211966613287,
13.442811140719));
#12509=CARTESIAN_POINT('Ctrl Pts',(-6.04381298133509,-3.04946076210659,
13.4515604750161));
#12510=CARTESIAN_POINT('Ctrl Pts',(-5.95549339426192,-3.21315848207067,
13.4603098093131));
#12511=CARTESIAN_POINT('Ctrl Pts',(-5.86717414355034,-3.37685557859857,
13.4690591102887));
#12512=CARTESIAN_POINT('Ctrl Pts',(-5.77210188986098,-3.5369090746754,13.4778084112642));
#12513=CARTESIAN_POINT('Ctrl Pts',(-5.67059953466914,-3.69277536785141,
13.4865577122398));
#12514=CARTESIAN_POINT('Ctrl Pts',(-5.56909755761607,-3.84864108036022,
13.4953069806206));
#12515=CARTESIAN_POINT('Ctrl Pts',(-5.46116568337908,-4.00031938104501,
13.5040562490013));
#12516=CARTESIAN_POINT('Ctrl Pts',(-5.34717048685949,-4.14729511663432,
13.5128055173821));
#12517=CARTESIAN_POINT('Ctrl Pts',(-5.23317570555347,-4.29427031688248,
13.5215547538947));
#12518=CARTESIAN_POINT('Ctrl Pts',(-5.1131178217863,-4.43654275987332,13.5303039904073));
#12519=CARTESIAN_POINT('Ctrl Pts',(-4.98740459171835,-4.57362924147845,
13.53905322692));
#12520=CARTESIAN_POINT('Ctrl Pts',(-4.86169180910641,-4.71071523514631,
13.5478024322911));
#12521=CARTESIAN_POINT('Ctrl Pts',(-4.73032391415233,-4.84261509316718,
13.5565516376622));
#12522=CARTESIAN_POINT('Ctrl Pts',(-4.59374707237085,-4.96888084331716,
13.5653008430333));
#12523=CARTESIAN_POINT('Ctrl Pts',(-4.45717070537192,-5.09514615452908,
13.5740500179895));
#12524=CARTESIAN_POINT('Ctrl Pts',(-4.31538563819297,-5.21577720253808,
13.5827991929458));
#12525=CARTESIAN_POINT('Ctrl Pts',(-4.16887341290434,-5.33036429028817,
13.591548367902));
#12526=CARTESIAN_POINT('Ctrl Pts',(-4.02236168477138,-5.44495098921324,
13.6002975131699));
#12527=CARTESIAN_POINT('Ctrl Pts',(-3.87112305634253,-5.55349359238888,
13.6090466584378));
#12528=CARTESIAN_POINT('Ctrl Pts',(-3.71567117316562,-5.65562346102585,
13.6177958037057));
#12529=CARTESIAN_POINT('Ctrl Pts',(-3.56021980457113,-5.75775299158886,
13.6265449200119));
#12530=CARTESIAN_POINT('Ctrl Pts',(-3.40055544862182,-5.85346967275473,
13.6352940363181));
#12531=CARTESIAN_POINT('Ctrl Pts',(-3.23722036323179,-5.94244842803683,
13.6440431526242));
#12532=CARTESIAN_POINT('Ctrl Pts',(-3.07388580495831,-6.03142689616585,
13.6527922406952));
#12533=CARTESIAN_POINT('Ctrl Pts',(-2.906880792575,-6.1136673448492,13.6615413287661));
#12534=CARTESIAN_POINT('Ctrl Pts',(-2.73677251094418,-6.18889046787389,
13.670290416837));
#12535=CARTESIAN_POINT('Ctrl Pts',(-2.5666647641648,-6.26411335438337,13.6790394773993));
#12536=CARTESIAN_POINT('Ctrl Pts',(-2.39345402971961,-6.3323188435034,13.6877885379615));
#12537=CARTESIAN_POINT('Ctrl Pts',(-2.2177285647394,-6.39327529621077,13.6965375985237));
#12538=CARTESIAN_POINT('Ctrl Pts',(-2.0420036376821,-6.45423156232099,13.7052866323037));
#12539=CARTESIAN_POINT('Ctrl Pts',(-1.86376426620073,-6.5079387425206,13.7140356660836));
#12540=CARTESIAN_POINT('Ctrl Pts',(-1.68361578194709,-6.55421443796117,
13.7227846998636));
#12541=CARTESIAN_POINT('Ctrl Pts',(-1.50346783419883,-6.60048999558676,
13.7315337075879));
#12542=CARTESIAN_POINT('Ctrl Pts',(-1.32141106257256,-6.63933404145494,
13.7402827153121));
#12543=CARTESIAN_POINT('Ctrl Pts',(-1.13806375959048,-6.67061465527029,
13.7490317230363));
#12544=CARTESIAN_POINT('Ctrl Pts',(-0.954716987419194,-6.7018951785248,
13.7577807054312));
#12545=CARTESIAN_POINT('Ctrl Pts',(-0.770079973809923,-6.72561226535827,
13.7665296878261));
#12546=CARTESIAN_POINT('Ctrl Pts',(-0.58477977055251,-6.74168536939782,
13.775278670221));
#12547=CARTESIAN_POINT('Ctrl Pts',(-0.391490647553973,-6.75845143942393,
13.784404850897));
#12548=CARTESIAN_POINT('Ctrl Pts',(-0.197480213104408,-6.76689975924026,
13.7935310315731));
#12549=CARTESIAN_POINT('Ctrl Pts',(-0.00346532629787789,-6.76699911271707,
13.8026572122491));
#12550=CARTESIAN_POINT('Ctrl Pts',(0.184486595295947,-6.76709536139774,
13.8114981997791));
#12551=CARTESIAN_POINT('Ctrl Pts',(0.372442378185097,-6.75935659726771,
13.820339187309));
#12552=CARTESIAN_POINT('Ctrl Pts',(0.559750217721928,-6.74380965729018,
13.8291801748389));
#12553=CARTESIAN_POINT('Ctrl Pts',(0.745129914457576,-6.72842275717255,
13.8379301534367));
#12554=CARTESIAN_POINT('Ctrl Pts',(0.929874656313986,-6.70538772273475,
13.8466801320344));
#12555=CARTESIAN_POINT('Ctrl Pts',(1.11335688289756,-6.67478280180746,13.8554301106322));
#12556=CARTESIAN_POINT('Ctrl Pts',(1.29683723118834,-6.64417819418028,13.8641799996572));
#12557=CARTESIAN_POINT('Ctrl Pts',(1.47905480730212,-6.6060039023008,13.8729298886821));
#12558=CARTESIAN_POINT('Ctrl Pts',(1.65939064804784,-6.5603895979714,13.881679777707));
#12559=CARTESIAN_POINT('Ctrl Pts',(1.83972470264243,-6.51477574543262,13.890429580068));
#12560=CARTESIAN_POINT('Ctrl Pts',(2.01817678125828,-6.46172209820106,13.8991793824289));
#12561=CARTESIAN_POINT('Ctrl Pts',(2.19414072347661,-6.40140886724021,13.9079291847899));
#12562=CARTESIAN_POINT('Ctrl Pts',(2.37010298132087,-6.34109621361378,13.9166789033954));
#12563=CARTESIAN_POINT('Ctrl Pts',(2.54357687926911,-6.27352420825972,13.9254286220009));
#12564=CARTESIAN_POINT('Ctrl Pts',(2.71397317789977,-6.19892237325494,13.9341783406063));
#12565=CARTESIAN_POINT('Ctrl Pts',(2.88436790207209,-6.1243212275696,13.9429279783646));
#12566=CARTESIAN_POINT('Ctrl Pts',(3.05168482126265,-6.04269049717413,13.9516776161229));
#12567=CARTESIAN_POINT('Ctrl Pts',(3.21535561997399,-5.95430745234924,13.9604272538812));
#12568=CARTESIAN_POINT('Ctrl Pts',(3.37902496075288,-5.86592519481512,13.9691768137002));
#12569=CARTESIAN_POINT('Ctrl Pts',(3.53904799384879,-5.77079087940229,13.9779263735192));
#12570=CARTESIAN_POINT('Ctrl Pts',(3.69488118814986,-5.66922763747023,13.9866759333382));
#12571=CARTESIAN_POINT('Ctrl Pts',(3.85071304610831,-5.56766526649053,13.9954254181256));
#12572=CARTESIAN_POINT('Ctrl Pts',(4.00235489705962,-5.45967423580718,14.0041749029131));
#12573=CARTESIAN_POINT('Ctrl Pts',(4.14929168607645,-5.34562133936335,14.0129243877005));
#12574=CARTESIAN_POINT('Ctrl Pts',(4.29622726385748,-5.23156938308538,14.0216738003638));
#12575=CARTESIAN_POINT('Ctrl Pts',(4.43845763092058,-5.1114558367721,14.0304232130271));
#12576=CARTESIAN_POINT('Ctrl Pts',(4.57549970660954,-4.98568866204219,14.0391726256904));
#12577=CARTESIAN_POINT('Ctrl Pts',(4.71254069815277,-4.85992248226178,14.0479219691367));
#12578=CARTESIAN_POINT('Ctrl Pts',(4.84439326931288,-4.72850295734028,14.056671312583));
#12579=CARTESIAN_POINT('Ctrl Pts',(4.97060959434664,-4.59187644221718,14.0654206560294));
#12580=CARTESIAN_POINT('Ctrl Pts',(5.0968249628049,-4.45525096256693,14.0741699331657));
#12581=CARTESIAN_POINT('Ctrl Pts',(5.21740397615822,-4.31341878218347,14.082919210302));
#12582=CARTESIAN_POINT('Ctrl Pts',(5.33193710451924,-4.16686161438689,14.0916684874383));
#12583=CARTESIAN_POINT('Ctrl Pts',(5.44646940289382,-4.02030550864516,14.1004177011712));
#12584=CARTESIAN_POINT('Ctrl Pts',(5.55495572749671,-3.86902470980125,14.1091669149042));
#12585=CARTESIAN_POINT('Ctrl Pts',(5.65702762491469,-3.71353301465762,14.1179161286372));
#12586=CARTESIAN_POINT('Ctrl Pts',(5.75909881655169,-3.55804239466869,14.1266652818733));
#12587=CARTESIAN_POINT('Ctrl Pts',(5.85475551250798,-3.39834117619525,14.1354144351094));
#12588=CARTESIAN_POINT('Ctrl Pts',(5.94367283728112,-3.23497174691937,14.1441635883455));
#12589=CARTESIAN_POINT('Ctrl Pts',(6.0325895767633,-3.0716033930093,14.1529126839911));
#12590=CARTESIAN_POINT('Ctrl Pts',(6.11476689685303,-2.90456712829465,14.1616617796366));
#12591=CARTESIAN_POINT('Ctrl Pts',(6.1899257052528,-2.73443024475861,14.1704108752821));
#12592=CARTESIAN_POINT('Ctrl Pts',(6.26508404388712,-2.56429442462993,14.1791599162431));
#12593=CARTESIAN_POINT('Ctrl Pts',(6.33322384283326,-2.39105828655963,14.1879089572042));
#12594=CARTESIAN_POINT('Ctrl Pts',(6.3941136872004,-2.21531017132059,14.1966579981652));
#12595=CARTESIAN_POINT('Ctrl Pts',(6.45500317120898,-2.03956309619489,14.2054069873476));
#12596=CARTESIAN_POINT('Ctrl Pts',(6.50864269270082,-1.86130434438603,14.21415597653));
#12597=CARTESIAN_POINT('Ctrl Pts',(6.55485008446342,-1.6811393071991,14.2229049657124));
#12598=CARTESIAN_POINT('Ctrl Pts',(6.60199664749412,-1.49731239211805,14.2318317792418));
#12599=CARTESIAN_POINT('Ctrl Pts',(6.64140563640914,-1.31150116499636,14.2407585927711));
#12600=CARTESIAN_POINT('Ctrl Pts',(6.67293772282178,-1.12436255155624,14.2496854063005));
#12601=CARTESIAN_POINT('Ctrl Pts',(6.70384494949876,-0.940932395050984,
14.258435320456));
#12602=CARTESIAN_POINT('Ctrl Pts',(6.72718449348934,-0.756227260506354,
14.2671852346116));
#12603=CARTESIAN_POINT('Ctrl Pts',(6.74287707373935,-0.57087456454133,14.2759351487671));
#12604=CARTESIAN_POINT('Ctrl Pts',(6.75856934538672,-0.385525513632149,
14.2846848908511));
#12605=CARTESIAN_POINT('Ctrl Pts',(6.76661493004104,-0.199529212417939,
14.293434632935));
#12606=CARTESIAN_POINT('Ctrl Pts',(6.76698649908907,-0.0135174386001735,
14.302184375019));
#12607=CARTESIAN_POINT('Ctrl Pts',(6.76735806132389,0.172490924446043,14.3109339566649));
#12608=CARTESIAN_POINT('Ctrl Pts',(6.76005588896288,0.358514472901682,14.3196835383108));
#12609=CARTESIAN_POINT('Ctrl Pts',(6.74510478454582,0.543921359662496,14.3284331199567));
#12610=CARTESIAN_POINT('Ctrl Pts',(6.73015393440685,0.729325093150733,14.3371825527958));
#12611=CARTESIAN_POINT('Ctrl Pts',(6.70755443556893,0.914111900256644,14.3459319856348));
#12612=CARTESIAN_POINT('Ctrl Pts',(6.67738304682314,1.09765415591568,14.3546814184738));
#12613=CARTESIAN_POINT('Ctrl Pts',(6.64721213111854,1.28119353391305,14.3634307141352));
#12614=CARTESIAN_POINT('Ctrl Pts',(6.60946960955487,1.46348811672688,14.3721800097965));
#12615=CARTESIAN_POINT('Ctrl Pts',(6.56428366991173,1.64391876348259,14.3809293054578));
#12616=CARTESIAN_POINT('Ctrl Pts',(6.51909837867706,1.82434682109758,14.3896784755687));
#12617=CARTESIAN_POINT('Ctrl Pts',(6.46646995271907,2.00291071820492,14.3984276456795));
#12618=CARTESIAN_POINT('Ctrl Pts',(6.40657713281532,2.17900400212755,14.4071768157903));
#12619=CARTESIAN_POINT('Ctrl Pts',(6.34668509279042,2.35509499309707,14.4159258719761));
#12620=CARTESIAN_POINT('Ctrl Pts',(6.27952894037507,2.5287151639817,14.4246749281619));
#12621=CARTESIAN_POINT('Ctrl Pts',(6.20533675061427,2.69927486771466,14.4334239843476));
#12622=CARTESIAN_POINT('Ctrl Pts',(6.12832117907898,2.87632521635964,14.4425059856299));
#12623=CARTESIAN_POINT('Ctrl Pts',(6.04372366626061,3.05007728920032,14.4515879869122));
#12624=CARTESIAN_POINT('Ctrl Pts',(5.95185378007852,3.21989527478226,14.4606699881944));
#12625=CARTESIAN_POINT('Ctrl Pts',(5.86334450817353,3.38350129286784,14.4694197685016));
#12626=CARTESIAN_POINT('Ctrl Pts',(5.76808562057235,3.54345567124996,14.4781695488087));
#12627=CARTESIAN_POINT('Ctrl Pts',(5.6664006880446,3.69921508465345,14.4869193291158));
#12628=CARTESIAN_POINT('Ctrl Pts',(5.56471941107898,3.85496889852319,14.4956687948693));
#12629=CARTESIAN_POINT('Ctrl Pts',(5.45661270815087,4.00652780919673,14.5044182606228));
#12630=CARTESIAN_POINT('Ctrl Pts',(5.34244776449086,4.15337704569265,14.5131677263763));
#12631=CARTESIAN_POINT('Ctrl Pts',(5.22828631819565,4.30022178356286,14.5219169240959));
#12632=CARTESIAN_POINT('Ctrl Pts',(5.10806717844037,4.44235690972716,14.5306661218155));
#12633=CARTESIAN_POINT('Ctrl Pts',(4.98219864544685,4.57929969070682,14.5394153195351));
#12634=CARTESIAN_POINT('Ctrl Pts',(4.85633329943983,4.71623900430044,14.5481642957253));
#12635=CARTESIAN_POINT('Ctrl Pts',(4.72481904033599,4.84798602483665,14.5569132719155));
#12636=CARTESIAN_POINT('Ctrl Pts',(4.58810250737141,4.97409332259178,14.5656622481058));
#12637=CARTESIAN_POINT('Ctrl Pts',(4.45137708685583,5.10020881822187,14.574411793042));
#12638=CARTESIAN_POINT('Ctrl Pts',(4.3094489263599,5.22068366307983,14.5831613379781));
#12639=CARTESIAN_POINT('Ctrl Pts',(4.16280009466598,5.33510865604899,14.5919108829143));
#12640=CARTESIAN_POINT('Ctrl Pts',(4.01615988348714,5.44952692272947,14.6006599135226));
#12641=CARTESIAN_POINT('Ctrl Pts',(3.86479978232144,5.55789587288687,14.6094089441309));
#12642=CARTESIAN_POINT('Ctrl Pts',(3.70923383580967,5.65984746713944,14.6181579747392));
#12643=CARTESIAN_POINT('Ctrl Pts',(3.5536657779943,5.76180044505452,14.6269071240872));
#12644=CARTESIAN_POINT('Ctrl Pts',(3.39389200026718,5.8573357357113,14.6356562734352));
#12645=CARTESIAN_POINT('Ctrl Pts',(3.23045513625908,5.94612887622,14.6444054227832));
#12646=CARTESIAN_POINT('Ctrl Pts',(3.18695122151489,5.96976399206735,14.6467342868962));
#12647=CARTESIAN_POINT('Ctrl Pts',(3.14318791262619,5.99292165435356,14.6490631510091));
#12648=CARTESIAN_POINT('Ctrl Pts',(3.09917575053259,6.01559628526639,14.6513920151221));
#12649=CARTESIAN_POINT('Origin',(0.,0.,-3.69717978381041));
#12650=CARTESIAN_POINT('',(3.0991757505326,6.01559628526638,17.0457515827422));
#12651=CARTESIAN_POINT('',(3.09917575053259,6.01559628526639,16.6515033120574));
#12652=CARTESIAN_POINT('',(3.09917575053259,6.01559628526639,-3.69717978381041));
#12653=CARTESIAN_POINT('',(-6.767,1.53662130762677E-12,15.69717978381));
#12654=CARTESIAN_POINT('Ctrl Pts',(-6.767,1.58470424476328E-12,15.69717978381));
#12655=CARTESIAN_POINT('Ctrl Pts',(-6.76700000000004,-0.186007249414097,
15.705929295616));
#12656=CARTESIAN_POINT('Ctrl Pts',(-6.75932637295447,-0.372014355525955,
15.7146788074219));
#12657=CARTESIAN_POINT('Ctrl Pts',(-6.74400518266941,-0.557389537153476,
15.7234283192279));
#12658=CARTESIAN_POINT('Ctrl Pts',(-6.72868405709662,-0.742763935809937,
15.7321777940784));
#12659=CARTESIAN_POINT('Ctrl Pts',(-6.7057154565301,-0.92750612969369,15.7409272689289));
#12660=CARTESIAN_POINT('Ctrl Pts',(-6.67517739415671,-1.11098863924853,
15.7496767437795));
#12661=CARTESIAN_POINT('Ctrl Pts',(-6.6446394582309,-1.29447038906553,15.7584261824015));
#12662=CARTESIAN_POINT('Ctrl Pts',(-6.60653217027144,-1.47669218228277,
15.7671756210235));
#12663=CARTESIAN_POINT('Ctrl Pts',(-6.56098496116694,-1.65703510504191,
15.7759250596455));
#12664=CARTESIAN_POINT('Ctrl Pts',(-6.51543793687494,-1.83737729604105,
15.7846744627657));
#12665=CARTESIAN_POINT('Ctrl Pts',(-6.46245112202609,-2.01584035397152,
15.7934238658859));
#12666=CARTESIAN_POINT('Ctrl Pts',(-6.40220448416204,-2.19181813638255,
15.8021732690062));
#12667=CARTESIAN_POINT('Ctrl Pts',(-6.34195808575144,-2.3677952193606,15.8109226373514));
#12668=CARTESIAN_POINT('Ctrl Pts',(-6.27445201489186,-2.54128677544947,
15.8196720056967));
#12669=CARTESIAN_POINT('Ctrl Pts',(-6.19991555136129,-2.71170355237965,
15.828421374042));
#12670=CARTESIAN_POINT('Ctrl Pts',(-6.12537937788975,-2.88211966613208,
15.8371707083391));
#12671=CARTESIAN_POINT('Ctrl Pts',(-6.04381298133543,-3.04946076210593,
15.8459200426361));
#12672=CARTESIAN_POINT('Ctrl Pts',(-5.95549339426221,-3.21315848207013,
15.8546693769332));
#12673=CARTESIAN_POINT('Ctrl Pts',(-5.86717414355068,-3.37685557859797,
15.8634186779088));
#12674=CARTESIAN_POINT('Ctrl Pts',(-5.77210188986139,-3.53690907467474,
15.8721679788843));
#12675=CARTESIAN_POINT('Ctrl Pts',(-5.67059953466961,-3.69277536785069,
15.8809172798599));
#12676=CARTESIAN_POINT('Ctrl Pts',(-5.56909755761669,-3.84864108035931,
15.8896665482406));
#12677=CARTESIAN_POINT('Ctrl Pts',(-5.46116568337986,-4.00031938104392,
15.8984158166214));
#12678=CARTESIAN_POINT('Ctrl Pts',(-5.34717048686045,-4.14729511663308,
15.9071650850021));
#12679=CARTESIAN_POINT('Ctrl Pts',(-5.2331757055545,-4.29427031688122,15.9159143215147));
#12680=CARTESIAN_POINT('Ctrl Pts',(-5.11311782178739,-4.43654275987205,
15.9246635580274));
#12681=CARTESIAN_POINT('Ctrl Pts',(-4.98740459171951,-4.57362924147719,
15.93341279454));
#12682=CARTESIAN_POINT('Ctrl Pts',(-4.86169180910741,-4.71071523514529,
15.9421619999111));
#12683=CARTESIAN_POINT('Ctrl Pts',(-4.73032391415315,-4.84261509316638,
15.9509112052822));
#12684=CARTESIAN_POINT('Ctrl Pts',(-4.59374707237148,-4.96888084331658,
15.9596604106534));
#12685=CARTESIAN_POINT('Ctrl Pts',(-4.4571707053728,-5.0951461545283,15.9684095856096));
#12686=CARTESIAN_POINT('Ctrl Pts',(-4.31538563819412,-5.21577720253712,
15.9771587605658));
#12687=CARTESIAN_POINT('Ctrl Pts',(-4.16887341290578,-5.33036429028705,
15.985907935522));
#12688=CARTESIAN_POINT('Ctrl Pts',(-4.02236168477261,-5.44495098921234,
15.9946570807899));
#12689=CARTESIAN_POINT('Ctrl Pts',(-3.87112305634355,-5.55349359238818,
16.0034062260579));
#12690=CARTESIAN_POINT('Ctrl Pts',(-3.71567117316642,-5.65562346102533,
16.0121553713258));
#12691=CARTESIAN_POINT('Ctrl Pts',(-3.56021980457218,-5.7577529915882,16.0209044876319));
#12692=CARTESIAN_POINT('Ctrl Pts',(-3.40055544862314,-5.85346967275396,
16.0296536039381));
#12693=CARTESIAN_POINT('Ctrl Pts',(-3.23722036323339,-5.94244842803596,
16.0384027202442));
#12694=CARTESIAN_POINT('Ctrl Pts',(-3.0738858049597,-6.03142689616515,16.0471518083152));
#12695=CARTESIAN_POINT('Ctrl Pts',(-2.90688079257619,-6.11366734484865,
16.0559008963862));
#12696=CARTESIAN_POINT('Ctrl Pts',(-2.73677251094514,-6.18889046787347,
16.0646499844571));
#12697=CARTESIAN_POINT('Ctrl Pts',(-2.56666476416559,-6.26411335438305,
16.0733990450193));
#12698=CARTESIAN_POINT('Ctrl Pts',(-2.39345402972023,-6.33231884350316,
16.0821481055815));
#12699=CARTESIAN_POINT('Ctrl Pts',(-2.21772856473985,-6.39327529621062,
16.0908971661438));
#12700=CARTESIAN_POINT('Ctrl Pts',(-2.04200363768211,-6.454231562321,16.0996461999238));
#12701=CARTESIAN_POINT('Ctrl Pts',(-1.8637642662003,-6.50793874252074,16.1083952337038));
#12702=CARTESIAN_POINT('Ctrl Pts',(-1.6836157819462,-6.5542144379614,16.1171442674838));
#12703=CARTESIAN_POINT('Ctrl Pts',(-1.50346783419814,-6.60048999558692,
16.125893275208));
#12704=CARTESIAN_POINT('Ctrl Pts',(-1.32141106257207,-6.63933404145503,
16.1346422829322));
#12705=CARTESIAN_POINT('Ctrl Pts',(-1.13806375959019,-6.67061465527034,
16.1433912906564));
#12706=CARTESIAN_POINT('Ctrl Pts',(-0.954716987418967,-6.70189517852483,
16.1521402730513));
#12707=CARTESIAN_POINT('Ctrl Pts',(-0.77007997380976,-6.72561226535829,
16.1608892554462));
#12708=CARTESIAN_POINT('Ctrl Pts',(-0.584779770552411,-6.74168536939782,
16.1696382378411));
#12709=CARTESIAN_POINT('Ctrl Pts',(-0.391490647553874,-6.75845143942394,
16.1787644185171));
#12710=CARTESIAN_POINT('Ctrl Pts',(-0.197480213104304,-6.76689975924027,
16.1878905991932));
#12711=CARTESIAN_POINT('Ctrl Pts',(-0.00346532629777421,-6.76699911271707,
16.1970167798692));
#12712=CARTESIAN_POINT('Ctrl Pts',(0.184486595296051,-6.76709536139773,
16.2058577673992));
#12713=CARTESIAN_POINT('Ctrl Pts',(0.372442378185195,-6.7593565972677,16.2146987549291));
#12714=CARTESIAN_POINT('Ctrl Pts',(0.559750217722025,-6.74380965729017,
16.223539742459));
#12715=CARTESIAN_POINT('Ctrl Pts',(0.745129914457625,-6.72842275717255,
16.2322897210568));
#12716=CARTESIAN_POINT('Ctrl Pts',(0.929874656313991,-6.70538772273475,
16.2410396996546));
#12717=CARTESIAN_POINT('Ctrl Pts',(1.11335688289751,-6.67478280180747,16.2497896782523));
#12718=CARTESIAN_POINT('Ctrl Pts',(1.29683723118834,-6.64417819418028,16.2585395672773));
#12719=CARTESIAN_POINT('Ctrl Pts',(1.47905480730217,-6.60600390230079,16.2672894563022));
#12720=CARTESIAN_POINT('Ctrl Pts',(1.65939064804794,-6.56038959797138,16.2760393453271));
#12721=CARTESIAN_POINT('Ctrl Pts',(1.83972470264254,-6.51477574543259,16.2847891476881));
#12722=CARTESIAN_POINT('Ctrl Pts',(2.0181767812584,-6.46172209820103,16.293538950049));
#12723=CARTESIAN_POINT('Ctrl Pts',(2.19414072347675,-6.40140886724016,16.30228875241));
#12724=CARTESIAN_POINT('Ctrl Pts',(2.37010298132085,-6.34109621361378,16.3110384710155));
#12725=CARTESIAN_POINT('Ctrl Pts',(2.54357687926895,-6.27352420825978,16.319788189621));
#12726=CARTESIAN_POINT('Ctrl Pts',(2.71397317789947,-6.19892237325507,16.3285379082264));
#12727=CARTESIAN_POINT('Ctrl Pts',(2.88436790207177,-6.12432122756975,16.3372875459847));
#12728=CARTESIAN_POINT('Ctrl Pts',(3.05168482126232,-6.04269049717429,16.346037183743));
#12729=CARTESIAN_POINT('Ctrl Pts',(3.21535561997365,-5.95430745234942,16.3547868215012));
#12730=CARTESIAN_POINT('Ctrl Pts',(3.37902496075253,-5.86592519481532,16.3635363813203));
#12731=CARTESIAN_POINT('Ctrl Pts',(3.53904799384844,-5.77079087940251,16.3722859411393));
#12732=CARTESIAN_POINT('Ctrl Pts',(3.6948811881495,-5.66922763747047,16.3810355009583));
#12733=CARTESIAN_POINT('Ctrl Pts',(3.85071304610794,-5.56766526649079,16.3897849857457));
#12734=CARTESIAN_POINT('Ctrl Pts',(4.00235489705925,-5.45967423580745,16.3985344705331));
#12735=CARTESIAN_POINT('Ctrl Pts',(4.14929168607607,-5.34562133936365,16.4072839553206));
#12736=CARTESIAN_POINT('Ctrl Pts',(4.2962272638571,-5.2315693830857,16.4160333679839));
#12737=CARTESIAN_POINT('Ctrl Pts',(4.4384576309202,-5.11145583677243,16.4247827806472));
#12738=CARTESIAN_POINT('Ctrl Pts',(4.57549970660915,-4.98568866204255,16.4335321933105));
#12739=CARTESIAN_POINT('Ctrl Pts',(4.71254069815248,-4.85992248226207,16.4422815367568));
#12740=CARTESIAN_POINT('Ctrl Pts',(4.84439326931267,-4.72850295734051,16.4510308802031));
#12741=CARTESIAN_POINT('Ctrl Pts',(4.97060959434651,-4.59187644221732,16.4597802236495));
#12742=CARTESIAN_POINT('Ctrl Pts',(5.09682496280474,-4.45525096256711,16.4685295007858));
#12743=CARTESIAN_POINT('Ctrl Pts',(5.21740397615804,-4.31341878218369,16.4772787779221));
#12744=CARTESIAN_POINT('Ctrl Pts',(5.33193710451904,-4.16686161438716,16.4860280550583));
#12745=CARTESIAN_POINT('Ctrl Pts',(5.4464694028936,-4.02030550864546,16.4947772687913));
#12746=CARTESIAN_POINT('Ctrl Pts',(5.55495572749648,-3.86902470980158,16.5035264825243));
#12747=CARTESIAN_POINT('Ctrl Pts',(5.65702762491445,-3.71353301465798,16.5122756962573));
#12748=CARTESIAN_POINT('Ctrl Pts',(5.75909881655151,-3.55804239466898,16.5210248494934));
#12749=CARTESIAN_POINT('Ctrl Pts',(5.85475551250787,-3.39834117619546,16.5297740027295));
#12750=CARTESIAN_POINT('Ctrl Pts',(5.94367283728105,-3.2349717469195,16.5385231559656));
#12751=CARTESIAN_POINT('Ctrl Pts',(6.03258957676328,-3.07160339300933,16.5472722516112));
#12752=CARTESIAN_POINT('Ctrl Pts',(6.11476689685307,-2.90456712829458,16.5560213472567));
#12753=CARTESIAN_POINT('Ctrl Pts',(6.18992570525288,-2.73443024475844,16.5647704429022));
#12754=CARTESIAN_POINT('Ctrl Pts',(6.26508404388724,-2.56429442462965,16.5735194838633));
#12755=CARTESIAN_POINT('Ctrl Pts',(6.33322384283341,-2.39105828655925,16.5822685248243));
#12756=CARTESIAN_POINT('Ctrl Pts',(6.39411368720057,-2.2153101713201,16.5910175657853));
#12757=CARTESIAN_POINT('Ctrl Pts',(6.4550031712091,-2.0395630961945,16.5997665549677));
#12758=CARTESIAN_POINT('Ctrl Pts',(6.5086426927009,-1.86130434438574,16.6085155441501));
#12759=CARTESIAN_POINT('Ctrl Pts',(6.55485008446347,-1.68113930719892,16.6172645333325));
#12760=CARTESIAN_POINT('Ctrl Pts',(6.60199664749416,-1.49731239211787,16.6261913468619));
#12761=CARTESIAN_POINT('Ctrl Pts',(6.64140563640917,-1.31150116499617,16.6351181603913));
#12762=CARTESIAN_POINT('Ctrl Pts',(6.67293772282181,-1.12436255155606,16.6440449739206));
#12763=CARTESIAN_POINT('Ctrl Pts',(6.70384494949879,-0.940932395050799,
16.6527948880762));
#12764=CARTESIAN_POINT('Ctrl Pts',(6.72718449348936,-0.756227260506168,
16.6615448022317));
#12765=CARTESIAN_POINT('Ctrl Pts',(6.74287707373937,-0.570874564541144,
16.6702947163872));
#12766=CARTESIAN_POINT('Ctrl Pts',(6.75856934538673,-0.385525513631947,
16.6790444584712));
#12767=CARTESIAN_POINT('Ctrl Pts',(6.76661493004104,-0.19952921241772,16.6877942005552));
#12768=CARTESIAN_POINT('Ctrl Pts',(6.76698649908907,-0.0135174385999383,
16.6965439426391));
#12769=CARTESIAN_POINT('Ctrl Pts',(6.76735806132388,0.172490924446294,16.705293524285));
#12770=CARTESIAN_POINT('Ctrl Pts',(6.76005588896286,0.358514472901948,16.7140431059309));
#12771=CARTESIAN_POINT('Ctrl Pts',(6.7451047845458,0.543921359662778,16.7227926875768));
#12772=CARTESIAN_POINT('Ctrl Pts',(6.73015393440681,0.729325093151046,16.7315421204159));
#12773=CARTESIAN_POINT('Ctrl Pts',(6.70755443556889,0.914111900256987,16.7402915532549));
#12774=CARTESIAN_POINT('Ctrl Pts',(6.67738304682308,1.09765415591605,16.749040986094));
#12775=CARTESIAN_POINT('Ctrl Pts',(6.64721213111846,1.28119353391347,16.7577902817553));
#12776=CARTESIAN_POINT('Ctrl Pts',(6.60946960955476,1.46348811672734,16.7665395774166));
#12777=CARTESIAN_POINT('Ctrl Pts',(6.56428366991161,1.6439187634831,16.775288873078));
#12778=CARTESIAN_POINT('Ctrl Pts',(6.51909837867692,1.82434682109806,16.7840380431888));
#12779=CARTESIAN_POINT('Ctrl Pts',(6.46646995271892,2.00291071820538,16.7927872132996));
#12780=CARTESIAN_POINT('Ctrl Pts',(6.40657713281517,2.17900400212799,16.8015363834104));
#12781=CARTESIAN_POINT('Ctrl Pts',(6.34668509279023,2.35509499309758,16.8102854395962));
#12782=CARTESIAN_POINT('Ctrl Pts',(6.27952894037484,2.52871516398226,16.819034495782));
#12783=CARTESIAN_POINT('Ctrl Pts',(6.205336750614,2.69927486771527,16.8277835519678));
#12784=CARTESIAN_POINT('Ctrl Pts',(6.12832117907871,2.87632521636021,16.83686555325));
#12785=CARTESIAN_POINT('Ctrl Pts',(6.04372366626034,3.05007728920086,16.8459475545323));
#12786=CARTESIAN_POINT('Ctrl Pts',(5.95185378007825,3.21989527478275,16.8550295558146));
#12787=CARTESIAN_POINT('Ctrl Pts',(5.86334450817326,3.3835012928683,16.8637793361217));
#12788=CARTESIAN_POINT('Ctrl Pts',(5.76808562057208,3.54345567125039,16.8725291164288));
#12789=CARTESIAN_POINT('Ctrl Pts',(5.66640068804435,3.69921508465385,16.8812788967359));
#12790=CARTESIAN_POINT('Ctrl Pts',(5.56471941107871,3.85496889852359,16.8900283624894));
#12791=CARTESIAN_POINT('Ctrl Pts',(5.45661270815058,4.00652780919714,16.8987778282429));
#12792=CARTESIAN_POINT('Ctrl Pts',(5.34244776449054,4.15337704569306,16.9075272939964));
#12793=CARTESIAN_POINT('Ctrl Pts',(5.22828631819538,4.30022178356319,16.916276491716));
#12794=CARTESIAN_POINT('Ctrl Pts',(5.10806717844015,4.4423569097274,16.9250256894356));
#12795=CARTESIAN_POINT('Ctrl Pts',(4.98219864544669,4.57929969070699,16.9337748871552));
#12796=CARTESIAN_POINT('Ctrl Pts',(4.85633329943964,4.71623900430064,16.9425238633454));
#12797=CARTESIAN_POINT('Ctrl Pts',(4.72481904033576,4.84798602483688,16.9512728395357));
#12798=CARTESIAN_POINT('Ctrl Pts',(4.58810250737114,4.97409332259204,16.9600218157259));
#12799=CARTESIAN_POINT('Ctrl Pts',(4.4513770868555,5.10020881822216,16.9687713606621));
#12800=CARTESIAN_POINT('Ctrl Pts',(4.30944892635952,5.22068366308015,16.9775209055983));
#12801=CARTESIAN_POINT('Ctrl Pts',(4.16280009466554,5.33510865604934,16.9862704505345));
#12802=CARTESIAN_POINT('Ctrl Pts',(4.01615988348669,5.4495269227298,16.9950194811427));
#12803=CARTESIAN_POINT('Ctrl Pts',(3.86479978232097,5.5578958728872,17.003768511751));
#12804=CARTESIAN_POINT('Ctrl Pts',(3.7092338358092,5.65984746713974,17.0125175423593));
#12805=CARTESIAN_POINT('Ctrl Pts',(3.55366577799386,5.76180044505479,17.0212666917073));
#12806=CARTESIAN_POINT('Ctrl Pts',(3.39389200026678,5.85733573571153,17.0300158410554));
#12807=CARTESIAN_POINT('Ctrl Pts',(3.23045513625871,5.9461288762202,17.0387649904034));
#12808=CARTESIAN_POINT('Ctrl Pts',(3.18695122151465,5.96976399206748,17.0410938545163));
#12809=CARTESIAN_POINT('Ctrl Pts',(3.14318791262608,5.99292165435362,17.0434227186293));
#12810=CARTESIAN_POINT('Ctrl Pts',(3.0991757505326,6.01559628526638,17.0457515827422));
#12811=CARTESIAN_POINT('Ctrl Pts',(3.09917575053257,6.0155962852664,15.0458593505058));
#12812=CARTESIAN_POINT('Ctrl Pts',(2.93718592831312,6.09905184063424,15.0544103860842));
#12813=CARTESIAN_POINT('Ctrl Pts',(2.77176774995393,6.17598800827926,15.0629614216626));
#12814=CARTESIAN_POINT('Ctrl Pts',(2.60349464973925,6.24612716879661,15.071512457241));
#12815=CARTESIAN_POINT('Ctrl Pts',(2.44214626671966,6.31337998651606,15.0797116035215));
#12816=CARTESIAN_POINT('Ctrl Pts',(2.27817359794682,6.37438389895123,15.0879107498019));
#12817=CARTESIAN_POINT('Ctrl Pts',(2.11210332844844,6.42894303365312,15.0961098960823));
#12818=CARTESIAN_POINT('Ctrl Pts',(1.9460151590607,6.48350804901311,15.104309926108));
#12819=CARTESIAN_POINT('Ctrl Pts',(1.77782927902566,6.53162679041381,15.1125099561337));
#12820=CARTESIAN_POINT('Ctrl Pts',(1.60808817656457,6.57315308024948,15.1207099861594));
#12821=CARTESIAN_POINT('Ctrl Pts',(1.43829798567515,6.6146913793173,15.1289123876));
#12822=CARTESIAN_POINT('Ctrl Pts',(1.26695202452738,6.6496333437127,15.1371147890406));
#12823=CARTESIAN_POINT('Ctrl Pts',(1.09460368215074,6.67788377998764,15.1453171904812));
#12824=CARTESIAN_POINT('Ctrl Pts',(0.922174230900824,6.70614751120366,15.1535234520549));
#12825=CARTESIAN_POINT('Ctrl Pts',(0.748741812018114,6.72771338321376,15.1617297136286));
#12826=CARTESIAN_POINT('Ctrl Pts',(0.57486570941015,6.74253798032643,15.1699359752023));
#12827=CARTESIAN_POINT('Ctrl Pts',(0.4007841667395,6.75738009316503,15.1781519327311));
#12828=CARTESIAN_POINT('Ctrl Pts',(0.226258250536156,6.76546499416257,15.18636789026));
#12829=CARTESIAN_POINT('Ctrl Pts',(0.0518489695518635,6.76680136285649,
15.1945838477888));
#12830=CARTESIAN_POINT('Ctrl Pts',(-0.122681401712306,6.76813865937523,
15.2028055095588));
#12831=CARTESIAN_POINT('Ctrl Pts',(-0.297094619409528,6.76271809633917,
15.2110271713288));
#12832=CARTESIAN_POINT('Ctrl Pts',(-0.470834143085268,6.750600285138,15.2192488330988));
#12833=CARTESIAN_POINT('Ctrl Pts',(-0.644813884131266,6.73846571949501,
15.22748186238));
#12834=CARTESIAN_POINT('Ctrl Pts',(-0.818117716461157,6.71961545386714,
15.2357148916611));
#12835=CARTESIAN_POINT('Ctrl Pts',(-0.99019775338741,6.69416144182276,15.2439479209422));
#12836=CARTESIAN_POINT('Ctrl Pts',(-1.03991667121275,6.68680703886141,15.2463266820908));
#12837=CARTESIAN_POINT('Ctrl Pts',(-1.08953351489694,6.67890167599312,15.2487054432393));
#12838=CARTESIAN_POINT('Ctrl Pts',(-1.13903530317154,6.6704488288367,15.2510842043879));
#12839=CARTESIAN_POINT('Ctrl Pts',(-1.30871700656454,6.64147424925049,15.2592380965546));
#12840=CARTESIAN_POINT('Ctrl Pts',(-1.47757036354887,6.60597347987454,15.2673919887213));
#12841=CARTESIAN_POINT('Ctrl Pts',(-1.64504892350012,6.56400053620436,15.2755458808881));
#12842=CARTESIAN_POINT('Ctrl Pts',(-1.81232311281691,6.52207881125214,15.2836898230283));
#12843=CARTESIAN_POINT('Ctrl Pts',(-1.97822549371729,6.47370072081307,15.2918337651685));
#12844=CARTESIAN_POINT('Ctrl Pts',(-2.14221597580984,6.41897185793684,15.2999777073087));
#12845=CARTESIAN_POINT('Ctrl Pts',(-2.30604086042381,6.36429826022955,15.3081134257016));
#12846=CARTESIAN_POINT('Ctrl Pts',(-2.46795734550539,6.30328677200131,15.3162491440945));
#12847=CARTESIAN_POINT('Ctrl Pts',(-2.62743676387958,6.23609373340507,15.3243848624874));
#12848=CARTESIAN_POINT('Ctrl Pts',(-2.78678868657676,6.16895441222286,15.3325140767876));
#12849=CARTESIAN_POINT('Ctrl Pts',(-2.9437070864688,6.09564352169102,15.3406432910878));
#12850=CARTESIAN_POINT('Ctrl Pts',(-3.09767967482999,6.0163668132973,15.3487725053879));
#12851=CARTESIAN_POINT('Ctrl Pts',(-3.25156154459385,5.93713681368379,15.3568969300634));
#12852=CARTESIAN_POINT('Ctrl Pts',(-3.40250073499562,5.85194816311061,15.3650213547388));
#12853=CARTESIAN_POINT('Ctrl Pts',(-3.55000613246669,5.76105419688523,15.3731457794143));
#12854=CARTESIAN_POINT('Ctrl Pts',(-3.69840698212802,5.66960844609784,15.3813195245484));
#12855=CARTESIAN_POINT('Ctrl Pts',(-3.84333186589893,5.57238802888942,15.3894932696826));
#12856=CARTESIAN_POINT('Ctrl Pts',(-3.98430646117621,5.46969752577138,15.3976670148168));
#12857=CARTESIAN_POINT('Ctrl Pts',(-4.12437829639739,5.36766462258596,15.405788417679));
#12858=CARTESIAN_POINT('Ctrl Pts',(-4.26055000252925,5.26023172297751,15.4139098205411));
#12859=CARTESIAN_POINT('Ctrl Pts',(-4.3923863096306,5.14774042731077,15.4220312234033));
#12860=CARTESIAN_POINT('Ctrl Pts',(-4.52423280962096,5.03524043440944,15.4301532541695));
#12861=CARTESIAN_POINT('Ctrl Pts',(-4.65174296446796,4.91768150396285,15.4382752849358));
#12862=CARTESIAN_POINT('Ctrl Pts',(-4.77451564793939,4.79544464336541,15.446397315702));
#12863=CARTESIAN_POINT('Ctrl Pts',(-4.89732120230261,4.67317505533621,15.4545215210431));
#12864=CARTESIAN_POINT('Ctrl Pts',(-5.01538650043006,4.54622530140399,15.4626457263843));
#12865=CARTESIAN_POINT('Ctrl Pts',(-5.12834828740515,4.41501221324117,15.4707699317254));
#12866=CARTESIAN_POINT('Ctrl Pts',(-5.24253280756064,4.28237883419153,15.4789820759679));
#12867=CARTESIAN_POINT('Ctrl Pts',(-5.3515024361904,4.14538957662682,15.4871942202103));
#12868=CARTESIAN_POINT('Ctrl Pts',(-5.45492525077838,4.00450739897186,15.4954063644527));
#12869=CARTESIAN_POINT('Ctrl Pts',(-5.55740392905579,3.86491132032675,15.5035435408692));
#12870=CARTESIAN_POINT('Ctrl Pts',(-5.65443649180515,3.72149344011123,15.5116807172856));
#12871=CARTESIAN_POINT('Ctrl Pts',(-5.74574511586462,3.57473104771784,15.5198178937021));
#12872=CARTESIAN_POINT('Ctrl Pts',(-5.8383155797852,3.42594047191086,15.5280675218575));
#12873=CARTESIAN_POINT('Ctrl Pts',(-5.92500254830411,3.27371260902382,15.5363171500129));
#12874=CARTESIAN_POINT('Ctrl Pts',(-6.00556614100093,3.11856767219555,15.5445667781684));
#12875=CARTESIAN_POINT('Ctrl Pts',(-6.08612973369775,2.9634227353673,15.5528164063238));
#12876=CARTESIAN_POINT('Ctrl Pts',(-6.16056984386216,2.80536109965522,15.5610660344792));
#12877=CARTESIAN_POINT('Ctrl Pts',(-6.22869846988963,2.64492048485292,15.5693156626347));
#12878=CARTESIAN_POINT('Ctrl Pts',(-6.30473358197508,2.46586036224554,15.5785226793916));
#12879=CARTESIAN_POINT('Ctrl Pts',(-6.37310104231516,2.28338407206856,15.5877296961485));
#12880=CARTESIAN_POINT('Ctrl Pts',(-6.43351813430323,2.09812616770096,15.5969367129054));
#12881=CARTESIAN_POINT('Ctrl Pts',(-6.49368700921999,1.91362937534562,15.6061059036323));
#12882=CARTESIAN_POINT('Ctrl Pts',(-6.54597060928338,1.72637396026775,15.6152750943593));
#12883=CARTESIAN_POINT('Ctrl Pts',(-6.59013575359022,1.53701000297717,15.6244442850862));
#12884=CARTESIAN_POINT('Ctrl Pts',(-6.63418090021955,1.34816055176226,15.6335885629183));
#12885=CARTESIAN_POINT('Ctrl Pts',(-6.6701515417064,1.15721418325689,15.6427328407505));
#12886=CARTESIAN_POINT('Ctrl Pts',(-6.69786384472593,0.964836212791147,
15.6518771185827));
#12887=CARTESIAN_POINT('Ctrl Pts',(-6.72544643478091,0.773358705807173,
15.6609785947976));
#12888=CARTESIAN_POINT('Ctrl Pts',(-6.74484773035244,0.580463161232371,
15.6700800710125));
#12889=CARTESIAN_POINT('Ctrl Pts',(-6.75593493639542,0.386823131665841,
15.6791815472275));
#12890=CARTESIAN_POINT('Ctrl Pts',(-6.7632432804006,0.259181601080143,15.6851809594216));
#12891=CARTESIAN_POINT('Ctrl Pts',(-6.76694011348344,0.131216943220901,
15.6911803716158));
#12892=CARTESIAN_POINT('Ctrl Pts',(-6.76699927814238,0.00312563922654881,
15.69717978381));
#12893=CARTESIAN_POINT('',(-6.767,1.40905773919446E-12,15.3028202161899));
#12894=CARTESIAN_POINT('Ctrl Pts',(3.09917575053259,6.01559628526639,14.6513920151221));
#12895=CARTESIAN_POINT('Ctrl Pts',(2.93382384459265,6.1007839529376,14.6601414630345));
#12896=CARTESIAN_POINT('Ctrl Pts',(2.76495772122983,6.17915010267049,14.6688909109469));
#12897=CARTESIAN_POINT('Ctrl Pts',(2.5931509331671,6.25042856433178,14.6776403588593));
#12898=CARTESIAN_POINT('Ctrl Pts',(2.42134553245609,6.32170645041454,14.6863897361193));
#12899=CARTESIAN_POINT('Ctrl Pts',(2.24659977927575,6.38589665313463,14.6951391133793));
#12900=CARTESIAN_POINT('Ctrl Pts',(2.06950718689896,6.44278115439083,14.7038884906393));
#12901=CARTESIAN_POINT('Ctrl Pts',(1.89241596572829,6.49966521519734,14.712637800154));
#12902=CARTESIAN_POINT('Ctrl Pts',(1.71297821457156,6.54924360009557,14.7213871096687));
#12903=CARTESIAN_POINT('Ctrl Pts',(1.53180337335793,6.59134792173568,14.7301364191833));
#12904=CARTESIAN_POINT('Ctrl Pts',(1.35062987477741,6.63345193135313,14.7388856638594));
#12905=CARTESIAN_POINT('Ctrl Pts',(1.1677195910292,6.66808192368243,14.7476349085356));
#12906=CARTESIAN_POINT('Ctrl Pts',(0.983693746906624,6.69512028363172,14.7563841532117));
#12907=CARTESIAN_POINT('Ctrl Pts',(0.799669205419539,6.72215845218871,14.7651333359559));
#12908=CARTESIAN_POINT('Ctrl Pts',(0.614529402873032,6.74160505424583,14.7738825187));
#12909=CARTESIAN_POINT('Ctrl Pts',(0.428903127362691,6.75339404354126,14.7826317014442));
#12910=CARTESIAN_POINT('Ctrl Pts',(0.243278104163457,6.76518295330331,14.7913808251628));
#12911=CARTESIAN_POINT('Ctrl Pts',(0.0571669005388305,6.76931433552276,
14.8001299488814));
#12912=CARTESIAN_POINT('Ctrl Pts',(-0.128798404777664,6.76577415902473,
14.8088790726));
#12913=CARTESIAN_POINT('Ctrl Pts',(-0.314762517259084,6.76223400523441,
14.8176281401992));
#12914=CARTESIAN_POINT('Ctrl Pts',(-0.500580446819331,6.7510223966509,14.8263772077984));
#12915=CARTESIAN_POINT('Ctrl Pts',(-0.685621118842269,6.73217741012501,
14.8351262753976));
#12916=CARTESIAN_POINT('Ctrl Pts',(-0.870660665414322,6.71333253821774,
14.8438752897834));
#12917=CARTESIAN_POINT('Ctrl Pts',(-1.05492267885487,6.68685441030612,14.8526243041692));
#12918=CARTESIAN_POINT('Ctrl Pts',(-1.2377813763527,6.65283295028174,14.861373318555));
#12919=CARTESIAN_POINT('Ctrl Pts',(-1.42999922978867,6.61707018861861,14.8705701289224));
#12920=CARTESIAN_POINT('Ctrl Pts',(-1.62066601233717,6.57297172934408,14.8797669392898));
#12921=CARTESIAN_POINT('Ctrl Pts',(-1.80906628500409,6.52070304311288,14.8889637496572));
#12922=CARTESIAN_POINT('Ctrl Pts',(-1.98831342545549,6.47097374915024,14.8977137473949));
#12923=CARTESIAN_POINT('Ctrl Pts',(-2.16550875896722,6.41384933989522,14.9064637451327));
#12924=CARTESIAN_POINT('Ctrl Pts',(-2.34005036714029,6.34952386240469,14.9152137428705));
#12925=CARTESIAN_POINT('Ctrl Pts',(-2.51458843547104,6.2851996894859,14.9239635631513));
#12926=CARTESIAN_POINT('Ctrl Pts',(-2.68647261718067,6.21367483971094,14.9327133834322));
#12927=CARTESIAN_POINT('Ctrl Pts',(-2.8551190590874,6.13519226743839,14.941463203713));
#12928=CARTESIAN_POINT('Ctrl Pts',(-3.02376230488892,6.05671118252933,14.9502128581716));
#12929=CARTESIAN_POINT('Ctrl Pts',(-3.18916767379911,5.97127275992629,14.9589625126301));
#12930=CARTESIAN_POINT('Ctrl Pts',(-3.35077334102793,5.87916720437993,14.9677121670886));
#12931=CARTESIAN_POINT('Ctrl Pts',(-3.51237616037376,5.78706327195638,14.9764616673571));
#12932=CARTESIAN_POINT('Ctrl Pts',(-3.6701791630231,5.68829258362292,14.9852111676255));
#12933=CARTESIAN_POINT('Ctrl Pts',(-3.82364636566474,5.58319061741034,14.993960667894));
#12934=CARTESIAN_POINT('Ctrl Pts',(-3.9771110677882,5.47809036367686,15.0027100256024));
#12935=CARTESIAN_POINT('Ctrl Pts',(-4.12623987481959,5.36665920043201,15.0114593833109));
#12936=CARTESIAN_POINT('Ctrl Pts',(-4.27052628213971,5.24927559512301,15.0202087410193));
#12937=CARTESIAN_POINT('Ctrl Pts',(-4.41481053025021,5.13189374643,15.0289579677958));
#12938=CARTESIAN_POINT('Ctrl Pts',(-4.55425230136573,5.00855981477314,15.0377071945723));
#12939=CARTESIAN_POINT('Ctrl Pts',(-4.68837800630592,4.87969268192035,15.0464564213489));
#12940=CARTESIAN_POINT('Ctrl Pts',(-4.82250188228941,4.75082730631762,15.0552055288197));
#12941=CARTESIAN_POINT('Ctrl Pts',(-4.95130963053016,4.61642907903473,15.0639546362906));
#12942=CARTESIAN_POINT('Ctrl Pts',(-5.07436379033419,4.4769544473163,15.0727037437614));
#12943=CARTESIAN_POINT('Ctrl Pts',(-5.19741643562879,4.33748153220499,15.0814527435512));
#12944=CARTESIAN_POINT('Ctrl Pts',(-5.31471544462867,4.19293255254472,15.0902017433409));
#12945=CARTESIAN_POINT('Ctrl Pts',(-5.42586245275738,4.04379841779454,15.0989507431307));
#12946=CARTESIAN_POINT('Ctrl Pts',(-5.53702160019253,3.894647994842,15.1077006984728));
#12947=CARTESIAN_POINT('Ctrl Pts',(-5.64202723081341,3.74091164443714,15.116450653815));
#12948=CARTESIAN_POINT('Ctrl Pts',(-5.74052265233047,3.58311159163104,15.1252006091571));
#12949=CARTESIAN_POINT('Ctrl Pts',(-5.83901427066998,3.42531763191648,15.1339502266396));
#12950=CARTESIAN_POINT('Ctrl Pts',(-5.93099603115819,3.26346052695469,15.142699844122));
#12951=CARTESIAN_POINT('Ctrl Pts',(-6.01615550622831,3.09809004466925,15.1514494616045));
#12952=CARTESIAN_POINT('Ctrl Pts',(-6.10131214578871,2.93272506863679,15.1601987877556));
#12953=CARTESIAN_POINT('Ctrl Pts',(-6.17964682328813,2.76384720416748,15.1689481139067));
#12954=CARTESIAN_POINT('Ctrl Pts',(-6.25089348288623,2.5920300279145,15.1776974400578));
#12955=CARTESIAN_POINT('Ctrl Pts',(-6.3221381488939,2.42021765936873,15.1864465213893));
#12956=CARTESIAN_POINT('Ctrl Pts',(-6.38629508412645,2.24546640831749,15.1951956027209));
#12957=CARTESIAN_POINT('Ctrl Pts',(-6.4431463981987,2.0683697665986,15.2039446840525));
#12958=CARTESIAN_POINT('Ctrl Pts',(-6.50000285283755,1.89125711158087,15.2126945564869));
#12959=CARTESIAN_POINT('Ctrl Pts',(-6.549552276733,1.7117989144006,15.2214444289213));
#12960=CARTESIAN_POINT('Ctrl Pts',(-6.59162635926432,1.5306047627823,15.2301943013557));
#12961=CARTESIAN_POINT('Ctrl Pts',(-6.63369752055237,1.34942319164494,15.2389435662782));
#12962=CARTESIAN_POINT('Ctrl Pts',(-6.66829431424289,1.16650618642502,15.2476928312007));
#12963=CARTESIAN_POINT('Ctrl Pts',(-6.69529923745447,0.982474997616538,
15.2564420961232));
#12964=CARTESIAN_POINT('Ctrl Pts',(-6.72230554731468,0.798434359175698,
15.2651918103029));
#12965=CARTESIAN_POINT('Ctrl Pts',(-6.74171916496722,0.613279706238272,
15.2739415244826));
#12966=CARTESIAN_POINT('Ctrl Pts',(-6.75347414817288,0.427639953653293,
15.2826912386623));
#12967=CARTESIAN_POINT('Ctrl Pts',(-6.76248837758749,0.285283364197127,
15.2894008978382));
#12968=CARTESIAN_POINT('Ctrl Pts',(-6.76699999999997,0.142641701104314,
15.296110557014));
#12969=CARTESIAN_POINT('Ctrl Pts',(-6.767,1.40905773244098E-12,15.3028202161899));
#12970=CARTESIAN_POINT('Ctrl Pts',(-6.76699999999571,7.62476850229202E-6,
15.3029847694131));
#12971=CARTESIAN_POINT('Ctrl Pts',(-6.76700019411946,-0.172277660166757,
15.3111106415999));
#12972=CARTESIAN_POINT('Ctrl Pts',(-6.76041659476757,-0.344787798069247,
15.3192365137866));
#12973=CARTESIAN_POINT('Ctrl Pts',(-6.74722363853828,-0.516974053072598,
15.3273623859734));
#12974=CARTESIAN_POINT('Ctrl Pts',(-6.73404536197283,-0.688968718238338,
15.3354792165876));
#12975=CARTESIAN_POINT('Ctrl Pts',(-6.71427240758308,-0.860639854770346,
15.3435960472017));
#12976=CARTESIAN_POINT('Ctrl Pts',(-6.68793124167346,-1.03143817393389,
15.3517128778159));
#12977=CARTESIAN_POINT('Ctrl Pts',(-6.66160701719624,-1.20212664343523,
15.359824488056));
#12978=CARTESIAN_POINT('Ctrl Pts',(-6.62872304411251,-1.37194305151308,
15.3679360982962));
#12979=CARTESIAN_POINT('Ctrl Pts',(-6.58935768176897,-1.54034228070008,
15.3760477085364));
#12980=CARTESIAN_POINT('Ctrl Pts',(-6.5500114938191,-1.70865948465161,15.3841553677089));
#12981=CARTESIAN_POINT('Ctrl Pts',(-6.50419028646302,-1.87556052756818,
15.3922630268815));
#12982=CARTESIAN_POINT('Ctrl Pts',(-6.45202365964257,-2.04050966560134,
15.400370686054));
#12983=CARTESIAN_POINT('Ctrl Pts',(-6.42396699379531,-2.12922390935568,
15.4047312111267));
#12984=CARTESIAN_POINT('Ctrl Pts',(-6.39407573517589,-2.21737372715716,
15.4090917361994));
#12985=CARTESIAN_POINT('Ctrl Pts',(-6.36237607960498,-2.30487735501704,
15.4134522612721));
#12986=CARTESIAN_POINT('Ctrl Pts',(-6.2998876065227,-2.47737033627018,15.4220480188197));
#12987=CARTESIAN_POINT('Ctrl Pts',(-6.23041695127076,-2.64721938535274,
15.4306437763672));
#12988=CARTESIAN_POINT('Ctrl Pts',(-6.15422180419717,-2.81386619879911,
15.4392395339148));
#12989=CARTESIAN_POINT('Ctrl Pts',(-6.07795556446078,-2.98066849938828,
15.4478433115964));
#12990=CARTESIAN_POINT('Ctrl Pts',(-5.99495243636424,-3.14426232293631,
15.456447089278));
#12991=CARTESIAN_POINT('Ctrl Pts',(-5.90551624899013,-3.30411362288186,
15.4650508669597));
#12992=CARTESIAN_POINT('Ctrl Pts',(-5.81256514124534,-3.47024721869621,
15.4739927806277));
#12993=CARTESIAN_POINT('Ctrl Pts',(-5.71266529432935,-3.63233785090521,
15.4829346942957));
#12994=CARTESIAN_POINT('Ctrl Pts',(-5.60620673434045,-3.78981992340477,
15.4918766079637));
#12995=CARTESIAN_POINT('Ctrl Pts',(-5.50349499153471,-3.94175940228537,
15.5005038102944));
#12996=CARTESIAN_POINT('Ctrl Pts',(-5.3946785514444,-4.08940898011079,15.5091310126252));
#12997=CARTESIAN_POINT('Ctrl Pts',(-5.28014860639894,-4.23229484964639,
15.5177582149559));
#12998=CARTESIAN_POINT('Ctrl Pts',(-5.1655095891114,-4.37531679610183,15.5263936333763));
#12999=CARTESIAN_POINT('Ctrl Pts',(-5.04514640347598,-4.51356574672446,
15.5350290517967));
#13000=CARTESIAN_POINT('Ctrl Pts',(-4.91948832618044,-4.64660344860355,
15.5436644702171));
#13001=CARTESIAN_POINT('Ctrl Pts',(-4.79364460697371,-4.77983769473804,
15.5523126462383));
#13002=CARTESIAN_POINT('Ctrl Pts',(-4.66249057938801,-4.90784509112603,
15.5609608222594));
#13003=CARTESIAN_POINT('Ctrl Pts',(-4.52649100017713,-5.03022546466015,
15.5696089982805));
#13004=CARTESIAN_POINT('Ctrl Pts',(-4.51210276036556,-5.043172844151,15.5705239425123));
#13005=CARTESIAN_POINT('Ctrl Pts',(-4.49766031399888,-5.05605727968782,
15.5714388867441));
#13006=CARTESIAN_POINT('Ctrl Pts',(-4.48316423160408,-5.06887832488272,
15.5723538309759));
#13007=CARTESIAN_POINT('Ctrl Pts',(-4.35283424916889,-5.18414854407318,
15.5805798235173));
#13008=CARTESIAN_POINT('Ctrl Pts',(-4.21788464793136,-5.29454029992256,
15.5888058160586));
#13009=CARTESIAN_POINT('Ctrl Pts',(-4.0787157418761,-5.3996635910927,15.5970318086));
#13010=CARTESIAN_POINT('Ctrl Pts',(-3.93969273643064,-5.5046766740797,15.6052491772514));
#13011=CARTESIAN_POINT('Ctrl Pts',(-3.7964595183313,-5.60443207715044,15.6134665459028));
#13012=CARTESIAN_POINT('Ctrl Pts',(-3.64945163446743,-5.69857804787151,
15.6216839145542));
#13013=CARTESIAN_POINT('Ctrl Pts',(-3.5025684537276,-5.79264415691198,15.6298943126166));
#13014=CARTESIAN_POINT('Ctrl Pts',(-3.35191728437171,-5.88111011833935,
15.638104710679));
#13015=CARTESIAN_POINT('Ctrl Pts',(-3.19796507179745,-5.96366568475829,
15.6463151087414));
#13016=CARTESIAN_POINT('Ctrl Pts',(-3.0441126565521,-6.04616773570722,15.6545201845302));
#13017=CARTESIAN_POINT('Ctrl Pts',(-2.88696377514848,-6.12276685466356,
15.6627252603189));
#13018=CARTESIAN_POINT('Ctrl Pts',(-2.72701263461551,-6.19319716226178,
15.6709303361077));
#13019=CARTESIAN_POINT('Ctrl Pts',(-2.56713319011603,-6.26359590038401,
15.6791317340772));
#13020=CARTESIAN_POINT('Ctrl Pts',(-2.40445431618188,-6.32783119193416,
15.6873331320468));
#13021=CARTESIAN_POINT('Ctrl Pts',(-2.23949308261818,-6.3856839675093,15.6955345300163));
#13022=CARTESIAN_POINT('Ctrl Pts',(-2.07454477019234,-6.44353221157317,
15.703735285584));
#13023=CARTESIAN_POINT('Ctrl Pts',(-1.90731478917572,-6.49499880875938,
15.7119360411517));
#13024=CARTESIAN_POINT('Ctrl Pts',(-1.73833872868661,-6.53991341413235,
15.7201367967194));
#13025=CARTESIAN_POINT('Ctrl Pts',(-1.56936352651522,-6.58482779136056,
15.7283375106312));
#13026=CARTESIAN_POINT('Ctrl Pts',(-1.39864260861118,-6.6231901499759,15.736538224543));
#13027=CARTESIAN_POINT('Ctrl Pts',(-1.22672509711896,-6.65488050502024,
15.7447389384548));
#13028=CARTESIAN_POINT('Ctrl Pts',(-1.05477730315248,-6.68657644217401,
15.7529410968843));
#13029=CARTESIAN_POINT('Ctrl Pts',(-0.881632848106059,-6.7115979693203,
15.761143255314));
#13030=CARTESIAN_POINT('Ctrl Pts',(-0.70784943497986,-6.72987653507839,
15.7693454137436));
#13031=CARTESIAN_POINT('Ctrl Pts',(-0.534003916493984,-6.74816163308763,
15.7775505033965));
#13032=CARTESIAN_POINT('Ctrl Pts',(-0.359519341230758,-6.75969893188969,
15.7857555930495));
#13033=CARTESIAN_POINT('Ctrl Pts',(-0.184956958686212,-6.76447188799196,
15.7939606827024));
#13034=CARTESIAN_POINT('Ctrl Pts',(-0.010195159258519,-6.76925029663227,
15.8021751457002));
#13035=CARTESIAN_POINT('Ctrl Pts',(0.164644266426632,-6.76724891465809,
15.810389608698));
#13036=CARTESIAN_POINT('Ctrl Pts',(0.339000575769034,-6.75850335574588,
15.8186040716958));
#13037=CARTESIAN_POINT('Ctrl Pts',(0.513460185714212,-6.74975261536641,
15.8268234015032));
#13038=CARTESIAN_POINT('Ctrl Pts',(0.687435752389432,-6.73424976481487,
15.8350427313107));
#13039=CARTESIAN_POINT('Ctrl Pts',(0.860373328558443,-6.71208214606357,
15.8432620611182));
#13040=CARTESIAN_POINT('Ctrl Pts',(1.03357886101643,-6.68988017993104,15.8514941262789));
#13041=CARTESIAN_POINT('Ctrl Pts',(1.20574283576622,-6.6609928681763,15.8597261914396));
#13042=CARTESIAN_POINT('Ctrl Pts',(1.37632182357283,-6.62555863591571,15.8679582566003));
#13043=CARTESIAN_POINT('Ctrl Pts',(1.52965046605641,-6.59370780364248,15.8753578278614));
#13044=CARTESIAN_POINT('Ctrl Pts',(1.681698490314,-6.55656798282131,15.8827573991225));
#13045=CARTESIAN_POINT('Ctrl Pts',(1.83208365428045,-6.51427344250442,15.8901569703836));
#13046=CARTESIAN_POINT('Ctrl Pts',(1.99783108834764,-6.46765839519737,15.8983124287904));
#13047=CARTESIAN_POINT('Ctrl Pts',(2.16206861792596,-6.41463733580045,15.9064678871972));
#13048=CARTESIAN_POINT('Ctrl Pts',(2.32425831719805,-6.35532157132396,15.914623345604));
#13049=CARTESIAN_POINT('Ctrl Pts',(2.48625061028653,-6.29607800192981,15.9227688777459));
#13050=CARTESIAN_POINT('Ctrl Pts',(2.64619969496623,-6.23055510214892,15.9309144098877));
#13051=CARTESIAN_POINT('Ctrl Pts',(2.80357940658717,-6.15891479978091,15.9390599420296));
#13052=CARTESIAN_POINT('Ctrl Pts',(2.9608006602082,-6.08734662855935,15.9471972728302));
#13053=CARTESIAN_POINT('Ctrl Pts',(3.11545736081302,-6.00967346715305,15.9553346036308));
#13054=CARTESIAN_POINT('Ctrl Pts',(3.26704005016765,-5.92610650516852,15.9634719344313));
#13055=CARTESIAN_POINT('Ctrl Pts',(3.41850197383363,-5.84260612085031,15.9716027822333));
#13056=CARTESIAN_POINT('Ctrl Pts',(3.56689444403819,-5.75322146108041,15.9797336300353));
#13057=CARTESIAN_POINT('Ctrl Pts',(3.71172949390902,-5.65821112756019,15.9878644778373));
#13058=CARTESIAN_POINT('Ctrl Pts',(3.85647957903511,-5.5632565300565,15.9959905558312));
#13059=CARTESIAN_POINT('Ctrl Pts',(3.99767609498685,-5.462683031053,16.0041166338249));
#13060=CARTESIAN_POINT('Ctrl Pts',(4.13485714190466,-5.35679432273072,16.0122427118188));
#13061=CARTESIAN_POINT('Ctrl Pts',(4.2725246077595,-5.2505301523887,16.0203976034009));
#13062=CARTESIAN_POINT('Ctrl Pts',(4.40614775341956,-5.13891319492401,16.0285524949831));
#13063=CARTESIAN_POINT('Ctrl Pts',(4.53529003060481,-5.02229363322144,16.0367073865653));
#13064=CARTESIAN_POINT('Ctrl Pts',(4.66392869806236,-4.90612884703464,16.0448304769216));
#13065=CARTESIAN_POINT('Ctrl Pts',(4.78812112006629,-4.78500066295599,16.0529535672779));
#13066=CARTESIAN_POINT('Ctrl Pts',(4.90747012568906,-4.65929457809543,16.0610766576342));
#13067=CARTESIAN_POINT('Ctrl Pts',(5.02682850314064,-4.53357862221917,16.0692003858527));
#13068=CARTESIAN_POINT('Ctrl Pts',(5.14134245472424,-4.4032843147964,16.0773241140711));
#13069=CARTESIAN_POINT('Ctrl Pts',(5.2506528988365,-4.268832760362,16.0854478422895));
#13070=CARTESIAN_POINT('Ctrl Pts',(5.35999272268617,-4.13434506892903,16.0935737539498));
#13071=CARTESIAN_POINT('Ctrl Pts',(5.46412602358371,-3.99569818934985,16.1016996656102));
#13072=CARTESIAN_POINT('Ctrl Pts',(5.56273513898187,-3.85334488120858,16.1098255772705));
#13073=CARTESIAN_POINT('Ctrl Pts',(5.66197486992334,-3.71008120886424,16.1180034549806));
#13074=CARTESIAN_POINT('Ctrl Pts',(5.75561930076206,-3.56306384617776,16.1261813326906));
#13075=CARTESIAN_POINT('Ctrl Pts',(5.84339034310917,-3.41278160714372,16.1343592104007));
#13076=CARTESIAN_POINT('Ctrl Pts',(5.93074247330753,-3.26321663264238,16.1424980568741));
#13077=CARTESIAN_POINT('Ctrl Pts',(6.01227703902131,-3.11041823033074,16.1506369033476));
#13078=CARTESIAN_POINT('Ctrl Pts',(6.08776746412453,-2.95489023531277,16.158775749821));
#13079=CARTESIAN_POINT('Ctrl Pts',(6.16380093018369,-2.79824344846164,16.1669731431494));
#13080=CARTESIAN_POINT('Ctrl Pts',(6.23370281893999,-2.63882799611478,16.1751705364778));
#13081=CARTESIAN_POINT('Ctrl Pts',(6.29729218555359,-2.47717583747414,16.1833679298062));
#13082=CARTESIAN_POINT('Ctrl Pts',(6.3608815521672,-2.31552367883348,16.1915653231345));
#13083=CARTESIAN_POINT('Ctrl Pts',(6.41815833152117,-2.15163518545198,16.1997627164629));
#13084=CARTESIAN_POINT('Ctrl Pts',(6.46899361040797,-1.98605404470796,16.2079601097913));
#13085=CARTESIAN_POINT('Ctrl Pts',(6.52000758876355,-1.81989084240084,16.2161863191283));
#13086=CARTESIAN_POINT('Ctrl Pts',(6.5646866391576,-1.6515285750688,16.2244125284653));
#13087=CARTESIAN_POINT('Ctrl Pts',(6.60283827210986,-1.48149105713174,16.2326387378022));
#13088=CARTESIAN_POINT('Ctrl Pts',(6.64094704333687,-1.31164456906182,16.2408557053454));
#13089=CARTESIAN_POINT('Ctrl Pts',(6.67254292186017,-1.14012692486209,16.2490726728886));
#13090=CARTESIAN_POINT('Ctrl Pts',(6.69748267882117,-0.967478561462939,
16.2572896404318));
#13091=CARTESIAN_POINT('Ctrl Pts',(6.7223994226426,-0.794989509194642,16.2654990257752));
#13092=CARTESIAN_POINT('Ctrl Pts',(6.74067222583302,-0.621372168358847,
16.2737084111186));
#13093=CARTESIAN_POINT('Ctrl Pts',(6.75220853874428,-0.447178766612269,
16.2819177964619));
#13094=CARTESIAN_POINT('Ctrl Pts',(6.76373652121989,-0.27311115088884,16.2901212537625));
#13095=CARTESIAN_POINT('Ctrl Pts',(6.76853767897606,-0.0984686592113893,
16.2983247110631));
#13096=CARTESIAN_POINT('Ctrl Pts',(6.76657107691549,0.0761896387359722,
16.3065281683637));
#13097=CARTESIAN_POINT('Ctrl Pts',(6.76460550045366,0.250756850980788,16.3147273474956));
#13098=CARTESIAN_POINT('Ctrl Pts',(6.7558791994782,0.42533949531331,16.3229265266274));
#13099=CARTESIAN_POINT('Ctrl Pts',(6.7404032964622,0.599376677091736,16.3311257057593));
#13100=CARTESIAN_POINT('Ctrl Pts',(6.72493030943986,0.773381066514288,16.3393233399891));
#13101=CARTESIAN_POINT('Ctrl Pts',(6.70271027915053,0.946839840694611,16.3475209742189));
#13102=CARTESIAN_POINT('Ctrl Pts',(6.67380636065729,1.11919509490095,16.3557186084487));
#13103=CARTESIAN_POINT('Ctrl Pts',(6.64490452848054,1.29153790831627,16.3639156509642));
#13104=CARTESIAN_POINT('Ctrl Pts',(6.60931982737665,1.46277700650654,16.3721126934798));
#13105=CARTESIAN_POINT('Ctrl Pts',(6.56716691202784,1.63236262808443,16.3803097359954));
#13106=CARTESIAN_POINT('Ctrl Pts',(6.52500937810087,1.80196683068908,16.3885076766382));
#13107=CARTESIAN_POINT('Ctrl Pts',(6.47628228269598,1.96991684758406,16.396705617281));
#13108=CARTESIAN_POINT('Ctrl Pts',(6.42115074664811,2.13567602618478,16.4049035579238));
#13109=CARTESIAN_POINT('Ctrl Pts',(6.36600314988914,2.30148349312409,16.4131038867598));
#13110=CARTESIAN_POINT('Ctrl Pts',(6.30444750937547,2.46509851023569,16.4213042155958));
#13111=CARTESIAN_POINT('Ctrl Pts',(6.23669788805495,2.62600237112059,16.4295045444317));
#13112=CARTESIAN_POINT('Ctrl Pts',(6.16887766987088,2.78707389800407,16.4377134182231));
#13113=CARTESIAN_POINT('Ctrl Pts',(6.0948507155596,2.9454282935398,16.4459222920146));
#13114=CARTESIAN_POINT('Ctrl Pts',(6.01487848943923,3.10056861837975,16.454131165806));
#13115=CARTESIAN_POINT('Ctrl Pts',(5.93486334310725,3.25579220532072,16.4623444452094));
#13116=CARTESIAN_POINT('Ctrl Pts',(5.84889674046926,3.40779797089882,16.4705577246128));
#13117=CARTESIAN_POINT('Ctrl Pts',(5.75728462341509,3.55611624739521,16.4787710040162));
#13118=CARTESIAN_POINT('Ctrl Pts',(5.66553850924091,3.70465146268238,16.4869962966317));
#13119=CARTESIAN_POINT('Ctrl Pts',(5.56813057882467,3.84948811265275,16.4952215892471));
#13120=CARTESIAN_POINT('Ctrl Pts',(5.46540911599033,3.99018698745433,16.5034468818626));
#13121=CARTESIAN_POINT('Ctrl Pts',(5.37250989221313,4.11743221834117,16.5108856709747));
#13122=CARTESIAN_POINT('Ctrl Pts',(5.27526536421087,4.24129342813061,16.5183244600868));
#13123=CARTESIAN_POINT('Ctrl Pts',(5.17395949578523,4.36147132696913,16.525763249199));
#13124=CARTESIAN_POINT('Ctrl Pts',(5.06191368188543,4.49438989030008,16.5339906618203));
#13125=CARTESIAN_POINT('Ctrl Pts',(4.94458594637151,4.62317381704289,16.5422180744416));
#13126=CARTESIAN_POINT('Ctrl Pts',(4.82231245014207,4.74737734261822,16.5504454870629));
#13127=CARTESIAN_POINT('Ctrl Pts',(4.69715469852805,4.87451065018614,16.5588669724791));
#13128=CARTESIAN_POINT('Ctrl Pts',(4.56681515025296,4.99684446344319,16.5672884578953));
#13129=CARTESIAN_POINT('Ctrl Pts',(4.43169984610697,5.11393444170098,16.5757099433115));
#13130=CARTESIAN_POINT('Ctrl Pts',(4.29999521699383,5.22806875281235,16.5839188477013));
#13131=CARTESIAN_POINT('Ctrl Pts',(4.16375330290666,5.33722049437015,16.592127752091));
#13132=CARTESIAN_POINT('Ctrl Pts',(4.02338898069103,5.44101370243212,16.6003366564807));
#13133=CARTESIAN_POINT('Ctrl Pts',(3.87757226368288,5.54883871528751,16.6088644324102));
#13134=CARTESIAN_POINT('Ctrl Pts',(3.72730670528221,5.65088024959378,16.6173922083396));
#13135=CARTESIAN_POINT('Ctrl Pts',(3.57309691048976,5.74676147654038,16.6259199842691));
#13136=CARTESIAN_POINT('Ctrl Pts',(3.41888711569731,5.84264270348698,16.6344477601985));
#13137=CARTESIAN_POINT('Ctrl Pts',(3.26073343455383,5.9323633632272,16.6429755361279));
#13138=CARTESIAN_POINT('Ctrl Pts',(3.09917575053259,6.01559628526639,16.6515033120574));
#13139=CARTESIAN_POINT('Origin',(0.,0.,-3.69717978381041));
#13140=CARTESIAN_POINT('',(3.09917575053257,6.0155962852664,19.0456175016683));
#13141=CARTESIAN_POINT('',(3.0991757505326,6.01559628526638,18.6513920151221));
#13142=CARTESIAN_POINT('',(3.09917575053259,6.01559628526639,-3.69717978381041));
#13143=CARTESIAN_POINT('',(-6.76699920193514,-0.00194542300215272,17.69717978381));
#13144=CARTESIAN_POINT('Ctrl Pts',(-6.76699772241609,-0.0055520100402695,
17.69717978381));
#13145=CARTESIAN_POINT('Ctrl Pts',(-6.76682955409667,-0.210521854514989,
17.7067908133179));
#13146=CARTESIAN_POINT('Ctrl Pts',(-6.75734493412658,-0.415082670399996,
17.7164018428258));
#13147=CARTESIAN_POINT('Ctrl Pts',(-6.73867812456815,-0.618470802436715,
17.7260128723337));
#13148=CARTESIAN_POINT('Ctrl Pts',(-6.71988957760058,-0.823185349904371,
17.7356865811028));
#13149=CARTESIAN_POINT('Ctrl Pts',(-6.69179878842976,-1.02671180498338,
17.7453602898719));
#13150=CARTESIAN_POINT('Ctrl Pts',(-6.65459139278692,-1.22829247129757,
17.7550339986409));
#13151=CARTESIAN_POINT('Ctrl Pts',(-6.61709441421887,-1.43144202782853,
17.7647829973042));
#13152=CARTESIAN_POINT('Ctrl Pts',(-6.5703384359958,-1.63261532843543,17.7745319959675));
#13153=CARTESIAN_POINT('Ctrl Pts',(-6.5145615175188,-1.83105904723556,17.7842809946309));
#13154=CARTESIAN_POINT('Ctrl Pts',(-6.49042741594287,-1.91692361267588,
17.7884992865414));
#13155=CARTESIAN_POINT('Ctrl Pts',(-6.46460501037005,-2.00227743012385,
17.7927175784519));
#13156=CARTESIAN_POINT('Ctrl Pts',(-6.43711629998103,-2.08706078984742,
17.7969358703624));
#13157=CARTESIAN_POINT('Ctrl Pts',(-6.38351853804928,-2.2523722310147,17.80516073804));
#13158=CARTESIAN_POINT('Ctrl Pts',(-6.32347339824635,-2.41584976197224,
17.8133856057175));
#13159=CARTESIAN_POINT('Ctrl Pts',(-6.25712366996655,-2.57695408937458,
17.8216104733951));
#13160=CARTESIAN_POINT('Ctrl Pts',(-6.19084869208219,-2.73787691471967,
17.8298260748387));
#13161=CARTESIAN_POINT('Ctrl Pts',(-6.11828340463295,-2.89643153177296,
17.8380416762822));
#13162=CARTESIAN_POINT('Ctrl Pts',(-6.03962048177441,-3.05209328758659,
17.8462572777258));
#13163=CARTESIAN_POINT('Ctrl Pts',(-5.96103037654355,-3.20761094857933,
17.8544652740539));
#13164=CARTESIAN_POINT('Ctrl Pts',(-5.87635403789743,-3.36024076323195,
17.8626732703821));
#13165=CARTESIAN_POINT('Ctrl Pts',(-5.78583241465863,-3.50947749237483,
17.8708812667102));
#13166=CARTESIAN_POINT('Ctrl Pts',(-5.69537640481127,-3.65860604926475,
17.8790833135816));
#13167=CARTESIAN_POINT('Ctrl Pts',(-5.59908373473887,-3.80434611386227,
17.8872853604531));
#13168=CARTESIAN_POINT('Ctrl Pts',(-5.49724155456428,-3.9462164526001,17.8954874073246));
#13169=CARTESIAN_POINT('Ctrl Pts',(-5.39545274251451,-4.0880124473487,17.9036851560961));
#13170=CARTESIAN_POINT('Ctrl Pts',(-5.28812042248059,-4.22594246526505,
17.9118829048677));
#13171=CARTESIAN_POINT('Ctrl Pts',(-5.17557542968355,-4.35955364362637,
17.9200806536393));
#13172=CARTESIAN_POINT('Ctrl Pts',(-5.06305190258383,-4.49313933833851,
17.928276838855));
#13173=CARTESIAN_POINT('Ctrl Pts',(-4.94531790921027,-4.62240755613955,
17.9364730240706));
#13174=CARTESIAN_POINT('Ctrl Pts',(-4.82274518599496,-4.74693773615817,
17.9446692092862));
#13175=CARTESIAN_POINT('Ctrl Pts',(-4.70018153043303,-4.87145870371516,
17.9528647881666));
#13176=CARTESIAN_POINT('Ctrl Pts',(-4.57278010898451,-4.99124207518212,
17.9610603670469));
#13177=CARTESIAN_POINT('Ctrl Pts',(-4.44095016519683,-5.1059035077289,17.9692559459273));
#13178=CARTESIAN_POINT('Ctrl Pts',(-4.30910598899387,-5.22057731917138,
17.9774524096057));
#13179=CARTESIAN_POINT('Ctrl Pts',(-4.17283260872368,-5.33012785447943,
17.9856488732841));
#13180=CARTESIAN_POINT('Ctrl Pts',(-4.03257307824404,-5.43421046414485,
17.9938453369626));
#13181=CARTESIAN_POINT('Ctrl Pts',(-3.8922728866202,-5.5383232472893,18.0020441767904));
#13182=CARTESIAN_POINT('Ctrl Pts',(-3.74798453110036,-5.63696473360017,
18.0102430166181));
#13183=CARTESIAN_POINT('Ctrl Pts',(-3.6001808504722,-5.72983305549937,18.0184418564459));
#13184=CARTESIAN_POINT('Ctrl Pts',(-3.45222278469464,-5.82279838100288,
18.0266492601952));
#13185=CARTESIAN_POINT('Ctrl Pts',(-3.30074236215719,-5.90997830331226,
18.0348566639444));
#13186=CARTESIAN_POINT('Ctrl Pts',(-3.14623875598282,-5.99111598037892,
18.0430640676936));
#13187=CARTESIAN_POINT('Ctrl Pts',(-2.99165238950068,-6.07229711907921,
18.0512758677627));
#13188=CARTESIAN_POINT('Ctrl Pts',(-2.83403993471587,-6.14742940613931,
18.0594876678317));
#13189=CARTESIAN_POINT('Ctrl Pts',(-2.67392133894803,-6.21630385945848,
18.0676994679007));
#13190=CARTESIAN_POINT('Ctrl Pts',(-2.51356702623398,-6.2852797055967,18.0759233568869));
#13191=CARTESIAN_POINT('Ctrl Pts',(-2.35069953427168,-6.34797917833961,
18.084147245873));
#13192=CARTESIAN_POINT('Ctrl Pts',(-2.18585602150401,-6.40424253548027,
18.0923711348592));
#13193=CARTESIAN_POINT('Ctrl Pts',(-2.03354346549322,-6.4562289048069,18.0999698661092));
#13194=CARTESIAN_POINT('Ctrl Pts',(-1.87954426568277,-6.5027209735621,18.1075685973592));
#13195=CARTESIAN_POINT('Ctrl Pts',(-1.7242895488774,-6.54363160268304,18.1151673286092));
#13196=CARTESIAN_POINT('Ctrl Pts',(-1.55624221900217,-6.58791316867184,
18.1233921769312));
#13197=CARTESIAN_POINT('Ctrl Pts',(-1.38625214432185,-6.62577927521689,
18.1316170252533));
#13198=CARTESIAN_POINT('Ctrl Pts',(-1.21485021538482,-6.65705850614064,
18.1398418735753));
#13199=CARTESIAN_POINT('Ctrl Pts',(-1.04364132302305,-6.68830250971514,
18.1480574588945));
#13200=CARTESIAN_POINT('Ctrl Pts',(-0.87102409234731,-6.71297434553958,
18.1562730442137));
#13201=CARTESIAN_POINT('Ctrl Pts',(-0.697544064591326,-6.73095247925236,
18.1644886295329));
#13202=CARTESIAN_POINT('Ctrl Pts',(-0.524224558219132,-6.74891397776545,
18.1726966129562));
#13203=CARTESIAN_POINT('Ctrl Pts',(-0.350044199304795,-6.76019407228817,
18.1809045963794));
#13204=CARTESIAN_POINT('Ctrl Pts',(-0.175558293589939,-6.76472233617551,
18.1891125798026));
#13205=CARTESIAN_POINT('Ctrl Pts',(-0.00119879361789976,-6.76924731957691,
18.1973146169792));
#13206=CARTESIAN_POINT('Ctrl Pts',(0.173465455065159,-6.76703020570275,
18.2055166541557));
#13207=CARTESIAN_POINT('Ctrl Pts',(0.347874366087304,-6.75805241363363,
18.2137186913322));
#13208=CARTESIAN_POINT('Ctrl Pts',(0.522191950001651,-6.74907932267628,
18.2219164336116));
#13209=CARTESIAN_POINT('Ctrl Pts',(0.69625410516685,-6.7333526244639,18.230114175891));
#13210=CARTESIAN_POINT('Ctrl Pts',(0.869500997231249,-6.71090582677286,
18.2383119181704));
#13211=CARTESIAN_POINT('Ctrl Pts',(1.04271494926622,-6.68846329696892,18.2465081017848));
#13212=CARTESIAN_POINT('Ctrl Pts',(1.21511359071987,-6.65930325260606,18.2547042853991));
#13213=CARTESIAN_POINT('Ctrl Pts',(1.38614215096062,-6.6235110732398,18.2629004690135));
#13214=CARTESIAN_POINT('Ctrl Pts',(1.55715812111292,-6.58772152867736,18.2710960492744));
#13215=CARTESIAN_POINT('Ctrl Pts',(1.72680385951244,-6.54530089403478,18.2792916295352));
#13216=CARTESIAN_POINT('Ctrl Pts',(1.8945347890943,-6.49638568227837,18.2874872097961));
#13217=CARTESIAN_POINT('Ctrl Pts',(2.06228388799807,-6.44746517181986,18.2956836778368));
#13218=CARTESIAN_POINT('Ctrl Pts',(2.22811742028913,-6.39204878310216,18.3038801458776));
#13219=CARTESIAN_POINT('Ctrl Pts',(2.39150592463515,-6.33032293113353,18.3120766139183));
#13220=CARTESIAN_POINT('Ctrl Pts',(2.55494185464408,-6.2685791624243,18.3202754610917));
#13221=CARTESIAN_POINT('Ctrl Pts',(2.71593100748238,-6.20052240932084,18.3284743082651));
#13222=CARTESIAN_POINT('Ctrl Pts',(2.8739638120376,-6.12638727204691,18.3366731554384));
#13223=CARTESIAN_POINT('Ctrl Pts',(3.03216177624101,-6.05217465634547,18.3448805712044));
#13224=CARTESIAN_POINT('Ctrl Pts',(3.18739689410575,-5.97187111760412,18.3530879869704));
#13225=CARTESIAN_POINT('Ctrl Pts',(3.33918323730906,-5.88575775135829,18.3612954027363));
#13226=CARTESIAN_POINT('Ctrl Pts',(3.49105093265376,-5.7995982313769,18.3695072173885));
#13227=CARTESIAN_POINT('Ctrl Pts',(3.63946586374253,-5.70762286516864,18.3777190320406));
#13228=CARTESIAN_POINT('Ctrl Pts',(3.78397113575172,-5.61015609798853,18.3859308466928));
#13229=CARTESIAN_POINT('Ctrl Pts',(3.9286892137422,-5.51254579617646,18.3941547544904));
#13230=CARTESIAN_POINT('Ctrl Pts',(4.06948583682063,-5.40942814392912,18.402378662288));
#13231=CARTESIAN_POINT('Ctrl Pts',(4.20593623048949,-5.30116868483318,18.4106025700856));
#13232=CARTESIAN_POINT('Ctrl Pts',(4.33201387423434,-5.2011389439954,18.4182013090091));
#13233=CARTESIAN_POINT('Ctrl Pts',(4.45438117505745,-5.09672000800723,18.4258000479326));
#13234=CARTESIAN_POINT('Ctrl Pts',(4.57273176015609,-4.98822746570962,18.4333987868561));
#13235=CARTESIAN_POINT('Ctrl Pts',(4.69968355033694,-4.87185015794663,18.4415497690304));
#13236=CARTESIAN_POINT('Ctrl Pts',(4.82238911410713,-4.75044043053605,18.4497007512046));
#13237=CARTESIAN_POINT('Ctrl Pts',(4.94041991225922,-4.62434212516252,18.4578517333789));
#13238=CARTESIAN_POINT('Ctrl Pts',(5.05831360669997,-4.49839029465767,18.4659932474319));
#13239=CARTESIAN_POINT('Ctrl Pts',(5.17154309735107,-4.36776099155392,18.474134761485));
#13240=CARTESIAN_POINT('Ctrl Pts',(5.27971338460312,-4.23283776873656,18.482276275538));
#13241=CARTESIAN_POINT('Ctrl Pts',(5.38778078503692,-4.09804287895275,18.4904100457411));
#13242=CARTESIAN_POINT('Ctrl Pts',(5.49079833506234,-3.95896248383105,18.4985438159441));
#13243=CARTESIAN_POINT('Ctrl Pts',(5.58840835794962,-3.81601638162087,18.5066775861472));
#13244=CARTESIAN_POINT('Ctrl Pts',(5.68594606787453,-3.67317617894645,18.5148053305652));
#13245=CARTESIAN_POINT('Ctrl Pts',(5.77808402204886,-3.52647627229731,18.5229330749832));
#13246=CARTESIAN_POINT('Ctrl Pts',(5.86450528316306,-3.37636887554553,18.5310608194012));
#13247=CARTESIAN_POINT('Ctrl Pts',(5.95088068976486,-3.22634112472113,18.5391842512952));
#13248=CARTESIAN_POINT('Ctrl Pts',(6.03154526199955,-3.07290980067348,18.5473076831893));
#13249=CARTESIAN_POINT('Ctrl Pts',(6.10622581672461,-2.91655537838147,18.5554311150833));
#13250=CARTESIAN_POINT('Ctrl Pts',(6.18138011551486,-2.75920910513308,18.5636060788341));
#13251=CARTESIAN_POINT('Ctrl Pts',(6.25047400739617,-2.59890283282634,18.571781042585));
#13252=CARTESIAN_POINT('Ctrl Pts',(6.31327624034627,-2.4361510858482,18.5799560063358));
#13253=CARTESIAN_POINT('Ctrl Pts',(6.37566843567783,-2.27446194979337,18.5880775955088));
#13254=CARTESIAN_POINT('Ctrl Pts',(6.43185077589508,-2.11035953200006,18.5961991846818));
#13255=CARTESIAN_POINT('Ctrl Pts',(6.48164509876486,-1.94436771564883,18.6043207738548));
#13256=CARTESIAN_POINT('Ctrl Pts',(6.53144599550652,-1.77835398497344,18.6124434352442));
#13257=CARTESIAN_POINT('Ctrl Pts',(6.57485708992834,-1.61045070948888,18.6205660966336));
#13258=CARTESIAN_POINT('Ctrl Pts',(6.61175036118388,-1.44119608706966,18.6286887580229));
#13259=CARTESIAN_POINT('Ctrl Pts',(6.648655528678,-1.27188688848241,18.6368140385652));
#13260=CARTESIAN_POINT('Ctrl Pts',(6.67903861002489,-1.10122583266907,18.6449393191074));
#13261=CARTESIAN_POINT('Ctrl Pts',(6.70282288382531,-0.929760392825894,
18.6530645996497));
#13262=CARTESIAN_POINT('Ctrl Pts',(6.72686628235356,-0.756426872594672,
18.6612784034374));
#13263=CARTESIAN_POINT('Ctrl Pts',(6.74416619288582,-0.582271718917682,
18.6694922072252));
#13264=CARTESIAN_POINT('Ctrl Pts',(6.75469733137347,-0.407863900751406,
18.677706011013));
#13265=CARTESIAN_POINT('Ctrl Pts',(6.76513299893489,-0.235037191404557,
18.6858453518681));
#13266=CARTESIAN_POINT('Ctrl Pts',(6.76892217191133,-0.0619627460209338,
18.6939846927233));
#13267=CARTESIAN_POINT('Ctrl Pts',(6.76609271128249,0.110808042713229,18.7021240335784));
#13268=CARTESIAN_POINT('Ctrl Pts',(6.76322442258271,0.285949727290164,18.7103750688325));
#13269=CARTESIAN_POINT('Ctrl Pts',(6.75355455256377,0.460778968813002,18.7186261040866));
#13270=CARTESIAN_POINT('Ctrl Pts',(6.73716613396148,0.634729456857475,18.7268771393406));
#13271=CARTESIAN_POINT('Ctrl Pts',(6.72077771535918,0.808679944901949,18.7351281745947));
#13272=CARTESIAN_POINT('Ctrl Pts',(6.69767086544942,0.981751307841,18.7433792098488));
#13273=CARTESIAN_POINT('Ctrl Pts',(6.66798156185886,1.15339103980841,18.7516302451028));
#13274=CARTESIAN_POINT('Ctrl Pts',(6.63835991892323,1.32463961215692,18.7598624765999));
#13275=CARTESIAN_POINT('Ctrl Pts',(6.60209348720382,1.49499773932892,18.768094708097));
#13276=CARTESIAN_POINT('Ctrl Pts',(6.55924460544374,1.66391081670778,18.7763269395941));
#13277=CARTESIAN_POINT('Ctrl Pts',(6.5164473513962,1.83262037428767,18.7845492522494));
#13278=CARTESIAN_POINT('Ctrl Pts',(6.46708352766374,1.99988800516014,18.7927715649046));
#13279=CARTESIAN_POINT('Ctrl Pts',(6.41126696586366,2.16516625052799,18.8009938775599));
#13280=CARTESIAN_POINT('Ctrl Pts',(6.35550647238797,2.33027847215706,18.8092079308155));
#13281=CARTESIAN_POINT('Ctrl Pts',(6.29330626382452,2.49340495096386,18.8174219840711));
#13282=CARTESIAN_POINT('Ctrl Pts',(6.2248307750094,2.65401032825721,18.8256360373266));
#13283=CARTESIAN_POINT('Ctrl Pts',(6.15641035538368,2.81448654388855,18.8338434846965));
#13284=CARTESIAN_POINT('Ctrl Pts',(6.08172484786925,2.97244536841968,18.8420509320663));
#13285=CARTESIAN_POINT('Ctrl Pts',(6.00098791682371,3.12736838606133,18.8502583794361));
#13286=CARTESIAN_POINT('Ctrl Pts',(5.92030108248002,3.28219527505251,18.8584607341422));
#13287=CARTESIAN_POINT('Ctrl Pts',(5.83357047121772,3.43398979344032,18.8666630888483));
#13288=CARTESIAN_POINT('Ctrl Pts',(5.74105711948312,3.58225517667742,18.8748654435543));
#13289=CARTESIAN_POINT('Ctrl Pts',(5.64857490749069,3.73047065419043,18.8830650373702));
#13290=CARTESIAN_POINT('Ctrl Pts',(5.55031402033129,3.87515905834221,18.891264631186));
#13291=CARTESIAN_POINT('Ctrl Pts',(5.44658064382876,4.01584963491786,18.8994642250018));
#13292=CARTESIAN_POINT('Ctrl Pts',(5.34286336599554,4.1565183773342,18.9076625463));
#13293=CARTESIAN_POINT('Ctrl Pts',(5.23367550300273,4.29319023963244,18.9158608675982));
#13294=CARTESIAN_POINT('Ctrl Pts',(5.11936566405895,4.42542474771114,18.9240591888964));
#13295=CARTESIAN_POINT('Ctrl Pts',(5.0050528293004,4.55766272137161,18.932257725055));
#13296=CARTESIAN_POINT('Ctrl Pts',(4.88561798615235,4.68546283861832,18.9404562612135));
#13297=CARTESIAN_POINT('Ctrl Pts',(4.76144902863808,4.80841888230232,18.9486547973721));
#13298=CARTESIAN_POINT('Ctrl Pts',(4.63720149033507,4.93145273917801,18.9568585220049));
#13299=CARTESIAN_POINT('Ctrl Pts',(4.50821410524588,5.04963614355232,18.9650622466377));
#13300=CARTESIAN_POINT('Ctrl Pts',(4.37491108046193,5.16260031748066,18.9732659712705));
#13301=CARTESIAN_POINT('Ctrl Pts',(4.24156691491425,5.27559935507693,18.981472227785));
#13302=CARTESIAN_POINT('Ctrl Pts',(4.10390473449447,5.38337572724731,18.9896784842996));
#13303=CARTESIAN_POINT('Ctrl Pts',(3.96238058832069,5.48560197911764,18.9978847408141));
#13304=CARTESIAN_POINT('Ctrl Pts',(3.82070029851786,5.58794101723952,19.0061000512937));
#13305=CARTESIAN_POINT('Ctrl Pts',(3.67514982443726,5.68471749589009,19.0143153617733));
#13306=CARTESIAN_POINT('Ctrl Pts',(3.52621376002927,5.77564762763279,19.0225306722529));
#13307=CARTESIAN_POINT('Ctrl Pts',(3.38669939347668,5.86082551776338,19.0302262820581));
#13308=CARTESIAN_POINT('Ctrl Pts',(3.24421469581168,5.94087365416285,19.0379218918632));
#13309=CARTESIAN_POINT('Ctrl Pts',(3.09917575053257,6.0155962852664,19.0456175016683));
#13310=CARTESIAN_POINT('Ctrl Pts',(3.0991757505326,6.01559628526638,17.0457515827422));
#13311=CARTESIAN_POINT('Ctrl Pts',(2.93382384459263,6.1007839529376,17.0545010306546));
#13312=CARTESIAN_POINT('Ctrl Pts',(2.76495772122979,6.17915010267051,17.063250478567));
#13313=CARTESIAN_POINT('Ctrl Pts',(2.59315093316703,6.25042856433181,17.0719999264794));
#13314=CARTESIAN_POINT('Ctrl Pts',(2.42134553245612,6.32170645041453,17.0807493037394));
#13315=CARTESIAN_POINT('Ctrl Pts',(2.24659977927588,6.38589665313458,17.0894986809994));
#13316=CARTESIAN_POINT('Ctrl Pts',(2.0695071868992,6.44278115439075,17.0982480582594));
#13317=CARTESIAN_POINT('Ctrl Pts',(1.89241596572863,6.49966521519724,17.1069973677741));
#13318=CARTESIAN_POINT('Ctrl Pts',(1.71297821457199,6.54924360009546,17.1157466772887));
#13319=CARTESIAN_POINT('Ctrl Pts',(1.53180337335846,6.59134792173556,17.1244959868034));
#13320=CARTESIAN_POINT('Ctrl Pts',(1.35062987477791,6.63345193135303,17.1332452314795));
#13321=CARTESIAN_POINT('Ctrl Pts',(1.16771959102967,6.66808192368235,17.1419944761556));
#13322=CARTESIAN_POINT('Ctrl Pts',(0.98369374690707,6.69512028363165,17.1507437208318));
#13323=CARTESIAN_POINT('Ctrl Pts',(0.799669205420161,6.72215845218863,17.1594929035759));
#13324=CARTESIAN_POINT('Ctrl Pts',(0.614529402873832,6.74160505424576,17.1682420863201));
#13325=CARTESIAN_POINT('Ctrl Pts',(0.428903127363669,6.75339404354119,17.1769912690643));
#13326=CARTESIAN_POINT('Ctrl Pts',(0.243278104164388,6.76518295330328,17.1857403927829));
#13327=CARTESIAN_POINT('Ctrl Pts',(0.0571669005397141,6.76931433552275,
17.1944895165015));
#13328=CARTESIAN_POINT('Ctrl Pts',(-0.128798404776829,6.76577415902474,
17.2032386402201));
#13329=CARTESIAN_POINT('Ctrl Pts',(-0.314762517258441,6.76223400523445,
17.2119877078193));
#13330=CARTESIAN_POINT('Ctrl Pts',(-0.500580446818881,6.75102239665094,
17.2207367754185));
#13331=CARTESIAN_POINT('Ctrl Pts',(-0.68562111884201,6.73217741012504,17.2294858430177));
#13332=CARTESIAN_POINT('Ctrl Pts',(-0.870660665413904,6.71333253821779,
17.2382348574035));
#13333=CARTESIAN_POINT('Ctrl Pts',(-1.0549226788543,6.68685441030621,17.2469838717893));
#13334=CARTESIAN_POINT('Ctrl Pts',(-1.23778137635197,6.65283295028187,17.2557328861751));
#13335=CARTESIAN_POINT('Ctrl Pts',(-1.42999922978796,6.61707018861876,17.2649296965425));
#13336=CARTESIAN_POINT('Ctrl Pts',(-1.62066601233648,6.57297172934425,17.2741265069098));
#13337=CARTESIAN_POINT('Ctrl Pts',(-1.80906628500342,6.52070304311306,17.2833233172772));
#13338=CARTESIAN_POINT('Ctrl Pts',(-1.98831342545484,6.47097374915044,17.292073315015));
#13339=CARTESIAN_POINT('Ctrl Pts',(-2.16550875896659,6.41384933989543,17.3008233127528));
#13340=CARTESIAN_POINT('Ctrl Pts',(-2.34005036713969,6.34952386240492,17.3095733104905));
#13341=CARTESIAN_POINT('Ctrl Pts',(-2.51458843547048,6.28519968948612,17.3183231307714));
#13342=CARTESIAN_POINT('Ctrl Pts',(-2.68647261718017,6.21367483971116,17.3270729510523));
#13343=CARTESIAN_POINT('Ctrl Pts',(-2.85511905908695,6.13519226743861,17.3358227713331));
#13344=CARTESIAN_POINT('Ctrl Pts',(-3.02376230488844,6.05671118252957,17.3445724257917));
#13345=CARTESIAN_POINT('Ctrl Pts',(-3.18916767379861,5.97127275992656,17.3533220802502));
#13346=CARTESIAN_POINT('Ctrl Pts',(-3.35077334102741,5.87916720438023,17.3620717347087));
#13347=CARTESIAN_POINT('Ctrl Pts',(-3.5123761603733,5.78706327195666,17.3708212349772));
#13348=CARTESIAN_POINT('Ctrl Pts',(-3.6701791630227,5.68829258362318,17.3795707352456));
#13349=CARTESIAN_POINT('Ctrl Pts',(-3.8236463656644,5.58319061741057,17.3883202355141));
#13350=CARTESIAN_POINT('Ctrl Pts',(-3.97711106778777,5.47809036367717,17.3970695932225));
#13351=CARTESIAN_POINT('Ctrl Pts',(-4.12623987481906,5.36665920043241,17.4058189509309));
#13352=CARTESIAN_POINT('Ctrl Pts',(-4.27052628213909,5.24927559512351,17.4145683086394));
#13353=CARTESIAN_POINT('Ctrl Pts',(-4.41481053024959,5.13189374643053,17.4233175354159));
#13354=CARTESIAN_POINT('Ctrl Pts',(-4.55425230136512,5.00855981477369,17.4320667621924));
#13355=CARTESIAN_POINT('Ctrl Pts',(-4.68837800630531,4.87969268192093,17.4408159889689));
#13356=CARTESIAN_POINT('Ctrl Pts',(-4.82250188228881,4.75082730631823,17.4495650964398));
#13357=CARTESIAN_POINT('Ctrl Pts',(-4.95130963052956,4.61642907903537,17.4583142039106));
#13358=CARTESIAN_POINT('Ctrl Pts',(-5.0743637903336,4.47695444731697,17.4670633113815));
#13359=CARTESIAN_POINT('Ctrl Pts',(-5.19741643562807,4.33748153220584,17.4758123111712));
#13360=CARTESIAN_POINT('Ctrl Pts',(-5.31471544462783,4.19293255254577,17.484561310961));
#13361=CARTESIAN_POINT('Ctrl Pts',(-5.42586245275645,4.0437984177958,17.4933103107507));
#13362=CARTESIAN_POINT('Ctrl Pts',(-5.53702160019165,3.89464799484326,17.5020602660929));
#13363=CARTESIAN_POINT('Ctrl Pts',(-5.64202723081258,3.74091164443839,17.510810221435));
#13364=CARTESIAN_POINT('Ctrl Pts',(-5.74052265232969,3.58311159163229,17.5195601767772));
#13365=CARTESIAN_POINT('Ctrl Pts',(-5.83901427066926,3.4253176319177,17.5283097942596));
#13366=CARTESIAN_POINT('Ctrl Pts',(-5.93099603115752,3.2634605269559,17.5370594117421));
#13367=CARTESIAN_POINT('Ctrl Pts',(-6.01615550622771,3.09809004467044,17.5458090292245));
#13368=CARTESIAN_POINT('Ctrl Pts',(-6.10131214578817,2.93272506863792,17.5545583553756));
#13369=CARTESIAN_POINT('Ctrl Pts',(-6.17964682328765,2.76384720416855,17.5633076815267));
#13370=CARTESIAN_POINT('Ctrl Pts',(-6.25089348288581,2.59203002791551,17.5720570076778));
#13371=CARTESIAN_POINT('Ctrl Pts',(-6.32213814889336,2.42021765937011,17.5808060890094));
#13372=CARTESIAN_POINT('Ctrl Pts',(-6.38629508412582,2.24546640831924,17.5895551703409));
#13373=CARTESIAN_POINT('Ctrl Pts',(-6.44314639819802,2.06836976660073,17.5983042516725));
#13374=CARTESIAN_POINT('Ctrl Pts',(-6.50000285283694,1.891257111583,17.6070541241069));
#13375=CARTESIAN_POINT('Ctrl Pts',(-6.54955227673245,1.71179891440271,17.6158039965413));
#13376=CARTESIAN_POINT('Ctrl Pts',(-6.59162635926383,1.53060476278439,17.6245538689757));
#13377=CARTESIAN_POINT('Ctrl Pts',(-6.63369752055197,1.34942319164694,17.6333031338982));
#13378=CARTESIAN_POINT('Ctrl Pts',(-6.66829431424256,1.16650618642692,17.6420523988207));
#13379=CARTESIAN_POINT('Ctrl Pts',(-6.69529923745421,0.982474997618328,
17.6508016637432));
#13380=CARTESIAN_POINT('Ctrl Pts',(-6.72230554731447,0.798434359177448,
17.6595513779229));
#13381=CARTESIAN_POINT('Ctrl Pts',(-6.74171916496706,0.613279706239981,
17.6683010921026));
#13382=CARTESIAN_POINT('Ctrl Pts',(-6.75347414817278,0.427639953654957,
17.6770508062823));
#13383=CARTESIAN_POINT('Ctrl Pts',(-6.76248837758745,0.285283364198298,
17.6837604654582));
#13384=CARTESIAN_POINT('Ctrl Pts',(-6.76699999999997,0.142641701104988,
17.6904701246341));
#13385=CARTESIAN_POINT('Ctrl Pts',(-6.767,1.58636168174125E-12,17.69717978381));
#13386=CARTESIAN_POINT('',(-6.767,1.31424060002827E-12,17.3028202161899));
#13387=CARTESIAN_POINT('Ctrl Pts',(3.09917575053259,6.01559628526639,16.6515033120574));
#13388=CARTESIAN_POINT('Ctrl Pts',(2.94387506767171,6.09560566214935,16.6597008139785));
#13389=CARTESIAN_POINT('Ctrl Pts',(2.78542944909053,6.16962022082759,16.6678983158995));
#13390=CARTESIAN_POINT('Ctrl Pts',(2.62434447208533,6.23739569787225,16.6760958178206));
#13391=CARTESIAN_POINT('Ctrl Pts',(2.46326803250356,6.30516758285043,16.6842928852782));
#13392=CARTESIAN_POINT('Ctrl Pts',(2.29955284339014,6.36670090486711,16.6924899527357));
#13393=CARTESIAN_POINT('Ctrl Pts',(2.13372505003637,6.42179931256399,16.7006870201933));
#13394=CARTESIAN_POINT('Ctrl Pts',(1.96787590654538,6.47690481411734,16.7088851430138));
#13395=CARTESIAN_POINT('Ctrl Pts',(1.79991395740129,6.52557363774467,16.7170832658344));
#13396=CARTESIAN_POINT('Ctrl Pts',(1.6303811634924,6.5676591158288,16.7252813886549));
#13397=CARTESIAN_POINT('Ctrl Pts',(1.46079572998701,6.60975766137047,16.7334820569763));
#13398=CARTESIAN_POINT('Ctrl Pts',(1.28963882818744,6.64526870335634,16.7416827252977));
#13399=CARTESIAN_POINT('Ctrl Pts',(1.11746332919481,6.67409654619297,16.7498833936192));
#13400=CARTESIAN_POINT('Ctrl Pts',(0.945107085032572,6.70295465171721,16.7580926707798));
#13401=CARTESIAN_POINT('Ctrl Pts',(0.771730461697409,6.72511548321223,16.7663019479404));
#13402=CARTESIAN_POINT('Ctrl Pts',(0.597893167046674,6.7405350500386,16.7745112251011));
#13403=CARTESIAN_POINT('Ctrl Pts',(0.42395958531355,6.75596315763929,16.7827250493145));
#13404=CARTESIAN_POINT('Ctrl Pts',(0.249565181382425,6.76464253932623,16.7909388735278));
#13405=CARTESIAN_POINT('Ctrl Pts',(0.0752703002990371,6.76658136594048,
16.7991526977412));
#13406=CARTESIAN_POINT('Ctrl Pts',(-0.0992746015544309,6.76852297374325,
16.8073783044386));
#13407=CARTESIAN_POINT('Ctrl Pts',(-0.273719337000601,6.76370471566187,
16.815603911136));
#13408=CARTESIAN_POINT('Ctrl Pts',(-0.447506833163368,6.75218680386378,
16.8238295178335));
#13409=CARTESIAN_POINT('Ctrl Pts',(-0.586504537929725,6.74297461461549,
16.8304084747578));
#13410=CARTESIAN_POINT('Ctrl Pts',(-0.725081847503001,6.72947766089104,
16.8369874316822));
#13411=CARTESIAN_POINT('Ctrl Pts',(-0.862958650407477,6.71175024622393,
16.8435663886066));
#13412=CARTESIAN_POINT('Ctrl Pts',(-1.0338137569393,6.68978266895436,16.8517189448199));
#13413=CARTESIAN_POINT('Ctrl Pts',(-1.20409674113898,6.66125251078687,16.8598715010332));
#13414=CARTESIAN_POINT('Ctrl Pts',(-1.37325904243192,6.62619412652384,16.8680240572464));
#13415=CARTESIAN_POINT('Ctrl Pts',(-1.54222536512024,6.59117635824424,16.8761671685268));
#13416=CARTESIAN_POINT('Ctrl Pts',(-1.71007323507123,6.54964549238403,16.8843102798071));
#13417=CARTESIAN_POINT('Ctrl Pts',(-1.8762586493363,6.50168766404468,16.8924533910874));
#13418=CARTESIAN_POINT('Ctrl Pts',(-2.04228647220672,6.45377531346933,16.9005887803648));
#13419=CARTESIAN_POINT('Ctrl Pts',(-2.20665462915627,6.39944823464897,16.9087241696421));
#13420=CARTESIAN_POINT('Ctrl Pts',(-2.36882876158522,6.33884368779407,16.9168595589195));
#13421=CARTESIAN_POINT('Ctrl Pts',(-2.53088318316271,6.27828387693865,16.9249889429582));
#13422=CARTESIAN_POINT('Ctrl Pts',(-2.69074646403248,6.21145595216779,16.9331183269968));
#13423=CARTESIAN_POINT('Ctrl Pts',(-2.84789888639288,6.13854713534744,16.9412477110355));
#13424=CARTESIAN_POINT('Ctrl Pts',(-3.00496831426195,6.06567682273895,16.9493728018276));
#13425=CARTESIAN_POINT('Ctrl Pts',(-3.1593294039289,5.98673216723843,16.9574978926197));
#13426=CARTESIAN_POINT('Ctrl Pts',(-3.31048193344775,5.90194869245032,16.9656229834118));
#13427=CARTESIAN_POINT('Ctrl Pts',(-3.46221144494007,5.81684158075877,16.9737790894369));
#13428=CARTESIAN_POINT('Ctrl Pts',(-3.61070750648893,5.72585112334431,16.981935195462));
#13429=CARTESIAN_POINT('Ctrl Pts',(-3.7554881793884,5.62926261018919,16.9900913014871));
#13430=CARTESIAN_POINT('Ctrl Pts',(-3.89968613626307,5.53306284833147,16.9982145806605));
#13431=CARTESIAN_POINT('Ctrl Pts',(-4.04019826204967,5.43131023172939,17.0063378598339));
#13432=CARTESIAN_POINT('Ctrl Pts',(-4.17657693742558,5.32433038848688,17.0144611390073));
#13433=CARTESIAN_POINT('Ctrl Pts',(-4.31297377277473,5.21733629997409,17.0225854998639));
#13434=CARTESIAN_POINT('Ctrl Pts',(-4.44523577354727,5.10511382422921,17.0307098607206));
#13435=CARTESIAN_POINT('Ctrl Pts',(-4.57294805431455,4.98802917919901,17.0388342215773));
#13436=CARTESIAN_POINT('Ctrl Pts',(-4.70070163897,4.87090666740255,17.0469612099627));
#13437=CARTESIAN_POINT('Ctrl Pts',(-4.82390230400096,4.74891910207833,17.0550881983481));
#13438=CARTESIAN_POINT('Ctrl Pts',(-4.94217174629426,4.62246984091089,17.0632151867336));
#13439=CARTESIAN_POINT('Ctrl Pts',(-5.06120578706661,4.49520309966668,17.0713947151736));
#13440=CARTESIAN_POINT('Ctrl Pts',(-5.1752443677409,4.36341704834046,17.0795742436137));
#13441=CARTESIAN_POINT('Ctrl Pts',(-5.28394330108761,4.22755629068277,17.0877537720537));
#13442=CARTESIAN_POINT('Ctrl Pts',(-5.39213033611443,4.09233534513216,17.0958947804574));
#13443=CARTESIAN_POINT('Ctrl Pts',(-5.49502774242374,3.95307832093067,17.1040357888611));
#13444=CARTESIAN_POINT('Ctrl Pts',(-5.5923402341602,3.81025192151295,17.1121767972648));
#13445=CARTESIAN_POINT('Ctrl Pts',(-5.69034339231075,3.66641182492886,17.1203755857231));
#13446=CARTESIAN_POINT('Ctrl Pts',(-5.7826818672945,3.51895182023507,17.1285743741813));
#13447=CARTESIAN_POINT('Ctrl Pts',(-5.86910172030054,3.3683726036122,17.1367731626396));
#13448=CARTESIAN_POINT('Ctrl Pts',(-5.95552157330658,3.21779338698933,17.1449719510978));
#13449=CARTESIAN_POINT('Ctrl Pts',(-6.03602268941887,3.06409531746996,17.153170739556));
#13450=CARTESIAN_POINT('Ctrl Pts',(-6.11040100682139,2.90779788428223,17.1613695280143));
#13451=CARTESIAN_POINT('Ctrl Pts',(-6.19254802448167,2.73517542584659,17.170424667251));
#13452=CARTESIAN_POINT('Ctrl Pts',(-6.26744643549823,2.55892230665628,17.1794798064877));
#13453=CARTESIAN_POINT('Ctrl Pts',(-6.33479437433313,2.37963636611087,17.1885349457244));
#13454=CARTESIAN_POINT('Ctrl Pts',(-6.40198623639121,2.20076591521835,17.1975690999545));
#13455=CARTESIAN_POINT('Ctrl Pts',(-6.46166245057633,2.01887688447162,17.2066032541845));
#13456=CARTESIAN_POINT('Ctrl Pts',(-6.51356849724899,1.83458835482121,17.2156374084146));
#13457=CARTESIAN_POINT('Ctrl Pts',(-6.56528345218299,1.65097828207134,17.2246383034706));
#13458=CARTESIAN_POINT('Ctrl Pts',(-6.60928523640393,1.46498655862471,17.2336391985266));
#13459=CARTESIAN_POINT('Ctrl Pts',(-6.64536888477817,1.27724758180319,17.2426400935826));
#13460=CARTESIAN_POINT('Ctrl Pts',(-6.68136586184701,1.08995954558578,17.2516193688923));
#13461=CARTESIAN_POINT('Ctrl Pts',(-6.70948258695721,0.900932855765144,
17.260598644202));
#13462=CARTESIAN_POINT('Ctrl Pts',(-6.72956382804599,0.710816209898906,
17.2695779195117));
#13463=CARTESIAN_POINT('Ctrl Pts',(-6.74957342088702,0.52137788488361,17.2785251574917));
#13464=CARTESIAN_POINT('Ctrl Pts',(-6.76160468038598,0.330857593982595,
17.2874723954717));
#13465=CARTESIAN_POINT('Ctrl Pts',(-6.7655534494534,0.139912553365295,17.2964196334517));
#13466=CARTESIAN_POINT('Ctrl Pts',(-6.76649505933669,0.0943804560610796,
17.2985531610311));
#13467=CARTESIAN_POINT('Ctrl Pts',(-6.76697731126835,0.0488242673506343,
17.3006866886105));
#13468=CARTESIAN_POINT('Ctrl Pts',(-6.76699921811354,0.00325300641797097,
17.3028202161899));
#13469=CARTESIAN_POINT('Ctrl Pts',(-6.767,1.3142405932883E-12,17.3028202161899));
#13470=CARTESIAN_POINT('Ctrl Pts',(-6.76700000000004,-0.186007249414463,
17.3115697279959));
#13471=CARTESIAN_POINT('Ctrl Pts',(-6.75932637295445,-0.372014355526415,
17.3203192398018));
#13472=CARTESIAN_POINT('Ctrl Pts',(-6.74400518266936,-0.55738953715403,
17.3290687516078));
#13473=CARTESIAN_POINT('Ctrl Pts',(-6.72868405709656,-0.742763935810426,
17.3378182264583));
#13474=CARTESIAN_POINT('Ctrl Pts',(-6.70571545653004,-0.927506129694114,
17.3465677013089));
#13475=CARTESIAN_POINT('Ctrl Pts',(-6.67517739415665,-1.11098863924889,
17.3553171761594));
#13476=CARTESIAN_POINT('Ctrl Pts',(-6.64463945823082,-1.29447038906596,
17.3640666147814));
#13477=CARTESIAN_POINT('Ctrl Pts',(-6.60653217027133,-1.47669218228329,
17.3728160534034));
#13478=CARTESIAN_POINT('Ctrl Pts',(-6.56098496116679,-1.6570351050425,17.3815654920254));
#13479=CARTESIAN_POINT('Ctrl Pts',(-6.51543793687478,-1.8373772960416,17.3903148951456));
#13480=CARTESIAN_POINT('Ctrl Pts',(-6.46245112202593,-2.01584035397204,
17.3990642982658));
#13481=CARTESIAN_POINT('Ctrl Pts',(-6.40220448416188,-2.19181813638304,
17.4078137013861));
#13482=CARTESIAN_POINT('Ctrl Pts',(-6.34195808575124,-2.36779521936114,
17.4165630697314));
#13483=CARTESIAN_POINT('Ctrl Pts',(-6.27445201489162,-2.54128677545007,
17.4253124380766));
#13484=CARTESIAN_POINT('Ctrl Pts',(-6.19991555136101,-2.71170355238029,
17.4340618064219));
#13485=CARTESIAN_POINT('Ctrl Pts',(-6.12537937788951,-2.88211966613258,
17.442811140719));
#13486=CARTESIAN_POINT('Ctrl Pts',(-6.04381298133524,-3.04946076210629,
17.451560475016));
#13487=CARTESIAN_POINT('Ctrl Pts',(-5.95549339426208,-3.21315848207036,
17.4603098093131));
#13488=CARTESIAN_POINT('Ctrl Pts',(-5.86717414355064,-3.37685557859803,
17.4690591102886));
#13489=CARTESIAN_POINT('Ctrl Pts',(-5.77210188986144,-3.53690907467464,
17.4778084112642));
#13490=CARTESIAN_POINT('Ctrl Pts',(-5.67059953466978,-3.69277536785043,
17.4865577122398));
#13491=CARTESIAN_POINT('Ctrl Pts',(-5.56909755761672,-3.84864108035928,
17.4953069806205));
#13492=CARTESIAN_POINT('Ctrl Pts',(-5.46116568337973,-4.00031938104412,
17.5040562490013));
#13493=CARTESIAN_POINT('Ctrl Pts',(-5.34717048686014,-4.14729511663348,
17.512805517382));
#13494=CARTESIAN_POINT('Ctrl Pts',(-5.23317570555423,-4.29427031688155,
17.5215547538947));
#13495=CARTESIAN_POINT('Ctrl Pts',(-5.11311782178717,-4.43654275987231,
17.5303039904073));
#13496=CARTESIAN_POINT('Ctrl Pts',(-4.98740459171933,-4.57362924147738,
17.5390532269199));
#13497=CARTESIAN_POINT('Ctrl Pts',(-4.86169180910726,-4.71071523514545,
17.547802432291));
#13498=CARTESIAN_POINT('Ctrl Pts',(-4.73032391415303,-4.8426150931665,17.5565516376621));
#13499=CARTESIAN_POINT('Ctrl Pts',(-4.59374707237139,-4.96888084331666,
17.5653008430333));
#13500=CARTESIAN_POINT('Ctrl Pts',(-4.45717070537242,-5.09514615452864,
17.5740500179895));
#13501=CARTESIAN_POINT('Ctrl Pts',(-4.31538563819344,-5.21577720253769,
17.5827991929457));
#13502=CARTESIAN_POINT('Ctrl Pts',(-4.16887341290477,-5.33036429028783,
17.591548367902));
#13503=CARTESIAN_POINT('Ctrl Pts',(-4.0223616847716,-5.44495098921308,17.6002975131699));
#13504=CARTESIAN_POINT('Ctrl Pts',(-3.87112305634253,-5.55349359238889,
17.6090466584378));
#13505=CARTESIAN_POINT('Ctrl Pts',(-3.71567117316539,-5.655623461026,17.6177958037057));
#13506=CARTESIAN_POINT('Ctrl Pts',(-3.56021980457122,-5.75775299158879,
17.6265449200119));
#13507=CARTESIAN_POINT('Ctrl Pts',(-3.40055544862225,-5.85346967275447,
17.635294036318));
#13508=CARTESIAN_POINT('Ctrl Pts',(-3.23722036323257,-5.94244842803641,
17.6440431526242));
#13509=CARTESIAN_POINT('Ctrl Pts',(-3.07388580495924,-6.03142689616537,
17.6527922406951));
#13510=CARTESIAN_POINT('Ctrl Pts',(-2.90688079257609,-6.11366734484868,
17.661541328766));
#13511=CARTESIAN_POINT('Ctrl Pts',(-2.73677251094543,-6.18889046787334,
17.670290416837));
#13512=CARTESIAN_POINT('Ctrl Pts',(-2.56666476416605,-6.26411335438286,
17.6790394773992));
#13513=CARTESIAN_POINT('Ctrl Pts',(-2.39345402972086,-6.33231884350292,
17.6877885379614));
#13514=CARTESIAN_POINT('Ctrl Pts',(-2.21772856474065,-6.39327529621034,
17.6965375985236));
#13515=CARTESIAN_POINT('Ctrl Pts',(-2.04200363768265,-6.45423156232084,
17.7052866323036));
#13516=CARTESIAN_POINT('Ctrl Pts',(-1.86376426620056,-6.50793874252067,
17.7140356660836));
#13517=CARTESIAN_POINT('Ctrl Pts',(-1.68361578194618,-6.55421443796141,
17.7227846998637));
#13518=CARTESIAN_POINT('Ctrl Pts',(-1.50346783419837,-6.60048999558686,
17.7315337075879));
#13519=CARTESIAN_POINT('Ctrl Pts',(-1.32141106257255,-6.63933404145493,
17.7402827153121));
#13520=CARTESIAN_POINT('Ctrl Pts',(-1.13806375959093,-6.67061465527022,
17.7490317230363));
#13521=CARTESIAN_POINT('Ctrl Pts',(-0.954716987419442,-6.70189517852477,
17.7577807054312));
#13522=CARTESIAN_POINT('Ctrl Pts',(-0.770079973809966,-6.72561226535827,
17.7665296878261));
#13523=CARTESIAN_POINT('Ctrl Pts',(-0.584779770552345,-6.74168536939783,
17.775278670221));
#13524=CARTESIAN_POINT('Ctrl Pts',(-0.391490647553809,-6.75845143942394,
17.784404850897));
#13525=CARTESIAN_POINT('Ctrl Pts',(-0.19748021310424,-6.76689975924027,
17.7935310315731));
#13526=CARTESIAN_POINT('Ctrl Pts',(-0.0034653262977096,-6.76699911271707,
17.8026572122491));
#13527=CARTESIAN_POINT('Ctrl Pts',(0.184486595296115,-6.76709536139773,
17.8114981997791));
#13528=CARTESIAN_POINT('Ctrl Pts',(0.372442378185263,-6.7593565972677,17.820339187309));
#13529=CARTESIAN_POINT('Ctrl Pts',(0.559750217722093,-6.74380965729016,
17.8291801748389));
#13530=CARTESIAN_POINT('Ctrl Pts',(0.745129914457804,-6.72842275717253,
17.8379301534367));
#13531=CARTESIAN_POINT('Ctrl Pts',(0.929874656314276,-6.70538772273472,
17.8466801320345));
#13532=CARTESIAN_POINT('Ctrl Pts',(1.11335688289791,-6.6747828018074,17.8554301106322));
#13533=CARTESIAN_POINT('Ctrl Pts',(1.29683723118871,-6.64417819418021,17.8641799996572));
#13534=CARTESIAN_POINT('Ctrl Pts',(1.47905480730249,-6.60600390230072,17.8729298886821));
#13535=CARTESIAN_POINT('Ctrl Pts',(1.65939064804823,-6.56038959797131,17.881679777707));
#13536=CARTESIAN_POINT('Ctrl Pts',(1.83972470264283,-6.51477574543251,17.890429580068));
#13537=CARTESIAN_POINT('Ctrl Pts',(2.01817678125869,-6.46172209820093,17.8991793824289));
#13538=CARTESIAN_POINT('Ctrl Pts',(2.19414072347704,-6.40140886724006,17.9079291847899));
#13539=CARTESIAN_POINT('Ctrl Pts',(2.37010298132117,-6.34109621361367,17.9166789033954));
#13540=CARTESIAN_POINT('Ctrl Pts',(2.54357687926929,-6.27352420825964,17.9254286220009));
#13541=CARTESIAN_POINT('Ctrl Pts',(2.71397317789983,-6.19892237325491,17.9341783406064));
#13542=CARTESIAN_POINT('Ctrl Pts',(2.8843679020721,-6.12432122756959,17.9429279783646));
#13543=CARTESIAN_POINT('Ctrl Pts',(3.05168482126262,-6.04269049717414,17.9516776161229));
#13544=CARTESIAN_POINT('Ctrl Pts',(3.21535561997391,-5.95430745234928,17.9604272538812));
#13545=CARTESIAN_POINT('Ctrl Pts',(3.37902496075278,-5.86592519481518,17.9691768137002));
#13546=CARTESIAN_POINT('Ctrl Pts',(3.53904799384867,-5.77079087940237,17.9779263735192));
#13547=CARTESIAN_POINT('Ctrl Pts',(3.69488118814971,-5.66922763747033,17.9866759333382));
#13548=CARTESIAN_POINT('Ctrl Pts',(3.85071304610825,-5.56766526649057,17.9954254181256));
#13549=CARTESIAN_POINT('Ctrl Pts',(4.00235489705966,-5.45967423580715,18.0041749029131));
#13550=CARTESIAN_POINT('Ctrl Pts',(4.14929168607657,-5.34562133936326,18.0129243877005));
#13551=CARTESIAN_POINT('Ctrl Pts',(4.29622726385759,-5.23156938308529,18.0216738003638));
#13552=CARTESIAN_POINT('Ctrl Pts',(4.43845763092068,-5.11145583677202,18.0304232130271));
#13553=CARTESIAN_POINT('Ctrl Pts',(4.57549970660961,-4.98568866204212,18.0391726256904));
#13554=CARTESIAN_POINT('Ctrl Pts',(4.71254069815295,-4.85992248226161,18.0479219691367));
#13555=CARTESIAN_POINT('Ctrl Pts',(4.84439326931316,-4.72850295734001,18.0566713125831));
#13556=CARTESIAN_POINT('Ctrl Pts',(4.97060959434701,-4.59187644221679,18.0654206560294));
#13557=CARTESIAN_POINT('Ctrl Pts',(5.09682496280519,-4.4552509625666,18.0741699331657));
#13558=CARTESIAN_POINT('Ctrl Pts',(5.21740397615844,-4.3134187821832,18.082919210302));
#13559=CARTESIAN_POINT('Ctrl Pts',(5.3319371045194,-4.1668616143867,18.0916684874383));
#13560=CARTESIAN_POINT('Ctrl Pts',(5.44646940289394,-4.020305508645,18.1004177011712));
#13561=CARTESIAN_POINT('Ctrl Pts',(5.5549557274968,-3.86902470980112,18.1091669149042));
#13562=CARTESIAN_POINT('Ctrl Pts',(5.65702762491475,-3.71353301465753,18.1179161286372));
#13563=CARTESIAN_POINT('Ctrl Pts',(5.75909881655179,-3.55804239466852,18.1266652818733));
#13564=CARTESIAN_POINT('Ctrl Pts',(5.85475551250813,-3.398341176195,18.1354144351094));
#13565=CARTESIAN_POINT('Ctrl Pts',(5.94367283728131,-3.23497174691903,18.1441635883455));
#13566=CARTESIAN_POINT('Ctrl Pts',(6.03258957676337,-3.07160339300914,18.1529126839911));
#13567=CARTESIAN_POINT('Ctrl Pts',(6.11476689685301,-2.90456712829467,18.1616617796366));
#13568=CARTESIAN_POINT('Ctrl Pts',(6.18992570525271,-2.73443024475883,18.1704108752821));
#13569=CARTESIAN_POINT('Ctrl Pts',(6.26508404388721,-2.56429442462974,18.1791599162432));
#13570=CARTESIAN_POINT('Ctrl Pts',(6.3332238428335,-2.39105828655902,18.1879089572042));
#13571=CARTESIAN_POINT('Ctrl Pts',(6.39411368720077,-2.21531017131955,18.1966579981652));
#13572=CARTESIAN_POINT('Ctrl Pts',(6.45500317120938,-2.03956309619365,18.2054069873477));
#13573=CARTESIAN_POINT('Ctrl Pts',(6.50864269270123,-1.8613043443846,18.2141559765301));
#13574=CARTESIAN_POINT('Ctrl Pts',(6.55485008446384,-1.68113930719747,18.2229049657125));
#13575=CARTESIAN_POINT('Ctrl Pts',(6.60199664749448,-1.49731239211644,18.2318317792419));
#13576=CARTESIAN_POINT('Ctrl Pts',(6.64140563640945,-1.31150116499477,18.2407585927712));
#13577=CARTESIAN_POINT('Ctrl Pts',(6.67293772282205,-1.12436255155468,18.2496854063006));
#13578=CARTESIAN_POINT('Ctrl Pts',(6.70384494949898,-0.940932395049429,
18.2584353204561));
#13579=CARTESIAN_POINT('Ctrl Pts',(6.72718449348952,-0.756227260504809,
18.2671852346116));
#13580=CARTESIAN_POINT('Ctrl Pts',(6.74287707373948,-0.570874564539798,
18.2759351487672));
#13581=CARTESIAN_POINT('Ctrl Pts',(6.75856934538681,-0.385525513630582,
18.2846848908511));
#13582=CARTESIAN_POINT('Ctrl Pts',(6.76661493004109,-0.199529212416338,
18.2934346329351));
#13583=CARTESIAN_POINT('Ctrl Pts',(6.76698649908907,-0.0135174385985409,
18.3021843750191));
#13584=CARTESIAN_POINT('Ctrl Pts',(6.76735806132385,0.172490924447659,18.310933956665));
#13585=CARTESIAN_POINT('Ctrl Pts',(6.76005588896279,0.358514472903279,18.3196835383109));
#13586=CARTESIAN_POINT('Ctrl Pts',(6.74510478454569,0.543921359664073,18.3284331199568));
#13587=CARTESIAN_POINT('Ctrl Pts',(6.73015393440668,0.729325093152307,18.3371825527958));
#13588=CARTESIAN_POINT('Ctrl Pts',(6.70755443556872,0.914111900258213,18.3459319856349));
#13589=CARTESIAN_POINT('Ctrl Pts',(6.67738304682288,1.09765415591724,18.3546814184739));
#13590=CARTESIAN_POINT('Ctrl Pts',(6.64721213111824,1.28119353391464,18.3634307141353));
#13591=CARTESIAN_POINT('Ctrl Pts',(6.60946960955451,1.46348811672849,18.3721800097966));
#13592=CARTESIAN_POINT('Ctrl Pts',(6.56428366991133,1.64391876348422,18.3809293054579));
#13593=CARTESIAN_POINT('Ctrl Pts',(6.51909837867661,1.82434682109919,18.3896784755687));
#13594=CARTESIAN_POINT('Ctrl Pts',(6.46646995271857,2.00291071820652,18.3984276456796));
#13595=CARTESIAN_POINT('Ctrl Pts',(6.40657713281478,2.17900400212913,18.4071768157904));
#13596=CARTESIAN_POINT('Ctrl Pts',(6.34668509278982,2.35509499309869,18.4159258719762));
#13597=CARTESIAN_POINT('Ctrl Pts',(6.27952894037441,2.52871516398334,18.4246749281619));
#13598=CARTESIAN_POINT('Ctrl Pts',(6.20533675061354,2.69927486771632,18.4334239843477));
#13599=CARTESIAN_POINT('Ctrl Pts',(6.12832117907823,2.87632521636121,18.44250598563));
#13600=CARTESIAN_POINT('Ctrl Pts',(6.04372366625987,3.0500772892018,18.4515879869122));
#13601=CARTESIAN_POINT('Ctrl Pts',(5.95185378007777,3.21989527478364,18.4606699881945));
#13602=CARTESIAN_POINT('Ctrl Pts',(5.86334450817275,3.38350129286918,18.4694197685016));
#13603=CARTESIAN_POINT('Ctrl Pts',(5.76808562057155,3.54345567125125,18.4781695488088));
#13604=CARTESIAN_POINT('Ctrl Pts',(5.6664006880438,3.69921508465469,18.4869193291159));
#13605=CARTESIAN_POINT('Ctrl Pts',(5.56471941107814,3.85496889852441,18.4956687948694));
#13606=CARTESIAN_POINT('Ctrl Pts',(5.45661270815,4.00652780919792,18.5044182606228));
#13607=CARTESIAN_POINT('Ctrl Pts',(5.34244776448995,4.15337704569382,18.5131677263763));
#13608=CARTESIAN_POINT('Ctrl Pts',(5.2282863181947,4.30022178356402,18.5219169240959));
#13609=CARTESIAN_POINT('Ctrl Pts',(5.10806717843938,4.4423569097283,18.5306661218155));
#13610=CARTESIAN_POINT('Ctrl Pts',(4.98219864544582,4.57929969070794,18.5394153195351));
#13611=CARTESIAN_POINT('Ctrl Pts',(4.8563332994389,4.71623900430139,18.5481642957254));
#13612=CARTESIAN_POINT('Ctrl Pts',(4.72481904033517,4.84798602483744,18.5569132719156));
#13613=CARTESIAN_POINT('Ctrl Pts',(4.58810250737072,4.97409332259242,18.5656622481058));
#13614=CARTESIAN_POINT('Ctrl Pts',(4.45137708685508,5.10020881822252,18.574411793042));
#13615=CARTESIAN_POINT('Ctrl Pts',(4.3094489263591,5.2206836630805,18.5831613379782));
#13616=CARTESIAN_POINT('Ctrl Pts',(4.16280009466513,5.33510865604966,18.5919108829144));
#13617=CARTESIAN_POINT('Ctrl Pts',(4.01615988348645,5.44952692272997,18.6006599135226));
#13618=CARTESIAN_POINT('Ctrl Pts',(3.86479978232093,5.55789587288722,18.6094089441309));
#13619=CARTESIAN_POINT('Ctrl Pts',(3.70923383580937,5.65984746713964,18.6181579747392));
#13620=CARTESIAN_POINT('Ctrl Pts',(3.55366577799398,5.76180044505471,18.6269071240872));
#13621=CARTESIAN_POINT('Ctrl Pts',(3.39389200026687,5.85733573571148,18.6356562734352));
#13622=CARTESIAN_POINT('Ctrl Pts',(3.23045513625876,5.94612887622018,18.6444054227833));
#13623=CARTESIAN_POINT('Ctrl Pts',(3.18695122151468,5.96976399206746,18.6467342868962));
#13624=CARTESIAN_POINT('Ctrl Pts',(3.1431879126261,5.99292165435361,18.6490631510091));
#13625=CARTESIAN_POINT('Ctrl Pts',(3.0991757505326,6.01559628526638,18.6513920151221));
#13626=CARTESIAN_POINT('Origin',(0.,0.,-3.69717978381041));
#13627=CARTESIAN_POINT('',(3.09917575053256,6.01559628526641,21.0459192328109));
#13628=CARTESIAN_POINT('',(3.09917575053258,6.01559628526639,20.6513153324719));
#13629=CARTESIAN_POINT('',(3.09917575053259,6.01559628526639,-3.69717978381041));
#13630=CARTESIAN_POINT('',(-6.76699999885939,0.000124246054141125,19.6971797837639));
#13631=CARTESIAN_POINT('Ctrl Pts',(-6.7669999988594,0.000124245080715397,
19.69717978381));
#13632=CARTESIAN_POINT('Ctrl Pts',(-6.76700118044791,-0.0642308935099812,
19.7002280624878));
#13633=CARTESIAN_POINT('Ctrl Pts',(-6.76608434959876,-0.128580038527749,
19.7032763411655));
#13634=CARTESIAN_POINT('Ctrl Pts',(-6.76424985513672,-0.192906446970697,
19.7063246198433));
#13635=CARTESIAN_POINT('Ctrl Pts',(-6.75934273488779,-0.364974244362719,
19.71447851201));
#13636=CARTESIAN_POINT('Ctrl Pts',(-6.74785774407388,-0.537136539239102,
19.7226324041768));
#13637=CARTESIAN_POINT('Ctrl Pts',(-6.72977177811207,-0.708844704096933,
19.7307862963435));
#13638=CARTESIAN_POINT('Ctrl Pts',(-6.71170788208171,-0.880343337020776,
19.7389302384837));
#13639=CARTESIAN_POINT('Ctrl Pts',(-6.68705908253956,-1.05138858338574,
19.7470741806239));
#13640=CARTESIAN_POINT('Ctrl Pts',(-6.65585423478447,-1.22143088437358,
19.7552181227641));
#13641=CARTESIAN_POINT('Ctrl Pts',(-6.62468089766368,-1.39130147676015,
19.763353841157));
#13642=CARTESIAN_POINT('Ctrl Pts',(-6.58696475753452,-1.56017078306157,
19.7714895595499));
#13643=CARTESIAN_POINT('Ctrl Pts',(-6.54278651691789,-1.72749344254543,
19.7796252779428));
#13644=CARTESIAN_POINT('Ctrl Pts',(-6.49864359455563,-1.894682336081,19.787754492243));
#13645=CARTESIAN_POINT('Ctrl Pts',(-6.44804895089964,-2.06032669284818,
19.7958837065432));
#13646=CARTESIAN_POINT('Ctrl Pts',(-6.39113450760167,-2.22389044373665,
19.8040129208434));
#13647=CARTESIAN_POINT('Ctrl Pts',(-6.33425359753551,-2.387357825042,19.8121373455189));
#13648=CARTESIAN_POINT('Ctrl Pts',(-6.27106042297508,-2.54874669725629,
19.8202617701943));
#13649=CARTESIAN_POINT('Ctrl Pts',(-6.20173698750099,-2.70753528838725,
19.8283861948698));
#13650=CARTESIAN_POINT('Ctrl Pts',(-6.13199271439522,-2.86728782791703,
19.8365599400039));
#13651=CARTESIAN_POINT('Ctrl Pts',(-6.05604360342782,-3.02440804940822,
19.8447336851381));
#13652=CARTESIAN_POINT('Ctrl Pts',(-5.97412475089426,-3.17838362391211,
19.8529074302723));
#13653=CARTESIAN_POINT('Ctrl Pts',(-5.89273048272117,-3.3313731838933,19.8610288331345));
#13654=CARTESIAN_POINT('Ctrl Pts',(-5.80544290068403,-3.48125793792535,
19.8691502359966));
#13655=CARTESIAN_POINT('Ctrl Pts',(-5.71253922890306,-3.62755903580405,
19.8772716388588));
#13656=CARTESIAN_POINT('Ctrl Pts',(-5.61962837429932,-3.77387144491337,
19.885393669625));
#13657=CARTESIAN_POINT('Ctrl Pts',(-5.52110076120839,-3.91659933698607,
19.8935157003913));
#13658=CARTESIAN_POINT('Ctrl Pts',(-5.41727741718297,-4.05529214549081,
19.9016377311575));
#13659=CARTESIAN_POINT('Ctrl Pts',(-5.31342627572112,-4.19402208730659,
19.9097619364987));
#13660=CARTESIAN_POINT('Ctrl Pts',(-5.20427679933225,-4.32871450152973,
19.9178861418398));
#13661=CARTESIAN_POINT('Ctrl Pts',(-5.0901907940493,-4.45895129825117,19.9260103471809));
#13662=CARTESIAN_POINT('Ctrl Pts',(-4.9748698867004,-4.59059781818042,19.9342224914233));
#13663=CARTESIAN_POINT('Ctrl Pts',(-4.85450520926144,-4.71769140998133,
19.9424346356658));
#13664=CARTESIAN_POINT('Ctrl Pts',(-4.72950863058107,-4.83983854206514,
19.9506467799082));
#13665=CARTESIAN_POINT('Ctrl Pts',(-4.60565313290003,-4.96087060545654,
19.9587839563246));
#13666=CARTESIAN_POINT('Ctrl Pts',(-4.47725026378617,-5.07704594622458,
19.9669211327411));
#13667=CARTESIAN_POINT('Ctrl Pts',(-4.34473366381677,-5.18802258962867,
19.9750583091576));
#13668=CARTESIAN_POINT('Ctrl Pts',(-4.21038575021389,-5.30053287515843,
19.983307937313));
#13669=CARTESIAN_POINT('Ctrl Pts',(-4.07180988413855,-5.40769948419134,
19.9915575654684));
#13670=CARTESIAN_POINT('Ctrl Pts',(-3.92948752405395,-5.50921199431501,
19.9998071936238));
#13671=CARTESIAN_POINT('Ctrl Pts',(-3.78716516396939,-5.61072450443865,
20.0080568217793));
#13672=CARTESIAN_POINT('Ctrl Pts',(-3.64109666627524,-5.70658275743039,
20.0163064499347));
#13673=CARTESIAN_POINT('Ctrl Pts',(-3.49178809428973,-5.79652524402133,
20.0245560780901));
#13674=CARTESIAN_POINT('Ctrl Pts',(-3.34292765784637,-5.88619777675459,
20.0327809457677));
#13675=CARTESIAN_POINT('Ctrl Pts',(-3.19040169834388,-5.97025819324048,
20.0410058134453));
#13676=CARTESIAN_POINT('Ctrl Pts',(-3.03467163341242,-6.04839293344621,
20.0492306811229));
#13677=CARTESIAN_POINT('Ctrl Pts',(-2.87911701583027,-6.12643964612132,
20.0574462825664));
#13678=CARTESIAN_POINT('Ctrl Pts',(-2.72036579856576,-6.19857381658468,
20.06566188401));
#13679=CARTESIAN_POINT('Ctrl Pts',(-2.55890746445812,-6.26452564751239,
20.0738774854535));
#13680=CARTESIAN_POINT('Ctrl Pts',(-2.39759859101656,-6.33041642736686,
20.0820854817816));
#13681=CARTESIAN_POINT('Ctrl Pts',(-2.23358792143174,-6.39013613022706,
20.0902934781098));
#13682=CARTESIAN_POINT('Ctrl Pts',(-2.06738865823994,-6.44346126982858,
20.0985014744379));
#13683=CARTESIAN_POINT('Ctrl Pts',(-1.90130986236754,-6.49674775741382,
20.1067035213094));
#13684=CARTESIAN_POINT('Ctrl Pts',(-1.7330459728758,-6.54364880464831,20.1149055681808));
#13685=CARTESIAN_POINT('Ctrl Pts',(-1.56312933574331,-6.58398934383545,
20.1231076150523));
#13686=CARTESIAN_POINT('Ctrl Pts',(-1.39330173963801,-6.62430874346198,
20.1313053638238));
#13687=CARTESIAN_POINT('Ctrl Pts',(-1.22182346951432,-6.65807440118618,
20.1395031125954));
#13688=CARTESIAN_POINT('Ctrl Pts',(-1.04924125274902,-6.6851613139497,20.147700861367));
#13689=CARTESIAN_POINT('Ctrl Pts',(-0.876691952575874,-6.71224306042856,
20.1558970465826));
#13690=CARTESIAN_POINT('Ctrl Pts',(-0.703039478270456,-6.73264853755229,
20.1640932317982));
#13691=CARTESIAN_POINT('Ctrl Pts',(-0.528840259173994,-6.74630394959172,
20.1722894170138));
#13692=CARTESIAN_POINT('Ctrl Pts',(-0.354653926942446,-6.75995835143459,
20.1804849958942));
#13693=CARTESIAN_POINT('Ctrl Pts',(-0.179921288127777,-6.76686365373732,
20.1886805747745));
#13694=CARTESIAN_POINT('Ctrl Pts',(-0.00520334358890041,-6.76699799949841,
20.1968761536548));
#13695=CARTESIAN_POINT('Ctrl Pts',(0.169533463571664,-6.76713235976353,
20.2050726173333));
#13696=CARTESIAN_POINT('Ctrl Pts',(0.344255214392696,-6.76049430684536,
20.2132690810117));
#13697=CARTESIAN_POINT('Ctrl Pts',(0.51840140640271,-6.74711412248524,20.2214655446901));
#13698=CARTESIAN_POINT('Ctrl Pts',(0.69259808327754,-6.73373005921859,20.2296643845179));
#13699=CARTESIAN_POINT('Ctrl Pts',(0.866218511303148,-6.7135999988006,20.2378632243457));
#13700=CARTESIAN_POINT('Ctrl Pts',(1.0387077508507,-6.68680605433735,20.2460620641735));
#13701=CARTESIAN_POINT('Ctrl Pts',(1.21137716031634,-6.65998412283682,20.2542694679227));
#13702=CARTESIAN_POINT('Ctrl Pts',(1.38291266565133,-6.62648445604016,20.262476871672));
#13703=CARTESIAN_POINT('Ctrl Pts',(1.55276896648187,-6.58644042990832,20.2706842754212));
#13704=CARTESIAN_POINT('Ctrl Pts',(1.72271625133604,-6.54637495407692,20.2788960754902));
#13705=CARTESIAN_POINT('Ctrl Pts',(1.89098219308985,-6.49975822630718,20.2871078755593));
#13706=CARTESIAN_POINT('Ctrl Pts',(2.0570371872062,-6.44677337979635,20.2953196756283));
#13707=CARTESIAN_POINT('Ctrl Pts',(2.22333663747637,-6.393710532188,20.3035435646145));
#13708=CARTESIAN_POINT('Ctrl Pts',(2.38741829806059,-6.33426095287712,20.3117674536006));
#13709=CARTESIAN_POINT('Ctrl Pts',(2.54877185531134,-6.26865623794867,20.3199913425867));
#13710=CARTESIAN_POINT('Ctrl Pts',(2.69785975275912,-6.20803861551756,20.3275900738368));
#13711=CARTESIAN_POINT('Ctrl Pts',(2.84461859164236,-6.1421667003386,20.3351888050869));
#13712=CARTESIAN_POINT('Ctrl Pts',(2.98866572065,-6.07125738296538,20.3427875363369));
#13713=CARTESIAN_POINT('Ctrl Pts',(3.14458198460576,-5.99450530938605,20.3510123846589));
#13714=CARTESIAN_POINT('Ctrl Pts',(3.29775856464863,-5.91163551488225,20.359237232981));
#13715=CARTESIAN_POINT('Ctrl Pts',(3.44768222515461,-5.82286667152469,20.367462081303));
#13716=CARTESIAN_POINT('Ctrl Pts',(3.59743703837766,-5.73419780156664,20.3756776666222));
#13717=CARTESIAN_POINT('Ctrl Pts',(3.74394592114233,-5.63964329305354,20.3838932519414));
#13718=CARTESIAN_POINT('Ctrl Pts',(3.88671728283139,-5.53946908677536,20.3921088372606));
#13719=CARTESIAN_POINT('Ctrl Pts',(4.0293565379205,-5.43938757187195,20.4003168206838));
#13720=CARTESIAN_POINT('Ctrl Pts',(4.16826486743913,-5.33369691971145,20.408524804107));
#13721=CARTESIAN_POINT('Ctrl Pts',(4.30297681881327,-5.22270806160517,20.4167327875303));
#13722=CARTESIAN_POINT('Ctrl Pts',(4.4375911785558,-5.11179960901334,20.4249348247068));
#13723=CARTESIAN_POINT('Ctrl Pts',(4.56801493959037,-4.99560082279134,20.4331368618833));
#13724=CARTESIAN_POINT('Ctrl Pts',(4.69381303428616,-4.87446491413831,20.4413388990598));
#13725=CARTESIAN_POINT('Ctrl Pts',(4.819545256338,-4.75339243683215,20.4495366413392));
#13726=CARTESIAN_POINT('Ctrl Pts',(4.94065637958802,-4.62738823562199,20.4577343836186));
#13727=CARTESIAN_POINT('Ctrl Pts',(5.05674568048418,-4.49684468521035,20.465932125898));
#13728=CARTESIAN_POINT('Ctrl Pts',(5.1728129089207,-4.36632595549472,20.4741283095124));
#13729=CARTESIAN_POINT('Ctrl Pts',(5.28385997404797,-4.23126985941285,20.4823244931267));
#13730=CARTESIAN_POINT('Ctrl Pts',(5.38952398716172,-4.09210461643008,20.4905206767411));
#13731=CARTESIAN_POINT('Ctrl Pts',(5.49518022192991,-3.95294961795082,20.4987162570019));
#13732=CARTESIAN_POINT('Ctrl Pts',(5.59545397616269,-3.8096863602303,20.5069118372628));
#13733=CARTESIAN_POINT('Ctrl Pts',(5.69002358507626,-3.662774986438,20.5151074175237));
#13734=CARTESIAN_POINT('Ctrl Pts',(5.78460343816883,-3.51584769858592,20.5233038855644));
#13735=CARTESIAN_POINT('Ctrl Pts',(5.87347772063902,-3.36527180912787,20.5315003536051));
#13736=CARTESIAN_POINT('Ctrl Pts',(5.95636890063675,-3.21153522781977,20.5396968216459));
#13737=CARTESIAN_POINT('Ctrl Pts',(6.03928414089027,-3.05775402244587,20.5478956688193));
#13738=CARTESIAN_POINT('Ctrl Pts',(6.11621264918396,-2.90081061357969,20.5560945159927));
#13739=CARTESIAN_POINT('Ctrl Pts',(6.18692350580496,-2.74121625073945,20.5642933631661));
#13740=CARTESIAN_POINT('Ctrl Pts',(6.25770826214694,-2.58145509627134,20.5725007789321));
#13741=CARTESIAN_POINT('Ctrl Pts',(6.32226223900874,-2.41903778123316,20.5807081946981));
#13742=CARTESIAN_POINT('Ctrl Pts',(6.38040285408827,-2.25449515846503,20.588915610464));
#13743=CARTESIAN_POINT('Ctrl Pts',(6.43857463049258,-2.08986434663835,20.5971274251162));
#13744=CARTESIAN_POINT('Ctrl Pts',(6.49032608644602,-1.92310629865883,20.6053392397683));
#13745=CARTESIAN_POINT('Ctrl Pts',(6.53552498470891,-1.75476556104959,20.6135510544205));
#13746=CARTESIAN_POINT('Ctrl Pts',(6.5807904452208,-1.58617691611236,20.6217749622181));
#13747=CARTESIAN_POINT('Ctrl Pts',(6.61948398395507,-1.4160012735088,20.6299988700157));
#13748=CARTESIAN_POINT('Ctrl Pts',(6.65152456319241,-1.24479314958272,20.6382227778133));
#13749=CARTESIAN_POINT('Ctrl Pts',(6.68112946667294,-1.08660000499665,20.6458215167368));
#13750=CARTESIAN_POINT('Ctrl Pts',(6.70505500320042,-0.927525685242328,
20.6534202556602));
#13751=CARTESIAN_POINT('Ctrl Pts',(6.72327677779544,-0.76800935486266,20.6610189945837));
#13752=CARTESIAN_POINT('Ctrl Pts',(6.74282283160828,-0.596900072318996,
20.669169976758));
#13753=CARTESIAN_POINT('Ctrl Pts',(6.7558631551989,-0.424775329034652,20.6773209589323));
#13754=CARTESIAN_POINT('Ctrl Pts',(6.76229963874382,-0.252175724139254,
20.6854719411065));
#13755=CARTESIAN_POINT('Ctrl Pts',(6.76872864571657,-0.0797766096819023,
20.6936134551596));
#13756=CARTESIAN_POINT('Ctrl Pts',(6.76856906881038,0.0930959066924904,
20.7017549692126));
#13757=CARTESIAN_POINT('Ctrl Pts',(6.76177415979962,0.265893233960796,20.7098964832656));
#13758=CARTESIAN_POINT('Ctrl Pts',(6.75498571380733,0.438526204014682,20.7180302534687));
#13759=CARTESIAN_POINT('Ctrl Pts',(6.7415745147216,0.61108376443959,20.7261640236718));
#13760=CARTESIAN_POINT('Ctrl Pts',(6.72154575992354,0.783014429786534,20.7342977938749));
#13761=CARTESIAN_POINT('Ctrl Pts',(6.70153184313653,0.954817722806097,20.7424255382929));
#13762=CARTESIAN_POINT('Ctrl Pts',(6.67491017445478,1.12599468377619,20.7505532827109));
#13763=CARTESIAN_POINT('Ctrl Pts',(6.641737965366,1.29599606458348,20.7586810271289));
#13764=CARTESIAN_POINT('Ctrl Pts',(6.60858335721769,1.46590724385568,20.766804459023));
#13765=CARTESIAN_POINT('Ctrl Pts',(6.56888520041666,1.63464372704615,20.774927890917));
#13766=CARTESIAN_POINT('Ctrl Pts',(6.52275227273907,1.80166361690447,20.7830513228111));
#13767=CARTESIAN_POINT('Ctrl Pts',(6.47632669591376,1.9697430152501,20.7912262865619));
#13768=CARTESIAN_POINT('Ctrl Pts',(6.42338447627585,2.13608359423184,20.7994012503127));
#13769=CARTESIAN_POINT('Ctrl Pts',(6.36408837673153,2.3001452417512,20.8075762140636));
#13770=CARTESIAN_POINT('Ctrl Pts',(6.30517942315793,2.46313572596849,20.8156978032366));
#13771=CARTESIAN_POINT('Ctrl Pts',(6.23999946279605,2.62387660952087,20.8238193924096));
#13772=CARTESIAN_POINT('Ctrl Pts',(6.16875747958513,2.78185552429715,20.8319409815827));
#13773=CARTESIAN_POINT('Ctrl Pts',(6.0975060909713,2.93985529553022,20.840063642972));
#13774=CARTESIAN_POINT('Ctrl Pts',(6.02019123589836,3.09509203803165,20.8481863043614));
#13775=CARTESIAN_POINT('Ctrl Pts',(5.937069142705,3.24707545257885,20.8563089657508));
#13776=CARTESIAN_POINT('Ctrl Pts',(5.85392024678543,3.39910787419136,20.864434246293));
#13777=CARTESIAN_POINT('Ctrl Pts',(5.76496055945822,3.54788455796296,20.8725595268353));
#13778=CARTESIAN_POINT('Ctrl Pts',(5.67049112359437,3.69294183778156,20.8806848073775));
#13779=CARTESIAN_POINT('Ctrl Pts',(5.57499246282927,3.8395794865643,20.8888986111653));
#13780=CARTESIAN_POINT('Ctrl Pts',(5.47386350464339,3.98241589044244,20.897112414953));
#13781=CARTESIAN_POINT('Ctrl Pts',(5.36745822332432,4.12100487998597,20.9053262187408));
#13782=CARTESIAN_POINT('Ctrl Pts',(5.26201756807798,4.25833747932921,20.913465559596));
#13783=CARTESIAN_POINT('Ctrl Pts',(5.15139614488266,4.39149911872647,20.9216049004511));
#13784=CARTESIAN_POINT('Ctrl Pts',(5.03597652983962,4.52009174585036,20.9297442413063));
#13785=CARTESIAN_POINT('Ctrl Pts',(4.91897303659917,4.65044902154262,20.9379952765603));
#13786=CARTESIAN_POINT('Ctrl Pts',(4.79703898083779,4.77611069478899,20.9462463118144));
#13787=CARTESIAN_POINT('Ctrl Pts',(4.67060837656458,4.89670362517121,20.9544973470684));
#13788=CARTESIAN_POINT('Ctrl Pts',(4.54417777229138,5.0172965555534,20.9627483823225));
#13789=CARTESIAN_POINT('Ctrl Pts',(4.41325095172409,5.13282053937636,20.9709994175765));
#13790=CARTESIAN_POINT('Ctrl Pts',(4.2782928526313,5.24294757432533,20.9792504528306));
#13791=CARTESIAN_POINT('Ctrl Pts',(4.14363336315362,5.35283094111553,20.987483231763));
#13792=CARTESIAN_POINT('Ctrl Pts',(4.00454009237542,5.45768443132887,20.9957160106954));
#13793=CARTESIAN_POINT('Ctrl Pts',(3.86142383748823,5.55713009990568,21.0039487896279));
#13794=CARTESIAN_POINT('Ctrl Pts',(3.71850616935632,5.65643777861778,21.0121701448345));
#13795=CARTESIAN_POINT('Ctrl Pts',(3.57157692998338,5.75035238284981,21.0203915000411));
#13796=CARTESIAN_POINT('Ctrl Pts',(3.42108087175425,5.83853531880361,21.0286128552477));
#13797=CARTESIAN_POINT('Ctrl Pts',(3.31548021184615,5.90041186453465,21.0343816477688));
#13798=CARTESIAN_POINT('Ctrl Pts',(3.20812414316205,5.95946715018402,21.0401504402898));
#13799=CARTESIAN_POINT('Ctrl Pts',(3.09917575053256,6.01559628526641,21.0459192328109));
#13800=CARTESIAN_POINT('Ctrl Pts',(3.09917575053257,6.0155962852664,19.0456175016683));
#13801=CARTESIAN_POINT('Ctrl Pts',(2.94686581755147,6.09406485737061,19.0536989022288));
#13802=CARTESIAN_POINT('Ctrl Pts',(2.79173928855776,6.16666014621092,19.0617803027892));
#13803=CARTESIAN_POINT('Ctrl Pts',(2.63429393795789,6.23320017715125,19.0698617033497));
#13804=CARTESIAN_POINT('Ctrl Pts',(2.46585430923732,6.30438664321037,19.0785074214021));
#13805=CARTESIAN_POINT('Ctrl Pts',(2.29437685241815,6.36880518518817,19.0871531394545));
#13806=CARTESIAN_POINT('Ctrl Pts',(2.12042019058826,6.42620472871396,19.0957988575068));
#13807=CARTESIAN_POINT('Ctrl Pts',(1.94668685366066,6.4835305829236,19.1044334762192));
#13808=CARTESIAN_POINT('Ctrl Pts',(1.77048094661389,6.53385531190139,19.1130680949316));
#13809=CARTESIAN_POINT('Ctrl Pts',(1.59238088160172,6.57697591054653,19.1217027136439));
#13810=CARTESIAN_POINT('Ctrl Pts',(1.40799101415761,6.62161936122547,19.1306422735464));
#13811=CARTESIAN_POINT('Ctrl Pts',(1.22157104283931,6.65854039925769,19.1395818334488));
#13812=CARTESIAN_POINT('Ctrl Pts',(1.03378289244469,6.68756920945785,19.1485213933512));
#13813=CARTESIAN_POINT('Ctrl Pts',(0.852903892918512,6.71552998406161,19.1571320466217));
#13814=CARTESIAN_POINT('Ctrl Pts',(0.67075593199652,6.73616881881119,19.1657426998922));
#13815=CARTESIAN_POINT('Ctrl Pts',(0.487943993382733,6.74938513194511,19.1743533531627));
#13816=CARTESIAN_POINT('Ctrl Pts',(0.305305098499116,6.76258893495447,19.1829558558738));
#13817=CARTESIAN_POINT('Ctrl Pts',(0.122003782177149,6.76838420221161,19.1915583585849));
#13818=CARTESIAN_POINT('Ctrl Pts',(-0.0613479792059813,6.76672191134284,
19.2001608612961));
#13819=CARTESIAN_POINT('Ctrl Pts',(-0.244493381872622,6.76506149134899,
19.2087536820635));
#13820=CARTESIAN_POINT('Ctrl Pts',(-0.427688812005436,6.7559602604347,19.217346502831));
#13821=CARTESIAN_POINT('Ctrl Pts',(-0.610320190322639,6.73942121144572,
19.2259393235985));
#13822=CARTESIAN_POINT('Ctrl Pts',(-0.63184412781484,6.73747200939787,19.2269520265567));
#13823=CARTESIAN_POINT('Ctrl Pts',(-0.653360229137335,6.73541955783007,
19.2279647295149));
#13824=CARTESIAN_POINT('Ctrl Pts',(-0.67486748832631,6.73326390936819,19.2289774324731));
#13825=CARTESIAN_POINT('Ctrl Pts',(-0.857409106226856,6.71496796777942,
19.2375726902332));
#13826=CARTESIAN_POINT('Ctrl Pts',(-1.03909871287128,6.68925533611982,19.2461679479932));
#13827=CARTESIAN_POINT('Ctrl Pts',(-1.21933193254209,6.65623907610621,19.2547632057533));
#13828=CARTESIAN_POINT('Ctrl Pts',(-1.39973393297972,6.62319189776526,19.2633665126077));
#13829=CARTESIAN_POINT('Ctrl Pts',(-1.57867652380709,6.58282749410883,19.2719698194621));
#13830=CARTESIAN_POINT('Ctrl Pts',(-1.75556754650928,6.53530960166719,19.2805731263166));
#13831=CARTESIAN_POINT('Ctrl Pts',(-1.93979253235329,6.48582160092713,19.2895331292566));
#13832=CARTESIAN_POINT('Ctrl Pts',(-2.12179184305956,6.42857441130441,19.2984931321966));
#13833=CARTESIAN_POINT('Ctrl Pts',(-2.30091763490059,6.3638091609824,19.3074531351366));
#13834=CARTESIAN_POINT('Ctrl Pts',(-2.47338299350447,6.3014520765723,19.3160799783413));
#13835=CARTESIAN_POINT('Ctrl Pts',(-2.64318441557393,6.23212609278477,19.324706821546));
#13836=CARTESIAN_POINT('Ctrl Pts',(-2.8097667941681,6.15609450564157,19.3333336647508));
#13837=CARTESIAN_POINT('Ctrl Pts',(-2.97650838340709,6.07999025152052,19.3419687530369));
#13838=CARTESIAN_POINT('Ctrl Pts',(-3.14002451471794,5.99716773639052,19.350603841323));
#13839=CARTESIAN_POINT('Ctrl Pts',(-3.29978523525656,5.90793588329992,19.3592389296092));
#13840=CARTESIAN_POINT('Ctrl Pts',(-3.45978323252651,5.81857150300013,19.3678868427343));
#13841=CARTESIAN_POINT('Ctrl Pts',(-3.61601441093366,5.72277891785642,19.3765347558595));
#13842=CARTESIAN_POINT('Ctrl Pts',(-3.76797705164576,5.62091077480073,19.3851826689846));
#13843=CARTESIAN_POINT('Ctrl Pts',(-3.78502494657996,5.60948271990633,19.3861528331886));
#13844=CARTESIAN_POINT('Ctrl Pts',(-3.80201915402101,5.59797824357036,19.3871229973926));
#13845=CARTESIAN_POINT('Ctrl Pts',(-3.81895899163695,5.58639787521398,19.3880931615965));
#13846=CARTESIAN_POINT('Ctrl Pts',(-3.96180337141138,5.48874696657306,19.3962740253766));
#13847=CARTESIAN_POINT('Ctrl Pts',(-4.10109921560093,5.38547745589563,19.4044548891568));
#13848=CARTESIAN_POINT('Ctrl Pts',(-4.23637342288947,5.27687684353499,19.4126357529369));
#13849=CARTESIAN_POINT('Ctrl Pts',(-4.37150439222093,5.16839122523096,19.4208079542363));
#13850=CARTESIAN_POINT('Ctrl Pts',(-4.50262192258611,5.05458596943124,19.4289801555357));
#13851=CARTESIAN_POINT('Ctrl Pts',(-4.62928112906176,4.93579225941619,19.4371523568351));
#13852=CARTESIAN_POINT('Ctrl Pts',(-4.75583236725597,4.8170998128866,19.4453175918937));
#13853=CARTESIAN_POINT('Ctrl Pts',(-4.8779325861,4.6934276263923,19.4534828269523));
#13854=CARTESIAN_POINT('Ctrl Pts',(-4.99516927669712,4.56514763147274,19.4616480620109));
#13855=CARTESIAN_POINT('Ctrl Pts',(-5.11233022516387,4.43695051333902,19.4698080218243));
#13856=CARTESIAN_POINT('Ctrl Pts',(-5.22463365932423,4.30415178243408,19.4779679816376));
#13857=CARTESIAN_POINT('Ctrl Pts',(-5.33170329322226,4.16716078320035,19.4861279414509));
#13858=CARTESIAN_POINT('Ctrl Pts',(-5.43872584437381,4.03023002431911,19.4942843130077));
#13859=CARTESIAN_POINT('Ctrl Pts',(-5.54051895685914,3.88911095464416,19.5024406845644));
#13860=CARTESIAN_POINT('Ctrl Pts',(-5.63674606322884,3.74424662898616,19.5105970561212));
#13861=CARTESIAN_POINT('Ctrl Pts',(-5.732967112403,3.59939142208462,19.5187529142598));
#13862=CARTESIAN_POINT('Ctrl Pts',(-5.82362264514526,3.45079172577715,19.5269087723985));
#13863=CARTESIAN_POINT('Ctrl Pts',(-5.90841877517819,3.29892051694518,19.5350646305372));
#13864=CARTESIAN_POINT('Ctrl Pts',(-5.99321614319239,3.14704709086921,19.5432206077473));
#13865=CARTESIAN_POINT('Ctrl Pts',(-6.07215376042459,2.99190237360781,19.5513765849574));
#13866=CARTESIAN_POINT('Ctrl Pts',(-6.14498326134584,2.83398477726672,19.5595325621675));
#13867=CARTESIAN_POINT('Ctrl Pts',(-6.21782743848746,2.67603535819696,19.5676901829276));
#13868=CARTESIAN_POINT('Ctrl Pts',(-6.28456089576236,2.51531227665795,19.5758478036876));
#13869=CARTESIAN_POINT('Ctrl Pts',(-6.34498306284489,2.35233478319125,19.5840054244476));
#13870=CARTESIAN_POINT('Ctrl Pts',(-6.40542870009563,2.18929398333603,19.5921662139243));
#13871=CARTESIAN_POINT('Ctrl Pts',(-6.4595580387042,2.02399736752226,19.6003270034011));
#13872=CARTESIAN_POINT('Ctrl Pts',(-6.5072201019049,1.85698022212537,19.6084877928778));
#13873=CARTESIAN_POINT('Ctrl Pts',(-6.55493670145495,1.68977197074656,19.6166579201725));
#13874=CARTESIAN_POINT('Ctrl Pts',(-6.59617114600952,1.52083960689443,19.6248280474671));
#13875=CARTESIAN_POINT('Ctrl Pts',(-6.63082319994865,1.35073042870248,19.6329981747617));
#13876=CARTESIAN_POINT('Ctrl Pts',(-6.66549711024586,1.18051395623243,19.6411734552639));
#13877=CARTESIAN_POINT('Ctrl Pts',(-6.69358029800513,1.0091195473852,19.6493487357661));
#13878=CARTESIAN_POINT('Ctrl Pts',(-6.7150243541446,0.837100306561233,19.6575240162684));
#13879=CARTESIAN_POINT('Ctrl Pts',(-6.73649992711584,0.664828245028345,
19.6657113121719));
#13880=CARTESIAN_POINT('Ctrl Pts',(-6.75131684692723,0.491929877684113,
19.6738986080754));
#13881=CARTESIAN_POINT('Ctrl Pts',(-6.75947878720754,0.31896006849034,19.682085903979));
#13882=CARTESIAN_POINT('Ctrl Pts',(-6.76449449881954,0.212665896920379,
19.6871171972406));
#13883=CARTESIAN_POINT('Ctrl Pts',(-6.76699804858992,0.106344709920844,
19.6921484905023));
#13884=CARTESIAN_POINT('Ctrl Pts',(-6.76699999885939,0.000124246054141125,
19.6971797837639));
#13885=CARTESIAN_POINT('',(-6.76699834151218,-0.0027926855951009,19.3028202161899));
#13886=CARTESIAN_POINT('Ctrl Pts',(3.0991757505326,6.01559628526638,18.6513920151221));
#13887=CARTESIAN_POINT('Ctrl Pts',(2.93382384459268,6.10078395293758,18.6601414630345));
#13888=CARTESIAN_POINT('Ctrl Pts',(2.76495772122988,6.17915010267047,18.6688909109469));
#13889=CARTESIAN_POINT('Ctrl Pts',(2.59315093316717,6.25042856433175,18.6776403588593));
#13890=CARTESIAN_POINT('Ctrl Pts',(2.4213455324562,6.3217064504145,18.6863897361193));
#13891=CARTESIAN_POINT('Ctrl Pts',(2.24659977927591,6.38589665313457,18.6951391133793));
#13892=CARTESIAN_POINT('Ctrl Pts',(2.06950718689916,6.44278115439076,18.7038884906393));
#13893=CARTESIAN_POINT('Ctrl Pts',(1.89241596572865,6.49966521519723,18.712637800154));
#13894=CARTESIAN_POINT('Ctrl Pts',(1.71297821457207,6.54924360009543,18.7213871096686));
#13895=CARTESIAN_POINT('Ctrl Pts',(1.53180337335861,6.59134792173552,18.7301364191833));
#13896=CARTESIAN_POINT('Ctrl Pts',(1.35062987477793,6.63345193135303,18.7388856638594));
#13897=CARTESIAN_POINT('Ctrl Pts',(1.16771959102957,6.66808192368237,18.7476349085355));
#13898=CARTESIAN_POINT('Ctrl Pts',(0.98369374690684,6.69512028363168,18.7563841532117));
#13899=CARTESIAN_POINT('Ctrl Pts',(0.799669205419867,6.72215845218867,18.7651333359558));
#13900=CARTESIAN_POINT('Ctrl Pts',(0.614529402873472,6.74160505424579,18.7738825187));
#13901=CARTESIAN_POINT('Ctrl Pts',(0.428903127363245,6.75339404354122,18.7826317014442));
#13902=CARTESIAN_POINT('Ctrl Pts',(0.243278104163867,6.7651829533033,18.7913808251628));
#13903=CARTESIAN_POINT('Ctrl Pts',(0.0571669005390976,6.76931433552276,
18.8001299488814));
#13904=CARTESIAN_POINT('Ctrl Pts',(-0.128798404777541,6.76577415902473,
18.8088790726));
#13905=CARTESIAN_POINT('Ctrl Pts',(-0.314762517259088,6.76223400523441,
18.8176281401992));
#13906=CARTESIAN_POINT('Ctrl Pts',(-0.500580446819462,6.75102239665089,
18.8263772077984));
#13907=CARTESIAN_POINT('Ctrl Pts',(-0.685621118842526,6.73217741012498,
18.8351262753976));
#13908=CARTESIAN_POINT('Ctrl Pts',(-0.870660665414259,6.71333253821774,
18.8438752897834));
#13909=CARTESIAN_POINT('Ctrl Pts',(-1.05492267885449,6.68685441030618,18.8526243041692));
#13910=CARTESIAN_POINT('Ctrl Pts',(-1.23778137635201,6.65283295028187,18.8613733185549));
#13911=CARTESIAN_POINT('Ctrl Pts',(-1.429999229788,6.61707018861876,18.8705701289223));
#13912=CARTESIAN_POINT('Ctrl Pts',(-1.62066601233652,6.57297172934424,18.8797669392897));
#13913=CARTESIAN_POINT('Ctrl Pts',(-1.80906628500346,6.52070304311305,18.8889637496571));
#13914=CARTESIAN_POINT('Ctrl Pts',(-1.98831342545488,6.47097374915043,18.8977137473949));
#13915=CARTESIAN_POINT('Ctrl Pts',(-2.16550875896663,6.41384933989542,18.9064637451327));
#13916=CARTESIAN_POINT('Ctrl Pts',(-2.34005036713972,6.3495238624049,18.9152137428704));
#13917=CARTESIAN_POINT('Ctrl Pts',(-2.51458843547052,6.28519968948611,18.9239635631513));
#13918=CARTESIAN_POINT('Ctrl Pts',(-2.6864726171802,6.21367483971114,18.9327133834321));
#13919=CARTESIAN_POINT('Ctrl Pts',(-2.85511905908698,6.13519226743859,18.941463203713));
#13920=CARTESIAN_POINT('Ctrl Pts',(-3.02376230488862,6.05671118252948,18.9502128581716));
#13921=CARTESIAN_POINT('Ctrl Pts',(-3.18916767379893,5.97127275992639,18.9589625126301));
#13922=CARTESIAN_POINT('Ctrl Pts',(-3.35077334102786,5.87916720437997,18.9677121670886));
#13923=CARTESIAN_POINT('Ctrl Pts',(-3.51237616037372,5.78706327195641,18.9764616673571));
#13924=CARTESIAN_POINT('Ctrl Pts',(-3.67017916302308,5.68829258362293,18.9852111676255));
#13925=CARTESIAN_POINT('Ctrl Pts',(-3.82364636566475,5.58319061741033,18.993960667894));
#13926=CARTESIAN_POINT('Ctrl Pts',(-3.97711106778813,5.47809036367691,19.0027100256024));
#13927=CARTESIAN_POINT('Ctrl Pts',(-4.12623987481945,5.36665920043212,19.0114593833108));
#13928=CARTESIAN_POINT('Ctrl Pts',(-4.27052628213949,5.24927559512319,19.0202087410193));
#13929=CARTESIAN_POINT('Ctrl Pts',(-4.41481053024993,5.13189374643023,19.0289579677958));
#13930=CARTESIAN_POINT('Ctrl Pts',(-4.55425230136541,5.00855981477343,19.0377071945723));
#13931=CARTESIAN_POINT('Ctrl Pts',(-4.68837800630554,4.87969268192071,19.0464564213488));
#13932=CARTESIAN_POINT('Ctrl Pts',(-4.82250188228897,4.75082730631807,19.0552055288197));
#13933=CARTESIAN_POINT('Ctrl Pts',(-4.95130963052964,4.61642907903527,19.0639546362905));
#13934=CARTESIAN_POINT('Ctrl Pts',(-5.07436379033362,4.47695444731695,19.0727037437614));
#13935=CARTESIAN_POINT('Ctrl Pts',(-5.19741643562807,4.33748153220584,19.0814527435511));
#13936=CARTESIAN_POINT('Ctrl Pts',(-5.31471544462781,4.19293255254579,19.0902017433409));
#13937=CARTESIAN_POINT('Ctrl Pts',(-5.42586245275641,4.04379841779585,19.0989507431306));
#13938=CARTESIAN_POINT('Ctrl Pts',(-5.53702160019161,3.89464799484331,19.1077006984728));
#13939=CARTESIAN_POINT('Ctrl Pts',(-5.64202723081255,3.74091164443845,19.1164506538149));
#13940=CARTESIAN_POINT('Ctrl Pts',(-5.74052265232966,3.58311159163235,19.1252006091571));
#13941=CARTESIAN_POINT('Ctrl Pts',(-5.83901427066916,3.42531763191787,19.1339502266395));
#13942=CARTESIAN_POINT('Ctrl Pts',(-5.93099603115737,3.26346052695618,19.142699844122));
#13943=CARTESIAN_POINT('Ctrl Pts',(-6.0161555062275,3.09809004467083,19.1514494616044));
#13944=CARTESIAN_POINT('Ctrl Pts',(-6.10131214578803,2.9327250686382,19.1601987877555));
#13945=CARTESIAN_POINT('Ctrl Pts',(-6.17964682328758,2.76384720416873,19.1689481139066));
#13946=CARTESIAN_POINT('Ctrl Pts',(-6.25089348288579,2.59203002791557,19.1776974400577));
#13947=CARTESIAN_POINT('Ctrl Pts',(-6.32213814889351,2.42021765936975,19.1864465213893));
#13948=CARTESIAN_POINT('Ctrl Pts',(-6.38629508412611,2.24546640831846,19.1951956027209));
#13949=CARTESIAN_POINT('Ctrl Pts',(-6.44314639819841,2.06836976659952,19.2039446840524));
#13950=CARTESIAN_POINT('Ctrl Pts',(-6.50000285283728,1.8912571115818,19.2126945564868));
#13951=CARTESIAN_POINT('Ctrl Pts',(-6.54955227673276,1.71179891440153,19.2214444289212));
#13952=CARTESIAN_POINT('Ctrl Pts',(-6.5916263592641,1.53060476278324,19.2301943013556));
#13953=CARTESIAN_POINT('Ctrl Pts',(-6.63369752055216,1.34942319164596,19.2389435662781));
#13954=CARTESIAN_POINT('Ctrl Pts',(-6.6682943142427,1.16650618642613,19.2476928312006));
#13955=CARTESIAN_POINT('Ctrl Pts',(-6.69529923745429,0.982474997617727,
19.2564420961231));
#13956=CARTESIAN_POINT('Ctrl Pts',(-6.72230554731454,0.798434359176876,
19.2651918103028));
#13957=CARTESIAN_POINT('Ctrl Pts',(-6.74171916496711,0.61327970623944,19.2739415244825));
#13958=CARTESIAN_POINT('Ctrl Pts',(-6.75347414817281,0.427639953654448,
19.2826912386622));
#13959=CARTESIAN_POINT('Ctrl Pts',(-6.76248837758747,0.285283364197852,
19.2894008978381));
#13960=CARTESIAN_POINT('Ctrl Pts',(-6.76699999999997,0.142641701104605,
19.296110557014));
#13961=CARTESIAN_POINT('Ctrl Pts',(-6.767,1.26781560333738E-12,19.3028202161899));
#13962=CARTESIAN_POINT('Ctrl Pts',(-6.76699522683441,-0.00803741253624945,
19.3028202161899));
#13963=CARTESIAN_POINT('Ctrl Pts',(-6.76673659893204,-0.225785820121706,
19.313053212668));
#13964=CARTESIAN_POINT('Ctrl Pts',(-6.75596462743227,-0.443030194641021,
19.3232862091462));
#13965=CARTESIAN_POINT('Ctrl Pts',(-6.73484541930834,-0.658897699207909,
19.3335192056243));
#13966=CARTESIAN_POINT('Ctrl Pts',(-6.71331152130556,-0.87900390765003,
19.3439531338819));
#13967=CARTESIAN_POINT('Ctrl Pts',(-6.68102007315153,-1.09767877436092,
19.3543870621396));
#13968=CARTESIAN_POINT('Ctrl Pts',(-6.63819493462871,-1.31402321511825,
19.3648209903972));
#13969=CARTESIAN_POINT('Ctrl Pts',(-6.60923076601765,-1.4603446766781,19.3718778282208));
#13970=CARTESIAN_POINT('Ctrl Pts',(-6.57544915666674,-1.60560067636746,
19.3789346660444));
#13971=CARTESIAN_POINT('Ctrl Pts',(-6.53693137322275,-1.74951914015714,
19.385991503868));
#13972=CARTESIAN_POINT('Ctrl Pts',(-6.49199356254967,-1.91742549664685,
19.3942245540001));
#13973=CARTESIAN_POINT('Ctrl Pts',(-6.44051669011873,-2.08384480851689,
19.4024576041321));
#13974=CARTESIAN_POINT('Ctrl Pts',(-6.38261306167999,-2.24823030512268,
19.4106906542641));
#13975=CARTESIAN_POINT('Ctrl Pts',(-6.32477838756202,-2.41242004387065,
19.4189139000989));
#13976=CARTESIAN_POINT('Ctrl Pts',(-6.26053231483941,-2.57458045555605,
19.4271371459338));
#13977=CARTESIAN_POINT('Ctrl Pts',(-6.19003777798889,-2.73417653180447,
19.4353603917686));
#13978=CARTESIAN_POINT('Ctrl Pts',(-6.11961307966196,-2.89361449715761,
19.4435754908821));
#13979=CARTESIAN_POINT('Ctrl Pts',(-6.04295238902611,-3.05049286106434,
19.4517905899957));
#13980=CARTESIAN_POINT('Ctrl Pts',(-5.960267938881,-3.20429322889577,19.4600056891092));
#13981=CARTESIAN_POINT('Ctrl Pts',(-5.87764886024245,-3.35797199996097,
19.468214293248));
#13982=CARTESIAN_POINT('Ctrl Pts',(-5.78901567682439,-3.50857730794951,
19.4764228973869));
#13983=CARTESIAN_POINT('Ctrl Pts',(-5.69462811767156,-3.65561206932909,
19.4846315015258));
#13984=CARTESIAN_POINT('Ctrl Pts',(-5.60029630252679,-3.80255999397937,
19.4928352577748));
#13985=CARTESIAN_POINT('Ctrl Pts',(-5.50021707480888,-3.94594127225762,
19.5010390140238));
#13986=CARTESIAN_POINT('Ctrl Pts',(-5.39469540380842,-4.0852846290226,19.5092427702727));
#13987=CARTESIAN_POINT('Ctrl Pts',(-5.28920495401075,-4.22458675760044,
19.517444099237));
#13988=CARTESIAN_POINT('Ctrl Pts',(-5.17827548143832,-4.35985305698951,
19.5256454282013));
#13989=CARTESIAN_POINT('Ctrl Pts',(-5.06225460862956,-4.49064218986648,
19.5338467571656));
#13990=CARTESIAN_POINT('Ctrl Pts',(-4.9462497362068,-4.62141328567339,19.5420469550883));
#13991=CARTESIAN_POINT('Ctrl Pts',(-4.82515509906916,-4.74770817623819,
19.550247153011));
#13992=CARTESIAN_POINT('Ctrl Pts',(-4.69935785601289,-4.86911950368134,
19.5584473509337));
#13993=CARTESIAN_POINT('Ctrl Pts',(-4.57355516457748,-4.9905360895461,19.5666479040135));
#13994=CARTESIAN_POINT('Ctrl Pts',(-4.4430497192283,-5.10706844203911,19.5748484570934));
#13995=CARTESIAN_POINT('Ctrl Pts',(-4.30826473397986,-5.21834686293902,
19.5830490101732));
#13996=CARTESIAN_POINT('Ctrl Pts',(-4.17344948540597,-5.32965026922629,
19.5912514045264));
#13997=CARTESIAN_POINT('Ctrl Pts',(-4.03435305935044,-5.43569716629838,
19.5994537988797));
#13998=CARTESIAN_POINT('Ctrl Pts',(-3.89143089432966,-5.53615883033143,
19.6076561932329));
#13999=CARTESIAN_POINT('Ctrl Pts',(-3.7483750719605,-5.63671444368036,19.6158662582667));
#14000=CARTESIAN_POINT('Ctrl Pts',(-3.60148665609892,-5.7316741822211,19.6240763233006));
#14001=CARTESIAN_POINT('Ctrl Pts',(-3.45124994273824,-5.82075277200031,
19.6322863883344));
#14002=CARTESIAN_POINT('Ctrl Pts',(-3.30094132875186,-5.90987399321227,
19.6405003825597));
#14003=CARTESIAN_POINT('Ctrl Pts',(-3.14728153713205,-5.99310828323021,
19.648714376785));
#14004=CARTESIAN_POINT('Ctrl Pts',(-2.99077841709905,-6.0702169203262,19.6569283710103));
#14005=CARTESIAN_POINT('Ctrl Pts',(-2.83406193118852,-6.14743068217635,
19.6651535636455));
#14006=CARTESIAN_POINT('Ctrl Pts',(-2.67449469719987,-6.2185019550956,19.6733787562807));
#14007=CARTESIAN_POINT('Ctrl Pts',(-2.51260457361605,-6.2832401877251,19.6816039489159));
#14008=CARTESIAN_POINT('Ctrl Pts',(-2.36701713221715,-6.34145914167096,
19.6890008470358));
#14009=CARTESIAN_POINT('Ctrl Pts',(-2.21955149458719,-6.39455693454562,
19.6963977451558));
#14010=CARTESIAN_POINT('Ctrl Pts',(-2.07060046963125,-6.44242987506755,
19.7037946432757));
#14011=CARTESIAN_POINT('Ctrl Pts',(-1.89649700765637,-6.49838682254241,
19.7124406097666));
#14012=CARTESIAN_POINT('Ctrl Pts',(-1.71996884025011,-6.54733190881197,
19.7210865762575));
#14013=CARTESIAN_POINT('Ctrl Pts',(-1.54159478382049,-6.58906476842484,
19.7297325427484));
#14014=CARTESIAN_POINT('Ctrl Pts',(-1.36344889205843,-6.63074424603682,
19.7383674498727));
#14015=CARTESIAN_POINT('Ctrl Pts',(-1.18346211504224,-6.66522982388226,
19.7470023569971));
#14016=CARTESIAN_POINT('Ctrl Pts',(-1.0022286978934,-6.69237077851481,19.7556372641214));
#14017=CARTESIAN_POINT('Ctrl Pts',(-0.81497847757186,-6.72041279093522,
19.7645588431929));
#14018=CARTESIAN_POINT('Ctrl Pts',(-0.626397716056642,-6.74061400251836,
19.7734804222645));
#14019=CARTESIAN_POINT('Ctrl Pts',(-0.437156738393943,-6.75286479844494,
19.782402001336));
#14020=CARTESIAN_POINT('Ctrl Pts',(-0.254502389179452,-6.7646891991903,
19.7910130603117));
#14021=CARTESIAN_POINT('Ctrl Pts',(-0.0712333493827942,-6.76910723061142,
19.7996241192873));
#14022=CARTESIAN_POINT('Ctrl Pts',(0.112038797017181,-6.76607244329847,
19.808235178263));
#14023=CARTESIAN_POINT('Ctrl Pts',(0.295138109321486,-6.76304051793007,
19.8168381166126));
#14024=CARTESIAN_POINT('Ctrl Pts',(0.478240218476588,-6.75256979155271,
19.8254410549621));
#14025=CARTESIAN_POINT('Ctrl Pts',(0.660731158458518,-6.73466579246826,
19.8340439933116));
#14026=CARTESIAN_POINT('Ctrl Pts',(0.843017750805112,-6.71678184172087,
19.8426372983603));
#14027=CARTESIAN_POINT('Ctrl Pts',(1.02469423641944,-6.69148125322093,19.8512306034091));
#14028=CARTESIAN_POINT('Ctrl Pts',(1.20514917349521,-6.65882155261904,19.8598239084579));
#14029=CARTESIAN_POINT('Ctrl Pts',(1.2252548072328,-6.65518272738698,19.8607813432984));
#14030=CARTESIAN_POINT('Ctrl Pts',(1.2453452804058,-6.65145260219814,19.861738778139));
#14031=CARTESIAN_POINT('Ctrl Pts',(1.26541975028478,-6.64763129660402,19.8626962129795));
#14032=CARTESIAN_POINT('Ctrl Pts',(1.44564640244671,-6.61332398396923,19.8712919705271));
#14033=CARTESIAN_POINT('Ctrl Pts',(1.62437129409007,-6.5717032616975,19.8798877280747));
#14034=CARTESIAN_POINT('Ctrl Pts',(1.80100228832431,-6.52293490366496,19.8884834856222));
#14035=CARTESIAN_POINT('Ctrl Pts',(1.97779808528164,-6.47412104309625,19.8970872633039));
#14036=CARTESIAN_POINT('Ctrl Pts',(2.15249579092547,-6.41814631648068,19.9056910409855));
#14037=CARTESIAN_POINT('Ctrl Pts',(2.32451989163915,-6.35522590262329,19.9142948186671));
#14038=CARTESIAN_POINT('Ctrl Pts',(2.50330468993618,-6.28983266148097,19.9232367323351));
#14039=CARTESIAN_POINT('Ctrl Pts',(2.67920113432479,-6.21693689126618,19.9321786460032));
#14040=CARTESIAN_POINT('Ctrl Pts',(2.85158887552337,-6.13683386486806,19.9411205596712));
#14041=CARTESIAN_POINT('Ctrl Pts',(3.01790941694981,-6.05955007062722,19.9497477620019));
#14042=CARTESIAN_POINT('Ctrl Pts',(3.18096378271897,-5.97555787295674,19.9583749643326));
#14043=CARTESIAN_POINT('Ctrl Pts',(3.34022206281018,-5.88516827041641,19.9670021666633));
#14044=CARTESIAN_POINT('Ctrl Pts',(3.49963201203655,-5.79469258561502,19.9756375850837));
#14045=CARTESIAN_POINT('Ctrl Pts',(3.65523839899704,-5.69780749315107,19.9842730035042));
#14046=CARTESIAN_POINT('Ctrl Pts',(3.80654036991904,-5.59486723811894,19.9929084219246));
#14047=CARTESIAN_POINT('Ctrl Pts',(3.95806586795211,-5.49177490352247,20.0015565979457));
#14048=CARTESIAN_POINT('Ctrl Pts',(4.10527399472444,-5.38260970808873,20.0102047739669));
#14049=CARTESIAN_POINT('Ctrl Pts',(4.24769585966207,-5.26776697318795,20.018852949988));
#14050=CARTESIAN_POINT('Ctrl Pts',(4.26276355295241,-5.2556170472839,20.0197678942198));
#14051=CARTESIAN_POINT('Ctrl Pts',(4.27777770771166,-5.24340360825008,20.0206828384516));
#14052=CARTESIAN_POINT('Ctrl Pts',(4.29273779262652,-5.23112714849831,20.0215977826834));
#14053=CARTESIAN_POINT('Ctrl Pts',(4.42723948425975,-5.12075313569843,20.0298237752247));
#14054=CARTESIAN_POINT('Ctrl Pts',(4.5576581037315,-5.00504350632935,20.0380497677661));
#14055=CARTESIAN_POINT('Ctrl Pts',(4.68354503541923,-4.88433157158684,20.0462757603074));
#14056=CARTESIAN_POINT('Ctrl Pts',(4.80929999093065,-4.76374618770522,20.0544931289588));
#14057=CARTESIAN_POINT('Ctrl Pts',(4.93053246295187,-4.63816918767513,20.0627104976103));
#14058=CARTESIAN_POINT('Ctrl Pts',(5.04682600525942,-4.50797474179229,20.0709278662617));
#14059=CARTESIAN_POINT('Ctrl Pts',(5.16302089865326,-4.37789073661323,20.0791382643241));
#14060=CARTESIAN_POINT('Ctrl Pts',(5.2742849690863,-4.24319735225379,20.0873486623865));
#14061=CARTESIAN_POINT('Ctrl Pts',(5.3802377633856,-4.1043063493652,20.0955590604488));
#14062=CARTESIAN_POINT('Ctrl Pts',(5.48612187529514,-3.96550538059094,20.1037641362376));
#14063=CARTESIAN_POINT('Ctrl Pts',(5.58670135266541,-3.82251249726049,20.1119692120264));
#14064=CARTESIAN_POINT('Ctrl Pts',(5.68163521889898,-3.67577342056971,20.1201742878152));
#14065=CARTESIAN_POINT('Ctrl Pts',(5.77652653225256,-3.52910011777573,20.1283756857847));
#14066=CARTESIAN_POINT('Ctrl Pts',(5.86577708189894,-3.37868426723918,20.1365770837541));
#14067=CARTESIAN_POINT('Ctrl Pts',(5.9490884772207,-3.22500159537944,20.1447784817236));
#14068=CARTESIAN_POINT('Ctrl Pts',(6.03239334690032,-3.07133096122613,20.1529792372913));
#14069=CARTESIAN_POINT('Ctrl Pts',(6.10975981060414,-2.91439432601712,20.1611799928591));
#14070=CARTESIAN_POINT('Ctrl Pts',(6.18093464356704,-2.75469343701849,20.1693807484268));
#14071=CARTESIAN_POINT('Ctrl Pts',(6.25210911499566,-2.59499335922441,20.1775814623385));
#14072=CARTESIAN_POINT('Ctrl Pts',(6.31709187146914,-2.43252938251092,20.1857821762503));
#14073=CARTESIAN_POINT('Ctrl Pts',(6.37567726055921,-2.2678246116462,20.1939828901621));
#14074=CARTESIAN_POINT('Ctrl Pts',(6.43427296919467,-2.10309082879767,20.2021850485917));
#14075=CARTESIAN_POINT('Ctrl Pts',(6.48646894525464,-1.93611580306841,20.2103872070213));
#14076=CARTESIAN_POINT('Ctrl Pts',(6.53210895493344,-1.76743927784759,20.2185893654509));
#14077=CARTESIAN_POINT('Ctrl Pts',(6.57776527508248,-1.59870247232743,20.2267944551038));
#14078=CARTESIAN_POINT('Ctrl Pts',(6.61686086807522,-1.42826330172146,20.2349995447568));
#14079=CARTESIAN_POINT('Ctrl Pts',(6.64929028510915,-1.256673268735,20.2432046344097));
#14080=CARTESIAN_POINT('Ctrl Pts',(6.6817567489179,-1.08488721442299,20.2514190974075));
#14081=CARTESIAN_POINT('Ctrl Pts',(6.7075417560825,-0.911948023638369,20.2596335604053));
#14082=CARTESIAN_POINT('Ctrl Pts',(6.72659143378814,-0.738414980135131,
20.267848023403));
#14083=CARTESIAN_POINT('Ctrl Pts',(6.74565239782574,-0.564779123788346,
20.2760673532105));
#14084=CARTESIAN_POINT('Ctrl Pts',(6.75797005263394,-0.390549070252429,
20.284286683018));
#14085=CARTESIAN_POINT('Ctrl Pts',(6.76354267643597,-0.216285607540968,
20.2925060128255));
#14086=CARTESIAN_POINT('Ctrl Pts',(6.76912393468072,-0.0417521341593407,
20.3007380779862));
#14087=CARTESIAN_POINT('Ctrl Pts',(6.7679392791419,0.132814493732021,20.3089701431468));
#14088=CARTESIAN_POINT('Ctrl Pts',(6.76003909319362,0.306855761709051,20.3172022083075));
#14089=CARTESIAN_POINT('Ctrl Pts',(6.75293783879879,0.463296550216326,20.3246017795687));
#14090=CARTESIAN_POINT('Ctrl Pts',(6.74041135547517,0.619312751898104,20.3320013508299));
#14091=CARTESIAN_POINT('Ctrl Pts',(6.72253151655136,0.774505654578253,20.339400922091));
#14092=CARTESIAN_POINT('Ctrl Pts',(6.7028249356549,0.945554258777326,20.3475564905097));
#14093=CARTESIAN_POINT('Ctrl Pts',(6.67655368957025,1.11612924680917,20.3557120589283));
#14094=CARTESIAN_POINT('Ctrl Pts',(6.64374226276057,1.2856818214508,20.363867627347));
#14095=CARTESIAN_POINT('Ctrl Pts',(6.61097086302003,1.45502755679018,20.3720132466859));
#14096=CARTESIAN_POINT('Ctrl Pts',(6.57167523285376,1.62335300655458,20.3801588660248));
#14097=CARTESIAN_POINT('Ctrl Pts',(6.52593170486439,1.790112952706,20.3883044853637));
#14098=CARTESIAN_POINT('Ctrl Pts',(6.48023436084529,1.95670453326049,20.3964418806531));
#14099=CARTESIAN_POINT('Ctrl Pts',(6.42810217534318,2.12173340702392,20.4045792759425));
#14100=CARTESIAN_POINT('Ctrl Pts',(6.36966277152329,2.28466303359384,20.4127166712318));
#14101=CARTESIAN_POINT('Ctrl Pts',(6.31127008840033,2.44746240240607,20.4208475608973));
#14102=CARTESIAN_POINT('Ctrl Pts',(6.24658035008016,2.60816552330735,20.4289784505629));
#14103=CARTESIAN_POINT('Ctrl Pts',(6.1757714027542,2.76624955145473,20.4371093402284));
#14104=CARTESIAN_POINT('Ctrl Pts',(6.10500419044534,2.92424040437682,20.4452354375218));
#14105=CARTESIAN_POINT('Ctrl Pts',(6.02812510095207,3.07961490612009,20.4533615348153));
#14106=CARTESIAN_POINT('Ctrl Pts',(5.94536063683131,3.23186879344086,20.4614876321088));
#14107=CARTESIAN_POINT('Ctrl Pts',(5.86261858878466,3.38408144404898,20.4696115285157));
#14108=CARTESIAN_POINT('Ctrl Pts',(5.7739945103782,3.53317484009894,20.4777354249226));
#14109=CARTESIAN_POINT('Ctrl Pts',(5.67976160219044,3.67866784886636,20.4858593213295));
#14110=CARTESIAN_POINT('Ctrl Pts',(5.58553966311416,3.82414392162849,20.4939822720802));
#14111=CARTESIAN_POINT('Ctrl Pts',(5.48571039220702,3.96602013413904,20.502105222831));
#14112=CARTESIAN_POINT('Ctrl Pts',(5.38059115512394,4.10384305516208,20.5102281735818));
#14113=CARTESIAN_POINT('Ctrl Pts',(5.27546415673589,4.24167615211251,20.5183517240772));
#14114=CARTESIAN_POINT('Ctrl Pts',(5.16504663618726,4.37545507073959,20.5264752745726));
#14115=CARTESIAN_POINT('Ctrl Pts',(5.04969716750023,4.50475831943737,20.534598825068));
#14116=CARTESIAN_POINT('Ctrl Pts',(4.93431723734688,4.63409571451309,20.5427245208291));
#14117=CARTESIAN_POINT('Ctrl Pts',(4.81400300928169,4.75895481355426,20.5508502165902));
#14118=CARTESIAN_POINT('Ctrl Pts',(4.68915089294007,4.87894997957956,20.5589759123514));
#14119=CARTESIAN_POINT('Ctrl Pts',(4.56417402353802,4.99906504556841,20.5671097273614));
#14120=CARTESIAN_POINT('Ctrl Pts',(4.4346504728083,5.1143062170843,20.5752435423715));
#14121=CARTESIAN_POINT('Ctrl Pts',(4.30101144510691,5.22432670772602,20.5833773573816));
#14122=CARTESIAN_POINT('Ctrl Pts',(4.16730180463402,5.33440533147375,20.5915154701722));
#14123=CARTESIAN_POINT('Ctrl Pts',(4.02947264447767,5.43925755620232,20.5996535829629));
#14124=CARTESIAN_POINT('Ctrl Pts',(3.88798505814178,5.5385793474199,20.6077916957536));
#14125=CARTESIAN_POINT('Ctrl Pts',(3.74629840095428,5.63804088286575,20.6159412587434));
#14126=CARTESIAN_POINT('Ctrl Pts',(3.60094334091334,5.73195624109692,20.6240908217332));
#14127=CARTESIAN_POINT('Ctrl Pts',(3.45240745000457,5.82006630539146,20.6322403847231));
#14128=CARTESIAN_POINT('Ctrl Pts',(3.33651925814909,5.88881006808,20.6385987006394));
#14129=CARTESIAN_POINT('Ctrl Pts',(3.21869538117158,5.9540209528432,20.6449570165556));
#14130=CARTESIAN_POINT('Ctrl Pts',(3.09917575053258,6.01559628526639,20.6513153324719));
#14131=CARTESIAN_POINT('Origin',(0.,0.,-3.69717978381041));
#14132=CARTESIAN_POINT('',(3.09917575053259,6.01559628526639,23.0457515827422));
#14133=CARTESIAN_POINT('',(3.09917575053257,6.0155962852664,22.6516519666359));
#14134=CARTESIAN_POINT('',(3.09917575053259,6.01559628526639,-3.69717978381041));
#14135=CARTESIAN_POINT('',(-6.76724104181633,0.00151419972611408,21.6967615973392));
#14136=CARTESIAN_POINT('Ctrl Pts',(-6.767,1.39537968873079E-12,21.69717978381));
#14137=CARTESIAN_POINT('Ctrl Pts',(-6.76700000000004,-0.186007249414254,
21.705929295616));
#14138=CARTESIAN_POINT('Ctrl Pts',(-6.75932637295446,-0.372014355526077,
21.7146788074219));
#14139=CARTESIAN_POINT('Ctrl Pts',(-6.7440051826694,-0.557389537153566,
21.7234283192278));
#14140=CARTESIAN_POINT('Ctrl Pts',(-6.72868405709661,-0.742763935809995,
21.7321777940784));
#14141=CARTESIAN_POINT('Ctrl Pts',(-6.7057154565301,-0.927506129693716,
21.7409272689289));
#14142=CARTESIAN_POINT('Ctrl Pts',(-6.67517739415671,-1.11098863924852,
21.7496767437795));
#14143=CARTESIAN_POINT('Ctrl Pts',(-6.64463945823089,-1.2944703890656,21.7584261824015));
#14144=CARTESIAN_POINT('Ctrl Pts',(-6.60653217027141,-1.47669218228292,
21.7671756210235));
#14145=CARTESIAN_POINT('Ctrl Pts',(-6.56098496116688,-1.65703510504214,
21.7759250596455));
#14146=CARTESIAN_POINT('Ctrl Pts',(-6.51543793687491,-1.83737729604112,
21.7846744627657));
#14147=CARTESIAN_POINT('Ctrl Pts',(-6.46245112202611,-2.01584035397144,
21.7934238658859));
#14148=CARTESIAN_POINT('Ctrl Pts',(-6.40220448416212,-2.19181813638232,
21.8021732690062));
#14149=CARTESIAN_POINT('Ctrl Pts',(-6.3419580857515,-2.36779521936043,21.8109226373514));
#14150=CARTESIAN_POINT('Ctrl Pts',(-6.27445201489191,-2.54128677544937,
21.8196720056967));
#14151=CARTESIAN_POINT('Ctrl Pts',(-6.19991555136132,-2.7117035523796,21.828421374042));
#14152=CARTESIAN_POINT('Ctrl Pts',(-6.12537937788981,-2.88211966613193,
21.837170708339));
#14153=CARTESIAN_POINT('Ctrl Pts',(-6.04381298133555,-3.04946076210567,
21.8459200426361));
#14154=CARTESIAN_POINT('Ctrl Pts',(-5.95549339426239,-3.21315848206978,
21.8546693769332));
#14155=CARTESIAN_POINT('Ctrl Pts',(-5.86717414355097,-3.37685557859746,
21.8634186779087));
#14156=CARTESIAN_POINT('Ctrl Pts',(-5.77210188986179,-3.53690907467407,
21.8721679788843));
#14157=CARTESIAN_POINT('Ctrl Pts',(-5.67059953467014,-3.69277536784988,
21.8809172798598));
#14158=CARTESIAN_POINT('Ctrl Pts',(-5.56909755761717,-3.84864108035863,
21.8896665482406));
#14159=CARTESIAN_POINT('Ctrl Pts',(-5.46116568338027,-4.00031938104338,
21.8984158166213));
#14160=CARTESIAN_POINT('Ctrl Pts',(-5.34717048686078,-4.14729511663265,
21.9071650850021));
#14161=CARTESIAN_POINT('Ctrl Pts',(-5.23317570555477,-4.2942703168809,21.9159143215147));
#14162=CARTESIAN_POINT('Ctrl Pts',(-5.1131178217876,-4.43654275987182,21.9246635580273));
#14163=CARTESIAN_POINT('Ctrl Pts',(-4.98740459171965,-4.57362924147704,
21.93341279454));
#14164=CARTESIAN_POINT('Ctrl Pts',(-4.86169180910783,-4.71071523514485,
21.9421619999111));
#14165=CARTESIAN_POINT('Ctrl Pts',(-4.73032391415386,-4.84261509316568,
21.9509112052822));
#14166=CARTESIAN_POINT('Ctrl Pts',(-4.59374707237251,-4.96888084331563,
21.9596604106533));
#14167=CARTESIAN_POINT('Ctrl Pts',(-4.45717070537357,-5.09514615452764,
21.9684095856095));
#14168=CARTESIAN_POINT('Ctrl Pts',(-4.31538563819461,-5.21577720253672,
21.9771587605658));
#14169=CARTESIAN_POINT('Ctrl Pts',(-4.16887341290597,-5.3303642902869,21.985907935522));
#14170=CARTESIAN_POINT('Ctrl Pts',(-4.0223616847728,-5.4449509892122,21.9946570807899));
#14171=CARTESIAN_POINT('Ctrl Pts',(-3.87112305634373,-5.55349359238805,
22.0034062260578));
#14172=CARTESIAN_POINT('Ctrl Pts',(-3.71567117316659,-5.65562346102522,
22.0121553713258));
#14173=CARTESIAN_POINT('Ctrl Pts',(-3.56021980457203,-5.7577529915883,22.0209044876319));
#14174=CARTESIAN_POINT('Ctrl Pts',(-3.40055544862266,-5.85346967275425,
22.0296536039381));
#14175=CARTESIAN_POINT('Ctrl Pts',(-3.23722036323256,-5.94244842803642,
22.0384027202443));
#14176=CARTESIAN_POINT('Ctrl Pts',(-3.07388580495894,-6.03142689616553,
22.0471518083152));
#14177=CARTESIAN_POINT('Ctrl Pts',(-2.9068807925755,-6.11366734484897,22.0559008963862));
#14178=CARTESIAN_POINT('Ctrl Pts',(-2.73677251094454,-6.18889046787373,
22.0646499844571));
#14179=CARTESIAN_POINT('Ctrl Pts',(-2.56666476416532,-6.26411335438315,
22.0733990450193));
#14180=CARTESIAN_POINT('Ctrl Pts',(-2.3934540297203,-6.33231884350313,22.0821481055815));
#14181=CARTESIAN_POINT('Ctrl Pts',(-2.21772856474027,-6.39327529621047,
22.0908971661437));
#14182=CARTESIAN_POINT('Ctrl Pts',(-2.04200363768254,-6.45423156232087,
22.0996461999237));
#14183=CARTESIAN_POINT('Ctrl Pts',(-1.86376426620073,-6.50793874252062,
22.1083952337037));
#14184=CARTESIAN_POINT('Ctrl Pts',(-1.68361578194663,-6.55421443796129,
22.1171442674837));
#14185=CARTESIAN_POINT('Ctrl Pts',(-1.50346783419832,-6.60048999558688,
22.125893275208));
#14186=CARTESIAN_POINT('Ctrl Pts',(-1.321411062572,-6.63933404145505,22.1346422829322));
#14187=CARTESIAN_POINT('Ctrl Pts',(-1.13806375958987,-6.6706146552704,22.1433912906564));
#14188=CARTESIAN_POINT('Ctrl Pts',(-0.95471698741806,-6.70189517852497,
22.1521402730514));
#14189=CARTESIAN_POINT('Ctrl Pts',(-0.770079973808261,-6.72561226535848,
22.1608892554463));
#14190=CARTESIAN_POINT('Ctrl Pts',(-0.584779770550317,-6.74168536939801,
22.1696382378412));
#14191=CARTESIAN_POINT('Ctrl Pts',(-0.391490647551807,-6.75845143942406,
22.1787644185172));
#14192=CARTESIAN_POINT('Ctrl Pts',(-0.197480213102271,-6.76689975924032,
22.1878905991933));
#14193=CARTESIAN_POINT('Ctrl Pts',(-0.00346532629577278,-6.76699911271708,
22.1970167798693));
#14194=CARTESIAN_POINT('Ctrl Pts',(0.18448659529802,-6.76709536139768,22.2058577673993));
#14195=CARTESIAN_POINT('Ctrl Pts',(0.37244237818713,-6.75935659726759,22.2146987549292));
#14196=CARTESIAN_POINT('Ctrl Pts',(0.559750217723924,-6.74380965729001,
22.2235397424591));
#14197=CARTESIAN_POINT('Ctrl Pts',(0.745129914459503,-6.72842275717234,
22.2322897210569));
#14198=CARTESIAN_POINT('Ctrl Pts',(0.929874656315842,-6.7053877227345,22.2410396996546));
#14199=CARTESIAN_POINT('Ctrl Pts',(1.11335688289934,-6.67478280180716,22.2497896782524));
#14200=CARTESIAN_POINT('Ctrl Pts',(1.29683723119004,-6.64417819417994,22.2585395672773));
#14201=CARTESIAN_POINT('Ctrl Pts',(1.47905480730373,-6.60600390230044,22.2672894563023));
#14202=CARTESIAN_POINT('Ctrl Pts',(1.65939064804936,-6.56038959797102,22.2760393453272));
#14203=CARTESIAN_POINT('Ctrl Pts',(1.83972470264396,-6.51477574543219,22.2847891476882));
#14204=CARTESIAN_POINT('Ctrl Pts',(2.01817678125981,-6.46172209820059,22.2935389500491));
#14205=CARTESIAN_POINT('Ctrl Pts',(2.19414072347814,-6.40140886723968,22.3022887524101));
#14206=CARTESIAN_POINT('Ctrl Pts',(2.37010298132226,-6.34109621361326,22.3110384710155));
#14207=CARTESIAN_POINT('Ctrl Pts',(2.54357687927037,-6.2735242082592,22.319788189621));
#14208=CARTESIAN_POINT('Ctrl Pts',(2.7139731779009,-6.19892237325444,22.3285379082265));
#14209=CARTESIAN_POINT('Ctrl Pts',(2.88436790207318,-6.12432122756908,22.3372875459848));
#14210=CARTESIAN_POINT('Ctrl Pts',(3.05168482126372,-6.04269049717358,22.346037183743));
#14211=CARTESIAN_POINT('Ctrl Pts',(3.21535561997503,-5.95430745234868,22.3547868215013));
#14212=CARTESIAN_POINT('Ctrl Pts',(3.37902496075387,-5.86592519481455,22.3635363813203));
#14213=CARTESIAN_POINT('Ctrl Pts',(3.53904799384974,-5.77079087940171,22.3722859411393));
#14214=CARTESIAN_POINT('Ctrl Pts',(3.69488118815077,-5.66922763746964,22.3810355009583));
#14215=CARTESIAN_POINT('Ctrl Pts',(3.85071304610924,-5.56766526648989,22.3897849857458));
#14216=CARTESIAN_POINT('Ctrl Pts',(4.00235489706057,-5.45967423580648,22.3985344705332));
#14217=CARTESIAN_POINT('Ctrl Pts',(4.14929168607742,-5.3456213393626,22.4072839553207));
#14218=CARTESIAN_POINT('Ctrl Pts',(4.29622726385834,-5.23156938308467,22.416033367984));
#14219=CARTESIAN_POINT('Ctrl Pts',(4.43845763092134,-5.11145583677144,22.4247827806472));
#14220=CARTESIAN_POINT('Ctrl Pts',(4.57549970661019,-4.98568866204159,22.4335321933105));
#14221=CARTESIAN_POINT('Ctrl Pts',(4.71254069815356,-4.85992248226102,22.4422815367569));
#14222=CARTESIAN_POINT('Ctrl Pts',(4.84439326931379,-4.72850295733935,22.4510308802032));
#14223=CARTESIAN_POINT('Ctrl Pts',(4.97060959434767,-4.59187644221607,22.4597802236495));
#14224=CARTESIAN_POINT('Ctrl Pts',(5.0968249628059,-4.45525096256579,22.4685295007858));
#14225=CARTESIAN_POINT('Ctrl Pts',(5.21740397615918,-4.3134187821823,22.4772787779221));
#14226=CARTESIAN_POINT('Ctrl Pts',(5.33193710452017,-4.1668616143857,22.4860280550584));
#14227=CARTESIAN_POINT('Ctrl Pts',(5.44646940289459,-4.02030550864411,22.4947772687914));
#14228=CARTESIAN_POINT('Ctrl Pts',(5.55495572749733,-3.86902470980035,22.5035264825243));
#14229=CARTESIAN_POINT('Ctrl Pts',(5.65702762491518,-3.71353301465688,22.5122756962573));
#14230=CARTESIAN_POINT('Ctrl Pts',(5.75909881655215,-3.55804239466794,22.5210248494934));
#14231=CARTESIAN_POINT('Ctrl Pts',(5.85475551250843,-3.39834117619448,22.5297740027295));
#14232=CARTESIAN_POINT('Ctrl Pts',(5.94367283728154,-3.2349717469186,22.5385231559657));
#14233=CARTESIAN_POINT('Ctrl Pts',(6.03258957676364,-3.07160339300861,22.5472722516112));
#14234=CARTESIAN_POINT('Ctrl Pts',(6.11476689685331,-2.90456712829405,22.5560213472567));
#14235=CARTESIAN_POINT('Ctrl Pts',(6.18992570525302,-2.73443024475811,22.5647704429022));
#14236=CARTESIAN_POINT('Ctrl Pts',(6.26508404388744,-2.56429442462916,22.5735194838633));
#14237=CARTESIAN_POINT('Ctrl Pts',(6.33322384283366,-2.39105828655859,22.5822685248243));
#14238=CARTESIAN_POINT('Ctrl Pts',(6.39411368720086,-2.21531017131926,22.5910175657854));
#14239=CARTESIAN_POINT('Ctrl Pts',(6.45500317120933,-2.03956309619376,22.5997665549678));
#14240=CARTESIAN_POINT('Ctrl Pts',(6.50864269270108,-1.86130434438511,22.6085155441501));
#14241=CARTESIAN_POINT('Ctrl Pts',(6.55485008446361,-1.68113930719839,22.6172645333325));
#14242=CARTESIAN_POINT('Ctrl Pts',(6.60199664749428,-1.49731239211733,22.6261913468619));
#14243=CARTESIAN_POINT('Ctrl Pts',(6.64140563640928,-1.31150116499564,22.6351181603913));
#14244=CARTESIAN_POINT('Ctrl Pts',(6.6729377228219,-1.12436255155552,22.6440449739206));
#14245=CARTESIAN_POINT('Ctrl Pts',(6.70384494949887,-0.940932395050242,
22.6527948880762));
#14246=CARTESIAN_POINT('Ctrl Pts',(6.72718449348943,-0.756227260505593,
22.6615448022317));
#14247=CARTESIAN_POINT('Ctrl Pts',(6.74287707373942,-0.570874564540552,
22.6702947163872));
#14248=CARTESIAN_POINT('Ctrl Pts',(6.75856934538677,-0.385525513631337,
22.6790444584712));
#14249=CARTESIAN_POINT('Ctrl Pts',(6.76661493004106,-0.199529212417095,
22.6877942005552));
#14250=CARTESIAN_POINT('Ctrl Pts',(6.76698649908907,-0.0135174385992982,
22.6965439426392));
#14251=CARTESIAN_POINT('Ctrl Pts',(6.76735806132386,0.172490924446901,22.7052935242851));
#14252=CARTESIAN_POINT('Ctrl Pts',(6.76005588896283,0.358514472902524,22.714043105931));
#14253=CARTESIAN_POINT('Ctrl Pts',(6.74510478454576,0.54392135966332,22.7227926875769));
#14254=CARTESIAN_POINT('Ctrl Pts',(6.73015393440676,0.729325093151587,22.7315421204159));
#14255=CARTESIAN_POINT('Ctrl Pts',(6.70755443556881,0.914111900257527,22.740291553255));
#14256=CARTESIAN_POINT('Ctrl Pts',(6.67738304682299,1.09765415591659,22.749040986094));
#14257=CARTESIAN_POINT('Ctrl Pts',(6.64721213111836,1.28119353391399,22.7577902817553));
#14258=CARTESIAN_POINT('Ctrl Pts',(6.60946960955465,1.46348811672784,22.7665395774166));
#14259=CARTESIAN_POINT('Ctrl Pts',(6.56428366991149,1.64391876348358,22.775288873078));
#14260=CARTESIAN_POINT('Ctrl Pts',(6.5190983786768,1.82434682109849,22.7840380431888));
#14261=CARTESIAN_POINT('Ctrl Pts',(6.46646995271881,2.00291071820576,22.7927872132996));
#14262=CARTESIAN_POINT('Ctrl Pts',(6.40657713281505,2.17900400212832,22.8015363834105));
#14263=CARTESIAN_POINT('Ctrl Pts',(6.34668509279012,2.35509499309786,22.8102854395962));
#14264=CARTESIAN_POINT('Ctrl Pts',(6.27952894037475,2.52871516398249,22.819034495782));
#14265=CARTESIAN_POINT('Ctrl Pts',(6.20533675061392,2.69927486771545,22.8277835519678));
#14266=CARTESIAN_POINT('Ctrl Pts',(6.12832117907861,2.87632521636041,22.83686555325));
#14267=CARTESIAN_POINT('Ctrl Pts',(6.04372366626024,3.05007728920107,22.8459475545323));
#14268=CARTESIAN_POINT('Ctrl Pts',(5.95185378007813,3.21989527478298,22.8550295558146));
#14269=CARTESIAN_POINT('Ctrl Pts',(5.86334450817313,3.38350129286852,22.8637793361217));
#14270=CARTESIAN_POINT('Ctrl Pts',(5.76808562057195,3.5434556712506,22.8725291164288));
#14271=CARTESIAN_POINT('Ctrl Pts',(5.66640068804421,3.69921508465406,22.8812788967359));
#14272=CARTESIAN_POINT('Ctrl Pts',(5.56471941107855,3.85496889852381,22.8900283624894));
#14273=CARTESIAN_POINT('Ctrl Pts',(5.45661270815041,4.00652780919736,22.8987778282429));
#14274=CARTESIAN_POINT('Ctrl Pts',(5.34244776449036,4.1533770456933,22.9075272939964));
#14275=CARTESIAN_POINT('Ctrl Pts',(5.22828631819518,4.30022178356343,22.916276491716));
#14276=CARTESIAN_POINT('Ctrl Pts',(5.10806717843994,4.44235690972765,22.9250256894356));
#14277=CARTESIAN_POINT('Ctrl Pts',(4.98219864544646,4.57929969070724,22.9337748871552));
#14278=CARTESIAN_POINT('Ctrl Pts',(4.8563332994395,4.71623900430078,22.9425238633454));
#14279=CARTESIAN_POINT('Ctrl Pts',(4.72481904033572,4.84798602483691,22.9512728395357));
#14280=CARTESIAN_POINT('Ctrl Pts',(4.5881025073712,4.97409332259198,22.9600218157259));
#14281=CARTESIAN_POINT('Ctrl Pts',(4.45137708685563,5.10020881822204,22.9687713606621));
#14282=CARTESIAN_POINT('Ctrl Pts',(4.30944892635971,5.22068366307999,22.9775209055982));
#14283=CARTESIAN_POINT('Ctrl Pts',(4.1628000946658,5.33510865604914,22.9862704505344));
#14284=CARTESIAN_POINT('Ctrl Pts',(4.01615988348696,5.4495269227296,22.9950194811427));
#14285=CARTESIAN_POINT('Ctrl Pts',(3.86479978232127,5.55789587288699,23.003768511751));
#14286=CARTESIAN_POINT('Ctrl Pts',(3.70923383580952,5.65984746713954,23.0125175423593));
#14287=CARTESIAN_POINT('Ctrl Pts',(3.55366577799422,5.76180044505456,23.0212666917073));
#14288=CARTESIAN_POINT('Ctrl Pts',(3.39389200026719,5.85733573571129,23.0300158410553));
#14289=CARTESIAN_POINT('Ctrl Pts',(3.23045513625917,5.94612887621995,23.0387649904033));
#14290=CARTESIAN_POINT('Ctrl Pts',(3.18695122151495,5.96976399206732,23.0410938545163));
#14291=CARTESIAN_POINT('Ctrl Pts',(3.14318791262623,5.99292165435354,23.0434227186292));
#14292=CARTESIAN_POINT('Ctrl Pts',(3.09917575053259,6.01559628526639,23.0457515827422));
#14293=CARTESIAN_POINT('Ctrl Pts',(3.09917575053256,6.01559628526641,21.0459192328109));
#14294=CARTESIAN_POINT('Ctrl Pts',(2.94414160813452,6.09546834313728,21.0541282552626));
#14295=CARTESIAN_POINT('Ctrl Pts',(2.78588209296763,6.16941313824782,21.0623372777142));
#14296=CARTESIAN_POINT('Ctrl Pts',(2.62489110093943,6.23716567907323,21.0705463001659));
#14297=CARTESIAN_POINT('Ctrl Pts',(2.46400520838181,6.30487398912472,21.0787499635357));
#14298=CARTESIAN_POINT('Ctrl Pts',(2.30039172030012,6.36639795900436,21.0869536269055));
#14299=CARTESIAN_POINT('Ctrl Pts',(2.1345674974083,6.42151933727588,21.0951572902753));
#14300=CARTESIAN_POINT('Ctrl Pts',(1.96416434180923,6.47816279161949,21.1035874828087));
#14301=CARTESIAN_POINT('Ctrl Pts',(1.7914269459188,6.52804479075767,21.1120176753421));
#14302=CARTESIAN_POINT('Ctrl Pts',(1.61693712927694,6.57098191444518,21.1204478678755));
#14303=CARTESIAN_POINT('Ctrl Pts',(1.44723353533284,6.61274128094362,21.1286468218208));
#14304=CARTESIAN_POINT('Ctrl Pts',(1.27587276456234,6.64793167648423,21.136845775766));
#14305=CARTESIAN_POINT('Ctrl Pts',(1.10340412986792,6.67643530083161,21.1450447297113));
#14306=CARTESIAN_POINT('Ctrl Pts',(0.930936761704805,6.70493871586132,21.1532436234472));
#14307=CARTESIAN_POINT('Ctrl Pts',(0.757361899396523,6.72675539869723,21.161442517183));
#14308=CARTESIAN_POINT('Ctrl Pts',(0.583237434654319,6.74181897523345,21.1696414109189));
#14309=CARTESIAN_POINT('Ctrl Pts',(0.409082661621966,6.75688517375188,21.1778417317629));
#14310=CARTESIAN_POINT('Ctrl Pts',(0.234378452688174,6.76519589389805,21.186042052607));
#14311=CARTESIAN_POINT('Ctrl Pts',(0.0596862445282713,6.76673677278894,
21.194242373451));
#14312=CARTESIAN_POINT('Ctrl Pts',(-0.123590555858885,6.76835337238363,
21.2028456682532));
#14313=CARTESIAN_POINT('Ctrl Pts',(-0.306853703567373,6.7625179702011,21.2114489630554));
#14314=CARTESIAN_POINT('Ctrl Pts',(-0.489457457335657,6.74927554612038,
21.2200522578576));
#14315=CARTESIAN_POINT('Ctrl Pts',(-0.663747179090622,6.73663605563477,
21.2282638407321));
#14316=CARTESIAN_POINT('Ctrl Pts',(-0.837435867117087,6.71724916567306,
21.2364754236065));
#14317=CARTESIAN_POINT('Ctrl Pts',(-1.00996988088243,6.6912069045659,21.2446870064809));
#14318=CARTESIAN_POINT('Ctrl Pts',(-1.18260814332675,6.66514890817699,21.2529035509664));
#14319=CARTESIAN_POINT('Ctrl Pts',(-1.35408998981319,6.63242759211696,21.2611200954519));
#14320=CARTESIAN_POINT('Ctrl Pts',(-1.52387379075133,6.59318569963422,21.2693366399373));
#14321=CARTESIAN_POINT('Ctrl Pts',(-1.69385881556009,6.55389729855966,21.2775629224831));
#14322=CARTESIAN_POINT('Ctrl Pts',(-1.86214143251141,6.5080729857557,21.2857892050288));
#14323=CARTESIAN_POINT('Ctrl Pts',(-2.02819624516931,6.45590497072882,21.2940154875745));
#14324=CARTESIAN_POINT('Ctrl Pts',(-2.05152052326467,6.44857738250242,21.2951709620755));
#14325=CARTESIAN_POINT('Ctrl Pts',(-2.07480088212925,6.44112471379489,21.2963264365764));
#14326=CARTESIAN_POINT('Ctrl Pts',(-2.0980359002287,6.43354757201278,21.2974819110774));
#14327=CARTESIAN_POINT('Ctrl Pts',(-2.27188951211167,6.37685239489128,21.3061276291298));
#14328=CARTESIAN_POINT('Ctrl Pts',(-2.44359915957589,6.31305534389745,21.3147733471822));
#14329=CARTESIAN_POINT('Ctrl Pts',(-2.61257843726977,6.24233313025771,21.3234190652346));
#14330=CARTESIAN_POINT('Ctrl Pts',(-2.78134078000741,6.1717017095278,21.3320536839469));
#14331=CARTESIAN_POINT('Ctrl Pts',(-2.94737946261302,6.09416297144666,21.3406883026592));
#14332=CARTESIAN_POINT('Ctrl Pts',(-3.11012465662858,6.00994289658654,21.3493229213716));
#14333=CARTESIAN_POINT('Ctrl Pts',(-3.27861737868219,5.92274849585121,21.358262481274));
#14334=CARTESIAN_POINT('Ctrl Pts',(-3.4435794258418,5.82839229969718,21.3672020411764));
#14335=CARTESIAN_POINT('Ctrl Pts',(-3.60439967688412,5.72718010623707,21.3761416010789));
#14336=CARTESIAN_POINT('Ctrl Pts',(-3.75930298708128,5.62969173833768,21.3847522543493));
#14337=CARTESIAN_POINT('Ctrl Pts',(-3.91036351788745,5.52584301566804,21.3933629076198));
#14338=CARTESIAN_POINT('Ctrl Pts',(-4.05705853589733,5.41595467450593,21.4019735608903));
#14339=CARTESIAN_POINT('Ctrl Pts',(-4.20361469726065,5.30617035000885,21.4105760636014));
#14340=CARTESIAN_POINT('Ctrl Pts',(-4.34581334112871,5.19035798723764,21.4191785663126));
#14341=CARTESIAN_POINT('Ctrl Pts',(-4.48316026112377,5.06888183656718,21.4277810690238));
#14342=CARTESIAN_POINT('Ctrl Pts',(-4.62035259992436,4.9475424048597,21.4363738897913));
#14343=CARTESIAN_POINT('Ctrl Pts',(-4.75270388045081,4.82055210377769,21.4449667105589));
#14344=CARTESIAN_POINT('Ctrl Pts',(-4.87975241417786,4.68831583581198,21.4535595313264));
#14345=CARTESIAN_POINT('Ctrl Pts',(-4.89472566096314,4.67273119098272,21.4545722342845));
#14346=CARTESIAN_POINT('Ctrl Pts',(-4.90962529197411,4.65707372729123,21.4555849372427));
#14347=CARTESIAN_POINT('Ctrl Pts',(-4.92445058217966,4.64134414406758,21.4565976402008));
#14348=CARTESIAN_POINT('Ctrl Pts',(-5.05027937497575,4.50784021660474,21.4651928979609));
#14349=CARTESIAN_POINT('Ctrl Pts',(-5.1706018550547,4.36929508541175,21.473788155721));
#14350=CARTESIAN_POINT('Ctrl Pts',(-5.28503583096103,4.22619039626211,21.482383413481));
#14351=CARTESIAN_POINT('Ctrl Pts',(-5.39957696943315,4.08295169563952,21.4909867203355));
#14352=CARTESIAN_POINT('Ctrl Pts',(-5.50821840620999,3.9351451527872,21.49959002719));
#14353=CARTESIAN_POINT('Ctrl Pts',(-5.61062040097536,3.78328266405764,21.5081933340445));
#14354=CARTESIAN_POINT('Ctrl Pts',(-5.71726801795294,3.62512390388505,21.5171533369844));
#14355=CARTESIAN_POINT('Ctrl Pts',(-5.81714758748002,3.46256603293383,21.5261133399244));
#14356=CARTESIAN_POINT('Ctrl Pts',(-5.90992806957095,3.29621589288345,21.5350733428644));
#14357=CARTESIAN_POINT('Ctrl Pts',(-5.9992586955561,3.13605114908684,21.5437001860691));
#14358=CARTESIAN_POINT('Ctrl Pts',(-6.0820085529776,2.97237135173396,21.5523270292738));
#14359=CARTESIAN_POINT('Ctrl Pts',(-6.15793115642692,2.80573927382902,21.5609538724786));
#14360=CARTESIAN_POINT('Ctrl Pts',(-6.23392632269387,2.63894793777788,21.5695889607647));
#14361=CARTESIAN_POINT('Ctrl Pts',(-6.30308109241908,2.46919897007563,21.5782240490509));
#14362=CARTESIAN_POINT('Ctrl Pts',(-6.36519788937159,2.29707310052151,21.5868591373371));
#14363=CARTESIAN_POINT('Ctrl Pts',(-6.4274069422329,2.12469158950962,21.5955070504622));
#14364=CARTESIAN_POINT('Ctrl Pts',(-6.4825570380835,1.94992641162066,21.6041549635874));
#14365=CARTESIAN_POINT('Ctrl Pts',(-6.53050058744835,1.77337279705559,21.6128028767125));
#14366=CARTESIAN_POINT('Ctrl Pts',(-6.53587912383372,1.75356616920917,21.6137730409164));
#14367=CARTESIAN_POINT('Ctrl Pts',(-6.54116701590315,1.73373704265969,21.6147432051203));
#14368=CARTESIAN_POINT('Ctrl Pts',(-6.54636409560635,1.71388626453336,21.6157133693242));
#14369=CARTESIAN_POINT('Ctrl Pts',(-6.60118239460743,1.50450215790442,21.6259465684371));
#14370=CARTESIAN_POINT('Ctrl Pts',(-6.64597801593179,1.29238336355856,21.6361797675501));
#14371=CARTESIAN_POINT('Ctrl Pts',(-6.68052239666622,1.07838282054242,21.646412966663));
#14372=CARTESIAN_POINT('Ctrl Pts',(-6.71463017949775,0.867086977576364,
21.6565168308979));
#14373=CARTESIAN_POINT('Ctrl Pts',(-6.73874421554605,0.653956575821893,
21.6666206951327));
#14374=CARTESIAN_POINT('Ctrl Pts',(-6.75269107268225,0.439832100826509,
21.6767245593675));
#14375=CARTESIAN_POINT('Ctrl Pts',(-6.76210285436492,0.29533411164576,21.683542967515));
#14376=CARTESIAN_POINT('Ctrl Pts',(-6.76688547413455,0.150383825806707,
21.6903613756625));
#14377=CARTESIAN_POINT('Ctrl Pts',(-6.76699796740266,0.0052449183330411,
21.69717978381));
#14378=CARTESIAN_POINT('',(-6.76699964607789,0.00218860269287247,21.3028202162152));
#14379=CARTESIAN_POINT('Ctrl Pts',(3.09917575053258,6.01559628526639,20.6513153324719));
#14380=CARTESIAN_POINT('Ctrl Pts',(3.06227820682817,6.03460553510302,20.6532782421475));
#14381=CARTESIAN_POINT('Ctrl Pts',(3.02521909496846,6.053268428723,20.6552411518232));
#14382=CARTESIAN_POINT('Ctrl Pts',(2.9880055900179,6.07158229739347,20.6572040614988));
#14383=CARTESIAN_POINT('Ctrl Pts',(2.83205033354915,6.14833250109595,20.6654302708357));
#14384=CARTESIAN_POINT('Ctrl Pts',(2.67291804970943,6.21917730927014,20.6736564801727));
#14385=CARTESIAN_POINT('Ctrl Pts',(2.51109534433012,6.28384350311842,20.6818826895097));
#14386=CARTESIAN_POINT('Ctrl Pts',(2.34945443982791,6.34843704726817,20.6900996570529));
#14387=CARTESIAN_POINT('Ctrl Pts',(2.18512946255633,6.40686566744847,20.6983166245961));
#14388=CARTESIAN_POINT('Ctrl Pts',(2.01863125158421,6.458902141241,20.7065335921393));
#14389=CARTESIAN_POINT('Ctrl Pts',(1.85228667669486,6.51089059842153,20.7147429774827));
#14390=CARTESIAN_POINT('Ctrl Pts',(1.68377320198984,6.55649854968249,20.722952362826));
#14391=CARTESIAN_POINT('Ctrl Pts',(1.51362135453083,6.59554693676789,20.7311617481694));
#14392=CARTESIAN_POINT('Ctrl Pts',(1.34359237466644,6.63456712679597,20.73936520547));
#14393=CARTESIAN_POINT('Ctrl Pts',(1.17192772666979,6.66703710744346,20.7475686627706));
#14394=CARTESIAN_POINT('Ctrl Pts',(0.999172888189012,6.69282769384571,20.7557721200712));
#14395=CARTESIAN_POINT('Ctrl Pts',(0.826508142741077,6.71860483025044,20.763971299203));
#14396=CARTESIAN_POINT('Ctrl Pts',(0.652754693309591,6.73770945905045,20.7721704783349));
#14397=CARTESIAN_POINT('Ctrl Pts',(0.478468085048685,6.75006350278202,20.7803696574667));
#14398=CARTESIAN_POINT('Ctrl Pts',(0.304214316140977,6.7624152187455,20.7885672916965));
#14399=CARTESIAN_POINT('Ctrl Pts',(0.129427945436976,6.76801885170962,20.7967649259264));
#14400=CARTESIAN_POINT('Ctrl Pts',(-0.0453301721559057,6.76684817145267,
20.8049625601562));
#14401=CARTESIAN_POINT('Ctrl Pts',(-0.220075675516464,6.7656775756967,20.8131596026718));
#14402=CARTESIAN_POINT('Ctrl Pts',(-0.394792571151051,6.75773364206391,
20.8213566451873));
#14403=CARTESIAN_POINT('Ctrl Pts',(-0.568919867081917,6.74304227962716,
20.8295536877029));
#14404=CARTESIAN_POINT('Ctrl Pts',(-0.743066241658224,6.72834930749853,
20.8377516283458));
#14405=CARTESIAN_POINT('Ctrl Pts',(-0.916622530342755,6.7069074638335,20.8459495689886));
#14406=CARTESIAN_POINT('Ctrl Pts',(-1.08903267064767,6.67879456505903,20.8541475096314));
#14407=CARTESIAN_POINT('Ctrl Pts',(-1.2614930368245,6.6506734765409,20.8623478384674));
#14408=CARTESIAN_POINT('Ctrl Pts',(-1.43280623563417,6.61587751963145,20.8705481673034));
#14409=CARTESIAN_POINT('Ctrl Pts',(-1.60242615208156,6.57453568148543,20.8787484961394));
#14410=CARTESIAN_POINT('Ctrl Pts',(-1.7722228168832,6.53315076407132,20.8869573699308));
#14411=CARTESIAN_POINT('Ctrl Pts',(-1.94032232529138,6.48520642318485,20.8951662437222));
#14412=CARTESIAN_POINT('Ctrl Pts',(-2.1061925268366,6.43088190218866,20.9033751175136));
#14413=CARTESIAN_POINT('Ctrl Pts',(-2.27215174908918,6.37652822582135,20.911588396917));
#14414=CARTESIAN_POINT('Ctrl Pts',(-2.43587894336696,6.31578766777315,20.9198016763204));
#14415=CARTESIAN_POINT('Ctrl Pts',(-2.59686182271381,6.24888771492427,20.9280149557239));
#14416=CARTESIAN_POINT('Ctrl Pts',(-2.75808016482367,6.18188991037957,20.9362402483393));
#14417=CARTESIAN_POINT('Ctrl Pts',(-2.9165458446842,6.10871485732904,20.9444655409547));
#14418=CARTESIAN_POINT('Ctrl Pts',(-3.07176992376616,6.02963668353622,20.9526908335702));
#14419=CARTESIAN_POINT('Ctrl Pts',(-3.21215145709171,5.95811997456119,20.9601296226823));
#14420=CARTESIAN_POINT('Ctrl Pts',(-3.34988184633226,5.88177577113918,20.9675684117943));
#14421=CARTESIAN_POINT('Ctrl Pts',(-3.48462051066236,5.80083691346957,20.9750072009064));
#14422=CARTESIAN_POINT('Ctrl Pts',(-3.63362155385508,5.7113305027629,20.9832334019253));
#14423=CARTESIAN_POINT('Ctrl Pts',(-3.77938003164929,5.61595440977538,20.9914596029441));
#14424=CARTESIAN_POINT('Ctrl Pts',(-3.92140267518536,5.51496963355639,20.999685803963));
#14425=CARTESIAN_POINT('Ctrl Pts',(-4.06326578621417,5.41409829244989,21.0079027645787));
#14426=CARTESIAN_POINT('Ctrl Pts',(-4.20140112957516,5.30763101940892,21.0161197251945));
#14427=CARTESIAN_POINT('Ctrl Pts',(-4.33534097028699,5.19587410079874,21.0243366858102));
#14428=CARTESIAN_POINT('Ctrl Pts',(-4.46915724060706,5.08422028703131,21.0325460656118));
#14429=CARTESIAN_POINT('Ctrl Pts',(-4.59878544326628,4.96728677497224,21.0407554454134));
#14430=CARTESIAN_POINT('Ctrl Pts',(-4.72378766162664,4.84542249219446,21.048964825215));
#14431=CARTESIAN_POINT('Ctrl Pts',(-4.84869963616683,4.72364618784269,21.0571682783554));
#14432=CARTESIAN_POINT('Ctrl Pts',(-4.96899202270647,4.59694645243934,21.0653717314959));
#14433=CARTESIAN_POINT('Ctrl Pts',(-5.08426072608249,4.46571179871868,21.0735751846363));
#14434=CARTESIAN_POINT('Ctrl Pts',(-5.19946933524446,4.33454556290452,21.0817743609864));
#14435=CARTESIAN_POINT('Ctrl Pts',(-5.30965924274331,4.19884938756544,21.0899735373366));
#14436=CARTESIAN_POINT('Ctrl Pts',(-5.41446385749655,4.0590479346595,21.0981727136867));
#14437=CARTESIAN_POINT('Ctrl Pts',(-5.5192487516799,3.91927278750669,21.1063703472381));
#14438=CARTESIAN_POINT('Ctrl Pts',(-5.61865015167468,3.7753941843924,21.1145679807895));
#14439=CARTESIAN_POINT('Ctrl Pts',(-5.71234216973286,3.62786933831577,21.1227656143408));
#14440=CARTESIAN_POINT('Ctrl Pts',(-5.8060274396663,3.48035511764871,21.1309626574614));
#14441=CARTESIAN_POINT('Ctrl Pts',(-5.89400395358346,3.32919547934301,21.139159700582));
#14442=CARTESIAN_POINT('Ctrl Pts',(-5.97598957491879,3.17487599765125,21.1473567437026));
#14443=CARTESIAN_POINT('Ctrl Pts',(-6.05798419202711,3.02053958344127,21.1555546862338));
#14444=CARTESIAN_POINT('Ctrl Pts',(-6.13398643861804,2.8630429519176,21.163752628765));
#14445=CARTESIAN_POINT('Ctrl Pts',(-6.20376047911267,2.70289565425669,21.1719505712962));
#14446=CARTESIAN_POINT('Ctrl Pts',(-6.27355485684178,2.54270167801562,21.1801509033046));
#14447=CARTESIAN_POINT('Ctrl Pts',(-6.33711726928226,2.37985582546049,21.188351235313));
#14448=CARTESIAN_POINT('Ctrl Pts',(-6.39426028112862,2.21488700776833,21.1965515673214));
#14449=CARTESIAN_POINT('Ctrl Pts',(-6.451462851438,2.04974624798018,21.2047604462921));
#14450=CARTESIAN_POINT('Ctrl Pts',(-6.50223253649237,1.88247844177856,21.2129693252629));
#14451=CARTESIAN_POINT('Ctrl Pts',(-6.54643170871449,1.7136279885487,21.2211782042337));
#14452=CARTESIAN_POINT('Ctrl Pts',(-6.59065460807742,1.5446868924792,21.229391489921));
#14453=CARTESIAN_POINT('Ctrl Pts',(-6.62829988576043,1.37416180557822,21.2376047756084));
#14454=CARTESIAN_POINT('Ctrl Pts',(-6.6592812259374,1.20260656653692,21.2458180612958));
#14455=CARTESIAN_POINT('Ctrl Pts',(-6.69030788799672,1.03080036332443,21.2540433620079));
#14456=CARTESIAN_POINT('Ctrl Pts',(-6.71465108074954,0.857961351510397,
21.26226866272));
#14457=CARTESIAN_POINT('Ctrl Pts',(-6.73227634093087,0.684649011788133,
21.2704939634321));
#14458=CARTESIAN_POINT('Ctrl Pts',(-6.74821626266822,0.52790890679864,21.2779327557261));
#14459=CARTESIAN_POINT('Ctrl Pts',(-6.75866224229275,0.37078189373866,21.2853715480201));
#14460=CARTESIAN_POINT('Ctrl Pts',(-6.76362548441819,0.213680384052582,
21.2928103403141));
#14461=CARTESIAN_POINT('Ctrl Pts',(-6.76585171665472,0.143213452069029,
21.2961469656061));
#14462=CARTESIAN_POINT('Ctrl Pts',(-6.76697683831429,0.0727085243909415,
21.299483590898));
#14463=CARTESIAN_POINT('Ctrl Pts',(-6.76699964607772,0.00218860322720043,
21.3028202161899));
#14464=CARTESIAN_POINT('Ctrl Pts',(-6.76699964607789,0.00218860269286346,
21.3028202162152));
#14465=CARTESIAN_POINT('Ctrl Pts',(-6.7670550866106,-0.169229474448601,
21.3109308023056));
#14466=CARTESIAN_POINT('Ctrl Pts',(-6.76059291480052,-0.340926580401995,
21.3190413883959));
#14467=CARTESIAN_POINT('Ctrl Pts',(-6.74757566434377,-0.512358911268055,
21.3271519744863));
#14468=CARTESIAN_POINT('Ctrl Pts',(-6.73457327164884,-0.683595570955248,
21.3352533032334));
#14469=CARTESIAN_POINT('Ctrl Pts',(-6.71503071894525,-0.854567692450595,
21.3433546319804));
#14470=CARTESIAN_POINT('Ctrl Pts',(-6.68896247809689,-1.0247292162381,21.3514559607275));
#14471=CARTESIAN_POINT('Ctrl Pts',(-6.66291838775061,-1.19473309662122,
21.3595497841289));
#14472=CARTESIAN_POINT('Ctrl Pts',(-6.63036069895213,-1.36392751142699,
21.3676436075304));
#14473=CARTESIAN_POINT('Ctrl Pts',(-6.59135583382869,-1.53176932723321,
21.3757374309319));
#14474=CARTESIAN_POINT('Ctrl Pts',(-6.55237872664589,-1.69949169785882,
21.3838254943373));
#14475=CARTESIAN_POINT('Ctrl Pts',(-6.50696366088859,-1.86586302745634,
21.3919135577427));
#14476=CARTESIAN_POINT('Ctrl Pts',(-6.45522849449401,-2.03034826664605,
21.4000016211481));
#14477=CARTESIAN_POINT('Ctrl Pts',(-6.40351904004577,-2.19475175804333,
21.4080856648534));
#14478=CARTESIAN_POINT('Ctrl Pts',(-6.34549585029914,-2.35727067388517,
21.4161697085587));
#14479=CARTESIAN_POINT('Ctrl Pts',(-6.28132718315745,-2.51738312899076,
21.4242537522641));
#14480=CARTESIAN_POINT('Ctrl Pts',(-6.217166373681,-2.67747597779737,21.4323368060515));
#14481=CARTESIAN_POINT('Ctrl Pts',(-6.14686171446634,-2.83516260657845,
21.440419859839));
#14482=CARTESIAN_POINT('Ctrl Pts',(-6.07063042492687,-2.98993900338321,
21.4485029136265));
#14483=CARTESIAN_POINT('Ctrl Pts',(-5.99440076094549,-3.14471209973189,
21.4565857950507));
#14484=CARTESIAN_POINT('Ctrl Pts',(-5.91224488069568,-3.29657475551216,
21.4646686764749));
#14485=CARTESIAN_POINT('Ctrl Pts',(-5.82442688351885,-3.44504578758293,
21.4727515578991));
#14486=CARTESIAN_POINT('Ctrl Pts',(-5.73659368802381,-3.59354251495607,
21.4808358381961));
#14487=CARTESIAN_POINT('Ctrl Pts',(-5.64309661274925,-3.738646131684,21.4889201184931));
#14488=CARTESIAN_POINT('Ctrl Pts',(-5.54424411578657,-3.87990285761977,
21.49700439879));
#14489=CARTESIAN_POINT('Ctrl Pts',(-5.44535529199878,-4.02121149330526,
21.50509164994));
#14490=CARTESIAN_POINT('Ctrl Pts',(-5.34110734030057,-4.15867012116083,
21.51317890109));
#14491=CARTESIAN_POINT('Ctrl Pts',(-5.23185009928415,-4.29185665401589,
21.5212661522399));
#14492=CARTESIAN_POINT('Ctrl Pts',(-5.12246746645082,-4.42519604174067,
21.5293626849268));
#14493=CARTESIAN_POINT('Ctrl Pts',(-5.00806429764822,-4.55425325694381,
21.5374592176137));
#14494=CARTESIAN_POINT('Ctrl Pts',(-4.88902910078328,-4.67864119715267,
21.5455557503006));
#14495=CARTESIAN_POINT('Ctrl Pts',(-4.76991955132648,-4.80310683342115,
21.5536573402999));
#14496=CARTESIAN_POINT('Ctrl Pts',(-4.64617247530951,-4.92289712879588,
21.5617589302993));
#14497=CARTESIAN_POINT('Ctrl Pts',(-4.51821047574782,-5.03766444861532,
21.5698605202987));
#14498=CARTESIAN_POINT('Ctrl Pts',(-4.39005486302091,-5.1526054173628,21.5779743684254));
#14499=CARTESIAN_POINT('Ctrl Pts',(-4.2576718730724,-5.26250799626261,21.5860882165521));
#14500=CARTESIAN_POINT('Ctrl Pts',(-4.12151497908504,-5.36706654301748,
21.5942020646789));
#14501=CARTESIAN_POINT('Ctrl Pts',(-4.02971606676951,-5.43756140070924,
21.5996725363598));
#14502=CARTESIAN_POINT('Ctrl Pts',(-3.93620226711389,-5.50562795751845,
21.6051430080408));
#14503=CARTESIAN_POINT('Ctrl Pts',(-3.84111885571986,-5.57118433874103,
21.6106134797217));
#14504=CARTESIAN_POINT('Ctrl Pts',(-3.69801849100092,-5.66984657566614,
21.6188465298537));
#14505=CARTESIAN_POINT('Ctrl Pts',(-3.55090515941149,-5.76313603609576,
21.6270795799858));
#14506=CARTESIAN_POINT('Ctrl Pts',(-3.40021895058611,-5.85070936622861,
21.6353126301178));
#14507=CARTESIAN_POINT('Ctrl Pts',(-3.24971218587267,-5.93817840998661,
21.6435358759526));
#14508=CARTESIAN_POINT('Ctrl Pts',(-3.09564132282225,-6.01994469972233,
21.6517591217875));
#14509=CARTESIAN_POINT('Ctrl Pts',(-2.93847736012107,-6.09570666978456,
21.6599823676223));
#14510=CARTESIAN_POINT('Ctrl Pts',(-2.78146909883463,-6.17139358290803,
21.6681974667358));
#14511=CARTESIAN_POINT('Ctrl Pts',(-2.62137416095189,-6.24108786829145,
21.6764125658494));
#14512=CARTESIAN_POINT('Ctrl Pts',(-2.45869029514056,-6.30453257843764,
21.6846276649629));
#14513=CARTESIAN_POINT('Ctrl Pts',(-2.29613504951535,-6.36792712829053,
21.6928362691018));
#14514=CARTESIAN_POINT('Ctrl Pts',(-2.1309952850655,-6.42508181484139,21.7010448732407));
#14515=CARTESIAN_POINT('Ctrl Pts',(-1.96379108229923,-6.47578671553364,
21.7092534773796));
#14516=CARTESIAN_POINT('Ctrl Pts',(-1.79668562806048,-6.52646167060134,
21.7174572336285));
#14517=CARTESIAN_POINT('Ctrl Pts',(-1.62751850622446,-6.57069432450043,
21.7256609898775));
#14518=CARTESIAN_POINT('Ctrl Pts',(-1.45682749523002,-6.60832373973475,
21.7338647461265));
#14519=CARTESIAN_POINT('Ctrl Pts',(-1.28618698740327,-6.6459420213736,21.7420660750907));
#14520=CARTESIAN_POINT('Ctrl Pts',(-1.11402383706335,-6.67696087532799,
21.750267404055));
#14521=CARTESIAN_POINT('Ctrl Pts',(-0.940888873299894,-6.70126981460234,
21.7584687330193));
#14522=CARTESIAN_POINT('Ctrl Pts',(-0.767777786500949,-6.72557540144188,
21.766668930942));
#14523=CARTESIAN_POINT('Ctrl Pts',(-0.593695507772916,-6.7431728660062,
21.7748691288647));
#14524=CARTESIAN_POINT('Ctrl Pts',(-0.419200923101633,-6.75400322668495,
21.7830693267874));
#14525=CARTESIAN_POINT('Ctrl Pts',(-0.244698780930254,-6.76483405643529,
21.7912698798672));
#14526=CARTESIAN_POINT('Ctrl Pts',(-0.069784654852228,-6.76889717613982,
21.7994704329471));
#14527=CARTESIAN_POINT('Ctrl Pts',(0.104979548719595,-6.76618565325772,
21.8076709860269));
#14528=CARTESIAN_POINT('Ctrl Pts',(0.279782992165525,-6.76347352155635,
21.8158733803801));
#14529=CARTESIAN_POINT('Ctrl Pts',(0.454436087892108,-6.75398372319741,
21.8240757747333));
#14530=CARTESIAN_POINT('Ctrl Pts',(0.628378974667604,-6.7377614134218,21.8322781690865));
#14531=CARTESIAN_POINT('Ctrl Pts',(0.802484528620172,-6.72152393293478,
21.8404882341204));
#14532=CARTESIAN_POINT('Ctrl Pts',(0.975878189466887,-6.69854139529803,
21.8486982991542));
#14533=CARTESIAN_POINT('Ctrl Pts',(1.14800630951264,-6.66891074414099,21.856908364188));
#14534=CARTESIAN_POINT('Ctrl Pts',(1.32021680702311,-6.63926591227996,21.8651223584133));
#14535=CARTESIAN_POINT('Ctrl Pts',(1.4911602058588,-6.60296669755028,21.8733363526387));
#14536=CARTESIAN_POINT('Ctrl Pts',(1.66029512134809,-6.56016075336784,21.881550346864));
#14537=CARTESIAN_POINT('Ctrl Pts',(1.82966062405915,-6.51729645042657,21.8897755394992));
#14538=CARTESIAN_POINT('Ctrl Pts',(1.99721237219837,-6.46790779087146,21.8980007321344));
#14539=CARTESIAN_POINT('Ctrl Pts',(2.16242499113894,-6.41219207117954,21.9062259247695));
#14540=CARTESIAN_POINT('Ctrl Pts',(2.3110003454966,-6.36208704379361,21.9136228228895));
#14541=CARTESIAN_POINT('Ctrl Pts',(2.4576840380658,-6.30686581396072,21.9210197210094));
#14542=CARTESIAN_POINT('Ctrl Pts',(2.60210982344173,-6.24670420836044,21.9284166191294));
#14543=CARTESIAN_POINT('Ctrl Pts',(2.77092389665618,-6.17638348504868,21.9370625856203));
#14544=CARTESIAN_POINT('Ctrl Pts',(2.93703609492105,-6.0991529668233,21.9457085521112));
#14545=CARTESIAN_POINT('Ctrl Pts',(3.09987589074755,-6.01523552838641,21.9543545186021));
#14546=CARTESIAN_POINT('Ctrl Pts',(3.26250739233755,-5.93142543176162,21.9629894257264));
#14547=CARTESIAN_POINT('Ctrl Pts',(3.421874568541,-5.8409456100945,21.9716243328508));
#14548=CARTESIAN_POINT('Ctrl Pts',(3.57742734294272,-5.74406673063308,21.9802592399751));
#14549=CARTESIAN_POINT('Ctrl Pts',(3.7381443439053,-5.64397155056613,21.9891808190466));
#14550=CARTESIAN_POINT('Ctrl Pts',(3.89478901331375,-5.53704522027752,21.9981023981181));
#14551=CARTESIAN_POINT('Ctrl Pts',(4.04678002526133,-5.4236390391642,22.0070239771897));
#14552=CARTESIAN_POINT('Ctrl Pts',(4.19348091275735,-5.31418001784657,22.0156350361653));
#14553=CARTESIAN_POINT('Ctrl Pts',(4.33584632806746,-5.19868478645936,22.024246095141));
#14554=CARTESIAN_POINT('Ctrl Pts',(4.47338062319848,-5.07751462824012,22.0328571541167));
#14555=CARTESIAN_POINT('Ctrl Pts',(4.61078521713796,-4.95645873907563,22.0414600924662));
#14556=CARTESIAN_POINT('Ctrl Pts',(4.74336754624104,-4.8297387939334,22.0500630308156));
#14557=CARTESIAN_POINT('Ctrl Pts',(4.8706638592181,-4.69775718513703,22.058665969165));
#14558=CARTESIAN_POINT('Ctrl Pts',(4.99781762977369,-4.56592336520955,22.0672592742137));
#14559=CARTESIAN_POINT('Ctrl Pts',(5.11969698141735,-4.42883985472765,22.0758525792624));
#14560=CARTESIAN_POINT('Ctrl Pts',(5.23587380683145,-4.28694698811827,22.0844458843111));
#14561=CARTESIAN_POINT('Ctrl Pts',(5.24881780680619,-4.27113780022508,22.0854033191518));
#14562=CARTESIAN_POINT('Ctrl Pts',(5.26169105482427,-4.25526894923221,22.0863607539925));
#14563=CARTESIAN_POINT('Ctrl Pts',(5.27449298695413,-4.23934107268708,22.0873181888332));
#14564=CARTESIAN_POINT('Ctrl Pts',(5.38942749743028,-4.09634213509955,22.0959139463808));
#14565=CARTESIAN_POINT('Ctrl Pts',(5.49847583092701,-3.94875035898457,22.1045097039283));
#14566=CARTESIAN_POINT('Ctrl Pts',(5.60129477837398,-3.79707595469993,22.1131054614759));
#14567=CARTESIAN_POINT('Ctrl Pts',(5.70420965939407,-3.64526003304019,22.1217092391574));
#14568=CARTESIAN_POINT('Ctrl Pts',(5.80088338163245,-3.48935413255895,22.1303130168389));
#14569=CARTESIAN_POINT('Ctrl Pts',(5.89101743056434,-3.32989528856196,22.1389167945205));
#14570=CARTESIAN_POINT('Ctrl Pts',(5.9846938264375,-3.16416957255617,22.1478587081885));
#14571=CARTESIAN_POINT('Ctrl Pts',(6.07130595035719,-2.99460633227664,22.1568006218566));
#14572=CARTESIAN_POINT('Ctrl Pts',(6.15057310451502,-2.82183264670613,22.1657425355246));
#14573=CARTESIAN_POINT('Ctrl Pts',(6.22705044510308,-2.65513974424968,22.1743697378554));
#14574=CARTESIAN_POINT('Ctrl Pts',(6.29669095046605,-2.48545882169553,22.1829969401861));
#14575=CARTESIAN_POINT('Ctrl Pts',(6.3592929618526,-2.31337027415241,22.1916241425168));
#14576=CARTESIAN_POINT('Ctrl Pts',(6.42195459207313,-2.14111783860764,22.2002595609373));
#14577=CARTESIAN_POINT('Ctrl Pts',(6.47756425296698,-1.96645349072783,22.2088949793578));
#14578=CARTESIAN_POINT('Ctrl Pts',(6.52597045002582,-1.78997169960584,22.2175303977782));
#14579=CARTESIAN_POINT('Ctrl Pts',(6.57444816034549,-1.61322918177679,22.2261785737993));
#14580=CARTESIAN_POINT('Ctrl Pts',(6.61570106750114,-1.43466415123393,22.2348267498204));
#14581=CARTESIAN_POINT('Ctrl Pts',(6.64962864642111,-1.25488161381691,22.2434749258415));
#14582=CARTESIAN_POINT('Ctrl Pts',(6.65321805562811,-1.23586130303719,22.2443898700734));
#14583=CARTESIAN_POINT('Ctrl Pts',(6.65672552145886,-1.21682736966386,22.2453048143052));
#14584=CARTESIAN_POINT('Ctrl Pts',(6.66015095884106,-1.19778053308965,22.2462197585371));
#14585=CARTESIAN_POINT('Ctrl Pts',(6.69094805157703,-1.02653606797389,22.2544457510784));
#14586=CARTESIAN_POINT('Ctrl Pts',(6.71517681990731,-0.853878309912253,
22.2626717436198));
#14587=CARTESIAN_POINT('Ctrl Pts',(6.73271195522136,-0.68035191483481,22.2708977361612));
#14588=CARTESIAN_POINT('Ctrl Pts',(6.75022870721254,-0.507007439753377,
22.2791151048126));
#14589=CARTESIAN_POINT('Ctrl Pts',(6.76106576472004,-0.332796494650787,
22.287332473464));
#14590=CARTESIAN_POINT('Ctrl Pts',(6.76514880467671,-0.158273973164549,
22.2955498421154));
#14591=CARTESIAN_POINT('Ctrl Pts',(6.76922838109235,0.0161005052164206,
22.3037602401778));
#14592=CARTESIAN_POINT('Ctrl Pts',(6.76656534222491,0.190785677408156,22.3119706382402));
#14593=CARTESIAN_POINT('Ctrl Pts',(6.75713714109871,0.365221379966116,22.3201810363026));
#14594=CARTESIAN_POINT('Ctrl Pts',(6.74771505166959,0.539544007064629,22.3283861120914));
#14595=CARTESIAN_POINT('Ctrl Pts',(6.73153655468924,0.713617130167781,22.3365911878803));
#14596=CARTESIAN_POINT('Ctrl Pts',(6.70863117675751,0.886880338172575,22.3447962636691));
#14597=CARTESIAN_POINT('Ctrl Pts',(6.68573606586565,1.06006588318192,22.3529976616386));
#14598=CARTESIAN_POINT('Ctrl Pts',(6.65612012811828,1.23244188190747,22.3611990596082));
#14599=CARTESIAN_POINT('Ctrl Pts',(6.61986476529523,1.40345270287342,22.3694004575777));
#14600=CARTESIAN_POINT('Ctrl Pts',(6.58361224229438,1.57445012884658,22.3776012131454));
#14601=CARTESIAN_POINT('Ctrl Pts',(6.54072139582365,1.7440822380292,22.3858019687131));
#14602=CARTESIAN_POINT('Ctrl Pts',(6.49132488253577,1.91180288454955,22.3940027242808));
#14603=CARTESIAN_POINT('Ctrl Pts',(6.4419286201587,2.07952267912875,22.4022034381926));
#14604=CARTESIAN_POINT('Ctrl Pts',(6.38602685701169,2.24533068631008,22.4104041521044));
#14605=CARTESIAN_POINT('Ctrl Pts',(6.32380231199367,2.40869535616763,22.4186048660161));
#14606=CARTESIAN_POINT('Ctrl Pts',(6.26156680640956,2.57208880195691,22.4268070244457));
#14607=CARTESIAN_POINT('Ctrl Pts',(6.1930064276042,2.73303771805244,22.4350091828754));
#14608=CARTESIAN_POINT('Ctrl Pts',(6.11835230166785,2.89102993977506,22.443211341305));
#14609=CARTESIAN_POINT('Ctrl Pts',(6.04367149642323,3.04907862352351,22.4514164309579));
#14610=CARTESIAN_POINT('Ctrl Pts',(5.96289275888009,3.20416818419458,22.4596215206108));
#14611=CARTESIAN_POINT('Ctrl Pts',(5.87629349793066,3.35581044252769,22.4678266102638));
#14612=CARTESIAN_POINT('Ctrl Pts',(5.78959530756407,3.50762593421255,22.4760410732615));
#14613=CARTESIAN_POINT('Ctrl Pts',(5.69706348763933,3.65598594434046,22.4842555362593));
#14614=CARTESIAN_POINT('Ctrl Pts',(5.59901975184601,3.80042982022274,22.4924699992571));
#14615=CARTESIAN_POINT('Ctrl Pts',(5.50091792823782,3.94495927453645,22.5006893290646));
#14616=CARTESIAN_POINT('Ctrl Pts',(5.39729789134114,4.08556768157093,22.5089086588721));
#14617=CARTESIAN_POINT('Ctrl Pts',(5.28852202658054,4.22182706590079,22.5171279886796));
#14618=CARTESIAN_POINT('Ctrl Pts',(5.17957762021267,4.35829757588515,22.5253600538403));
#14619=CARTESIAN_POINT('Ctrl Pts',(5.06546165565918,4.49040532590808,22.533592119001));
#14620=CARTESIAN_POINT('Ctrl Pts',(4.94657470504804,4.61775786365839,22.5418241841616));
#14621=CARTESIAN_POINT('Ctrl Pts',(4.83971057728852,4.73223146900103,22.5492237554227));
#14622=CARTESIAN_POINT('Ctrl Pts',(4.72899225507448,4.84286338617217,22.5566233266837));
#14623=CARTESIAN_POINT('Ctrl Pts',(4.61473302931236,4.94939673780286,22.5640228979448));
#14624=CARTESIAN_POINT('Ctrl Pts',(4.4888109016867,5.06680438003875,22.5721777734088));
#14625=CARTESIAN_POINT('Ctrl Pts',(4.35819986244688,5.17959482414312,22.5803326488729));
#14626=CARTESIAN_POINT('Ctrl Pts',(4.22327437086737,5.28736631872379,22.5884875243369));
#14627=CARTESIAN_POINT('Ctrl Pts',(4.08849295352132,5.39502273426872,22.596633691977));
#14628=CARTESIAN_POINT('Ctrl Pts',(3.94940653117599,5.49767063625115,22.6047798596171));
#14629=CARTESIAN_POINT('Ctrl Pts',(3.80642688585204,5.59494444678969,22.6129260272572));
#14630=CARTESIAN_POINT('Ctrl Pts',(3.66360947720701,5.69210788231693,22.6210629515733));
#14631=CARTESIAN_POINT('Ctrl Pts',(3.51690794436196,5.78390916785031,22.6291998758894));
#14632=CARTESIAN_POINT('Ctrl Pts',(3.36676732264903,5.87002272526629,22.6373368002054));
#14633=CARTESIAN_POINT('Ctrl Pts',(3.27872062325342,5.92052214652344,22.6421085223489));
#14634=CARTESIAN_POINT('Ctrl Pts',(3.18949186057883,5.96906631801721,22.6468802444924));
#14635=CARTESIAN_POINT('Ctrl Pts',(3.09917575053257,6.0155962852664,22.6516519666359));
#14636=CARTESIAN_POINT('Origin',(0.,0.,-3.69717978381041));
#14637=CARTESIAN_POINT('',(3.09917575053259,6.01559628526639,25.045602228898));
#14638=CARTESIAN_POINT('',(3.09917575053259,6.01559628526639,24.6513135168612));
#14639=CARTESIAN_POINT('',(3.09917575053259,6.01559628526639,-3.69717978381041));
#14640=CARTESIAN_POINT('',(-6.76701668052783,-0.00100310113704692,23.6971507773732));
#14641=CARTESIAN_POINT('Ctrl Pts',(-6.76699991253939,-0.00108797603646345,
23.69717978381));
#14642=CARTESIAN_POINT('Ctrl Pts',(-6.76696999291398,-0.187182242599655,
23.7058996157294));
#14643=CARTESIAN_POINT('Ctrl Pts',(-6.75925933188796,-0.373124448303,23.7146194476488));
#14644=CARTESIAN_POINT('Ctrl Pts',(-6.74393107196761,-0.558285497348596,
23.7233392795683));
#14645=CARTESIAN_POINT('Ctrl Pts',(-6.72858154856933,-0.743703403200013,
23.7320712077044));
#14646=CARTESIAN_POINT('Ctrl Pts',(-6.70559334447299,-0.928337704410554,
23.7408031358405));
#14647=CARTESIAN_POINT('Ctrl Pts',(-6.6750810980413,-1.11156706256156,23.7495350639766));
#14648=CARTESIAN_POINT('Ctrl Pts',(-6.64450122138508,-1.29520254756596,
23.7582863463829));
#14649=CARTESIAN_POINT('Ctrl Pts',(-6.60636399465147,-1.47742657928581,
23.7670376287892));
#14650=CARTESIAN_POINT('Ctrl Pts',(-6.56083512384141,-1.65762826887358,
23.7757889111954));
#14651=CARTESIAN_POINT('Ctrl Pts',(-6.51525403539874,-1.83803663403789,
23.7845502305572));
#14652=CARTESIAN_POINT('Ctrl Pts',(-6.46226445221919,-2.01641775159363,
23.7933115499189));
#14653=CARTESIAN_POINT('Ctrl Pts',(-6.40208151698484,-2.19217728523061,
23.8020728692807));
#14654=CARTESIAN_POINT('Ctrl Pts',(-6.34178547102113,-2.36826714986534,
23.8108506550913));
#14655=CARTESIAN_POINT('Ctrl Pts',(-6.2742691383388,-2.54172531063156,23.8196284409018));
#14656=CARTESIAN_POINT('Ctrl Pts',(-6.19979607302999,-2.7119767058074,23.8284062267124));
#14657=CARTESIAN_POINT('Ctrl Pts',(-6.1575802052052,-2.80848556261255,23.8333820101589));
#14658=CARTESIAN_POINT('Ctrl Pts',(-6.11312976889147,-2.90396441822418,
23.8383577936054));
#14659=CARTESIAN_POINT('Ctrl Pts',(-6.06649922755934,-2.9983122122324,23.8433335770519));
#14660=CARTESIAN_POINT('Ctrl Pts',(-5.98942166532854,-3.15426360709636,
23.8515582565707));
#14661=CARTESIAN_POINT('Ctrl Pts',(-5.90622510604941,-3.30744646288433,
23.8597829360895));
#14662=CARTESIAN_POINT('Ctrl Pts',(-5.81713249635009,-3.45734848112072,
23.8680076156083));
#14663=CARTESIAN_POINT('Ctrl Pts',(-5.72813353306276,-3.6070929353773,23.8762236500584));
#14664=CARTESIAN_POINT('Ctrl Pts',(-5.63325104221724,-3.75356311375887,
23.8844396845086));
#14665=CARTESIAN_POINT('Ctrl Pts',(-5.53275505583176,-3.89626879105743,
23.8926557189587));
#14666=CARTESIAN_POINT('Ctrl Pts',(-5.43234457257446,-4.03885305274271,
23.9008647631133));
#14667=CARTESIAN_POINT('Ctrl Pts',(-5.32633031100458,-4.17767890086226,
23.9090738072679));
#14668=CARTESIAN_POINT('Ctrl Pts',(-5.21502707051333,-4.31228265003735,
23.9172828514225));
#14669=CARTESIAN_POINT('Ctrl Pts',(-5.10379624014698,-4.44679883056443,
23.9254865550505));
#14670=CARTESIAN_POINT('Ctrl Pts',(-4.98728351227486,-4.57709810820803,
23.9336902586786));
#14671=CARTESIAN_POINT('Ctrl Pts',(-4.86584570656518,-4.70274755434536,
23.9418939623066));
#14672=CARTESIAN_POINT('Ctrl Pts',(-4.74446259179439,-4.82834041278217,
23.9500939713006));
#14673=CARTESIAN_POINT('Ctrl Pts',(-4.61815906675208,-4.94928735456051,
23.9582939802945));
#14674=CARTESIAN_POINT('Ctrl Pts',(-4.48733082216692,-5.06519013388745,
23.9664939892885));
#14675=CARTESIAN_POINT('Ctrl Pts',(-4.35651303888417,-5.18108364538367,
23.9746933425924));
#14676=CARTESIAN_POINT('Ctrl Pts',(-4.22117151899888,-5.29193355379242,
23.9828926958964));
#14677=CARTESIAN_POINT('Ctrl Pts',(-4.08173752687484,-5.39737971257365,
23.9910920492003));
#14678=CARTESIAN_POINT('Ctrl Pts',(-3.94230444381934,-5.50282518387701,
23.9992913490469));
#14679=CARTESIAN_POINT('Ctrl Pts',(-3.79877922696904,-5.60286675861065,
24.0074906488935));
#14680=CARTESIAN_POINT('Ctrl Pts',(-3.65162471579024,-5.69718579081197,
24.0156899487401));
#14681=CARTESIAN_POINT('Ctrl Pts',(-3.50444446874297,-5.7915213184791,24.0238906825631));
#14682=CARTESIAN_POINT('Ctrl Pts',(-3.35363396462095,-5.88013211618855,
24.0320914163861));
#14683=CARTESIAN_POINT('Ctrl Pts',(-3.19968343820939,-5.96274390656253,
24.0402921502092));
#14684=CARTESIAN_POINT('Ctrl Pts',(-3.04567805893446,-6.04538513167347,
24.0484958059691));
#14685=CARTESIAN_POINT('Ctrl Pts',(-2.88853074437985,-6.12202292211131,
24.0566994617291));
#14686=CARTESIAN_POINT('Ctrl Pts',(-2.72875467973028,-6.19242980564577,
24.0649031174891));
#14687=CARTESIAN_POINT('Ctrl Pts',(-2.56879558132745,-6.26291734479142,
24.0731161710641));
#14688=CARTESIAN_POINT('Ctrl Pts',(-2.40620204493545,-6.32715957189716,
24.0813292246391));
#14689=CARTESIAN_POINT('Ctrl Pts',(-2.24150651470688,-6.38497748974314,
24.0895422782141));
#14690=CARTESIAN_POINT('Ctrl Pts',(-2.076713530438,-6.44282961974831,24.0977601916372));
#14691=CARTESIAN_POINT('Ctrl Pts',(-1.90981641503736,-6.49424975748081,
24.1059781050603));
#14692=CARTESIAN_POINT('Ctrl Pts',(-1.74136087992587,-6.53910936488019,
24.1141960184834));
#14693=CARTESIAN_POINT('Ctrl Pts',(-1.5726426110025,-6.58403893813521,24.1224267490794));
#14694=CARTESIAN_POINT('Ctrl Pts',(-1.4023614145147,-6.62238745400381,24.1306574796754));
#14695=CARTESIAN_POINT('Ctrl Pts',(-1.23107259454728,-6.65407764208945,
24.1388882102714));
#14696=CARTESIAN_POINT('Ctrl Pts',(-1.07376429915945,-6.68318128977188,
24.1464471519472));
#14697=CARTESIAN_POINT('Ctrl Pts',(-0.915606438550584,-6.7066697315308,
24.154006093623));
#14698=CARTESIAN_POINT('Ctrl Pts',(-0.757030461101615,-6.72452183288628,
24.1615650352988));
#14699=CARTESIAN_POINT('Ctrl Pts',(-0.585973258148032,-6.74377904052793,
24.1697189274655));
#14700=CARTESIAN_POINT('Ctrl Pts',(-0.413900579235927,-6.75653654667477,
24.1778728196322));
#14701=CARTESIAN_POINT('Ctrl Pts',(-0.241352398616212,-6.76269458275932,
24.1860267117989));
#14702=CARTESIAN_POINT('Ctrl Pts',(-0.069014774984084,-6.76884510431939,
24.1941706539391));
#14703=CARTESIAN_POINT('Ctrl Pts',(0.103796833982148,-6.76841217302138,
24.2023145960794));
#14704=CARTESIAN_POINT('Ctrl Pts',(0.276534249552371,-6.76134733679794,
24.2104585382196));
#14705=CARTESIAN_POINT('Ctrl Pts',(0.449097234996015,-6.75428963464137,
24.2185942566125));
#14706=CARTESIAN_POINT('Ctrl Pts',(0.621585813597099,-6.74061337458658,
24.2267299750054));
#14707=CARTESIAN_POINT('Ctrl Pts',(0.79344869670889,-6.72032202842178,24.2348656933983));
#14708=CARTESIAN_POINT('Ctrl Pts',(0.965174184194921,-6.70004690415523,
24.2429949076985));
#14709=CARTESIAN_POINT('Ctrl Pts',(1.13627461073451,-6.67316726625826,24.2511241219987));
#14710=CARTESIAN_POINT('Ctrl Pts',(1.30620070905545,-6.63973860235951,24.2592533362989));
#14711=CARTESIAN_POINT('Ctrl Pts',(1.47602668918245,-6.60632963418431,24.2673777609743));
#14712=CARTESIAN_POINT('Ctrl Pts',(1.64467936110587,-6.56637939465361,24.2755021856497));
#14713=CARTESIAN_POINT('Ctrl Pts',(1.81161659440151,-6.5199949627963,24.2836266103252));
#14714=CARTESIAN_POINT('Ctrl Pts',(1.97956724357085,-6.47332894774386,24.2918003554593));
#14715=CARTESIAN_POINT('Ctrl Pts',(2.14578118558417,-6.420150409417,24.2999741005935));
#14716=CARTESIAN_POINT('Ctrl Pts',(2.30971819872949,-6.3606203189986,24.3081478457277));
#14717=CARTESIAN_POINT('Ctrl Pts',(2.472605407214,-6.3014714418595,24.3162692485899));
#14718=CARTESIAN_POINT('Ctrl Pts',(2.63324442302417,-6.2360522698325,24.324390651452));
#14719=CARTESIAN_POINT('Ctrl Pts',(2.79112226839095,-6.16457017827619,24.3325120543142));
#14720=CARTESIAN_POINT('Ctrl Pts',(2.9490123200416,-6.09308256010088,24.3406340850804));
#14721=CARTESIAN_POINT('Ctrl Pts',(3.10414044258936,-6.01553123959777,24.3487561158467));
#14722=CARTESIAN_POINT('Ctrl Pts',(3.25601552357071,-5.93217092726319,24.356878146613));
#14723=CARTESIAN_POINT('Ctrl Pts',(3.40793126725568,-5.84878829622001,24.3650023519541));
#14724=CARTESIAN_POINT('Ctrl Pts',(3.55659191443109,-5.75959375251632,24.3731265572952));
#14725=CARTESIAN_POINT('Ctrl Pts',(3.70153279346057,-5.66488693434706,24.3812507626363));
#14726=CARTESIAN_POINT('Ctrl Pts',(3.84804255721475,-5.56915498040281,24.3894629068787));
#14727=CARTESIAN_POINT('Ctrl Pts',(3.99075123289452,-5.46779093087044,24.3976750511212));
#14728=CARTESIAN_POINT('Ctrl Pts',(4.12921144831235,-5.36114743456345,24.4058871953636));
#14729=CARTESIAN_POINT('Ctrl Pts',(4.26640767456626,-5.25547747584145,24.41402437178));
#14730=CARTESIAN_POINT('Ctrl Pts',(4.39943244478516,-5.14462434278932,24.4221615481965));
#14731=CARTESIAN_POINT('Ctrl Pts',(4.52788638337047,-5.02896946692742,24.430298724613));
#14732=CARTESIAN_POINT('Ctrl Pts',(4.65811549162559,-4.91171629808941,24.4385483527684));
#14733=CARTESIAN_POINT('Ctrl Pts',(4.78364622864028,-4.78952797289121,24.4467979809238));
#14734=CARTESIAN_POINT('Ctrl Pts',(4.90410375787502,-4.66283769093415,24.4550476090793));
#14735=CARTESIAN_POINT('Ctrl Pts',(5.02456128710975,-4.53614740897711,24.4632972372347));
#14736=CARTESIAN_POINT('Ctrl Pts',(5.13994540195293,-4.40495550096769,24.4715468653901));
#14737=CARTESIAN_POINT('Ctrl Pts',(5.24992624777084,-4.26972638385258,24.4797964935456));
#14738=CARTESIAN_POINT('Ctrl Pts',(5.35957699649299,-4.13490314412902,24.4880213612232));
#14739=CARTESIAN_POINT('Ctrl Pts',(5.46418475736251,-3.99566400341141,24.4962462289007));
#14740=CARTESIAN_POINT('Ctrl Pts',(5.56337439598018,-3.85242187852683,24.5044710965783));
#14741=CARTESIAN_POINT('Ctrl Pts',(5.66245228636759,-3.7093411319291,24.5126866980219));
#14742=CARTESIAN_POINT('Ctrl Pts',(5.75612400697941,-3.5622666736126,24.5209022994654));
#14743=CARTESIAN_POINT('Ctrl Pts',(5.84405382074282,-3.41164534209833,24.529117900909));
#14744=CARTESIAN_POINT('Ctrl Pts',(5.93190223859301,-3.26116343952523,24.5373258972371));
#14745=CARTESIAN_POINT('Ctrl Pts',(6.01401915525824,-3.10714151042175,24.5455338935652));
#14746=CARTESIAN_POINT('Ctrl Pts',(6.0901113632285,-2.95005636954197,24.5537418898934));
#14747=CARTESIAN_POINT('Ctrl Pts',(6.16614841677648,-2.79308508973186,24.5619439367648));
#14748=CARTESIAN_POINT('Ctrl Pts',(6.23616930395717,-2.63305534219442,24.5701459836362));
#14749=CARTESIAN_POINT('Ctrl Pts',(6.29992607490795,-2.47046968220516,24.5783480305077));
#14750=CARTESIAN_POINT('Ctrl Pts',(6.36364943554375,-2.30796922160778,24.5865457792793));
#14751=CARTESIAN_POINT('Ctrl Pts',(6.42111508868612,-2.14291585001234,24.5947435280508));
#14752=CARTESIAN_POINT('Ctrl Pts',(6.47212263936009,-1.97583337887651,24.6029412768224));
#14753=CARTESIAN_POINT('Ctrl Pts',(6.52312046136822,-1.80878277536633,24.611137462038));
#14754=CARTESIAN_POINT('Ctrl Pts',(6.56766252380892,-1.63970418416487,24.6193336472536));
#14755=CARTESIAN_POINT('Ctrl Pts',(6.60559777384592,-1.46913819981712,24.6275298324693));
#14756=CARTESIAN_POINT('Ctrl Pts',(6.64353021751874,-1.29858483355591,24.6357254113496));
#14757=CARTESIAN_POINT('Ctrl Pts',(6.67485674338557,-1.12654464335548,24.64392099023));
#14758=CARTESIAN_POINT('Ctrl Pts',(6.69947708397811,-0.953570029548029,
24.6521165691103));
#14759=CARTESIAN_POINT('Ctrl Pts',(6.72410008259282,-0.780576741329532,
24.6603130327888));
#14760=CARTESIAN_POINT('Ctrl Pts',(6.74201540292445,-0.606649183840778,
24.6685094964672));
#14761=CARTESIAN_POINT('Ctrl Pts',(6.75317447147819,-0.432346571369847,
24.6767059601457));
#14762=CARTESIAN_POINT('Ctrl Pts',(6.76433677503846,-0.257993428687848,
24.6849047999734));
#14763=CARTESIAN_POINT('Ctrl Pts',(6.76873890255556,-0.0832653724586005,
24.6931036398012));
#14764=CARTESIAN_POINT('Ctrl Pts',(6.76638437996487,0.0912766266220258,
24.701302479629));
#14765=CARTESIAN_POINT('Ctrl Pts',(6.76402739800834,0.266000939786163,24.7095098833783));
#14766=CARTESIAN_POINT('Ctrl Pts',(6.75489967079978,0.440538448253572,24.7177172871275));
#14767=CARTESIAN_POINT('Ctrl Pts',(6.73905683212934,0.614330540776603,24.7259246908768));
#14768=CARTESIAN_POINT('Ctrl Pts',(6.72320550719611,0.788215725541392,24.7341364909458));
#14769=CARTESIAN_POINT('Ctrl Pts',(6.70063194649767,0.961354342896304,24.7423482910148));
#14770=CARTESIAN_POINT('Ctrl Pts',(6.6714432497719,1.13319634886146,24.7505600910838));
#14771=CARTESIAN_POINT('Ctrl Pts',(6.64221158320605,1.30529133027071,24.75878398007));
#14772=CARTESIAN_POINT('Ctrl Pts',(6.60634539242851,1.4760855344447,24.7670078690561));
#14773=CARTESIAN_POINT('Ctrl Pts',(6.56400246541083,1.64504122564772,24.7752317580423));
#14774=CARTESIAN_POINT('Ctrl Pts',(6.52487833286369,1.80115336344255,24.7828304892923));
#14775=CARTESIAN_POINT('Ctrl Pts',(6.48022534294035,1.95569583815561,24.7904292205423));
#14776=CARTESIAN_POINT('Ctrl Pts',(6.43020461554308,2.10825937736523,24.7980279517924));
#14777=CARTESIAN_POINT('Ctrl Pts',(6.37605374060706,2.27341989304355,24.8062541005711));
#14778=CARTESIAN_POINT('Ctrl Pts',(6.31545951335835,2.43672459867157,24.8144802493499));
#14779=CARTESIAN_POINT('Ctrl Pts',(6.24856658841284,2.59763442196371,24.8227063981287));
#14780=CARTESIAN_POINT('Ctrl Pts',(6.18175110838258,2.75835795279459,24.8309230231291));
#14781=CARTESIAN_POINT('Ctrl Pts',(6.10865158953743,2.91669179442607,24.8391396481294));
#14782=CARTESIAN_POINT('Ctrl Pts',(6.02946253448876,3.07211174035001,24.8473562731298));
#14783=CARTESIAN_POINT('Ctrl Pts',(5.94985305419825,3.22835683147,24.8556165212868));
#14784=CARTESIAN_POINT('Ctrl Pts',(5.8640892762609,3.38165663939372,24.8638767694438));
#14785=CARTESIAN_POINT('Ctrl Pts',(5.77241866115026,3.53149710468582,24.8721370176008));
#14786=CARTESIAN_POINT('Ctrl Pts',(5.68139864332798,3.68027413432529,24.8803386417915));
#14787=CARTESIAN_POINT('Ctrl Pts',(5.58455554029678,3.82564044827875,24.8885402659822));
#14788=CARTESIAN_POINT('Ctrl Pts',(5.48217835860883,3.96711601095821,24.8967418901729));
#14789=CARTESIAN_POINT('Ctrl Pts',(5.37985045323717,4.10852347843854,24.9049395667473));
#14790=CARTESIAN_POINT('Ctrl Pts',(5.27199398363578,4.24604363414918,24.9131372433217));
#14791=CARTESIAN_POINT('Ctrl Pts',(5.15894156231535,4.37922492646989,24.9213349198962));
#14792=CARTESIAN_POINT('Ctrl Pts',(5.04592298669535,4.51236634689694,24.9295301422454));
#14793=CARTESIAN_POINT('Ctrl Pts',(4.92771179009345,4.64117121842162,24.9377253645945));
#14794=CARTESIAN_POINT('Ctrl Pts',(4.80468123110802,4.76522058958852,24.9459205869437));
#14795=CARTESIAN_POINT('Ctrl Pts',(4.67997556310149,4.89095894130153,24.9542273904399));
#14796=CARTESIAN_POINT('Ctrl Pts',(4.5503185772531,5.01181105886853,24.9625341939361));
#14797=CARTESIAN_POINT('Ctrl Pts',(4.4161382224553,5.12737868702608,24.9708409974323));
#14798=CARTESIAN_POINT('Ctrl Pts',(4.28373757719628,5.24141347671026,24.9790376231201));
#14799=CARTESIAN_POINT('Ctrl Pts',(4.14693311670552,5.35030288602503,24.9872342488079));
#14800=CARTESIAN_POINT('Ctrl Pts',(4.00616969368798,5.45370455611376,24.9954308744957));
#14801=CARTESIAN_POINT('Ctrl Pts',(3.86256808956303,5.5591910907236,25.0037927668961));
#14802=CARTESIAN_POINT('Ctrl Pts',(3.71484648524175,5.65896599588524,25.0121546592965));
#14803=CARTESIAN_POINT('Ctrl Pts',(3.563508406535,5.75271212877495,25.0205165516968));
#14804=CARTESIAN_POINT('Ctrl Pts',(3.41217032782821,5.84645826166468,25.0288784440972));
#14805=CARTESIAN_POINT('Ctrl Pts',(3.25721612815034,5.93417544472269,25.0372403364976));
#14806=CARTESIAN_POINT('Ctrl Pts',(3.09917575053259,6.01559628526639,25.045602228898));
#14807=CARTESIAN_POINT('Ctrl Pts',(3.09917575053259,6.01559628526639,23.0457515827422));
#14808=CARTESIAN_POINT('Ctrl Pts',(2.93382384459267,6.10078395293758,23.0545010306546));
#14809=CARTESIAN_POINT('Ctrl Pts',(2.76495772122987,6.17915010267048,23.063250478567));
#14810=CARTESIAN_POINT('Ctrl Pts',(2.59315093316716,6.25042856433175,23.0719999264794));
#14811=CARTESIAN_POINT('Ctrl Pts',(2.42134553245622,6.32170645041449,23.0807493037394));
#14812=CARTESIAN_POINT('Ctrl Pts',(2.24659977927596,6.38589665313456,23.0894986809994));
#14813=CARTESIAN_POINT('Ctrl Pts',(2.06950718689924,6.44278115439073,23.0982480582594));
#14814=CARTESIAN_POINT('Ctrl Pts',(1.89241596572858,6.49966521519725,23.1069973677741));
#14815=CARTESIAN_POINT('Ctrl Pts',(1.71297821457185,6.5492436000955,23.1157466772887));
#14816=CARTESIAN_POINT('Ctrl Pts',(1.53180337335822,6.59134792173561,23.1244959868034));
#14817=CARTESIAN_POINT('Ctrl Pts',(1.35062987477754,6.63345193135311,23.1332452314795));
#14818=CARTESIAN_POINT('Ctrl Pts',(1.16771959102918,6.66808192368244,23.1419944761557));
#14819=CARTESIAN_POINT('Ctrl Pts',(0.983693746906448,6.69512028363174,23.1507437208318));
#14820=CARTESIAN_POINT('Ctrl Pts',(0.799669205419473,6.72215845218872,23.159492903576));
#14821=CARTESIAN_POINT('Ctrl Pts',(0.614529402873077,6.74160505424583,23.1682420863201));
#14822=CARTESIAN_POINT('Ctrl Pts',(0.428903127362849,6.75339404354125,23.1769912690643));
#14823=CARTESIAN_POINT('Ctrl Pts',(0.243278104163375,6.76518295330332,23.1857403927829));
#14824=CARTESIAN_POINT('Ctrl Pts',(0.0571669005385083,6.76931433552277,
23.1944895165015));
#14825=CARTESIAN_POINT('Ctrl Pts',(-0.128798404778226,6.76577415902472,
23.2032386402201));
#14826=CARTESIAN_POINT('Ctrl Pts',(-0.314762517259805,6.76223400523438,
23.2119877078194));
#14827=CARTESIAN_POINT('Ctrl Pts',(-0.500580446820209,6.75102239665084,
23.2207367754186));
#14828=CARTESIAN_POINT('Ctrl Pts',(-0.685621118843303,6.7321774101249,23.2294858430178));
#14829=CARTESIAN_POINT('Ctrl Pts',(-0.870660665415034,6.71333253821764,
23.2382348574035));
#14830=CARTESIAN_POINT('Ctrl Pts',(-1.05492267885527,6.68685441030605,23.2469838717893));
#14831=CARTESIAN_POINT('Ctrl Pts',(-1.23778137635278,6.65283295028172,23.2557328861751));
#14832=CARTESIAN_POINT('Ctrl Pts',(-1.42999922978873,6.6170701886186,23.2649296965425));
#14833=CARTESIAN_POINT('Ctrl Pts',(-1.62066601233722,6.57297172934407,23.2741265069099));
#14834=CARTESIAN_POINT('Ctrl Pts',(-1.80906628500412,6.52070304311287,23.2833233172773));
#14835=CARTESIAN_POINT('Ctrl Pts',(-1.98831342545551,6.47097374915023,23.292073315015));
#14836=CARTESIAN_POINT('Ctrl Pts',(-2.16550875896721,6.41384933989522,23.3008233127528));
#14837=CARTESIAN_POINT('Ctrl Pts',(-2.34005036714027,6.3495238624047,23.3095733104905));
#14838=CARTESIAN_POINT('Ctrl Pts',(-2.51458843547106,6.28519968948589,23.3183231307714));
#14839=CARTESIAN_POINT('Ctrl Pts',(-2.68647261718074,6.21367483971091,23.3270729510523));
#14840=CARTESIAN_POINT('Ctrl Pts',(-2.85511905908751,6.13519226743834,23.3358227713331));
#14841=CARTESIAN_POINT('Ctrl Pts',(-3.023762304889,6.05671118252929,23.3445724257917));
#14842=CARTESIAN_POINT('Ctrl Pts',(-3.18916767379916,5.97127275992626,23.3533220802502));
#14843=CARTESIAN_POINT('Ctrl Pts',(-3.35077334102795,5.87916720437992,23.3620717347087));
#14844=CARTESIAN_POINT('Ctrl Pts',(-3.5123761603737,5.78706327195642,23.3708212349772));
#14845=CARTESIAN_POINT('Ctrl Pts',(-3.67017916302295,5.68829258362301,23.3795707352456));
#14846=CARTESIAN_POINT('Ctrl Pts',(-3.82364636566452,5.58319061741049,23.3883202355141));
#14847=CARTESIAN_POINT('Ctrl Pts',(-3.97711106778796,5.47809036367704,23.3970695932225));
#14848=CARTESIAN_POINT('Ctrl Pts',(-4.12623987481933,5.36665920043221,23.4058189509309));
#14849=CARTESIAN_POINT('Ctrl Pts',(-4.27052628213943,5.24927559512324,23.4145683086394));
#14850=CARTESIAN_POINT('Ctrl Pts',(-4.41481053025014,5.13189374643006,23.4233175354159));
#14851=CARTESIAN_POINT('Ctrl Pts',(-4.55425230136587,5.00855981477302,23.4320667621924));
#14852=CARTESIAN_POINT('Ctrl Pts',(-4.68837800630624,4.87969268192003,23.440815988969));
#14853=CARTESIAN_POINT('Ctrl Pts',(-4.82250188228972,4.75082730631731,23.4495650964398));
#14854=CARTESIAN_POINT('Ctrl Pts',(-4.95130963053044,4.61642907903442,23.4583142039107));
#14855=CARTESIAN_POINT('Ctrl Pts',(-5.07436379033446,4.476954447316,23.4670633113815));
#14856=CARTESIAN_POINT('Ctrl Pts',(-5.19741643562872,4.33748153220506,23.4758123111713));
#14857=CARTESIAN_POINT('Ctrl Pts',(-5.31471544462827,4.1929325525452,23.484561310961));
#14858=CARTESIAN_POINT('Ctrl Pts',(-5.42586245275671,4.04379841779545,23.4933103107507));
#14859=CARTESIAN_POINT('Ctrl Pts',(-5.53702160019195,3.89464799484283,23.5020602660929));
#14860=CARTESIAN_POINT('Ctrl Pts',(-5.64202723081293,3.74091164443788,23.510810221435));
#14861=CARTESIAN_POINT('Ctrl Pts',(-5.74052265233007,3.58311159163169,23.5195601767772));
#14862=CARTESIAN_POINT('Ctrl Pts',(-5.83901427066957,3.42531763191717,23.5283097942597));
#14863=CARTESIAN_POINT('Ctrl Pts',(-5.93099603115777,3.26346052695544,23.5370594117421));
#14864=CARTESIAN_POINT('Ctrl Pts',(-6.0161555062279,3.09809004467005,23.5458090292246));
#14865=CARTESIAN_POINT('Ctrl Pts',(-6.10131214578841,2.93272506863742,23.5545583553757));
#14866=CARTESIAN_POINT('Ctrl Pts',(-6.17964682328794,2.76384720416793,23.5633076815268));
#14867=CARTESIAN_POINT('Ctrl Pts',(-6.25089348288613,2.59203002791476,23.5720570076779));
#14868=CARTESIAN_POINT('Ctrl Pts',(-6.32213814889384,2.4202176593689,23.5808060890094));
#14869=CARTESIAN_POINT('Ctrl Pts',(-6.38629508412642,2.24546640831757,23.589555170341));
#14870=CARTESIAN_POINT('Ctrl Pts',(-6.4431463981987,2.06836976659859,23.5983042516726));
#14871=CARTESIAN_POINT('Ctrl Pts',(-6.50000285283756,1.89125711158086,23.607054124107));
#14872=CARTESIAN_POINT('Ctrl Pts',(-6.54955227673301,1.71179891440059,23.6158039965414));
#14873=CARTESIAN_POINT('Ctrl Pts',(-6.59162635926432,1.53060476278229,23.6245538689758));
#14874=CARTESIAN_POINT('Ctrl Pts',(-6.63369752055239,1.34942319164485,23.6333031338983));
#14875=CARTESIAN_POINT('Ctrl Pts',(-6.66829431424292,1.16650618642485,23.6420523988208));
#14876=CARTESIAN_POINT('Ctrl Pts',(-6.69529923745451,0.982474997616288,
23.6508016637433));
#14877=CARTESIAN_POINT('Ctrl Pts',(-6.72230554731471,0.798434359175432,
23.659551377923));
#14878=CARTESIAN_POINT('Ctrl Pts',(-6.74171916496724,0.613279706237988,
23.6683010921027));
#14879=CARTESIAN_POINT('Ctrl Pts',(-6.7534741481729,0.427639953652993,23.6770508062824));
#14880=CARTESIAN_POINT('Ctrl Pts',(-6.7624883775875,0.285283364196907,23.6837604654583));
#14881=CARTESIAN_POINT('Ctrl Pts',(-6.76699999999997,0.142641701104177,
23.6904701246341));
#14882=CARTESIAN_POINT('Ctrl Pts',(-6.767,1.35195985046293E-12,23.69717978381));
#14883=CARTESIAN_POINT('',(-6.76699789935467,0.00533199113308135,23.302820216162));
#14884=CARTESIAN_POINT('Ctrl Pts',(3.09917575053257,6.0155962852664,22.6516519666359));
#14885=CARTESIAN_POINT('Ctrl Pts',(2.94533715167372,6.09485241092214,22.6597798083722));
#14886=CARTESIAN_POINT('Ctrl Pts',(2.78834244546162,6.16826210053875,22.6679076501086));
#14887=CARTESIAN_POINT('Ctrl Pts',(2.62868129189148,6.23556923349102,22.6760354918449));
#14888=CARTESIAN_POINT('Ctrl Pts',(2.46909412599147,6.30284517602633,22.6841595671042));
#14889=CARTESIAN_POINT('Ctrl Pts',(2.30684331009307,6.36402405269745,22.6922836423634));
#14890=CARTESIAN_POINT('Ctrl Pts',(2.14244081522303,6.41889681746533,22.7004077176227));
#14891=CARTESIAN_POINT('Ctrl Pts',(1.97805439270852,6.47376421774902,22.7085309986542));
#14892=CARTESIAN_POINT('Ctrl Pts',(1.81151705421439,6.5223266105014,22.7166542796857));
#14893=CARTESIAN_POINT('Ctrl Pts',(1.64335859477935,6.56442392971119,22.7247775607172));
#14894=CARTESIAN_POINT('Ctrl Pts',(1.47520027491876,6.60652121397947,22.7329008350062));
#14895=CARTESIAN_POINT('Ctrl Pts',(1.30542119148423,6.64215334585694,22.7410241092953));
#14896=CARTESIAN_POINT('Ctrl Pts',(1.13456388177708,6.67121081949648,22.7491473835843));
#14897=CARTESIAN_POINT('Ctrl Pts',(0.963674209275419,6.7002737970331,22.7572721965366));
#14898=CARTESIAN_POINT('Ctrl Pts',(0.791706264416511,6.72275957520087,22.7653970094888));
#14899=CARTESIAN_POINT('Ctrl Pts',(0.619210258008934,6.7386102169792,22.773521822441));
#14900=CARTESIAN_POINT('Ctrl Pts',(0.446648759875735,6.75446687678603,22.7816497201489));
#14901=CARTESIAN_POINT('Ctrl Pts',(0.273559164896786,6.76368335065464,22.7897776178567));
#14902=CARTESIAN_POINT('Ctrl Pts',(0.100494212842556,6.76625375767013,22.7979055155646));
#14903=CARTESIAN_POINT('Ctrl Pts',(-0.0727613266221251,6.76882699534089,
22.8060423641025));
#14904=CARTESIAN_POINT('Ctrl Pts',(-0.245991803204344,6.7647395454642,22.8141792126404));
#14905=CARTESIAN_POINT('Ctrl Pts',(-0.418646239134824,6.75403763140673,
22.8223160611783));
#14906=CARTESIAN_POINT('Ctrl Pts',(-0.591409460085532,6.74332897435462,
22.8304580365305));
#14907=CARTESIAN_POINT('Ctrl Pts',(-0.76359555454526,6.72599758616071,22.8386000118827));
#14908=CARTESIAN_POINT('Ctrl Pts',(-0.934661545511393,6.70214120974352,
22.846741987235));
#14909=CARTESIAN_POINT('Ctrl Pts',(-1.10596394295794,6.67825186475114,22.8548952144773));
#14910=CARTESIAN_POINT('Ctrl Pts',(-1.27614278741816,6.64781958978234,22.8630484417197));
#14911=CARTESIAN_POINT('Ctrl Pts',(-1.44466726065743,6.61099277763821,22.871201668962));
#14912=CARTESIAN_POINT('Ctrl Pts',(-1.51786797138082,6.59499659161958,22.8747431250922));
#14913=CARTESIAN_POINT('Ctrl Pts',(-1.59075676567098,6.5777945740722,22.8782845812223));
#14914=CARTESIAN_POINT('Ctrl Pts',(-1.66329124058518,6.5594017447472,22.8818260373524));
#14915=CARTESIAN_POINT('Ctrl Pts',(-1.83177667506952,6.51667828333269,22.8900522466894));
#14916=CARTESIAN_POINT('Ctrl Pts',(-1.9988504768118,6.46739932862912,22.8982784560264));
#14917=CARTESIAN_POINT('Ctrl Pts',(-2.16396505822729,6.41167249840253,22.9065046653633));
#14918=CARTESIAN_POINT('Ctrl Pts',(-2.32889414048451,6.35600827488222,22.9147216329066));
#14919=CARTESIAN_POINT('Ctrl Pts',(-2.49186804868475,6.2939107140796,22.9229386004498));
#14920=CARTESIAN_POINT('Ctrl Pts',(-2.65235058016763,6.2255381614672,22.931155567993));
#14921=CARTESIAN_POINT('Ctrl Pts',(-2.81268502653112,6.15722869956956,22.9393649533364));
#14922=CARTESIAN_POINT('Ctrl Pts',(-2.97053234668703,6.08265591703279,22.9475743386798));
#14923=CARTESIAN_POINT('Ctrl Pts',(-3.12537258853758,6.00202758930829,22.9557837240232));
#14924=CARTESIAN_POINT('Ctrl Pts',(-3.28010101938799,5.92145748374784,22.9639871813238));
#14925=CARTESIAN_POINT('Ctrl Pts',(-3.43182638023916,5.83484070771945,22.9721906386244));
#14926=CARTESIAN_POINT('Ctrl Pts',(-3.58004968407034,5.74243269525972,22.980394095925));
#14927=CARTESIAN_POINT('Ctrl Pts',(-3.72819568826127,5.65007287431871,22.9885932750569));
#14928=CARTESIAN_POINT('Ctrl Pts',(-3.87284297023566,5.55192802295851,22.9967924541887));
#14929=CARTESIAN_POINT('Ctrl Pts',(-4.01351802524722,5.44829900620512,23.0049916333206));
#14930=CARTESIAN_POINT('Ctrl Pts',(-4.15416657404645,5.34468951539199,23.0131892675504));
#14931=CARTESIAN_POINT('Ctrl Pts',(-4.29084409458544,5.23559812496321,23.0213869017803));
#14932=CARTESIAN_POINT('Ctrl Pts',(-4.42310666570275,5.12136860846941,23.0295845360101));
#14933=CARTESIAN_POINT('Ctrl Pts',(-4.55535968996264,5.00714733718738,23.0377815785257));
#14934=CARTESIAN_POINT('Ctrl Pts',(-4.6831981274305,4.88778891223321,23.0459786210413));
#14935=CARTESIAN_POINT('Ctrl Pts',(-4.80621176726464,4.76367688327062,23.0541756635569));
#14936=CARTESIAN_POINT('Ctrl Pts',(-4.9292388853625,4.63955125569686,23.0623736041997));
#14937=CARTESIAN_POINT('Ctrl Pts',(-5.04743990007538,4.51067124125496,23.0705715448425));
#14938=CARTESIAN_POINT('Ctrl Pts',(-5.16044201700532,4.377456703284,23.0787694854853));
#14939=CARTESIAN_POINT('Ctrl Pts',(-5.27347705328596,4.24420335775606,23.0869698143213));
#14940=CARTESIAN_POINT('Ctrl Pts',(-5.38130994307094,4.1066132469765,23.0951701431573));
#14941=CARTESIAN_POINT('Ctrl Pts',(-5.4836086502579,3.96513873285876,23.1033704719933));
#14942=CARTESIAN_POINT('Ctrl Pts',(-5.58601395535202,3.82351679862657,23.1115793457847));
#14943=CARTESIAN_POINT('Ctrl Pts',(-5.68287334628282,3.67800266550344,23.1197882195761));
#14944=CARTESIAN_POINT('Ctrl Pts',(-5.77389800980859,3.52907789264113,23.1279970933675));
#14945=CARTESIAN_POINT('Ctrl Pts',(-5.86497152526677,3.3800731934967,23.1362103727709));
#14946=CARTESIAN_POINT('Ctrl Pts',(-5.95020389580566,3.22765451829543,23.1444236521743));
#14947=CARTESIAN_POINT('Ctrl Pts',(-6.02935271589693,3.07232726565812,23.1526369315777));
#14948=CARTESIAN_POINT('Ctrl Pts',(-6.10861730357792,2.91677282250004,23.1608622241931));
#14949=CARTESIAN_POINT('Ctrl Pts',(-6.181780408104,2.75830162568904,23.1690875168086));
#14950=CARTESIAN_POINT('Ctrl Pts',(-6.24864764491561,2.59743943330554,23.177312809424));
#14951=CARTESIAN_POINT('Ctrl Pts',(-6.30912102822251,2.45195890377503,23.184751598536));
#14952=CARTESIAN_POINT('Ctrl Pts',(-6.36444557725428,2.304523182898,23.192190387648));
#14953=CARTESIAN_POINT('Ctrl Pts',(-6.41451305705658,2.15553038504463,23.1996291767601));
#14954=CARTESIAN_POINT('Ctrl Pts',(-6.47963464030889,1.96173898736063,23.2093046332913));
#14955=CARTESIAN_POINT('Ctrl Pts',(-6.53601141367244,1.764872190024,23.2189800898225));
#14956=CARTESIAN_POINT('Ctrl Pts',(-6.58338801998961,1.56565998168735,23.2286555463537));
#14957=CARTESIAN_POINT('Ctrl Pts',(-6.6305625635036,1.36729742005137,23.2382897367407));
#14958=CARTESIAN_POINT('Ctrl Pts',(-6.66881347663304,1.16660948169976,23.2479239271277));
#14959=CARTESIAN_POINT('Ctrl Pts',(-6.69793560061278,0.964337954269142,
23.2575581175147));
#14960=CARTESIAN_POINT('Ctrl Pts',(-6.72681638638656,0.763742672966011,
23.2671124683191));
#14961=CARTESIAN_POINT('Ctrl Pts',(-6.74671899741591,0.561590026758002,
23.2766668191235));
#14962=CARTESIAN_POINT('Ctrl Pts',(-6.75749054399143,0.358623127902209,
23.2862211699278));
#14963=CARTESIAN_POINT('Ctrl Pts',(-6.76372844904924,0.241083066587632,
23.2917541853392));
#14964=CARTESIAN_POINT('Ctrl Pts',(-6.76690497100265,0.123270289833604,
23.2972872007506));
#14965=CARTESIAN_POINT('Ctrl Pts',(-6.76699789935467,0.00533199113308068,
23.302820216162));
#14966=CARTESIAN_POINT('Ctrl Pts',(-6.76699789935514,0.00533199053770156,
23.3028202161899));
#14967=CARTESIAN_POINT('Ctrl Pts',(-6.76713557607511,-0.169397890966532,
23.3110175798778));
#14968=CARTESIAN_POINT('Ctrl Pts',(-6.76050144710687,-0.344207078147022,
23.3192149435658));
#14969=CARTESIAN_POINT('Ctrl Pts',(-6.74710394238392,-0.518533885746455,
23.3274123072538));
#14970=CARTESIAN_POINT('Ctrl Pts',(-6.73370718007129,-0.692851033187286,
23.3356092166924));
#14971=CARTESIAN_POINT('Ctrl Pts',(-6.71354780721192,-0.866685496773059,
23.343806126131));
#14972=CARTESIAN_POINT('Ctrl Pts',(-6.68668630651549,-1.03947834910508,
23.3520030355696));
#14973=CARTESIAN_POINT('Ctrl Pts',(-6.6598244339166,-1.21227359378621,23.360200058496));
#14974=CARTESIAN_POINT('Ctrl Pts',(-6.62626030277704,-1.38402684436315,
23.3683970814224));
#14975=CARTESIAN_POINT('Ctrl Pts',(-6.58610592683122,-1.55418715750668,
23.3765941043487));
#14976=CARTESIAN_POINT('Ctrl Pts',(-6.54594372530683,-1.72438063273699,
23.3847927247709));
#14977=CARTESIAN_POINT('Ctrl Pts',(-6.49918880253525,-1.89298020342746,
23.3929913451931));
#14978=CARTESIAN_POINT('Ctrl Pts',(-6.44600368172677,-2.05944787143666,
23.4011899656152));
#14979=CARTESIAN_POINT('Ctrl Pts',(-6.39279856696449,-2.22597811985954,
23.4093916681558));
#14980=CARTESIAN_POINT('Ctrl Pts',(-6.33315854772807,-2.39037452811281,
23.4175933706963));
#14981=CARTESIAN_POINT('Ctrl Pts',(-6.26729514571851,-2.55211687750645,
23.4257950732368));
#14982=CARTESIAN_POINT('Ctrl Pts',(-6.20135727800738,-2.71404209412457,
23.4340060486894));
#14983=CARTESIAN_POINT('Ctrl Pts',(-6.12918210721176,-2.87330692569047,
23.442217024142));
#14984=CARTESIAN_POINT('Ctrl Pts',(-6.05102862629684,-3.02941274238691,
23.4504279995946));
#14985=CARTESIAN_POINT('Ctrl Pts',(-5.97282751887836,-3.18561368951322,
23.4586439787917));
#14986=CARTESIAN_POINT('Ctrl Pts',(-5.88864101160007,-3.33865147122337,
23.4668599579887));
#14987=CARTESIAN_POINT('Ctrl Pts',(-5.79877265229455,-3.48805457626466,
23.4750759371858));
#14988=CARTESIAN_POINT('Ctrl Pts',(-5.70877164640232,-3.63767820176588,
23.4833040432494));
#14989=CARTESIAN_POINT('Ctrl Pts',(-5.6130722286129,-3.78365613277414,23.4915321493131));
#14990=CARTESIAN_POINT('Ctrl Pts',(-5.51202031121251,-3.92554723430768,
23.4997602553767));
#14991=CARTESIAN_POINT('Ctrl Pts',(-5.43967496168524,-4.02713027794834,
23.505650942307));
#14992=CARTESIAN_POINT('Ctrl Pts',(-5.36458708274533,-4.12661930799459,
23.5115416292374));
#14993=CARTESIAN_POINT('Ctrl Pts',(-5.28689545463958,-4.22386380600883,
23.5174323161678));
#14994=CARTESIAN_POINT('Ctrl Pts',(-5.17937227900346,-4.35844764077412,
23.525584872381));
#14995=CARTESIAN_POINT('Ctrl Pts',(-5.0665385954702,-4.48913361742515,23.5337374285943));
#14996=CARTESIAN_POINT('Ctrl Pts',(-4.94870871398186,-4.61547083883757,
23.5418899848075));
#14997=CARTESIAN_POINT('Ctrl Pts',(-4.83101534125174,-4.74166169553339,
23.5500330960879));
#14998=CARTESIAN_POINT('Ctrl Pts',(-4.70833753934842,-4.86351356128222,
23.5581762073682));
#14999=CARTESIAN_POINT('Ctrl Pts',(-4.58103149679524,-4.98060633109765,
23.5663193186486));
#15000=CARTESIAN_POINT('Ctrl Pts',(-4.45384617685171,-5.09758806341274,
23.5744547079259));
#15001=CARTESIAN_POINT('Ctrl Pts',(-4.32204162120189,-5.20981943880274,
23.5825900972033));
#15002=CARTESIAN_POINT('Ctrl Pts',(-4.18601269475671,-5.31691515066168,
23.5907254864806));
#15003=CARTESIAN_POINT('Ctrl Pts',(-4.05008417975476,-5.42393180848944,
23.5988548705192));
#15004=CARTESIAN_POINT('Ctrl Pts',(-3.90993778899949,-5.52582012606068,
23.6069842545578));
#15005=CARTESIAN_POINT('Ctrl Pts',(-3.76600347417976,-5.62223326023263,
23.6151136385964));
#15006=CARTESIAN_POINT('Ctrl Pts',(-3.6221451731738,-5.71859547722034,23.6232387293886));
#15007=CARTESIAN_POINT('Ctrl Pts',(-3.47450323514168,-5.80948806641062,
23.6313638201807));
#15008=CARTESIAN_POINT('Ctrl Pts',(-3.32353875816129,-5.89460593449636,
23.6394889109729));
#15009=CARTESIAN_POINT('Ctrl Pts',(-3.17199801704549,-5.98004871593683,
23.647645016998));
#15010=CARTESIAN_POINT('Ctrl Pts',(-3.0171096184973,-6.05967237844505,23.6558011230231));
#15011=CARTESIAN_POINT('Ctrl Pts',(-2.85936768841479,-6.13321330319185,
23.6639572290482));
#15012=CARTESIAN_POINT('Ctrl Pts',(-2.70226064107286,-6.2064582390166,23.6720805082216));
#15013=CARTESIAN_POINT('Ctrl Pts',(-2.54232333238472,-6.27366917390214,
23.680203787395));
#15014=CARTESIAN_POINT('Ctrl Pts',(-2.38006652956413,-6.33463276874426,
23.6883270665684));
#15015=CARTESIAN_POINT('Ctrl Pts',(-2.21778812087925,-6.39560448140415,
23.6964514274251));
#15016=CARTESIAN_POINT('Ctrl Pts',(-2.05318994535597,-6.45032706837799,
23.7045757882818));
#15017=CARTESIAN_POINT('Ctrl Pts',(-1.88680045021287,-6.49863624625017,
23.7127001491384));
#15018=CARTESIAN_POINT('Ctrl Pts',(-1.72035714244404,-6.54696104796751,
23.7208271375239));
#15019=CARTESIAN_POINT('Ctrl Pts',(-1.552121712547,-6.58886820827906,23.7289541259094));
#15020=CARTESIAN_POINT('Ctrl Pts',(-1.38263534055174,-6.62424399573698,
23.7370811142948));
#15021=CARTESIAN_POINT('Ctrl Pts',(-1.21205325845893,-6.65984848363298,
23.7452606427349));
#15022=CARTESIAN_POINT('Ctrl Pts',(-1.04020437169081,-6.68883677994144,
23.7534401711749));
#15023=CARTESIAN_POINT('Ctrl Pts',(-0.867647383137596,-6.7111457306882,
23.761619699615));
#15024=CARTESIAN_POINT('Ctrl Pts',(-0.695903021073178,-6.73334962139384,
23.7697607080187));
#15025=CARTESIAN_POINT('Ctrl Pts',(-0.523457581893076,-6.7489369726926,
23.7779017164223));
#15026=CARTESIAN_POINT('Ctrl Pts',(-0.350863250401583,-6.75789789649989,
23.786042724826));
#15027=CARTESIAN_POINT('Ctrl Pts',(-0.177043946597487,-6.76692241963553,
23.7942415132843));
#15028=CARTESIAN_POINT('Ctrl Pts',(-0.00307400670362995,-6.76922610362182,
23.8024403017425));
#15029=CARTESIAN_POINT('Ctrl Pts',(0.17048681583121,-6.76485204905678,23.8106390902007));
#15030=CARTESIAN_POINT('Ctrl Pts',(0.34404763836605,-6.76047799449174,23.818837878659));
#15031=CARTESIAN_POINT('Ctrl Pts',(0.517198977055867,-6.74942628968219,
23.8270366671172));
#15032=CARTESIAN_POINT('Ctrl Pts',(0.689390928840013,-6.73179241712288,
23.8352354555755));
#15033=CARTESIAN_POINT('Ctrl Pts',(0.862302448461131,-6.71408485489688,
23.8434685057075));
#15034=CARTESIAN_POINT('Ctrl Pts',(1.03478406018257,-6.68968507259293,23.8517015558395));
#15035=CARTESIAN_POINT('Ctrl Pts',(1.20627809779211,-6.65861713502038,23.8599346059715));
#15036=CARTESIAN_POINT('Ctrl Pts',(1.3775679123646,-6.62758619458578,23.8681578518063));
#15037=CARTESIAN_POINT('Ctrl Pts',(1.54787214564144,-6.58990297409811,23.8763810976412));
#15038=CARTESIAN_POINT('Ctrl Pts',(1.71663670563642,-6.54564339242994,23.8846043434761));
#15039=CARTESIAN_POINT('Ctrl Pts',(1.88523407157315,-6.50142765846935,23.8928194425896));
#15040=CARTESIAN_POINT('Ctrl Pts',(2.05229445788805,-6.45064862859255,23.9010345417031));
#15041=CARTESIAN_POINT('Ctrl Pts',(2.21727234799183,-6.39343353252623,23.9092496408166));
#15042=CARTESIAN_POINT('Ctrl Pts',(2.38211980422056,-6.33626367153163,23.9174582449555));
#15043=CARTESIAN_POINT('Ctrl Pts',(2.54488770675343,-6.2726679963467,23.9256668490944));
#15044=CARTESIAN_POINT('Ctrl Pts',(2.70504403829243,-6.20282401418085,23.9338754532333));
#15045=CARTESIAN_POINT('Ctrl Pts',(2.86510578368002,-6.13302128092104,23.9420792094822));
#15046=CARTESIAN_POINT('Ctrl Pts',(3.02255870322167,-6.05697773478686,23.9502829657311));
#15047=CARTESIAN_POINT('Ctrl Pts',(3.17688907735988,-5.97491964717112,23.95848672198));
#15048=CARTESIAN_POINT('Ctrl Pts',(3.33117378903145,-5.89288583847462,23.9666880509443));
#15049=CARTESIAN_POINT('Ctrl Pts',(3.48233747797266,-5.80484119763091,23.9748893799086));
#15050=CARTESIAN_POINT('Ctrl Pts',(3.62988921017095,-5.71105886170722,23.9830907088729));
#15051=CARTESIAN_POINT('Ctrl Pts',(3.77742059357683,-5.6172894592629,23.9912909067956));
#15052=CARTESIAN_POINT('Ctrl Pts',(3.92134070962703,-5.51778412914224,23.9994911047183));
#15053=CARTESIAN_POINT('Ctrl Pts',(4.06118589512329,-5.41286043836821,24.007691302641));
#15054=CARTESIAN_POINT('Ctrl Pts',(4.20103713742628,-5.30793220326529,24.0158918557209));
#15055=CARTESIAN_POINT('Ctrl Pts',(4.33681281092668,-5.19758535496905,24.0240924088007));
#15056=CARTESIAN_POINT('Ctrl Pts',(4.46808070948705,-5.08217903792357,24.0322929618806));
#15057=CARTESIAN_POINT('Ctrl Pts',(4.59937808167961,-4.96674680865295,24.0404953562338));
#15058=CARTESIAN_POINT('Ctrl Pts',(4.72616539402512,-4.84625308455035,24.048697750587));
#15059=CARTESIAN_POINT('Ctrl Pts',(4.8480457783765,-4.72109533167525,24.0569001449402));
#15060=CARTESIAN_POINT('Ctrl Pts',(4.97004014231265,-4.59582053429968,24.065110209974));
#15061=CARTESIAN_POINT('Ctrl Pts',(5.08711815984872,-4.46587325088116,24.0733202750079));
#15062=CARTESIAN_POINT('Ctrl Pts',(5.19892127951334,-4.33168633783927,24.0815303400417));
#15063=CARTESIAN_POINT('Ctrl Pts',(5.3107779061677,-4.19743520532121,24.089744334267));
#15064=CARTESIAN_POINT('Ctrl Pts',(5.41735438318175,-4.05894068144835,24.0979583284923));
#15065=CARTESIAN_POINT('Ctrl Pts',(5.51833438096683,-3.91666626863197,24.1061723227177));
#15066=CARTESIAN_POINT('Ctrl Pts',(5.61945204812114,-3.77419788840521,24.1143975153528));
#15067=CARTESIAN_POINT('Ctrl Pts',(5.7149577917135,-3.62793962047484,24.122622707988));
#15068=CARTESIAN_POINT('Ctrl Pts',(5.80457966436447,-3.47838237116717,24.1308479006232));
#15069=CARTESIAN_POINT('Ctrl Pts',(5.88517642248584,-3.34388585718901,24.1382447987432));
#15070=CARTESIAN_POINT('Ctrl Pts',(5.96101520657425,-3.20672183596591,24.1456416968632));
#15071=CARTESIAN_POINT('Ctrl Pts',(6.03193127058848,-3.06726166912717,24.1530385949831));
#15072=CARTESIAN_POINT('Ctrl Pts',(6.11482249109594,-2.90425172769677,24.161684561474));
#15073=CARTESIAN_POINT('Ctrl Pts',(6.19117579758961,-2.7377344975215,24.1703305279649));
#15074=CARTESIAN_POINT('Ctrl Pts',(6.26070146200113,-2.56824963811873,24.1789764944558));
#15075=CARTESIAN_POINT('Ctrl Pts',(6.3301381936358,-2.39898157289271,24.1876114015801));
#15076=CARTESIAN_POINT('Ctrl Pts',(6.3927645830851,-2.22675372867375,24.1962463087045));
#15077=CARTESIAN_POINT('Ctrl Pts',(6.44833746475606,-2.0521288801202,24.2048812158288));
#15078=CARTESIAN_POINT('Ctrl Pts',(6.50575532124491,-1.87170662753666,24.2138027949003));
#15079=CARTESIAN_POINT('Ctrl Pts',(6.55564310865245,-1.68872575085632,24.2227243739718));
#15080=CARTESIAN_POINT('Ctrl Pts',(6.59778616853993,-1.50383066673852,24.2316459530433));
#15081=CARTESIAN_POINT('Ctrl Pts',(6.63846241780019,-1.32537095003421,24.2402570120191));
#15082=CARTESIAN_POINT('Ctrl Pts',(6.67192385554868,-1.14512835758297,24.2488680709948));
#15083=CARTESIAN_POINT('Ctrl Pts',(6.69802751434444,-0.963699339568564,
24.2574791299705));
#15084=CARTESIAN_POINT('Ctrl Pts',(6.72410655618508,-0.782441417492405,
24.2660820683201));
#15085=CARTESIAN_POINT('Ctrl Pts',(6.74284160978644,-0.599999601410085,
24.2746850066698));
#15086=CARTESIAN_POINT('Ctrl Pts',(6.75414064780855,-0.416980946351574,
24.2832879450194));
#15087=CARTESIAN_POINT('Ctrl Pts',(6.76542703352186,-0.234167229849509,
24.2918812500682));
#15088=CARTESIAN_POINT('Ctrl Pts',(6.76929399627383,-0.0507782667061611,
24.3004745551169));
#15089=CARTESIAN_POINT('Ctrl Pts',(6.76570124722964,0.132573124106202,24.3090678601657));
#15090=CARTESIAN_POINT('Ctrl Pts',(6.76530095617885,0.15300147019735,24.3100252950061));
#15091=CARTESIAN_POINT('Ctrl Pts',(6.76480811620918,0.17342934465578,24.3109827298466));
#15092=CARTESIAN_POINT('Ctrl Pts',(6.76422271154694,0.193855896460541,24.311940164687));
#15093=CARTESIAN_POINT('Ctrl Pts',(6.75896700501599,0.377243506179835,24.3205359222346));
#15094=CARTESIAN_POINT('Ctrl Pts',(6.74625221732102,0.560309629723236,24.3291316797821));
#15095=CARTESIAN_POINT('Ctrl Pts',(6.72614799984899,0.742443320481379,24.3377274373297));
#15096=CARTESIAN_POINT('Ctrl Pts',(6.70602502445856,0.924746948165146,24.3463312150113));
#15097=CARTESIAN_POINT('Ctrl Pts',(6.67849889093654,1.10611610306767,24.3549349926929));
#15098=CARTESIAN_POINT('Ctrl Pts',(6.64369066829049,1.2859484064572,24.3635387703745));
#15099=CARTESIAN_POINT('Ctrl Pts',(6.60751445205653,1.4728482766237,24.3724806840425));
#15100=CARTESIAN_POINT('Ctrl Pts',(6.56347227113019,1.65808768593789,24.3814225977106));
#15101=CARTESIAN_POINT('Ctrl Pts',(6.51175715352324,1.84100727145195,24.3903645113786));
#15102=CARTESIAN_POINT('Ctrl Pts',(6.46186215344655,2.01748898812556,24.3989917137093));
#15103=CARTESIAN_POINT('Ctrl Pts',(6.40482524950864,2.19181112399806,24.40761891604));
#15104=CARTESIAN_POINT('Ctrl Pts',(6.34086935583955,2.36340111114786,24.4162461183707));
#15105=CARTESIAN_POINT('Ctrl Pts',(6.2768525539714,2.53515451149533,24.4248815367911));
#15106=CARTESIAN_POINT('Ctrl Pts',(6.2059037247145,2.70417028718337,24.4335169552115));
#15107=CARTESIAN_POINT('Ctrl Pts',(6.1282930936579,2.869897691247,24.4421523736319));
#15108=CARTESIAN_POINT('Ctrl Pts',(6.05056780394805,3.03586993394548,24.450800549653));
#15109=CARTESIAN_POINT('Ctrl Pts',(5.96616118165986,3.19854382427801,24.4594487256742));
#15110=CARTESIAN_POINT('Ctrl Pts',(5.87538908268016,3.35739365090286,24.4680969016953));
#15111=CARTESIAN_POINT('Ctrl Pts',(5.86578573878774,3.37419936025052,24.4690118459272));
#15112=CARTESIAN_POINT('Ctrl Pts',(5.85611118664697,3.39096229487044,24.469926790159));
#15113=CARTESIAN_POINT('Ctrl Pts',(5.84636582806103,3.40768185200442,24.4708417343908));
#15114=CARTESIAN_POINT('Ctrl Pts',(5.75875476621719,3.55799116501222,24.4790671100886));
#15115=CARTESIAN_POINT('Ctrl Pts',(5.66522835322318,3.70511687059272,24.4872924857864));
#15116=CARTESIAN_POINT('Ctrl Pts',(5.56604438093354,3.84856323184096,24.4955178614842));
#15117=CARTESIAN_POINT('Ctrl Pts',(5.46695943896388,3.99186636895002,24.5037350245488));
#15118=CARTESIAN_POINT('Ctrl Pts',(5.36222838635197,4.13149718368364,24.5119521876134));
#15119=CARTESIAN_POINT('Ctrl Pts',(5.25215449663794,4.26698513513298,24.5201693506779));
#15120=CARTESIAN_POINT('Ctrl Pts',(5.14217055389574,4.40236237248852,24.5283797990808));
#15121=CARTESIAN_POINT('Ctrl Pts',(5.02685269264245,4.53360321139852,24.5365902474836));
#15122=CARTESIAN_POINT('Ctrl Pts',(4.90654704385762,4.66026663469078,24.5448006958865));
#15123=CARTESIAN_POINT('Ctrl Pts',(4.78631789509974,4.78684951517067,24.5530059234245));
#15124=CARTESIAN_POINT('Ctrl Pts',(4.66110752185817,4.90886051858895,24.5612111509626));
#15125=CARTESIAN_POINT('Ctrl Pts',(4.53130186876925,5.0258921968232,24.5694163785007));
#15126=CARTESIAN_POINT('Ctrl Pts',(4.40155390317331,5.14287186450201,24.577617959518));
#15127=CARTESIAN_POINT('Ctrl Pts',(4.26721499183724,5.25487637611436,24.5858195405353));
#15128=CARTESIAN_POINT('Ctrl Pts',(4.1287074736729,5.36153556332862,24.5940211215526));
#15129=CARTESIAN_POINT('Ctrl Pts',(3.99023523451358,5.46816758356992,24.6022206135598));
#15130=CARTESIAN_POINT('Ctrl Pts',(3.84759678834175,5.56945677466129,24.6104201055669));
#15131=CARTESIAN_POINT('Ctrl Pts',(3.7012470958779,5.66507360369267,24.618619597574));
#15132=CARTESIAN_POINT('Ctrl Pts',(3.55489272125638,5.760693491788,24.626819351907));
#15133=CARTESIAN_POINT('Ctrl Pts',(3.40482716178231,5.85064045758079,24.63501910624));
#15134=CARTESIAN_POINT('Ctrl Pts',(3.25153405582535,5.93462848742935,24.6432188605731));
#15135=CARTESIAN_POINT('Ctrl Pts',(3.20109128426322,5.96226566639547,24.6459170793358));
#15136=CARTESIAN_POINT('Ctrl Pts',(3.15029924130007,5.98925796810617,24.6486152980985));
#15137=CARTESIAN_POINT('Ctrl Pts',(3.0991757505326,6.01559628526638,24.6513135168612));
#15138=CARTESIAN_POINT('Origin',(0.,0.,-3.69717978381041));
#15139=CARTESIAN_POINT('',(3.09917575053259,6.01559628526639,27.0457515827422));
#15140=CARTESIAN_POINT('',(3.09917575053263,6.01559628526637,26.6512724846455));
#15141=CARTESIAN_POINT('',(3.09917575053259,6.01559628526639,-3.69717978381041));
#15142=CARTESIAN_POINT('',(-6.767,1.30221998277929E-12,25.69717978381));
#15143=CARTESIAN_POINT('Ctrl Pts',(-6.767,1.30221998655608E-12,25.69717978381));
#15144=CARTESIAN_POINT('Ctrl Pts',(-6.76700000000004,-0.186007249414475,
25.705929295616));
#15145=CARTESIAN_POINT('Ctrl Pts',(-6.75932637295444,-0.372014355526427,
25.7146788074219));
#15146=CARTESIAN_POINT('Ctrl Pts',(-6.74400518266936,-0.557389537154042,
25.7234283192279));
#15147=CARTESIAN_POINT('Ctrl Pts',(-6.72868405709656,-0.742763935810438,
25.7321777940784));
#15148=CARTESIAN_POINT('Ctrl Pts',(-6.70571545653004,-0.927506129694126,
25.740927268929));
#15149=CARTESIAN_POINT('Ctrl Pts',(-6.67517739415664,-1.1109886392489,25.7496767437795));
#15150=CARTESIAN_POINT('Ctrl Pts',(-6.64463945823084,-1.29447038906585,
25.7584261824015));
#15151=CARTESIAN_POINT('Ctrl Pts',(-6.60653217027138,-1.47669218228305,
25.7671756210235));
#15152=CARTESIAN_POINT('Ctrl Pts',(-6.56098496116688,-1.65703510504214,
25.7759250596455));
#15153=CARTESIAN_POINT('Ctrl Pts',(-6.51543793687485,-1.83737729604137,
25.7846744627657));
#15154=CARTESIAN_POINT('Ctrl Pts',(-6.46245112202596,-2.01584035397192,
25.7934238658859));
#15155=CARTESIAN_POINT('Ctrl Pts',(-6.40220448416187,-2.19181813638304,
25.8021732690062));
#15156=CARTESIAN_POINT('Ctrl Pts',(-6.34195808575128,-2.36779521936102,
25.8109226373515));
#15157=CARTESIAN_POINT('Ctrl Pts',(-6.27445201489171,-2.54128677544984,
25.8196720056967));
#15158=CARTESIAN_POINT('Ctrl Pts',(-6.19991555136116,-2.71170355237995,
25.828421374042));
#15159=CARTESIAN_POINT('Ctrl Pts',(-6.12537937788965,-2.88211966613227,
25.8371707083391));
#15160=CARTESIAN_POINT('Ctrl Pts',(-6.04381298133538,-3.04946076210601,
25.8459200426361));
#15161=CARTESIAN_POINT('Ctrl Pts',(-5.95549339426221,-3.21315848207012,
25.8546693769332));
#15162=CARTESIAN_POINT('Ctrl Pts',(-5.86717414355083,-3.3768555785977,25.8634186779087));
#15163=CARTESIAN_POINT('Ctrl Pts',(-5.77210188986169,-3.53690907467423,
25.8721679788843));
#15164=CARTESIAN_POINT('Ctrl Pts',(-5.67059953467009,-3.69277536784996,
25.8809172798598));
#15165=CARTESIAN_POINT('Ctrl Pts',(-5.56909755761702,-3.84864108035884,
25.8896665482406));
#15166=CARTESIAN_POINT('Ctrl Pts',(-5.46116568338003,-4.00031938104371,
25.8984158166213));
#15167=CARTESIAN_POINT('Ctrl Pts',(-5.34717048686043,-4.1472951166331,25.9071650850021));
#15168=CARTESIAN_POINT('Ctrl Pts',(-5.2331757055546,-4.29427031688109,25.9159143215147));
#15169=CARTESIAN_POINT('Ctrl Pts',(-5.11311782178764,-4.43654275987176,
25.9246635580273));
#15170=CARTESIAN_POINT('Ctrl Pts',(-4.98740459171991,-4.57362924147675,
25.9334127945399));
#15171=CARTESIAN_POINT('Ctrl Pts',(-4.86169180910809,-4.71071523514457,
25.9421619999111));
#15172=CARTESIAN_POINT('Ctrl Pts',(-4.73032391415414,-4.8426150931654,25.9509112052822));
#15173=CARTESIAN_POINT('Ctrl Pts',(-4.59374707237279,-4.96888084331536,
25.9596604106533));
#15174=CARTESIAN_POINT('Ctrl Pts',(-4.45717070537384,-5.0951461545274,25.9684095856095));
#15175=CARTESIAN_POINT('Ctrl Pts',(-4.31538563819486,-5.21577720253652,
25.9771587605657));
#15176=CARTESIAN_POINT('Ctrl Pts',(-4.1688734129062,-5.33036429028672,25.985907935522));
#15177=CARTESIAN_POINT('Ctrl Pts',(-4.02236168477306,-5.444950989212,25.9946570807899));
#15178=CARTESIAN_POINT('Ctrl Pts',(-3.87112305634402,-5.55349359238785,
26.0034062260578));
#15179=CARTESIAN_POINT('Ctrl Pts',(-3.71567117316691,-5.65562346102501,
26.0121553713257));
#15180=CARTESIAN_POINT('Ctrl Pts',(-3.56021980457252,-5.75775299158799,
26.0209044876319));
#15181=CARTESIAN_POINT('Ctrl Pts',(-3.40055544862332,-5.85346967275385,
26.0296536039381));
#15182=CARTESIAN_POINT('Ctrl Pts',(-3.2372203632334,-5.94244842803596,26.0384027202442));
#15183=CARTESIAN_POINT('Ctrl Pts',(-3.07388580496,-6.03142689616498,26.0471518083152));
#15184=CARTESIAN_POINT('Ctrl Pts',(-2.90688079257678,-6.11366734484836,
26.0559008963861));
#15185=CARTESIAN_POINT('Ctrl Pts',(-2.73677251094603,-6.18889046787307,
26.064649984457));
#15186=CARTESIAN_POINT('Ctrl Pts',(-2.56666476416654,-6.26411335438266,
26.0733990450193));
#15187=CARTESIAN_POINT('Ctrl Pts',(-2.39345402972124,-6.33231884350278,
26.0821481055815));
#15188=CARTESIAN_POINT('Ctrl Pts',(-2.21772856474091,-6.39327529621025,
26.0908971661437));
#15189=CARTESIAN_POINT('Ctrl Pts',(-2.04200363768364,-6.4542315623205,26.0996461999237));
#15190=CARTESIAN_POINT('Ctrl Pts',(-1.8637642662023,-6.50793874252015,26.1083952337037));
#15191=CARTESIAN_POINT('Ctrl Pts',(-1.68361578194868,-6.55421443796076,
26.1171442674836));
#15192=CARTESIAN_POINT('Ctrl Pts',(-1.50346783420026,-6.60048999558644,
26.1258932752079));
#15193=CARTESIAN_POINT('Ctrl Pts',(-1.32141106257383,-6.63933404145469,
26.1346422829321));
#15194=CARTESIAN_POINT('Ctrl Pts',(-1.13806375959158,-6.6706146552701,26.1433912906564));
#15195=CARTESIAN_POINT('Ctrl Pts',(-0.954716987419779,-6.70189517852473,
26.1521402730513));
#15196=CARTESIAN_POINT('Ctrl Pts',(-0.770079973809986,-6.72561226535828,
26.1608892554462));
#15197=CARTESIAN_POINT('Ctrl Pts',(-0.584779770552046,-6.74168536939786,
26.1696382378411));
#15198=CARTESIAN_POINT('Ctrl Pts',(-0.391490647553508,-6.75845143942396,
26.1787644185171));
#15199=CARTESIAN_POINT('Ctrl Pts',(-0.197480213103939,-6.76689975924028,
26.1878905991932));
#15200=CARTESIAN_POINT('Ctrl Pts',(-0.00346532629740909,-6.76699911271707,
26.1970167798692));
#15201=CARTESIAN_POINT('Ctrl Pts',(0.184486595296416,-6.76709536139772,
26.2058577673992));
#15202=CARTESIAN_POINT('Ctrl Pts',(0.37244237818556,-6.75935659726768,26.2146987549291));
#15203=CARTESIAN_POINT('Ctrl Pts',(0.559750217722389,-6.74380965729014,
26.223539742459));
#15204=CARTESIAN_POINT('Ctrl Pts',(0.745129914458067,-6.7284227571725,26.2322897210568));
#15205=CARTESIAN_POINT('Ctrl Pts',(0.929874656314509,-6.70538772273468,
26.2410396996546));
#15206=CARTESIAN_POINT('Ctrl Pts',(1.11335688289811,-6.67478280180737,26.2497896782523));
#15207=CARTESIAN_POINT('Ctrl Pts',(1.29683723118884,-6.64417819418018,26.2585395672773));
#15208=CARTESIAN_POINT('Ctrl Pts',(1.47905480730257,-6.6060039023007,26.2672894563022));
#15209=CARTESIAN_POINT('Ctrl Pts',(1.65939064804824,-6.5603895979713,26.2760393453271));
#15210=CARTESIAN_POINT('Ctrl Pts',(1.83972470264284,-6.51477574543251,26.2847891476881));
#15211=CARTESIAN_POINT('Ctrl Pts',(2.0181767812587,-6.46172209820093,26.2935389500491));
#15212=CARTESIAN_POINT('Ctrl Pts',(2.19414072347705,-6.40140886724006,26.30228875241));
#15213=CARTESIAN_POINT('Ctrl Pts',(2.37010298132121,-6.34109621361365,26.3110384710155));
#15214=CARTESIAN_POINT('Ctrl Pts',(2.54357687926936,-6.27352420825962,26.319788189621));
#15215=CARTESIAN_POINT('Ctrl Pts',(2.71397317789993,-6.19892237325487,26.3285379082265));
#15216=CARTESIAN_POINT('Ctrl Pts',(2.88436790207219,-6.12432122756955,26.3372875459847));
#15217=CARTESIAN_POINT('Ctrl Pts',(3.05168482126272,-6.04269049717409,26.346037183743));
#15218=CARTESIAN_POINT('Ctrl Pts',(3.21535561997401,-5.95430745234923,26.3547868215012));
#15219=CARTESIAN_POINT('Ctrl Pts',(3.3790249607529,-5.86592519481511,26.3635363813203));
#15220=CARTESIAN_POINT('Ctrl Pts',(3.53904799384881,-5.77079087940228,26.3722859411393));
#15221=CARTESIAN_POINT('Ctrl Pts',(3.69488118814988,-5.66922763747022,26.3810355009583));
#15222=CARTESIAN_POINT('Ctrl Pts',(3.85071304610837,-5.56766526649049,26.3897849857457));
#15223=CARTESIAN_POINT('Ctrl Pts',(4.00235489705972,-5.45967423580711,26.3985344705332));
#15224=CARTESIAN_POINT('Ctrl Pts',(4.14929168607658,-5.34562133936325,26.4072839553206));
#15225=CARTESIAN_POINT('Ctrl Pts',(4.29622726385752,-5.23156938308534,26.4160333679839));
#15226=CARTESIAN_POINT('Ctrl Pts',(4.43845763092054,-5.11145583677213,26.4247827806472));
#15227=CARTESIAN_POINT('Ctrl Pts',(4.57549970660941,-4.98568866204231,26.4335321933105));
#15228=CARTESIAN_POINT('Ctrl Pts',(4.71254069815276,-4.8599224822618,26.4422815367568));
#15229=CARTESIAN_POINT('Ctrl Pts',(4.84439326931296,-4.7285029573402,26.4510308802031));
#15230=CARTESIAN_POINT('Ctrl Pts',(4.97060959434682,-4.59187644221699,26.4597802236495));
#15231=CARTESIAN_POINT('Ctrl Pts',(5.09682496280503,-4.45525096256678,26.4685295007858));
#15232=CARTESIAN_POINT('Ctrl Pts',(5.2174039761583,-4.31341878218337,26.4772787779221));
#15233=CARTESIAN_POINT('Ctrl Pts',(5.33193710451928,-4.16686161438684,26.4860280550584));
#15234=CARTESIAN_POINT('Ctrl Pts',(5.44646940289381,-4.02030550864517,26.4947772687913));
#15235=CARTESIAN_POINT('Ctrl Pts',(5.55495572749666,-3.86902470980132,26.5035264825243));
#15236=CARTESIAN_POINT('Ctrl Pts',(5.65702762491459,-3.71353301465776,26.5122756962572));
#15237=CARTESIAN_POINT('Ctrl Pts',(5.75909881655154,-3.55804239466892,26.5210248494934));
#15238=CARTESIAN_POINT('Ctrl Pts',(5.8547555125078,-3.39834117619557,26.5297740027295));
#15239=CARTESIAN_POINT('Ctrl Pts',(5.9436728372809,-3.23497174691978,26.5385231559656));
#15240=CARTESIAN_POINT('Ctrl Pts',(6.032589576763,-3.07160339300987,26.5472722516111));
#15241=CARTESIAN_POINT('Ctrl Pts',(6.11476689685268,-2.90456712829538,26.5560213472566));
#15242=CARTESIAN_POINT('Ctrl Pts',(6.1899257052524,-2.73443024475952,26.5647704429022));
#15243=CARTESIAN_POINT('Ctrl Pts',(6.26508404388683,-2.56429442463065,26.5735194838632));
#15244=CARTESIAN_POINT('Ctrl Pts',(6.33322384283307,-2.39105828656015,26.5822685248242));
#15245=CARTESIAN_POINT('Ctrl Pts',(6.3941136872003,-2.2153101713209,26.5910175657853));
#15246=CARTESIAN_POINT('Ctrl Pts',(6.45500317120886,-2.03956309619526,26.5997665549677));
#15247=CARTESIAN_POINT('Ctrl Pts',(6.50864269270069,-1.86130434438647,26.6085155441501));
#15248=CARTESIAN_POINT('Ctrl Pts',(6.55485008446329,-1.6811393071996,26.6172645333325));
#15249=CARTESIAN_POINT('Ctrl Pts',(6.601996647494,-1.49731239211855,26.6261913468618));
#15250=CARTESIAN_POINT('Ctrl Pts',(6.64140563640904,-1.31150116499687,26.6351181603912));
#15251=CARTESIAN_POINT('Ctrl Pts',(6.6729377228217,-1.12436255155675,26.6440449739206));
#15252=CARTESIAN_POINT('Ctrl Pts',(6.70384494949869,-0.940932395051482,
26.6527948880761));
#15253=CARTESIAN_POINT('Ctrl Pts',(6.72718449348929,-0.756227260506838,
26.6615448022316));
#15254=CARTESIAN_POINT('Ctrl Pts',(6.74287707373931,-0.5708745645418,26.6702947163872));
#15255=CARTESIAN_POINT('Ctrl Pts',(6.75856934538669,-0.385525513632588,
26.6790444584711));
#15256=CARTESIAN_POINT('Ctrl Pts',(6.76661493004103,-0.199529212418346,
26.6877942005551));
#15257=CARTESIAN_POINT('Ctrl Pts',(6.76698649908907,-0.0135174386005491,
26.6965439426391));
#15258=CARTESIAN_POINT('Ctrl Pts',(6.7673580613239,0.172490924445683,26.705293524285));
#15259=CARTESIAN_POINT('Ctrl Pts',(6.7600558889629,0.358514472901337,26.7140431059309));
#15260=CARTESIAN_POINT('Ctrl Pts',(6.74510478454585,0.543921359662168,26.7227926875768));
#15261=CARTESIAN_POINT('Ctrl Pts',(6.73015393440688,0.729325093150405,26.7315421204158));
#15262=CARTESIAN_POINT('Ctrl Pts',(6.70755443556898,0.914111900256317,26.7402915532549));
#15263=CARTESIAN_POINT('Ctrl Pts',(6.67738304682319,1.09765415591535,26.7490409860939));
#15264=CARTESIAN_POINT('Ctrl Pts',(6.64721213111861,1.28119353391273,26.7577902817553));
#15265=CARTESIAN_POINT('Ctrl Pts',(6.60946960955494,1.46348811672655,26.7665395774166));
#15266=CARTESIAN_POINT('Ctrl Pts',(6.56428366991182,1.64391876348227,26.7752888730779));
#15267=CARTESIAN_POINT('Ctrl Pts',(6.51909837867718,1.82434682109713,26.7840380431887));
#15268=CARTESIAN_POINT('Ctrl Pts',(6.46646995271924,2.00291071820435,26.7927872132996));
#15269=CARTESIAN_POINT('Ctrl Pts',(6.40657713281555,2.17900400212687,26.8015363834104));
#15270=CARTESIAN_POINT('Ctrl Pts',(6.34668509279064,2.35509499309648,26.8102854395962));
#15271=CARTESIAN_POINT('Ctrl Pts',(6.27952894037528,2.52871516398118,26.8190344957819));
#15272=CARTESIAN_POINT('Ctrl Pts',(6.20533675061446,2.69927486771422,26.8277835519677));
#15273=CARTESIAN_POINT('Ctrl Pts',(6.12832117907917,2.87632521635922,26.83686555325));
#15274=CARTESIAN_POINT('Ctrl Pts',(6.04372366626082,3.05007728919992,26.8459475545322));
#15275=CARTESIAN_POINT('Ctrl Pts',(5.95185378007872,3.21989527478188,26.8550295558145));
#15276=CARTESIAN_POINT('Ctrl Pts',(5.86334450817376,3.38350129286744,26.8637793361216));
#15277=CARTESIAN_POINT('Ctrl Pts',(5.76808562057261,3.54345567124954,26.8725291164288));
#15278=CARTESIAN_POINT('Ctrl Pts',(5.66640068804489,3.69921508465301,26.8812788967359));
#15279=CARTESIAN_POINT('Ctrl Pts',(5.56471941107929,3.85496889852276,26.8900283624894));
#15280=CARTESIAN_POINT('Ctrl Pts',(5.45661270815119,4.0065278091963,26.8987778282429));
#15281=CARTESIAN_POINT('Ctrl Pts',(5.34244776449119,4.15337704569223,26.9075272939963));
#15282=CARTESIAN_POINT('Ctrl Pts',(5.22828631819598,4.30022178356246,26.9162764917159));
#15283=CARTESIAN_POINT('Ctrl Pts',(5.1080671784407,4.44235690972678,26.9250256894355));
#15284=CARTESIAN_POINT('Ctrl Pts',(4.98219864544718,4.57929969070646,26.9337748871551));
#15285=CARTESIAN_POINT('Ctrl Pts',(4.85633329944022,4.71623900430004,26.9425238633454));
#15286=CARTESIAN_POINT('Ctrl Pts',(4.72481904033643,4.84798602483622,26.9512728395356));
#15287=CARTESIAN_POINT('Ctrl Pts',(4.58810250737191,4.97409332259132,26.9600218157258));
#15288=CARTESIAN_POINT('Ctrl Pts',(4.45137708685635,5.10020881822141,26.968771360662));
#15289=CARTESIAN_POINT('Ctrl Pts',(4.30944892636045,5.22068366307938,26.9775209055982));
#15290=CARTESIAN_POINT('Ctrl Pts',(4.16280009466656,5.33510865604855,26.9862704505344));
#15291=CARTESIAN_POINT('Ctrl Pts',(4.01615988348789,5.44952692272891,26.9950194811427));
#15292=CARTESIAN_POINT('Ctrl Pts',(3.86479978232237,5.55789587288621,27.0037685117509));
#15293=CARTESIAN_POINT('Ctrl Pts',(3.7092338358108,5.65984746713869,27.0125175423592));
#15294=CARTESIAN_POINT('Ctrl Pts',(3.5536657779955,5.76180044505377,27.0212666917072));
#15295=CARTESIAN_POINT('Ctrl Pts',(3.39389200026846,5.85733573571056,27.0300158410552));
#15296=CARTESIAN_POINT('Ctrl Pts',(3.23045513626044,5.94612887621926,27.0387649904033));
#15297=CARTESIAN_POINT('Ctrl Pts',(3.18695122151581,5.96976399206687,27.0410938545162));
#15298=CARTESIAN_POINT('Ctrl Pts',(3.14318791262666,5.99292165435332,27.0434227186292));
#15299=CARTESIAN_POINT('Ctrl Pts',(3.09917575053259,6.01559628526639,27.0457515827422));
#15300=CARTESIAN_POINT('Ctrl Pts',(3.09917575053259,6.01559628526639,25.045602228898));
#15301=CARTESIAN_POINT('Ctrl Pts',(2.94396618243902,6.09555872072177,25.0538143435959));
#15302=CARTESIAN_POINT('Ctrl Pts',(2.78578041257525,6.16944837392768,25.0620264582939));
#15303=CARTESIAN_POINT('Ctrl Pts',(2.62514014159034,6.23706086526427,25.0702385729919));
#15304=CARTESIAN_POINT('Ctrl Pts',(2.46426588794036,6.30477183844988,25.0784626491517));
#15305=CARTESIAN_POINT('Ctrl Pts',(2.30093032461335,6.36618725259255,25.0866867253116));
#15306=CARTESIAN_POINT('Ctrl Pts',(2.1356718718031,6.4211521283948,25.0949108014715));
#15307=CARTESIAN_POINT('Ctrl Pts',(1.99267554601726,6.46871263228031,25.1020270043274));
#15308=CARTESIAN_POINT('Ctrl Pts',(1.84823986788398,6.51144423155273,25.1091432071833));
#15309=CARTESIAN_POINT('Ctrl Pts',(1.70271931047384,6.54927751356892,25.1162594100391));
#15310=CARTESIAN_POINT('Ctrl Pts',(1.53603835808051,6.59261219830938,25.1244103922134));
#15311=CARTESIAN_POINT('Ctrl Pts',(1.36744016728447,6.62964768602582,25.1325613743877));
#15312=CARTESIAN_POINT('Ctrl Pts',(1.19744625096259,6.66021106843136,25.140712356562));
#15313=CARTESIAN_POINT('Ctrl Pts',(1.02764979832998,6.69073894863555,25.148853870615));
#15314=CARTESIAN_POINT('Ctrl Pts',(0.856461203662327,6.71480962453299,25.1569953846681));
#15315=CARTESIAN_POINT('Ctrl Pts',(0.684417091352962,6.73229992239383,25.1651368987211));
#15316=CARTESIAN_POINT('Ctrl Pts',(0.51253661983395,6.74977358425285,25.1732706689242));
#15317=CARTESIAN_POINT('Ctrl Pts',(0.339802612011201,6.76067929202203,25.1814044391272));
#15318=CARTESIAN_POINT('Ctrl Pts',(0.166761838490786,6.76494489920082,25.1895382093303));
#15319=CARTESIAN_POINT('Ctrl Pts',(-0.00615074029530097,6.76920734626672,
25.1976659537483));
#15320=CARTESIAN_POINT('Ctrl Pts',(-0.179369268211578,6.76683947870447,
25.2057936981662));
#15321=CARTESIAN_POINT('Ctrl Pts',(-0.352341899948757,6.75782096430059,
25.2139214425842));
#15322=CARTESIAN_POINT('Ctrl Pts',(-0.525222753625955,6.74880723505692,
25.2220448744783));
#15323=CARTESIAN_POINT('Ctrl Pts',(-0.697857606560665,6.7331499056229,25.2301683063723));
#15324=CARTESIAN_POINT('Ctrl Pts',(-0.869694664559225,6.71088073135242,
25.2382917382664));
#15325=CARTESIAN_POINT('Ctrl Pts',(-1.04262178926545,6.68847029019945,25.2464667020172));
#15326=CARTESIAN_POINT('Ctrl Pts',(-1.21474058701269,6.65936382531185,25.254641665768));
#15327=CARTESIAN_POINT('Ctrl Pts',(-1.38549346493782,6.6236467945245,25.2628166295188));
#15328=CARTESIAN_POINT('Ctrl Pts',(-1.55513149232127,6.58816296127738,25.2709382186919));
#15329=CARTESIAN_POINT('Ctrl Pts',(-1.72342102622658,6.54615472808624,25.2790598078649));
#15330=CARTESIAN_POINT('Ctrl Pts',(-1.88982546590237,6.49775720602324,25.2871813970379));
#15331=CARTESIAN_POINT('Ctrl Pts',(-2.05625187437702,6.44935329449473,25.2953040584273));
#15332=CARTESIAN_POINT('Ctrl Pts',(-2.22079234145552,6.39455851617661,25.3034267198166));
#15333=CARTESIAN_POINT('Ctrl Pts',(-2.38292549598552,6.33355785325927,25.311549381206));
#15334=CARTESIAN_POINT('Ctrl Pts',(-2.54511093036561,6.27253752067276,25.3196746617483));
#15335=CARTESIAN_POINT('Ctrl Pts',(-2.70488716410205,6.20530744751755,25.3277999422905));
#15336=CARTESIAN_POINT('Ctrl Pts',(-2.86175291536794,6.13210072090985,25.3359252228328));
#15337=CARTESIAN_POINT('Ctrl Pts',(-3.02032768644431,6.05809642220611,25.3441390266205));
#15338=CARTESIAN_POINT('Ctrl Pts',(-3.17592783722615,5.97798464071692,25.3523528304083));
#15339=CARTESIAN_POINT('Ctrl Pts',(-3.32806199135273,5.89205332475134,25.3605666341961));
#15340=CARTESIAN_POINT('Ctrl Pts',(-3.4788169604441,5.80690102639503,25.3687059750512));
#15341=CARTESIAN_POINT('Ctrl Pts',(-3.62616824026076,5.71603452094295,25.3768453159064));
#15342=CARTESIAN_POINT('Ctrl Pts',(-3.76966808797646,5.61977681998955,25.3849846567616));
#15343=CARTESIAN_POINT('Ctrl Pts',(-3.91513715279711,5.52219819560511,25.3932356920156));
#15344=CARTESIAN_POINT('Ctrl Pts',(-4.05664799702019,5.41907956952353,25.4014867272697));
#15345=CARTESIAN_POINT('Ctrl Pts',(-4.19377033464324,5.31079837503424,25.4097377625238));
#15346=CARTESIAN_POINT('Ctrl Pts',(-4.33089267226627,5.20251718054497,25.4179887977779));
#15347=CARTESIAN_POINT('Ctrl Pts',(-4.46362625504326,5.0890737180381,25.4262398330319));
#15348=CARTESIAN_POINT('Ctrl Pts',(-4.59158115548176,4.97088236559917,25.434490868286));
#15349=CARTESIAN_POINT('Ctrl Pts',(-4.71781145313423,4.85428402081374,25.4426306943692));
#15350=CARTESIAN_POINT('Ctrl Pts',(-4.83980275031117,4.73268470718957,25.4507705204524));
#15351=CARTESIAN_POINT('Ctrl Pts',(-4.95712802364735,4.60642711406249,25.4589103465356));
#15352=CARTESIAN_POINT('Ctrl Pts',(-5.07431167281898,4.48032192736615,25.4670403469773));
#15353=CARTESIAN_POINT('Ctrl Pts',(-5.18684026234713,4.3495699206802,25.4751703474191));
#15354=CARTESIAN_POINT('Ctrl Pts',(-5.29432033801962,4.21455349455098,25.4833003478608));
#15355=CARTESIAN_POINT('Ctrl Pts',(-5.40169352152022,4.07967134632338,25.4914222627723));
#15356=CARTESIAN_POINT('Ctrl Pts',(-5.50402796004642,3.9405335077515,25.4995441776838));
#15357=CARTESIAN_POINT('Ctrl Pts',(-5.60096756501489,3.79755860200356,25.5076660925953));
#15358=CARTESIAN_POINT('Ctrl Pts',(-5.69782189370204,3.65470946908383,25.515780862783));
#15359=CARTESIAN_POINT('Ctrl Pts',(-5.78929063807354,3.5080302962892,25.5238956329707));
#15360=CARTESIAN_POINT('Ctrl Pts',(-5.8750585907684,3.35797194077593,25.5320104031585));
#15361=CARTESIAN_POINT('Ctrl Pts',(-5.96078454882321,3.20798705847063,25.5401212001039));
#15362=CARTESIAN_POINT('Ctrl Pts',(-6.04081508903707,3.05462660479748,25.5482319970494));
#15363=CARTESIAN_POINT('Ctrl Pts',(-6.11487873275084,2.89836972861496,25.5563427939948));
#15364=CARTESIAN_POINT('Ctrl Pts',(-6.18892035088505,2.74215932122717,25.5644511788931));
#15365=CARTESIAN_POINT('Ctrl Pts',(-6.25699844812174,2.58305453792936,25.5725595637914));
#15366=CARTESIAN_POINT('Ctrl Pts',(-6.31888789351101,2.42155833901229,25.5806679486897));
#15367=CARTESIAN_POINT('Ctrl Pts',(-6.38077083111304,2.26007912171298,25.5887754809766));
#15368=CARTESIAN_POINT('Ctrl Pts',(-6.43646628214497,2.09620933294143,25.5968830132635));
#15369=CARTESIAN_POINT('Ctrl Pts',(-6.48579761055905,1.93047101891392,25.6049905455504));
#15370=CARTESIAN_POINT('Ctrl Pts',(-6.53515040741879,1.76466057741481,25.6131016061453));
#15371=CARTESIAN_POINT('Ctrl Pts',(-6.57813344044233,1.5969803377804,25.6212126667401));
#15372=CARTESIAN_POINT('Ctrl Pts',(-6.61462009762341,1.42796707389088,25.6293237273349));
#15373=CARTESIAN_POINT('Ctrl Pts',(-6.65111460209694,1.25891745982261,25.6374365323994));
#15374=CARTESIAN_POINT('Ctrl Pts',(-6.68110987827748,1.0885346114493,25.6455493374638));
#15375=CARTESIAN_POINT('Ctrl Pts',(-6.70453068608186,0.917364311158205,
25.6536621425283));
#15376=CARTESIAN_POINT('Ctrl Pts',(-6.72797283468183,0.746038042276231,
25.661782339896));
#15377=CARTESIAN_POINT('Ctrl Pts',(-6.74482850646066,0.573923253531824,
25.6699025372637));
#15378=CARTESIAN_POINT('Ctrl Pts',(-6.75507440440881,0.401570405907753,
25.6780227346314));
#15379=CARTESIAN_POINT('Ctrl Pts',(-6.76302860803167,0.267767624353762,
25.6843266919466));
#15380=CARTESIAN_POINT('Ctrl Pts',(-6.76700022310181,0.133821483113563,
25.6906306492618));
#15381=CARTESIAN_POINT('Ctrl Pts',(-6.7669999999906,-1.12811956310505E-5,
25.6969346065769));
#15382=CARTESIAN_POINT('',(-6.76699880620097,-0.00401956150071273,25.3028202162185));
#15383=CARTESIAN_POINT('Ctrl Pts',(3.0991757505326,6.01559628526638,24.6513135168612));
#15384=CARTESIAN_POINT('Ctrl Pts',(2.94375327653849,6.09566840773745,24.6595164746245));
#15385=CARTESIAN_POINT('Ctrl Pts',(2.78526591770003,6.16969254101118,24.6677194323877));
#15386=CARTESIAN_POINT('Ctrl Pts',(2.62422874726044,6.23744438709091,24.675922390151));
#15387=CARTESIAN_POINT('Ctrl Pts',(2.46312443454218,6.30522448139009,24.684128768027));
#15388=CARTESIAN_POINT('Ctrl Pts',(2.29946852245279,6.36672694014881,24.692335145903));
#15389=CARTESIAN_POINT('Ctrl Pts',(2.1337942026006,6.42177633532561,24.700541523779));
#15390=CARTESIAN_POINT('Ctrl Pts',(1.96792736579282,6.476889699028,24.7087574376343));
#15391=CARTESIAN_POINT('Ctrl Pts',(1.80003777664869,6.52553490838256,24.7169733514896));
#15392=CARTESIAN_POINT('Ctrl Pts',(1.63067283231014,6.56758670395493,24.7251892653449));
#15393=CARTESIAN_POINT('Ctrl Pts',(1.46119849244701,6.60966566145421,24.7334104859903));
#15394=CARTESIAN_POINT('Ctrl Pts',(1.29024724786503,6.64514264390263,24.7416317066357));
#15395=CARTESIAN_POINT('Ctrl Pts',(1.11837460373133,6.67394390489827,24.7498529272811));
#15396=CARTESIAN_POINT('Ctrl Pts',(0.946251757426406,6.70278709308991,24.7580861159));
#15397=CARTESIAN_POINT('Ctrl Pts',(0.773205186618674,6.72493510158126,24.7663193045189));
#15398=CARTESIAN_POINT('Ctrl Pts',(0.599794505029058,6.7403661289085,24.7745524931378));
#15399=CARTESIAN_POINT('Ctrl Pts',(0.500854736219013,6.74917032863982,24.779249953358));
#15400=CARTESIAN_POINT('Ctrl Pts',(0.401796439857815,6.75578891228401,24.7839474135782));
#15401=CARTESIAN_POINT('Ctrl Pts',(0.302723114336111,6.7602254190261,24.7886448737984));
#15402=CARTESIAN_POINT('Ctrl Pts',(0.130717743851077,6.76792782511588,24.7968003322052));
#15403=CARTESIAN_POINT('Ctrl Pts',(-0.0418623406125811,6.76907382164679,
24.804955790612));
#15404=CARTESIAN_POINT('Ctrl Pts',(-0.214471438378831,6.76360044666446,
24.8131112490188));
#15405=CARTESIAN_POINT('Ctrl Pts',(-0.386870448183795,6.75813373349896,
24.8212567811607));
#15406=CARTESIAN_POINT('Ctrl Pts',(-0.559298039694058,6.74606369739774,
24.8294023133026));
#15407=CARTESIAN_POINT('Ctrl Pts',(-0.731203809171472,6.72737913228124,
24.8375478454444));
#15408=CARTESIAN_POINT('Ctrl Pts',(-0.90293649506536,6.70871337974735,24.845685176245));
#15409=CARTESIAN_POINT('Ctrl Pts',(-1.07414804425433,6.68344639597504,24.8538225070455));
#15410=CARTESIAN_POINT('Ctrl Pts',(-1.24428847192027,6.65161899079061,24.8619598378461));
#15411=CARTESIAN_POINT('Ctrl Pts',(-1.41429334897801,6.61981694244929,24.8700906856481));
#15412=CARTESIAN_POINT('Ctrl Pts',(-1.58322844606182,6.58146494655465,24.8782215334501));
#15413=CARTESIAN_POINT('Ctrl Pts',(-1.75054932089481,6.53665557262387,24.8863523812522));
#15414=CARTESIAN_POINT('Ctrl Pts',(-1.91777204009729,6.49187248526586,24.8944784592459));
#15415=CARTESIAN_POINT('Ctrl Pts',(-2.08338207071149,6.44063965811015,24.9026045372397));
#15416=CARTESIAN_POINT('Ctrl Pts',(-2.24684558583775,6.38310065042072,24.9107306152335));
#15417=CARTESIAN_POINT('Ctrl Pts',(-2.41088871273391,6.32535761991887,24.9188855068157));
#15418=CARTESIAN_POINT('Ctrl Pts',(-2.57276970953988,6.26126368008906,24.9270403983979));
#15419=CARTESIAN_POINT('Ctrl Pts',(-2.73196424635951,6.19101448525307,24.9351952899801));
#15420=CARTESIAN_POINT('Ctrl Pts',(-2.89053798014637,6.12103923771499,24.9433183803364));
#15421=CARTESIAN_POINT('Ctrl Pts',(-3.0464458387807,6.04495682005173,24.9514414706927));
#15422=CARTESIAN_POINT('Ctrl Pts',(-3.19918981210989,5.96300876622635,24.959564561049));
#15423=CARTESIAN_POINT('Ctrl Pts',(-3.35194577959302,5.88105427746576,24.9676882892674));
#15424=CARTESIAN_POINT('Ctrl Pts',(-3.50153704451353,5.79323340800121,24.9758120174858));
#15425=CARTESIAN_POINT('Ctrl Pts',(-3.64749060145182,5.69983344601583,24.9839357457043));
#15426=CARTESIAN_POINT('Ctrl Pts',(-3.79348338682098,5.60640838060694,24.9920616573646));
#15427=CARTESIAN_POINT('Ctrl Pts',(-3.93583620938079,5.50740143397097,25.0001875690249));
#15428=CARTESIAN_POINT('Ctrl Pts',(-4.07410546947808,5.40314293939822,25.0083134806852));
#15429=CARTESIAN_POINT('Ctrl Pts',(-4.21325897586662,5.29821770091512,25.0164913583953));
#15430=CARTESIAN_POINT('Ctrl Pts',(-4.34827620899244,5.18797373909642,25.0246692361054));
#15431=CARTESIAN_POINT('Ctrl Pts',(-4.47873984375709,5.07278803144215,25.0328471138155));
#15432=CARTESIAN_POINT('Ctrl Pts',(-4.6085808038887,4.95815208018838,25.0409859602889));
#15433=CARTESIAN_POINT('Ctrl Pts',(-4.73391131479579,4.83862174851114,25.0491248067623));
#15434=CARTESIAN_POINT('Ctrl Pts',(-4.85435825669402,4.714604428334,25.0572636532357));
#15435=CARTESIAN_POINT('Ctrl Pts',(-4.97567163459911,4.58969498860628,25.0654610465641));
#15436=CARTESIAN_POINT('Ctrl Pts',(-5.09203066609562,4.46023404357679,25.0736584398925));
#15437=CARTESIAN_POINT('Ctrl Pts',(-5.20309674407,4.32666999802946,25.0818558332209));
#15438=CARTESIAN_POINT('Ctrl Pts',(-5.31416282204437,4.19310595248212,25.0900532265493));
#15439=CARTESIAN_POINT('Ctrl Pts',(-5.41993576816953,4.05543913881916,25.0982506198777));
#15440=CARTESIAN_POINT('Ctrl Pts',(-5.52012270626552,3.91414541219049,25.1064480132061));
#15441=CARTESIAN_POINT('Ctrl Pts',(-5.62195064967377,3.7705373743313,25.1147796751952));
#15442=CARTESIAN_POINT('Ctrl Pts',(-5.71830642439719,3.62276230979212,25.1231113371843));
#15443=CARTESIAN_POINT('Ctrl Pts',(-5.80883672877185,3.47126847974501,25.1314429991735));
#15444=CARTESIAN_POINT('Ctrl Pts',(-5.89926017322852,3.31995346957887,25.1397648266577));
#15445=CARTESIAN_POINT('Ctrl Pts',(-5.98387166682184,3.16492873101086,25.148086654142));
#15446=CARTESIAN_POINT('Ctrl Pts',(-6.06235947374681,3.00667367884716,25.1564084816262));
#15447=CARTESIAN_POINT('Ctrl Pts',(-6.14076752079736,2.84857944660672,25.1647218524095));
#15448=CARTESIAN_POINT('Ctrl Pts',(-6.21306412428561,2.68726174791271,25.1730352231928));
#15449=CARTESIAN_POINT('Ctrl Pts',(-6.27898191581495,2.52322712034981,25.181348593976));
#15450=CARTESIAN_POINT('Ctrl Pts',(-6.34484353585997,2.35933227399465,25.189654880566));
#15451=CARTESIAN_POINT('Ctrl Pts',(-6.40433704480477,2.19272543122517,25.197961167156));
#15452=CARTESIAN_POINT('Ctrl Pts',(-6.45724184116955,2.02393596851515,25.206267453746));
#15453=CARTESIAN_POINT('Ctrl Pts',(-6.51010470651423,1.85528028411708,25.2145671569807));
#15454=CARTESIAN_POINT('Ctrl Pts',(-6.55638916665807,1.68444575796112,25.2228668602154));
#15455=CARTESIAN_POINT('Ctrl Pts',(-6.59592341309155,1.5119799365834,25.2311665634501));
#15456=CARTESIAN_POINT('Ctrl Pts',(-6.6354389109427,1.33959590479173,25.2394623306626));
#15457=CARTESIAN_POINT('Ctrl Pts',(-6.66821049592097,1.16558245606088,25.2477580978752));
#15458=CARTESIAN_POINT('Ctrl Pts',(-6.69411659456468,0.99050089266686,25.2560538650878));
#15459=CARTESIAN_POINT('Ctrl Pts',(-6.72001635095464,0.815462192218633,
25.2643476013554));
#15460=CARTESIAN_POINT('Ctrl Pts',(-6.73905391639905,0.639356240041771,
25.272641337623));
#15461=CARTESIAN_POINT('Ctrl Pts',(-6.75115903176224,0.462753420144147,
25.2809350738906));
#15462=CARTESIAN_POINT('Ctrl Pts',(-6.76180651172889,0.307416198606293,
25.2882301213237));
#15463=CARTESIAN_POINT('Ctrl Pts',(-6.76709129972569,0.15169485322347,25.2955251687568));
#15464=CARTESIAN_POINT('Ctrl Pts',(-6.76699880620133,-0.00401956088942276,
25.3028202161899));
#15465=CARTESIAN_POINT('Ctrl Pts',(-6.76699880620097,-0.00401956150070087,
25.3028202162186));
#15466=CARTESIAN_POINT('Ctrl Pts',(-6.76688334084871,-0.198407407234547,
25.3119270709894));
#15467=CARTESIAN_POINT('Ctrl Pts',(-6.75838791804712,-0.392497961171036,
25.3210339257603));
#15468=CARTESIAN_POINT('Ctrl Pts',(-6.74161346978387,-0.585608080569804,
25.3301407805311));
#15469=CARTESIAN_POINT('Ctrl Pts',(-6.72474577620206,-0.7797916549233,25.3392982582233));
#15470=CARTESIAN_POINT('Ctrl Pts',(-6.69950683604764,-0.972983664605142,
25.3484557359154));
#15471=CARTESIAN_POINT('Ctrl Pts',(-6.66604947769159,-1.16450562942723,
25.3576132136076));
#15472=CARTESIAN_POINT('Ctrl Pts',(-6.63249811463724,-1.35656571098672,
25.366796420944));
#15473=CARTESIAN_POINT('Ctrl Pts',(-6.59068219033038,-1.54694616423987,
25.3759796282803));
#15474=CARTESIAN_POINT('Ctrl Pts',(-6.54080477051408,-1.73498183103464,
25.3851628356167));
#15475=CARTESIAN_POINT('Ctrl Pts',(-6.49074514784345,-1.92370439453197,
25.3943795893273));
#15476=CARTESIAN_POINT('Ctrl Pts',(-6.43256512569696,-2.11006482645954,
25.4035963430379));
#15477=CARTESIAN_POINT('Ctrl Pts',(-6.36651770178052,-2.29341259979867,
25.4128130967484));
#15478=CARTESIAN_POINT('Ctrl Pts',(-6.33919592999244,-2.36925788980367,
25.4166257820369));
#15479=CARTESIAN_POINT('Ctrl Pts',(-6.31052842599154,-2.44458792191119,
25.4204384673254));
#15480=CARTESIAN_POINT('Ctrl Pts',(-6.2805354090269,-2.51935784992116,25.4242511526138));
#15481=CARTESIAN_POINT('Ctrl Pts',(-6.21582285919771,-2.68068049038025,
25.4324773536327));
#15482=CARTESIAN_POINT('Ctrl Pts',(-6.14480023546957,-2.83973368865429,
25.4407035546515));
#15483=CARTESIAN_POINT('Ctrl Pts',(-6.06764690463886,-2.99598899207365,
25.4489297556703));
#15484=CARTESIAN_POINT('Ctrl Pts',(-5.99058023931446,-3.15206877559208,
25.4571467162861));
#15485=CARTESIAN_POINT('Ctrl Pts',(-5.90739673723445,-3.30535660386273,
25.4653636769019));
#15486=CARTESIAN_POINT('Ctrl Pts',(-5.81832453226442,-3.45534204345244,
25.4735806375176));
#15487=CARTESIAN_POINT('Ctrl Pts',(-5.72933450364474,-3.60518910928082,
25.4817900173192));
#15488=CARTESIAN_POINT('Ctrl Pts',(-5.63446677374864,-3.75173954766778,
25.4899993971208));
#15489=CARTESIAN_POINT('Ctrl Pts',(-5.53399631125849,-3.89450559467789,
25.4982087769224));
#15490=CARTESIAN_POINT('Ctrl Pts',(-5.43359838218822,-4.03716857348891,
25.5064122300627));
#15491=CARTESIAN_POINT('Ctrl Pts',(-5.32760598268406,-4.17605231068577,
25.5146156832031));
#15492=CARTESIAN_POINT('Ctrl Pts',(-5.21633853458503,-4.31069614941755,
25.5228191363435));
#15493=CARTESIAN_POINT('Ctrl Pts',(-5.10512909468399,-4.44526979289827,
25.5310183126936));
#15494=CARTESIAN_POINT('Ctrl Pts',(-4.98865031278193,-4.5756076656865,25.5392174890438));
#15495=CARTESIAN_POINT('Ctrl Pts',(-4.86726325624927,-4.70128039946202,
25.547416665394));
#15496=CARTESIAN_POINT('Ctrl Pts',(-4.74589904052343,-4.82692948601586,
25.5556142989453));
#15497=CARTESIAN_POINT('Ctrl Pts',(-4.61962863423834,-4.94791492006309,
25.5638119324967));
#15498=CARTESIAN_POINT('Ctrl Pts',(-4.48885170573719,-5.06384235180168,
25.5720095660481));
#15499=CARTESIAN_POINT('Ctrl Pts',(-4.35808419638442,-5.17976143392009,
25.5802066091687));
#15500=CARTESIAN_POINT('Ctrl Pts',(-4.22281107905283,-5.29062300066486,
25.5884036522892));
#15501=CARTESIAN_POINT('Ctrl Pts',(-4.08346697035957,-5.39607139518951,
25.5966006954098));
#15502=CARTESIAN_POINT('Ctrl Pts',(-3.94410757230295,-5.50153135991139,
25.604798637941));
#15503=CARTESIAN_POINT('Ctrl Pts',(-3.80067657903412,-5.6015767525989,25.6129965804722));
#15504=CARTESIAN_POINT('Ctrl Pts',(-3.6536396315922,-5.69589382296219,25.6211945230034));
#15505=CARTESIAN_POINT('Ctrl Pts',(-3.50655982687992,-5.7902383841858,25.6293948550118));
#15506=CARTESIAN_POINT('Ctrl Pts',(-3.35587227628556,-5.87885110373377,
25.6375951870202));
#15507=CARTESIAN_POINT('Ctrl Pts',(-3.20206942024186,-5.96146294360302,
25.6457955190286));
#15508=CARTESIAN_POINT('Ctrl Pts',(-3.0481062600525,-6.04416088733765,25.6540043979994));
#15509=CARTESIAN_POINT('Ctrl Pts',(-2.89102162381837,-6.12084528582415,
25.6622132769702));
#15510=CARTESIAN_POINT('Ctrl Pts',(-2.73133115216674,-6.19129381770915,
25.6704221559409));
#15511=CARTESIAN_POINT('Ctrl Pts',(-2.57155495496598,-6.26178016800009,
25.6786354416283));
#15512=CARTESIAN_POINT('Ctrl Pts',(-2.40917046684931,-6.32602384639378,
25.6868487273157));
#15513=CARTESIAN_POINT('Ctrl Pts',(-2.24471079528138,-6.38385169357397,
25.6950620130031));
#15514=CARTESIAN_POINT('Ctrl Pts',(-2.0800105394831,-6.44176413576747,25.7032873137152));
#15515=CARTESIAN_POINT('Ctrl Pts',(-1.91322937621344,-6.49324188452043,
25.7115126144273));
#15516=CARTESIAN_POINT('Ctrl Pts',(-1.74491421651305,-6.53816207943874,
25.7197379151393));
#15517=CARTESIAN_POINT('Ctrl Pts',(-1.59269345805365,-6.57878697711747,
25.7271767074334));
#15518=CARTESIAN_POINT('Ctrl Pts',(-1.43921837185263,-6.61404906212829,
25.7346154997274));
#15519=CARTESIAN_POINT('Ctrl Pts',(-1.28489791656797,-6.64389391426438,
25.7420542920215));
#15520=CARTESIAN_POINT('Ctrl Pts',(-1.11577016883261,-6.67660242729955,
25.7502068482347));
#15521=CARTESIAN_POINT('Ctrl Pts',(-0.945128120729877,-6.70289988064057,
25.758359404448));
#15522=CARTESIAN_POINT('Ctrl Pts',(-0.773503444533528,-6.72264690589166,
25.7665119606613));
#15523=CARTESIAN_POINT('Ctrl Pts',(-0.60207759966208,-6.74237105373794,
25.7746550719416));
#15524=CARTESIAN_POINT('Ctrl Pts',(-0.429671752241763,-6.75555983842487,
25.7827981832219));
#15525=CARTESIAN_POINT('Ctrl Pts',(-0.2568294814744,-6.76212448993995,25.7909412945023));
#15526=CARTESIAN_POINT('Ctrl Pts',(-0.0841511147097744,-6.76868291628421,
25.7990766837796));
#15527=CARTESIAN_POINT('Ctrl Pts',(0.088962488684636,-6.76862970149317,
25.807212073057));
#15528=CARTESIAN_POINT('Ctrl Pts',(0.261960878240891,-6.7619276466309,25.8153474623343));
#15529=CARTESIAN_POINT('Ctrl Pts',(0.434831566884902,-6.75523053897376,
25.8234768463729));
#15530=CARTESIAN_POINT('Ctrl Pts',(0.60758684728569,-6.74189437787547,25.8316062304115));
#15531=CARTESIAN_POINT('Ctrl Pts',(0.779674507005852,-6.72193399723065,
25.8397356144501));
#15532=CARTESIAN_POINT('Ctrl Pts',(0.951671284719478,-6.70198415795438,
25.8478607052422));
#15533=CARTESIAN_POINT('Ctrl Pts',(1.12300078161399,-6.6754171082616,25.8559857960344));
#15534=CARTESIAN_POINT('Ctrl Pts',(1.29311415397371,-6.64229966086994,25.8641108868265));
#15535=CARTESIAN_POINT('Ctrl Pts',(1.46387688595396,-6.60905579700217,25.8722669928516));
#15536=CARTESIAN_POINT('Ctrl Pts',(1.6334138190361,-6.56921145038738,25.8804230988767));
#15537=CARTESIAN_POINT('Ctrl Pts',(1.80117786754283,-6.52288642316221,25.8885792049018));
#15538=CARTESIAN_POINT('Ctrl Pts',(1.96826669609484,-6.47674784579363,25.8967024840752));
#15539=CARTESIAN_POINT('Ctrl Pts',(2.13359653534583,-6.42418077690206,25.9048257632487));
#15540=CARTESIAN_POINT('Ctrl Pts',(2.29664024127731,-6.36535408301422,25.9129490424221));
#15541=CARTESIAN_POINT('Ctrl Pts',(2.45970565785597,-6.30651955585499,25.9210734032787));
#15542=CARTESIAN_POINT('Ctrl Pts',(2.62048399062375,-6.24142386764794,25.9291977641354));
#15543=CARTESIAN_POINT('Ctrl Pts',(2.77846645275301,-6.17028469123801,25.9373221249921));
#15544=CARTESIAN_POINT('Ctrl Pts',(2.93650000855845,-6.09912250745122,25.9454491133775));
#15545=CARTESIAN_POINT('Ctrl Pts',(3.09173555973837,-6.02191309346784,25.9535761017629));
#15546=CARTESIAN_POINT('Ctrl Pts',(3.2436874127479,-5.9389208589087,25.9617030901484));
#15547=CARTESIAN_POINT('Ctrl Pts',(3.39662161718698,-5.85539208900204,25.9698826185884));
#15548=CARTESIAN_POINT('Ctrl Pts',(3.54622918895365,-5.76600564888686,25.9780621470285));
#15549=CARTESIAN_POINT('Ctrl Pts',(3.69204389825408,-5.67107581093436,25.9862416754686));
#15550=CARTESIAN_POINT('Ctrl Pts',(3.83717191907995,-5.57659302819273,25.9943826838722));
#15551=CARTESIAN_POINT('Ctrl Pts',(3.97854246301319,-5.47661921000716,26.0025236922759));
#15552=CARTESIAN_POINT('Ctrl Pts',(4.11572880697669,-5.37150494623455,26.0106647006796));
#15553=CARTESIAN_POINT('Ctrl Pts',(4.25388881833464,-5.26564464369182,26.0188634891379));
#15554=CARTESIAN_POINT('Ctrl Pts',(4.38780472688166,-5.15457090068877,26.0270622775961));
#15555=CARTESIAN_POINT('Ctrl Pts',(4.51707841398514,-5.03867954943649,26.0352610660544));
#15556=CARTESIAN_POINT('Ctrl Pts',(4.64635210108859,-4.92278819818424,26.0434598545126));
#15557=CARTESIAN_POINT('Ctrl Pts',(4.77098334505881,-4.80207954358236,26.0516586429709));
#15558=CARTESIAN_POINT('Ctrl Pts',(4.89061549714208,-4.67698290130654,26.0598574314291));
#15559=CARTESIAN_POINT('Ctrl Pts',(5.01074757647513,-4.55136349638505,26.0680904815612));
#15560=CARTESIAN_POINT('Ctrl Pts',(5.12621221717435,-4.42092894380504,26.0763235316931));
#15561=CARTESIAN_POINT('Ctrl Pts',(5.23660054380631,-4.28605923251271,26.0845565818252));
#15562=CARTESIAN_POINT('Ctrl Pts',(5.3468574149097,-4.15135013031492,26.09277982766));
#15563=CARTESIAN_POINT('Ctrl Pts',(5.45204978461543,-4.01221666081912,26.1010030734949));
#15564=CARTESIAN_POINT('Ctrl Pts',(5.55180512777695,-3.86907596503216,26.1092263193297));
#15565=CARTESIAN_POINT('Ctrl Pts',(5.65146164390596,-3.72607707789172,26.1174414184432));
#15566=CARTESIAN_POINT('Ctrl Pts',(5.7456916572478,-3.57907916247656,26.1256565175568));
#15567=CARTESIAN_POINT('Ctrl Pts',(5.83416244742233,-3.42853285489392,26.1338716166703));
#15568=CARTESIAN_POINT('Ctrl Pts',(5.92256329132739,-3.27810557137085,26.1420802208092));
#15569=CARTESIAN_POINT('Ctrl Pts',(6.00521380071724,-3.12413579091115,26.150288824948));
#15570=CARTESIAN_POINT('Ctrl Pts',(6.08182413774452,-2.96710366477954,26.1584974290869));
#15571=CARTESIAN_POINT('Ctrl Pts',(6.15838922974909,-2.81016427968508,26.1667011853359));
#15572=CARTESIAN_POINT('Ctrl Pts',(6.22892109919551,-2.65016647290736,26.1749049415849));
#15573=CARTESIAN_POINT('Ctrl Pts',(6.29317546179498,-2.48761564697233,26.1831086978339));
#15574=CARTESIAN_POINT('Ctrl Pts',(6.35741081314813,-2.32511291572949,26.1913100267981));
#15575=CARTESIAN_POINT('Ctrl Pts',(6.41537222234622,-2.16005900126699,26.1995113557624));
#15576=CARTESIAN_POINT('Ctrl Pts',(6.4668631434036,-1.99298020173009,26.2077126847267));
#15577=CARTESIAN_POINT('Ctrl Pts',(6.51834696337138,-1.82592444395474,26.2159128826494));
#15578=CARTESIAN_POINT('Ctrl Pts',(6.56336196618395,-1.65684469931315,26.2241130805721));
#15579=CARTESIAN_POINT('Ctrl Pts',(6.60176117856937,-1.48628339866069,26.2323132784949));
#15580=CARTESIAN_POINT('Ctrl Pts',(6.6401620540554,-1.31571471086187,26.2405138315747));
#15581=CARTESIAN_POINT('Ctrl Pts',(6.67194648951085,-1.14366468875732,26.2487143846546));
#15582=CARTESIAN_POINT('Ctrl Pts',(6.69701842085514,-0.970687009662231,
26.2569149377344));
#15583=CARTESIAN_POINT('Ctrl Pts',(6.7220959816099,-0.797670491821714,26.2651173320876));
#15584=CARTESIAN_POINT('Ctrl Pts',(6.7404579850306,-0.623726256647637,26.2733197264408));
#15585=CARTESIAN_POINT('Ctrl Pts',(6.75206011876615,-0.449414232715902,
26.281522120794));
#15586=CARTESIAN_POINT('Ctrl Pts',(6.76367310253629,-0.274939196399476,
26.2897321858279));
#15587=CARTESIAN_POINT('Ctrl Pts',(6.7685135626335,-0.100096042103787,26.2979422508617));
#15588=CARTESIAN_POINT('Ctrl Pts',(6.76658930469254,0.0745532133478711,
26.3061523158955));
#15589=CARTESIAN_POINT('Ctrl Pts',(6.76466412583587,0.249286052834895,26.3143663101209));
#15590=CARTESIAN_POINT('Ctrl Pts',(6.75596779176654,0.423824450814262,26.3225803043462));
#15591=CARTESIAN_POINT('Ctrl Pts',(6.74056012172359,0.597610446218733,26.3307942985715));
#15592=CARTESIAN_POINT('Ctrl Pts',(6.72513144589468,0.771633369816078,26.3390194912067));
#15593=CARTESIAN_POINT('Ctrl Pts',(6.70297319358434,0.944901485324106,26.3472446838419));
#15594=CARTESIAN_POINT('Ctrl Pts',(6.67419673939501,1.11686475629284,26.3554698764771));
#15595=CARTESIAN_POINT('Ctrl Pts',(6.64831813577658,1.27151095756032,26.362866774597));
#15596=CARTESIAN_POINT('Ctrl Pts',(6.6170878758833,1.42510184517037,26.3702636727169));
#15597=CARTESIAN_POINT('Ctrl Pts',(6.58062140342001,1.57724790215442,26.3776605708368));
#15598=CARTESIAN_POINT('Ctrl Pts',(6.53799706361612,1.75508592142644,26.3863065373277));
#15599=CARTESIAN_POINT('Ctrl Pts',(6.48812158297308,1.93135347881673,26.3949525038186));
#15600=CARTESIAN_POINT('Ctrl Pts',(6.43112442046256,2.10545189651299,26.4035984703095));
#15601=CARTESIAN_POINT('Ctrl Pts',(6.37420016507141,2.27932761866508,26.4122333774339));
#15602=CARTESIAN_POINT('Ctrl Pts',(6.31017248731797,2.45103944546087,26.4208682845582));
#15603=CARTESIAN_POINT('Ctrl Pts',(6.23922127964424,2.62000130221999,26.4295031916826));
#15604=CARTESIAN_POINT('Ctrl Pts',(6.16591454914174,2.79457255625137,26.4384247707541));
#15605=CARTESIAN_POINT('Ctrl Pts',(6.08521672373981,2.96620779021715,26.4473463498256));
#15606=CARTESIAN_POINT('Ctrl Pts',(5.99738234333584,3.13427727360608,26.4562679288971));
#15607=CARTESIAN_POINT('Ctrl Pts',(5.91260508320171,3.29649701316977,26.4648789878728));
#15608=CARTESIAN_POINT('Ctrl Pts',(5.8211798022406,3.45539470966287,26.4734900468485));
#15609=CARTESIAN_POINT('Ctrl Pts',(5.72338450147232,3.61042363834308,26.4821011058242));
#15610=CARTESIAN_POINT('Ctrl Pts',(5.62568142618739,3.76530636758661,26.4907040441737));
#15611=CARTESIAN_POINT('Ctrl Pts',(5.52162047009277,3.9163273459469,26.4993069825233));
#15612=CARTESIAN_POINT('Ctrl Pts',(5.41152528634193,4.06296481344373,26.5079099208728));
#15613=CARTESIAN_POINT('Ctrl Pts',(5.301553383728,4.20943808089938,26.5165032259216));
#15614=CARTESIAN_POINT('Ctrl Pts',(5.18556091607221,4.35153738649489,26.5250965309703));
#15615=CARTESIAN_POINT('Ctrl Pts',(5.06391465684653,4.48877013759614,26.5336898360191));
#15616=CARTESIAN_POINT('Ctrl Pts',(5.05036127242228,4.50406011234023,26.5346472708596));
#15617=CARTESIAN_POINT('Ctrl Pts',(5.03673774779103,4.519289705993,26.5356047057001));
#15618=CARTESIAN_POINT('Ctrl Pts',(5.02304462287122,4.53445826054718,26.5365621405406));
#15619=CARTESIAN_POINT('Ctrl Pts',(4.90014406771514,4.67060130945246,26.5451554509876));
#15620=CARTESIAN_POINT('Ctrl Pts',(4.77177744694847,4.80166499942981,26.5537487614345));
#15621=CARTESIAN_POINT('Ctrl Pts',(4.63839361530321,4.92722981699803,26.5623420718815));
#15622=CARTESIAN_POINT('Ctrl Pts',(4.50480522001602,5.05298720660488,26.5709485614286));
#15623=CARTESIAN_POINT('Ctrl Pts',(4.36618445496601,5.17322865585952,26.5795550509758));
#15624=CARTESIAN_POINT('Ctrl Pts',(4.22301459726595,5.28757380196993,26.5881615405229));
#15625=CARTESIAN_POINT('Ctrl Pts',(4.07972726804998,5.40201276879,26.5967750917337));
#15626=CARTESIAN_POINT('Ctrl Pts',(3.93188363982436,5.51054559246033,26.6053886429444));
#15627=CARTESIAN_POINT('Ctrl Pts',(3.77999676986812,5.61283470447746,26.6140021941552));
#15628=CARTESIAN_POINT('Ctrl Pts',(3.62789099708477,5.71527123789981,26.6226281594128));
#15629=CARTESIAN_POINT('Ctrl Pts',(3.47173059280552,5.81144590923214,26.6312541246703));
#15630=CARTESIAN_POINT('Ctrl Pts',(3.31205548077479,5.90106579291146,26.6398800899279));
#15631=CARTESIAN_POINT('Ctrl Pts',(3.2417606655077,5.94051973840976,26.6436775548337));
#15632=CARTESIAN_POINT('Ctrl Pts',(3.17078496699069,5.97870392470271,26.6474750197396));
#15633=CARTESIAN_POINT('Ctrl Pts',(3.09917575053263,6.01559628526637,26.6512724846455));
#15634=CARTESIAN_POINT('Origin',(0.,0.,-3.69717978381041));
#15635=CARTESIAN_POINT('',(3.09917575053261,6.01559628526638,29.0458547647091));
#15636=CARTESIAN_POINT('',(3.09917575053261,6.01559628526638,28.6513920151221));
#15637=CARTESIAN_POINT('',(3.09917575053259,6.01559628526639,-3.69717978381041));
#15638=CARTESIAN_POINT('',(-6.76699999999596,7.3958191851709E-6,27.697339049466));
#15639=CARTESIAN_POINT('Ctrl Pts',(-6.76699999999596,7.39581918517091E-6,
27.6973390494661));
#15640=CARTESIAN_POINT('Ctrl Pts',(-6.7670001871494,-0.171233584460114,
27.7054383317461));
#15641=CARTESIAN_POINT('Ctrl Pts',(-6.76049611965891,-0.342743673478981,
27.7135376140262));
#15642=CARTESIAN_POINT('Ctrl Pts',(-6.74745237752025,-0.513979973439041,
27.7216368963063));
#15643=CARTESIAN_POINT('Ctrl Pts',(-6.73442294962769,-0.685028358112737,
27.729727290407));
#15644=CARTESIAN_POINT('Ctrl Pts',(-6.71486815859784,-0.855803185644681,
27.7378176845078));
#15645=CARTESIAN_POINT('Ctrl Pts',(-6.68880455166524,-1.02575955741215,
27.7459080786085));
#15646=CARTESIAN_POINT('Ctrl Pts',(-6.66276391060138,-1.19556617263457,
27.7539913438828));
#15647=CARTESIAN_POINT('Ctrl Pts',(-6.63022592605018,-1.36455540354692,
27.7620746091571));
#15648=CARTESIAN_POINT('Ctrl Pts',(-6.59125909384202,-1.53218554941786,
27.7701578744315));
#15649=CARTESIAN_POINT('Ctrl Pts',(-6.55231817769273,-1.69970420783952,
27.7782357636881));
#15650=CARTESIAN_POINT('Ctrl Pts',(-6.50695701034635,-1.8658652211098,27.7863136529448));
#15651=CARTESIAN_POINT('Ctrl Pts',(-6.45529548783639,-2.03013525774001,
27.7943915422014));
#15652=CARTESIAN_POINT('Ctrl Pts',(-6.40365324082806,-2.19434400335125,
27.8024664175057));
#15653=CARTESIAN_POINT('Ctrl Pts',(-6.34571542684727,-2.35666282306734,
27.81054129281));
#15654=CARTESIAN_POINT('Ctrl Pts',(-6.28165231030984,-2.51657172605493,
27.8186161681143));
#15655=CARTESIAN_POINT('Ctrl Pts',(-6.21760043702092,-2.67645256460179,
27.8266896262563));
#15656=CARTESIAN_POINT('Ctrl Pts',(-6.14742553805268,-2.83392398395428,
27.8347630843984));
#15657=CARTESIAN_POINT('Ctrl Pts',(-6.07134667402418,-2.98848432550943,
27.8428365425405));
#15658=CARTESIAN_POINT('Ctrl Pts',(-5.99526628605105,-3.14304776308088,
27.8509101624029));
#15659=CARTESIAN_POINT('Ctrl Pts',(-5.91328186144791,-3.29469967410902,
27.8589837822653));
#15660=CARTESIAN_POINT('Ctrl Pts',(-5.8256591765079,-3.44296153901975,27.8670574021278));
#15661=CARTESIAN_POINT('Ctrl Pts',(-5.73801760162649,-3.59125536663447,
27.8751327625236));
#15662=CARTESIAN_POINT('Ctrl Pts',(-5.64473553593836,-3.73615737450748,
27.8832081229194));
#15663=CARTESIAN_POINT('Ctrl Pts',(-5.54612290580404,-3.87721674835387,
27.8912834833152));
#15664=CARTESIAN_POINT('Ctrl Pts',(-5.44741973880581,-4.01840562968135,
27.8993662577492));
#15665=CARTESIAN_POINT('Ctrl Pts',(-5.34337644596035,-4.15574452702552,
27.9074490321831));
#15666=CARTESIAN_POINT('Ctrl Pts',(-5.23434462480224,-4.28881397927259,
27.9155318066171));
#15667=CARTESIAN_POINT('Ctrl Pts',(-5.12525870432285,-4.42194945781337,
27.9236185915556));
#15668=CARTESIAN_POINT('Ctrl Pts',(-5.01117956973517,-4.55081099376952,
27.9317053764941));
#15669=CARTESIAN_POINT('Ctrl Pts',(-4.89249644265667,-4.67501524688335,
27.9397921614326));
#15670=CARTESIAN_POINT('Ctrl Pts',(-4.77365744848353,-4.79938261801195,
27.9478895667828));
#15671=CARTESIAN_POINT('Ctrl Pts',(-4.65020265096941,-4.91908023243594,
27.955986972133));
#15672=CARTESIAN_POINT('Ctrl Pts',(-4.52255582591572,-5.0337637808578,27.9640843774833));
#15673=CARTESIAN_POINT('Ctrl Pts',(-4.43712508178286,-5.11051853662517,
27.9695037630757));
#15674=CARTESIAN_POINT('Ctrl Pts',(-4.3498172885982,-5.18502819536259,27.9749231486681));
#15675=CARTESIAN_POINT('Ctrl Pts',(-4.26076671589499,-5.25720039495561,
27.9803425342605));
#15676=CARTESIAN_POINT('Ctrl Pts',(-4.1187015074195,-5.3723389984488,27.9889882523129));
#15677=CARTESIAN_POINT('Ctrl Pts',(-3.97183944392423,-5.48181868174055,
27.9976339703653));
#15678=CARTESIAN_POINT('Ctrl Pts',(-3.82064751921616,-5.58524319380163,
28.0062796884177));
#15679=CARTESIAN_POINT('Ctrl Pts',(-3.66964969412752,-5.68853492986644,
28.01491430713));
#15680=CARTESIAN_POINT('Ctrl Pts',(-3.51433334259644,-5.78578682430486,
28.0235489258424));
#15681=CARTESIAN_POINT('Ctrl Pts',(-3.35519781121756,-5.87664331464833,
28.0321835445547));
#15682=CARTESIAN_POINT('Ctrl Pts',(-3.19044223106302,-5.97070850328118,
28.0411231044572));
#15683=CARTESIAN_POINT('Ctrl Pts',(-3.02159302174582,-6.05791809718382,
28.0500626643596));
#15684=CARTESIAN_POINT('Ctrl Pts',(-2.84923897316472,-6.13792524178971,
28.059002224262));
#15685=CARTESIAN_POINT('Ctrl Pts',(-2.68322621993108,-6.214988742553,28.0676128775325));
#15686=CARTESIAN_POINT('Ctrl Pts',(-2.51396222508625,-6.28537014078503,
28.076223530803));
#15687=CARTESIAN_POINT('Ctrl Pts',(-2.3420002894792,-6.34880489888289,28.0848341840735));
#15688=CARTESIAN_POINT('Ctrl Pts',(-2.17020112735028,-6.41217961173775,
28.0934366867846));
#15689=CARTESIAN_POINT('Ctrl Pts',(-1.99570940121295,-6.46862068895084,
28.1020391894956));
#15690=CARTESIAN_POINT('Ctrl Pts',(-1.81909943967783,-6.51791118599846,
28.1106416922067));
#15691=CARTESIAN_POINT('Ctrl Pts',(-1.64268824909843,-6.56714620758409,
28.1192345129741));
#15692=CARTESIAN_POINT('Ctrl Pts',(-1.46416387233321,-6.60924662238,28.1278273337415));
#15693=CARTESIAN_POINT('Ctrl Pts',(-1.28411709459676,-6.64404487397281,
28.136420154509));
#15694=CARTESIAN_POINT('Ctrl Pts',(-1.26289776402047,-6.64814600598588,
28.1374328574673));
#15695=CARTESIAN_POINT('Ctrl Pts',(-1.24165730587066,-6.6521457698848,28.1384455604256));
#15696=CARTESIAN_POINT('Ctrl Pts',(-1.22039670119667,-6.65604393703259,
28.1394582633839));
#15697=CARTESIAN_POINT('Ctrl Pts',(-1.0399485492394,-6.68912940513782,28.148053521144));
#15698=CARTESIAN_POINT('Ctrl Pts',(-0.858260506854818,-6.71485308769088,
28.1566487789041));
#15699=CARTESIAN_POINT('Ctrl Pts',(-0.675944585442873,-6.73315586611587,
28.1652440366641));
#15700=CARTESIAN_POINT('Ctrl Pts',(-0.49345793290357,-6.75147578431653,
28.1738473435185));
#15701=CARTESIAN_POINT('Ctrl Pts',(-0.310342531523026,-6.76236089669446,
28.1824506503729));
#15702=CARTESIAN_POINT('Ctrl Pts',(-0.127212719760841,-6.76580415944262,
28.1910539572273));
#15703=CARTESIAN_POINT('Ctrl Pts',(0.0635097175020141,-6.76939018105836,
28.2000139601673));
#15704=CARTESIAN_POINT('Ctrl Pts',(0.254247404219202,-6.76490412677074,
28.2089739631073));
#15705=CARTESIAN_POINT('Ctrl Pts',(0.444311025072017,-6.75239784913474,
28.2179339660473));
#15706=CARTESIAN_POINT('Ctrl Pts',(0.627307511456925,-6.74035659234465,
28.226560809252));
#15707=CARTESIAN_POINT('Ctrl Pts',(0.809678866323325,-6.72088086671166,
28.2351876524568));
#15708=CARTESIAN_POINT('Ctrl Pts',(0.990818715418065,-6.69406955992969,
28.2438144956615));
#15709=CARTESIAN_POINT('Ctrl Pts',(1.17213168842088,-6.66723262831568,28.2524495839477));
#15710=CARTESIAN_POINT('Ctrl Pts',(1.35221050620472,-6.63304617489905,28.2610846722338));
#15711=CARTESIAN_POINT('Ctrl Pts',(1.53046029707631,-6.59165990317106,28.26971976052));
#15712=CARTESIAN_POINT('Ctrl Pts',(1.70897482465772,-6.55021216452434,28.2783676736451));
#15713=CARTESIAN_POINT('Ctrl Pts',(1.88565460173273,-6.50154331568327,28.2870155867703));
#15714=CARTESIAN_POINT('Ctrl Pts',(2.05991974628415,-6.44585290236045,28.2956634998954));
#15715=CARTESIAN_POINT('Ctrl Pts',(2.07946964263483,-6.43960528577028,28.2966336640994));
#15716=CARTESIAN_POINT('Ctrl Pts',(2.09898917067941,-6.43326934959204,28.2976038283034));
#15717=CARTESIAN_POINT('Ctrl Pts',(2.11847752795635,-6.42684541307351,28.2985739925073));
#15718=CARTESIAN_POINT('Ctrl Pts',(2.2836923362251,-6.37238574645526,28.3067986720261));
#15719=CARTESIAN_POINT('Ctrl Pts',(2.44702352994461,-6.31147945826268,28.3150233515449));
#15720=CARTESIAN_POINT('Ctrl Pts',(2.60793262039289,-6.24427549420193,28.3232480310637));
#15721=CARTESIAN_POINT('Ctrl Pts',(2.76867257718289,-6.17714216911042,28.3314640655139));
#15722=CARTESIAN_POINT('Ctrl Pts',(2.92699517249097,-6.1037244870511,28.339680099964));
#15723=CARTESIAN_POINT('Ctrl Pts',(3.08237717381573,-6.02422110802216,28.3478961344141));
#15724=CARTESIAN_POINT('Ctrl Pts',(3.2376269743666,-5.94478537137229,28.3561051785687));
#15725=CARTESIAN_POINT('Ctrl Pts',(3.38994084646355,-5.85927441225564,28.3643142227233));
#15726=CARTESIAN_POINT('Ctrl Pts',(3.53881556117961,-5.76793493582869,28.3725232668779));
#15727=CARTESIAN_POINT('Ctrl Pts',(3.68759342304055,-5.6766548817764,28.3807269705059));
#15728=CARTESIAN_POINT('Ctrl Pts',(3.83293627981061,-5.57955405018017,28.3889306741339));
#15729=CARTESIAN_POINT('Ctrl Pts',(3.97436546645699,-5.47692506238986,28.397134377762));
#15730=CARTESIAN_POINT('Ctrl Pts',(4.11573095881104,-5.37434229476742,28.4053343867559));
#15731=CARTESIAN_POINT('Ctrl Pts',(4.25318600307345,-5.26623654112658,28.4135343957499));
#15732=CARTESIAN_POINT('Ctrl Pts',(4.38628082680189,-5.15294377113026,28.4217344047438));
#15733=CARTESIAN_POINT('Ctrl Pts',(4.5193650079878,-5.03966006026253,28.4299337580477));
#15734=CARTESIAN_POINT('Ctrl Pts',(4.64808938472012,-4.92119038467458,28.4381331113517));
#15735=CARTESIAN_POINT('Ctrl Pts',(4.77203692199466,-4.79791127628677,28.4463324646556));
#15736=CARTESIAN_POINT('Ctrl Pts',(4.895983651168,-4.67463297164222,28.4545317645022));
#15737=CARTESIAN_POINT('Ctrl Pts',(5.01515334795759,-4.54654554870679,28.4627310643488));
#15738=CARTESIAN_POINT('Ctrl Pts',(5.12916564295834,-4.41406261929934,28.4709303641954));
#15739=CARTESIAN_POINT('Ctrl Pts',(5.24319787758171,-4.28155651993802,28.4791310980184));
#15740=CARTESIAN_POINT('Ctrl Pts',(5.3520706795134,-4.14465365428574,28.4873318318415));
#15741=CARTESIAN_POINT('Ctrl Pts',(5.45544377045798,-4.00380097749267,28.4955325656645));
#15742=CARTESIAN_POINT('Ctrl Pts',(5.55885369343053,-3.86289811462424,28.5037362214245));
#15743=CARTESIAN_POINT('Ctrl Pts',(5.65675978988914,-3.71804292599986,28.5119398771845));
#15744=CARTESIAN_POINT('Ctrl Pts',(5.74886490813213,-3.56971165054643,28.5201435329445));
#15745=CARTESIAN_POINT('Ctrl Pts',(5.84107553870865,-3.42121045208214,28.5283565865195));
#15746=CARTESIAN_POINT('Ctrl Pts',(5.92747172529262,-3.2692255161059,28.5365696400945));
#15747=CARTESIAN_POINT('Ctrl Pts',(6.00780161352396,-3.11425894436203,28.5447826936696));
#15748=CARTESIAN_POINT('Ctrl Pts',(6.08817903475258,-2.95920067542058,28.5530006070927));
#15749=CARTESIAN_POINT('Ctrl Pts',(6.16248284999782,-2.80115757771115,28.5612185205158));
#15750=CARTESIAN_POINT('Ctrl Pts',(6.2305093065635,-2.64065196132048,28.5694364339389));
#15751=CARTESIAN_POINT('Ctrl Pts',(6.29864186145479,-2.47989601030985,28.5776671645348));
#15752=CARTESIAN_POINT('Ctrl Pts',(6.36047736501064,-2.31667020032072,28.5858978951308));
#15753=CARTESIAN_POINT('Ctrl Pts',(6.41586148173165,-2.15151352476162,28.5941286257268));
#15754=CARTESIAN_POINT('Ctrl Pts',(6.46672516912585,-1.99983687062231,28.6016875674026));
#15755=CARTESIAN_POINT('Ctrl Pts',(6.51214814331083,-1.8465320462207,28.6092465090784));
#15756=CARTESIAN_POINT('Ctrl Pts',(6.55204900943375,-1.69202327938424,28.6168054507542));
#15757=CARTESIAN_POINT('Ctrl Pts',(6.59509039983991,-1.5253534097605,28.6249593429209));
#15758=CARTESIAN_POINT('Ctrl Pts',(6.63183856457751,-1.35676713161329,28.6331132350877));
#15759=CARTESIAN_POINT('Ctrl Pts',(6.66211904056673,-1.18678510662979,28.6412671272544));
#15760=CARTESIAN_POINT('Ctrl Pts',(6.69236256591543,-1.01701050720664,28.6494110693946));
#15761=CARTESIAN_POINT('Ctrl Pts',(6.71615404910189,-0.845843907220032,
28.6575550115349));
#15762=CARTESIAN_POINT('Ctrl Pts',(6.73336868715609,-0.67382128404045,28.6656989536751));
#15763=CARTESIAN_POINT('Ctrl Pts',(6.75056594188028,-0.501972369190823,
28.673834672068));
#15764=CARTESIAN_POINT('Ctrl Pts',(6.7611995368463,-0.32926951311978,28.6819703904609));
#15765=CARTESIAN_POINT('Ctrl Pts',(6.76519564457517,-0.156259049725841,
28.6901061088538));
#15766=CARTESIAN_POINT('Ctrl Pts',(6.76918855761934,0.016613100610356,28.6982353231541));
#15767=CARTESIAN_POINT('Ctrl Pts',(6.76655454048679,0.189792004779849,28.7063645374543));
#15768=CARTESIAN_POINT('Ctrl Pts',(6.7572715514346,0.362726040108322,28.7144937517545));
#15769=CARTESIAN_POINT('Ctrl Pts',(6.7479940317959,0.535558185006852,28.72261817643));
#15770=CARTESIAN_POINT('Ctrl Pts',(6.7320753613025,0.708145384171316,28.7307426011054));
#15771=CARTESIAN_POINT('Ctrl Pts',(6.7095455806479,0.879935850621083,28.7388670257809));
#15772=CARTESIAN_POINT('Ctrl Pts',(6.68687902980205,1.05276919517562,28.747040770915));
#15773=CARTESIAN_POINT('Ctrl Pts',(6.65752083013231,1.22479572676368,28.7552145160492));
#15774=CARTESIAN_POINT('Ctrl Pts',(6.6215546500722,1.39545799510671,28.7633882611834));
#15775=CARTESIAN_POINT('Ctrl Pts',(6.58581878690473,1.56502739222267,28.7715096640455));
#15776=CARTESIAN_POINT('Ctrl Pts',(6.54355942600176,1.73324959017862,28.7796310669077));
#15777=CARTESIAN_POINT('Ctrl Pts',(6.49491000028617,1.89958761003085,28.7877524697698));
#15778=CARTESIAN_POINT('Ctrl Pts',(6.4462568132529,2.06593849026376,28.7958745005361));
#15779=CARTESIAN_POINT('Ctrl Pts',(6.39121268000612,2.23040455093347,28.8039965313024));
#15780=CARTESIAN_POINT('Ctrl Pts',(6.32996096589675,2.39246382840441,28.8121185620687));
#15781=CARTESIAN_POINT('Ctrl Pts',(6.26869285238683,2.5545664952734,28.8202427674098));
#15782=CARTESIAN_POINT('Ctrl Pts',(6.20121397800711,2.71426075364746,28.8283669727509));
#15783=CARTESIAN_POINT('Ctrl Pts',(6.12775589813451,2.8710445229703,28.836491178092));
#15784=CARTESIAN_POINT('Ctrl Pts',(6.05350268537644,3.02952536810989,28.8447033223344));
#15785=CARTESIAN_POINT('Ctrl Pts',(5.97314023139421,3.1850320002565,28.8529154665768));
#15786=CARTESIAN_POINT('Ctrl Pts',(5.88695500353489,3.33707203793319,28.8611276108192));
#15787=CARTESIAN_POINT('Ctrl Pts',(5.80155655181722,3.48772411763622,28.8692647872357));
#15788=CARTESIAN_POINT('Ctrl Pts',(5.71044144084553,3.63497235413459,28.8774019636521));
#15789=CARTESIAN_POINT('Ctrl Pts',(5.61393136346961,3.77836785480878,28.8855391400686));
#15790=CARTESIAN_POINT('Ctrl Pts',(5.5160875647302,3.92374501012336,28.893788768224));
#15791=CARTESIAN_POINT('Ctrl Pts',(5.41269882774057,4.06516184721682,28.9020383963794));
#15792=CARTESIAN_POINT('Ctrl Pts',(5.30414154170348,4.20218651484861,28.9102880245348));
#15793=CARTESIAN_POINT('Ctrl Pts',(5.19558425566639,4.3392111824804,28.9185376526901));
#15794=CARTESIAN_POINT('Ctrl Pts',(5.08185871906685,4.47184342972856,28.9267872808455));
#15795=CARTESIAN_POINT('Ctrl Pts',(4.96337853470024,4.59969156805942,28.9350369090009));
#15796=CARTESIAN_POINT('Ctrl Pts',(4.84522764745455,4.72718437250814,28.9432636086066));
#15797=CARTESIAN_POINT('Ctrl Pts',(4.72199538861972,4.85030091817577,28.9514903082122));
#15798=CARTESIAN_POINT('Ctrl Pts',(4.59403826583033,4.9686116181572,28.9597170078178));
#15799=CARTESIAN_POINT('Ctrl Pts',(4.46626343348551,5.0867537701936,28.9679319874919));
#15800=CARTESIAN_POINT('Ctrl Pts',(4.33377741238652,5.20010347884628,28.9761469671659));
#15801=CARTESIAN_POINT('Ctrl Pts',(4.19697549336839,5.30826579101548,28.9843619468399));
#15802=CARTESIAN_POINT('Ctrl Pts',(4.06028604074079,5.41633918173585,28.9925701728871));
#15803=CARTESIAN_POINT('Ctrl Pts',(3.91928803241086,5.51923344367897,29.0007783989343));
#15804=CARTESIAN_POINT('Ctrl Pts',(3.77441252464447,5.61659141239658,29.0089866249815));
#15805=CARTESIAN_POINT('Ctrl Pts',(3.62965041303379,5.71387317762368,29.0171884263315));
#15806=CARTESIAN_POINT('Ctrl Pts',(3.4810171454555,5.80562708406218,29.0253902276814));
#15807=CARTESIAN_POINT('Ctrl Pts',(3.32897552920618,5.89153722944585,29.0335920290313));
#15808=CARTESIAN_POINT('Ctrl Pts',(3.25320168097652,5.93435275902437,29.0376796075906));
#15809=CARTESIAN_POINT('Ctrl Pts',(3.17658175697615,5.97571747579524,29.0417671861499));
#15810=CARTESIAN_POINT('Ctrl Pts',(3.09917575053261,6.01559628526638,29.0458547647091));
#15811=CARTESIAN_POINT('Ctrl Pts',(3.09917575053259,6.01559628526639,27.0457515827422));
#15812=CARTESIAN_POINT('Ctrl Pts',(2.93382384459261,6.10078395293761,27.0545010306546));
#15813=CARTESIAN_POINT('Ctrl Pts',(2.76495772122976,6.17915010267053,27.063250478567));
#15814=CARTESIAN_POINT('Ctrl Pts',(2.59315093316698,6.25042856433183,27.0719999264794));
#15815=CARTESIAN_POINT('Ctrl Pts',(2.42134553245604,6.32170645041456,27.0807493037394));
#15816=CARTESIAN_POINT('Ctrl Pts',(2.24659977927578,6.38589665313462,27.0894986809994));
#15817=CARTESIAN_POINT('Ctrl Pts',(2.06950718689906,6.44278115439079,27.0982480582594));
#15818=CARTESIAN_POINT('Ctrl Pts',(1.89241596572848,6.49966521519728,27.1069973677741));
#15819=CARTESIAN_POINT('Ctrl Pts',(1.71297821457185,6.54924360009549,27.1157466772887));
#15820=CARTESIAN_POINT('Ctrl Pts',(1.53180337335832,6.59134792173559,27.1244959868034));
#15821=CARTESIAN_POINT('Ctrl Pts',(1.35062987477783,6.63345193135304,27.1332452314795));
#15822=CARTESIAN_POINT('Ctrl Pts',(1.16771959102965,6.66808192368235,27.1419944761556));
#15823=CARTESIAN_POINT('Ctrl Pts',(0.983693746907115,6.69512028363164,27.1507437208317));
#15824=CARTESIAN_POINT('Ctrl Pts',(0.799669205420143,6.72215845218864,27.1594929035759));
#15825=CARTESIAN_POINT('Ctrl Pts',(0.614529402873749,6.74160505424577,27.1682420863201));
#15826=CARTESIAN_POINT('Ctrl Pts',(0.428903127363522,6.7533940435412,27.1769912690643));
#15827=CARTESIAN_POINT('Ctrl Pts',(0.243278104164177,6.76518295330329,27.1857403927829));
#15828=CARTESIAN_POINT('Ctrl Pts',(0.0571669005394398,6.76931433552275,
27.1944895165015));
#15829=CARTESIAN_POINT('Ctrl Pts',(-0.128798404777167,6.76577415902474,
27.2032386402201));
#15830=CARTESIAN_POINT('Ctrl Pts',(-0.314762517258715,6.76223400523443,
27.2119877078193));
#15831=CARTESIAN_POINT('Ctrl Pts',(-0.500580446819089,6.75102239665092,
27.2207367754185));
#15832=CARTESIAN_POINT('Ctrl Pts',(-0.685621118842153,6.73217741012502,
27.2294858430177));
#15833=CARTESIAN_POINT('Ctrl Pts',(-0.870660665414015,6.71333253821778,
27.2382348574035));
#15834=CARTESIAN_POINT('Ctrl Pts',(-1.05492267885438,6.6868544103062,27.2469838717893));
#15835=CARTESIAN_POINT('Ctrl Pts',(-1.23778137635202,6.65283295028187,27.255732886175));
#15836=CARTESIAN_POINT('Ctrl Pts',(-1.429999229788,6.61707018861875,27.2649296965424));
#15837=CARTESIAN_POINT('Ctrl Pts',(-1.62066601233653,6.57297172934423,27.2741265069098));
#15838=CARTESIAN_POINT('Ctrl Pts',(-1.80906628500347,6.52070304311305,27.2833233172772));
#15839=CARTESIAN_POINT('Ctrl Pts',(-1.98831342545486,6.47097374915043,27.292073315015));
#15840=CARTESIAN_POINT('Ctrl Pts',(-2.16550875896657,6.41384933989543,27.3008233127528));
#15841=CARTESIAN_POINT('Ctrl Pts',(-2.34005036713964,6.34952386240493,27.3095733104905));
#15842=CARTESIAN_POINT('Ctrl Pts',(-2.51458843547038,6.28519968948616,27.3183231307714));
#15843=CARTESIAN_POINT('Ctrl Pts',(-2.68647261718,6.21367483971123,27.3270729510522));
#15844=CARTESIAN_POINT('Ctrl Pts',(-2.85511905908673,6.13519226743871,27.3358227713331));
#15845=CARTESIAN_POINT('Ctrl Pts',(-3.02376230488819,6.05671118252969,27.3445724257916));
#15846=CARTESIAN_POINT('Ctrl Pts',(-3.18916767379834,5.9712727599267,27.3533220802502));
#15847=CARTESIAN_POINT('Ctrl Pts',(-3.35077334102712,5.8791672043804,27.3620717347087));
#15848=CARTESIAN_POINT('Ctrl Pts',(-3.5123761603729,5.7870632719569,27.3708212349771));
#15849=CARTESIAN_POINT('Ctrl Pts',(-3.6701791630222,5.6882925836235,27.3795707352456));
#15850=CARTESIAN_POINT('Ctrl Pts',(-3.82364636566381,5.58319061741098,27.388320235514));
#15851=CARTESIAN_POINT('Ctrl Pts',(-3.97711106778721,5.47809036367758,27.3970695932225));
#15852=CARTESIAN_POINT('Ctrl Pts',(-4.12623987481854,5.36665920043281,27.4058189509309));
#15853=CARTESIAN_POINT('Ctrl Pts',(-4.27052628213861,5.24927559512391,27.4145683086393));
#15854=CARTESIAN_POINT('Ctrl Pts',(-4.41481053024924,5.13189374643084,27.4233175354159));
#15855=CARTESIAN_POINT('Ctrl Pts',(-4.5542523013649,5.00855981477391,27.4320667621924));
#15856=CARTESIAN_POINT('Ctrl Pts',(-4.6883780063052,4.87969268192103,27.4408159889689));
#15857=CARTESIAN_POINT('Ctrl Pts',(-4.82250188228861,4.75082730631843,27.4495650964397));
#15858=CARTESIAN_POINT('Ctrl Pts',(-4.95130963052928,4.61642907903566,27.4583142039106));
#15859=CARTESIAN_POINT('Ctrl Pts',(-5.07436379033325,4.47695444731737,27.4670633113814));
#15860=CARTESIAN_POINT('Ctrl Pts',(-5.19741643562769,4.3374815322063,27.4758123111712));
#15861=CARTESIAN_POINT('Ctrl Pts',(-5.31471544462742,4.19293255254629,27.4845613109609));
#15862=CARTESIAN_POINT('Ctrl Pts',(-5.42586245275601,4.04379841779638,27.4933103107507));
#15863=CARTESIAN_POINT('Ctrl Pts',(-5.53702160019125,3.89464799484383,27.5020602660928));
#15864=CARTESIAN_POINT('Ctrl Pts',(-5.64202723081222,3.74091164443895,27.510810221435));
#15865=CARTESIAN_POINT('Ctrl Pts',(-5.74052265232936,3.58311159163283,27.5195601767771));
#15866=CARTESIAN_POINT('Ctrl Pts',(-5.83901427066894,3.42531763191825,27.5283097942596));
#15867=CARTESIAN_POINT('Ctrl Pts',(-5.93099603115722,3.26346052695645,27.537059411742));
#15868=CARTESIAN_POINT('Ctrl Pts',(-6.01615550622742,3.09809004467099,27.5458090292245));
#15869=CARTESIAN_POINT('Ctrl Pts',(-6.10131214578801,2.93272506863826,27.5545583553756));
#15870=CARTESIAN_POINT('Ctrl Pts',(-6.17964682328761,2.76384720416866,27.5633076815267));
#15871=CARTESIAN_POINT('Ctrl Pts',(-6.25089348288587,2.59203002791538,27.5720570076778));
#15872=CARTESIAN_POINT('Ctrl Pts',(-6.3221381488934,2.42021765937001,27.5808060890094));
#15873=CARTESIAN_POINT('Ctrl Pts',(-6.38629508412584,2.24546640831917,27.5895551703409));
#15874=CARTESIAN_POINT('Ctrl Pts',(-6.44314639819803,2.0683697666007,27.5983042516725));
#15875=CARTESIAN_POINT('Ctrl Pts',(-6.50000285283692,1.89125711158305,27.6070541241069));
#15876=CARTESIAN_POINT('Ctrl Pts',(-6.54955227673241,1.71179891440286,27.6158039965413));
#15877=CARTESIAN_POINT('Ctrl Pts',(-6.59162635926377,1.53060476278464,27.6245538689757));
#15878=CARTESIAN_POINT('Ctrl Pts',(-6.63369752055188,1.34942319164737,27.6333031338982));
#15879=CARTESIAN_POINT('Ctrl Pts',(-6.66829431424245,1.16650618642754,27.6420523988207));
#15880=CARTESIAN_POINT('Ctrl Pts',(-6.69529923745409,0.982474997619145,
27.6508016637432));
#15881=CARTESIAN_POINT('Ctrl Pts',(-6.72230554731437,0.7984343591783,27.6595513779229));
#15882=CARTESIAN_POINT('Ctrl Pts',(-6.74171916496698,0.613279706240868,
27.6683010921026));
#15883=CARTESIAN_POINT('Ctrl Pts',(-6.75347414817272,0.427639953655878,
27.6770508062823));
#15884=CARTESIAN_POINT('Ctrl Pts',(-6.76248837758744,0.285283364198805,
27.6837604654582));
#15885=CARTESIAN_POINT('Ctrl Pts',(-6.76699999999997,0.142641701105077,
27.6904701246341));
#15886=CARTESIAN_POINT('Ctrl Pts',(-6.767,1.25880014828821E-12,27.69717978381));
#15887=CARTESIAN_POINT('',(-6.76699999814636,-0.000158389305696416,27.3028276665937));
#15888=CARTESIAN_POINT('Ctrl Pts',(3.09917575053263,6.01559628526637,26.6512724846455));
#15889=CARTESIAN_POINT('Ctrl Pts',(2.93615363517035,6.09958366785864,26.6599176115243));
#15890=CARTESIAN_POINT('Ctrl Pts',(2.7698470990166,6.17687257815703,26.6685627384031));
#15891=CARTESIAN_POINT('Ctrl Pts',(2.60082787562788,6.24723805864296,26.6772078652819));
#15892=CARTESIAN_POINT('Ctrl Pts',(2.48185569699916,6.29676813188447,26.6832931469361));
#15893=CARTESIAN_POINT('Ctrl Pts',(2.36153985499742,6.342868865374,26.6893784285903));
#15894=CARTESIAN_POINT('Ctrl Pts',(2.24008408109763,6.38547667050887,26.6954637102445));
#15895=CARTESIAN_POINT('Ctrl Pts',(2.07590198617098,6.44307326293634,26.7036897027858));
#15896=CARTESIAN_POINT('Ctrl Pts',(1.90928160896034,6.49440925938956,26.7119156953272));
#15897=CARTESIAN_POINT('Ctrl Pts',(1.7407407993885,6.53927446046916,26.7201416878685));
#15898=CARTESIAN_POINT('Ctrl Pts',(1.57237668307084,6.58409262618447,26.7283590565199));
#15899=CARTESIAN_POINT('Ctrl Pts',(1.40209648705597,6.62245341415902,26.7365764251714));
#15900=CARTESIAN_POINT('Ctrl Pts',(1.23043626458179,6.65419533819094,26.7447937938228));
#15901=CARTESIAN_POINT('Ctrl Pts',(1.05892165719612,6.68591033633979,26.7530041918852));
#15902=CARTESIAN_POINT('Ctrl Pts',(0.886029705179472,6.71101758802962,26.7612145899475));
#15903=CARTESIAN_POINT('Ctrl Pts',(0.712309885730461,6.72940588957827,26.7694249880099));
#15904=CARTESIAN_POINT('Ctrl Pts',(0.538702677679996,6.74778227117236,26.7776300637987));
#15905=CARTESIAN_POINT('Ctrl Pts',(0.364269026195079,6.75944834081458,26.7858351395875));
#15906=CARTESIAN_POINT('Ctrl Pts',(0.189566921231981,6.76434426846939,26.7940402153763));
#15907=CARTESIAN_POINT('Ctrl Pts',(0.0149431242319189,6.76923800158783,
26.8022416133458));
#15908=CARTESIAN_POINT('Ctrl Pts',(-0.159948529112916,6.76736762857281,
26.8104430113153));
#15909=CARTESIAN_POINT('Ctrl Pts',(-0.334546531099286,6.75872529538888,
26.8186444092848));
#15910=CARTESIAN_POINT('Ctrl Pts',(-0.509130857116212,6.75008363914445,
26.8268451648525));
#15911=CARTESIAN_POINT('Ctrl Pts',(-0.683421219594534,6.73467108828651,
26.8350459204202));
#15912=CARTESIAN_POINT('Ctrl Pts',(-0.856857337853241,6.71253189955676,
26.8432466759879));
#15913=CARTESIAN_POINT('Ctrl Pts',(-1.03029257513892,6.69039282328356,26.8514473898997));
#15914=CARTESIAN_POINT('Ctrl Pts',(-1.202873221224,6.6615272215178,26.8596481038115));
#15915=CARTESIAN_POINT('Ctrl Pts',(-1.37404545732681,6.62603109570123,26.8678488177232));
#15916=CARTESIAN_POINT('Ctrl Pts',(-1.5452478446275,6.59052871740623,26.8760509761528));
#15917=CARTESIAN_POINT('Ctrl Pts',(-1.71504097676692,6.54839356091663,26.8842531345824));
#15918=CARTESIAN_POINT('Ctrl Pts',(-1.88288248819614,6.49977249876058,26.892455293012));
#15919=CARTESIAN_POINT('Ctrl Pts',(-2.05078398151387,6.45113406078906,26.900660382665));
#15920=CARTESIAN_POINT('Ctrl Pts',(-2.21673212074827,6.39600519944694,26.9088654723179));
#15921=CARTESIAN_POINT('Ctrl Pts',(-2.38020087270768,6.33458229132447,26.9170705619708));
#15922=CARTESIAN_POINT('Ctrl Pts',(-2.54385636838946,6.27308921479145,26.9252850249686));
#15923=CARTESIAN_POINT('Ctrl Pts',(-2.70502648233334,6.20528785289478,26.9334994879664));
#15924=CARTESIAN_POINT('Ctrl Pts',(-2.86320532400266,6.13142269563948,26.9417139509642));
#15925=CARTESIAN_POINT('Ctrl Pts',(-3.02147788163616,6.05751377561312,26.9499332807716));
#15926=CARTESIAN_POINT('Ctrl Pts',(-3.17675531619248,5.97753406260601,26.9581526105791));
#15927=CARTESIAN_POINT('Ctrl Pts',(-3.32855754199713,5.89177339089124,26.9663719403866));
#15928=CARTESIAN_POINT('Ctrl Pts',(-3.48059497614724,5.80587983821513,26.9746040055473));
#15929=CARTESIAN_POINT('Ctrl Pts',(-3.62914613621989,5.71418761486332,26.982836070708));
#15930=CARTESIAN_POINT('Ctrl Pts',(-3.77375994572452,5.61702989773468,26.9910681358687));
#15931=CARTESIAN_POINT('Ctrl Pts',(-3.90374922154912,5.52969756527221,26.9984677071298));
#15932=CARTESIAN_POINT('Ctrl Pts',(-4.03055751378548,5.43794994954438,27.005867278391));
#15933=CARTESIAN_POINT('Ctrl Pts',(-4.15388145949066,5.34205558006464,27.0132668496522));
#15934=CARTESIAN_POINT('Ctrl Pts',(-4.28824747095195,5.23757510893708,27.0213289569031));
#15935=CARTESIAN_POINT('Ctrl Pts',(-4.41891022822859,5.12783417337497,27.0293910641541));
#15936=CARTESIAN_POINT('Ctrl Pts',(-4.5454190056654,5.01312827114326,27.037453171405));
#15937=CARTESIAN_POINT('Ctrl Pts',(-4.67177407218353,4.89856173907991,27.0455054830202));
#15938=CARTESIAN_POINT('Ctrl Pts',(-4.79398492773395,4.7790424921065,27.0535577946353));
#15939=CARTESIAN_POINT('Ctrl Pts',(-4.91163038948578,4.65490879793362,27.0616101062505));
#15940=CARTESIAN_POINT('Ctrl Pts',(-5.02915884175316,4.53089856640299,27.0696544090838));
#15941=CARTESIAN_POINT('Ctrl Pts',(-5.1421306812953,4.40228329063955,27.0776987119172));
#15942=CARTESIAN_POINT('Ctrl Pts',(-5.25015845764759,4.26944084975907,27.0857430147505));
#15943=CARTESIAN_POINT('Ctrl Pts',(-5.35810256470482,4.13670129754073,27.0937810871386));
#15944=CARTESIAN_POINT('Ctrl Pts',(-5.4611099955365,3.9997413858845,27.1018191595267));
#15945=CARTESIAN_POINT('Ctrl Pts',(-5.55883087639642,3.85897503070722,27.1098572319148));
#15946=CARTESIAN_POINT('Ctrl Pts',(-5.65650147768686,3.7182811029546,27.1178911685357));
#15947=CARTESIAN_POINT('Ctrl Pts',(-5.748890729455,3.57378493610329,27.1259251051565));
#15948=CARTESIAN_POINT('Ctrl Pts',(-5.83568975566038,3.42593258481256,27.1339590417774));
#15949=CARTESIAN_POINT('Ctrl Pts',(-5.92246553100392,3.27811983874258,27.141990826347));
#15950=CARTESIAN_POINT('Ctrl Pts',(-6.00365387041939,3.12695301925926,27.1500226109166));
#15951=CARTESIAN_POINT('Ctrl Pts',(-6.07898992023337,2.97290607818362,27.1580543954862));
#15952=CARTESIAN_POINT('Ctrl Pts',(-6.15432077633269,2.81886975720098,27.1660856263396));
#15953=CARTESIAN_POINT('Ctrl Pts',(-6.22379998117649,2.66195404604556,27.1741168571929));
#15954=CARTESIAN_POINT('Ctrl Pts',(-6.28720931491777,2.50265619500786,27.1821480880463));
#15955=CARTESIAN_POINT('Ctrl Pts',(-6.35062689211165,2.34333763464859,27.1901803629899));
#15956=CARTESIAN_POINT('Ctrl Pts',(-6.40797288983725,2.18163666614524,27.1982126379336));
#15957=CARTESIAN_POINT('Ctrl Pts',(-6.45907784002637,2.01806899200207,27.2062449128772));
#15958=CARTESIAN_POINT('Ctrl Pts',(-6.51022689465075,1.85436015619322,27.2142841198098));
#15959=CARTESIAN_POINT('Ctrl Pts',(-6.55512403028306,1.68878175439402,27.2223233267424));
#15960=CARTESIAN_POINT('Ctrl Pts',(-6.59364995435232,1.52186375194027,27.230362533675));
#15961=CARTESIAN_POINT('Ctrl Pts',(-6.6321922737588,1.35487471479997,27.2384051618236));
#15962=CARTESIAN_POINT('Ctrl Pts',(-6.66435790990869,1.18654530878259,27.2464477899723));
#15963=CARTESIAN_POINT('Ctrl Pts',(-6.69007911768547,1.01741358311594,27.2544904181209));
#15964=CARTESIAN_POINT('Ctrl Pts',(-6.71583589395875,0.848047974140052,
27.2625441679942));
#15965=CARTESIAN_POINT('Ctrl Pts',(-6.73513039384976,0.677878200650345,
27.2705979178675));
#15966=CARTESIAN_POINT('Ctrl Pts',(-6.74794688764199,0.507446353384106,
27.2786516677408));
#15967=CARTESIAN_POINT('Ctrl Pts',(-6.76066490161465,0.338324076257635,
27.2866435339315));
#15968=CARTESIAN_POINT('Ctrl Pts',(-6.76700418638193,0.16894409523193,27.2946354001221));
#15969=CARTESIAN_POINT('Ctrl Pts',(-6.76699999792448,-0.000167601012896156,
27.3026272663128));
#15970=CARTESIAN_POINT('Ctrl Pts',(-6.76699999814636,-0.000158389305696416,
27.3028276665937));
#15971=CARTESIAN_POINT('Ctrl Pts',(-6.76699564443585,-0.186165638445246,
27.311577178389));
#15972=CARTESIAN_POINT('Ctrl Pts',(-6.75931766370376,-0.37217256467103,
27.3203266901844));
#15973=CARTESIAN_POINT('Ctrl Pts',(-6.74399213454365,-0.557547387415058,
27.3290762019797));
#15974=CARTESIAN_POINT('Ctrl Pts',(-6.72866667011378,-0.742921427193918,
27.3378256768199));
#15975=CARTESIAN_POINT('Ctrl Pts',(-6.70569374550785,-0.927663083204684,
27.3465751516601));
#15976=CARTESIAN_POINT('Ctrl Pts',(-6.67515138859919,-1.11114487771953,
27.3553246265002));
#15977=CARTESIAN_POINT('Ctrl Pts',(-6.64460915815518,-1.29462591250379,
27.364074065112));
#15978=CARTESIAN_POINT('Ctrl Pts',(-6.60649760518768,-1.47684681352381,
27.3728235037238));
#15979=CARTESIAN_POINT('Ctrl Pts',(-6.56094617507105,-1.657188669953,27.3815729423356));
#15980=CARTESIAN_POINT('Ctrl Pts',(-6.51539492978294,-1.83752979463085,
27.3903223454459));
#15981=CARTESIAN_POINT('Ctrl Pts',(-6.46240393793969,-2.01599161211029,
27.3990717485562));
#15982=CARTESIAN_POINT('Ctrl Pts',(-6.4021531812695,-2.19196798415506,27.4078211516664));
#15983=CARTESIAN_POINT('Ctrl Pts',(-6.34190266406773,-2.36794365677655,
27.416570520002));
#15984=CARTESIAN_POINT('Ctrl Pts',(-6.27439253261081,-2.54143363259705,
27.4253198883375));
#15985=CARTESIAN_POINT('Ctrl Pts',(-6.19985208046774,-2.71184866471561,
27.434069256673));
#15986=CARTESIAN_POINT('Ctrl Pts',(-6.12531191839751,-2.88226303366712,
27.4428185909605));
#15987=CARTESIAN_POINT('Ctrl Pts',(-6.04374160523462,-3.04960222030065,
27.451567925248));
#15988=CARTESIAN_POINT('Ctrl Pts',(-5.95541818684473,-3.21329787287127,
27.4603172595355));
#15989=CARTESIAN_POINT('Ctrl Pts',(-5.86709510482902,-3.3769929020173,27.4690665605017));
#15990=CARTESIAN_POINT('Ctrl Pts',(-5.77201910513236,-3.53704417266323,
27.4778158614679));
#15991=CARTESIAN_POINT('Ctrl Pts',(-5.67051310195223,-3.69290808991886,
27.4865651624341));
#15992=CARTESIAN_POINT('Ctrl Pts',(-5.56900747692194,-3.84877142652,27.4953144308057));
#15993=CARTESIAN_POINT('Ctrl Pts',(-5.46107205273131,-4.00044720081222,
27.5040636991773));
#15994=CARTESIAN_POINT('Ctrl Pts',(-5.34707341633779,-4.14742026810568,
27.5128129675489));
#15995=CARTESIAN_POINT('Ctrl Pts',(-5.23307519516778,-4.29439280007104,
27.5215622040526));
#15996=CARTESIAN_POINT('Ctrl Pts',(-5.11301398162055,-4.43666243288071,
27.5303114405563));
#15997=CARTESIAN_POINT('Ctrl Pts',(-4.98729754316467,-4.57374597195161,
27.5390606770599));
#15998=CARTESIAN_POINT('Ctrl Pts',(-4.8615815521733,-4.71082902309892,27.5478098824223));
#15999=CARTESIAN_POINT('Ctrl Pts',(-4.73021057023571,-4.84272580625139,
27.5565590877847));
#16000=CARTESIAN_POINT('Ctrl Pts',(-4.59363077335013,-4.96898835962922,
27.5653082931471));
#16001=CARTESIAN_POINT('Ctrl Pts',(-4.45705145125412,-5.0952504740831,27.5740574680948));
#16002=CARTESIAN_POINT('Ctrl Pts',(-4.31526356086088,-5.21587820343581,
27.5828066430424));
#16003=CARTESIAN_POINT('Ctrl Pts',(-4.16874865382824,-5.33046186190327,
27.5915558179901));
#16004=CARTESIAN_POINT('Ctrl Pts',(-4.02223424395669,-5.4450451315602,27.6003049632497));
#16005=CARTESIAN_POINT('Ctrl Pts',(-3.87099307526245,-5.55358419484709,
27.6090541085093));
#16006=CARTESIAN_POINT('Ctrl Pts',(-3.71553880191979,-5.65571042499777,
27.6178032537689));
#16007=CARTESIAN_POINT('Ctrl Pts',(-3.56008504316433,-5.75783631708858,
27.6265523700669));
#16008=CARTESIAN_POINT('Ctrl Pts',(-3.4004184471562,-5.85354926119071,27.635301486365));
#16009=CARTESIAN_POINT('Ctrl Pts',(-3.23708127941626,-5.94252419351009,
27.644050602663));
#16010=CARTESIAN_POINT('Ctrl Pts',(-3.07374463879529,-6.03149883869107,
27.652799690726));
#16011=CARTESIAN_POINT('Ctrl Pts',(-2.90673770177539,-6.11373537853349,
27.6615487787891));
#16012=CARTESIAN_POINT('Ctrl Pts',(-2.73662765975433,-6.18895452010011,
27.6702978668521));
#16013=CARTESIAN_POINT('Ctrl Pts',(-2.56651815258613,-6.26417342516586,
27.6790469274066));
#16014=CARTESIAN_POINT('Ctrl Pts',(-2.39330582200001,-6.33237486023128,
27.6877959879611));
#16015=CARTESIAN_POINT('Ctrl Pts',(-2.21757893054653,-6.39332720004194,
27.6965450485156));
#16016=CARTESIAN_POINT('Ctrl Pts',(-2.04185257701619,-6.45427935326946,
27.7052940822881));
#16017=CARTESIAN_POINT('Ctrl Pts',(-1.86361194873049,-6.50798236175061,
27.7140431160606));
#16018=CARTESIAN_POINT('Ctrl Pts',(-1.68346238160849,-6.55425384080515,
27.7227921498331));
#16019=CARTESIAN_POINT('Ctrl Pts',(-1.50331335099113,-6.60052518205829,
27.73154115755));
#16020=CARTESIAN_POINT('Ctrl Pts',(-1.32125567043228,-6.63936496689287,
27.740290165267));
#16021=CARTESIAN_POINT('Ctrl Pts',(-1.13790763553999,-6.67064128948483,
27.7490391729839));
#16022=CARTESIAN_POINT('Ctrl Pts',(-0.954560131456165,-6.70191752152912,
27.7577881553717));
#16023=CARTESIAN_POINT('Ctrl Pts',(-0.769922562956765,-6.725630286969,27.7665371377595));
#16024=CARTESIAN_POINT('Ctrl Pts',(-0.584621983715095,-6.74169905410773,
27.7752861201473));
#16025=CARTESIAN_POINT('Ctrl Pts',(-0.39133411198032,-6.75846045773829,
27.7844122232199));
#16026=CARTESIAN_POINT('Ctrl Pts',(-0.197325135735471,-6.76690423582442,
27.7935383262926));
#16027=CARTESIAN_POINT('Ctrl Pts',(-0.00331189650882545,-6.76699918954787,
27.8026644293652));
#16028=CARTESIAN_POINT('Ctrl Pts',(0.18463842899198,-6.76709117596747,27.8115053417169));
#16029=CARTESIAN_POINT('Ctrl Pts',(0.372592438084156,-6.75934828281543,
27.8203462540685));
#16030=CARTESIAN_POINT('Ctrl Pts',(0.559898343344746,-6.74379736091765,
27.8291871664201));
#16031=CARTESIAN_POINT('Ctrl Pts',(0.74527770155342,-6.7284063890369,27.8379371449937));
#16032=CARTESIAN_POINT('Ctrl Pts',(0.930021936897552,-6.70536729682682,
27.8466871235672));
#16033=CARTESIAN_POINT('Ctrl Pts',(1.11350349070759,-6.67475834590152,27.8554371021407));
#16034=CARTESIAN_POINT('Ctrl Pts',(1.29698316624787,-6.6441497083149,27.8641869911422));
#16035=CARTESIAN_POINT('Ctrl Pts',(1.47919990335411,-6.60597141425457,27.8729368801437));
#16036=CARTESIAN_POINT('Ctrl Pts',(1.65953474168855,-6.56035314911695,27.8816867691451));
#16037=CARTESIAN_POINT('Ctrl Pts',(1.83986779389779,-6.51473533580514,27.8904365714834));
#16038=CARTESIAN_POINT('Ctrl Pts',(2.01831870672899,-6.46167776917716,27.8991863738216));
#16039=CARTESIAN_POINT('Ctrl Pts',(2.19428132372643,-6.40136067350883,27.9079361761599));
#16040=CARTESIAN_POINT('Ctrl Pts',(2.37024225637796,-6.34104415520662,27.9166858947434));
#16041=CARTESIAN_POINT('Ctrl Pts',(2.54371466970189,-6.27346833986935,27.925435613327));
#16042=CARTESIAN_POINT('Ctrl Pts',(2.71410932932242,-6.19886276251419,27.9341853319106));
#16043=CARTESIAN_POINT('Ctrl Pts',(2.88450241451495,-6.12425787450639,27.9429349696477));
#16044=CARTESIAN_POINT('Ctrl Pts',(3.05181754034475,-6.04262346942454,27.9516846073848));
#16045=CARTESIAN_POINT('Ctrl Pts',(3.21548639740849,-5.9542368300296,27.9604342451219));
#16046=CARTESIAN_POINT('Ctrl Pts',(3.37915379657157,-5.86585097794964,27.9691838049206));
#16047=CARTESIAN_POINT('Ctrl Pts',(3.53917473976983,-5.77071314811019,27.9779333647192));
#16048=CARTESIAN_POINT('Ctrl Pts',(3.69500570299244,-5.6691464838063,27.9866829245179));
#16049=CARTESIAN_POINT('Ctrl Pts',(3.85083532990542,-5.56758069047509,27.9954324092857));
#16050=CARTESIAN_POINT('Ctrl Pts',(4.00247480863557,-5.45958632949755,28.0041818940535));
#16051=CARTESIAN_POINT('Ctrl Pts',(4.14940909231515,-5.34553020612664,28.0129313788214));
#16052=CARTESIAN_POINT('Ctrl Pts',(4.29634216479246,-5.2314750229382,28.0216807914658));
#16053=CARTESIAN_POINT('Ctrl Pts',(4.43856989344099,-5.11135835308375,28.0304302041103));
#16054=CARTESIAN_POINT('Ctrl Pts',(4.57560920656789,-4.98558816878923,28.0391796167548));
#16055=CARTESIAN_POINT('Ctrl Pts',(4.71264743558326,-4.8598189794567,28.0479289601831));
#16056=CARTESIAN_POINT('Ctrl Pts',(4.8444971200733,-4.72839655896145,28.0566783036114));
#16057=CARTESIAN_POINT('Ctrl Pts',(4.97071044410098,-4.59176727207569,28.0654276470396));
#16058=CARTESIAN_POINT('Ctrl Pts',(5.09692281158692,-4.45513902067185,28.0741769241587));
#16059=CARTESIAN_POINT('Ctrl Pts',(5.21749870963727,-4.31330419234739,28.0829262012777));
#16060=CARTESIAN_POINT('Ctrl Pts',(5.33202861894698,-4.16674450941384,28.0916754783967));
#16061=CARTESIAN_POINT('Ctrl Pts',(5.44655769830365,-4.02018588854046,28.1004246921132));
#16062=CARTESIAN_POINT('Ctrl Pts',(5.5550407001457,-3.86890270737006,28.1091739058296));
#16063=CARTESIAN_POINT('Ctrl Pts',(5.65710918234642,-3.71340877079427,28.1179231195461));
#16064=CARTESIAN_POINT('Ctrl Pts',(5.75917695879893,-3.55791590937474,28.1266722727665));
#16065=CARTESIAN_POINT('Ctrl Pts',(5.85483014711972,-3.39821259036579,28.1354214259869));
#16066=CARTESIAN_POINT('Ctrl Pts',(5.94374388372034,-3.2348412085815,28.1441705792073));
#16067=CARTESIAN_POINT('Ctrl Pts',(6.03265703506149,-3.07147090216142,28.1529196748378));
#16068=CARTESIAN_POINT('Ctrl Pts',(6.1148306864786,-2.90443283296427,28.1616687704684));
#16069=CARTESIAN_POINT('Ctrl Pts',(6.18998575813472,-2.73429429909975,28.170417866099));
#16070=CARTESIAN_POINT('Ctrl Pts',(6.26514036005544,-2.56415682863772,28.1791669070459));
#16071=CARTESIAN_POINT('Ctrl Pts',(6.33327635422231,-2.39091919438814,28.1879159479927));
#16072=CARTESIAN_POINT('Ctrl Pts',(6.39416233866698,-2.21516974220327,28.1966649889396));
#16073=CARTESIAN_POINT('Ctrl Pts',(6.45504796278121,-2.03942133012435,28.2054139781086));
#16074=CARTESIAN_POINT('Ctrl Pts',(6.50868356924084,-1.86116140059545,28.2141629672776));
#16075=CARTESIAN_POINT('Ctrl Pts',(6.55488700412989,-1.68099534891952,28.2229119564466));
#16076=CARTESIAN_POINT('Ctrl Pts',(6.60202876080853,-1.49717039758741,28.2318386243357));
#16077=CARTESIAN_POINT('Ctrl Pts',(6.64143315241961,-1.31136136892039,28.2407652922247));
#16078=CARTESIAN_POINT('Ctrl Pts',(6.67296087137084,-1.12422515945592,28.2496919601138));
#16079=CARTESIAN_POINT('Ctrl Pts',(6.7038643211654,-0.940794367558994,28.2584418742249));
#16080=CARTESIAN_POINT('Ctrl Pts',(6.72720006210098,-0.756088753450049,
28.267191788336));
#16081=CARTESIAN_POINT('Ctrl Pts',(6.74288882604265,-0.570735735370709,
28.2759417024471));
#16082=CARTESIAN_POINT('Ctrl Pts',(6.75857728146194,-0.385386362292,28.2846914444896));
#16083=CARTESIAN_POINT('Ctrl Pts',(6.76661903663616,-0.199389896352124,
28.2934411865321));
#16084=CARTESIAN_POINT('Ctrl Pts',(6.76698677596,-0.0133781158060973,28.3021909285745));
#16085=CARTESIAN_POINT('Ctrl Pts',(6.76735450854098,0.172630254029962,28.3109405101818));
#16086=CARTESIAN_POINT('Ctrl Pts',(6.76004850628286,0.358653651283843,28.3196900917891));
#16087=CARTESIAN_POINT('Ctrl Pts',(6.74509358473383,0.544060229370441,28.3284396733964));
#16088=CARTESIAN_POINT('Ctrl Pts',(6.73013891752283,0.729463654251187,28.3371891061998));
#16089=CARTESIAN_POINT('Ctrl Pts',(6.70753561437841,0.914249995282579,28.3459385390031));
#16090=CARTESIAN_POINT('Ctrl Pts',(6.67736044701224,1.09779162898819,28.3546879718065));
#16091=CARTESIAN_POINT('Ctrl Pts',(6.64718575273648,1.2813303851029,28.363437267435));
#16092=CARTESIAN_POINT('Ctrl Pts',(6.60943947828775,1.46362419016019,28.3721865630635));
#16093=CARTESIAN_POINT('Ctrl Pts',(6.56424982419094,1.64405390593169,28.380935858692));
#16094=CARTESIAN_POINT('Ctrl Pts',(6.5190608185409,1.82448103263563,28.389685028773));
#16095=CARTESIAN_POINT('Ctrl Pts',(6.46642871659859,2.00304384560883,28.3984341988539));
#16096=CARTESIAN_POINT('Ctrl Pts',(6.406532271625,2.17913589586042,28.4071833689349));
#16097=CARTESIAN_POINT('Ctrl Pts',(6.34663660655764,2.35522565323327,28.4159324250936));
#16098=CARTESIAN_POINT('Ctrl Pts',(6.27947688001376,2.52884444098845,28.4246814812524));
#16099=CARTESIAN_POINT('Ctrl Pts',(6.20528117917537,2.69940261676022,28.4334305374112));
#16100=CARTESIAN_POINT('Ctrl Pts',(6.12826427824231,2.8764460569907,28.4425122656491));
#16101=CARTESIAN_POINT('Ctrl Pts',(6.04366596008219,3.05019126379016,28.4515939938871));
#16102=CARTESIAN_POINT('Ctrl Pts',(5.95179577696798,3.22000248901552,28.4606757221251));
#16103=CARTESIAN_POINT('Ctrl Pts',(5.86328355867829,3.3836069113176,28.4694255023584));
#16104=CARTESIAN_POINT('Ctrl Pts',(5.76802179058685,3.54355957239308,28.4781752825917));
#16105=CARTESIAN_POINT('Ctrl Pts',(5.66633405324216,3.69931715280918,28.4869250628251));
#16106=CARTESIAN_POINT('Ctrl Pts',(5.56464997144232,3.85506913393835,28.4956745285149));
#16107=CARTESIAN_POINT('Ctrl Pts',(5.45654053933722,4.00662609619198,28.5044239942048));
#16108=CARTESIAN_POINT('Ctrl Pts',(5.34237295142181,4.15347327521397,28.5131734598946));
#16109=CARTESIAN_POINT('Ctrl Pts',(5.22820886081963,4.30031595584379,28.5219226575608));
#16110=CARTESIAN_POINT('Ctrl Pts',(5.10798716166375,4.44244891571258,28.5306718552269));
#16111=CARTESIAN_POINT('Ctrl Pts',(4.9821161628635,4.57938942870491,28.539421052893));
#16112=CARTESIAN_POINT('Ctrl Pts',(4.85624835096625,4.71632647452739,28.54817002904));
#16113=CARTESIAN_POINT('Ctrl Pts',(4.724731719552,4.84807112559724,28.5569190051869));
#16114=CARTESIAN_POINT('Ctrl Pts',(4.58801291590907,4.97417596024221,28.5656679813338));
#16115=CARTESIAN_POINT('Ctrl Pts',(4.45128522596351,5.10028899131442,28.5744175261373));
#16116=CARTESIAN_POINT('Ctrl Pts',(4.30935489779267,5.22076127807759,28.5831670709409));
#16117=CARTESIAN_POINT('Ctrl Pts',(4.16270400752698,5.33518362811617,28.5919166157444));
#16118=CARTESIAN_POINT('Ctrl Pts',(4.01606173721642,5.44959925255274,28.6006656462606));
#16119=CARTESIAN_POINT('Ctrl Pts',(3.86469968596859,5.55796547558829,28.6094146767769));
#16120=CARTESIAN_POINT('Ctrl Pts',(3.70913190503631,5.65991426711057,28.6181637072932));
#16121=CARTESIAN_POINT('Ctrl Pts',(3.55356201479594,5.76186444093327,28.6269128564356));
#16122=CARTESIAN_POINT('Ctrl Pts',(3.39378652042069,5.85739685205832,28.6356620055779));
#16123=CARTESIAN_POINT('Ctrl Pts',(3.23034806134602,5.94618704739079,28.6444111547203));
#16124=CARTESIAN_POINT('Ctrl Pts',(3.18687941281391,5.96980198977251,28.6467381081876));
#16125=CARTESIAN_POINT('Ctrl Pts',(3.14315180418704,5.99294025706453,28.6490650616548));
#16126=CARTESIAN_POINT('Ctrl Pts',(3.09917575053261,6.01559628526638,28.6513920151221));
#16127=CARTESIAN_POINT('Origin',(0.,0.,-3.69717978381041));
#16128=CARTESIAN_POINT('',(3.09917575053259,6.01559628526639,31.0457515827422));
#16129=CARTESIAN_POINT('',(3.09917575053255,6.01559628526641,30.6514573492524));
#16130=CARTESIAN_POINT('',(3.09917575053259,6.01559628526639,-3.69717978381041));
#16131=CARTESIAN_POINT('',(-6.767,1.20905997887111E-12,29.69717978381));
#16132=CARTESIAN_POINT('Ctrl Pts',(-6.767,1.20906028438136E-12,29.69717978381));
#16133=CARTESIAN_POINT('Ctrl Pts',(-6.76700000000003,-0.18600724941446,
29.705929295616));
#16134=CARTESIAN_POINT('Ctrl Pts',(-6.75932637295445,-0.372014355526306,
29.7146788074219));
#16135=CARTESIAN_POINT('Ctrl Pts',(-6.74400518266938,-0.557389537153815,
29.7234283192279));
#16136=CARTESIAN_POINT('Ctrl Pts',(-6.72868405709658,-0.742763935810295,
29.7321777940784));
#16137=CARTESIAN_POINT('Ctrl Pts',(-6.70571545653005,-0.927506129694064,
29.7409272689289));
#16138=CARTESIAN_POINT('Ctrl Pts',(-6.67517739415664,-1.11098863924892,
29.7496767437795));
#16139=CARTESIAN_POINT('Ctrl Pts',(-6.64463945823084,-1.29447038906586,
29.7584261824015));
#16140=CARTESIAN_POINT('Ctrl Pts',(-6.60653217027138,-1.47669218228305,
29.7671756210235));
#16141=CARTESIAN_POINT('Ctrl Pts',(-6.56098496116689,-1.65703510504212,
29.7759250596455));
#16142=CARTESIAN_POINT('Ctrl Pts',(-6.51543793687488,-1.83737729604125,
29.7846744627657));
#16143=CARTESIAN_POINT('Ctrl Pts',(-6.46245112202603,-2.0158403539717,29.7934238658859));
#16144=CARTESIAN_POINT('Ctrl Pts',(-6.40220448416198,-2.19181813638273,
29.8021732690062));
#16145=CARTESIAN_POINT('Ctrl Pts',(-6.34195808575137,-2.36779521936079,
29.8109226373514));
#16146=CARTESIAN_POINT('Ctrl Pts',(-6.27445201489178,-2.54128677544968,
29.8196720056967));
#16147=CARTESIAN_POINT('Ctrl Pts',(-6.1999155513612,-2.71170355237987,29.828421374042));
#16148=CARTESIAN_POINT('Ctrl Pts',(-6.12537937788967,-2.88211966613225,
29.8371707083391));
#16149=CARTESIAN_POINT('Ctrl Pts',(-6.04381298133537,-3.04946076210603,
29.8459200426361));
#16150=CARTESIAN_POINT('Ctrl Pts',(-5.95549339426218,-3.21315848207019,
29.8546693769332));
#16151=CARTESIAN_POINT('Ctrl Pts',(-5.86717414355064,-3.37685557859804,
29.8634186779087));
#16152=CARTESIAN_POINT('Ctrl Pts',(-5.77210188986133,-3.53690907467483,
29.8721679788843));
#16153=CARTESIAN_POINT('Ctrl Pts',(-5.67059953466954,-3.6927753678508,29.8809172798599));
#16154=CARTESIAN_POINT('Ctrl Pts',(-5.56909755761641,-3.84864108035974,
29.8896665482406));
#16155=CARTESIAN_POINT('Ctrl Pts',(-5.46116568337934,-4.00031938104466,
29.8984158166214));
#16156=CARTESIAN_POINT('Ctrl Pts',(-5.34717048685966,-4.1472951166341,29.9071650850022));
#16157=CARTESIAN_POINT('Ctrl Pts',(-5.23317570555366,-4.29427031688225,
29.9159143215148));
#16158=CARTESIAN_POINT('Ctrl Pts',(-5.1131178217865,-4.43654275987308,29.9246635580274));
#16159=CARTESIAN_POINT('Ctrl Pts',(-4.98740459171857,-4.57362924147821,
29.93341279454));
#16160=CARTESIAN_POINT('Ctrl Pts',(-4.86169180910672,-4.71071523514599,
29.9421619999111));
#16161=CARTESIAN_POINT('Ctrl Pts',(-4.73032391415273,-4.84261509316678,
29.9509112052823));
#16162=CARTESIAN_POINT('Ctrl Pts',(-4.59374707237136,-4.96888084331669,
29.9596604106534));
#16163=CARTESIAN_POINT('Ctrl Pts',(-4.4571707053724,-5.09514615452866,29.9684095856096));
#16164=CARTESIAN_POINT('Ctrl Pts',(-4.31538563819343,-5.2157772025377,29.9771587605658));
#16165=CARTESIAN_POINT('Ctrl Pts',(-4.16887341290477,-5.33036429028784,
29.9859079355221));
#16166=CARTESIAN_POINT('Ctrl Pts',(-4.02236168477174,-5.44495098921298,
29.99465708079));
#16167=CARTESIAN_POINT('Ctrl Pts',(-3.87112305634281,-5.55349359238869,
30.0034062260579));
#16168=CARTESIAN_POINT('Ctrl Pts',(-3.71567117316582,-5.65562346102572,
30.0121553713258));
#16169=CARTESIAN_POINT('Ctrl Pts',(-3.5602198045717,-5.75775299158849,30.0209044876319));
#16170=CARTESIAN_POINT('Ctrl Pts',(-3.40055544862277,-5.85346967275417,
30.0296536039381));
#16171=CARTESIAN_POINT('Ctrl Pts',(-3.23722036323314,-5.9424484280361,30.0384027202442));
#16172=CARTESIAN_POINT('Ctrl Pts',(-3.07388580495985,-6.03142689616506,
30.0471518083152));
#16173=CARTESIAN_POINT('Ctrl Pts',(-2.90688079257675,-6.11366734484837,
30.0559008963861));
#16174=CARTESIAN_POINT('Ctrl Pts',(-2.73677251094613,-6.18889046787303,
30.064649984457));
#16175=CARTESIAN_POINT('Ctrl Pts',(-2.56666476416645,-6.2641133543827,30.0733990450193));
#16176=CARTESIAN_POINT('Ctrl Pts',(-2.39345402972095,-6.3323188435029,30.0821481055815));
#16177=CARTESIAN_POINT('Ctrl Pts',(-2.21772856474042,-6.39327529621042,
30.0908971661437));
#16178=CARTESIAN_POINT('Ctrl Pts',(-2.04200363768294,-6.45423156232073,
30.0996461999237));
#16179=CARTESIAN_POINT('Ctrl Pts',(-1.86376426620139,-6.50793874252042,
30.1083952337037));
#16180=CARTESIAN_POINT('Ctrl Pts',(-1.68361578194756,-6.55421443796105,
30.1171442674837));
#16181=CARTESIAN_POINT('Ctrl Pts',(-1.50346783419914,-6.6004899955867,30.1258932752079));
#16182=CARTESIAN_POINT('Ctrl Pts',(-1.32141106257271,-6.63933404145491,
30.1346422829322));
#16183=CARTESIAN_POINT('Ctrl Pts',(-1.13806375959047,-6.67061465527029,
30.1433912906564));
#16184=CARTESIAN_POINT('Ctrl Pts',(-0.954716987419053,-6.70189517852482,
30.1521402730513));
#16185=CARTESIAN_POINT('Ctrl Pts',(-0.770079973809654,-6.72561226535831,
30.1608892554462));
#16186=CARTESIAN_POINT('Ctrl Pts',(-0.584779770552109,-6.74168536939785,
30.1696382378411));
#16187=CARTESIAN_POINT('Ctrl Pts',(-0.391490647553584,-6.75845143942396,
30.1787644185171));
#16188=CARTESIAN_POINT('Ctrl Pts',(-0.197480213104026,-6.76689975924027,
30.1878905991932));
#16189=CARTESIAN_POINT('Ctrl Pts',(-0.00346532629750826,-6.76699911271707,
30.1970167798692));
#16190=CARTESIAN_POINT('Ctrl Pts',(0.184486595296305,-6.76709536139773,
30.2058577673992));
#16191=CARTESIAN_POINT('Ctrl Pts',(0.372442378185438,-6.75935659726769,
30.2146987549291));
#16192=CARTESIAN_POINT('Ctrl Pts',(0.559750217722256,-6.74380965729015,
30.223539742459));
#16193=CARTESIAN_POINT('Ctrl Pts',(0.745129914457859,-6.72842275717252,
30.2322897210568));
#16194=CARTESIAN_POINT('Ctrl Pts',(0.929874656314225,-6.70538772273472,
30.2410396996545));
#16195=CARTESIAN_POINT('Ctrl Pts',(1.11335688289775,-6.67478280180743,30.2497896782523));
#16196=CARTESIAN_POINT('Ctrl Pts',(1.29683723118851,-6.64417819418024,30.2585395672773));
#16197=CARTESIAN_POINT('Ctrl Pts',(1.47905480730225,-6.60600390230077,30.2672894563022));
#16198=CARTESIAN_POINT('Ctrl Pts',(1.65939064804795,-6.56038959797138,30.2760393453271));
#16199=CARTESIAN_POINT('Ctrl Pts',(1.83972470264242,-6.51477574543262,30.2847891476881));
#16200=CARTESIAN_POINT('Ctrl Pts',(2.01817678125815,-6.4617220982011,30.293538950049));
#16201=CARTESIAN_POINT('Ctrl Pts',(2.19414072347636,-6.40140886724029,30.30228875241));
#16202=CARTESIAN_POINT('Ctrl Pts',(2.37010298132055,-6.3410962136139,30.3110384710154));
#16203=CARTESIAN_POINT('Ctrl Pts',(2.54357687926873,-6.27352420825987,30.3197881896209));
#16204=CARTESIAN_POINT('Ctrl Pts',(2.71397317789932,-6.19892237325513,30.3285379082264));
#16205=CARTESIAN_POINT('Ctrl Pts',(2.88436790207167,-6.12432122756979,30.3372875459847));
#16206=CARTESIAN_POINT('Ctrl Pts',(3.05168482126228,-6.04269049717432,30.346037183743));
#16207=CARTESIAN_POINT('Ctrl Pts',(3.21535561997365,-5.95430745234942,30.3547868215012));
#16208=CARTESIAN_POINT('Ctrl Pts',(3.37902496075248,-5.86592519481535,30.3635363813202));
#16209=CARTESIAN_POINT('Ctrl Pts',(3.53904799384833,-5.77079087940257,30.3722859411392));
#16210=CARTESIAN_POINT('Ctrl Pts',(3.69488118814934,-5.66922763747057,30.3810355009583));
#16211=CARTESIAN_POINT('Ctrl Pts',(3.85071304610783,-5.56766526649086,30.3897849857457));
#16212=CARTESIAN_POINT('Ctrl Pts',(4.00235489705919,-5.4596742358075,30.3985344705331));
#16213=CARTESIAN_POINT('Ctrl Pts',(4.14929168607605,-5.34562133936366,30.4072839553206));
#16214=CARTESIAN_POINT('Ctrl Pts',(4.29622726385707,-5.23156938308572,30.4160333679839));
#16215=CARTESIAN_POINT('Ctrl Pts',(4.43845763092016,-5.11145583677246,30.4247827806472));
#16216=CARTESIAN_POINT('Ctrl Pts',(4.5754997066091,-4.98568866204259,30.4335321933105));
#16217=CARTESIAN_POINT('Ctrl Pts',(4.7125406981524,-4.85992248226215,30.4422815367568));
#16218=CARTESIAN_POINT('Ctrl Pts',(4.84439326931256,-4.72850295734061,30.4510308802031));
#16219=CARTESIAN_POINT('Ctrl Pts',(4.97060959434638,-4.59187644221747,30.4597802236494));
#16220=CARTESIAN_POINT('Ctrl Pts',(5.09682496280455,-4.45525096256732,30.4685295007857));
#16221=CARTESIAN_POINT('Ctrl Pts',(5.21740397615779,-4.31341878218398,30.477278777922));
#16222=CARTESIAN_POINT('Ctrl Pts',(5.33193710451875,-4.16686161438753,30.4860280550583));
#16223=CARTESIAN_POINT('Ctrl Pts',(5.44646940289336,-4.02030550864578,30.4947772687913));
#16224=CARTESIAN_POINT('Ctrl Pts',(5.55495572749629,-3.86902470980185,30.5035264825242));
#16225=CARTESIAN_POINT('Ctrl Pts',(5.65702762491431,-3.7135330146582,30.5122756962572));
#16226=CARTESIAN_POINT('Ctrl Pts',(5.7590988165514,-3.55804239466916,30.5210248494933));
#16227=CARTESIAN_POINT('Ctrl Pts',(5.85475551250779,-3.3983411761956,30.5297740027295));
#16228=CARTESIAN_POINT('Ctrl Pts',(5.943672837281,-3.2349717469196,30.5385231559656));
#16229=CARTESIAN_POINT('Ctrl Pts',(6.03258957676317,-3.07160339300955,30.5472722516111));
#16230=CARTESIAN_POINT('Ctrl Pts',(6.1147668968529,-2.90456712829493,30.5560213472567));
#16231=CARTESIAN_POINT('Ctrl Pts',(6.18992570525266,-2.73443024475892,30.5647704429022));
#16232=CARTESIAN_POINT('Ctrl Pts',(6.265084043887,-2.56429442463023,30.5735194838632));
#16233=CARTESIAN_POINT('Ctrl Pts',(6.33322384283315,-2.39105828655991,30.5822685248242));
#16234=CARTESIAN_POINT('Ctrl Pts',(6.39411368720031,-2.21531017132086,30.5910175657853));
#16235=CARTESIAN_POINT('Ctrl Pts',(6.45500317120888,-2.0395630961952,30.5997665549677));
#16236=CARTESIAN_POINT('Ctrl Pts',(6.50864269270072,-1.86130434438638,30.6085155441501));
#16237=CARTESIAN_POINT('Ctrl Pts',(6.55485008446332,-1.6811393071995,30.6172645333325));
#16238=CARTESIAN_POINT('Ctrl Pts',(6.60199664749403,-1.49731239211843,30.6261913468619));
#16239=CARTESIAN_POINT('Ctrl Pts',(6.64140563640906,-1.31150116499672,30.6351181603912));
#16240=CARTESIAN_POINT('Ctrl Pts',(6.67293772282172,-1.12436255155659,30.6440449739206));
#16241=CARTESIAN_POINT('Ctrl Pts',(6.70384494949871,-0.940932395051362,
30.6527948880761));
#16242=CARTESIAN_POINT('Ctrl Pts',(6.7271844934893,-0.75622726050676,30.6615448022316));
#16243=CARTESIAN_POINT('Ctrl Pts',(6.74287707373931,-0.570874564541765,
30.6702947163872));
#16244=CARTESIAN_POINT('Ctrl Pts',(6.7585693453867,-0.385525513632534,30.6790444584711));
#16245=CARTESIAN_POINT('Ctrl Pts',(6.76661493004103,-0.199529212418273,
30.6877942005551));
#16246=CARTESIAN_POINT('Ctrl Pts',(6.76698649908907,-0.0135174386004552,
30.6965439426391));
#16247=CARTESIAN_POINT('Ctrl Pts',(6.76735806132389,0.172490924445765,30.705293524285));
#16248=CARTESIAN_POINT('Ctrl Pts',(6.76005588896289,0.358514472901408,30.7140431059309));
#16249=CARTESIAN_POINT('Ctrl Pts',(6.74510478454584,0.543921359662228,30.7227926875768));
#16250=CARTESIAN_POINT('Ctrl Pts',(6.73015393440687,0.729325093150549,30.7315421204158));
#16251=CARTESIAN_POINT('Ctrl Pts',(6.70755443556895,0.914111900256543,30.7402915532549));
#16252=CARTESIAN_POINT('Ctrl Pts',(6.67738304682314,1.09765415591566,30.7490409860939));
#16253=CARTESIAN_POINT('Ctrl Pts',(6.64721213111855,1.28119353391299,30.7577902817553));
#16254=CARTESIAN_POINT('Ctrl Pts',(6.60946960955489,1.46348811672678,30.7665395774166));
#16255=CARTESIAN_POINT('Ctrl Pts',(6.56428366991177,1.64391876348245,30.7752888730779));
#16256=CARTESIAN_POINT('Ctrl Pts',(6.51909837867709,1.82434682109748,30.7840380431887));
#16257=CARTESIAN_POINT('Ctrl Pts',(6.46646995271908,2.00291071820487,30.7927872132996));
#16258=CARTESIAN_POINT('Ctrl Pts',(6.40657713281532,2.17900400212755,30.8015363834104));
#16259=CARTESIAN_POINT('Ctrl Pts',(6.3466850927904,2.35509499309711,30.8102854395962));
#16260=CARTESIAN_POINT('Ctrl Pts',(6.27952894037504,2.52871516398177,30.819034495782));
#16261=CARTESIAN_POINT('Ctrl Pts',(6.20533675061422,2.69927486771476,30.8277835519677));
#16262=CARTESIAN_POINT('Ctrl Pts',(6.12832117907893,2.87632521635974,30.83686555325));
#16263=CARTESIAN_POINT('Ctrl Pts',(6.04372366626056,3.05007728920043,30.8459475545323));
#16264=CARTESIAN_POINT('Ctrl Pts',(5.95185378007846,3.21989527478236,30.8550295558145));
#16265=CARTESIAN_POINT('Ctrl Pts',(5.86334450817347,3.38350129286793,30.8637793361217));
#16266=CARTESIAN_POINT('Ctrl Pts',(5.7680856205723,3.54345567125004,30.8725291164288));
#16267=CARTESIAN_POINT('Ctrl Pts',(5.66640068804456,3.69921508465352,30.8812788967359));
#16268=CARTESIAN_POINT('Ctrl Pts',(5.56471941107894,3.85496889852325,30.8900283624894));
#16269=CARTESIAN_POINT('Ctrl Pts',(5.45661270815084,4.00652780919678,30.8987778282429));
#16270=CARTESIAN_POINT('Ctrl Pts',(5.34244776449083,4.15337704569269,30.9075272939964));
#16271=CARTESIAN_POINT('Ctrl Pts',(5.22828631819568,4.30022178356283,30.916276491716));
#16272=CARTESIAN_POINT('Ctrl Pts',(5.10806717844046,4.44235690972705,30.9250256894356));
#16273=CARTESIAN_POINT('Ctrl Pts',(4.98219864544701,4.57929969070665,30.9337748871551));
#16274=CARTESIAN_POINT('Ctrl Pts',(4.85633329944005,4.71623900430022,30.9425238633454));
#16275=CARTESIAN_POINT('Ctrl Pts',(4.72481904033626,4.84798602483638,30.9512728395356));
#16276=CARTESIAN_POINT('Ctrl Pts',(4.58810250737175,4.97409332259147,30.9600218157259));
#16277=CARTESIAN_POINT('Ctrl Pts',(4.45137708685615,5.10020881822159,30.968771360662));
#16278=CARTESIAN_POINT('Ctrl Pts',(4.3094489263602,5.22068366307959,30.9775209055982));
#16279=CARTESIAN_POINT('Ctrl Pts',(4.16280009466626,5.33510865604878,30.9862704505344));
#16280=CARTESIAN_POINT('Ctrl Pts',(4.01615988348752,5.44952692272918,30.9950194811427));
#16281=CARTESIAN_POINT('Ctrl Pts',(3.86479978232193,5.55789587288653,31.0037685117509));
#16282=CARTESIAN_POINT('Ctrl Pts',(3.70923383581028,5.65984746713904,31.0125175423592));
#16283=CARTESIAN_POINT('Ctrl Pts',(3.55366577799506,5.76180044505404,31.0212666917072));
#16284=CARTESIAN_POINT('Ctrl Pts',(3.3938920002681,5.85733573571076,31.0300158410553));
#16285=CARTESIAN_POINT('Ctrl Pts',(3.23045513626017,5.94612887621941,31.0387649904033));
#16286=CARTESIAN_POINT('Ctrl Pts',(3.18695122151562,5.96976399206697,31.0410938545162));
#16287=CARTESIAN_POINT('Ctrl Pts',(3.14318791262656,5.99292165435337,31.0434227186292));
#16288=CARTESIAN_POINT('Ctrl Pts',(3.09917575053259,6.01559628526639,31.0457515827422));
#16289=CARTESIAN_POINT('Ctrl Pts',(3.09917575053261,6.01559628526638,29.0458547647091));
#16290=CARTESIAN_POINT('Ctrl Pts',(2.9439648467836,6.09555940883824,29.0540509860553));
#16291=CARTESIAN_POINT('Ctrl Pts',(2.78559192492888,6.1695453142795,29.0622472074014));
#16292=CARTESIAN_POINT('Ctrl Pts',(2.62455973683121,6.23730512223064,29.0704434287475));
#16293=CARTESIAN_POINT('Ctrl Pts',(2.46353786135157,6.30506059079456,29.0786391252017));
#16294=CARTESIAN_POINT('Ctrl Pts',(2.29985738630005,6.36659060972087,29.0868348216559));
#16295=CARTESIAN_POINT('Ctrl Pts',(2.13404236957982,6.42169387037705,29.09503051811));
#16296=CARTESIAN_POINT('Ctrl Pts',(1.96822457599583,6.47679805383413,29.1032263518155));
#16297=CARTESIAN_POINT('Ctrl Pts',(1.8002725099202,6.52547515085438,29.111422185521));
#16298=CARTESIAN_POINT('Ctrl Pts',(1.63072665516705,6.5675733399885,29.1196180192265));
#16299=CARTESIAN_POINT('Ctrl Pts',(1.46114711416693,6.60967989340848,29.1278154813227));
#16300=CARTESIAN_POINT('Ctrl Pts',(1.2899735019906,6.64520484872491,29.1360129434188));
#16301=CARTESIAN_POINT('Ctrl Pts',(1.11775783933176,6.67404722882693,29.1442104055149));
#16302=CARTESIAN_POINT('Ctrl Pts',(0.945476627084163,6.70290058706023,29.1524109877701));
#16303=CARTESIAN_POINT('Ctrl Pts',(0.772152927961196,6.72506624441566,29.1606115700254));
#16304=CARTESIAN_POINT('Ctrl Pts',(0.598345299828283,6.74049493006066,29.1688121522806));
#16305=CARTESIAN_POINT('Ctrl Pts',(0.424350213897592,6.75594025609978,29.1770215791596));
#16306=CARTESIAN_POINT('Ctrl Pts',(0.249870514114099,6.76463406695162,29.1852310060387));
#16307=CARTESIAN_POINT('Ctrl Pts',(0.0754671020344008,6.76657917388916,
29.1934404329178));
#16308=CARTESIAN_POINT('Ctrl Pts',(-0.0990439248821634,6.76852548104615,
29.2016549253866));
#16309=CARTESIAN_POINT('Ctrl Pts',(-0.273478212496277,6.76371479392963,
29.2098694178554));
#16310=CARTESIAN_POINT('Ctrl Pts',(-0.447278673085257,6.75220192149221,
29.2180839103242));
#16311=CARTESIAN_POINT('Ctrl Pts',(-0.621311993572233,6.74067362397311,
29.2263094086665));
#16312=CARTESIAN_POINT('Ctrl Pts',(-0.794709435215398,6.72242524414566,
29.2345349070087));
#16313=CARTESIAN_POINT('Ctrl Pts',(-0.966921867799625,6.6975630718621,29.242760405351));
#16314=CARTESIAN_POINT('Ctrl Pts',(-1.04025487874001,6.68697604324452,29.2462630593166));
#16315=CARTESIAN_POINT('Ctrl Pts',(-1.11337316883411,6.67519036143643,29.2497657132823));
#16316=CARTESIAN_POINT('Ctrl Pts',(-1.18623513486506,6.66221698872167,29.2532683672479));
#16317=CARTESIAN_POINT('Ctrl Pts',(-1.35732786195949,6.63175322500115,29.26149321557));
#16318=CARTESIAN_POINT('Ctrl Pts',(-1.52748644973448,6.59465170857477,29.269718063892));
#16319=CARTESIAN_POINT('Ctrl Pts',(-1.69615713523828,6.55098007725411,29.277942912214));
#16320=CARTESIAN_POINT('Ctrl Pts',(-1.86463786015288,6.50735762987311,29.2861584975332));
#16321=CARTESIAN_POINT('Ctrl Pts',(-2.03163367540517,6.45717989081006,29.2943740828525));
#16322=CARTESIAN_POINT('Ctrl Pts',(-2.19659849373558,6.40056591695755,29.3025896681717));
#16323=CARTESIAN_POINT('Ctrl Pts',(-2.36141066982093,6.34400432811753,29.310797651595));
#16324=CARTESIAN_POINT('Ctrl Pts',(-2.52419525441327,6.28101848063391,29.3190056350182));
#16325=CARTESIAN_POINT('Ctrl Pts',(-2.68441878475981,6.21177790878173,29.3272136184415));
#16326=CARTESIAN_POINT('Ctrl Pts',(-2.84452624169426,6.14258749803517,29.335415655618));
#16327=CARTESIAN_POINT('Ctrl Pts',(-3.00207601188468,6.06715152999008,29.3436176927945));
#16328=CARTESIAN_POINT('Ctrl Pts',(-3.15655208945124,5.98568859084576,29.3518197299711));
#16329=CARTESIAN_POINT('Ctrl Pts',(-3.31094727749595,5.90426830878011,29.3600174722504));
#16330=CARTESIAN_POINT('Ctrl Pts',(-3.46227166270541,5.81682750973103,29.3682152145298));
#16331=CARTESIAN_POINT('Ctrl Pts',(-3.61003136459167,5.72363193668709,29.3764129568092));
#16332=CARTESIAN_POINT('Ctrl Pts',(-3.75776297241603,5.63045408323899,29.3846091404236));
#16333=CARTESIAN_POINT('Ctrl Pts',(-3.90193094046812,5.5315238211852,29.3928053240379));
#16334=CARTESIAN_POINT('Ctrl Pts',(-4.04206778836664,5.42715183077172,29.4010015076523));
#16335=CARTESIAN_POINT('Ctrl Pts',(-4.18219432023783,5.32278752359302,29.4091970879132));
#16336=CARTESIAN_POINT('Ctrl Pts',(-4.31829003462124,5.21298249944986,29.4173926681741));
#16337=CARTESIAN_POINT('Ctrl Pts',(-4.44991819542317,5.09808954943338,29.4255882484349));
#16338=CARTESIAN_POINT('Ctrl Pts',(-4.58156061474275,4.98318415372787,29.4337847164757));
#16339=CARTESIAN_POINT('Ctrl Pts',(-4.70873424592737,4.86318997011062,29.4419811845164));
#16340=CARTESIAN_POINT('Ctrl Pts',(-4.831037045668,4.73849871408482,29.4501776525571));
#16341=CARTESIAN_POINT('Ctrl Pts',(-4.95337534540559,4.61377126478118,29.4583764997305));
#16342=CARTESIAN_POINT('Ctrl Pts',(-5.07083974634128,4.48434428348448,29.4665753469039));
#16343=CARTESIAN_POINT('Ctrl Pts',(-5.18306650837798,4.35064484527645,29.4747741940773));
#16344=CARTESIAN_POINT('Ctrl Pts',(-5.29541055829393,4.21680567815457,29.4829816098433));
#16345=CARTESIAN_POINT('Ctrl Pts',(-5.40250580228175,4.07868540857729,29.4911890256093));
#16346=CARTESIAN_POINT('Ctrl Pts',(-5.50402949796317,3.93674336038702,29.4993964413752));
#16347=CARTESIAN_POINT('Ctrl Pts',(-5.60560760677499,3.79472523625088,29.5076082560274));
#16348=CARTESIAN_POINT('Ctrl Pts',(-5.70160801720471,3.64888154952859,29.5158200706796));
#16349=CARTESIAN_POINT('Ctrl Pts',(-5.79175255353429,3.49969875255415,29.5240318853317));
#16350=CARTESIAN_POINT('Ctrl Pts',(-5.88202984139744,3.3502962612323,29.5322557931293));
#16351=CARTESIAN_POINT('Ctrl Pts',(-5.96643384746372,3.19754514655468,29.540479700927));
#16352=CARTESIAN_POINT('Ctrl Pts',(-6.04473281708655,3.04195564892667,29.5487036087246));
#16353=CARTESIAN_POINT('Ctrl Pts',(-6.1170796189689,2.89819382659247,29.5563023476479));
#16354=CARTESIAN_POINT('Ctrl Pts',(-6.18421473488204,2.75200919431501,29.5639010865713));
#16355=CARTESIAN_POINT('Ctrl Pts',(-6.24599284241516,2.60381689304347,29.5714998254947));
#16356=CARTESIAN_POINT('Ctrl Pts',(-6.31984132294676,2.42667038091511,29.5805832264899));
#16357=CARTESIAN_POINT('Ctrl Pts',(-6.38622117172981,2.2462088131756,29.589666627485));
#16358=CARTESIAN_POINT('Ctrl Pts',(-6.44485266720639,2.06304704212065,29.5987500284802));
#16359=CARTESIAN_POINT('Ctrl Pts',(-6.50324037875175,1.88064683950657,29.6077956615968));
#16360=CARTESIAN_POINT('Ctrl Pts',(-6.5539439232451,1.69556904279107,29.6168412947134));
#16361=CARTESIAN_POINT('Ctrl Pts',(-6.59673275028268,1.50844490166128,29.62588692783));
#16362=CARTESIAN_POINT('Ctrl Pts',(-6.63940881009013,1.32181391429492,29.6349087217562));
#16363=CARTESIAN_POINT('Ctrl Pts',(-6.67421169874369,1.13314755734616,29.6439305156825));
#16364=CARTESIAN_POINT('Ctrl Pts',(-6.70095996871385,0.943093048269617,
29.6529523096087));
#16365=CARTESIAN_POINT('Ctrl Pts',(-6.72759269831094,0.753859488320121,
29.6619351334843));
#16366=CARTESIAN_POINT('Ctrl Pts',(-6.74624015093949,0.563249957731145,
29.6709179573599));
#16367=CARTESIAN_POINT('Ctrl Pts',(-6.75677169811228,0.371920985679566,
29.6799007812355));
#16368=CARTESIAN_POINT('Ctrl Pts',(-6.76352438647371,0.249243386502655,
29.6856604487603));
#16369=CARTESIAN_POINT('Ctrl Pts',(-6.76694144236585,0.126270358197117,
29.6914201162852));
#16370=CARTESIAN_POINT('Ctrl Pts',(-6.76699925367029,0.0031781796254976,
29.69717978381));
#16371=CARTESIAN_POINT('',(-6.767,1.13258374575577E-12,29.3028202161899));
#16372=CARTESIAN_POINT('Ctrl Pts',(3.09917575053261,6.01559628526638,28.6513920151221));
#16373=CARTESIAN_POINT('Ctrl Pts',(2.93382384459268,6.10078395293758,28.6601414630345));
#16374=CARTESIAN_POINT('Ctrl Pts',(2.76495772122988,6.17915010267047,28.6688909109469));
#16375=CARTESIAN_POINT('Ctrl Pts',(2.59315093316716,6.25042856433175,28.6776403588593));
#16376=CARTESIAN_POINT('Ctrl Pts',(2.42134553245622,6.32170645041449,28.6863897361193));
#16377=CARTESIAN_POINT('Ctrl Pts',(2.24659977927595,6.38589665313456,28.6951391133793));
#16378=CARTESIAN_POINT('Ctrl Pts',(2.06950718689923,6.44278115439074,28.7038884906393));
#16379=CARTESIAN_POINT('Ctrl Pts',(1.89241596572865,6.49966521519723,28.712637800154));
#16380=CARTESIAN_POINT('Ctrl Pts',(1.71297821457201,6.54924360009545,28.7213871096686));
#16381=CARTESIAN_POINT('Ctrl Pts',(1.53180337335847,6.59134792173556,28.7301364191833));
#16382=CARTESIAN_POINT('Ctrl Pts',(1.35062987477779,6.63345193135306,28.7388856638594));
#16383=CARTESIAN_POINT('Ctrl Pts',(1.16771959102942,6.6680819236824,28.7476349085355));
#16384=CARTESIAN_POINT('Ctrl Pts',(0.983693746906687,6.69512028363171,28.7563841532116));
#16385=CARTESIAN_POINT('Ctrl Pts',(0.799669205419707,6.72215845218869,28.7651333359558));
#16386=CARTESIAN_POINT('Ctrl Pts',(0.614529402873306,6.74160505424581,28.7738825187));
#16387=CARTESIAN_POINT('Ctrl Pts',(0.428903127363072,6.75339404354123,28.7826317014442));
#16388=CARTESIAN_POINT('Ctrl Pts',(0.243278104163657,6.76518295330331,28.7913808251628));
#16389=CARTESIAN_POINT('Ctrl Pts',(0.0571669005388484,6.76931433552276,
28.8001299488814));
#16390=CARTESIAN_POINT('Ctrl Pts',(-0.128798404777828,6.76577415902472,
28.8088790726));
#16391=CARTESIAN_POINT('Ctrl Pts',(-0.314762517259509,6.7622340052344,28.8176281401992));
#16392=CARTESIAN_POINT('Ctrl Pts',(-0.500580446820015,6.75102239665086,
28.8263772077984));
#16393=CARTESIAN_POINT('Ctrl Pts',(-0.68562111884321,6.73217741012491,28.8351262753976));
#16394=CARTESIAN_POINT('Ctrl Pts',(-0.870660665414947,6.71333253821765,
28.8438752897834));
#16395=CARTESIAN_POINT('Ctrl Pts',(-1.05492267885519,6.68685441030607,28.8526243041692));
#16396=CARTESIAN_POINT('Ctrl Pts',(-1.2377813763527,6.65283295028174,28.861373318555));
#16397=CARTESIAN_POINT('Ctrl Pts',(-1.42999922978866,6.61707018861861,28.8705701289224));
#16398=CARTESIAN_POINT('Ctrl Pts',(-1.62066601233715,6.57297172934408,28.8797669392898));
#16399=CARTESIAN_POINT('Ctrl Pts',(-1.80906628500406,6.52070304311288,28.8889637496572));
#16400=CARTESIAN_POINT('Ctrl Pts',(-1.98831342545545,6.47097374915025,28.8977137473949));
#16401=CARTESIAN_POINT('Ctrl Pts',(-2.16550875896717,6.41384933989523,28.9064637451327));
#16402=CARTESIAN_POINT('Ctrl Pts',(-2.34005036714024,6.34952386240471,28.9152137428704));
#16403=CARTESIAN_POINT('Ctrl Pts',(-2.51458843547097,6.28519968948593,28.9239635631513));
#16404=CARTESIAN_POINT('Ctrl Pts',(-2.6864726171806,6.21367483971097,28.9327133834322));
#16405=CARTESIAN_POINT('Ctrl Pts',(-2.85511905908732,6.13519226743843,28.941463203713));
#16406=CARTESIAN_POINT('Ctrl Pts',(-3.02376230488879,6.0567111825294,28.9502128581716));
#16407=CARTESIAN_POINT('Ctrl Pts',(-3.18916767379893,5.97127275992639,28.9589625126301));
#16408=CARTESIAN_POINT('Ctrl Pts',(-3.3507733410277,5.87916720438006,28.9677121670886));
#16409=CARTESIAN_POINT('Ctrl Pts',(-3.51237616037351,5.78706327195653,28.9764616673571));
#16410=CARTESIAN_POINT('Ctrl Pts',(-3.67017916302283,5.68829258362309,28.9852111676255));
#16411=CARTESIAN_POINT('Ctrl Pts',(-3.82364636566446,5.58319061741053,28.9939606678939));
#16412=CARTESIAN_POINT('Ctrl Pts',(-3.97711106778796,5.47809036367704,29.0027100256024));
#16413=CARTESIAN_POINT('Ctrl Pts',(-4.12623987481938,5.36665920043217,29.0114593833108));
#16414=CARTESIAN_POINT('Ctrl Pts',(-4.27052628213953,5.24927559512316,29.0202087410193));
#16415=CARTESIAN_POINT('Ctrl Pts',(-4.41481053025014,5.13189374643006,29.0289579677958));
#16416=CARTESIAN_POINT('Ctrl Pts',(-4.55425230136578,5.0085598147731,29.0377071945723));
#16417=CARTESIAN_POINT('Ctrl Pts',(-4.68837800630607,4.8796926819202,29.0464564213489));
#16418=CARTESIAN_POINT('Ctrl Pts',(-4.8225018822896,4.75082730631744,29.0552055288197));
#16419=CARTESIAN_POINT('Ctrl Pts',(-4.95130963053038,4.61642907903449,29.0639546362905));
#16420=CARTESIAN_POINT('Ctrl Pts',(-5.07436379033444,4.47695444731602,29.0727037437614));
#16421=CARTESIAN_POINT('Ctrl Pts',(-5.197416435629,4.33748153220474,29.0814527435512));
#16422=CARTESIAN_POINT('Ctrl Pts',(-5.31471544462883,4.19293255254451,29.0902017433409));
#16423=CARTESIAN_POINT('Ctrl Pts',(-5.4258624527575,4.04379841779438,29.0989507431307));
#16424=CARTESIAN_POINT('Ctrl Pts',(-5.53702160019268,3.89464799484178,29.1077006984728));
#16425=CARTESIAN_POINT('Ctrl Pts',(-5.6420272308136,3.74091164443686,29.116450653815));
#16426=CARTESIAN_POINT('Ctrl Pts',(-5.74052265233068,3.5831115916307,29.1252006091571));
#16427=CARTESIAN_POINT('Ctrl Pts',(-5.83901427067014,3.42531763191619,29.1339502266396));
#16428=CARTESIAN_POINT('Ctrl Pts',(-5.93099603115831,3.26346052695447,29.142699844122));
#16429=CARTESIAN_POINT('Ctrl Pts',(-6.0161555062284,3.09809004466909,29.1514494616045));
#16430=CARTESIAN_POINT('Ctrl Pts',(-6.10131214578882,2.93272506863655,29.1601987877556));
#16431=CARTESIAN_POINT('Ctrl Pts',(-6.17964682328827,2.76384720416716,29.1689481139067));
#16432=CARTESIAN_POINT('Ctrl Pts',(-6.2508934828864,2.5920300279141,29.1776974400578));
#16433=CARTESIAN_POINT('Ctrl Pts',(-6.32213814889399,2.4202176593685,29.1864465213893));
#16434=CARTESIAN_POINT('Ctrl Pts',(-6.38629508412646,2.24546640831743,29.1951956027209));
#16435=CARTESIAN_POINT('Ctrl Pts',(-6.44314639819866,2.06836976659872,29.2039446840525));
#16436=CARTESIAN_POINT('Ctrl Pts',(-6.5000028528375,1.89125711158105,29.2126945564869));
#16437=CARTESIAN_POINT('Ctrl Pts',(-6.54955227673294,1.71179891440083,29.2214444289213));
#16438=CARTESIAN_POINT('Ctrl Pts',(-6.59162635926425,1.53060476278259,29.2301943013557));
#16439=CARTESIAN_POINT('Ctrl Pts',(-6.63369752055233,1.34942319164515,29.2389435662782));
#16440=CARTESIAN_POINT('Ctrl Pts',(-6.66829431424287,1.16650618642515,29.2476928312007));
#16441=CARTESIAN_POINT('Ctrl Pts',(-6.69529923745446,0.98247499761658,29.2564420961232));
#16442=CARTESIAN_POINT('Ctrl Pts',(-6.72230554731467,0.798434359175782,
29.2651918103029));
#16443=CARTESIAN_POINT('Ctrl Pts',(-6.74171916496721,0.613279706238397,
29.2739415244826));
#16444=CARTESIAN_POINT('Ctrl Pts',(-6.75347414817287,0.427639953653461,
29.2826912386623));
#16445=CARTESIAN_POINT('Ctrl Pts',(-6.76248837758749,0.285283364197147,
29.2894008978381));
#16446=CARTESIAN_POINT('Ctrl Pts',(-6.76699999999998,0.142641701104186,
29.296110557014));
#16447=CARTESIAN_POINT('Ctrl Pts',(-6.767,1.13258377759989E-12,29.3028202161899));
#16448=CARTESIAN_POINT('Ctrl Pts',(-6.7669999999775,1.74501576113346E-5,
29.303194762523));
#16449=CARTESIAN_POINT('Ctrl Pts',(-6.76700043912407,-0.170279283280337,
29.3112153743689));
#16450=CARTESIAN_POINT('Ctrl Pts',(-6.76056808912486,-0.340797073679393,
29.3192359862148));
#16451=CARTESIAN_POINT('Ctrl Pts',(-6.74767885333058,-0.51099813337755,
29.3272565980607));
#16452=CARTESIAN_POINT('Ctrl Pts',(-6.73479999248599,-0.68106219291069,
29.3352707538648));
#16453=CARTESIAN_POINT('Ctrl Pts',(-6.71547461738373,-0.850809655833912,
29.343284909669));
#16454=CARTESIAN_POINT('Ctrl Pts',(-6.68973068447703,-1.01970209824563,
29.3512990654731));
#16455=CARTESIAN_POINT('Ctrl Pts',(-6.66400175719607,-1.18849609661654,
29.3593085499854));
#16456=CARTESIAN_POINT('Ctrl Pts',(-6.63186177571983,-1.3564356954542,29.3673180344978));
#16457=CARTESIAN_POINT('Ctrl Pts',(-6.59339057337646,-1.52298711317939,
29.3753275190101));
#16458=CARTESIAN_POINT('Ctrl Pts',(-6.55492856997583,-1.68949870639008,
29.3833350883551));
#16459=CARTESIAN_POINT('Ctrl Pts',(-6.5101384373662,-1.8546224113429,29.3913426577001));
#16460=CARTESIAN_POINT('Ctrl Pts',(-6.45915121506458,-2.01783413117376,
29.3993502270452));
#16461=CARTESIAN_POINT('Ctrl Pts',(-6.40816847654063,-2.18103149828973,
29.4073570922106));
#16462=CARTESIAN_POINT('Ctrl Pts',(-6.35098984433623,-2.34231685517073,
29.415363957376));
#16463=CARTESIAN_POINT('Ctrl Pts',(-6.28779630693183,-2.50118104153508,
29.4233708225415));
#16464=CARTESIAN_POINT('Ctrl Pts',(-6.22459563317648,-2.66006316819256,
29.4313785919101));
#16465=CARTESIAN_POINT('Ctrl Pts',(-6.15537884183735,-2.81652323027482,
29.4393863612788));
#16466=CARTESIAN_POINT('Ctrl Pts',(-6.08037508791807,-2.9700720176833,29.4473941306474));
#16467=CARTESIAN_POINT('Ctrl Pts',(-6.00534779332565,-3.12366899790382,
29.455404413334));
#16468=CARTESIAN_POINT('Ctrl Pts',(-5.92453008738743,-3.27435254718969,
29.4634146960207));
#16469=CARTESIAN_POINT('Ctrl Pts',(-5.83819699347893,-3.42165820404867,
29.4714249787073));
#16470=CARTESIAN_POINT('Ctrl Pts',(-5.75177343064882,-3.56911822331169,
29.479443655413));
#16471=CARTESIAN_POINT('Ctrl Pts',(-5.65982313140622,-3.71319295820093,
29.4874623321186));
#16472=CARTESIAN_POINT('Ctrl Pts',(-5.56266471935812,-3.85344653784226,
29.4954810088243));
#16473=CARTESIAN_POINT('Ctrl Pts',(-5.46544895291773,-3.99378291174356,
29.5035044191019));
#16474=CARTESIAN_POINT('Ctrl Pts',(-5.36301917750028,-4.13029333907179,
29.5115278293795));
#16475=CARTESIAN_POINT('Ctrl Pts',(-5.25573379739927,-4.26257565925522,
29.519551239657));
#16476=CARTESIAN_POINT('Ctrl Pts',(-5.14829994362497,-4.39504104671185,
29.5275857536395));
#16477=CARTESIAN_POINT('Ctrl Pts',(-5.03599731748076,-4.52326636412461,
29.5356202676219));
#16478=CARTESIAN_POINT('Ctrl Pts',(-4.91922110787673,-4.64688634375967,
29.5436547816044));
#16479=CARTESIAN_POINT('Ctrl Pts',(-4.86090367700977,-4.70862151773549,
29.5476671760408));
#16480=CARTESIAN_POINT('Ctrl Pts',(-4.80147108011093,-4.76920876799802,
29.5516795704772));
#16481=CARTESIAN_POINT('Ctrl Pts',(-4.74097547761352,-4.82860647813293,
29.5556919649136));
#16482=CARTESIAN_POINT('Ctrl Pts',(-4.61694741955579,-4.95038363774422,
29.5639181742506));
#16483=CARTESIAN_POINT('Ctrl Pts',(-4.48805099989343,-5.06754926241064,
29.5721443835875));
#16484=CARTESIAN_POINT('Ctrl Pts',(-4.35466262607329,-5.17969134341811,
29.5803705929245));
#16485=CARTESIAN_POINT('Ctrl Pts',(-4.22142410837691,-5.29170743760162,
29.5885875604677));
#16486=CARTESIAN_POINT('Ctrl Pts',(-4.08370395753063,-5.3987109976466,29.5968045280109));
#16487=CARTESIAN_POINT('Ctrl Pts',(-3.94191601363492,-5.50032609410102,
29.6050214955541));
#16488=CARTESIAN_POINT('Ctrl Pts',(-3.80025890444357,-5.60184742531182,
29.6132308808975));
#16489=CARTESIAN_POINT('Ctrl Pts',(-3.65454176721587,-5.69798998765376,
29.6214402662408));
#16490=CARTESIAN_POINT('Ctrl Pts',(-3.50521223831033,-5.78841741449245,
29.6296496515842));
#16491=CARTESIAN_POINT('Ctrl Pts',(-3.35599054108758,-5.87877954318363,
29.6378531088848));
#16492=CARTESIAN_POINT('Ctrl Pts',(-3.20316195345764,-5.96343457149376,
29.6460565661854));
#16493=CARTESIAN_POINT('Ctrl Pts',(-3.04720394539792,-6.04208880397759,
29.654260023486));
#16494=CARTESIAN_POINT('Ctrl Pts',(-2.89132727068957,-6.12070201764868,
29.6624592026179));
#16495=CARTESIAN_POINT('Ctrl Pts',(-2.73232474627738,-6.19332050883013,
29.6706583817498));
#16496=CARTESIAN_POINT('Ctrl Pts',(-2.57069942579331,-6.25969595605298,
29.6788575608816));
#16497=CARTESIAN_POINT('Ctrl Pts',(-2.40910455900307,-6.326058896711,29.6870551951114));
#16498=CARTESIAN_POINT('Ctrl Pts',(-2.24488820956445,-6.38618099467243,
29.6952528293412));
#16499=CARTESIAN_POINT('Ctrl Pts',(-2.07857472887093,-6.43986149668602,
29.703450463571));
#16500=CARTESIAN_POINT('Ctrl Pts',(-1.91227325286635,-6.49353812398227,
29.7116475060866));
#16501=CARTESIAN_POINT('Ctrl Pts',(-1.7438752881423,-6.54077397031308,29.7198445486022));
#16502=CARTESIAN_POINT('Ctrl Pts',(-1.57392166355624,-6.58141774977006,
29.7280415911178));
#16503=CARTESIAN_POINT('Ctrl Pts',(-1.40394941762237,-6.62206598245335,
29.7362395317607));
#16504=CARTESIAN_POINT('Ctrl Pts',(-1.23242152115803,-6.65612062584086,
29.7444374724035));
#16505=CARTESIAN_POINT('Ctrl Pts',(-1.05989039667072,-6.68348122964711,
29.7526354130463));
#16506=CARTESIAN_POINT('Ctrl Pts',(-0.887309011067003,-6.71084980404126,
29.7608357418823));
#16507=CARTESIAN_POINT('Ctrl Pts',(-0.713724169464792,-6.73152039836163,
29.7690360707183));
#16508=CARTESIAN_POINT('Ctrl Pts',(-0.539694892081964,-6.74544427176303,
29.7772363995543));
#16509=CARTESIAN_POINT('Ctrl Pts',(-0.365484271676276,-6.75938265420182,
29.7854452733457));
#16510=CARTESIAN_POINT('Ctrl Pts',(-0.190828648268228,-6.76656024168427,
29.7936541471371));
#16511=CARTESIAN_POINT('Ctrl Pts',(-0.0162895385699319,-6.76698039386351,
29.8018630209285));
#16512=CARTESIAN_POINT('Ctrl Pts',(0.158343244343235,-6.7674007715338,29.810076300332));
#16513=CARTESIAN_POINT('Ctrl Pts',(0.332859030791997,-6.76105649708345,
29.8182895797354));
#16514=CARTESIAN_POINT('Ctrl Pts',(0.506700040159683,-6.7480029689755,29.8265028591388));
#16515=CARTESIAN_POINT('Ctrl Pts',(0.680795319326209,-6.73493034803107,
29.8347281517543));
#16516=CARTESIAN_POINT('Ctrl Pts',(0.854213492679924,-6.71512890280006,
29.8429534443697));
#16517=CARTESIAN_POINT('Ctrl Pts',(1.02640432737228,-6.68870564135928,29.8511787369851));
#16518=CARTESIAN_POINT('Ctrl Pts',(1.18213025302498,-6.66480897546541,29.8586175260972));
#16519=CARTESIAN_POINT('Ctrl Pts',(1.33685228200919,-6.63549701095803,29.8660563152092));
#16520=CARTESIAN_POINT('Ctrl Pts',(1.49017400361122,-6.60088406495382,29.8734951043213));
#16521=CARTESIAN_POINT('Ctrl Pts',(1.6597251608569,-6.56260726379757,29.8817213053401));
#16522=CARTESIAN_POINT('Ctrl Pts',(1.82803757945248,-6.5177400964149,29.889947506359));
#16523=CARTESIAN_POINT('Ctrl Pts',(1.99456103082754,-6.46637574645212,29.8981737073778));
#16524=CARTESIAN_POINT('Ctrl Pts',(2.16089742820167,-6.41506909351091,29.9063906679936));
#16525=CARTESIAN_POINT('Ctrl Pts',(2.32544852027893,-6.35727989546785,29.9146076286094));
#16526=CARTESIAN_POINT('Ctrl Pts',(2.48767412589913,-6.29315234547297,29.9228245892251));
#16527=CARTESIAN_POINT('Ctrl Pts',(2.64975006520956,-6.2290839583564,29.9310339690267));
#16528=CARTESIAN_POINT('Ctrl Pts',(2.8095044593794,-6.15868899610454,29.9392433488283));
#16529=CARTESIAN_POINT('Ctrl Pts',(2.9664120727298,-6.08216149199961,29.9474527286298));
#16530=CARTESIAN_POINT('Ctrl Pts',(3.12320640855058,-6.00568923598894,29.9556561817702));
#16531=CARTESIAN_POINT('Ctrl Pts',(3.27715773611907,-5.92309341315075,29.9638596349106));
#16532=CARTESIAN_POINT('Ctrl Pts',(3.42776052468915,-5.83461625005302,29.972063088051));
#16533=CARTESIAN_POINT('Ctrl Pts',(3.57828479796524,-5.74618521366076,29.9802622644011));
#16534=CARTESIAN_POINT('Ctrl Pts',(3.72546370155774,-5.65187912661656,29.9884614407513));
#16535=CARTESIAN_POINT('Ctrl Pts',(3.86881598384822,-5.55198630069641,29.9966606171014));
#16536=CARTESIAN_POINT('Ctrl Pts',(4.01214129224333,-5.45211227111902,30.0048582506528));
#16537=CARTESIAN_POINT('Ctrl Pts',(4.15164111607589,-5.34665379632587,30.0130558842042));
#16538=CARTESIAN_POINT('Ctrl Pts',(4.28686264893904,-5.23594285961291,30.0212535177555));
#16539=CARTESIAN_POINT('Ctrl Pts',(4.42207444253328,-5.1252398968044,30.0294505608761));
#16540=CARTESIAN_POINT('Ctrl Pts',(4.55300828075326,-5.00928545203083,30.0376476039967));
#16541=CARTESIAN_POINT('Ctrl Pts',(4.67924401020246,-4.88845215717454,30.0458446471173));
#16542=CARTESIAN_POINT('Ctrl Pts',(4.80549359071392,-4.76760560403158,30.0540425896485));
#16543=CARTESIAN_POINT('Ctrl Pts',(4.92704377627779,-4.64187938235337,30.0622405321797));
#16544=CARTESIAN_POINT('Ctrl Pts',(5.04351086237034,-4.51168340879016,30.0704384747108));
#16545=CARTESIAN_POINT('Ctrl Pts',(5.16001189545016,-4.38144948664246,30.0786388067193));
#16546=CARTESIAN_POINT('Ctrl Pts',(5.2714266388413,-4.24674348482788,30.0868391387277));
#16547=CARTESIAN_POINT('Ctrl Pts',(5.37741127787934,-4.10800887882878,30.0950394707361));
#16548=CARTESIAN_POINT('Ctrl Pts',(5.48350638155685,-3.96912967387295,30.1032483497069));
#16549=CARTESIAN_POINT('Ctrl Pts',(5.58415985575435,-3.82621376137857,30.1114572286777));
#16550=CARTESIAN_POINT('Ctrl Pts',(5.67907032608305,-3.67973494037315,30.1196661076484));
#16551=CARTESIAN_POINT('Ctrl Pts',(5.7740317465538,-3.53317748613884,30.1278793933358));
#16552=CARTESIAN_POINT('Ctrl Pts',(5.86324383407599,-3.38305361850086,30.1360926790232));
#16553=CARTESIAN_POINT('Ctrl Pts',(5.94645097924401,-3.22986218768665,30.1443059647107));
#16554=CARTESIAN_POINT('Ctrl Pts',(6.02977984621011,-3.07644665669003,30.1525312654227));
#16555=CARTESIAN_POINT('Ctrl Pts',(6.10708605674115,-2.91995491616811,30.1607565661348));
#16556=CARTESIAN_POINT('Ctrl Pts',(6.17816147052971,-2.76090743127367,30.1689818668469));
#16557=CARTESIAN_POINT('Ctrl Pts',(6.2424406086294,-2.61706816673768,30.1764206591409));
#16558=CARTESIAN_POINT('Ctrl Pts',(6.3016241288705,-2.47113897961145,30.1838594514349));
#16559=CARTESIAN_POINT('Ctrl Pts',(6.35559336697599,-2.32351499966124,30.1912982437289));
#16560=CARTESIAN_POINT('Ctrl Pts',(6.41474103907805,-2.16172626468913,30.1994507999422));
#16561=CARTESIAN_POINT('Ctrl Pts',(6.46779942281192,-1.99742449187936,30.2076033561554));
#16562=CARTESIAN_POINT('Ctrl Pts',(6.51454649890016,-1.83111247979684,30.2157559123687));
#16563=CARTESIAN_POINT('Ctrl Pts',(6.56123941737387,-1.66499314418938,30.2238990236491));
#16564=CARTESIAN_POINT('Ctrl Pts',(6.60163548513474,-1.49686855355554,30.2320421349294));
#16565=CARTESIAN_POINT('Ctrl Pts',(6.6355607488154,-1.32726129634689,30.2401852462098));
#16566=CARTESIAN_POINT('Ctrl Pts',(6.66945384162423,-1.15781487542191,30.2483206354871));
#16567=CARTESIAN_POINT('Ctrl Pts',(6.69688827548844,-0.986888943069949,
30.2564560247644));
#16568=CARTESIAN_POINT('Ctrl Pts',(6.71773992286671,-0.815021060294054,
30.2645914140417));
#16569=CARTESIAN_POINT('Ctrl Pts',(6.73857617834234,-0.643280043931621,
30.2727207980803));
#16570=CARTESIAN_POINT('Ctrl Pts',(6.75283927894112,-0.470598823004949,
30.2808501821189));
#16571=CARTESIAN_POINT('Ctrl Pts',(6.76045619009791,-0.297524959905691,
30.2889795661576));
#16572=CARTESIAN_POINT('Ctrl Pts',(6.7680690786526,-0.124542499642788,30.2971046569497));
#16573=CARTESIAN_POINT('Ctrl Pts',(6.76904275194078,0.0488318254332298,
30.3052297477418));
#16574=CARTESIAN_POINT('Ctrl Pts',(6.76335602970208,0.222045525720619,30.3133548385339));
#16575=CARTESIAN_POINT('Ctrl Pts',(6.75764760001176,0.395920420253286,30.321510944559));
#16576=CARTESIAN_POINT('Ctrl Pts',(6.74522778903052,0.569633090865725,30.3296670505841));
#16577=CARTESIAN_POINT('Ctrl Pts',(6.72612801283416,0.742624370033458,30.3378231566093));
#16578=CARTESIAN_POINT('Ctrl Pts',(6.70710510978276,0.914919390588353,30.3459464357827));
#16579=CARTESIAN_POINT('Ctrl Pts',(6.68145597482379,1.08649845211539,30.3540697149561));
#16580=CARTESIAN_POINT('Ctrl Pts',(6.64926363232801,1.25681428532626,30.3621929941295));
#16581=CARTESIAN_POINT('Ctrl Pts',(6.6170670031498,1.42715279752948,30.3703173549862));
#16582=CARTESIAN_POINT('Ctrl Pts',(6.57832549895059,1.59622738687732,30.3784417158428));
#16583=CARTESIAN_POINT('Ctrl Pts',(6.53317324601633,1.76350115892689,30.3865660766995));
#16584=CARTESIAN_POINT('Ctrl Pts',(6.48800639022984,1.93082902958763,30.3946930650849));
#16585=CARTESIAN_POINT('Ctrl Pts',(6.43642475235122,2.09635457018854,30.4028200534703));
#16586=CARTESIAN_POINT('Ctrl Pts',(6.37861226929006,2.25955626574386,30.4109470418557));
#16587=CARTESIAN_POINT('Ctrl Pts',(6.32042603510757,2.42381304168124,30.4191265702958));
#16588=CARTESIAN_POINT('Ctrl Pts',(6.25592823851356,2.58571546736119,30.4273060987359));
#16589=CARTESIAN_POINT('Ctrl Pts',(6.18535513706265,2.74475332742539,30.4354856271759));
#16590=CARTESIAN_POINT('Ctrl Pts',(6.11511438709857,2.90304222693424,30.4436266355796));
#16591=CARTESIAN_POINT('Ctrl Pts',(6.03885564892182,3.05849318339986,30.4517676439833));
#16592=CARTESIAN_POINT('Ctrl Pts',(5.9568573097243,3.21062922050869,30.4599086523869));
#16593=CARTESIAN_POINT('Ctrl Pts',(5.87427699489374,3.36384502907839,30.4681074408452));
#16594=CARTESIAN_POINT('Ctrl Pts',(5.78587549881093,3.51369836550209,30.4763062293035));
#16595=CARTESIAN_POINT('Ctrl Pts',(5.69198041889014,3.65973331145471,30.4845050177618));
#16596=CARTESIAN_POINT('Ctrl Pts',(5.59808533896934,3.80576825740733,30.4927038062201));
#16597=CARTESIAN_POINT('Ctrl Pts',(5.49869694104231,3.94798454559957,30.5009025946784));
#16598=CARTESIAN_POINT('Ctrl Pts',(5.3941824658027,4.08596188499436,30.5091013831367));
#16599=CARTESIAN_POINT('Ctrl Pts',(5.28922318646113,4.22452644339782,30.5173350648931));
#16600=CARTESIAN_POINT('Ctrl Pts',(5.17876790491029,4.35924673323055,30.5255687466494));
#16601=CARTESIAN_POINT('Ctrl Pts',(5.06312694145214,4.48965862563531,30.5338024284058));
#16602=CARTESIAN_POINT('Ctrl Pts',(4.94761961040267,4.61991981663823,30.5420265954825));
#16603=CARTESIAN_POINT('Ctrl Pts',(4.82693876392312,4.74588225737914,30.5502507625592));
#16604=CARTESIAN_POINT('Ctrl Pts',(4.70143722576662,4.86711177313362,30.5584749296358));
#16605=CARTESIAN_POINT('Ctrl Pts',(4.57608811390686,4.98819405112183,30.566689108155));
#16606=CARTESIAN_POINT('Ctrl Pts',(4.44593023459203,5.10455461276947,30.5749032866742));
#16607=CARTESIAN_POINT('Ctrl Pts',(4.31135555119798,5.21579354567974,30.5831174651934));
#16608=CARTESIAN_POINT('Ctrl Pts',(4.17687549472523,5.3269542603287,30.5913258678682));
#16609=CARTESIAN_POINT('Ctrl Pts',(4.0379850917432,5.43300028865593,30.599534270543));
#16610=CARTESIAN_POINT('Ctrl Pts',(3.89511235262337,5.53356926047202,30.6077426732179));
#16611=CARTESIAN_POINT('Ctrl Pts',(3.75232278353098,5.63407968841055,30.6159462975628));
#16612=CARTESIAN_POINT('Ctrl Pts',(3.60555578833066,5.72911920548128,30.6241499219078));
#16613=CARTESIAN_POINT('Ctrl Pts',(3.45527154973213,5.81836639595787,30.6323535462528));
#16614=CARTESIAN_POINT('Ctrl Pts',(3.33861577388611,5.88764312347243,30.638721480586));
#16615=CARTESIAN_POINT('Ctrl Pts',(3.21984142160767,5.95343052413751,30.6450894149192));
#16616=CARTESIAN_POINT('Ctrl Pts',(3.09917575053255,6.01559628526641,30.6514573492524));
#16617=CARTESIAN_POINT('Origin',(0.,0.,-3.69717978381041));
#16618=CARTESIAN_POINT('',(3.09917575053263,6.01559628526637,33.0456763245139));
#16619=CARTESIAN_POINT('',(3.0991757505326,6.01559628526638,32.6511251802053));
#16620=CARTESIAN_POINT('',(3.09917575053259,6.01559628526639,-3.69717978381041));
#16621=CARTESIAN_POINT('',(-6.76699986099963,-0.000377079920512664,31.69717978381));
#16622=CARTESIAN_POINT('Ctrl Pts',(-6.76699816095994,-0.00498894425489755,
31.69717978381));
#16623=CARTESIAN_POINT('Ctrl Pts',(-6.76684478702294,-0.213025173280864,
31.706943004568));
#16624=CARTESIAN_POINT('Ctrl Pts',(-6.75709420253893,-0.420655042332459,
31.7167062253261));
#16625=CARTESIAN_POINT('Ctrl Pts',(-6.73788167899273,-0.62708809580008,
31.7264694460841));
#16626=CARTESIAN_POINT('Ctrl Pts',(-6.71853295542026,-0.834984579474335,
31.7363018795575));
#16627=CARTESIAN_POINT('Ctrl Pts',(-6.68958775694725,-1.04166719573885,
31.7461343130309));
#16628=CARTESIAN_POINT('Ctrl Pts',(-6.65123312178949,-1.24634945324755,
31.7559667465042));
#16629=CARTESIAN_POINT('Ctrl Pts',(-6.61257356191642,-1.45265896333844,
31.7658773491993));
#16630=CARTESIAN_POINT('Ctrl Pts',(-6.56435440770036,-1.65693616212937,
31.7757879518943));
#16631=CARTESIAN_POINT('Ctrl Pts',(-6.50681559014289,-1.858397125448,31.7856985545894));
#16632=CARTESIAN_POINT('Ctrl Pts',(-6.48084152195962,-1.94934026643764,
31.7901723808004));
#16633=CARTESIAN_POINT('Ctrl Pts',(-6.45296895452249,-2.03970981023404,
31.7946462070114));
#16634=CARTESIAN_POINT('Ctrl Pts',(-6.42322312053385,-2.12943507622078,
31.7991200332224));
#16635=CARTESIAN_POINT('Ctrl Pts',(-6.36902839969197,-2.2929079089029,31.8072710153967));
#16636=CARTESIAN_POINT('Ctrl Pts',(-6.30850382475154,-2.45456728264385,
31.8154219975709));
#16637=CARTESIAN_POINT('Ctrl Pts',(-6.24178762935317,-2.61388144146856,
31.8235729797452));
#16638=CARTESIAN_POINT('Ctrl Pts',(-6.17514893099906,-2.77301054213242,
31.8317144937982));
#16639=CARTESIAN_POINT('Ctrl Pts',(-6.10233306850275,-2.92979951671739,
31.8398560078513));
#16640=CARTESIAN_POINT('Ctrl Pts',(-6.02352823808606,-3.08373094886371,
31.8479975219043));
#16641=CARTESIAN_POINT('Ctrl Pts',(-5.94479836335716,-3.23751596820376,
31.8561312921074));
#16642=CARTESIAN_POINT('Ctrl Pts',(-5.86009102698877,-3.38844853289979,
31.8642650623104));
#16643=CARTESIAN_POINT('Ctrl Pts',(-5.76964277484345,-3.53603043690191,
31.8723988325135));
#16644=CARTESIAN_POINT('Ctrl Pts',(-5.67926152996687,-3.68350300700242,
31.8805265769315));
#16645=CARTESIAN_POINT('Ctrl Pts',(-5.58314802813492,-3.82762954854115,
31.8886543213494));
#16646=CARTESIAN_POINT('Ctrl Pts',(-5.48158506974634,-3.96793575088283,
31.8967820657674));
#16647=CARTESIAN_POINT('Ctrl Pts',(-5.38007599994814,-4.10816750774175,
31.9049054976615));
#16648=CARTESIAN_POINT('Ctrl Pts',(-5.27312344592436,-4.24458266672557,
31.9130289295555));
#16649=CARTESIAN_POINT('Ctrl Pts',(-5.161053906689,-4.3767352641267,31.9211523614496));
#16650=CARTESIAN_POINT('Ctrl Pts',(-5.04827344237681,-4.50972618562644,
31.9293273252004));
#16651=CARTESIAN_POINT('Ctrl Pts',(-4.93031104950779,-4.63839996191676,
31.9375022889512));
#16652=CARTESIAN_POINT('Ctrl Pts',(-4.80754146012847,-4.76233494298184,
31.945677252702));
#16653=CARTESIAN_POINT('Ctrl Pts',(-4.68557343699443,-4.88546074892519,
31.9537988418751));
#16654=CARTESIAN_POINT('Ctrl Pts',(-4.55886108246186,-5.00390921065724,
31.9619204310481));
#16655=CARTESIAN_POINT('Ctrl Pts',(-4.42780940443511,-5.11730328180733,
31.9700420202211));
#16656=CARTESIAN_POINT('Ctrl Pts',(-4.29674042489908,-5.23071232330044,
31.9781646816105));
#16657=CARTESIAN_POINT('Ctrl Pts',(-4.16133125758528,-5.33906540560404,
31.9862873429998));
#16658=CARTESIAN_POINT('Ctrl Pts',(-4.02202050047103,-5.44202536688233,
31.9944100043892));
#16659=CARTESIAN_POINT('Ctrl Pts',(-3.88266482259069,-5.54501852760934,
32.0025352849314));
#16660=CARTESIAN_POINT('Ctrl Pts',(-3.73940534388417,-5.64261488698913,
32.0106605654737));
#16661=CARTESIAN_POINT('Ctrl Pts',(-3.59271012898014,-5.73452028761984,
32.018785846016));
#16662=CARTESIAN_POINT('Ctrl Pts',(-3.44441670014892,-5.82742697852009,
32.0269996498037));
#16663=CARTESIAN_POINT('Ctrl Pts',(-3.29261255875426,-5.91451777661114,
32.0352134535915));
#16664=CARTESIAN_POINT('Ctrl Pts',(-3.13780644165434,-5.99553665110243,
32.0434272573792));
#16665=CARTESIAN_POINT('Ctrl Pts',(-2.98440373249586,-6.07582104213792,
32.0515665982344));
#16666=CARTESIAN_POINT('Ctrl Pts',(-2.8280536103083,-6.15014304943466,32.0597059390896));
#16667=CARTESIAN_POINT('Ctrl Pts',(-2.66927053666758,-6.218302324757,32.0678452799447));
#16668=CARTESIAN_POINT('Ctrl Pts',(-2.50830851754669,-6.28739693494528,
32.0760963151988));
#16669=CARTESIAN_POINT('Ctrl Pts',(-2.34484665549254,-6.35015830627715,
32.0843473504529));
#16670=CARTESIAN_POINT('Ctrl Pts',(-2.17943561200694,-6.40643031751037,
32.092598385707));
#16671=CARTESIAN_POINT('Ctrl Pts',(-2.01402456852133,-6.46270232874358,
32.100849420961));
#16672=CARTESIAN_POINT('Ctrl Pts',(-1.84666473067044,-6.51248493471082,
32.1091004562151));
#16673=CARTESIAN_POINT('Ctrl Pts',(-1.67791584378681,-6.5556759698119,32.1173514914692));
#16674=CARTESIAN_POINT('Ctrl Pts',(-1.50956092534225,-6.59876616925714,
32.1255832635));
#16675=CARTESIAN_POINT('Ctrl Pts',(-1.33929790619343,-6.63543023282369,
32.1338150355308));
#16676=CARTESIAN_POINT('Ctrl Pts',(-1.16765820561721,-6.66549797951022,
32.1420468075617));
#16677=CARTESIAN_POINT('Ctrl Pts',(-0.996223459996037,-6.69552982230243,
32.1502687500341));
#16678=CARTESIAN_POINT('Ctrl Pts',(-0.823415655782832,-6.71898097124773,
32.1584906925064));
#16679=CARTESIAN_POINT('Ctrl Pts',(-0.649780791222935,-6.73573113502593,
32.1667126349788));
#16680=CARTESIAN_POINT('Ctrl Pts',(-0.476318474771694,-6.75246465347725,
32.1749264069687));
#16681=CARTESIAN_POINT('Ctrl Pts',(-0.302031088948244,-6.76251041405279,
32.1831401789586));
#16682=CARTESIAN_POINT('Ctrl Pts',(-0.127474328789869,-6.76579923553009,
32.1913539509485));
#16683=CARTESIAN_POINT('Ctrl Pts',(0.0469439284113645,-6.76908544747512,
32.1995612056789));
#16684=CARTESIAN_POINT('Ctrl Pts',(0.221630777597417,-6.76562539220543,
32.2077684604092));
#16685=CARTESIAN_POINT('Ctrl Pts',(0.396025806211847,-6.75540173200782,
32.2159757151396));
#16686=CARTESIAN_POINT('Ctrl Pts',(0.570317379979352,-6.74518413670329,
32.2241781011516));
#16687=CARTESIAN_POINT('Ctrl Pts',(0.744317121298345,-6.72821095039046,
32.2323804871635));
#16688=CARTESIAN_POINT('Ctrl Pts',(0.917464927668259,-6.70451691820512,
32.2405828731755));
#16689=CARTESIAN_POINT('Ctrl Pts',(1.09056105361766,-6.68082995811369,32.2487828109742));
#16690=CARTESIAN_POINT('Ctrl Pts',(1.26280539605337,-6.65042619271413,32.2569827487729));
#16691=CARTESIAN_POINT('Ctrl Pts',(1.43364303215575,-6.61339222006009,32.2651826865716));
#16692=CARTESIAN_POINT('Ctrl Pts',(1.60445678074731,-6.57636342571127,32.2733814778073));
#16693=CARTESIAN_POINT('Ctrl Pts',(1.77386386440957,-6.53270634561018,32.2815802690431));
#16694=CARTESIAN_POINT('Ctrl Pts',(1.94131959180215,-6.4825586956452,32.2897790602788));
#16695=CARTESIAN_POINT('Ctrl Pts',(2.10878228190038,-6.43240896057192,32.2979781924153));
#16696=CARTESIAN_POINT('Ctrl Pts',(2.27429311068322,-6.37576822073721,32.3061773245517));
#16697=CARTESIAN_POINT('Ctrl Pts',(2.43732253438915,-6.31282407986781,32.3143764566881));
#16698=CARTESIAN_POINT('Ctrl Pts',(2.60038831103241,-6.24986590346816,32.322577417099));
#16699=CARTESIAN_POINT('Ctrl Pts',(2.76097124625396,-6.18060165564131,32.3307783775099));
#16700=CARTESIAN_POINT('Ctrl Pts',(2.91856171277046,-6.10526711362823,32.3389793379208));
#16701=CARTESIAN_POINT('Ctrl Pts',(3.07629987949085,-6.029861965014,32.3471879846059));
#16702=CARTESIAN_POINT('Ctrl Pts',(3.2310396501565,-5.9483753100772,32.3553966312909));
#16703=CARTESIAN_POINT('Ctrl Pts',(3.38229511921994,-5.86108938052483,32.3636052779759));
#16704=CARTESIAN_POINT('Ctrl Pts',(3.53362280189238,-5.77376177821824,32.3718178436994));
#16705=CARTESIAN_POINT('Ctrl Pts',(3.68146256310972,-5.68062957185078,32.380030409423));
#16706=CARTESIAN_POINT('Ctrl Pts',(3.82535752992038,-5.58201834180804,32.3882429751465));
#16707=CARTESIAN_POINT('Ctrl Pts',(3.96944994138975,-5.48327180292795,32.3964668096952));
#16708=CARTESIAN_POINT('Ctrl Pts',(4.10958645295233,-5.37903142924726,32.404690644244));
#16709=CARTESIAN_POINT('Ctrl Pts',(4.24534236141756,-5.2696638635072,32.4129144787927));
#16710=CARTESIAN_POINT('Ctrl Pts',(4.37007650441145,-5.16917564359735,32.4204706357671));
#16711=CARTESIAN_POINT('Ctrl Pts',(4.49111271303223,-5.06435956603924,32.4280267927415));
#16712=CARTESIAN_POINT('Ctrl Pts',(4.60814964621003,-4.95552679723704,32.4355829497159));
#16713=CARTESIAN_POINT('Ctrl Pts',(4.74206273581399,-4.83100087260165,32.4442286677683));
#16714=CARTESIAN_POINT('Ctrl Pts',(4.8710450556412,-4.70093232175336,32.4528743858207));
#16715=CARTESIAN_POINT('Ctrl Pts',(4.9946388149526,-4.56572799323053,32.4615201038731));
#16716=CARTESIAN_POINT('Ctrl Pts',(5.11807390506471,-4.4306972395117,32.4701547225855));
#16717=CARTESIAN_POINT('Ctrl Pts',(5.2361340243519,-4.29054407950895,32.4787893412978));
#16718=CARTESIAN_POINT('Ctrl Pts',(5.34839713467694,-4.14571309786139,32.4874239600102));
#16719=CARTESIAN_POINT('Ctrl Pts',(5.46462494195089,-3.99576724856602,32.4963635199126));
#16720=CARTESIAN_POINT('Ctrl Pts',(5.57463855681819,-3.84080733988134,32.505303079815));
#16721=CARTESIAN_POINT('Ctrl Pts',(5.67801202730815,-3.68136773736936,32.5142426397175));
#16722=CARTESIAN_POINT('Ctrl Pts',(5.77758215396685,-3.5277942785188,32.522853292988));
#16723=CARTESIAN_POINT('Ctrl Pts',(5.87099180450186,-3.37006514882201,32.5314639462585));
#16724=CARTESIAN_POINT('Ctrl Pts',(5.95790150533329,-3.20869111208096,32.540074599529));
#16725=CARTESIAN_POINT('Ctrl Pts',(6.04472894031823,-3.04746982666234,32.5486771022401));
#16726=CARTESIAN_POINT('Ctrl Pts',(6.12506854816439,-2.88261078050792,32.5572796049512));
#16727=CARTESIAN_POINT('Ctrl Pts',(6.19862503150459,-2.71465222796674,32.5658821076623));
#16728=CARTESIAN_POINT('Ctrl Pts',(6.27209872850359,-2.54688270939516,32.5744749284298));
#16729=CARTESIAN_POINT('Ctrl Pts',(6.33880440904753,-2.37602092253564,32.5830677491973));
#16730=CARTESIAN_POINT('Ctrl Pts',(6.39849336995919,-2.20262833782468,32.5916605699648));
#16731=CARTESIAN_POINT('Ctrl Pts',(6.40552798512501,-2.18219323412346,32.592673272923));
#16732=CARTESIAN_POINT('Ctrl Pts',(6.41246519380273,-2.16172300429233,32.5936859758812));
#16733=CARTESIAN_POINT('Ctrl Pts',(6.41930463211463,-2.14121858765322,32.5946986788394));
#16734=CARTESIAN_POINT('Ctrl Pts',(6.47735396903799,-1.96718853787127,32.6032939365995));
#16735=CARTESIAN_POINT('Ctrl Pts',(6.52828795764044,-1.79089905606792,32.6118891943595));
#16736=CARTESIAN_POINT('Ctrl Pts',(6.57196228735581,-1.61294782729417,32.6204844521196));
#16737=CARTESIAN_POINT('Ctrl Pts',(6.61567751622878,-1.43482995474136,32.629087758974));
#16738=CARTESIAN_POINT('Ctrl Pts',(6.65211944363989,-1.25504752561917,32.6376910658284));
#16739=CARTESIAN_POINT('Ctrl Pts',(6.68119499365782,-1.07420782752765,32.6462943726829));
#16740=CARTESIAN_POINT('Ctrl Pts',(6.71147602606209,-0.885870452843098,
32.6552543756229));
#16741=CARTESIAN_POINT('Ctrl Pts',(6.7337667928603,-0.696386650018505,32.6642143785629));
#16742=CARTESIAN_POINT('Ctrl Pts',(6.7480220248994,-0.506446198003862,32.6731743815029));
#16743=CARTESIAN_POINT('Ctrl Pts',(6.76174720473161,-0.323568300670539,
32.6818012247076));
#16744=CARTESIAN_POINT('Ctrl Pts',(6.7680236811107,-0.140267398301859,32.6904280679123));
#16745=CARTESIAN_POINT('Ctrl Pts',(6.76686438025181,0.042842260436053,32.6990549111171));
#16746=CARTESIAN_POINT('Ctrl Pts',(6.76570397139435,0.226126925720858,32.7076899994032));
#16747=CARTESIAN_POINT('Ctrl Pts',(6.7570936109133,0.409219677908722,32.7163250876894));
#16748=CARTESIAN_POINT('Ctrl Pts',(6.74109815138213,0.591510535351992,32.7249601759755));
#16749=CARTESIAN_POINT('Ctrl Pts',(6.72507893538356,0.774072131301086,32.7336080891007));
#16750=CARTESIAN_POINT('Ctrl Pts',(6.7016527364256,0.955829149535095,32.7422560022258));
#16751=CARTESIAN_POINT('Ctrl Pts',(6.67093585820488,1.13617946457256,32.7509039153509));
#16752=CARTESIAN_POINT('Ctrl Pts',(6.66748989207677,1.15641202441624,32.7518740795549));
#16753=CARTESIAN_POINT('Ctrl Pts',(6.66395222187037,1.17662689398922,32.7528442437589));
#16754=CARTESIAN_POINT('Ctrl Pts',(6.66032305121468,1.19682323400673,32.7538144079629));
#16755=CARTESIAN_POINT('Ctrl Pts',(6.62955477662437,1.3680487271933,32.762039504399));
#16756=CARTESIAN_POINT('Ctrl Pts',(6.59213884052978,1.53831261615814,32.7702646008351));
#16757=CARTESIAN_POINT('Ctrl Pts',(6.54814725973299,1.70706076776762,32.7784896972711));
#16758=CARTESIAN_POINT('Ctrl Pts',(6.504202434922,1.87562956719112,32.7867060517506));
#16759=CARTESIAN_POINT('Ctrl Pts',(6.45369597298111,2.04268549338548,32.79492240623));
#16760=CARTESIAN_POINT('Ctrl Pts',(6.39675125827712,2.20768257223046,32.8031387607094));
#16761=CARTESIAN_POINT('Ctrl Pts',(6.33985566006461,2.37253733624149,32.8113480283414));
#16762=CARTESIAN_POINT('Ctrl Pts',(6.27653298579924,2.53533645288026,32.8195572959734));
#16763=CARTESIAN_POINT('Ctrl Pts',(6.20695699571139,2.69554704158349,32.8277665636055));
#16764=CARTESIAN_POINT('Ctrl Pts',(6.1374270842959,2.85565152628134,32.8359703944172));
#16765=CARTESIAN_POINT('Ctrl Pts',(6.06165224929661,3.01317057045485,32.8441742252289));
#16766=CARTESIAN_POINT('Ctrl Pts',(5.97985515367365,3.16758920017775,32.8523780560406));
#16767=CARTESIAN_POINT('Ctrl Pts',(5.89809132361558,3.32194503032434,32.8605785504862));
#16768=CARTESIAN_POINT('Ctrl Pts',(5.81031027763882,3.47320264082487,32.8687790449317));
#16769=CARTESIAN_POINT('Ctrl Pts',(5.71678168752888,3.62086952777016,32.8769795393772));
#16770=CARTESIAN_POINT('Ctrl Pts',(5.623272236074,3.76850619779878,32.8851783557643));
#16771=CARTESIAN_POINT('Ctrl Pts',(5.52401777391962,3.9125533046984,32.8933771721514));
#16772=CARTESIAN_POINT('Ctrl Pts',(5.41933261281328,4.05254525350408,32.9015759885386));
#16773=CARTESIAN_POINT('Ctrl Pts',(5.31464988302334,4.19253395099201,32.9097746145079));
#16774=CARTESIAN_POINT('Ctrl Pts',(5.20453692011565,4.32846739096257,32.9179732404773));
#16775=CARTESIAN_POINT('Ctrl Pts',(5.08934985901588,4.45991109917395,32.9261718664466));
#16776=CARTESIAN_POINT('Ctrl Pts',(4.97414457798132,4.59137559874654,32.9343717892494));
#16777=CARTESIAN_POINT('Ctrl Pts',(4.85386383666108,4.71834868284553,32.9425717120522));
#16778=CARTESIAN_POINT('Ctrl Pts',(4.72890237018331,4.84043090780921,32.9507716348549));
#16779=CARTESIAN_POINT('Ctrl Pts',(4.60383805510605,4.9626136116342,32.9589783065428));
#16780=CARTESIAN_POINT('Ctrl Pts',(4.47408557458634,5.0798971630359,32.9671849782306));
#16781=CARTESIAN_POINT('Ctrl Pts',(4.34007529857162,5.19192020380981,32.9753916499185));
#16782=CARTESIAN_POINT('Ctrl Pts',(4.20600842139092,5.3039905591249,32.983601787812));
#16783=CARTESIAN_POINT('Ctrl Pts',(4.06768044618244,5.41079575412562,32.9918119257056));
#16784=CARTESIAN_POINT('Ctrl Pts',(3.92555273277976,5.51201639530992,33.0000220635992));
#16785=CARTESIAN_POINT('Ctrl Pts',(3.78324764619229,5.61336335828653,33.0082424476177));
#16786=CARTESIAN_POINT('Ctrl Pts',(3.63713364440716,5.70911164252225,33.0164628316361));
#16787=CARTESIAN_POINT('Ctrl Pts',(3.4876997688326,5.79898605986297,33.0246832156546));
#16788=CARTESIAN_POINT('Ctrl Pts',(3.3604923451832,5.87549276249613,33.0316809186077));
#16789=CARTESIAN_POINT('Ctrl Pts',(3.2308797291331,5.94774369719842,33.0386786215608));
#16790=CARTESIAN_POINT('Ctrl Pts',(3.09917575053263,6.01559628526637,33.0456763245139));
#16791=CARTESIAN_POINT('Ctrl Pts',(3.09917575053259,6.01559628526639,31.0457515827422));
#16792=CARTESIAN_POINT('Ctrl Pts',(2.93382384459264,6.1007839529376,31.0545010306546));
#16793=CARTESIAN_POINT('Ctrl Pts',(2.76495772122983,6.1791501026705,31.063250478567));
#16794=CARTESIAN_POINT('Ctrl Pts',(2.5931509331671,6.25042856433178,31.0719999264794));
#16795=CARTESIAN_POINT('Ctrl Pts',(2.42134553245611,6.32170645041454,31.0807493037394));
#16796=CARTESIAN_POINT('Ctrl Pts',(2.24659977927579,6.38589665313461,31.0894986809994));
#16797=CARTESIAN_POINT('Ctrl Pts',(2.06950718689903,6.4427811543908,31.0982480582594));
#16798=CARTESIAN_POINT('Ctrl Pts',(1.89241596572849,6.49966521519727,31.1069973677741));
#16799=CARTESIAN_POINT('Ctrl Pts',(1.7129782145719,6.54924360009548,31.1157466772887));
#16800=CARTESIAN_POINT('Ctrl Pts',(1.53180337335841,6.59134792173557,31.1244959868034));
#16801=CARTESIAN_POINT('Ctrl Pts',(1.35062987477784,6.63345193135304,31.1332452314795));
#16802=CARTESIAN_POINT('Ctrl Pts',(1.16771959102958,6.66808192368237,31.1419944761556));
#16803=CARTESIAN_POINT('Ctrl Pts',(0.98369374690696,6.69512028363167,31.1507437208317));
#16804=CARTESIAN_POINT('Ctrl Pts',(0.799669205419936,6.72215845218866,31.1594929035759));
#16805=CARTESIAN_POINT('Ctrl Pts',(0.61452940287349,6.74160505424579,31.1682420863201));
#16806=CARTESIAN_POINT('Ctrl Pts',(0.42890312736321,6.75339404354122,31.1769912690643));
#16807=CARTESIAN_POINT('Ctrl Pts',(0.243278104163749,6.76518295330331,31.1857403927829));
#16808=CARTESIAN_POINT('Ctrl Pts',(0.0571669005388933,6.76931433552276,
31.1944895165015));
#16809=CARTESIAN_POINT('Ctrl Pts',(-0.12879840477783,6.76577415902472,31.2032386402201));
#16810=CARTESIAN_POINT('Ctrl Pts',(-0.314762517259429,6.7622340052344,31.2119877078193));
#16811=CARTESIAN_POINT('Ctrl Pts',(-0.500580446819854,6.75102239665086,
31.2207367754185));
#16812=CARTESIAN_POINT('Ctrl Pts',(-0.685621118842968,6.73217741012494,
31.2294858430177));
#16813=CARTESIAN_POINT('Ctrl Pts',(-0.870660665414657,6.71333253821769,
31.2382348574035));
#16814=CARTESIAN_POINT('Ctrl Pts',(-1.05492267885485,6.68685441030612,31.2469838717893));
#16815=CARTESIAN_POINT('Ctrl Pts',(-1.23778137635232,6.65283295028181,31.2557328861751));
#16816=CARTESIAN_POINT('Ctrl Pts',(-1.42999922978829,6.61707018861869,31.2649296965424));
#16817=CARTESIAN_POINT('Ctrl Pts',(-1.6206660123368,6.57297172934417,31.2741265069098));
#16818=CARTESIAN_POINT('Ctrl Pts',(-1.80906628500372,6.52070304311298,31.2833233172772));
#16819=CARTESIAN_POINT('Ctrl Pts',(-1.98831342545513,6.47097374915035,31.292073315015));
#16820=CARTESIAN_POINT('Ctrl Pts',(-2.16550875896686,6.41384933989534,31.3008233127528));
#16821=CARTESIAN_POINT('Ctrl Pts',(-2.34005036713995,6.34952386240482,31.3095733104905));
#16822=CARTESIAN_POINT('Ctrl Pts',(-2.51458843547073,6.28519968948602,31.3183231307714));
#16823=CARTESIAN_POINT('Ctrl Pts',(-2.6864726171804,6.21367483971106,31.3270729510523));
#16824=CARTESIAN_POINT('Ctrl Pts',(-2.85511905908717,6.13519226743851,31.3358227713331));
#16825=CARTESIAN_POINT('Ctrl Pts',(-3.02376230488868,6.05671118252945,31.3445724257917));
#16826=CARTESIAN_POINT('Ctrl Pts',(-3.18916767379886,5.97127275992643,31.3533220802502));
#16827=CARTESIAN_POINT('Ctrl Pts',(-3.35077334102767,5.87916720438008,31.3620717347087));
#16828=CARTESIAN_POINT('Ctrl Pts',(-3.51237616037355,5.78706327195651,31.3708212349772));
#16829=CARTESIAN_POINT('Ctrl Pts',(-3.67017916302293,5.68829258362303,31.3795707352456));
#16830=CARTESIAN_POINT('Ctrl Pts',(-3.82364636566462,5.58319061741042,31.3883202355141));
#16831=CARTESIAN_POINT('Ctrl Pts',(-3.97711106778789,5.47809036367708,31.3970695932225));
#16832=CARTESIAN_POINT('Ctrl Pts',(-4.1262398748191,5.36665920043238,31.4058189509309));
#16833=CARTESIAN_POINT('Ctrl Pts',(-4.27052628213905,5.24927559512355,31.4145683086394));
#16834=CARTESIAN_POINT('Ctrl Pts',(-4.41481053024949,5.13189374643061,31.4233175354159));
#16835=CARTESIAN_POINT('Ctrl Pts',(-4.55425230136496,5.00855981477383,31.4320667621924));
#16836=CARTESIAN_POINT('Ctrl Pts',(-4.6883780063051,4.87969268192113,31.4408159889689));
#16837=CARTESIAN_POINT('Ctrl Pts',(-4.82250188228876,4.75082730631829,31.4495650964398));
#16838=CARTESIAN_POINT('Ctrl Pts',(-4.95130963052966,4.61642907903527,31.4583142039106));
#16839=CARTESIAN_POINT('Ctrl Pts',(-5.07436379033383,4.47695444731671,31.4670633113815));
#16840=CARTESIAN_POINT('Ctrl Pts',(-5.19741643562795,4.33748153220597,31.4758123111712));
#16841=CARTESIAN_POINT('Ctrl Pts',(-5.31471544462739,4.19293255254631,31.4845613109609));
#16842=CARTESIAN_POINT('Ctrl Pts',(-5.42586245275572,4.04379841779678,31.4933103107506));
#16843=CARTESIAN_POINT('Ctrl Pts',(-5.53702160019097,3.89464799484422,31.5020602660928));
#16844=CARTESIAN_POINT('Ctrl Pts',(-5.64202723081196,3.74091164443933,31.5108102214349));
#16845=CARTESIAN_POINT('Ctrl Pts',(-5.74052265232913,3.5831115916332,31.5195601767771));
#16846=CARTESIAN_POINT('Ctrl Pts',(-5.83901427066876,3.42531763191855,31.5283097942596));
#16847=CARTESIAN_POINT('Ctrl Pts',(-5.93099603115709,3.26346052695669,31.537059411742));
#16848=CARTESIAN_POINT('Ctrl Pts',(-6.01615550622733,3.09809004467116,31.5458090292245));
#16849=CARTESIAN_POINT('Ctrl Pts',(-6.10131214578781,2.93272506863866,31.5545583553756));
#16850=CARTESIAN_POINT('Ctrl Pts',(-6.17964682328731,2.76384720416932,31.5633076815267));
#16851=CARTESIAN_POINT('Ctrl Pts',(-6.25089348288549,2.59203002791629,31.5720570076778));
#16852=CARTESIAN_POINT('Ctrl Pts',(-6.32213814889314,2.4202176593707,31.5808060890093));
#16853=CARTESIAN_POINT('Ctrl Pts',(-6.38629508412568,2.24546640831965,31.5895551703409));
#16854=CARTESIAN_POINT('Ctrl Pts',(-6.44314639819795,2.06836976660094,31.5983042516725));
#16855=CARTESIAN_POINT('Ctrl Pts',(-6.50000285283686,1.89125711158325,31.6070541241069));
#16856=CARTESIAN_POINT('Ctrl Pts',(-6.54955227673237,1.71179891440301,31.6158039965413));
#16857=CARTESIAN_POINT('Ctrl Pts',(-6.59162635926375,1.53060476278473,31.6245538689757));
#16858=CARTESIAN_POINT('Ctrl Pts',(-6.63369752055184,1.34942319164754,31.6333031338981));
#16859=CARTESIAN_POINT('Ctrl Pts',(-6.66829431424241,1.16650618642779,31.6420523988206));
#16860=CARTESIAN_POINT('Ctrl Pts',(-6.69529923745404,0.982474997619467,
31.6508016637431));
#16861=CARTESIAN_POINT('Ctrl Pts',(-6.72230554731433,0.798434359178603,
31.6595513779228));
#16862=CARTESIAN_POINT('Ctrl Pts',(-6.74171916496696,0.613279706241152,
31.6683010921025));
#16863=CARTESIAN_POINT('Ctrl Pts',(-6.7534741481727,0.427639953656142,31.6770508062822));
#16864=CARTESIAN_POINT('Ctrl Pts',(-6.76248837758744,0.28528336419895,31.6837604654582));
#16865=CARTESIAN_POINT('Ctrl Pts',(-6.76699999999998,0.142641701105103,
31.6904701246341));
#16866=CARTESIAN_POINT('Ctrl Pts',(-6.767,1.1656404461135E-12,31.69717978381));
#16867=CARTESIAN_POINT('',(-6.76699987500998,-0.00130062097133924,31.3028202162256));
#16868=CARTESIAN_POINT('Ctrl Pts',(3.09917575053255,6.01559628526641,30.6514573492524));
#16869=CARTESIAN_POINT('Ctrl Pts',(2.9437882613957,6.09565038388479,30.6596576710026));
#16870=CARTESIAN_POINT('Ctrl Pts',(2.78526378870031,6.16969705802948,30.6678579927529));
#16871=CARTESIAN_POINT('Ctrl Pts',(2.62410961849097,6.23749450582068,30.6760583145031));
#16872=CARTESIAN_POINT('Ctrl Pts',(2.46295499662551,6.30529214362329,30.6842586592359));
#16873=CARTESIAN_POINT('Ctrl Pts',(2.29917099269971,6.36684038095351,30.6924590039686));
#16874=CARTESIAN_POINT('Ctrl Pts',(2.13328512866462,6.42194546534136,30.7006593487014));
#16875=CARTESIAN_POINT('Ctrl Pts',(1.96736873792929,6.47706069029423,30.7088612024805));
#16876=CARTESIAN_POINT('Ctrl Pts',(1.79935005669109,6.52573028780835,30.7170630562597));
#16877=CARTESIAN_POINT('Ctrl Pts',(1.62977208218026,6.56781028655258,30.7252649100388));
#16878=CARTESIAN_POINT('Ctrl Pts',(1.4546507002461,6.61126585649397,30.7337348777476));
#16879=CARTESIAN_POINT('Ctrl Pts',(1.27786675017466,6.64769359432657,30.7422048454564));
#16880=CARTESIAN_POINT('Ctrl Pts',(1.10002932849864,6.67699217286068,30.7506748131651));
#16881=CARTESIAN_POINT('Ctrl Pts',(0.927584372820258,6.70540234676637,30.7588879507172));
#16882=CARTESIAN_POINT('Ctrl Pts',(0.754149264606598,6.72710940622123,30.7671010882693));
#16883=CARTESIAN_POINT('Ctrl Pts',(0.580283964397827,6.74207382936903,30.7753142258214));
#16884=CARTESIAN_POINT('Ctrl Pts',(0.398263342545787,6.75774017339368,30.7839126086085));
#16885=CARTESIAN_POINT('Ctrl Pts',(0.215771653946936,6.76601607239216,30.7925109913956));
#16886=CARTESIAN_POINT('Ctrl Pts',(0.0334502721502293,6.76691732469764,
30.8011093741828));
#16887=CARTESIAN_POINT('Ctrl Pts',(-0.148871109646478,6.76781857700313,
30.8097077569699));
#16888=CARTESIAN_POINT('Ctrl Pts',(-0.331021742430141,6.76134525818256,
30.818306139757));
#16889=CARTESIAN_POINT('Ctrl Pts',(-0.512368023175418,6.74757497244953,
30.8269045225441));
#16890=CARTESIAN_POINT('Ctrl Pts',(-0.694717879583281,6.7337284815494,30.835550489035));
#16891=CARTESIAN_POINT('Ctrl Pts',(-0.876668532959975,6.71247347993989,
30.8441964555258));
#16892=CARTESIAN_POINT('Ctrl Pts',(-1.05760834483217,6.68384272622728,30.8528424220167));
#16893=CARTESIAN_POINT('Ctrl Pts',(-1.23831671008625,6.65524859514102,30.861477329141));
#16894=CARTESIAN_POINT('Ctrl Pts',(-1.41801651240011,6.61929757251252,30.8701122362654));
#16895=CARTESIAN_POINT('Ctrl Pts',(-1.59610054872383,6.57607421174393,30.8787471433897));
#16896=CARTESIAN_POINT('Ctrl Pts',(-1.78009683132037,6.53141587028375,30.8876687224612));
#16897=CARTESIAN_POINT('Ctrl Pts',(-1.96236789808547,6.47899401621822,30.8965903015328));
#16898=CARTESIAN_POINT('Ctrl Pts',(-2.14225159143541,6.41895997175496,30.9055118806043));
#16899=CARTESIAN_POINT('Ctrl Pts',(-2.31587434137413,6.36101544273433,30.91412293958));
#16900=CARTESIAN_POINT('Ctrl Pts',(-2.48727276428476,6.29597975581458,30.9227339985557));
#16901=CARTESIAN_POINT('Ctrl Pts',(-2.65586293018433,6.22404057635173,30.9313450575313));
#16902=CARTESIAN_POINT('Ctrl Pts',(-2.82429410777394,6.15216923885641,30.9399479958808));
#16903=CARTESIAN_POINT('Ctrl Pts',(-2.98992202883562,6.073407507968,30.9485509342303));
#16904=CARTESIAN_POINT('Ctrl Pts',(-3.15218016280069,5.98799208593714,30.9571538725798));
#16905=CARTESIAN_POINT('Ctrl Pts',(-3.31425660519236,5.90267230941904,30.9657471776285));
#16906=CARTESIAN_POINT('Ctrl Pts',(-3.47297051900245,5.81071384723926,30.9743404826773));
#16907=CARTESIAN_POINT('Ctrl Pts',(-3.62777732434809,5.71240060613276,30.982933787726));
#16908=CARTESIAN_POINT('Ctrl Pts',(-3.64502533639689,5.70144690184711,30.9838912225667));
#16909=CARTESIAN_POINT('Ctrl Pts',(-3.66222487020964,5.69041435984547,30.9848486574074));
#16910=CARTESIAN_POINT('Ctrl Pts',(-3.67937519039829,5.6793034087185,30.9858060922482));
#16911=CARTESIAN_POINT('Ctrl Pts',(-3.83334910897148,5.57955036240354,30.9944018497958));
#16912=CARTESIAN_POINT('Ctrl Pts',(-3.9831736433357,5.47359055720332,31.0029976073434));
#16913=CARTESIAN_POINT('Ctrl Pts',(-4.12836292280519,5.36180087075298,31.0115933648909));
#16914=CARTESIAN_POINT('Ctrl Pts',(-4.27368766880941,5.24990688072391,31.0201971425726));
#16915=CARTESIAN_POINT('Ctrl Pts',(-4.41436828545345,5.13217233830758,31.0288009202543));
#16916=CARTESIAN_POINT('Ctrl Pts',(-4.54995293253852,5.00901360665791,31.037404697936));
#16917=CARTESIAN_POINT('Ctrl Pts',(-4.69086617481371,4.88101462916037,31.046346611604));
#16918=CARTESIAN_POINT('Ctrl Pts',(-4.82627452527868,4.74715675270992,31.0552885252719));
#16919=CARTESIAN_POINT('Ctrl Pts',(-4.95571483057532,4.60794743004039,31.0642304389399));
#16920=CARTESIAN_POINT('Ctrl Pts',(-5.08059947440093,4.47363759015746,31.0728576412706));
#16921=CARTESIAN_POINT('Ctrl Pts',(-5.19992884907543,4.33434683021309,31.0814848436014));
#16922=CARTESIAN_POINT('Ctrl Pts',(-5.31332949183721,4.19056305419367,31.0901120459321));
#16923=CARTESIAN_POINT('Ctrl Pts',(-5.42683813135508,4.04664234613391,31.0987474643527));
#16924=CARTESIAN_POINT('Ctrl Pts',(-5.53440658728367,3.89822032588502,31.1073828827732));
#16925=CARTESIAN_POINT('Ctrl Pts',(-5.63570461907915,3.74581398984119,31.1160183011937));
#16926=CARTESIAN_POINT('Ctrl Pts',(-5.73715230428661,3.59318249514627,31.1246664772149));
#16927=CARTESIAN_POINT('Ctrl Pts',(-5.83231089144553,3.43655518024921,31.133314653236));
#16928=CARTESIAN_POINT('Ctrl Pts',(-5.9208952358588,3.27647502752342,31.1419628292572));
#16929=CARTESIAN_POINT('Ctrl Pts',(-5.93026712361037,3.25953915434473,31.1428777734887));
#16930=CARTESIAN_POINT('Ctrl Pts',(-5.93956547085843,3.2425646536331,31.1437927177202));
#16931=CARTESIAN_POINT('Ctrl Pts',(-5.94878997126802,3.22555218183509,31.1447076619518));
#16932=CARTESIAN_POINT('Ctrl Pts',(-6.03489620025897,3.0667490242332,31.1532482217672));
#16933=CARTESIAN_POINT('Ctrl Pts',(-6.11473540022817,2.90431951038833,31.1617887815826));
#16934=CARTESIAN_POINT('Ctrl Pts',(-6.18800286363856,2.73877884459498,31.170329341398));
#16935=CARTESIAN_POINT('Ctrl Pts',(-6.26116971371862,2.57346550477845,31.1788581730311));
#16936=CARTESIAN_POINT('Ctrl Pts',(-6.3277826876891,2.40504981867954,31.1873870046642));
#16937=CARTESIAN_POINT('Ctrl Pts',(-6.38758252318929,2.23407218089451,31.1959158362974));
#16938=CARTESIAN_POINT('Ctrl Pts',(-6.45004579098903,2.05547934886741,31.2048245346218));
#16939=CARTESIAN_POINT('Ctrl Pts',(-6.50507492820516,1.87409140196102,31.2137332329461));
#16940=CARTESIAN_POINT('Ctrl Pts',(-6.5524289823788,1.69055122101708,31.2226419312705));
#16941=CARTESIAN_POINT('Ctrl Pts',(-6.59763534842354,1.51533529181184,31.2311465859292));
#16942=CARTESIAN_POINT('Ctrl Pts',(-6.63584728569493,1.33815838867071,31.2396512405878));
#16943=CARTESIAN_POINT('Ctrl Pts',(-6.66690478959617,1.1595988644612,31.2481558952465));
#16944=CARTESIAN_POINT('Ctrl Pts',(-6.69793377371252,0.981203309617538,
31.2566527401687));
#16945=CARTESIAN_POINT('Ctrl Pts',(-6.72182136437854,0.801427977178822,
31.2651495850908));
#16946=CARTESIAN_POINT('Ctrl Pts',(-6.73845808253665,0.620863648393569,
31.273646430013));
#16947=CARTESIAN_POINT('Ctrl Pts',(-6.75507757981683,0.440486224034566,
31.2821344797432));
#16948=CARTESIAN_POINT('Ctrl Pts',(-6.76446114528484,0.259321749013042,
31.2906225294735));
#16949=CARTESIAN_POINT('Ctrl Pts',(-6.76655081321516,0.0779685332507414,
31.2991105792037));
#16950=CARTESIAN_POINT('Ctrl Pts',(-6.76685523765853,0.0515488562485993,
31.3003471248658));
#16951=CARTESIAN_POINT('Ctrl Pts',(-6.76700495406095,0.0251251850256775,
31.3015836705278));
#16952=CARTESIAN_POINT('Ctrl Pts',(-6.76699987501013,-0.00130062020750468,
31.3028202161899));
#16953=CARTESIAN_POINT('Ctrl Pts',(-6.76699987500998,-0.00130062097129432,
31.3028202162256));
#16954=CARTESIAN_POINT('Ctrl Pts',(-6.76696418572452,-0.186988377484985,
31.3115091241998));
#16955=CARTESIAN_POINT('Ctrl Pts',(-6.75928127931588,-0.372492585525971,
31.320198032174));
#16956=CARTESIAN_POINT('Ctrl Pts',(-6.74402186049804,-0.557187710852092,
31.3288869401482));
#16957=CARTESIAN_POINT('Ctrl Pts',(-6.72873714990478,-0.742188959739467,
31.3375902495824));
#16958=CARTESIAN_POINT('Ctrl Pts',(-6.70585086745089,-0.926378161231628,
31.3462935590165));
#16959=CARTESIAN_POINT('Ctrl Pts',(-6.67548509089492,-1.10913831474692,
31.3549968684507));
#16960=CARTESIAN_POINT('Ctrl Pts',(-6.64422548702367,-1.297278077674,31.3639563628598));
#16961=CARTESIAN_POINT('Ctrl Pts',(-6.60503944955329,-1.48390304693927,
31.3729158572688));
#16962=CARTESIAN_POINT('Ctrl Pts',(-6.55811497097053,-1.66835758383274,
31.3818753516779));
#16963=CARTESIAN_POINT('Ctrl Pts',(-6.51233849186315,-1.84829947150813,
31.3906156535633));
#16964=CARTESIAN_POINT('Ctrl Pts',(-6.45919792650325,-2.02617564230019,
31.3993559554488));
#16965=CARTESIAN_POINT('Ctrl Pts',(-6.3989168635405,-2.20139773178247,31.4080962573342));
#16966=CARTESIAN_POINT('Ctrl Pts',(-6.33636817438614,-2.38321124782446,
31.4171653480051));
#16967=CARTESIAN_POINT('Ctrl Pts',(-6.26613152823398,-2.56216680451879,
31.426234438676));
#16968=CARTESIAN_POINT('Ctrl Pts',(-6.18850929400993,-2.73763432875041,
31.4353035293469));
#16969=CARTESIAN_POINT('Ctrl Pts',(-6.11088705978587,-2.91310185298206,
31.4443726200178));
#16970=CARTESIAN_POINT('Ctrl Pts',(-6.02587944881343,-3.08508107139603,
31.4534417106886));
#16971=CARTESIAN_POINT('Ctrl Pts',(-5.93383941563804,-3.25297383780141,
31.4625108013595));
#16972=CARTESIAN_POINT('Ctrl Pts',(-5.85107161789943,-3.40395286347316,
31.4706662597663));
#16973=CARTESIAN_POINT('Ctrl Pts',(-5.76240285295694,-3.5520172041671,31.4788217181731));
#16974=CARTESIAN_POINT('Ctrl Pts',(-5.66806278834808,-3.69666785461499,
31.4869771765799));
#16975=CARTESIAN_POINT('Ctrl Pts',(-5.57383754799868,-3.84114244620722,
31.4951227087218));
#16976=CARTESIAN_POINT('Ctrl Pts',(-5.47395494562947,-3.98221131530862,
31.5032682408637));
#16977=CARTESIAN_POINT('Ctrl Pts',(-5.36869131702243,-4.11939832287775,
31.5114137730056));
#16978=CARTESIAN_POINT('Ctrl Pts',(-5.26353367325877,-4.25644720350119,
31.5195511038061));
#16979=CARTESIAN_POINT('Ctrl Pts',(-5.15300601015973,-4.38962171583212,
31.5276884346067));
#16980=CARTESIAN_POINT('Ctrl Pts',(-5.03742889329539,-4.51847309884576,
31.5358257654072));
#16981=CARTESIAN_POINT('Ctrl Pts',(-4.9219438565367,-4.64722182616697,31.5439566132092));
#16982=CARTESIAN_POINT('Ctrl Pts',(-4.80141761900865,-4.77165401124391,
31.5520874610112));
#16983=CARTESIAN_POINT('Ctrl Pts',(-4.67621209563142,-4.89135251609107,
31.5602183088133));
#16984=CARTESIAN_POINT('Ctrl Pts',(-4.55108002170852,-5.01098080207225,
31.568344386807));
#16985=CARTESIAN_POINT('Ctrl Pts',(-4.4212743921104,-5.12588068607262,31.5764704648008));
#16986=CARTESIAN_POINT('Ctrl Pts',(-4.28719517807036,-5.23567058791233,
31.5845965427946));
#16987=CARTESIAN_POINT('Ctrl Pts',(-4.15264054362595,-5.34584978469161,
31.5927514343768));
#16988=CARTESIAN_POINT('Ctrl Pts',(-4.01378221527217,-5.45088242198391,
31.600906325959));
#16989=CARTESIAN_POINT('Ctrl Pts',(-3.87105974598709,-5.55042209593094,
31.6090612175412));
#16990=CARTESIAN_POINT('Ctrl Pts',(-3.72889384443081,-5.64957359995257,
31.6171843078975));
#16991=CARTESIAN_POINT('Ctrl Pts',(-3.58289419735056,-5.74327470834417,
31.6253073982538));
#16992=CARTESIAN_POINT('Ctrl Pts',(-3.43352588972085,-5.83122533989355,
31.6334304886101));
#16993=CARTESIAN_POINT('Ctrl Pts',(-3.28414585300972,-5.91918287772804,
31.6415542168285));
#16994=CARTESIAN_POINT('Ctrl Pts',(-3.13139694407138,-6.00138885361899,
31.649677945047));
#16995=CARTESIAN_POINT('Ctrl Pts',(-2.97577035579683,-6.07758832017774,
31.6578016732654));
#16996=CARTESIAN_POINT('Ctrl Pts',(-2.82010193923835,-6.15380826712455,
31.6659275849257));
#16997=CARTESIAN_POINT('Ctrl Pts',(-2.6615546316913,-6.22401832938343,31.674053496586));
#16998=CARTESIAN_POINT('Ctrl Pts',(-2.50064113288644,-6.28801104678709,
31.6821794082463));
#16999=CARTESIAN_POINT('Ctrl Pts',(-2.33869857552963,-6.35241300427063,
31.6903572859564));
#17000=CARTESIAN_POINT('Ctrl Pts',(-2.17435980680415,-6.41051768095202,
31.6985351636665));
#17001=CARTESIAN_POINT('Ctrl Pts',(-2.00816373523178,-6.46216429785718,
31.7067130413765));
#17002=CARTESIAN_POINT('Ctrl Pts',(-1.84276088146323,-6.51356441666134,
31.71485188785));
#17003=CARTESIAN_POINT('Ctrl Pts',(-1.6755187842758,-6.55856795078435,31.7229907343234));
#17004=CARTESIAN_POINT('Ctrl Pts',(-1.50697937842296,-6.5970676935293,31.7311295807969));
#17005=CARTESIAN_POINT('Ctrl Pts',(-1.33722758305271,-6.63584438447096,
31.7393269741253));
#17006=CARTESIAN_POINT('Ctrl Pts',(-1.1661601154976,-6.66802329127322,31.7475243674537));
#17007=CARTESIAN_POINT('Ctrl Pts',(-0.994336027983862,-6.69354800262561,
31.7557217607821));
#17008=CARTESIAN_POINT('Ctrl Pts',(-0.822511940470152,-6.71907271397799,
31.7639191541104));
#17009=CARTESIAN_POINT('Ctrl Pts',(-0.649931609667629,-6.73794325016948,
31.7721165474388));
#17010=CARTESIAN_POINT('Ctrl Pts',(-0.477153788763507,-6.75015653610112,
31.7803139407672));
#17011=CARTESIAN_POINT('Ctrl Pts',(-0.303768608059589,-6.76241275496743,
31.7885401501042));
#17012=CARTESIAN_POINT('Ctrl Pts',(-0.129668529657173,-6.76800143151726,
31.7967663594412));
#17013=CARTESIAN_POINT('Ctrl Pts',(0.0445927278613814,-6.76685307130441,
31.8049925687782));
#17014=CARTESIAN_POINT('Ctrl Pts',(0.218658210322328,-6.76570600122506,
31.8132095363214));
#17015=CARTESIAN_POINT('Ctrl Pts',(0.392884155952847,-6.75783696820683,
31.8214265038646));
#17016=CARTESIAN_POINT('Ctrl Pts',(0.566711752314562,-6.74322821724051,
31.8296434714077));
#17017=CARTESIAN_POINT('Ctrl Pts',(0.740378949409586,-6.72863294648671,
31.8378528567511));
#17018=CARTESIAN_POINT('Ctrl Pts',(0.913648174147453,-6.70731037313801,
31.8460622420945));
#17019=CARTESIAN_POINT('Ctrl Pts',(1.08596054741427,-6.67929477485907,31.8542716274379));
#17020=CARTESIAN_POINT('Ctrl Pts',(1.25814849295863,-6.65129940679936,31.8624750847385));
#17021=CARTESIAN_POINT('Ctrl Pts',(1.42938061072744,-6.61662069777632,31.8706785420391));
#17022=CARTESIAN_POINT('Ctrl Pts',(1.59910298711738,-6.57534475420052,31.8788819993397));
#17023=CARTESIAN_POINT('Ctrl Pts',(1.76873685192792,-6.53409033636007,31.8870811784716));
#17024=CARTESIAN_POINT('Ctrl Pts',(1.93686219623547,-6.48624562262405,31.8952803576035));
#17025=CARTESIAN_POINT('Ctrl Pts',(2.10293505979891,-6.43194784915647,31.9034795367353));
#17026=CARTESIAN_POINT('Ctrl Pts',(2.26897663165553,-6.37766030655968,31.9116771709651));
#17027=CARTESIAN_POINT('Ctrl Pts',(2.4329661506371,-6.31692223159436,31.9198748051949));
#17028=CARTESIAN_POINT('Ctrl Pts',(2.59437429525009,-6.24992088079086,31.9280724394248));
#17029=CARTESIAN_POINT('Ctrl Pts',(2.75577078924634,-6.18292436621828,31.9362694819404));
#17030=CARTESIAN_POINT('Ctrl Pts',(2.91458594834338,-6.10966561286604,31.9444665244559));
#17031=CARTESIAN_POINT('Ctrl Pts',(3.0703099905606,-6.03038021702312,31.9526635669715));
#17032=CARTESIAN_POINT('Ctrl Pts',(3.22605109502979,-5.95108613409898,31.9608615076144));
#17033=CARTESIAN_POINT('Ctrl Pts',(3.37870008815778,-5.86576425590392,31.9690594482572));
#17034=CARTESIAN_POINT('Ctrl Pts',(3.5277713323129,-5.77469639261765,31.9772573889));
#17035=CARTESIAN_POINT('Ctrl Pts',(3.67688600334077,-5.68360199978483,31.985457717736));
#17036=CARTESIAN_POINT('Ctrl Pts',(3.82242054334053,-5.58675847459734,31.993658046572));
#17037=CARTESIAN_POINT('Ctrl Pts',(3.96391782853191,-5.48449126616561,32.001858375408));
#17038=CARTESIAN_POINT('Ctrl Pts',(4.105562557566,-5.38211749264909,32.0100672491994));
#17039=CARTESIAN_POINT('Ctrl Pts',(4.24316133590766,-5.27430895519029,32.0182761229908));
#17040=CARTESIAN_POINT('Ctrl Pts',(4.37628892899677,-5.16143237967334,32.0264849967823));
#17041=CARTESIAN_POINT('Ctrl Pts',(4.50948797019639,-5.04849522454359,32.0346982761857));
#17042=CARTESIAN_POINT('Ctrl Pts',(4.63821077825436,-4.93048485117022,32.0429115555891));
#17043=CARTESIAN_POINT('Ctrl Pts',(4.76206871192509,-4.80780517314337,32.0511248349925));
#17044=CARTESIAN_POINT('Ctrl Pts',(4.8861078072909,-4.68494605680551,32.059350127608));
#17045=CARTESIAN_POINT('Ctrl Pts',(5.00526756326862,-4.55740424939333,32.0675754202234));
#17046=CARTESIAN_POINT('Ctrl Pts',(5.1191985549309,-4.4256180534693,32.0758007128389));
#17047=CARTESIAN_POINT('Ctrl Pts',(5.22223545099334,-4.30643326999845,32.0832395019509));
#17048=CARTESIAN_POINT('Ctrl Pts',(5.32099614197417,-4.18377755902988,32.0906782910629));
#17049=CARTESIAN_POINT('Ctrl Pts',(5.4152530290108,-4.05799502609224,32.098117080175));
#17050=CARTESIAN_POINT('Ctrl Pts',(5.51948721128105,-3.91889814015816,32.1063432811938));
#17051=CARTESIAN_POINT('Ctrl Pts',(5.61850434854473,-3.77558819810754,32.1145694822127));
#17052=CARTESIAN_POINT('Ctrl Pts',(5.71194605337206,-3.62849297689377,32.1227956832315));
#17053=CARTESIAN_POINT('Ctrl Pts',(5.80528279613786,-3.48156298615912,32.1310126438473));
#17054=CARTESIAN_POINT('Ctrl Pts',(5.89305638689484,-3.33085648304833,32.139229604463));
#17055=CARTESIAN_POINT('Ctrl Pts',(5.97494916800274,-3.17683355556809,32.1474465650788));
#17056=CARTESIAN_POINT('Ctrl Pts',(6.05676639636252,-3.02295272675988,32.1556559448804));
#17057=CARTESIAN_POINT('Ctrl Pts',(6.1327134529015,-2.86576188170144,32.163865324682));
#17058=CARTESIAN_POINT('Ctrl Pts',(6.20251637967704,-2.70574935273724,32.1720747044836));
#17059=CARTESIAN_POINT('Ctrl Pts',(6.27226891308459,-2.54585234285841,32.180278157624));
#17060=CARTESIAN_POINT('Ctrl Pts',(6.33588600902273,-2.38313803397643,32.1884816107644));
#17061=CARTESIAN_POINT('Ctrl Pts',(6.39313996397682,-2.21811866251615,32.1966850639048));
#17062=CARTESIAN_POINT('Ctrl Pts',(6.45036407014013,-2.05318532229507,32.2048842402549));
#17063=CARTESIAN_POINT('Ctrl Pts',(6.50123152681869,-1.88594965155674,32.213083416605));
#17064=CARTESIAN_POINT('Ctrl Pts',(6.5455629995142,-1.71694321961754,32.2212825929552));
#17065=CARTESIAN_POINT('Ctrl Pts',(6.58988613057413,-1.54796858878896,32.2294802265066));
#17066=CARTESIAN_POINT('Ctrl Pts',(6.6276756304514,-1.37722420541406,32.2376778600579));
#17067=CARTESIAN_POINT('Ctrl Pts',(6.65880213940589,-1.20525643256677,32.2458754936093));
#17068=CARTESIAN_POINT('Ctrl Pts',(6.68992640648781,-1.03330104561965,32.2540725367299));
#17069=CARTESIAN_POINT('Ctrl Pts',(6.71438857363848,-0.860122797470459,
32.2622695798505));
#17070=CARTESIAN_POINT('Ctrl Pts',(6.73211049824738,-0.686277815019089,
32.270466622971));
#17071=CARTESIAN_POINT('Ctrl Pts',(6.74983436737299,-0.512413757637681,
32.2786645655022));
#17072=CARTESIAN_POINT('Ctrl Pts',(6.76081648414606,-0.337883177110012,
32.2868625080334));
#17073=CARTESIAN_POINT('Ctrl Pts',(6.76503063082165,-0.163246941915793,
32.2950604505646));
#17074=CARTESIAN_POINT('Ctrl Pts',(6.76924600580636,0.0114401949902511,
32.3032607825731));
#17075=CARTESIAN_POINT('Ctrl Pts',(6.7666894727042,0.186232689418164,32.3114611145815));
#17076=CARTESIAN_POINT('Ctrl Pts',(6.75738694139935,0.360569999036963,32.3196614465899));
#17077=CARTESIAN_POINT('Ctrl Pts',(6.74807471434261,0.53508901525204,32.3278703255607));
#17078=CARTESIAN_POINT('Ctrl Pts',(6.73200246103901,0.709151540184308,32.3360792045314));
#17079=CARTESIAN_POINT('Ctrl Pts',(6.70924806209167,0.88220147433519,32.3442880835022));
#17080=CARTESIAN_POINT('Ctrl Pts',(6.68648144805519,1.05534430570459,32.3525013691896));
#17081=CARTESIAN_POINT('Ctrl Pts',(6.6570255977479,1.22747310944518,32.360714654877));
#17082=CARTESIAN_POINT('Ctrl Pts',(6.6210094738311,1.39804239829802,32.3689279405644));
#17083=CARTESIAN_POINT('Ctrl Pts',(6.5849406627639,1.56886120899821,32.3771532412764));
#17084=CARTESIAN_POINT('Ctrl Pts',(6.5422924869989,1.73811559783988,32.3853785419886));
#17085=CARTESIAN_POINT('Ctrl Pts',(6.49324405981116,1.90527441061046,32.3936038427006));
#17086=CARTESIAN_POINT('Ctrl Pts',(6.44888567402466,2.05644939275844,32.4010426349946));
#17087=CARTESIAN_POINT('Ctrl Pts',(6.39929321471691,2.20591044020288,32.4084814272886));
#17088=CARTESIAN_POINT('Ctrl Pts',(6.3446326166538,2.35327983029913,32.4159202195826));
#17089=CARTESIAN_POINT('Ctrl Pts',(6.28471566292562,2.51482078009176,32.4240743523486));
#17090=CARTESIAN_POINT('Ctrl Pts',(6.21853144286844,2.67432463303835,32.4322284851145));
#17091=CARTESIAN_POINT('Ctrl Pts',(6.14623714389316,2.83126437674549,32.4403826178805));
#17092=CARTESIAN_POINT('Ctrl Pts',(6.07402941856448,2.98801618245334,32.4485269859344));
#17093=CARTESIAN_POINT('Ctrl Pts',(5.99572633284242,3.14220966305313,32.4566713539884));
#17094=CARTESIAN_POINT('Ctrl Pts',(5.91153450832306,3.29333398805916,32.4648157220424));
#17095=CARTESIAN_POINT('Ctrl Pts',(5.82744327266781,3.44427775605412,32.4729503595466));
#17096=CARTESIAN_POINT('Ctrl Pts',(5.73747749404295,3.59215935775243,32.4810849970509));
#17097=CARTESIAN_POINT('Ctrl Pts',(5.64189126552677,3.73648925436334,32.4892196345552));
#17098=CARTESIAN_POINT('Ctrl Pts',(5.5463704465614,3.88072038618511,32.497348705536));
#17099=CARTESIAN_POINT('Ctrl Pts',(5.44523703419817,4.02140434728218,32.5054777765168));
#17100=CARTESIAN_POINT('Ctrl Pts',(5.33879053080062,4.15807703971843,32.5136068474976));
#17101=CARTESIAN_POINT('Ctrl Pts',(5.23239661581678,4.2946822109129,32.521731902424));
#17102=CARTESIAN_POINT('Ctrl Pts',(5.12069505983306,4.42727977118434,32.5298569573504));
#17103=CARTESIAN_POINT('Ctrl Pts',(5.00402805947163,4.55543545448957,32.5379820122768));
#17104=CARTESIAN_POINT('Ctrl Pts',(4.88739650143855,4.68355220531352,32.5461045988885));
#17105=CARTESIAN_POINT('Ctrl Pts',(4.76580274928459,4.80722949669052,32.5542271855003));
#17106=CARTESIAN_POINT('Ctrl Pts',(4.63962854518207,4.92606698723553,32.5623497721121));
#17107=CARTESIAN_POINT('Ctrl Pts',(4.51344096484698,5.04491707621873,32.5704732198318));
#17108=CARTESIAN_POINT('Ctrl Pts',(4.38267222337509,5.15892608295491,32.5785966675515));
#17109=CARTESIAN_POINT('Ctrl Pts',(4.24774033827205,5.26773110728105,32.5867201152712));
#17110=CARTESIAN_POINT('Ctrl Pts',(4.11280270583172,5.37654076608757,32.5948439090039));
#17111=CARTESIAN_POINT('Ctrl Pts',(3.97370186490346,5.48014577588667,32.6029677027367));
#17112=CARTESIAN_POINT('Ctrl Pts',(3.83088789796103,5.57822435128382,32.6110914964694));
#17113=CARTESIAN_POINT('Ctrl Pts',(3.68799082433446,5.67636000082686,32.6192200176219));
#17114=CARTESIAN_POINT('Ctrl Pts',(3.54137661311616,5.76896258923199,32.6273485387743));
#17115=CARTESIAN_POINT('Ctrl Pts',(3.39152367184721,5.85575410884884,32.6354770599267));
#17116=CARTESIAN_POINT('Ctrl Pts',(3.29536362809119,5.91144788605024,32.6406931000196));
#17117=CARTESIAN_POINT('Ctrl Pts',(3.19787050428405,5.96474972359129,32.6459091401124));
#17118=CARTESIAN_POINT('Ctrl Pts',(3.0991757505326,6.01559628526638,32.6511251802053));
#17119=CARTESIAN_POINT('Origin',(0.,0.,-3.69717978381041));
#17120=CARTESIAN_POINT('',(3.09917575053259,6.01559628526639,35.0459310802154));
#17121=CARTESIAN_POINT('',(3.09917575053259,6.01559628526639,34.6514942595564));
#17122=CARTESIAN_POINT('',(3.09917575053259,6.01559628526639,-3.69717978381041));
#17123=CARTESIAN_POINT('',(-6.76699984329972,-0.00145629033198537,33.6971797837663));
#17124=CARTESIAN_POINT('Ctrl Pts',(-6.76699984329952,-0.00145629125626415,
33.69717978381));
#17125=CARTESIAN_POINT('Ctrl Pts',(-6.76698266837336,-0.081263625227222,
33.7009561167744));
#17126=CARTESIAN_POINT('Ctrl Pts',(-6.76555371680281,-0.161054131447447,
33.7047324497388));
#17127=CARTESIAN_POINT('Ctrl Pts',(-6.76271448371177,-0.240794127409707,
33.7085087827031));
#17128=CARTESIAN_POINT('Ctrl Pts',(-6.75653063770426,-0.414467735690516,
33.7167336310252));
#17129=CARTESIAN_POINT('Ctrl Pts',(-6.74364363212401,-0.588146728668887,
33.7249584793472));
#17130=CARTESIAN_POINT('Ctrl Pts',(-6.72404282540133,-0.761273329474309,
33.7331833276693));
#17131=CARTESIAN_POINT('Ctrl Pts',(-6.70446409353292,-0.934204951341491,
33.7413989129885));
#17132=CARTESIAN_POINT('Ctrl Pts',(-6.67818665685065,-1.10658506658277,
33.7496144983077));
#17133=CARTESIAN_POINT('Ctrl Pts',(-6.64525186112367,-1.27785629169811,
33.7578300836269));
#17134=CARTESIAN_POINT('Ctrl Pts',(-6.61234754002283,-1.44896903923858,
33.7660380670502));
#17135=CARTESIAN_POINT('Ctrl Pts',(-6.57279819509873,-1.61897458997166,
33.7742460504734));
#17136=CARTESIAN_POINT('Ctrl Pts',(-6.52669692064897,-1.78732098571891,
33.7824540338966));
#17137=CARTESIAN_POINT('Ctrl Pts',(-6.48062904411642,-1.95554542347145,
33.7906560710732));
#17138=CARTESIAN_POINT('Ctrl Pts',(-6.42801878661428,-2.12211275570558,
33.7988581082497));
#17139=CARTESIAN_POINT('Ctrl Pts',(-6.36901025685276,-2.28648143401699,
33.8070601454263));
#17140=CARTESIAN_POINT('Ctrl Pts',(-6.31003262619114,-2.45076404266638,
33.8152578877057));
#17141=CARTESIAN_POINT('Ctrl Pts',(-6.24466351869628,-2.61284995409234,
33.8234556299851));
#17142=CARTESIAN_POINT('Ctrl Pts',(-6.17309683537031,-2.77221291771412,
33.8316533722645));
#17143=CARTESIAN_POINT('Ctrl Pts',(-6.10154375926479,-2.93154558110572,
33.8398495558788));
#17144=CARTESIAN_POINT('Ctrl Pts',(-6.0237955956277,-3.08815599842659,33.8480457394932));
#17145=CARTESIAN_POINT('Ctrl Pts',(-5.94009443924441,-3.24153776051701,
33.8562419231075));
#17146=CARTESIAN_POINT('Ctrl Pts',(-5.85639944443407,-3.39490823156968,
33.8644375033684));
#17147=CARTESIAN_POINT('Ctrl Pts',(-5.76675250070972,-3.5450502053198,33.8726330836293));
#17148=CARTESIAN_POINT('Ctrl Pts',(-5.67144170697693,-3.69148181146307,
33.8808286638902));
#17149=CARTESIAN_POINT('Ctrl Pts',(-5.57612058877703,-3.83792927969542,
33.8890251319309));
#17150=CARTESIAN_POINT('Ctrl Pts',(-5.47513459401187,-3.9806652787704,33.8972215999717));
#17151=CARTESIAN_POINT('Ctrl Pts',(-5.36881522412025,-4.11923683335332,
33.9054180680124));
#17152=CARTESIAN_POINT('Ctrl Pts',(-5.26246499363265,-4.25784861015317,
33.9136169151858));
#17153=CARTESIAN_POINT('Ctrl Pts',(-5.15077852280994,-4.39229325009773,
33.9218157623592));
#17154=CARTESIAN_POINT('Ctrl Pts',(-5.03412769199013,-4.52215074723722,
33.9300146095326));
#17155=CARTESIAN_POINT('Ctrl Pts',(-4.91735494970878,-4.65214395808878,
33.9382220252985));
#17156=CARTESIAN_POINT('Ctrl Pts',(-4.79560772212199,-4.77754018102969,
33.9464294410645));
#17157=CARTESIAN_POINT('Ctrl Pts',(-4.66929556599789,-4.8979554833984,33.9546368568305));
#17158=CARTESIAN_POINT('Ctrl Pts',(-4.54291571100061,-5.01843532413408,
33.9628486714826));
#17159=CARTESIAN_POINT('Ctrl Pts',(-4.41196631888719,-5.13392868526123,
33.9710604861348));
#17160=CARTESIAN_POINT('Ctrl Pts',(-4.27689005332436,-5.24409195874511,
33.9792723007869));
#17161=CARTESIAN_POINT('Ctrl Pts',(-4.14161486742574,-5.35441746439659,
33.9874962085845));
#17162=CARTESIAN_POINT('Ctrl Pts',(-4.00220094912176,-5.45939697981976,
33.9957201163822));
#17163=CARTESIAN_POINT('Ctrl Pts',(-3.85912102143023,-5.55872952588587,
34.0039440241798));
#17164=CARTESIAN_POINT('Ctrl Pts',(-3.72691781068673,-5.65051096394738,
34.0115427631032));
#17165=CARTESIAN_POINT('Ctrl Pts',(-3.59158526791413,-5.7374717215886,34.0191415020265));
#17166=CARTESIAN_POINT('Ctrl Pts',(-3.45351406910012,-5.81940972732867,
34.0267402409499));
#17167=CARTESIAN_POINT('Ctrl Pts',(-3.3054084568843,-5.90730263046935,34.0348912231242));
#17168=CARTESIAN_POINT('Ctrl Pts',(-3.15371264648572,-5.98967591738706,
34.0430422052985));
#17169=CARTESIAN_POINT('Ctrl Pts',(-2.99887967364111,-6.06621873188086,
34.0511931874728));
#17170=CARTESIAN_POINT('Ctrl Pts',(-2.84422655364465,-6.14267263480149,
34.0593347015258));
#17171=CARTESIAN_POINT('Ctrl Pts',(-2.68644384953959,-6.21330938633918,
34.0674762155788));
#17172=CARTESIAN_POINT('Ctrl Pts',(-2.52601291824701,-6.27786171692633,
34.0756177296319));
#17173=CARTESIAN_POINT('Ctrl Pts',(-2.36573458179814,-6.3423526481766,34.0837514998349));
#17174=CARTESIAN_POINT('Ctrl Pts',(-2.20281336980553,-6.40077054443534,
34.091885270038));
#17175=CARTESIAN_POINT('Ctrl Pts',(-2.03775454890624,-6.45289434272807,
34.1000190402411));
#17176=CARTESIAN_POINT('Ctrl Pts',(-1.87281800942803,-6.50497952586474,
34.108146784659));
#17177=CARTESIAN_POINT('Ctrl Pts',(-1.70574736152882,-6.5507797859163,34.116274529077));
#17178=CARTESIAN_POINT('Ctrl Pts',(-1.53706712773142,-6.59012243018652,
34.124402273495));
#17179=CARTESIAN_POINT('Ctrl Pts',(-1.36847639447767,-6.62944419952687,
34.1325257053891));
#17180=CARTESIAN_POINT('Ctrl Pts',(-1.19827813151021,-6.66231509388206,
34.1406491372831));
#17181=CARTESIAN_POINT('Ctrl Pts',(-1.02701126863786,-6.6886124759991,34.1487725691772));
#17182=CARTESIAN_POINT('Ctrl Pts',(-0.854657956151481,-6.7150766783648,
34.156947532928));
#17183=CARTESIAN_POINT('Ctrl Pts',(-0.681222798994661,-6.73488357358447,
34.1651224966788));
#17184=CARTESIAN_POINT('Ctrl Pts',(-0.507265202436242,-6.74796050776806,
34.1732974604296));
#17185=CARTESIAN_POINT('Ctrl Pts',(-0.334443380121393,-6.7609520622653,
34.1814190496027));
#17186=CARTESIAN_POINT('Ctrl Pts',(-0.161106291187816,-6.76730127307965,
34.1895406387757));
#17187=CARTESIAN_POINT('Ctrl Pts',(0.0121930457427909,-6.7669890150373,
34.1976622279487));
#17188=CARTESIAN_POINT('Ctrl Pts',(0.185515261740115,-6.76667671577049,
34.2057848893381));
#17189=CARTESIAN_POINT('Ctrl Pts',(0.358799349785193,-6.75970119659649,
34.2139075507275));
#17190=CARTESIAN_POINT('Ctrl Pts',(0.531493081306014,-6.74609547105019,
34.2220302121168));
#17191=CARTESIAN_POINT('Ctrl Pts',(0.704242497935716,-6.73248535833649,
34.2301554926591));
#17192=CARTESIAN_POINT('Ctrl Pts',(0.876400814308157,-6.71224081074426,
34.2382807732013));
#17193=CARTESIAN_POINT('Ctrl Pts',(1.04742175089768,-6.68544663248062,34.2464060537436));
#17194=CARTESIAN_POINT('Ctrl Pts',(1.22030592510498,-6.65836053720451,34.2546198575314));
#17195=CARTESIAN_POINT('Ctrl Pts',(1.39202741182048,-6.62458132085763,34.2628336613191));
#17196=CARTESIAN_POINT('Ctrl Pts',(1.56203422165276,-6.58424924272963,34.2710474651069));
#17197=CARTESIAN_POINT('Ctrl Pts',(1.73049982037851,-6.54428279846548,34.2791868059621));
#17198=CARTESIAN_POINT('Ctrl Pts',(1.89728136921399,-6.49788197471459,34.2873261468172));
#17199=CARTESIAN_POINT('Ctrl Pts',(2.06185906664541,-6.44523282661628,34.2954654876724));
#17200=CARTESIAN_POINT('Ctrl Pts',(2.22869522791532,-6.39186118574427,34.3037165229265));
#17201=CARTESIAN_POINT('Ctrl Pts',(2.39326624427484,-6.33206862222528,34.3119675581806));
#17202=CARTESIAN_POINT('Ctrl Pts',(2.55505398101794,-6.26609831985458,34.3202185934347));
#17203=CARTESIAN_POINT('Ctrl Pts',(2.71684171776106,-6.20012801748387,34.3284696286888));
#17204=CARTESIAN_POINT('Ctrl Pts',(2.87584585302401,-6.1279801959522,34.3367206639428));
#17205=CARTESIAN_POINT('Ctrl Pts',(3.03157677142156,-6.04994473354734,34.3449716991969));
#17206=CARTESIAN_POINT('Ctrl Pts',(3.18694411369143,-5.97209145610316,34.3532034712278));
#17207=CARTESIAN_POINT('Ctrl Pts',(3.33953861418369,-5.88813511228987,34.3614352432586));
#17208=CARTESIAN_POINT('Ctrl Pts',(3.48884744795318,-5.79829565345806,34.3696670152895));
#17209=CARTESIAN_POINT('Ctrl Pts',(3.63797799205412,-5.7085634719181,34.3778889577619));
#17210=CARTESIAN_POINT('Ctrl Pts',(3.78383037786145,-5.61296234672479,34.3861109002343));
#17211=CARTESIAN_POINT('Ctrl Pts',(3.92591348474255,-5.51175945686281,34.3943328427067));
#17212=CARTESIAN_POINT('Ctrl Pts',(4.06785539779484,-5.41065713647611,34.4025466146966));
#17213=CARTESIAN_POINT('Ctrl Pts',(4.20603520160814,-5.30396434393153,34.4107603866865));
#17214=CARTESIAN_POINT('Ctrl Pts',(4.33998796628217,-5.19199320613249,34.4189741586764));
#17215=CARTESIAN_POINT('Ctrl Pts',(4.47383444544757,-5.08011091240742,34.4271814134068));
#17216=CARTESIAN_POINT('Ctrl Pts',(4.6034602921703,-4.962958844041,34.4353886681372));
#17217=CARTESIAN_POINT('Ctrl Pts',(4.72843100769114,-4.84089136477003,34.4435959228675));
#17218=CARTESIAN_POINT('Ctrl Pts',(4.85332758792063,-4.7188962985288,34.4517983088795));
#17219=CARTESIAN_POINT('Ctrl Pts',(4.97357428259048,-4.59199187995433,34.4600006948915));
#17220=CARTESIAN_POINT('Ctrl Pts',(5.08877097700547,-4.46057159381921,34.4682030809035));
#17221=CARTESIAN_POINT('Ctrl Pts',(5.20393328800127,-4.32919053345189,34.4764030187022));
#17222=CARTESIAN_POINT('Ctrl Pts',(5.31404836241997,-4.19329655699442,34.4846029565009));
#17223=CARTESIAN_POINT('Ctrl Pts',(5.41875399560152,-4.0533189037075,34.4928028942996));
#17224=CARTESIAN_POINT('Ctrl Pts',(5.5234449882331,-3.91336082290932,34.5010016855354));
#17225=CARTESIAN_POINT('Ctrl Pts',(5.62272783078984,-3.76932048893365,34.5092004767711));
#17226=CARTESIAN_POINT('Ctrl Pts',(5.71628156094439,-3.62165902812609,34.5173992680069));
#17227=CARTESIAN_POINT('Ctrl Pts',(5.80983918100523,-3.47399142764621,34.5255984001433));
#17228=CARTESIAN_POINT('Ctrl Pts',(5.89766702218114,-3.32270270312299,34.5337975322797));
#17229=CARTESIAN_POINT('Ctrl Pts',(5.97948826981045,-3.16828171588311,34.5419966644162));
#17230=CARTESIAN_POINT('Ctrl Pts',(6.061327762261,-3.01382629524862,34.5501976248271));
#17231=CARTESIAN_POINT('Ctrl Pts',(6.13715782573818,-2.85623753744992,34.558398585238));
#17232=CARTESIAN_POINT('Ctrl Pts',(6.20674826987113,-2.69602761752393,34.566599545649));
#17233=CARTESIAN_POINT('Ctrl Pts',(6.27640393700271,-2.53566754233571,34.574808192334));
#17234=CARTESIAN_POINT('Ctrl Pts',(6.33980815780448,-2.37268172594962,34.5830168390191));
#17235=CARTESIAN_POINT('Ctrl Pts',(6.39677911214155,-2.2076018641208,34.5912254857041));
#17236=CARTESIAN_POINT('Ctrl Pts',(6.45377726601229,-2.04244318852952,34.5994380514276));
#17237=CARTESIAN_POINT('Ctrl Pts',(6.50433592586619,-1.8751888170663,34.6076506171512));
#17238=CARTESIAN_POINT('Ctrl Pts',(6.54832361526619,-1.70638413897548,34.6158631828747));
#17239=CARTESIAN_POINT('Ctrl Pts',(6.59237166212351,-1.53734783650767,34.6240870174234));
#17240=CARTESIAN_POINT('Ctrl Pts',(6.62983064205607,-1.36675732621911,34.6323108519722));
#17241=CARTESIAN_POINT('Ctrl Pts',(6.66062029188332,-1.19516790759801,34.640534686521));
#17242=CARTESIAN_POINT('Ctrl Pts',(6.68891018826879,-1.03750950937422,34.6480908434952));
#17243=CARTESIAN_POINT('Ctrl Pts',(6.71157030468227,-0.87900811179361,34.6556470004694));
#17244=CARTESIAN_POINT('Ctrl Pts',(6.72857714554799,-0.720096241074283,
34.6632031574437));
#17245=CARTESIAN_POINT('Ctrl Pts',(6.74803629013535,-0.538270051637305,
34.671848875496));
#17246=CARTESIAN_POINT('Ctrl Pts',(6.76013831584193,-0.355492023085606,
34.6804945935484));
#17247=CARTESIAN_POINT('Ctrl Pts',(6.76480433960703,-0.172369506682167,
34.6891403116007));
#17248=CARTESIAN_POINT('Ctrl Pts',(6.76946437314853,0.0105179177294988,
34.697774930313));
#17249=CARTESIAN_POINT('Ctrl Pts',(6.76670743285558,0.193748644696248,34.7064095490253));
#17250=CARTESIAN_POINT('Ctrl Pts',(6.75650637311489,0.37671027336384,34.7150441677377));
#17251=CARTESIAN_POINT('Ctrl Pts',(6.74594505157208,0.566133396007559,34.7239837276401));
#17252=CARTESIAN_POINT('Ctrl Pts',(6.72740415662827,0.755267750292087,34.7329232875426));
#17253=CARTESIAN_POINT('Ctrl Pts',(6.70091245562786,0.943430581448054,34.741862847445));
#17254=CARTESIAN_POINT('Ctrl Pts',(6.6753954442371,1.12467047638163,34.7504735007155));
#17255=CARTESIAN_POINT('Ctrl Pts',(6.64250224987259,1.3050087111855,34.759084153986));
#17256=CARTESIAN_POINT('Ctrl Pts',(6.60231145869739,1.48383705384156,34.7676948072564));
#17257=CARTESIAN_POINT('Ctrl Pts',(6.56215871079495,1.66249612350699,34.7762973099675));
#17258=CARTESIAN_POINT('Ctrl Pts',(6.51472220476322,1.83964785390516,34.7848998126785));
#17259=CARTESIAN_POINT('Ctrl Pts',(6.46013190646794,2.01469222240889,34.7935023153896));
#17260=CARTESIAN_POINT('Ctrl Pts',(6.40560304845452,2.18953958199941,34.802095136157));
#17261=CARTESIAN_POINT('Ctrl Pts',(6.34393655118883,2.36228402081068,34.8106879569245));
#17262=CARTESIAN_POINT('Ctrl Pts',(6.2753127831944,2.53233853840219,34.8192807776919));
#17263=CARTESIAN_POINT('Ctrl Pts',(6.26722516042807,2.55238023573515,34.8202934806503));
#17264=CARTESIAN_POINT('Ctrl Pts',(6.25904096073811,2.57238458649186,34.8213061836087));
#17265=CARTESIAN_POINT('Ctrl Pts',(6.25076052528401,2.59235064286281,34.8223188865671));
#17266=CARTESIAN_POINT('Ctrl Pts',(6.18048080851004,2.76181139098665,34.8309141443272));
#17267=CARTESIAN_POINT('Ctrl Pts',(6.10334728356888,2.92831265800815,34.8395094020873));
#17268=CARTESIAN_POINT('Ctrl Pts',(6.01964288437314,3.09130854891838,34.8481046598474));
#17269=CARTESIAN_POINT('Ctrl Pts',(5.9358600995574,3.2544570785679,34.8567079667018));
#17270=CARTESIAN_POINT('Ctrl Pts',(5.84549429766296,3.41409340821317,34.8653112735563));
#17271=CARTESIAN_POINT('Ctrl Pts',(5.74887339275734,3.56969798639139,34.8739145804107));
#17272=CARTESIAN_POINT('Ctrl Pts',(5.64824655162947,3.73175398433929,34.8828745833507));
#17273=CARTESIAN_POINT('Ctrl Pts',(5.54083509015897,3.88943647468561,34.8918345862906));
#17274=CARTESIAN_POINT('Ctrl Pts',(5.42705710653814,4.04219496837719,34.9007945892306));
#17275=CARTESIAN_POINT('Ctrl Pts',(5.31750972899516,4.18927344392038,34.9094214324354));
#17276=CARTESIAN_POINT('Ctrl Pts',(5.20206096701656,4.33178729701084,34.9180482756402));
#17277=CARTESIAN_POINT('Ctrl Pts',(5.08112333419013,4.46928122439712,34.9266751188449));
#17278=CARTESIAN_POINT('Ctrl Pts',(4.96007011555765,4.60690656122189,34.9353102071311));
#17279=CARTESIAN_POINT('Ctrl Pts',(4.83351776288989,4.73950217293558,34.9439452954172));
#17280=CARTESIAN_POINT('Ctrl Pts',(4.70191519813217,4.86665002538437,34.9525803837034));
#17281=CARTESIAN_POINT('Ctrl Pts',(4.57011717715539,4.99398671791047,34.9612282968285));
#17282=CARTESIAN_POINT('Ctrl Pts',(4.43325418017205,5.11585927647829,34.9698762099537));
#17283=CARTESIAN_POINT('Ctrl Pts',(4.2918088253146,5.23188933435635,34.9785241230789));
#17284=CARTESIAN_POINT('Ctrl Pts',(4.27594080974908,5.24490614050267,34.9794942872827));
#17285=CARTESIAN_POINT('Ctrl Pts',(4.26001515371489,5.25784946086792,34.9804644514865));
#17286=CARTESIAN_POINT('Ctrl Pts',(4.24403256126565,5.27071879527991,34.9814346156904));
#17287=CARTESIAN_POINT('Ctrl Pts',(4.10852187633418,5.37983327882315,34.9896602909789));
#17288=CARTESIAN_POINT('Ctrl Pts',(3.96862187091144,5.48386222780802,34.9978859662674));
#17289=CARTESIAN_POINT('Ctrl Pts',(3.82475034660732,5.58243439604329,35.0061116415559));
#17290=CARTESIAN_POINT('Ctrl Pts',(3.68105229940655,5.68088770813729,35.014327398507));
#17291=CARTESIAN_POINT('Ctrl Pts',(3.53339256754797,5.77389714739813,35.022543155458));
#17292=CARTESIAN_POINT('Ctrl Pts',(3.38222220039914,5.86113145963535,35.0307589124091));
#17293=CARTESIAN_POINT('Ctrl Pts',(3.28916596746455,5.91483045258312,35.0358163016779));
#17294=CARTESIAN_POINT('Ctrl Pts',(3.19478012133075,5.96634185834478,35.0408736909467));
#17295=CARTESIAN_POINT('Ctrl Pts',(3.09917575053259,6.01559628526639,35.0459310802154));
#17296=CARTESIAN_POINT('Ctrl Pts',(3.09917575053263,6.01559628526637,33.0456763245139));
#17297=CARTESIAN_POINT('Ctrl Pts',(2.94420350634443,6.09543645379131,33.0539103182196));
#17298=CARTESIAN_POINT('Ctrl Pts',(2.7863355469165,6.16918564830321,33.0621443119252));
#17299=CARTESIAN_POINT('Ctrl Pts',(2.62609851799988,6.23665740391108,33.0703783056308));
#17300=CARTESIAN_POINT('Ctrl Pts',(2.61528137133451,6.24121223047716,33.0709341591571));
#17301=CARTESIAN_POINT('Ctrl Pts',(2.60445343349253,6.24573846840104,33.0714900126833));
#17302=CARTESIAN_POINT('Ctrl Pts',(2.59361486864044,6.25023606859511,33.0720458662095));
#17303=CARTESIAN_POINT('Ctrl Pts',(2.43462246349058,6.31621198717994,33.0801997583762));
#17304=CARTESIAN_POINT('Ctrl Pts',(2.27285054793751,6.37622538676165,33.088353650543));
#17305=CARTESIAN_POINT('Ctrl Pts',(2.10879019303076,6.43003055372036,33.0965075427097));
#17306=CARTESIAN_POINT('Ctrl Pts',(1.9449300375929,6.48377006334305,33.1046514848499));
#17307=CARTESIAN_POINT('Ctrl Pts',(1.77878734502059,6.53131630744089,33.1127954269901));
#17308=CARTESIAN_POINT('Ctrl Pts',(1.61087531091298,6.5724705958027,33.1209393691303));
#17309=CARTESIAN_POINT('Ctrl Pts',(1.44313283426488,6.61358332659169,33.1290750875232));
#17310=CARTESIAN_POINT('Ctrl Pts',(1.27362492547906,6.6483168650809,33.1372108059161));
#17311=CARTESIAN_POINT('Ctrl Pts',(1.10288217885207,6.67652154190867,33.145346524309));
#17312=CARTESIAN_POINT('Ctrl Pts',(0.932275932358765,6.70470367053317,33.1534757386092));
#17313=CARTESIAN_POINT('Ctrl Pts',(0.760437172698095,6.72636727073683,33.1616049529094));
#17314=CARTESIAN_POINT('Ctrl Pts',(0.587908988690094,6.74141320651816,33.1697341672096));
#17315=CARTESIAN_POINT('Ctrl Pts',(0.415482455990325,6.75645027743451,33.177858591885));
#17316=CARTESIAN_POINT('Ctrl Pts',(0.24236767122647,6.7648774170212,33.1859830165605));
#17317=CARTESIAN_POINT('Ctrl Pts',(0.0691151854357627,6.76664703462078,
33.1941074412359));
#17318=CARTESIAN_POINT('Ctrl Pts',(-0.105189053854327,6.76842739493204,
33.2022811863701));
#17319=CARTESIAN_POINT('Ctrl Pts',(-0.279632301184222,6.76346907674447,
33.2104549315043));
#17320=CARTESIAN_POINT('Ctrl Pts',(-0.45365088200447,6.75177679409328,33.2186286766385));
#17321=CARTESIAN_POINT('Ctrl Pts',(-0.626555098754313,6.74015938539881,
33.2267500795006));
#17322=CARTESIAN_POINT('Ctrl Pts',(-0.799039704118879,6.72189405262479,
33.2348714823628));
#17323=CARTESIAN_POINT('Ctrl Pts',(-0.970554318162976,6.69703765223813,
33.2429928852249));
#17324=CARTESIAN_POINT('Ctrl Pts',(-1.14208219281405,6.67217933008546,33.2511149159912));
#17325=CARTESIAN_POINT('Ctrl Pts',(-1.31263956454788,6.64072897771616,33.2592369467574));
#17326=CARTESIAN_POINT('Ctrl Pts',(-1.48168392233174,6.60279499562902,33.2673589775237));
#17327=CARTESIAN_POINT('Ctrl Pts',(-1.65077353968421,6.56485085718004,33.2754831828648));
#17328=CARTESIAN_POINT('Ctrl Pts',(-1.81834897952148,6.52041971260246,33.2836073882059));
#17329=CARTESIAN_POINT('Ctrl Pts',(-1.98388066364218,6.46966046345762,33.291731593547));
#17330=CARTESIAN_POINT('Ctrl Pts',(-2.15120411370535,6.41835178056318,33.2999437377895));
#17331=CARTESIAN_POINT('Ctrl Pts',(-2.31643893803346,6.36057730971967,33.3081558820319));
#17332=CARTESIAN_POINT('Ctrl Pts',(-2.47905746567104,6.29655168182559,33.3163680262744));
#17333=CARTESIAN_POINT('Ctrl Pts',(-2.64019146537982,6.23311053734893,33.3245052026908));
#17334=CARTESIAN_POINT('Ctrl Pts',(-2.79875642796621,6.16353209787753,33.3326423791073));
#17335=CARTESIAN_POINT('Ctrl Pts',(-2.95426280511298,6.08807196724267,33.3407795555238));
#17336=CARTESIAN_POINT('Ctrl Pts',(-3.11191820320259,6.01156901505888,33.3490291836792));
#17337=CARTESIAN_POINT('Ctrl Pts',(-3.26642951438578,5.92902080207527,33.3572788118347));
#17338=CARTESIAN_POINT('Ctrl Pts',(-3.41731639764043,5.84073947701983,33.3655284399901));
#17339=CARTESIAN_POINT('Ctrl Pts',(-3.56820328089505,5.7524581519644,33.3737780681456));
#17340=CARTESIAN_POINT('Ctrl Pts',(-3.71546544594209,5.65844397520847,33.382027696301));
#17341=CARTESIAN_POINT('Ctrl Pts',(-3.85865710243923,5.55905157070838,33.3902773244565));
#17342=CARTESIAN_POINT('Ctrl Pts',(-4.00063037221616,5.46050487460146,33.3984567583168));
#17343=CARTESIAN_POINT('Ctrl Pts',(-4.13903662439936,5.35636963765497,33.4066361921772));
#17344=CARTESIAN_POINT('Ctrl Pts',(-4.27340384810683,5.24693325200405,33.4148156260376));
#17345=CARTESIAN_POINT('Ctrl Pts',(-4.40761908259811,5.13762065510174,33.4229858077477));
#17346=CARTESIAN_POINT('Ctrl Pts',(-4.53780410542421,5.02301907483016,33.4311559894578));
#17347=CARTESIAN_POINT('Ctrl Pts',(-4.66351509958021,4.90345958645397,33.4393261711679));
#17348=CARTESIAN_POINT('Ctrl Pts',(-4.78910994358985,4.78401056456616,33.4474888040729));
#17349=CARTESIAN_POINT('Ctrl Pts',(-4.91023872837106,4.6596130045306,33.4556514369778));
#17350=CARTESIAN_POINT('Ctrl Pts',(-5.02648999868304,4.53063872904686,33.4638140698828));
#17351=CARTESIAN_POINT('Ctrl Pts',(-5.14265793676042,4.40175690601164,33.471970851579));
#17352=CARTESIAN_POINT('Ctrl Pts',(-5.25395508100174,4.26830516978556,33.4801276332753));
#17353=CARTESIAN_POINT('Ctrl Pts',(-5.36000619247849,4.13069275262543,33.4882844149716));
#17354=CARTESIAN_POINT('Ctrl Pts',(-5.46600324239429,3.99315048599908,33.4964370385941));
#17355=CARTESIAN_POINT('Ctrl Pts',(-5.56675936506153,3.85145205028661,33.5045896622165));
#17356=CARTESIAN_POINT('Ctrl Pts',(-5.66193904021825,3.7060403808988,33.512742285839));
#17357=CARTESIAN_POINT('Ctrl Pts',(-5.75710247557083,3.56065352202884,33.5208935184396));
#17358=CARTESIAN_POINT('Ctrl Pts',(-5.84669115424689,3.41155499152871,33.5290447510402));
#17359=CARTESIAN_POINT('Ctrl Pts',(-5.93041227645633,3.25921757961264,33.5371959836407));
#17360=CARTESIAN_POINT('Ctrl Pts',(-6.01412923751425,3.10688773925123,33.5453468111045));
#17361=CARTESIAN_POINT('Ctrl Pts',(-6.09197904718912,2.9513196561671,33.5534976385682));
#17362=CARTESIAN_POINT('Ctrl Pts',(-6.16371442687925,2.79301154023406,33.5616484660319));
#17363=CARTESIAN_POINT('Ctrl Pts',(-6.23545969583281,2.63468160033258,33.5698004171486));
#17364=CARTESIAN_POINT('Ctrl Pts',(-6.30108870615159,2.47361120636607,33.5779523682654));
#17365=CARTESIAN_POINT('Ctrl Pts',(-6.36040197912863,2.31031938569034,33.5861043193822));
#17366=CARTESIAN_POINT('Ctrl Pts',(-6.41973455400394,2.14697442611413,33.5942589233307));
#17367=CARTESIAN_POINT('Ctrl Pts',(-6.47274717479817,1.98140694165762,33.6024135272792));
#17368=CARTESIAN_POINT('Ctrl Pts',(-6.51928996406023,1.81415196841487,33.6105681312277));
#17369=CARTESIAN_POINT('Ctrl Pts',(-6.56588084541217,1.64672417267195,33.6187311612278));
#17370=CARTESIAN_POINT('Ctrl Pts',(-6.60598844634254,1.47760575605507,33.6268941912279));
#17371=CARTESIAN_POINT('Ctrl Pts',(-6.63951365496063,1.30734365244618,33.635057221228));
#17372=CARTESIAN_POINT('Ctrl Pts',(-6.67305825389327,1.13698307261951,33.6432249725625));
#17373=CARTESIAN_POINT('Ctrl Pts',(-6.70001281730768,0.965477845723865,
33.651392723897));
#17374=CARTESIAN_POINT('Ctrl Pts',(-6.72033005790458,0.793380685941044,
33.6595604752315));
#17375=CARTESIAN_POINT('Ctrl Pts',(-6.74067470280054,0.621051398079019,
33.6677392433918));
#17376=CARTESIAN_POINT('Ctrl Pts',(-6.75436411559209,0.448128943948057,
33.6759180115521));
#17377=CARTESIAN_POINT('Ctrl Pts',(-6.76140309140205,0.275167649949594,
33.6840967797123));
#17378=CARTESIAN_POINT('Ctrl Pts',(-6.76515634402121,0.182942950328629,
33.6884577810636));
#17379=CARTESIAN_POINT('Ctrl Pts',(-6.76701967731049,0.0907071641554947,
33.692818782415));
#17380=CARTESIAN_POINT('Ctrl Pts',(-6.76699984329972,-0.00145629033193495,
33.6971797837663));
#17381=CARTESIAN_POINT('',(-6.76699867180277,-0.0042397900355361,33.3028202161613));
#17382=CARTESIAN_POINT('Ctrl Pts',(3.0991757505326,6.01559628526638,32.6511251802053));
#17383=CARTESIAN_POINT('Ctrl Pts',(2.94517234236558,6.09493731904879,32.6592642952129));
#17384=CARTESIAN_POINT('Ctrl Pts',(2.78824240218256,6.16829766025846,32.6674034102206));
#17385=CARTESIAN_POINT('Ctrl Pts',(2.62890093239468,6.23547663676598,32.6755425252283));
#17386=CARTESIAN_POINT('Ctrl Pts',(2.46945010388479,6.30270171933131,32.683687226247));
#17387=CARTESIAN_POINT('Ctrl Pts',(2.30758478925735,6.36373685678097,32.6918319272657));
#17388=CARTESIAN_POINT('Ctrl Pts',(2.14383537037269,6.41843118719357,32.6999766282845));
#17389=CARTESIAN_POINT('Ctrl Pts',(1.97985080910237,6.47320405807014,32.7081330250053));
#17390=CARTESIAN_POINT('Ctrl Pts',(1.8139770908749,6.52161784001265,32.7162894217262));
#17391=CARTESIAN_POINT('Ctrl Pts',(1.64675585234037,6.56357251523763,32.7244458184471));
#17392=CARTESIAN_POINT('Ctrl Pts',(1.58335359791805,6.57947971109463,32.7275383319615));
#17393=CARTESIAN_POINT('Ctrl Pts',(1.51975769263817,6.59445890225035,32.7306308454759));
#17394=CARTESIAN_POINT('Ctrl Pts',(1.45599782810842,6.60850658806841,32.7337233589903));
#17395=CARTESIAN_POINT('Ctrl Pts',(1.28625300447666,6.64590506702078,32.7419564091223));
#17396=CARTESIAN_POINT('Ctrl Pts',(1.11481819085282,6.67681397247402,32.7501894592543));
#17397=CARTESIAN_POINT('Ctrl Pts',(0.942230479786608,6.70108130997984,32.7584225093863));
#17398=CARTESIAN_POINT('Ctrl Pts',(0.769848294154741,6.72531974881697,32.7666457552212));
#17399=CARTESIAN_POINT('Ctrl Pts',(0.596316296124643,6.74293231927,32.7748690010561));
#17400=CARTESIAN_POINT('Ctrl Pts',(0.422184442116325,6.75381738699196,32.7830922468909));
#17401=CARTESIAN_POINT('Ctrl Pts',(0.248225099513035,6.76469167094127,32.7913073460044));
#17402=CARTESIAN_POINT('Ctrl Pts',(0.0736674394620265,6.76885170319191,
32.7995224451179));
#17403=CARTESIAN_POINT('Ctrl Pts',(-0.10093063706062,6.76624726170294,32.8077375442314));
#17404=CARTESIAN_POINT('Ctrl Pts',(-0.275390673851752,6.76364487932259,
32.8159461483703));
#17405=CARTESIAN_POINT('Ctrl Pts',(-0.449890706938323,6.75428868084474,
32.8241547525092));
#17406=CARTESIAN_POINT('Ctrl Pts',(-0.623869890403432,6.7381804190633,32.8323633566481));
#17407=CARTESIAN_POINT('Ctrl Pts',(-0.79774632413001,6.72208167060209,32.8405671128971));
#17408=CARTESIAN_POINT('Ctrl Pts',(-0.971102165329179,6.69923883576472,
32.848770869146));
#17409=CARTESIAN_POINT('Ctrl Pts',(-1.14337865411116,6.66970570964889,32.856974625395));
#17410=CARTESIAN_POINT('Ctrl Pts',(-1.3156041706225,6.64018132164066,32.8651759543593));
#17411=CARTESIAN_POINT('Ctrl Pts',(-1.48675061762056,6.60397064206156,32.8733772833236));
#17412=CARTESIAN_POINT('Ctrl Pts',(-1.65626617800443,6.56117911259848,32.8815786122879));
#17413=CARTESIAN_POINT('Ctrl Pts',(-1.82575836057417,6.51839348449585,32.8897788102106));
#17414=CARTESIAN_POINT('Ctrl Pts',(-1.99361975702006,6.46902890094111,32.8979790081333));
#17415=CARTESIAN_POINT('Ctrl Pts',(-2.15931051581672,6.41324154357867,32.906179206056));
#17416=CARTESIAN_POINT('Ctrl Pts',(-2.32500845081249,6.35745177002122,32.9143797591359));
#17417=CARTESIAN_POINT('Ctrl Pts',(-2.48853522127145,6.29523878273873,32.9225803122157));
#17418=CARTESIAN_POINT('Ctrl Pts',(-2.6493678107698,6.22680810714903,32.9307808652955));
#17419=CARTESIAN_POINT('Ctrl Pts',(-2.81023651207198,6.15836206679313,32.9389832596488));
#17420=CARTESIAN_POINT('Ctrl Pts',(-2.96840949795698,6.08369569781668,32.947185654002));
#17421=CARTESIAN_POINT('Ctrl Pts',(-3.1233852931445,6.00306199456316,32.9553880483552));
#17422=CARTESIAN_POINT('Ctrl Pts',(-3.27850601794381,5.92235288462246,32.963598113389));
#17423=CARTESIAN_POINT('Ctrl Pts',(-3.43042326015574,5.83566545660226,32.9718081784228));
#17424=CARTESIAN_POINT('Ctrl Pts',(-3.57866083317763,5.74329832422802,32.9800182434567));
#17425=CARTESIAN_POINT('Ctrl Pts',(-3.72696935007209,5.65088698658291,32.988232237682));
#17426=CARTESIAN_POINT('Ctrl Pts',(-3.87159439023403,5.55279072593261,32.9964462319073));
#17427=CARTESIAN_POINT('Ctrl Pts',(-4.01209025154482,5.44935049464237,33.0046602261326));
#17428=CARTESIAN_POINT('Ctrl Pts',(-4.15277765550822,5.34576923986501,33.0128854187678));
#17429=CARTESIAN_POINT('Ctrl Pts',(-4.28932434994916,5.23682967756364,33.021110611403));
#17430=CARTESIAN_POINT('Ctrl Pts',(-4.42131818512401,5.12291269746926,33.0293358040382));
#17431=CARTESIAN_POINT('Ctrl Pts',(-4.54001995838984,5.02046740125994,33.0367327021581));
#17432=CARTESIAN_POINT('Ctrl Pts',(-4.65504001218599,4.91399732511296,33.0441296002781));
#17433=CARTESIAN_POINT('Ctrl Pts',(-4.76610547379797,4.80380345274795,33.051526498398));
#17434=CARTESIAN_POINT('Ctrl Pts',(-4.89592587200022,4.67500182367038,33.0601724648889));
#17435=CARTESIAN_POINT('Ctrl Pts',(-5.02063765702566,4.54081990971175,33.0688184313798));
#17436=CARTESIAN_POINT('Ctrl Pts',(-5.1397965093271,4.40167932074895,33.0774643978707));
#17437=CARTESIAN_POINT('Ctrl Pts',(-5.258802941257,4.26271671151537,33.0860993049951));
#17438=CARTESIAN_POINT('Ctrl Pts',(-5.37227040676659,4.11880830574691,33.0947342121194));
#17439=CARTESIAN_POINT('Ctrl Pts',(-5.47979155368142,3.97041226174333,33.1033691192438));
#17440=CARTESIAN_POINT('Ctrl Pts',(-5.59088231589151,3.81708958885203,33.1122906983153));
#17441=CARTESIAN_POINT('Ctrl Pts',(-5.69562490032188,3.65897639025737,33.1212122773868));
#17442=CARTESIAN_POINT('Ctrl Pts',(-5.79361342723059,3.49661728758145,33.1301338564583));
#17443=CARTESIAN_POINT('Ctrl Pts',(-5.88819141363774,3.33990917602604,33.138744915434));
#17444=CARTESIAN_POINT('Ctrl Pts',(-5.97647736241497,3.17924601535045,33.1473559744097));
#17445=CARTESIAN_POINT('Ctrl Pts',(-6.05814850899848,3.01514935665209,33.1559670333854));
#17446=CARTESIAN_POINT('Ctrl Pts',(-6.13974263592032,2.8512074486786,33.164569971735));
#17447=CARTESIAN_POINT('Ctrl Pts',(-6.21473426228188,2.68383877041427,33.1731729100845));
#17448=CARTESIAN_POINT('Ctrl Pts',(-6.2828456701583,2.51359091440375,33.1817758484341));
#17449=CARTESIAN_POINT('Ctrl Pts',(-6.35088080901431,2.34353369660803,33.1903691534828));
#17450=CARTESIAN_POINT('Ctrl Pts',(-6.41205098612041,2.17060401541842,33.1989624585316));
#17451=CARTESIAN_POINT('Ctrl Pts',(-6.4661258061129,1.99537115833642,33.2075557635804));
#17452=CARTESIAN_POINT('Ctrl Pts',(-6.47215062617444,1.97584734978866,33.2085131984208));
#17453=CARTESIAN_POINT('Ctrl Pts',(-6.4780874159619,1.95629497210247,33.2094706332613));
#17454=CARTESIAN_POINT('Ctrl Pts',(-6.48393589367517,1.93671482844296,33.2104280681017));
#17455=CARTESIAN_POINT('Ctrl Pts',(-6.53278554370796,1.77317087525512,33.2184250818853));
#17456=CARTESIAN_POINT('Ctrl Pts',(-6.57543908001728,1.60779208142203,33.2264220956689));
#17457=CARTESIAN_POINT('Ctrl Pts',(-6.61177080042785,1.44110231510803,33.2344191094524));
#17458=CARTESIAN_POINT('Ctrl Pts',(-6.64810882117877,1.27438364286145,33.2424175100107));
#17459=CARTESIAN_POINT('Ctrl Pts',(-6.67812277164572,1.10635391685539,33.2504159105689));
#17460=CARTESIAN_POINT('Ctrl Pts',(-6.70173829295727,0.937546186974363,
33.2584143111271));
#17461=CARTESIAN_POINT('Ctrl Pts',(-6.7253752626298,0.768585140591094,33.2664199760848));
#17462=CARTESIAN_POINT('Ctrl Pts',(-6.74260215172067,0.598845054670808,
33.2744256410426));
#17463=CARTESIAN_POINT('Ctrl Pts',(-6.75339654668035,0.428863711784925,
33.2824313060004));
#17464=CARTESIAN_POINT('Ctrl Pts',(-6.76256030552012,0.28456029882994,33.2892276093873));
#17465=CARTESIAN_POINT('Ctrl Pts',(-6.76708909581097,0.140083192540306,
33.2960239127743));
#17466=CARTESIAN_POINT('Ctrl Pts',(-6.76699867180277,-0.0042397900354902,
33.3028202161613));
#17467=CARTESIAN_POINT('Ctrl Pts',(-6.76699867180239,-0.00423979064372843,
33.3028202161899));
#17468=CARTESIAN_POINT('Ctrl Pts',(-6.76685118845725,-0.239633394842735,
33.3139051197925));
#17469=CARTESIAN_POINT('Ctrl Pts',(-6.75441678713885,-0.47460457998798,
33.3249900233951));
#17470=CARTESIAN_POINT('Ctrl Pts',(-6.72985396171361,-0.708064018297538,
33.3360749269978));
#17471=CARTESIAN_POINT('Ctrl Pts',(-6.70529113628837,-0.941523456607097,
33.3471598306004));
#17472=CARTESIAN_POINT('Ctrl Pts',(-6.66859999616083,-1.17347154533364,
33.358244734203));
#17473=CARTESIAN_POINT('Ctrl Pts',(-6.61999462935251,-1.40284001487838,
33.3693296378057));
#17474=CARTESIAN_POINT('Ctrl Pts',(-6.58392508836533,-1.57305198850748,
33.377555630347));
#17475=CARTESIAN_POINT('Ctrl Pts',(-6.5412393073043,-1.74209535196447,33.3857816228884));
#17476=CARTESIAN_POINT('Ctrl Pts',(-6.49202667257248,-1.90941841475552,
33.3940076154297));
#17477=CARTESIAN_POINT('Ctrl Pts',(-6.44286563092718,-2.07656606094264,
33.4022249840811));
#17478=CARTESIAN_POINT('Ctrl Pts',(-6.38719146195261,-2.24199665701822,
33.4104423527325));
#17479=CARTESIAN_POINT('Ctrl Pts',(-6.32514463314709,-2.40516826225746,
33.418659721384));
#17480=CARTESIAN_POINT('Ctrl Pts',(-6.26315043712016,-2.56820145309043,
33.4268701194463));
#17481=CARTESIAN_POINT('Ctrl Pts',(-6.19479447420671,-2.72897913653461,
33.4350805175087));
#17482=CARTESIAN_POINT('Ctrl Pts',(-6.12026715130905,-2.88697402077113,
33.4432909155711));
#17483=CARTESIAN_POINT('Ctrl Pts',(-6.0457881396868,-3.0448664870746,33.4514959913599));
#17484=CARTESIAN_POINT('Ctrl Pts',(-5.96514588908751,-3.19997942454144,
33.4597010671487));
#17485=CARTESIAN_POINT('Ctrl Pts',(-5.87857912702016,-3.35180495365749,
33.4679061429375));
#17486=CARTESIAN_POINT('Ctrl Pts',(-5.79205116738638,-3.5035624289401,33.476107540907));
#17487=CARTESIAN_POINT('Ctrl Pts',(-5.69960416408486,-3.65203512099309,
33.4843089388765));
#17488=CARTESIAN_POINT('Ctrl Pts',(-5.60152308524453,-3.79673914372224,
33.492510336846));
#17489=CARTESIAN_POINT('Ctrl Pts',(-5.50344968893109,-3.94143183202726,
33.5007110924137));
#17490=CARTESIAN_POINT('Ctrl Pts',(-5.39974328975629,-4.08235613776238,
33.5089118479814));
#17491=CARTESIAN_POINT('Ctrl Pts',(-5.29073274692962,-4.21905629265202,
33.5171126035491));
#17492=CARTESIAN_POINT('Ctrl Pts',(-5.18172275782461,-4.35575575316995,
33.5253133174609));
#17493=CARTESIAN_POINT('Ctrl Pts',(-5.06740890133723,-4.48823082472467,
33.5335140313726));
#17494=CARTESIAN_POINT('Ctrl Pts',(-4.94816089564999,-4.61605813988086,
33.5417147452844));
#17495=CARTESIAN_POINT('Ctrl Pts',(-4.82889188497798,-4.74390797122751,
33.549916903714));
#17496=CARTESIAN_POINT('Ctrl Pts',(-4.70468723798313,-4.86710815304147,
33.5581190621436));
#17497=CARTESIAN_POINT('Ctrl Pts',(-4.57595419253586,-4.98527152999849,
33.5663212205732));
#17498=CARTESIAN_POINT('Ctrl Pts',(-4.44717514147813,-5.10347713526039,
33.5745263102262));
#17499=CARTESIAN_POINT('Ctrl Pts',(-4.31386473202012,-5.21664210774924,
33.5827313998791));
#17500=CARTESIAN_POINT('Ctrl Pts',(-4.17646401910527,-5.32441896333478,
33.590936489532));
#17501=CARTESIAN_POINT('Ctrl Pts',(-4.03890634212075,-5.43231894123542,
33.5991509525298));
#17502=CARTESIAN_POINT('Ctrl Pts',(-3.89724930873116,-5.53481828364786,
33.6073654155276));
#17503=CARTESIAN_POINT('Ctrl Pts',(-3.75196462336234,-5.63161171113896,
33.6155798785254));
#17504=CARTESIAN_POINT('Ctrl Pts',(-3.60659386140927,-5.72846248567662,
33.6237992083329));
#17505=CARTESIAN_POINT('Ctrl Pts',(-3.45759146836291,-5.81960041982921,
33.6320185381403));
#17506=CARTESIAN_POINT('Ctrl Pts',(-3.30545449063006,-5.90476583874192,
33.6402378679478));
#17507=CARTESIAN_POINT('Ctrl Pts',(-3.15308178587413,-5.99006321630775,
33.6484699331085));
#17508=CARTESIAN_POINT('Ctrl Pts',(-2.99756510958667,-6.06936942273954,
33.6567019982692));
#17509=CARTESIAN_POINT('Ctrl Pts',(-2.83942347525055,-6.14247208607383,
33.6649340634299));
#17510=CARTESIAN_POINT('Ctrl Pts',(-2.69727441911673,-6.20818200893797,
33.672333634691));
#17511=CARTESIAN_POINT('Ctrl Pts',(-2.55300490545345,-6.26888024119241,
33.6797332059522));
#17512=CARTESIAN_POINT('Ctrl Pts',(-2.4070019758854,-6.32444704998657,33.6871327772133));
#17513=CARTESIAN_POINT('Ctrl Pts',(-2.2460844338632,-6.3856901655571,33.6952882356201));
#17514=CARTESIAN_POINT('Ctrl Pts',(-2.08256551603612,-6.44088765077319,
33.7034436940269));
#17515=CARTESIAN_POINT('Ctrl Pts',(-1.91694366712445,-6.4898086240714,33.7115991524337));
#17516=CARTESIAN_POINT('Ctrl Pts',(-1.75152340177355,-6.53867005411454,
33.7197446845756));
#17517=CARTESIAN_POINT('Ctrl Pts',(-1.58400564690597,-6.58127007629404,
33.7278902167174));
#17518=CARTESIAN_POINT('Ctrl Pts',(-1.41490954025648,-6.61742548072067,
33.7360357488593));
#17519=CARTESIAN_POINT('Ctrl Pts',(-1.245983688277,-6.65354448202383,33.7441730796599));
#17520=CARTESIAN_POINT('Ctrl Pts',(-1.07548300301375,-6.68323170772014,
33.7523104104605));
#17521=CARTESIAN_POINT('Ctrl Pts',(-0.903942533023143,-6.70635347241642,
33.760447741261));
#17522=CARTESIAN_POINT('Ctrl Pts',(-0.732538729053215,-6.72945681603939,
33.768578589063));
#17523=CARTESIAN_POINT('Ctrl Pts',(-0.560097150334056,-6.74600506502437,
33.7767094368651));
#17524=CARTESIAN_POINT('Ctrl Pts',(-0.387163810635177,-6.75591542159421,
33.7848402846671));
#17525=CARTESIAN_POINT('Ctrl Pts',(-0.214331919012058,-6.76581996444065,
33.7929663626609));
#17526=CARTESIAN_POINT('Ctrl Pts',(-0.04100920490468,-6.76909434882516,
33.8010924406546));
#17527=CARTESIAN_POINT('Ctrl Pts',(0.132252411158641,-6.76570752395806,
33.8092185186484));
#17528=CARTESIAN_POINT('Ctrl Pts',(0.306128381267504,-6.76230869002857,
33.8173734102306));
#17529=CARTESIAN_POINT('Ctrl Pts',(0.479942449932698,-6.75220127770795,
33.8255283018128));
#17530=CARTESIAN_POINT('Ctrl Pts',(0.653135381334614,-6.73540668212758,
33.833683193395));
#17531=CARTESIAN_POINT('Ctrl Pts',(0.825652920859281,-6.71867757959791,
33.8418062837513));
#17532=CARTESIAN_POINT('Ctrl Pts',(0.997553793903495,-6.69531340813728,
33.8499293741076));
#17533=CARTESIAN_POINT('Ctrl Pts',(1.16828937258548,-6.66538738123328,33.8580524644639));
#17534=CARTESIAN_POINT('Ctrl Pts',(1.33903835820453,-6.63545900440103,33.8661761926823));
#17535=CARTESIAN_POINT('Ctrl Pts',(1.50862150684899,-6.59896780888909,33.8742999209008));
#17536=CARTESIAN_POINT('Ctrl Pts',(1.6764995891936,-6.55603829514698,33.8824236491192));
#17537=CARTESIAN_POINT('Ctrl Pts',(1.84442279269734,-6.51309724309448,33.8905495607795));
#17538=CARTESIAN_POINT('Ctrl Pts',(2.01063966311429,-6.46371451775911,33.8986754724398));
#17539=CARTESIAN_POINT('Ctrl Pts',(2.17462539819144,-6.40806471390081,33.9068013841001));
#17540=CARTESIAN_POINT('Ctrl Pts',(2.339659839091,-6.35205902376195,33.9149792618102));
#17541=CARTESIAN_POINT('Ctrl Pts',(2.5024341532386,-6.28970594034005,33.9231571395203));
#17542=CARTESIAN_POINT('Ctrl Pts',(2.66243386369257,-6.22123258860036,33.9313350172304));
#17543=CARTESIAN_POINT('Ctrl Pts',(2.82166993023045,-6.15308604531752,33.9394738637038));
#17544=CARTESIAN_POINT('Ctrl Pts',(2.97815751599557,-6.07887773947098,33.9476127101772));
#17545=CARTESIAN_POINT('Ctrl Pts',(3.13141458455669,-5.99887753664181,33.9557515566507));
#17546=CARTESIAN_POINT('Ctrl Pts',(3.28577410902384,-5.91830185173588,33.9639489499791));
#17547=CARTESIAN_POINT('Ctrl Pts',(3.43685613567875,-5.83185081518611,33.9721463433075));
#17548=CARTESIAN_POINT('Ctrl Pts',(3.58419854173878,-5.73984405828222,33.9803437366358));
#17549=CARTESIAN_POINT('Ctrl Pts',(3.73154094779878,-5.64783730137834,33.9885411299642));
#17550=CARTESIAN_POINT('Ctrl Pts',(3.87514345970992,-5.55027508385098,33.9967385232926));
#17551=CARTESIAN_POINT('Ctrl Pts',(4.01457877321954,-5.44751744133189,34.004935916621));
#17552=CARTESIAN_POINT('Ctrl Pts',(4.15450423878479,-5.34439857848456,34.013162125958));
#17553=CARTESIAN_POINT('Ctrl Pts',(4.29064966970499,-5.23574089470283,34.021388335295));
#17554=CARTESIAN_POINT('Ctrl Pts',(4.42254851804683,-5.12185060359259,34.0296145446319));
#17555=CARTESIAN_POINT('Ctrl Pts',(4.55429918368309,-5.00808826334537,34.0378315121751));
#17556=CARTESIAN_POINT('Ctrl Pts',(4.68181249782518,-4.88910525393652,34.0460484797183));
#17557=CARTESIAN_POINT('Ctrl Pts',(4.80465159054427,-4.76525047541894,34.0542654472615));
#17558=CARTESIAN_POINT('Ctrl Pts',(4.9273773335949,-4.64150998379304,34.0624748326049));
#17559=CARTESIAN_POINT('Ctrl Pts',(5.04543719402836,-4.51290692889217,34.0706842179482));
#17560=CARTESIAN_POINT('Ctrl Pts',(5.15842799667021,-4.37982986007093,34.0788936032916));
#17561=CARTESIAN_POINT('Ctrl Pts',(5.27133720802551,-4.24684888694069,34.0870970605922));
#17562=CARTESIAN_POINT('Ctrl Pts',(5.37918442128618,-4.10940060718806,34.0953005178928));
#17563=CARTESIAN_POINT('Ctrl Pts',(5.48160385415867,-3.96790980064729,34.1035039751934));
#17564=CARTESIAN_POINT('Ctrl Pts',(5.5839698744761,-3.82649278269609,34.1117031543252));
#17565=CARTESIAN_POINT('Ctrl Pts',(5.68091354373583,-3.68103772770865,34.1199023334571));
#17566=CARTESIAN_POINT('Ctrl Pts',(5.77210981583395,-3.53200187909823,34.128101512589));
#17567=CARTESIAN_POINT('Ctrl Pts',(5.86328890458893,-3.38299411205371,34.1362991468188));
#17568=CARTESIAN_POINT('Ctrl Pts',(5.94872256097374,-3.23040719766393,34.1444967810486));
#17569=CARTESIAN_POINT('Ctrl Pts',(6.02812932199339,-3.07472695980042,34.1526944152784));
#17570=CARTESIAN_POINT('Ctrl Pts',(6.10753035134604,-2.91905795910703,34.160891457794));
#17571=CARTESIAN_POINT('Ctrl Pts',(6.18090518795532,-2.76029639872704,34.1690885003095));
#17572=CARTESIAN_POINT('Ctrl Pts',(6.2480185923347,-2.59895222538622,34.1772855428251));
#17573=CARTESIAN_POINT('Ctrl Pts',(6.31513935014388,-2.43759037401126,34.185483483468));
#17574=CARTESIAN_POINT('Ctrl Pts',(6.375997171133,-2.27364567715848,34.1936814241108));
#17575=CARTESIAN_POINT('Ctrl Pts',(6.43040516569789,-2.10764759980551,34.2018793647536));
#17576=CARTESIAN_POINT('Ctrl Pts',(6.48482901019461,-1.94160116451853,34.2100796935896));
#17577=CARTESIAN_POINT('Ctrl Pts',(6.53279917396162,-1.77350049797662,34.2182800224256));
#17578=CARTESIAN_POINT('Ctrl Pts',(6.57417877326439,-1.60388978959275,34.2264803512616));
#17579=CARTESIAN_POINT('Ctrl Pts',(6.61560149118333,-1.4341023424498,34.234689225053));
#17580=CARTESIAN_POINT('Ctrl Pts',(6.65041983920748,-1.26280205876364,34.2428980988444));
#17581=CARTESIAN_POINT('Ctrl Pts',(6.67854797676003,-1.09054386528675,34.2511069726358));
#17582=CARTESIAN_POINT('Ctrl Pts',(6.70669121037371,-0.918193222737659,
34.2593202520392));
#17583=CARTESIAN_POINT('Ctrl Pts',(6.7281370315992,-0.744884001142171,34.2675335314427));
#17584=CARTESIAN_POINT('Ctrl Pts',(6.74285157172199,-0.5711757012744,34.2757468108461));
#17585=CARTESIAN_POINT('Ctrl Pts',(6.75758763417243,-0.397213325716036,
34.2839721034615));
#17586=CARTESIAN_POINT('Ctrl Pts',(6.76557272340834,-0.222851063650834,
34.292197396077));
#17587=CARTESIAN_POINT('Ctrl Pts',(6.76682512404348,-0.0486491584089832,
34.3004226886924));
#17588=CARTESIAN_POINT('Ctrl Pts',(6.76795776997406,0.108895538978431,34.3078614778045));
#17589=CARTESIAN_POINT('Ctrl Pts',(6.76358441712264,0.266308916115103,34.3153002669166));
#17590=CARTESIAN_POINT('Ctrl Pts',(6.753754990295,0.423181439887758,34.3227390560288));
#17591=CARTESIAN_POINT('Ctrl Pts',(6.74288509739099,0.596659259387358,34.3309652570476));
#17592=CARTESIAN_POINT('Ctrl Pts',(6.72531175680491,0.769960473067657,34.3391914580664));
#17593=CARTESIAN_POINT('Ctrl Pts',(6.70103960477615,0.942527036865035,34.3474176590853));
#17594=CARTESIAN_POINT('Ctrl Pts',(6.67679471739456,1.11489975849825,34.355634619701));
#17595=CARTESIAN_POINT('Ctrl Pts',(6.64586605179754,1.28653912157858,34.3638515803168));
#17596=CARTESIAN_POINT('Ctrl Pts',(6.60831020194873,1.45688890270342,34.3720685409326));
#17597=CARTESIAN_POINT('Ctrl Pts',(6.57078900042455,1.6270815223064,34.3802779207342));
#17598=CARTESIAN_POINT('Ctrl Pts',(6.52665286786645,1.79598658134815,34.3884873005357));
#17599=CARTESIAN_POINT('Ctrl Pts',(6.47600997914114,1.96305469869396,34.3966966803373));
#17600=CARTESIAN_POINT('Ctrl Pts',(6.42540365142904,2.13000220325879,34.4049001334777));
#17601=CARTESIAN_POINT('Ctrl Pts',(6.36830002772615,2.29511506578169,34.4131035866181));
#17602=CARTESIAN_POINT('Ctrl Pts',(6.30485799355328,2.45785570795507,34.4213070397585));
#17603=CARTESIAN_POINT('Ctrl Pts',(6.24144903426589,2.6205115068826,34.4295062161086));
#17604=CARTESIAN_POINT('Ctrl Pts',(6.17170837754986,2.78079721590573,34.4377053924588));
#17605=CARTESIAN_POINT('Ctrl Pts',(6.095844264536,2.93819191043124,34.4459045688089));
#17606=CARTESIAN_POINT('Ctrl Pts',(6.01999442649988,3.09555698876971,34.4541022023603));
#17607=CARTESIAN_POINT('Ctrl Pts',(5.93802357722017,3.25003181074202,34.4622998359117));
#17608=CARTESIAN_POINT('Ctrl Pts',(5.85018759186039,3.40111660194747,34.4704974694631));
#17609=CARTESIAN_POINT('Ctrl Pts',(5.76235793284728,3.55219051133994,34.4786945125836));
#17610=CARTESIAN_POINT('Ctrl Pts',(5.66866415856292,3.69987456570618,34.4868915557042));
#17611=CARTESIAN_POINT('Ctrl Pts',(5.56940746173311,3.84369477523795,34.4950885988248));
#17612=CARTESIAN_POINT('Ctrl Pts',(5.47013987408253,3.98753076526794,34.503286541356));
#17613=CARTESIAN_POINT('Ctrl Pts',(5.36530835159771,4.12750177055697,34.5114844838872));
#17614=CARTESIAN_POINT('Ctrl Pts',(5.25525668612859,4.26316386770445,34.5196824264183));
#17615=CARTESIAN_POINT('Ctrl Pts',(5.14517294359279,4.39886550666276,34.5278827584268));
#17616=CARTESIAN_POINT('Ctrl Pts',(5.02986625327844,4.53025545733841,34.5360830904352));
#17617=CARTESIAN_POINT('Ctrl Pts',(4.90971987385085,4.65692385167656,34.5442834224436));
#17618=CARTESIAN_POINT('Ctrl Pts',(4.78944826942286,4.7837242687174,34.5524923014144));
#17619=CARTESIAN_POINT('Ctrl Pts',(4.66432714536748,4.90579303715201,34.5607011803851));
#17620=CARTESIAN_POINT('Ctrl Pts',(4.53477643787629,5.02275737603181,34.5689100593559));
#17621=CARTESIAN_POINT('Ctrl Pts',(4.40515618456044,5.13978450408168,34.5771233450433));
#17622=CARTESIAN_POINT('Ctrl Pts',(4.27110188244815,5.25170151029451,34.5853366307307));
#17623=CARTESIAN_POINT('Ctrl Pts',(4.13306546769413,5.35817682050101,34.5935499164181));
#17624=CARTESIAN_POINT('Ctrl Pts',(3.99482712267796,5.46480789096354,34.6017752171302));
#17625=CARTESIAN_POINT('Ctrl Pts',(3.8525953157173,5.5659811489269,34.6100005178422));
#17626=CARTESIAN_POINT('Ctrl Pts',(3.70685086082731,5.66140845510937,34.6182258185543));
#17627=CARTESIAN_POINT('Ctrl Pts',(3.57504258221534,5.7477109423634,34.6256646108483));
#17628=CARTESIAN_POINT('Ctrl Pts',(3.44036181171218,5.82931429266173,34.6331034031423));
#17629=CARTESIAN_POINT('Ctrl Pts',(3.30317982495396,5.90603860840895,34.6405421954363));
#17630=CARTESIAN_POINT('Ctrl Pts',(3.23585590749851,5.94369210521459,34.6441928834763));
#17631=CARTESIAN_POINT('Ctrl Pts',(3.16784100521239,5.980220624714,34.6478435715163));
#17632=CARTESIAN_POINT('Ctrl Pts',(3.09917575053259,6.01559628526639,34.6514942595564));
#17633=CARTESIAN_POINT('Origin',(0.,0.,-3.69717978381041));
#17634=CARTESIAN_POINT('',(3.09917575053255,6.01559628526641,37.0457515827422));
#17635=CARTESIAN_POINT('',(3.09917575053261,6.01559628526638,36.6515495189894));
#17636=CARTESIAN_POINT('',(3.09917575053259,6.01559628526639,-3.69717978381041));
#17637=CARTESIAN_POINT('',(-6.76699911870181,0.00214833398699119,35.69717978381));
#17638=CARTESIAN_POINT('Ctrl Pts',(-6.767,1.16698816081859E-12,35.69717978381));
#17639=CARTESIAN_POINT('Ctrl Pts',(-6.76700000000003,-0.186007249414598,
35.705929295616));
#17640=CARTESIAN_POINT('Ctrl Pts',(-6.75932637295444,-0.37201435552654,
35.7146788074219));
#17641=CARTESIAN_POINT('Ctrl Pts',(-6.74400518266935,-0.557389537154144,
35.7234283192279));
#17642=CARTESIAN_POINT('Ctrl Pts',(-6.72868405709653,-0.742763935810719,
35.7321777940784));
#17643=CARTESIAN_POINT('Ctrl Pts',(-6.70571545652998,-0.927506129694582,
35.740927268929));
#17644=CARTESIAN_POINT('Ctrl Pts',(-6.67517739415654,-1.11098863924953,
35.7496767437795));
#17645=CARTESIAN_POINT('Ctrl Pts',(-6.64463945823072,-1.29447038906647,
35.7584261824015));
#17646=CARTESIAN_POINT('Ctrl Pts',(-6.60653217027124,-1.47669218228365,
35.7671756210235));
#17647=CARTESIAN_POINT('Ctrl Pts',(-6.56098496116673,-1.65703510504273,
35.7759250596455));
#17648=CARTESIAN_POINT('Ctrl Pts',(-6.51543793687469,-1.83737729604194,
35.7846744627657));
#17649=CARTESIAN_POINT('Ctrl Pts',(-6.46245112202579,-2.01584035397248,
35.793423865886));
#17650=CARTESIAN_POINT('Ctrl Pts',(-6.40220448416169,-2.19181813638359,
35.8021732690062));
#17651=CARTESIAN_POINT('Ctrl Pts',(-6.34195808575099,-2.36779521936179,
35.8109226373515));
#17652=CARTESIAN_POINT('Ctrl Pts',(-6.27445201489132,-2.54128677545082,
35.8196720056968));
#17653=CARTESIAN_POINT('Ctrl Pts',(-6.19991555136064,-2.71170355238114,
35.8284213740421));
#17654=CARTESIAN_POINT('Ctrl Pts',(-6.12537937788914,-2.88211966613336,
35.8371707083391));
#17655=CARTESIAN_POINT('Ctrl Pts',(-6.04381298133488,-3.04946076210699,
35.8459200426362));
#17656=CARTESIAN_POINT('Ctrl Pts',(-5.95549339426175,-3.21315848207099,
35.8546693769332));
#17657=CARTESIAN_POINT('Ctrl Pts',(-5.86717414355025,-3.37685557859871,
35.8634186779088));
#17658=CARTESIAN_POINT('Ctrl Pts',(-5.77210188986099,-3.53690907467538,
35.8721679788843));
#17659=CARTESIAN_POINT('Ctrl Pts',(-5.67059953466926,-3.69277536785123,
35.8809172798599));
#17660=CARTESIAN_POINT('Ctrl Pts',(-5.5690975576162,-3.84864108036004,35.8896665482407));
#17661=CARTESIAN_POINT('Ctrl Pts',(-5.46116568337921,-4.00031938104482,
35.8984158166214));
#17662=CARTESIAN_POINT('Ctrl Pts',(-5.34717048685964,-4.14729511663413,
35.9071650850022));
#17663=CARTESIAN_POINT('Ctrl Pts',(-5.23317570555359,-4.29427031688233,
35.9159143215148));
#17664=CARTESIAN_POINT('Ctrl Pts',(-5.11311782178639,-4.43654275987321,
35.9246635580274));
#17665=CARTESIAN_POINT('Ctrl Pts',(-4.9874045917184,-4.57362924147839,35.93341279454));
#17666=CARTESIAN_POINT('Ctrl Pts',(-4.86169180910634,-4.7107152351464,35.9421619999112));
#17667=CARTESIAN_POINT('Ctrl Pts',(-4.73032391415212,-4.84261509316739,
35.9509112052823));
#17668=CARTESIAN_POINT('Ctrl Pts',(-4.59374707237049,-4.9688808433175,35.9596604106534));
#17669=CARTESIAN_POINT('Ctrl Pts',(-4.45717070537167,-5.09514615452929,
35.9684095856097));
#17670=CARTESIAN_POINT('Ctrl Pts',(-4.31538563819284,-5.21577720253818,
35.9771587605659));
#17671=CARTESIAN_POINT('Ctrl Pts',(-4.16887341290435,-5.33036429028816,
35.9859079355221));
#17672=CARTESIAN_POINT('Ctrl Pts',(-4.02236168477091,-5.44495098921361,
35.99465708079));
#17673=CARTESIAN_POINT('Ctrl Pts',(-3.87112305634155,-5.55349359238958,
36.003406226058));
#17674=CARTESIAN_POINT('Ctrl Pts',(-3.7156711731641,-5.65562346102685,36.0121553713259));
#17675=CARTESIAN_POINT('Ctrl Pts',(-3.56021980456983,-5.75775299158965,
36.0209044876321));
#17676=CARTESIAN_POINT('Ctrl Pts',(-3.40055544862076,-5.85346967275534,
36.0296536039382));
#17677=CARTESIAN_POINT('Ctrl Pts',(-3.23722036323099,-5.94244842803727,
36.0384027202444));
#17678=CARTESIAN_POINT('Ctrl Pts',(-3.07388580495719,-6.03142689616643,
36.0471518083153));
#17679=CARTESIAN_POINT('Ctrl Pts',(-2.90688079257356,-6.1136673448499,36.0559008963863));
#17680=CARTESIAN_POINT('Ctrl Pts',(-2.7367725109424,-6.18889046787468,36.0646499844572));
#17681=CARTESIAN_POINT('Ctrl Pts',(-2.56666476416297,-6.26411335438412,
36.0733990450195));
#17682=CARTESIAN_POINT('Ctrl Pts',(-2.39345402971772,-6.33231884350411,
36.0821481055817));
#17683=CARTESIAN_POINT('Ctrl Pts',(-2.21772856473747,-6.39327529621144,
36.0908971661439));
#17684=CARTESIAN_POINT('Ctrl Pts',(-2.04200363767981,-6.45423156232173,
36.0996461999239));
#17685=CARTESIAN_POINT('Ctrl Pts',(-1.86376426619808,-6.50793874252137,
36.1083952337039));
#17686=CARTESIAN_POINT('Ctrl Pts',(-1.68361578194407,-6.55421443796195,
36.1171442674839));
#17687=CARTESIAN_POINT('Ctrl Pts',(-1.50346783419563,-6.6004899955875,36.1258932752081));
#17688=CARTESIAN_POINT('Ctrl Pts',(-1.32141106256918,-6.63933404145561,
36.1346422829324));
#17689=CARTESIAN_POINT('Ctrl Pts',(-1.13806375958692,-6.6706146552709,36.1433912906566));
#17690=CARTESIAN_POINT('Ctrl Pts',(-0.954716987415489,-6.70189517852533,
36.1521402730515));
#17691=CARTESIAN_POINT('Ctrl Pts',(-0.770079973806076,-6.72561226535872,
36.1608892554464));
#17692=CARTESIAN_POINT('Ctrl Pts',(-0.584779770548522,-6.74168536939816,
36.1696382378413));
#17693=CARTESIAN_POINT('Ctrl Pts',(-0.39149064755002,-6.75845143942416,
36.1787644185173));
#17694=CARTESIAN_POINT('Ctrl Pts',(-0.197480213100493,-6.76689975924038,
36.1878905991934));
#17695=CARTESIAN_POINT('Ctrl Pts',(-0.00346532629400725,-6.76699911271708,
36.1970167798694));
#17696=CARTESIAN_POINT('Ctrl Pts',(0.184486595299774,-6.76709536139763,
36.2058577673994));
#17697=CARTESIAN_POINT('Ctrl Pts',(0.372442378188871,-6.7593565972675,36.2146987549293));
#17698=CARTESIAN_POINT('Ctrl Pts',(0.559750217725649,-6.74380965728987,
36.2235397424592));
#17699=CARTESIAN_POINT('Ctrl Pts',(0.745129914461276,-6.72842275717214,
36.232289721057));
#17700=CARTESIAN_POINT('Ctrl Pts',(0.929874656317667,-6.70538772273424,
36.2410396996547));
#17701=CARTESIAN_POINT('Ctrl Pts',(1.11335688290121,-6.67478280180685,36.2497896782525));
#17702=CARTESIAN_POINT('Ctrl Pts',(1.29683723119207,-6.64417819417955,36.2585395672774));
#17703=CARTESIAN_POINT('Ctrl Pts',(1.47905480730593,-6.60600390229995,36.2672894563024));
#17704=CARTESIAN_POINT('Ctrl Pts',(1.65939064805172,-6.56038959797042,36.2760393453273));
#17705=CARTESIAN_POINT('Ctrl Pts',(1.83972470264625,-6.51477574543154,36.2847891476883));
#17706=CARTESIAN_POINT('Ctrl Pts',(2.01817678126204,-6.46172209819989,36.2935389500492));
#17707=CARTESIAN_POINT('Ctrl Pts',(2.19414072348031,-6.40140886723894,36.3022887524102));
#17708=CARTESIAN_POINT('Ctrl Pts',(2.3701029813244,-6.34109621361246,36.3110384710157));
#17709=CARTESIAN_POINT('Ctrl Pts',(2.54357687927248,-6.27352420825835,36.3197881896211));
#17710=CARTESIAN_POINT('Ctrl Pts',(2.71397317790297,-6.19892237325354,36.3285379082266));
#17711=CARTESIAN_POINT('Ctrl Pts',(2.88436790207525,-6.12432122756811,36.3372875459849));
#17712=CARTESIAN_POINT('Ctrl Pts',(3.05168482126578,-6.04269049717255,36.3460371837432));
#17713=CARTESIAN_POINT('Ctrl Pts',(3.21535561997707,-5.95430745234758,36.3547868215014));
#17714=CARTESIAN_POINT('Ctrl Pts',(3.37902496075585,-5.86592519481341,36.3635363813205));
#17715=CARTESIAN_POINT('Ctrl Pts',(3.53904799385165,-5.77079087940054,36.3722859411395));
#17716=CARTESIAN_POINT('Ctrl Pts',(3.6948811881526,-5.66922763746844,36.3810355009585));
#17717=CARTESIAN_POINT('Ctrl Pts',(3.85071304611103,-5.56766526648865,36.3897849857459));
#17718=CARTESIAN_POINT('Ctrl Pts',(4.00235489706232,-5.4596742358052,36.3985344705333));
#17719=CARTESIAN_POINT('Ctrl Pts',(4.14929168607912,-5.34562133936128,36.4072839553208));
#17720=CARTESIAN_POINT('Ctrl Pts',(4.29622726386008,-5.23156938308325,36.4160333679841));
#17721=CARTESIAN_POINT('Ctrl Pts',(4.4384576309231,-5.11145583676991,36.4247827806474));
#17722=CARTESIAN_POINT('Ctrl Pts',(4.57549970661197,-4.98568866203996,36.4335321933107));
#17723=CARTESIAN_POINT('Ctrl Pts',(4.71254069815517,-4.85992248225946,36.442281536757));
#17724=CARTESIAN_POINT('Ctrl Pts',(4.84439326931523,-4.72850295733787,36.4510308802033));
#17725=CARTESIAN_POINT('Ctrl Pts',(4.97060959434895,-4.59187644221468,36.4597802236496));
#17726=CARTESIAN_POINT('Ctrl Pts',(5.09682496280707,-4.45525096256444,36.4685295007859));
#17727=CARTESIAN_POINT('Ctrl Pts',(5.21740397616025,-4.31341878218101,36.4772787779222));
#17728=CARTESIAN_POINT('Ctrl Pts',(5.33193710452114,-4.16686161438447,36.4860280550585));
#17729=CARTESIAN_POINT('Ctrl Pts',(5.44646940289561,-4.02030550864273,36.4947772687915));
#17730=CARTESIAN_POINT('Ctrl Pts',(5.55495572749841,-3.86902470979881,36.5035264825245));
#17731=CARTESIAN_POINT('Ctrl Pts',(5.65702762491628,-3.71353301465519,36.5122756962574));
#17732=CARTESIAN_POINT('Ctrl Pts',(5.75909881655322,-3.5580423946662,36.5210248494935));
#17733=CARTESIAN_POINT('Ctrl Pts',(5.85475551250946,-3.39834117619271,36.5297740027297));
#17734=CARTESIAN_POINT('Ctrl Pts',(5.94367283728254,-3.23497174691677,36.5385231559658));
#17735=CARTESIAN_POINT('Ctrl Pts',(6.03258957676467,-3.0716033930066,36.5472722516113));
#17736=CARTESIAN_POINT('Ctrl Pts',(6.11476689685436,-2.90456712829185,36.5560213472569));
#17737=CARTESIAN_POINT('Ctrl Pts',(6.18992570525408,-2.73443024475572,36.5647704429024));
#17738=CARTESIAN_POINT('Ctrl Pts',(6.26508404388838,-2.56429442462687,36.5735194838634));
#17739=CARTESIAN_POINT('Ctrl Pts',(6.33322384283449,-2.39105828655639,36.5822685248245));
#17740=CARTESIAN_POINT('Ctrl Pts',(6.39411368720159,-2.21531017131718,36.5910175657855));
#17741=CARTESIAN_POINT('Ctrl Pts',(6.45500317121009,-2.0395630961914,36.5997665549679));
#17742=CARTESIAN_POINT('Ctrl Pts',(6.50864269270184,-1.86130434438246,36.6085155441503));
#17743=CARTESIAN_POINT('Ctrl Pts',(6.55485008446436,-1.68113930719546,36.6172645333327));
#17744=CARTESIAN_POINT('Ctrl Pts',(6.60199664749493,-1.49731239211445,36.6261913468621));
#17745=CARTESIAN_POINT('Ctrl Pts',(6.64140563640983,-1.31150116499281,36.6351181603915));
#17746=CARTESIAN_POINT('Ctrl Pts',(6.67293772282237,-1.12436255155276,36.6440449739208));
#17747=CARTESIAN_POINT('Ctrl Pts',(6.70384494949925,-0.940932395047478,
36.6527948880764));
#17748=CARTESIAN_POINT('Ctrl Pts',(6.72718449348974,-0.756227260502834,
36.6615448022319));
#17749=CARTESIAN_POINT('Ctrl Pts',(6.74287707373965,-0.570874564537798,
36.6702947163874));
#17750=CARTESIAN_POINT('Ctrl Pts',(6.75856934538692,-0.385525513628589,
36.6790444584714));
#17751=CARTESIAN_POINT('Ctrl Pts',(6.76661493004114,-0.199529212414354,
36.6877942005554));
#17752=CARTESIAN_POINT('Ctrl Pts',(6.76698649908907,-0.013517438596568,
36.6965439426393));
#17753=CARTESIAN_POINT('Ctrl Pts',(6.76735806132379,0.17249092444962,36.7052935242852));
#17754=CARTESIAN_POINT('Ctrl Pts',(6.76005588896269,0.358514472905227,36.7140431059311));
#17755=CARTESIAN_POINT('Ctrl Pts',(6.74510478454554,0.543921359666006,36.722792687577));
#17756=CARTESIAN_POINT('Ctrl Pts',(6.73015393440646,0.729325093154255,36.7315421204161));
#17757=CARTESIAN_POINT('Ctrl Pts',(6.70755443556845,0.914111900260174,36.7402915532551));
#17758=CARTESIAN_POINT('Ctrl Pts',(6.67738304682256,1.09765415591921,36.7490409860942));
#17759=CARTESIAN_POINT('Ctrl Pts',(6.64721213111786,1.28119353391662,36.7577902817555));
#17760=CARTESIAN_POINT('Ctrl Pts',(6.60946960955407,1.46348811673048,36.7665395774168));
#17761=CARTESIAN_POINT('Ctrl Pts',(6.56428366991083,1.64391876348622,36.7752888730781));
#17762=CARTESIAN_POINT('Ctrl Pts',(6.51909837867606,1.82434682110113,36.784038043189));
#17763=CARTESIAN_POINT('Ctrl Pts',(6.46646995271799,2.0029107182084,36.7927872132998));
#17764=CARTESIAN_POINT('Ctrl Pts',(6.40657713281416,2.17900400213096,36.8015363834106));
#17765=CARTESIAN_POINT('Ctrl Pts',(6.34668509278916,2.35509499310046,36.8102854395964));
#17766=CARTESIAN_POINT('Ctrl Pts',(6.27952894037372,2.52871516398505,36.8190344957822));
#17767=CARTESIAN_POINT('Ctrl Pts',(6.20533675061283,2.69927486771797,36.827783551968));
#17768=CARTESIAN_POINT('Ctrl Pts',(6.1283211790775,2.87632521636277,36.8368655532502));
#17769=CARTESIAN_POINT('Ctrl Pts',(6.04372366625912,3.05007728920327,36.8459475545325));
#17770=CARTESIAN_POINT('Ctrl Pts',(5.95185378007702,3.21989527478502,36.8550295558147));
#17771=CARTESIAN_POINT('Ctrl Pts',(5.86334450817198,3.38350129287052,36.8637793361219));
#17772=CARTESIAN_POINT('Ctrl Pts',(5.76808562057075,3.54345567125256,36.872529116429));
#17773=CARTESIAN_POINT('Ctrl Pts',(5.66640068804296,3.69921508465597,36.8812788967361));
#17774=CARTESIAN_POINT('Ctrl Pts',(5.56471941107727,3.85496889852566,36.8900283624896));
#17775=CARTESIAN_POINT('Ctrl Pts',(5.4566127081491,4.00652780919914,36.8987778282431));
#17776=CARTESIAN_POINT('Ctrl Pts',(5.34244776448903,4.153377045695,36.9075272939966));
#17777=CARTESIAN_POINT('Ctrl Pts',(5.22828631819376,4.30022178356516,36.9162764917161));
#17778=CARTESIAN_POINT('Ctrl Pts',(5.10806717843841,4.44235690972941,36.9250256894357));
#17779=CARTESIAN_POINT('Ctrl Pts',(4.98219864544483,4.57929969070902,36.9337748871553));
#17780=CARTESIAN_POINT('Ctrl Pts',(4.85633329943774,4.71623900430259,36.9425238633456));
#17781=CARTESIAN_POINT('Ctrl Pts',(4.72481904033382,4.84798602483876,36.9512728395358));
#17782=CARTESIAN_POINT('Ctrl Pts',(4.58810250736918,4.97409332259385,36.9600218157261));
#17783=CARTESIAN_POINT('Ctrl Pts',(4.45137708685356,5.10020881822385,36.9687713606622));
#17784=CARTESIAN_POINT('Ctrl Pts',(4.3094489263576,5.22068366308174,36.9775209055984));
#17785=CARTESIAN_POINT('Ctrl Pts',(4.16280009466365,5.33510865605081,36.9862704505346));
#17786=CARTESIAN_POINT('Ctrl Pts',(4.01615988348486,5.44952692273115,36.9950194811429));
#17787=CARTESIAN_POINT('Ctrl Pts',(3.86479978231921,5.55789587288842,37.0037685117512));
#17788=CARTESIAN_POINT('Ctrl Pts',(3.70923383580751,5.65984746714085,37.0125175423594));
#17789=CARTESIAN_POINT('Ctrl Pts',(3.55366577799218,5.76180044505581,37.0212666917075));
#17790=CARTESIAN_POINT('Ctrl Pts',(3.39389200026513,5.85733573571249,37.0300158410555));
#17791=CARTESIAN_POINT('Ctrl Pts',(3.23045513625709,5.94612887622108,37.0387649904035));
#17792=CARTESIAN_POINT('Ctrl Pts',(3.18695122151355,5.96976399206807,37.0410938545164));
#17793=CARTESIAN_POINT('Ctrl Pts',(3.1431879126255,5.99292165435392,37.0434227186293));
#17794=CARTESIAN_POINT('Ctrl Pts',(3.09917575053255,6.01559628526641,37.0457515827422));
#17795=CARTESIAN_POINT('Ctrl Pts',(3.09917575053259,6.01559628526639,35.0459310802154));
#17796=CARTESIAN_POINT('Ctrl Pts',(2.9440586973841,6.09551105793644,35.0541366393698));
#17797=CARTESIAN_POINT('Ctrl Pts',(2.78573265664416,6.16948200765193,35.0623421985241));
#17798=CARTESIAN_POINT('Ctrl Pts',(2.6246942276003,6.23724852892697,35.0705477576784));
#17799=CARTESIAN_POINT('Ctrl Pts',(2.46374070143196,6.30497932225462,35.0787489906879));
#17800=CARTESIAN_POINT('Ctrl Pts',(2.30007796525645,6.36651206492384,35.0869502236974));
#17801=CARTESIAN_POINT('Ctrl Pts',(2.13422506491495,6.4216331546024,35.0951514567069));
#17802=CARTESIAN_POINT('Ctrl Pts',(1.96189659516602,6.47890639501991,35.1036728990915));
#17803=CARTESIAN_POINT('Ctrl Pts',(1.78720384805667,6.52925703590783,35.1121943414761));
#17804=CARTESIAN_POINT('Ctrl Pts',(1.6107499787808,6.57250131273153,35.1207157838607));
#17805=CARTESIAN_POINT('Ctrl Pts',(1.44096982551859,6.61411003447263,35.1289149341543));
#17806=CARTESIAN_POINT('Ctrl Pts',(1.26955970154868,6.64914001105007,35.1371140844478));
#17807=CARTESIAN_POINT('Ctrl Pts',(1.09707021372699,6.6774790112851,35.1453132347414));
#17808=CARTESIAN_POINT('Ctrl Pts',(0.924561343545949,6.70582119592686,35.1535133063599));
#17809=CARTESIAN_POINT('Ctrl Pts',(0.750973221621192,6.72747084782639,35.1617133779785));
#17810=CARTESIAN_POINT('Ctrl Pts',(0.576864392437851,6.74236727512951,35.1699134495971));
#17811=CARTESIAN_POINT('Ctrl Pts',(0.402704413692092,6.75726807869397,35.1781159302266));
#17812=CARTESIAN_POINT('Ctrl Pts',(0.228023780045558,6.76541167489834,35.1863184108561));
#17813=CARTESIAN_POINT('Ctrl Pts',(0.0533839308849914,6.76678942748504,
35.1945208914856));
#17814=CARTESIAN_POINT('Ctrl Pts',(-0.121338906013691,6.76816783477094,
35.2027272698814));
#17815=CARTESIAN_POINT('Ctrl Pts',(-0.296020561820025,6.7627739909933,35.2109336482771));
#17816=CARTESIAN_POINT('Ctrl Pts',(-0.470101770653946,6.75065132600018,
35.2191400266729));
#17817=CARTESIAN_POINT('Ctrl Pts',(-0.644388886027253,6.73851432209012,
35.227356111728));
#17818=CARTESIAN_POINT('Ctrl Pts',(-0.81807377860967,6.7196326277004,35.235572196783));
#17819=CARTESIAN_POINT('Ctrl Pts',(-0.990603530442371,6.69410140687121,
35.243788281838));
#17820=CARTESIAN_POINT('Ctrl Pts',(-1.16325377716496,6.66855235502094,35.2520101050122));
#17821=CARTESIAN_POINT('Ctrl Pts',(-1.33474692428573,6.63634458684152,35.2602319281863));
#17822=CARTESIAN_POINT('Ctrl Pts',(-1.50454249032188,6.59762388249103,35.2684537513604));
#17823=CARTESIAN_POINT('Ctrl Pts',(-1.6745716687148,6.55884990445849,35.2766868864877));
#17824=CARTESIAN_POINT('Ctrl Pts',(-1.8428982578737,6.51354519028979,35.284920021615));
#17825=CARTESIAN_POINT('Ctrl Pts',(-2.00899827364353,6.46190489998865,35.2931531567423));
#17826=CARTESIAN_POINT('Ctrl Pts',(-2.05279672271923,6.44828801612187,35.2953241291407));
#17827=CARTESIAN_POINT('Ctrl Pts',(-2.09644047195137,6.43423086992658,35.297495101539));
#17828=CARTESIAN_POINT('Ctrl Pts',(-2.139920175324,6.41973758367438,35.2996660739374));
#17829=CARTESIAN_POINT('Ctrl Pts',(-2.30322433018449,6.3653026708535,35.3078199661041));
#17830=CARTESIAN_POINT('Ctrl Pts',(-2.46471757423055,6.30454336770894,35.3159738582709));
#17831=CARTESIAN_POINT('Ctrl Pts',(-2.623868021179,6.23759614013558,35.3241277504376));
#17832=CARTESIAN_POINT('Ctrl Pts',(-2.78282426011805,6.17073060688385,35.3322716925778));
#17833=CARTESIAN_POINT('Ctrl Pts',(-2.93944305928883,6.09769231987377,35.340415634718));
#17834=CARTESIAN_POINT('Ctrl Pts',(-3.09320666017572,6.01866775602746,35.3485595768583));
#17835=CARTESIAN_POINT('Ctrl Pts',(-3.24681499068139,5.93972299113281,35.3566952952512));
#17836=CARTESIAN_POINT('Ctrl Pts',(-3.39757353997227,5.85480414956821,35.3648310136441));
#17837=CARTESIAN_POINT('Ctrl Pts',(-3.54498355517324,5.7641461287472,35.372966732037));
#17838=CARTESIAN_POINT('Ctrl Pts',(-3.69227572357141,5.67356058439862,35.3810959463372));
#17839=CARTESIAN_POINT('Ctrl Pts',(-3.83622437802582,5.57724518699878,35.3892251606374));
#17840=CARTESIAN_POINT('Ctrl Pts',(-3.97635446585219,5.47548118085501,35.3973543749376));
#17841=CARTESIAN_POINT('Ctrl Pts',(-4.11640199089731,5.37377713270818,35.405478799613));
#17842=CARTESIAN_POINT('Ctrl Pts',(-4.25263513467597,5.26663108321617,35.4136032242885));
#17843=CARTESIAN_POINT('Ctrl Pts',(-4.38460700780134,5.15436808805303,35.4217276489639));
#17844=CARTESIAN_POINT('Ctrl Pts',(-4.51738003468018,5.04142358464255,35.4299013940981));
#17845=CARTESIAN_POINT('Ctrl Pts',(-4.64583956460938,4.92330000262571,35.4380751392323));
#17846=CARTESIAN_POINT('Ctrl Pts',(-4.76956309492173,4.80037049440569,35.4462488843664));
#17847=CARTESIAN_POINT('Ctrl Pts',(-4.89249433595027,4.67822819078433,35.4543702872286));
#17848=CARTESIAN_POINT('Ctrl Pts',(-5.01074980957345,4.55134160982569,35.4624916900908));
#17849=CARTESIAN_POINT('Ctrl Pts',(-5.12395124004177,4.42011455617096,35.4706130929529));
#17850=CARTESIAN_POINT('Ctrl Pts',(-5.23716142264873,4.28887735673132,35.4787351237192));
#17851=CARTESIAN_POINT('Ctrl Pts',(-5.34531654466242,4.15329929324313,35.4868571544854));
#17852=CARTESIAN_POINT('Ctrl Pts',(-5.44807806829093,4.013817928333,35.4949791852517));
#17853=CARTESIAN_POINT('Ctrl Pts',(-5.55086710506615,3.87429921898576,35.5031033905928));
#17854=CARTESIAN_POINT('Ctrl Pts',(-5.64825945106151,3.73087542184351,35.511227595934));
#17855=CARTESIAN_POINT('Ctrl Pts',(-5.73995944602269,3.58401374969668,35.5193518012751));
#17856=CARTESIAN_POINT('Ctrl Pts',(-5.83265202997786,3.43556240156926,35.5275639455175));
#17857=CARTESIAN_POINT('Ctrl Pts',(-5.91952810752149,3.28359864338214,35.5357760897599));
#17858=CARTESIAN_POINT('Ctrl Pts',(-6.0003299993453,3.12863051493092,35.5439882340023));
#17859=CARTESIAN_POINT('Ctrl Pts',(-6.08039425895217,2.97507707469507,35.5521254104188));
#17860=CARTESIAN_POINT('Ctrl Pts',(-6.15449467311389,2.81857424654053,35.5602625868353));
#17861=CARTESIAN_POINT('Ctrl Pts',(-6.22242921177155,2.65963600977505,35.5683997632517));
#17862=CARTESIAN_POINT('Ctrl Pts',(-6.29130257203203,2.4985013254714,35.5766493914071));
#17863=CARTESIAN_POINT('Ctrl Pts',(-6.35383825003811,2.33486379393832,35.5848990195625));
#17864=CARTESIAN_POINT('Ctrl Pts',(-6.40987824321453,2.16927405072873,35.5931486477179));
#17865=CARTESIAN_POINT('Ctrl Pts',(-6.46591823639095,2.00368430751914,35.6013982758733));
#17866=CARTESIAN_POINT('Ctrl Pts',(-6.51546249628877,1.836142739554,35.6096479040287));
#17867=CARTESIAN_POINT('Ctrl Pts',(-6.5584069576644,1.66720939826383,35.6178975321841));
#17868=CARTESIAN_POINT('Ctrl Pts',(-6.61564801371588,1.44203663912329,35.6288935352197));
#17869=CARTESIAN_POINT('Ctrl Pts',(-6.66130674986052,1.21384317140458,35.6398895382552));
#17870=CARTESIAN_POINT('Ctrl Pts',(-6.69512707799532,0.983647502662358,
35.6508855412908));
#17871=CARTESIAN_POINT('Ctrl Pts',(-6.72814535798224,0.758910917848252,
35.661620774418));
#17872=CARTESIAN_POINT('Ctrl Pts',(-6.74988016006797,0.532265633934366,
35.6723560075452));
#17873=CARTESIAN_POINT('Ctrl Pts',(-6.76013745111812,0.304681213713947,
35.6830912406724));
#17874=CARTESIAN_POINT('Ctrl Pts',(-6.7646245540288,0.205123278835854,35.6877874217182));
#17875=CARTESIAN_POINT('Ctrl Pts',(-6.76691581385178,0.105385939787265,
35.6924836027641));
#17876=CARTESIAN_POINT('Ctrl Pts',(-6.76699772244824,0.00555197085342392,
35.69717978381));
#17877=CARTESIAN_POINT('',(-6.76699973985247,0.00187638925443544,35.3028202162328));
#17878=CARTESIAN_POINT('Ctrl Pts',(3.09917575053259,6.01559628526639,34.6514942595564));
#17879=CARTESIAN_POINT('Ctrl Pts',(2.94591905660335,6.0945526192537,34.6596423743809));
#17880=CARTESIAN_POINT('Ctrl Pts',(2.78942067268773,6.1677630348461,34.6677904892054));
#17881=CARTESIAN_POINT('Ctrl Pts',(2.63015446617675,6.23494799369253,34.6759386040299));
#17882=CARTESIAN_POINT('Ctrl Pts',(2.47105778204377,6.30206144111015,34.6840780460302));
#17883=CARTESIAN_POINT('Ctrl Pts',(2.30919947399828,6.36316205833891,34.6922174880306));
#17884=CARTESIAN_POINT('Ctrl Pts',(2.14507860761712,6.41801579673527,34.7003569300309));
#17885=CARTESIAN_POINT('Ctrl Pts',(1.98109793576011,6.47282267823937,34.7084894191969));
#17886=CARTESIAN_POINT('Ctrl Pts',(1.81485889836932,6.52139319002899,34.7166219083629));
#17887=CARTESIAN_POINT('Ctrl Pts',(1.64688117360616,6.56354107170981,34.7247543975289));
#17888=CARTESIAN_POINT('Ctrl Pts',(1.47901164815922,6.60566180471968,34.7328816483232));
#17889=CARTESIAN_POINT('Ctrl Pts',(1.30940601892574,6.64136805707052,34.7410088991174));
#17890=CARTESIAN_POINT('Ctrl Pts',(1.13859978220374,6.67052318307684,34.7491361499117));
#17891=CARTESIAN_POINT('Ctrl Pts',(0.967867693566158,6.69966565265571,34.7572598726141));
#17892=CARTESIAN_POINT('Ctrl Pts',(0.795936395311186,6.72226259879266,34.7653835953166));
#17893=CARTESIAN_POINT('Ctrl Pts',(0.623352247553659,6.73822832616036,34.7735073180191));
#17894=CARTESIAN_POINT('Ctrl Pts',(0.450776092652785,6.75419331411038,34.7816306644892));
#17895=CARTESIAN_POINT('Ctrl Pts',(0.27754751151336,6.76352765156302,34.7897540109592));
#17896=CARTESIAN_POINT('Ctrl Pts',(0.10421895937072,6.76619741128706,34.7978773574293));
#17897=CARTESIAN_POINT('Ctrl Pts',(-0.0691143255496477,6.76886724390953,
34.8060009257093));
#17898=CARTESIAN_POINT('Ctrl Pts',(-0.242547221102038,6.76487212990511,
34.8141244939893));
#17899=CARTESIAN_POINT('Ctrl Pts',(-0.415526524812408,6.75423028236211,
34.8222480622693));
#17900=CARTESIAN_POINT('Ctrl Pts',(-0.588543460688567,6.74358611965329,
34.8303733978559));
#17901=CARTESIAN_POINT('Ctrl Pts',(-0.761106243098924,6.7262923662018,34.8384987334425));
#17902=CARTESIAN_POINT('Ctrl Pts',(-0.932666087647813,6.70241918779718,
34.8466240690291));
#17903=CARTESIAN_POINT('Ctrl Pts',(-1.10429589693067,6.67853627354451,34.8547527182521));
#17904=CARTESIAN_POINT('Ctrl Pts',(-1.27492159193006,6.6480686416746,34.8628813674751));
#17905=CARTESIAN_POINT('Ctrl Pts',(-1.44400392512547,6.61113769817437,34.871010016698));
#17906=CARTESIAN_POINT('Ctrl Pts',(-1.61328476000066,6.57416339796038,34.8791482089081));
#17907=CARTESIAN_POINT('Ctrl Pts',(-1.7810182570976,6.53071071045453,34.8872864011182));
#17908=CARTESIAN_POINT('Ctrl Pts',(-1.94667882281563,6.48095136232337,34.8954245933283));
#17909=CARTESIAN_POINT('Ctrl Pts',(-2.11244759646717,6.43115951185099,34.9035681013295));
#17910=CARTESIAN_POINT('Ctrl Pts',(-2.27614039622114,6.37505291156961,34.9117116093307));
#17911=CARTESIAN_POINT('Ctrl Pts',(-2.43725129985825,6.31285158239439,34.9198551173319));
#17912=CARTESIAN_POINT('Ctrl Pts',(-2.59860229952536,6.25055755749305,34.9280107612215));
#17913=CARTESIAN_POINT('Ctrl Pts',(-2.75736338394079,6.18215080816633,34.9361664051111));
#17914=CARTESIAN_POINT('Ctrl Pts',(-2.91305202609664,6.10789791116831,34.9443220490006));
#17915=CARTESIAN_POINT('Ctrl Pts',(-3.00228537832362,6.06533966915433,34.9489964776151));
#17916=CARTESIAN_POINT('Ctrl Pts',(-3.09050991945001,6.02086176861545,34.9536709062295));
#17917=CARTESIAN_POINT('Ctrl Pts',(-3.17763918594097,5.97452075098685,34.9583453348439));
#17918=CARTESIAN_POINT('Ctrl Pts',(-3.33109957183084,5.89290052469292,34.9665783849759));
#17919=CARTESIAN_POINT('Ctrl Pts',(-3.4816375613256,5.80524455240668,34.974811435108));
#17920=CARTESIAN_POINT('Ctrl Pts',(-3.62874575691539,5.71178546793108,34.98304448524));
#17921=CARTESIAN_POINT('Ctrl Pts',(-3.77567876925723,5.61843767885884,34.9912677310748));
#17922=CARTESIAN_POINT('Ctrl Pts',(-3.91918982129634,5.51930072852775,34.9994909769097));
#17923=CARTESIAN_POINT('Ctrl Pts',(-4.05879438461281,5.41465392646987,35.0077142227446));
#17924=CARTESIAN_POINT('Ctrl Pts',(-4.1982606425083,5.3101107973842,35.0159293218581));
#17925=CARTESIAN_POINT('Ctrl Pts',(-4.33382783447221,5.20006890075457,35.0241444209716));
#17926=CARTESIAN_POINT('Ctrl Pts',(-4.46503872804362,5.08485183236155,35.0323595200851));
#17927=CARTESIAN_POINT('Ctrl Pts',(-4.59614588440986,4.96972585622724,35.040568124224));
#17928=CARTESIAN_POINT('Ctrl Pts',(-4.72290333451079,4.84943309318149,35.0487767283629));
#17929=CARTESIAN_POINT('Ctrl Pts',(-4.84488531226018,4.72433861096403,35.0569853325018));
#17930=CARTESIAN_POINT('Ctrl Pts',(-4.96679524911309,4.59931800784586,35.0651890887508));
#17931=CARTESIAN_POINT('Ctrl Pts',(-5.08393508270115,4.46950159067045,35.0733928449997));
#17932=CARTESIAN_POINT('Ctrl Pts',(-5.19591438652508,4.33529268768578,35.0815966012487));
#17933=CARTESIAN_POINT('Ctrl Pts',(-5.3078605584955,4.20112349373268,35.089797930213));
#17934=CARTESIAN_POINT('Ctrl Pts',(-5.41464901003014,4.06256467497881,35.0979992591773));
#17935=CARTESIAN_POINT('Ctrl Pts',(-5.51592809443204,3.92005436914532,35.1062005881416));
#17936=CARTESIAN_POINT('Ctrl Pts',(-5.61719321148133,3.7775637168435,35.1144007860643));
#17937=CARTESIAN_POINT('Ctrl Pts',(-5.71295026651222,3.63112295428702,35.122600983987));
#17938=CARTESIAN_POINT('Ctrl Pts',(-5.80288962786727,3.48120108106247,35.1308011819097));
#17939=CARTESIAN_POINT('Ctrl Pts',(-5.89283288456784,3.33127271460192,35.1390017349896));
#17940=CARTESIAN_POINT('Ctrl Pts',(-5.97695776123205,3.17786324432855,35.1472022880694));
#17941=CARTESIAN_POINT('Ctrl Pts',(-6.05499944232427,3.02146831084704,35.1554028411492));
#17942=CARTESIAN_POINT('Ctrl Pts',(-6.13305864614557,2.86503826195012,35.1636052355025));
#17943=CARTESIAN_POINT('Ctrl Pts',(-6.20503177404148,2.70562173526347,35.1718076298557));
#17944=CARTESIAN_POINT('Ctrl Pts',(-6.27070119280544,2.54373653324168,35.1800100242089));
#17945=CARTESIAN_POINT('Ctrl Pts',(-6.33643202401997,2.38169994009822,35.1882200892427));
#17946=CARTESIAN_POINT('Ctrl Pts',(-6.39584723337748,2.21719039157581,35.1964301542766));
#17947=CARTESIAN_POINT('Ctrl Pts',(-6.44877802302472,2.05074401370658,35.2046402193104));
#17948=CARTESIAN_POINT('Ctrl Pts',(-6.50173414440882,1.88421797755389,35.2128542135357));
#17949=CARTESIAN_POINT('Ctrl Pts',(-6.54819956334234,1.71575360909952,35.221068207761));
#17950=CARTESIAN_POINT('Ctrl Pts',(-6.58805614454478,1.54589949101675,35.2292822019863));
#17951=CARTESIAN_POINT('Ctrl Pts',(-6.62796706354206,1.37581380519926,35.2375073946215));
#17952=CARTESIAN_POINT('Ctrl Pts',(-6.66125106982199,1.20433493500494,35.2457325872567));
#17953=CARTESIAN_POINT('Ctrl Pts',(-6.68784146855085,1.03202010229044,35.2539577798919));
#17954=CARTESIAN_POINT('Ctrl Pts',(-6.7117541571757,0.877057742298748,35.2613546780118));
#17955=CARTESIAN_POINT('Ctrl Pts',(-6.73025415764975,0.721419572584288,
35.2687515761317));
#17956=CARTESIAN_POINT('Ctrl Pts',(-6.74332896696352,0.565511665052691,
35.2761484742516));
#17957=CARTESIAN_POINT('Ctrl Pts',(-6.75904402005099,0.378120707003798,
35.2850390548977));
#17958=CARTESIAN_POINT('Ctrl Pts',(-6.76694755464435,0.190076741669039,
35.2939296355438));
#17959=CARTESIAN_POINT('Ctrl Pts',(-6.76699973985222,0.00187639016204831,
35.3028202161899));
#17960=CARTESIAN_POINT('Ctrl Pts',(-6.76699973985247,0.00187638925439036,
35.3028202162328));
#17961=CARTESIAN_POINT('Ctrl Pts',(-6.76704855127815,-0.17415686403976,
35.3111360234152));
#17962=CARTESIAN_POINT('Ctrl Pts',(-6.76022425514039,-0.350411533394409,
35.3194518305977));
#17963=CARTESIAN_POINT('Ctrl Pts',(-6.74650123491233,-0.526317477694271,
35.3277676377801));
#17964=CARTESIAN_POINT('Ctrl Pts',(-6.73279357865191,-0.702026481875204,
35.3360741347822));
#17965=CARTESIAN_POINT('Ctrl Pts',(-6.71220261027407,-0.877387194927201,
35.3443806317844));
#17966=CARTESIAN_POINT('Ctrl Pts',(-6.6847547233564,-1.05182854523171,35.3526871287865));
#17967=CARTESIAN_POINT('Ctrl Pts',(-6.65733965931409,-1.22606129417046,
35.3609836926701));
#17968=CARTESIAN_POINT('Ctrl Pts',(-6.62308407785982,-1.39937653084823,
35.3692802565536));
#17969=CARTESIAN_POINT('Ctrl Pts',(-6.5820662189394,-1.57120758956186,35.3775768204372));
#17970=CARTESIAN_POINT('Ctrl Pts',(-6.54107691905235,-1.74291900943844,
35.3858676077675));
#17971=CARTESIAN_POINT('Ctrl Pts',(-6.49333479971102,-1.91314797307148,
35.3941583950978));
#17972=CARTESIAN_POINT('Ctrl Pts',(-6.43896942157368,-2.08133653887091,
35.4024491824282));
#17973=CARTESIAN_POINT('Ctrl Pts',(-6.38463862630875,-2.24941811665863,
35.4107346958278));
#17974=CARTESIAN_POINT('Ctrl Pts',(-6.3236930770421,-2.41546155410251,35.4190202092273));
#17975=CARTESIAN_POINT('Ctrl Pts',(-6.25631258088812,-2.57892262199181,
35.4273057226269));
#17976=CARTESIAN_POINT('Ctrl Pts',(-6.23531946562246,-2.62985066846694,
35.4298871630698));
#17977=CARTESIAN_POINT('Ctrl Pts',(-6.21370207339749,-2.68052815658692,
35.4324686035126));
#17978=CARTESIAN_POINT('Ctrl Pts',(-6.19146682236525,-2.73093895712636,
35.4350500439555));
#17979=CARTESIAN_POINT('Ctrl Pts',(-6.11742721885216,-2.89879834757379,
35.4436458015031));
#17980=CARTESIAN_POINT('Ctrl Pts',(-6.03660075632427,-3.06354650195075,
35.4522415590507));
#17981=CARTESIAN_POINT('Ctrl Pts',(-5.94928238480897,-3.2246438727093,35.4608373165982));
#17982=CARTESIAN_POINT('Ctrl Pts',(-5.86188254228419,-3.38589155279215,
35.4694410942799));
#17983=CARTESIAN_POINT('Ctrl Pts',(-5.76797884592166,-3.54348138173558,
35.4780448719615));
#17984=CARTESIAN_POINT('Ctrl Pts',(-5.66791063371377,-3.69690114125796,
35.4866486496431));
#17985=CARTESIAN_POINT('Ctrl Pts',(-5.56390965326238,-3.85635043148607,
35.4955905633111));
#17986=CARTESIAN_POINT('Ctrl Pts',(-5.45325003331208,-4.01129494083088,
35.5045324769791));
#17987=CARTESIAN_POINT('Ctrl Pts',(-5.33635924956896,-4.161196818169,35.5134743906471));
#17988=CARTESIAN_POINT('Ctrl Pts',(-5.2235824459241,-4.30582288743815,35.5221015929778));
#17989=CARTESIAN_POINT('Ctrl Pts',(-5.10500584471209,-4.44575503210426,
35.5307287953086));
#17990=CARTESIAN_POINT('Ctrl Pts',(-4.98105186195777,-4.58054705777455,
35.5393559976393));
#17991=CARTESIAN_POINT('Ctrl Pts',(-4.85697983200792,-4.71546745221731,
35.5479914160597));
#17992=CARTESIAN_POINT('Ctrl Pts',(-4.72752041134947,-4.84523773852067,
35.5566268344801));
#17993=CARTESIAN_POINT('Ctrl Pts',(-4.59313160217126,-4.96944977690043,
35.5652622529005));
#17994=CARTESIAN_POINT('Ctrl Pts',(-4.4585442526691,-5.0938453208748,35.5739104289216));
#17995=CARTESIAN_POINT('Ctrl Pts',(-4.31901319114098,-5.21266600657686,
35.5825586049427));
#17996=CARTESIAN_POINT('Ctrl Pts',(-4.17502923641397,-5.32554409192982,
35.5912067809639));
#17997=CARTESIAN_POINT('Ctrl Pts',(-4.15979627994705,-5.33748616536092,
35.5921217251957));
#17998=CARTESIAN_POINT('Ctrl Pts',(-4.14451350921705,-5.34936176450257,
35.5930366694274));
#17999=CARTESIAN_POINT('Ctrl Pts',(-4.12918152370299,-5.36117048267539,
35.5939516136592));
#18000=CARTESIAN_POINT('Ctrl Pts',(-3.99133618395422,-5.46733916950572,
35.6021776062006));
#18001=CARTESIAN_POINT('Ctrl Pts',(-3.84921261207773,-5.56832741115146,
35.6104035987419));
#18002=CARTESIAN_POINT('Ctrl Pts',(-3.70323664277618,-5.66377324471944,
35.6186295912833));
#18003=CARTESIAN_POINT('Ctrl Pts',(-3.55741371041034,-5.75911901566777,
35.6268469599347));
#18004=CARTESIAN_POINT('Ctrl Pts',(-3.40774672066166,-5.8489337549284,35.6350643285861));
#18005=CARTESIAN_POINT('Ctrl Pts',(-3.25469406681355,-5.93289604927043,
35.6432816972375));
#18006=CARTESIAN_POINT('Ctrl Pts',(-3.10177124371692,-6.0167871204909,35.6514920952999));
#18007=CARTESIAN_POINT('Ctrl Pts',(-2.94546878880561,-6.09483546287145,
35.6597024933623));
#18008=CARTESIAN_POINT('Ctrl Pts',(-2.78627360760646,-6.16676320151469,
35.6679128914247));
#18009=CARTESIAN_POINT('Ctrl Pts',(-2.62718162241656,-6.23864431402562,
35.6761179672135));
#18010=CARTESIAN_POINT('Ctrl Pts',(-2.46520097147916,-6.30441257896438,
35.6843230430023));
#18011=CARTESIAN_POINT('Ctrl Pts',(-2.30084275109753,-6.36383623569321,
35.692528118791));
#18012=CARTESIAN_POINT('Ctrl Pts',(-2.13655820216616,-6.42323325653514,
35.7007295167605));
#18013=CARTESIAN_POINT('Ctrl Pts',(-1.96989854324486,-6.47629121346023,
35.70893091473));
#18014=CARTESIAN_POINT('Ctrl Pts',(-1.80139450711859,-6.52282659816455,
35.7171323126995));
#18015=CARTESIAN_POINT('Ctrl Pts',(-1.63290366963153,-6.56935833783006,
35.7253330682672));
#18016=CARTESIAN_POINT('Ctrl Pts',(-1.46256908546389,-6.6093684192243,35.7335338238349));
#18017=CARTESIAN_POINT('Ctrl Pts',(-1.29093666061151,-6.64272320199248,
35.7417345794026));
#18018=CARTESIAN_POINT('Ctrl Pts',(-1.1193051075701,-6.67607781533425,35.7499352933144));
#18019=CARTESIAN_POINT('Ctrl Pts',(-0.946376078563808,-6.70277712797335,
35.7581360072262));
#18020=CARTESIAN_POINT('Ctrl Pts',(-0.772705567099336,-6.72273866118368,
35.766336721138));
#18021=CARTESIAN_POINT('Ctrl Pts',(-0.599004464377042,-6.74270371052581,
35.7745388795676));
#18022=CARTESIAN_POINT('Ctrl Pts',(-0.424561975015007,-6.75592857496403,
35.7827410379972));
#18023=CARTESIAN_POINT('Ctrl Pts',(-0.249939166465919,-6.76238267277639,
35.7909431964268));
#18024=CARTESIAN_POINT('Ctrl Pts',(-0.0752539525814367,-6.76883907710381,
35.7991482860798));
#18025=CARTESIAN_POINT('Ctrl Pts',(0.0996113509594036,-6.76851988142677,
35.8073533757327));
#18026=CARTESIAN_POINT('Ctrl Pts',(0.274095664471448,-6.76144663269022,
35.8155584653856));
#18027=CARTESIAN_POINT('Ctrl Pts',(0.448779305682482,-6.75436530360326,
35.8237729283834));
#18028=CARTESIAN_POINT('Ctrl Pts',(0.623080728898286,-6.7405145213614,35.8319873913812));
#18029=CARTESIAN_POINT('Ctrl Pts',(0.796442896387099,-6.71996783569643,
35.840201854379));
#18030=CARTESIAN_POINT('Ctrl Pts',(0.969907775480884,-6.6994089767696,35.8484211841865));
#18031=CARTESIAN_POINT('Ctrl Pts',(1.14243193618498,-6.6721463622853,35.856640513994));
#18032=CARTESIAN_POINT('Ctrl Pts',(1.3134686276419,-6.63830469052156,35.8648598438014));
#18033=CARTESIAN_POINT('Ctrl Pts',(1.48477033008232,-6.60441058313923,35.8730919089621));
#18034=CARTESIAN_POINT('Ctrl Pts',(1.65457960914523,-6.56391713025827,35.8813239741228));
#18035=CARTESIAN_POINT('Ctrl Pts',(1.82236367117798,-6.5169992826431,35.8895560392835));
#18036=CARTESIAN_POINT('Ctrl Pts',(1.9731800336904,-6.4748261523201,35.8969556105447));
#18037=CARTESIAN_POINT('Ctrl Pts',(2.12236013454246,-6.42746302867524,35.9043551818058));
#18038=CARTESIAN_POINT('Ctrl Pts',(2.26953171457694,-6.37506978758111,35.911754753067));
#18039=CARTESIAN_POINT('Ctrl Pts',(2.4317372880176,-6.31732442863275,35.9199102114738));
#18040=CARTESIAN_POINT('Ctrl Pts',(2.5920021076197,-6.25329016858809,35.9280656698806));
#18041=CARTESIAN_POINT('Ctrl Pts',(2.74979703189377,-6.18311452937662,35.9362211282874));
#18042=CARTESIAN_POINT('Ctrl Pts',(2.90739989900286,-6.11302430314265,35.9443666604293));
#18043=CARTESIAN_POINT('Ctrl Pts',(3.062538524441,-6.03680772369536,35.9525121925711));
#18044=CARTESIAN_POINT('Ctrl Pts',(3.21469893288176,-5.95466201987391,35.960657724713));
#18045=CARTESIAN_POINT('Ctrl Pts',(3.36670613838588,-5.87259902457821,35.9687950555135));
#18046=CARTESIAN_POINT('Ctrl Pts',(3.51574077739738,-5.78461896195355,35.9769323863141));
#18047=CARTESIAN_POINT('Ctrl Pts',(3.66130888248412,-5.69096707660859,35.9850697171147));
#18048=CARTESIAN_POINT('Ctrl Pts',(3.80676101369243,-5.59738980357214,35.9932005649167));
#18049=CARTESIAN_POINT('Ctrl Pts',(3.94875180407487,-5.49814990200906,36.0013314127187));
#18050=CARTESIAN_POINT('Ctrl Pts',(4.08681194261969,-5.39353846242531,36.0094622605207));
#18051=CARTESIAN_POINT('Ctrl Pts',(4.22479109079321,-5.28898839116569,36.0175883385145));
#18052=CARTESIAN_POINT('Ctrl Pts',(4.3588438885813,-5.17907327744657,36.0257144165083));
#18053=CARTESIAN_POINT('Ctrl Pts',(4.48853008911084,-5.06412743117179,36.0338404945021));
#18054=CARTESIAN_POINT('Ctrl Pts',(4.61867613322107,-4.94877400792029,36.0419953860843));
#18055=CARTESIAN_POINT('Ctrl Pts',(4.74442424754717,-4.82835431686768,36.0501502776665));
#18056=CARTESIAN_POINT('Ctrl Pts',(4.86536263050205,-4.7032473328238,36.0583051692487));
#18057=CARTESIAN_POINT('Ctrl Pts',(4.98582939604845,-4.57862822227513,36.066428259605));
#18058=CARTESIAN_POINT('Ctrl Pts',(5.1015236317425,-4.44935858744685,36.0745513499613));
#18059=CARTESIAN_POINT('Ctrl Pts',(5.21207521702403,-4.31584996635471,36.0826744403176));
#18060=CARTESIAN_POINT('Ctrl Pts',(5.32263548332115,-4.18233086155563,36.0907981685361));
#18061=CARTESIAN_POINT('Ctrl Pts',(5.42805206148019,-4.04457238920789,36.0989218967546));
#18062=CARTESIAN_POINT('Ctrl Pts',(5.52799524678218,-3.90301903038579,36.107045624973));
#18063=CARTESIAN_POINT('Ctrl Pts',(5.62796529415142,-3.76142762578967,36.1151715366334));
#18064=CARTESIAN_POINT('Ctrl Pts',(5.72245880851381,-3.616039602499,36.1232974482937));
#18065=CARTESIAN_POINT('Ctrl Pts',(5.81118955509305,-3.46732821561176,36.131423359954));
#18066=CARTESIAN_POINT('Ctrl Pts',(5.90048774401992,-3.31766580394733,36.1396012376641));
#18067=CARTESIAN_POINT('Ctrl Pts',(5.98394900987722,-3.16463769718322,36.1477791153741));
#18068=CARTESIAN_POINT('Ctrl Pts',(6.06132904545269,-3.00875043876217,36.1559569930842));
#18069=CARTESIAN_POINT('Ctrl Pts',(6.13833976290137,-2.85360719641508,36.1640958395576));
#18070=CARTESIAN_POINT('Ctrl Pts',(6.20932707781422,-2.69563239375103,36.1722346860311));
#18071=CARTESIAN_POINT('Ctrl Pts',(6.27409909513282,-2.53534406825849,36.1803735325045));
#18072=CARTESIAN_POINT('Ctrl Pts',(6.33933705045781,-2.37390270745969,36.1885709258329));
#18073=CARTESIAN_POINT('Ctrl Pts',(6.39826982357931,-2.21011476910446,36.1967683191613));
#18074=CARTESIAN_POINT('Ctrl Pts',(6.45075295252284,-2.04452325629177,36.2049657124896));
#18075=CARTESIAN_POINT('Ctrl Pts',(6.50323608146636,-1.87893174347908,36.213163105818));
#18076=CARTESIAN_POINT('Ctrl Pts',(6.54926952645588,-1.7115370313218,36.2213604991463));
#18077=CARTESIAN_POINT('Ctrl Pts',(6.5887615325862,-1.54289029639584,36.2295578924747));
#18078=CARTESIAN_POINT('Ctrl Pts',(6.62839236357748,-1.3736507235307,36.2377841018117));
#18079=CARTESIAN_POINT('Ctrl Pts',(6.66155374818316,-1.20264664996418,36.2460103111486));
#18080=CARTESIAN_POINT('Ctrl Pts',(6.68808915414159,-1.03041373547409,36.2542365204856));
#18081=CARTESIAN_POINT('Ctrl Pts',(6.71459474870817,-0.858374317285196,
36.2624534880288));
#18082=CARTESIAN_POINT('Ctrl Pts',(6.73448913354669,-0.68510915845815,36.270670455572));
#18083=CARTESIAN_POINT('Ctrl Pts',(6.74766605066327,-0.511167163192595,
36.2788874231152));
#18084=CARTESIAN_POINT('Ctrl Pts',(6.76083080879079,-0.337385672755159,
36.2870968084586));
#18085=CARTESIAN_POINT('Ctrl Pts',(6.76729041689434,-0.162928945058542,
36.2953061938019));
#18086=CARTESIAN_POINT('Ctrl Pts',(6.76698997898025,0.0116457881213388,
36.3035155791453));
#18087=CARTESIAN_POINT('Ctrl Pts',(6.76668975801404,0.186094459915643,36.3117190364459));
#18088=CARTESIAN_POINT('Ctrl Pts',(6.75963921468863,0.360660610282066,36.3199224937465));
#18089=CARTESIAN_POINT('Ctrl Pts',(6.74583541268007,0.534783680595766,36.3281259510471));
#18090=CARTESIAN_POINT('Ctrl Pts',(6.73203880946492,0.708815944332309,36.3363251301789));
#18091=CARTESIAN_POINT('Ctrl Pts',(6.71149599205064,0.88240523168416,36.3445243093107));
#18092=CARTESIAN_POINT('Ctrl Pts',(6.68425608562888,1.0549926927393,36.3527234884425));
#18093=CARTESIAN_POINT('Ctrl Pts',(6.65702131179242,1.22754763459811,36.3609211226723));
#18094=CARTESIAN_POINT('Ctrl Pts',(6.6230920121863,1.39910077130668,36.3691187569021));
#18095=CARTESIAN_POINT('Ctrl Pts',(6.58256902214978,1.56909976376078,36.3773163911319));
#18096=CARTESIAN_POINT('Ctrl Pts',(6.54204895710705,1.73908648550145,36.3855134336475));
#18097=CARTESIAN_POINT('Ctrl Pts',(6.49493623180321,1.90751893729221,36.3937104761631));
#18098=CARTESIAN_POINT('Ctrl Pts',(6.44138251058095,2.07385639627768,36.4019075186787));
#18099=CARTESIAN_POINT('Ctrl Pts',(6.38782292162592,2.24021208039742,36.4101054593216));
#18100=CARTESIAN_POINT('Ctrl Pts',(6.32782104069586,2.40447197290469,36.4183033999644));
#18101=CARTESIAN_POINT('Ctrl Pts',(6.26157799339354,2.56611185115726,36.4265013406072));
#18102=CARTESIAN_POINT('Ctrl Pts',(6.19531564841639,2.72779881772985,36.4347016694432));
#18103=CARTESIAN_POINT('Ctrl Pts',(6.12280865150704,2.88686391793369,36.4429019982792));
#18104=CARTESIAN_POINT('Ctrl Pts',(6.04430574102376,3.04280415226272,36.4511023271151));
#18105=CARTESIAN_POINT('Ctrl Pts',(5.96572102847087,3.19890688036204,36.4593112009065));
#18106=CARTESIAN_POINT('Ctrl Pts',(5.88112808148358,3.35187791641154,36.467520074698));
#18107=CARTESIAN_POINT('Ctrl Pts',(5.79082145492598,3.50123919165329,36.4757289484894));
#18108=CARTESIAN_POINT('Ctrl Pts',(5.70046636179806,3.65068062744389,36.4839422278928));
#18109=CARTESIAN_POINT('Ctrl Pts',(5.60439167312652,3.79650814108492,36.4921555072962));
#18110=CARTESIAN_POINT('Ctrl Pts',(5.50293447000345,3.93827388824697,36.5003687866996));
#18111=CARTESIAN_POINT('Ctrl Pts',(5.40132886977468,4.0802469900957,36.5085940793151));
#18112=CARTESIAN_POINT('Ctrl Pts',(5.29432524174133,4.21814616946329,36.5168193719305));
#18113=CARTESIAN_POINT('Ctrl Pts',(5.18230084647513,4.35155684055984,36.5250446645459));
#18114=CARTESIAN_POINT('Ctrl Pts',(5.08098823782267,4.47221076668682,36.5324834536581));
#18115=CARTESIAN_POINT('Ctrl Pts',(4.97556975815014,4.58919384948255,36.5399222427702));
#18116=CARTESIAN_POINT('Ctrl Pts',(4.8663490095192,4.70222674033819,36.5473610318823));
#18117=CARTESIAN_POINT('Ctrl Pts',(4.74553618816832,4.82725630313545,36.5555893320115));
#18118=CARTESIAN_POINT('Ctrl Pts',(4.61973284761794,4.94780166435287,36.5638176321407));
#18119=CARTESIAN_POINT('Ctrl Pts',(4.4893047183625,5.06344074179685,36.5720459322699));
#18120=CARTESIAN_POINT('Ctrl Pts',(4.35906136466715,5.17891599510699,36.5802625754906));
#18121=CARTESIAN_POINT('Ctrl Pts',(4.22420654514427,5.28949858003894,36.5884792187114));
#18122=CARTESIAN_POINT('Ctrl Pts',(4.08514403561056,5.3948018692363,36.5966958619321));
#18123=CARTESIAN_POINT('Ctrl Pts',(3.94619570525636,5.50001869772473,36.6049057587653));
#18124=CARTESIAN_POINT('Ctrl Pts',(3.80304684589757,5.59996464364973,36.6131156555985));
#18125=CARTESIAN_POINT('Ctrl Pts',(3.65613618718165,5.6942916311672,36.6213255524317));
#18126=CARTESIAN_POINT('Ctrl Pts',(3.50934064317129,5.78854470693798,36.6295290162404));
#18127=CARTESIAN_POINT('Ctrl Pts',(3.35878947344755,5.87718740374395,36.6377324800492));
#18128=CARTESIAN_POINT('Ctrl Pts',(3.20495227163709,5.95991358465274,36.6459359438579));
#18129=CARTESIAN_POINT('Ctrl Pts',(3.16986235065928,5.97878324112545,36.6478071355684));
#18130=CARTESIAN_POINT('Ctrl Pts',(3.1346015831711,5.99734524642513,36.6496783272789));
#18131=CARTESIAN_POINT('Ctrl Pts',(3.09917575053261,6.01559628526638,36.6515495189894));
#18132=CARTESIAN_POINT('Origin',(0.,0.,-3.69717978381041));
#18133=CARTESIAN_POINT('',(3.09917575053254,6.01559628526642,39.0455765095777));
#18134=CARTESIAN_POINT('',(3.09917575053265,6.01559628526636,38.651392015122));
#18135=CARTESIAN_POINT('',(3.09917575053259,6.01559628526639,-3.69717978381041));
#18136=CARTESIAN_POINT('',(-6.767,1.02740353117442E-12,37.6971797838101));
#18137=CARTESIAN_POINT('Ctrl Pts',(-6.7669999895289,-0.000376451654302756,
37.6971797838101));
#18138=CARTESIAN_POINT('Ctrl Pts',(-6.76698972560559,-0.184878148371141,
37.7058050730204));
#18139=CARTESIAN_POINT('Ctrl Pts',(-6.75942954819334,-0.369194955863458,
37.7144303622308));
#18140=CARTESIAN_POINT('Ctrl Pts',(-6.74439035844876,-0.552709410869264,
37.7230556514411));
#18141=CARTESIAN_POINT('Ctrl Pts',(-6.72932680744503,-0.736521132102261,
37.7316949123421));
#18142=CARTESIAN_POINT('Ctrl Pts',(-6.70676007374303,-0.919527610808517,
37.740334173243));
#18143=CARTESIAN_POINT('Ctrl Pts',(-6.67681236999359,-1.101120145988,37.7489734341439));
#18144=CARTESIAN_POINT('Ctrl Pts',(-6.64678371593247,-1.28320353590694,
37.7576360474484));
#18145=CARTESIAN_POINT('Ctrl Pts',(-6.60933423103168,-1.46386504386166,
37.7662986607528));
#18146=CARTESIAN_POINT('Ctrl Pts',(-6.56463702324489,-1.64250715463966,
37.7749612740573));
#18147=CARTESIAN_POINT('Ctrl Pts',(-6.51987617494603,-1.82140361856344,
37.7836362213122));
#18148=CARTESIAN_POINT('Ctrl Pts',(-6.46784708064659,-1.99827466048662,
37.7923111685671));
#18149=CARTESIAN_POINT('Ctrl Pts',(-6.40877185034757,-2.17254053361327,
37.800986115822));
#18150=CARTESIAN_POINT('Ctrl Pts',(-6.34955095524285,-2.34723610298352,
37.8096824533364));
#18151=CARTESIAN_POINT('Ctrl Pts',(-6.28324927916287,-2.51931337808984,
37.8183787908509));
#18152=CARTESIAN_POINT('Ctrl Pts',(-6.21013697863793,-2.68821273461639,
37.8270751283653));
#18153=CARTESIAN_POINT('Ctrl Pts',(-6.15845308467603,-2.8076095580001,37.8332226655475));
#18154=CARTESIAN_POINT('Ctrl Pts',(-6.10336673855936,-2.92541880724379,
37.8393702027297));
#18155=CARTESIAN_POINT('Ctrl Pts',(-6.04498666341758,-3.04145117322366,
37.8455177399119));
#18156=CARTESIAN_POINT('Ctrl Pts',(-5.96687922318279,-3.1966923418769,37.8537426075895));
#18157=CARTESIAN_POINT('Ctrl Pts',(-5.88267816686097,-3.34914070709008,
37.8619674752671));
#18158=CARTESIAN_POINT('Ctrl Pts',(-5.79260661415228,-3.49828495318481,
37.8701923429446));
#18159=CARTESIAN_POINT('Ctrl Pts',(-5.70263653712959,-3.64726117159235,
37.8784079443882));
#18160=CARTESIAN_POINT('Ctrl Pts',(-5.60680931720374,-3.79294037893727,
37.8866235458317));
#18161=CARTESIAN_POINT('Ctrl Pts',(-5.50539515313227,-3.93483331386067,
37.8948391472752));
#18162=CARTESIAN_POINT('Ctrl Pts',(-5.40407486732728,-4.07659489964878,
37.9030471436034));
#18163=CARTESIAN_POINT('Ctrl Pts',(-5.29717814439985,-4.21457690309378,
37.9112551399315));
#18164=CARTESIAN_POINT('Ctrl Pts',(-5.18501994507776,-4.34831659026178,
37.9194631362596));
#18165=CARTESIAN_POINT('Ctrl Pts',(-5.07294304213086,-4.4819593380009,37.927665183131));
#18166=CARTESIAN_POINT('Ctrl Pts',(-4.95561248858411,-4.61136562047138,
37.9358672300025));
#18167=CARTESIAN_POINT('Ctrl Pts',(-4.83338525976377,-4.73610345439141,
37.9440692768739));
#18168=CARTESIAN_POINT('Ctrl Pts',(-4.71122208139883,-4.86077592222941,
37.9522670256455));
#18169=CARTESIAN_POINT('Ctrl Pts',(-4.58416759013228,-4.98078455948131,
37.960464774417));
#18170=CARTESIAN_POINT('Ctrl Pts',(-4.45261762527738,-5.09573206547099,
37.9686625231886));
#18171=CARTESIAN_POINT('Ctrl Pts',(-4.32109275093618,-5.21065764753256,
37.9768587084042));
#18172=CARTESIAN_POINT('Ctrl Pts',(-4.18507437668023,-5.32052378059402,
37.9850548936199));
#18173=CARTESIAN_POINT('Ctrl Pts',(-4.04499385664279,-5.42497130865427,
37.9932510788355));
#18174=CARTESIAN_POINT('Ctrl Pts',(-3.90492369944608,-5.52941110992213,
38.0014466577158));
#18175=CARTESIAN_POINT('Ctrl Pts',(-3.7607922820659,-5.62843288929932,38.0096422365962));
#18176=CARTESIAN_POINT('Ctrl Pts',(-3.61306252342612,-5.72171899011247,
38.0178378154765));
#18177=CARTESIAN_POINT('Ctrl Pts',(-3.46531681582039,-5.81501516213172,
38.0260342791549));
#18178=CARTESIAN_POINT('Ctrl Pts',(-3.3139722964519,-5.90257423027229,38.0342307428334));
#18179=CARTESIAN_POINT('Ctrl Pts',(-3.15951926684773,-5.98412291003602,
38.0424272065118));
#18180=CARTESIAN_POINT('Ctrl Pts',(-3.00502146141335,-6.0656952307076,38.0506260463396));
#18181=CARTESIAN_POINT('Ctrl Pts',(-2.84741366799579,-6.1412535248539,38.0588248861674));
#18182=CARTESIAN_POINT('Ctrl Pts',(-2.68720912256893,-6.21057132086754,
38.0670237259952));
#18183=CARTESIAN_POINT('Ctrl Pts',(-2.52683723893663,-6.27996152129117,
38.0752311297444));
#18184=CARTESIAN_POINT('Ctrl Pts',(-2.36386351407683,-6.34309805802945,
38.0834385334936));
#18185=CARTESIAN_POINT('Ctrl Pts',(-2.19882036682686,-6.39980296528162,
38.0916459372429));
#18186=CARTESIAN_POINT('Ctrl Pts',(-2.03368881373325,-6.4565382466829,38.0998577373119));
#18187=CARTESIAN_POINT('Ctrl Pts',(-1.86648597173678,-6.50683492739292,
38.1080695373809));
#18188=CARTESIAN_POINT('Ctrl Pts',(-1.69775751610964,-6.55056550356481,
38.1162813374499));
#18189=CARTESIAN_POINT('Ctrl Pts',(-1.52878066861958,-6.59436045725524,
38.1245052264361));
#18190=CARTESIAN_POINT('Ctrl Pts',(-1.35827406968175,-6.63156991222203,
38.1327291154222));
#18191=CARTESIAN_POINT('Ctrl Pts',(-1.18679291955195,-6.66211764877365,
38.1409530044084));
#18192=CARTESIAN_POINT('Ctrl Pts',(-1.02834730136684,-6.69034322924366,
38.1485517356585));
#18193=CARTESIAN_POINT('Ctrl Pts',(-0.869069958548886,-6.71288195291813,
38.1561504669086));
#18194=CARTESIAN_POINT('Ctrl Pts',(-0.709400254238555,-6.7297132390085,
38.1637491981587));
#18195=CARTESIAN_POINT('Ctrl Pts',(-0.536574152570794,-6.74793138235397,
38.1719740464807));
#18196=CARTESIAN_POINT('Ctrl Pts',(-0.362803248484585,-6.75951328236136,
38.1801988948027));
#18197=CARTESIAN_POINT('Ctrl Pts',(-0.188638322026488,-6.76437022814859,
38.1884237431248));
#18198=CARTESIAN_POINT('Ctrl Pts',(-0.0146695438915345,-6.76922170393799,
38.196639328444));
#18199=CARTESIAN_POINT('Ctrl Pts',(0.159692017619453,-6.76736329694443,
38.2048549137632));
#18200=CARTESIAN_POINT('Ctrl Pts',(0.333888685743401,-6.75875782563132,
38.2130704990824));
#18201=CARTESIAN_POINT('Ctrl Pts',(0.50792416937496,-6.75016031697638,38.2212784825056));
#18202=CARTESIAN_POINT('Ctrl Pts',(0.681794707400922,-6.73482819479659,
38.2294864659289));
#18203=CARTESIAN_POINT('Ctrl Pts',(0.854940742096523,-6.71277627569275,
38.2376944493521));
#18204=CARTESIAN_POINT('Ctrl Pts',(1.02796134171457,-6.69074033202946,38.2458964865286));
#18205=CARTESIAN_POINT('Ctrl Pts',(1.20025812897806,-6.66199433299192,38.2540985237052));
#18206=CARTESIAN_POINT('Ctrl Pts',(1.37127470334437,-6.62660506503653,38.2623005608817));
#18207=CARTESIAN_POINT('Ctrl Pts',(1.54220172695864,-6.59123432824148,38.2704983031611));
#18208=CARTESIAN_POINT('Ctrl Pts',(1.71184952265965,-6.54922732512061,38.2786960454405));
#18209=CARTESIAN_POINT('Ctrl Pts',(1.87966985817477,-6.50070228700479,38.2868937877199));
#18210=CARTESIAN_POINT('Ctrl Pts',(2.04745828543029,-6.45218647512193,38.2950899713342));
#18211=CARTESIAN_POINT('Ctrl Pts',(2.21341959856338,-6.39715519033401,38.3032861549486));
#18212=CARTESIAN_POINT('Ctrl Pts',(2.37701845635905,-6.33577716291604,38.3114823385629));
#18213=CARTESIAN_POINT('Ctrl Pts',(2.5406052709962,-6.27440365377726,38.3196779188238));
#18214=CARTESIAN_POINT('Ctrl Pts',(2.70182964036839,-6.20668445767194,38.3278734990847));
#18215=CARTESIAN_POINT('Ctrl Pts',(2.86017407227692,-6.13283729413025,38.3360690793456));
#18216=CARTESIAN_POINT('Ctrl Pts',(3.01853565672223,-6.05898213115232,38.3442655473863));
#18217=CARTESIAN_POINT('Ctrl Pts',(3.17401635690134,-5.97899782992739,38.352462015427));
#18218=CARTESIAN_POINT('Ctrl Pts',(3.3261212073716,-5.89314913385644,38.3606584834677));
#18219=CARTESIAN_POINT('Ctrl Pts',(3.47827020827584,-5.80727551907201,38.3688573306411));
#18220=CARTESIAN_POINT('Ctrl Pts',(3.62704109525103,-5.71553429516912,38.3770561778145));
#18221=CARTESIAN_POINT('Ctrl Pts',(3.77196588758327,-5.61823480667266,38.3852550249879));
#18222=CARTESIAN_POINT('Ctrl Pts',(3.91704214041628,-5.52083363074911,38.3934624407538));
#18223=CARTESIAN_POINT('Ctrl Pts',(4.05826396977074,-5.4178627850371,38.4016698565198));
#18224=CARTESIAN_POINT('Ctrl Pts',(4.19519383168902,-5.30967397441297,38.4098772722858));
#18225=CARTESIAN_POINT('Ctrl Pts',(4.3321970831972,-5.20142717839156,38.4180890869379));
#18226=CARTESIAN_POINT('Ctrl Pts',(4.46490350900989,-5.08795707524879,38.42630090159));
#18227=CARTESIAN_POINT('Ctrl Pts',(4.59291085173824,-4.96965380162291,38.4345127162422));
#18228=CARTESIAN_POINT('Ctrl Pts',(4.72110670473902,-4.85117630844163,38.4427366240398));
#18229=CARTESIAN_POINT('Ctrl Pts',(4.84458939110564,-4.72785167406962,38.4509605318374));
#18230=CARTESIAN_POINT('Ctrl Pts',(4.96299464867785,-4.60010577239209,38.459184439635));
#18231=CARTESIAN_POINT('Ctrl Pts',(5.07239891993161,-4.48207091849077,38.4667831785585));
#18232=CARTESIAN_POINT('Ctrl Pts',(5.17746867850984,-4.36026198476384,38.4743819174819));
#18233=CARTESIAN_POINT('Ctrl Pts',(5.277949092835,-4.23503747013438,38.4819806564054));
#18234=CARTESIAN_POINT('Ctrl Pts',(5.3857319860596,-4.10071218316122,38.4901316385797));
#18235=CARTESIAN_POINT('Ctrl Pts',(5.4885529214214,-3.96205854079507,38.498282620754));
#18236=CARTESIAN_POINT('Ctrl Pts',(5.58604061641682,-3.8194815396519,38.5064336029282));
#18237=CARTESIAN_POINT('Ctrl Pts',(5.6834150704192,-3.6770701549098,38.5145751169813));
#18238=CARTESIAN_POINT('Ctrl Pts',(5.77546841148473,-3.53074478191807,38.5227166310343));
#18239=CARTESIAN_POINT('Ctrl Pts',(5.86186854422283,-3.3809445677578,38.5308581450874));
#18240=CARTESIAN_POINT('Ctrl Pts',(5.94818649695584,-3.23128683697077,38.5389919152904));
#18241=CARTESIAN_POINT('Ctrl Pts',(6.02886176488743,-3.07816115961845,38.5471256854935));
#18242=CARTESIAN_POINT('Ctrl Pts',(6.10360465212269,-2.92203683251705,38.5552594556965));
#18243=CARTESIAN_POINT('Ctrl Pts',(6.17829216717965,-2.76602816784719,38.5633872001145));
#18244=CARTESIAN_POINT('Ctrl Pts',(6.24705589525814,-2.60702560525452,38.5715149445325));
#18245=CARTESIAN_POINT('Ctrl Pts',(6.30965133453841,-2.44552428664238,38.5796426889505));
#18246=CARTESIAN_POINT('Ctrl Pts',(6.37221356111953,-2.28410865949224,38.5877661208446));
#18247=CARTESIAN_POINT('Ctrl Pts',(6.42861388498426,-2.12019725695791,38.5958895527386));
#18248=CARTESIAN_POINT('Ctrl Pts',(6.478655346468,-1.95430650146839,38.6040129846326));
#18249=CARTESIAN_POINT('Ctrl Pts',(6.52901425130072,-1.78736340027538,38.6121879483835));
#18250=CARTESIAN_POINT('Ctrl Pts',(6.57293318221682,-1.61841608794561,38.6203629121343));
#18251=CARTESIAN_POINT('Ctrl Pts',(6.61026179986248,-1.44800826561137,38.6285378758851));
#18252=CARTESIAN_POINT('Ctrl Pts',(6.64734669787008,-1.27871304094087,38.6366594650582));
#18253=CARTESIAN_POINT('Ctrl Pts',(6.67792702986911,-1.10797668812534,38.6447810542312));
#18254=CARTESIAN_POINT('Ctrl Pts',(6.70190635199328,-0.936344086921117,
38.6529026434042));
#18255=CARTESIAN_POINT('Ctrl Pts',(6.72588883987977,-0.764688826693477,
38.6610253047936));
#18256=CARTESIAN_POINT('Ctrl Pts',(6.74326853143352,-0.592137444899972,
38.6691479661829));
#18257=CARTESIAN_POINT('Ctrl Pts',(6.75400071760543,-0.419241346464561,
38.6772706275723));
#18258=CARTESIAN_POINT('Ctrl Pts',(6.76473636437172,-0.246289497666847,
38.6853959081145));
#18259=CARTESIAN_POINT('Ctrl Pts',(6.76882021474938,-0.0729930759797391,
38.6935211886568));
#18260=CARTESIAN_POINT('Ctrl Pts',(6.76625967295635,0.100095145360026,38.701646469199));
#18261=CARTESIAN_POINT('Ctrl Pts',(6.76367123459179,0.275069126955801,38.7098602729868));
#18262=CARTESIAN_POINT('Ctrl Pts',(6.75429278297422,0.449829960960584,38.7180740767746));
#18263=CARTESIAN_POINT('Ctrl Pts',(6.73818582979381,0.623811448408874,38.7262878805624));
#18264=CARTESIAN_POINT('Ctrl Pts',(6.7222248955591,0.796215691974586,38.7344272214175));
#18265=CARTESIAN_POINT('Ctrl Pts',(6.69965706508996,0.967854307981028,38.7425665622727));
#18266=CARTESIAN_POINT('Ctrl Pts',(6.6705937051536,1.13818654919355,38.7507059031279));
#18267=CARTESIAN_POINT('Ctrl Pts',(6.64113151506911,1.3108562225937,38.758956938382));
#18268=CARTESIAN_POINT('Ctrl Pts',(6.60499431030248,1.48218302291829,38.767207973636));
#18269=CARTESIAN_POINT('Ctrl Pts',(6.56235025601427,1.65161984651114,38.7754590088901));
#18270=CARTESIAN_POINT('Ctrl Pts',(6.51970620172607,1.82105667010392,38.7837100441442));
#18271=CARTESIAN_POINT('Ctrl Pts',(6.47055547032833,1.98860316748763,38.7919610793983));
#18272=CARTESIAN_POINT('Ctrl Pts',(6.41511645767085,2.15373392844164,38.8002121146524));
#18273=CARTESIAN_POINT('Ctrl Pts',(6.35979709247321,2.31850830721741,38.8084453426736));
#18274=CARTESIAN_POINT('Ctrl Pts',(6.29804399928013,2.48139190946777,38.8166785706948));
#18275=CARTESIAN_POINT('Ctrl Pts',(6.23000316624065,2.64184586011968,38.824911798716));
#18276=CARTESIAN_POINT('Ctrl Pts',(6.16204578460794,2.80210301559281,38.8331349287647));
#18277=CARTESIAN_POINT('Ctrl Pts',(6.08781615935948,2.95993612690317,38.8413580588134));
#18278=CARTESIAN_POINT('Ctrl Pts',(6.00751009732845,3.114821251773,38.8495811888621));
#18279=CARTESIAN_POINT('Ctrl Pts',(5.92730567465883,3.26951034629613,38.8577939113069));
#18280=CARTESIAN_POINT('Ctrl Pts',(5.84104030739634,3.42125857489348,38.8660066337517));
#18281=CARTESIAN_POINT('Ctrl Pts',(5.74895779903885,3.56956204944954,38.8742193561965));
#18282=CARTESIAN_POINT('Ctrl Pts',(5.65694254141812,3.7177572133383,38.8824260806331));
#18283=CARTESIAN_POINT('Ctrl Pts',(5.55911878981143,3.86251232953619,38.8906328050697));
#18284=CARTESIAN_POINT('Ctrl Pts',(5.45577646498682,4.0033476196923,38.8988395295064));
#18285=CARTESIAN_POINT('Ctrl Pts',(5.3524908650151,4.14410560501586,38.9070417492521));
#18286=CARTESIAN_POINT('Ctrl Pts',(5.24369293567096,4.28094776110854,38.9152439689977));
#18287=CARTESIAN_POINT('Ctrl Pts',(5.12971618532012,4.41342280526859,38.9234461887434));
#18288=CARTESIAN_POINT('Ctrl Pts',(5.01578131994848,4.54584916656609,38.9316453942796));
#18289=CARTESIAN_POINT('Ctrl Pts',(4.89667165805555,4.67391134162312,38.9398445998157));
#18290=CARTESIAN_POINT('Ctrl Pts',(4.77276134030782,4.79719065583839,38.9480438053519));
#18291=CARTESIAN_POINT('Ctrl Pts',(4.64884851108807,4.9204724687362,38.9562431770734));
#18292=CARTESIAN_POINT('Ctrl Pts',(4.52013507833853,5.03897096712496,38.9644425487949));
#18293=CARTESIAN_POINT('Ctrl Pts',(4.38703272241468,5.15230364909357,38.9726419205164));
#18294=CARTESIAN_POINT('Ctrl Pts',(4.2539342249196,5.26563304572527,38.9808410545509));
#18295=CARTESIAN_POINT('Ctrl Pts',(4.11644733341651,5.37379669510969,38.9890401885855));
#18296=CARTESIAN_POINT('Ctrl Pts',(3.97501729072259,5.47645200275292,38.99723932262));
#18297=CARTESIAN_POINT('Ctrl Pts',(3.83350849451294,5.57916447269513,39.0054430222378));
#18298=CARTESIAN_POINT('Ctrl Pts',(3.68805245071846,5.67636226201041,39.0136467218556));
#18299=CARTESIAN_POINT('Ctrl Pts',(3.53912450002771,5.76774538041543,39.0218504214734));
#18300=CARTESIAN_POINT('Ctrl Pts',(3.39555197202584,5.85584237809284,39.0297591175081));
#18301=CARTESIAN_POINT('Ctrl Pts',(3.24875316198388,5.93853548124723,39.0376678135429));
#18302=CARTESIAN_POINT('Ctrl Pts',(3.09917575053254,6.01559628526642,39.0455765095776));
#18303=CARTESIAN_POINT('Ctrl Pts',(3.09917575053255,6.01559628526641,37.0457515827422));
#18304=CARTESIAN_POINT('Ctrl Pts',(2.93382384459258,6.10078395293763,37.0545010306546));
#18305=CARTESIAN_POINT('Ctrl Pts',(2.76495772122973,6.17915010267054,37.0632504785671));
#18306=CARTESIAN_POINT('Ctrl Pts',(2.59315093316697,6.25042856433183,37.0719999264795));
#18307=CARTESIAN_POINT('Ctrl Pts',(2.42134553245598,6.32170645041459,37.0807493037395));
#18308=CARTESIAN_POINT('Ctrl Pts',(2.24659977927567,6.38589665313466,37.0894986809995));
#18309=CARTESIAN_POINT('Ctrl Pts',(2.0695071868989,6.44278115439085,37.0982480582595));
#18310=CARTESIAN_POINT('Ctrl Pts',(1.89241596572836,6.49966521519731,37.1069973677741));
#18311=CARTESIAN_POINT('Ctrl Pts',(1.71297821457177,6.54924360009551,37.1157466772888));
#18312=CARTESIAN_POINT('Ctrl Pts',(1.53180337335828,6.5913479217356,37.1244959868034));
#18313=CARTESIAN_POINT('Ctrl Pts',(1.35062987477768,6.63345193135308,37.1332452314796));
#18314=CARTESIAN_POINT('Ctrl Pts',(1.16771959102939,6.6680819236824,37.1419944761557));
#18315=CARTESIAN_POINT('Ctrl Pts',(0.983693746906732,6.6951202836317,37.1507437208318));
#18316=CARTESIAN_POINT('Ctrl Pts',(0.799669205419833,6.72215845218867,37.159492903576));
#18317=CARTESIAN_POINT('Ctrl Pts',(0.614529402873514,6.74160505424578,37.1682420863202));
#18318=CARTESIAN_POINT('Ctrl Pts',(0.428903127363362,6.75339404354121,37.1769912690643));
#18319=CARTESIAN_POINT('Ctrl Pts',(0.243278104164028,6.7651829533033,37.1857403927829));
#18320=CARTESIAN_POINT('Ctrl Pts',(0.0571669005393018,6.76931433552276,
37.1944895165015));
#18321=CARTESIAN_POINT('Ctrl Pts',(-0.128798404777293,6.76577415902473,
37.2032386402202));
#18322=CARTESIAN_POINT('Ctrl Pts',(-0.314762517258765,6.76223400523443,
37.2119877078194));
#18323=CARTESIAN_POINT('Ctrl Pts',(-0.500580446819064,6.75102239665092,
37.2207367754186));
#18324=CARTESIAN_POINT('Ctrl Pts',(-0.685621118842053,6.73217741012503,
37.2294858430178));
#18325=CARTESIAN_POINT('Ctrl Pts',(-0.870660665414095,6.71333253821777,
37.2382348574035));
#18326=CARTESIAN_POINT('Ctrl Pts',(-1.05492267885464,6.68685441030616,37.2469838717893));
#18327=CARTESIAN_POINT('Ctrl Pts',(-1.23778137635245,6.65283295028179,37.2557328861751));
#18328=CARTESIAN_POINT('Ctrl Pts',(-1.42999922978842,6.61707018861866,37.2649296965425));
#18329=CARTESIAN_POINT('Ctrl Pts',(-1.62066601233693,6.57297172934414,37.2741265069099));
#18330=CARTESIAN_POINT('Ctrl Pts',(-1.80906628500386,6.52070304311294,37.2833233172773));
#18331=CARTESIAN_POINT('Ctrl Pts',(-1.98831342545523,6.47097374915032,37.2920733150151));
#18332=CARTESIAN_POINT('Ctrl Pts',(-2.16550875896693,6.41384933989531,37.3008233127528));
#18333=CARTESIAN_POINT('Ctrl Pts',(-2.34005036713999,6.3495238624048,37.3095733104906));
#18334=CARTESIAN_POINT('Ctrl Pts',(-2.51458843547074,6.28519968948602,37.3183231307715));
#18335=CARTESIAN_POINT('Ctrl Pts',(-2.68647261718038,6.21367483971106,37.3270729510523));
#18336=CARTESIAN_POINT('Ctrl Pts',(-2.85511905908712,6.13519226743853,37.3358227713332));
#18337=CARTESIAN_POINT('Ctrl Pts',(-3.02376230488866,6.05671118252946,37.3445724257917));
#18338=CARTESIAN_POINT('Ctrl Pts',(-3.18916767379887,5.97127275992642,37.3533220802503));
#18339=CARTESIAN_POINT('Ctrl Pts',(-3.35077334102771,5.87916720438006,37.3620717347088));
#18340=CARTESIAN_POINT('Ctrl Pts',(-3.5123761603735,5.78706327195654,37.3708212349772));
#18341=CARTESIAN_POINT('Ctrl Pts',(-3.6701791630228,5.68829258362311,37.3795707352457));
#18342=CARTESIAN_POINT('Ctrl Pts',(-3.82364636566442,5.58319061741056,37.3883202355141));
#18343=CARTESIAN_POINT('Ctrl Pts',(-3.97711106778777,5.47809036367717,37.3970695932226));
#18344=CARTESIAN_POINT('Ctrl Pts',(-4.12623987481906,5.36665920043241,37.405818950931));
#18345=CARTESIAN_POINT('Ctrl Pts',(-4.27052628213908,5.24927559512352,37.4145683086394));
#18346=CARTESIAN_POINT('Ctrl Pts',(-4.41481053024952,5.13189374643059,37.4233175354159));
#18347=CARTESIAN_POINT('Ctrl Pts',(-4.55425230136499,5.00855981477381,37.4320667621925));
#18348=CARTESIAN_POINT('Ctrl Pts',(-4.68837800630513,4.8796926819211,37.440815988969));
#18349=CARTESIAN_POINT('Ctrl Pts',(-4.8225018822886,4.75082730631844,37.4495650964398));
#18350=CARTESIAN_POINT('Ctrl Pts',(-4.95130963052933,4.61642907903561,37.4583142039107));
#18351=CARTESIAN_POINT('Ctrl Pts',(-5.07436379033335,4.47695444731726,37.4670633113815));
#18352=CARTESIAN_POINT('Ctrl Pts',(-5.19741643562761,4.33748153220638,37.4758123111712));
#18353=CARTESIAN_POINT('Ctrl Pts',(-5.31471544462718,4.19293255254658,37.484561310961));
#18354=CARTESIAN_POINT('Ctrl Pts',(-5.42586245275563,4.0437984177969,37.4933103107507));
#18355=CARTESIAN_POINT('Ctrl Pts',(-5.53702160019089,3.89464799484434,37.5020602660929));
#18356=CARTESIAN_POINT('Ctrl Pts',(-5.64202723081188,3.74091164443945,37.510810221435));
#18357=CARTESIAN_POINT('Ctrl Pts',(-5.74052265232905,3.58311159163332,37.5195601767772));
#18358=CARTESIAN_POINT('Ctrl Pts',(-5.83901427066862,3.42531763191879,37.5283097942596));
#18359=CARTESIAN_POINT('Ctrl Pts',(-5.93099603115689,3.26346052695704,37.5370594117421));
#18360=CARTESIAN_POINT('Ctrl Pts',(-6.01615550622709,3.09809004467164,37.5458090292245));
#18361=CARTESIAN_POINT('Ctrl Pts',(-6.10131214578765,2.932725068639,37.5545583553756));
#18362=CARTESIAN_POINT('Ctrl Pts',(-6.17964682328723,2.76384720416951,37.5633076815267));
#18363=CARTESIAN_POINT('Ctrl Pts',(-6.25089348288547,2.59203002791634,37.5720570076778));
#18364=CARTESIAN_POINT('Ctrl Pts',(-6.32213814889322,2.42021765937052,37.5808060890094));
#18365=CARTESIAN_POINT('Ctrl Pts',(-6.38629508412584,2.24546640831922,37.589555170341));
#18366=CARTESIAN_POINT('Ctrl Pts',(-6.44314639819817,2.06836976660026,37.5983042516726));
#18367=CARTESIAN_POINT('Ctrl Pts',(-6.50000285283708,1.8912571115825,37.607054124107));
#18368=CARTESIAN_POINT('Ctrl Pts',(-6.54955227673259,1.71179891440219,37.6158039965414));
#18369=CARTESIAN_POINT('Ctrl Pts',(-6.59162635926396,1.53060476278385,37.6245538689758));
#18370=CARTESIAN_POINT('Ctrl Pts',(-6.63369752055207,1.34942319164646,37.6333031338983));
#18371=CARTESIAN_POINT('Ctrl Pts',(-6.66829431424263,1.16650618642651,37.6420523988208));
#18372=CARTESIAN_POINT('Ctrl Pts',(-6.69529923745425,0.982474997617998,
37.6508016637433));
#18373=CARTESIAN_POINT('Ctrl Pts',(-6.72230554731451,0.798434359177128,
37.659551377923));
#18374=CARTESIAN_POINT('Ctrl Pts',(-6.74171916496709,0.61327970623967,37.6683010921027));
#18375=CARTESIAN_POINT('Ctrl Pts',(-6.75347414817279,0.427639953654658,
37.6770508062824));
#18376=CARTESIAN_POINT('Ctrl Pts',(-6.76248837758747,0.285283364197911,
37.6837604654583));
#18377=CARTESIAN_POINT('Ctrl Pts',(-6.76699999999998,0.142641701104516,
37.6904701246342));
#18378=CARTESIAN_POINT('Ctrl Pts',(-6.767,1.02740346869295E-12,37.6971797838101));
#18379=CARTESIAN_POINT('',(-6.76798064037177,0.0012455647848279,37.3045171512176));
#18380=CARTESIAN_POINT('Ctrl Pts',(3.09917575053261,6.01559628526638,36.6515495189894));
#18381=CARTESIAN_POINT('Ctrl Pts',(2.94396117623734,6.09556129986739,36.6597479494324));
#18382=CARTESIAN_POINT('Ctrl Pts',(2.78557597437919,6.1695531728888,36.6679463798753));
#18383=CARTESIAN_POINT('Ctrl Pts',(2.62452199755003,6.23732100219125,36.6761448103182));
#18384=CARTESIAN_POINT('Ctrl Pts',(2.46348890435358,6.30508004413876,36.6843421776827));
#18385=CARTESIAN_POINT('Ctrl Pts',(2.29978805308302,6.36661650452126,36.6925395450472));
#18386=CARTESIAN_POINT('Ctrl Pts',(2.1339428144838,6.42172695343807,36.7007369124117));
#18387=CARTESIAN_POINT('Ctrl Pts',(1.9681026353072,6.47683572110642,36.7089340297));
#18388=CARTESIAN_POINT('Ctrl Pts',(1.80011853925938,6.5255187538798,36.7171311469883));
#18389=CARTESIAN_POINT('Ctrl Pts',(1.63053057587416,6.56762202331555,36.7253282642766));
#18390=CARTESIAN_POINT('Ctrl Pts',(1.46091696375125,6.60973166051286,36.7335266213092));
#18391=CARTESIAN_POINT('Ctrl Pts',(1.28969934923995,6.64525946555615,36.7417249783418));
#18392=CARTESIAN_POINT('Ctrl Pts',(1.11742958154676,6.67410219657178,36.7499233353744));
#18393=CARTESIAN_POINT('Ctrl Pts',(0.945102449594142,6.70295453195344,36.758124422385));
#18394=CARTESIAN_POINT('Ctrl Pts',(0.771722820188464,6.72511730005566,36.7663255093956));
#18395=CARTESIAN_POINT('Ctrl Pts',(0.59784934942649,6.74053893656808,36.7745265964062));
#18396=CARTESIAN_POINT('Ctrl Pts',(0.423791854826353,6.75597689499971,36.7827363632661));
#18397=CARTESIAN_POINT('Ctrl Pts',(0.249239832417566,6.76465943836995,36.7909461301259));
#18398=CARTESIAN_POINT('Ctrl Pts',(0.0747546027331646,6.7665870828188,36.7991558969858));
#18399=CARTESIAN_POINT('Ctrl Pts',(-0.0998307939834776,6.76851583387377,
36.8073703768404));
#18400=CARTESIAN_POINT('Ctrl Pts',(-0.274348963605343,6.76368196601679,
36.8155848566951));
#18401=CARTESIAN_POINT('Ctrl Pts',(-0.448242117126577,6.75213803209279,
36.8237993365497));
#18402=CARTESIAN_POINT('Ctrl Pts',(-0.622378968351616,6.74057792024498,
36.8320253283578));
#18403=CARTESIAN_POINT('Ctrl Pts',(-0.795888697323502,6.72228899251469,
36.8402513201658));
#18404=CARTESIAN_POINT('Ctrl Pts',(-0.968221020471342,6.69737538559079,
36.8484773119738));
#18405=CARTESIAN_POINT('Ctrl Pts',(-1.08474943022036,6.680529195956,36.8540395984125));
#18406=CARTESIAN_POINT('Ctrl Pts',(-1.20073970968487,6.66065510271486,36.8596018848513));
#18407=CARTESIAN_POINT('Ctrl Pts',(-1.31602549799756,6.63779827116042,36.86516417129));
#18408=CARTESIAN_POINT('Ctrl Pts',(-1.48499807432253,6.60429737073804,36.8733167275033));
#18409=CARTESIAN_POINT('Ctrl Pts',(-1.65295490583598,6.56428777962686,36.8814692837165));
#18410=CARTESIAN_POINT('Ctrl Pts',(-1.81935102344975,6.51784096564747,36.8896218399298));
#18411=CARTESIAN_POINT('Ctrl Pts',(-1.98555436714975,6.47144796142183,36.8977649512101));
#18412=CARTESIAN_POINT('Ctrl Pts',(-2.1502002476918,6.41863267682765,36.9059080624905));
#18413=CARTESIAN_POINT('Ctrl Pts',(-2.31275175379891,6.35951793183257,36.9140511737708));
#18414=CARTESIAN_POINT('Ctrl Pts',(-2.4751491144978,6.30045924455556,36.9221865630482));
#18415=CARTESIAN_POINT('Ctrl Pts',(-2.63545571358102,6.23511311381613,36.9303219523256));
#18416=CARTESIAN_POINT('Ctrl Pts',(-2.79314772817954,6.16365271316981,36.9384573416029));
#18417=CARTESIAN_POINT('Ctrl Pts',(-2.95072334045501,6.09224506190754,36.9465867256415));
#18418=CARTESIAN_POINT('Ctrl Pts',(-3.10568787962654,6.01473227781286,36.95471610968));
#18419=CARTESIAN_POINT('Ctrl Pts',(-3.25753551730379,5.93133638849664,36.9628454937185));
#18420=CARTESIAN_POINT('Ctrl Pts',(-3.40930296202517,5.84798454176794,36.9709705845106));
#18421=CARTESIAN_POINT('Ctrl Pts',(-3.55795646378905,5.75875595303,36.9790956753026));
#18422=CARTESIAN_POINT('Ctrl Pts',(-3.70301292002846,5.66391951868159,36.9872207660947));
#18423=CARTESIAN_POINT('Ctrl Pts',(-3.84862308820951,5.56872107310279,36.9953768721198));
#18424=CARTESIAN_POINT('Ctrl Pts',(-3.99060835947779,5.46787204544738,37.003532978145));
#18425=CARTESIAN_POINT('Ctrl Pts',(-4.128507246566,5.36168974438582,37.0116890841701));
#18426=CARTESIAN_POINT('Ctrl Pts',(-4.26585111557264,5.255934807883,37.0198123633435));
#18427=CARTESIAN_POINT('Ctrl Pts',(-4.39914115454755,5.14488969097722,37.0279356425169));
#18428=CARTESIAN_POINT('Ctrl Pts',(-4.52795285153677,5.02890962080847,37.0360589216903));
#18429=CARTESIAN_POINT('Ctrl Pts',(-4.65678170089149,4.91291410691373,37.0441832825469));
#18430=CARTESIAN_POINT('Ctrl Pts',(-4.78113074859226,4.79198257568056,37.0523076434036));
#18431=CARTESIAN_POINT('Ctrl Pts',(-4.90061089322392,4.66650853135565,37.0604320042602));
#18432=CARTESIAN_POINT('Ctrl Pts',(-5.02012967935872,4.54099390701895,37.0685589926456));
#18433=CARTESIAN_POINT('Ctrl Pts',(-5.13477617461776,4.41093410891703,37.076685981031));
#18434=CARTESIAN_POINT('Ctrl Pts',(-5.24420029377589,4.27675721531639,37.0848129694164));
#18435=CARTESIAN_POINT('Ctrl Pts',(-5.3543318274073,4.14171288337363,37.0929924978565));
#18436=CARTESIAN_POINT('Ctrl Pts',(-5.45917298917913,4.00249832951863,37.1011720262966));
#18437=CARTESIAN_POINT('Ctrl Pts',(-5.55841052770631,3.85958047013969,37.1093515547367));
#18438=CARTESIAN_POINT('Ctrl Pts',(-5.657180724671,3.71733565703638,37.1174925631404));
#18439=CARTESIAN_POINT('Ctrl Pts',(-5.75039982084009,3.57142268597552,37.125633571544));
#18440=CARTESIAN_POINT('Ctrl Pts',(-5.83780485202429,3.42232720669454,37.1337745799477));
#18441=CARTESIAN_POINT('Ctrl Pts',(-5.92583023233854,3.27217353603015,37.141973368406));
#18442=CARTESIAN_POINT('Ctrl Pts',(-6.00795853652428,3.11879234879113,37.1501721568644));
#18443=CARTESIAN_POINT('Ctrl Pts',(-6.08397035698332,2.96270040593853,37.1583709453227));
#18444=CARTESIAN_POINT('Ctrl Pts',(-6.15998217744236,2.80660846308593,37.166569733781));
#18445=CARTESIAN_POINT('Ctrl Pts',(-6.22987742386527,2.64780613061743,37.1747685222393));
#18446=CARTESIAN_POINT('Ctrl Pts',(-6.29348772503758,2.48682553766871,37.1829673106977));
#18447=CARTESIAN_POINT('Ctrl Pts',(-6.37097762342811,2.2907194108222,37.192955052822));
#18448=CARTESIAN_POINT('Ctrl Pts',(-6.43934951496975,2.09085568620677,37.2029427949464));
#18449=CARTESIAN_POINT('Ctrl Pts',(-6.4982789485285,1.88803064252446,37.2129305370707));
#18450=CARTESIAN_POINT('Ctrl Pts',(-6.55421706784962,1.69550119145653,37.2224112918814));
#18451=CARTESIAN_POINT('Ctrl Pts',(-6.60164731541451,1.50030373926963,37.231892046692));
#18452=CARTESIAN_POINT('Ctrl Pts',(-6.6403394713027,1.30314262682923,37.2413728015027));
#18453=CARTESIAN_POINT('Ctrl Pts',(-6.67886840719424,1.10681322395306,37.2508135624507));
#18454=CARTESIAN_POINT('Ctrl Pts',(-6.70873272479008,0.908536806826755,
37.2602543233986));
#18455=CARTESIAN_POINT('Ctrl Pts',(-6.72975228847598,0.709029714294338,
37.2696950843466));
#18456=CARTESIAN_POINT('Ctrl Pts',(-6.75062773480303,0.51089051101398,37.2790711161901));
#18457=CARTESIAN_POINT('Ctrl Pts',(-6.76277921401833,0.311537577722562,
37.2884471480337));
#18458=CARTESIAN_POINT('Ctrl Pts',(-6.7660781861477,0.111691445224431,37.2978231798772));
#18459=CARTESIAN_POINT('Ctrl Pts',(-6.76666425794581,0.0761882103907818,
37.2994888586481));
#18460=CARTESIAN_POINT('Ctrl Pts',(-6.7669710646382,0.040669455310506,37.301154537419));
#18461=CARTESIAN_POINT('Ctrl Pts',(-6.76699804845725,0.00513927774541282,
37.3028202161899));
#18462=CARTESIAN_POINT('Ctrl Pts',(-6.767,8.48442082414717E-13,37.3028202161899));
#18463=CARTESIAN_POINT('Ctrl Pts',(-6.76700000000002,-0.18600724941485,
37.3115697279959));
#18464=CARTESIAN_POINT('Ctrl Pts',(-6.75932637295443,-0.372014355526724,
37.3203192398018));
#18465=CARTESIAN_POINT('Ctrl Pts',(-6.74400518266934,-0.557389537154261,
37.3290687516078));
#18466=CARTESIAN_POINT('Ctrl Pts',(-6.72868405709653,-0.742763935810769,
37.3378182264583));
#18467=CARTESIAN_POINT('Ctrl Pts',(-6.70571545652998,-0.927506129694568,
37.3465677013089));
#18468=CARTESIAN_POINT('Ctrl Pts',(-6.67517739415655,-1.11098863924945,
37.3553171761594));
#18469=CARTESIAN_POINT('Ctrl Pts',(-6.64463945823072,-1.29447038906648,
37.3640666147814));
#18470=CARTESIAN_POINT('Ctrl Pts',(-6.60653217027122,-1.47669218228375,
37.3728160534034));
#18471=CARTESIAN_POINT('Ctrl Pts',(-6.56098496116669,-1.65703510504292,
37.3815654920254));
#18472=CARTESIAN_POINT('Ctrl Pts',(-6.51543793687462,-1.83737729604219,
37.3903148951456));
#18473=CARTESIAN_POINT('Ctrl Pts',(-6.4624511220257,-2.01584035397278,37.3990642982659));
#18474=CARTESIAN_POINT('Ctrl Pts',(-6.40220448416156,-2.19181813638394,
37.4078137013861));
#18475=CARTESIAN_POINT('Ctrl Pts',(-6.34195808575086,-2.36779521936214,
37.4165630697314));
#18476=CARTESIAN_POINT('Ctrl Pts',(-6.27445201489118,-2.54128677545116,
37.4253124380767));
#18477=CARTESIAN_POINT('Ctrl Pts',(-6.19991555136049,-2.71170355238148,
37.434061806422));
#18478=CARTESIAN_POINT('Ctrl Pts',(-6.125379377889,-2.88211966613366,37.442811140719));
#18479=CARTESIAN_POINT('Ctrl Pts',(-6.04381298133475,-3.04946076210725,
37.4515604750161));
#18480=CARTESIAN_POINT('Ctrl Pts',(-5.95549339426162,-3.21315848207122,
37.4603098093131));
#18481=CARTESIAN_POINT('Ctrl Pts',(-5.86717414355011,-3.37685557859897,
37.4690591102887));
#18482=CARTESIAN_POINT('Ctrl Pts',(-5.77210188986082,-3.53690907467566,
37.4778084112642));
#18483=CARTESIAN_POINT('Ctrl Pts',(-5.67059953466907,-3.69277536785153,
37.4865577122398));
#18484=CARTESIAN_POINT('Ctrl Pts',(-5.56909755761611,-3.84864108036016,
37.4953069806205));
#18485=CARTESIAN_POINT('Ctrl Pts',(-5.46116568337923,-4.00031938104478,
37.5040562490013));
#18486=CARTESIAN_POINT('Ctrl Pts',(-5.34717048685978,-4.14729511663394,
37.512805517382));
#18487=CARTESIAN_POINT('Ctrl Pts',(-5.23317570555368,-4.29427031688223,
37.5215547538947));
#18488=CARTESIAN_POINT('Ctrl Pts',(-5.11311782178643,-4.43654275987318,
37.5303039904073));
#18489=CARTESIAN_POINT('Ctrl Pts',(-4.98740459171838,-4.57362924147842,
37.5390532269199));
#18490=CARTESIAN_POINT('Ctrl Pts',(-4.8616918091064,-4.71071523514633,37.547802432291));
#18491=CARTESIAN_POINT('Ctrl Pts',(-4.73032391415227,-4.84261509316724,
37.5565516376622));
#18492=CARTESIAN_POINT('Ctrl Pts',(-4.59374707237074,-4.96888084331726,
37.5653008430333));
#18493=CARTESIAN_POINT('Ctrl Pts',(-4.4571707053716,-5.09514615452937,37.5740500179895));
#18494=CARTESIAN_POINT('Ctrl Pts',(-4.31538563819243,-5.21577720253853,
37.5827991929458));
#18495=CARTESIAN_POINT('Ctrl Pts',(-4.16887341290358,-5.33036429028877,
37.591548367902));
#18496=CARTESIAN_POINT('Ctrl Pts',(-4.02236168477022,-5.44495098921411,
37.6002975131699));
#18497=CARTESIAN_POINT('Ctrl Pts',(-3.87112305634095,-5.55349359239,37.6090466584379));
#18498=CARTESIAN_POINT('Ctrl Pts',(-3.7156711731636,-5.65562346102718,37.6177958037058));
#18499=CARTESIAN_POINT('Ctrl Pts',(-3.56021980456936,-5.75775299158994,
37.626544920012));
#18500=CARTESIAN_POINT('Ctrl Pts',(-3.40055544862031,-5.8534696727556,37.6352940363181));
#18501=CARTESIAN_POINT('Ctrl Pts',(-3.23722036323056,-5.94244842803751,
37.6440431526243));
#18502=CARTESIAN_POINT('Ctrl Pts',(-3.07388580495718,-6.03142689616642,
37.6527922406952));
#18503=CARTESIAN_POINT('Ctrl Pts',(-2.90688079257399,-6.11366734484968,
37.6615413287661));
#18504=CARTESIAN_POINT('Ctrl Pts',(-2.73677251094328,-6.18889046787429,
37.6702904168371));
#18505=CARTESIAN_POINT('Ctrl Pts',(-2.56666476416375,-6.2641133543838,37.6790394773993));
#18506=CARTESIAN_POINT('Ctrl Pts',(-2.39345402971839,-6.33231884350386,
37.6877885379615));
#18507=CARTESIAN_POINT('Ctrl Pts',(-2.21772856473802,-6.39327529621125,
37.6965375985237));
#18508=CARTESIAN_POINT('Ctrl Pts',(-2.04200363768062,-6.45423156232146,
37.7052866323037));
#18509=CARTESIAN_POINT('Ctrl Pts',(-1.86376426619915,-6.50793874252106,
37.7140356660837));
#18510=CARTESIAN_POINT('Ctrl Pts',(-1.6836157819454,-6.55421443796161,37.7227846998637));
#18511=CARTESIAN_POINT('Ctrl Pts',(-1.50346783419716,-6.60048999558714,
37.7315337075879));
#18512=CARTESIAN_POINT('Ctrl Pts',(-1.3214110625709,-6.63933404145526,37.7402827153121));
#18513=CARTESIAN_POINT('Ctrl Pts',(-1.13806375958884,-6.67061465527057,
37.7490317230364));
#18514=CARTESIAN_POINT('Ctrl Pts',(-0.954716987417457,-6.70189517852505,
37.7577807054313));
#18515=CARTESIAN_POINT('Ctrl Pts',(-0.770079973808082,-6.72561226535849,
37.7665296878261));
#18516=CARTESIAN_POINT('Ctrl Pts',(-0.584779770550568,-6.74168536939798,
37.775278670221));
#18517=CARTESIAN_POINT('Ctrl Pts',(-0.391490647552041,-6.75845143942405,
37.7844048508971));
#18518=CARTESIAN_POINT('Ctrl Pts',(-0.197480213102489,-6.76689975924032,
37.7935310315731));
#18519=CARTESIAN_POINT('Ctrl Pts',(-0.00346532629597262,-6.76699911271708,
37.8026572122492));
#18520=CARTESIAN_POINT('Ctrl Pts',(0.184486595297806,-6.76709536139768,
37.8114981997791));
#18521=CARTESIAN_POINT('Ctrl Pts',(0.372442378186903,-6.75935659726761,
37.820339187309));
#18522=CARTESIAN_POINT('Ctrl Pts',(0.559750217723683,-6.74380965729003,
37.829180174839));
#18523=CARTESIAN_POINT('Ctrl Pts',(0.745129914459311,-6.72842275717236,
37.8379301534367));
#18524=CARTESIAN_POINT('Ctrl Pts',(0.929874656315701,-6.70538772273452,
37.8466801320345));
#18525=CARTESIAN_POINT('Ctrl Pts',(1.11335688289925,-6.67478280180718,37.8554301106323));
#18526=CARTESIAN_POINT('Ctrl Pts',(1.29683723118999,-6.64417819417995,37.8641799996572));
#18527=CARTESIAN_POINT('Ctrl Pts',(1.47905480730373,-6.60600390230044,37.8729298886821));
#18528=CARTESIAN_POINT('Ctrl Pts',(1.65939064804941,-6.56038959797101,37.8816797777071));
#18529=CARTESIAN_POINT('Ctrl Pts',(1.83972470264399,-6.51477574543218,37.890429580068));
#18530=CARTESIAN_POINT('Ctrl Pts',(2.01817678125983,-6.46172209820058,37.899179382429));
#18531=CARTESIAN_POINT('Ctrl Pts',(2.19414072347815,-6.40140886723968,37.9079291847899));
#18532=CARTESIAN_POINT('Ctrl Pts',(2.37010298132229,-6.34109621361325,37.9166789033954));
#18533=CARTESIAN_POINT('Ctrl Pts',(2.54357687927041,-6.27352420825919,37.9254286220009));
#18534=CARTESIAN_POINT('Ctrl Pts',(2.71397317790095,-6.19892237325442,37.9341783406064));
#18535=CARTESIAN_POINT('Ctrl Pts',(2.88436790207325,-6.12432122756905,37.9429279783647));
#18536=CARTESIAN_POINT('Ctrl Pts',(3.05168482126381,-6.04269049717354,37.9516776161229));
#18537=CARTESIAN_POINT('Ctrl Pts',(3.21535561997512,-5.95430745234863,37.9604272538812));
#18538=CARTESIAN_POINT('Ctrl Pts',(3.37902496075404,-5.86592519481446,37.9691768137002));
#18539=CARTESIAN_POINT('Ctrl Pts',(3.53904799384998,-5.77079087940157,37.9779263735192));
#18540=CARTESIAN_POINT('Ctrl Pts',(3.69488118815106,-5.66922763746945,37.9866759333382));
#18541=CARTESIAN_POINT('Ctrl Pts',(3.85071304610952,-5.5676652664897,37.9954254181257));
#18542=CARTESIAN_POINT('Ctrl Pts',(4.00235489706083,-5.45967423580629,38.0041749029131));
#18543=CARTESIAN_POINT('Ctrl Pts',(4.14929168607766,-5.34562133936241,38.0129243877005));
#18544=CARTESIAN_POINT('Ctrl Pts',(4.29622726385859,-5.23156938308446,38.0216738003638));
#18545=CARTESIAN_POINT('Ctrl Pts',(4.4384576309216,-5.11145583677121,38.0304232130271));
#18546=CARTESIAN_POINT('Ctrl Pts',(4.57549970661046,-4.98568866204134,38.0391726256904));
#18547=CARTESIAN_POINT('Ctrl Pts',(4.71254069815386,-4.85992248226073,38.0479219691368));
#18548=CARTESIAN_POINT('Ctrl Pts',(4.84439326931412,-4.72850295733903,38.0566713125831));
#18549=CARTESIAN_POINT('Ctrl Pts',(4.97060959434801,-4.5918764422157,38.0654206560294));
#18550=CARTESIAN_POINT('Ctrl Pts',(5.09682496280622,-4.45525096256542,38.0741699331657));
#18551=CARTESIAN_POINT('Ctrl Pts',(5.21740397615949,-4.31341878218193,38.082919210302));
#18552=CARTESIAN_POINT('Ctrl Pts',(5.33193710452046,-4.16686161438534,38.0916684874383));
#18553=CARTESIAN_POINT('Ctrl Pts',(5.44646940289493,-4.02030550864364,38.1004177011713));
#18554=CARTESIAN_POINT('Ctrl Pts',(5.55495572749773,-3.86902470979978,38.1091669149043));
#18555=CARTESIAN_POINT('Ctrl Pts',(5.65702762491562,-3.7135330146562,38.1179161286372));
#18556=CARTESIAN_POINT('Ctrl Pts',(5.75909881655262,-3.55804239466718,38.1266652818733));
#18557=CARTESIAN_POINT('Ctrl Pts',(5.85475551250892,-3.39834117619365,38.1354144351095));
#18558=CARTESIAN_POINT('Ctrl Pts',(5.94367283728205,-3.23497174691767,38.1441635883456));
#18559=CARTESIAN_POINT('Ctrl Pts',(6.03258957676428,-3.07160339300738,38.1529126839911));
#18560=CARTESIAN_POINT('Ctrl Pts',(6.11476689685406,-2.90456712829249,38.1616617796367));
#18561=CARTESIAN_POINT('Ctrl Pts',(6.18992570525385,-2.73443024475622,38.1704108752822));
#18562=CARTESIAN_POINT('Ctrl Pts',(6.26508404388818,-2.56429442462735,38.1791599162432));
#18563=CARTESIAN_POINT('Ctrl Pts',(6.33322384283431,-2.39105828655686,38.1879089572043));
#18564=CARTESIAN_POINT('Ctrl Pts',(6.39411368720143,-2.21531017131763,38.1966579981653));
#18565=CARTESIAN_POINT('Ctrl Pts',(6.45500317120991,-2.03956309619194,38.2054069873477));
#18566=CARTESIAN_POINT('Ctrl Pts',(6.50864269270166,-1.8613043443831,38.2141559765301));
#18567=CARTESIAN_POINT('Ctrl Pts',(6.55485008446417,-1.6811393071962,38.2229049657125));
#18568=CARTESIAN_POINT('Ctrl Pts',(6.60199664749477,-1.49731239211517,38.2318317792419));
#18569=CARTESIAN_POINT('Ctrl Pts',(6.6414056364097,-1.31150116499351,38.2407585927713));
#18570=CARTESIAN_POINT('Ctrl Pts',(6.67293772282226,-1.12436255155342,38.2496854063006));
#18571=CARTESIAN_POINT('Ctrl Pts',(6.70384494949916,-0.940932395048121,
38.2584353204561));
#18572=CARTESIAN_POINT('Ctrl Pts',(6.72718449348967,-0.756227260503447,
38.2671852346117));
#18573=CARTESIAN_POINT('Ctrl Pts',(6.7428770737396,-0.570874564538384,38.2759351487672));
#18574=CARTESIAN_POINT('Ctrl Pts',(6.75856934538689,-0.385525513629147,
38.2846848908512));
#18575=CARTESIAN_POINT('Ctrl Pts',(6.76661493004113,-0.199529212414885,
38.2934346329352));
#18576=CARTESIAN_POINT('Ctrl Pts',(6.76698649908907,-0.0135174385970706,
38.3021843750191));
#18577=CARTESIAN_POINT('Ctrl Pts',(6.76735806132381,0.172490924449114,38.310933956665));
#18578=CARTESIAN_POINT('Ctrl Pts',(6.76005588896272,0.358514472904719,38.3196835383109));
#18579=CARTESIAN_POINT('Ctrl Pts',(6.74510478454558,0.543921359665496,38.3284331199568));
#18580=CARTESIAN_POINT('Ctrl Pts',(6.73015393440652,0.729325093153743,38.3371825527959));
#18581=CARTESIAN_POINT('Ctrl Pts',(6.70755443556852,0.91411190025966,38.3459319856349));
#18582=CARTESIAN_POINT('Ctrl Pts',(6.67738304682264,1.09765415591869,38.354681418474));
#18583=CARTESIAN_POINT('Ctrl Pts',(6.64721213111796,1.28119353391607,38.3634307141353));
#18584=CARTESIAN_POINT('Ctrl Pts',(6.6094696095542,1.4634881167299,38.3721800097966));
#18585=CARTESIAN_POINT('Ctrl Pts',(6.56428366991098,1.64391876348561,38.380929305458));
#18586=CARTESIAN_POINT('Ctrl Pts',(6.51909837867623,1.82434682110053,38.3896784755688));
#18587=CARTESIAN_POINT('Ctrl Pts',(6.46646995271818,2.0029107182078,38.3984276456796));
#18588=CARTESIAN_POINT('Ctrl Pts',(6.40657713281436,2.17900400213036,38.4071768157904));
#18589=CARTESIAN_POINT('Ctrl Pts',(6.34668509278937,2.35509499309989,38.4159258719762));
#18590=CARTESIAN_POINT('Ctrl Pts',(6.27952894037393,2.52871516398452,38.424674928162));
#18591=CARTESIAN_POINT('Ctrl Pts',(6.20533675061305,2.69927486771747,38.4334239843477));
#18592=CARTESIAN_POINT('Ctrl Pts',(6.12832117907774,2.87632521636227,38.44250598563));
#18593=CARTESIAN_POINT('Ctrl Pts',(6.04372366625937,3.05007728920278,38.4515879869123));
#18594=CARTESIAN_POINT('Ctrl Pts',(5.95185378007728,3.21989527478453,38.4606699881945));
#18595=CARTESIAN_POINT('Ctrl Pts',(5.86334450817225,3.38350129287004,38.4694197685017));
#18596=CARTESIAN_POINT('Ctrl Pts',(5.76808562057104,3.54345567125209,38.4781695488088));
#18597=CARTESIAN_POINT('Ctrl Pts',(5.66640068804327,3.6992150846555,38.4869193291159));
#18598=CARTESIAN_POINT('Ctrl Pts',(5.56471941107758,3.85496889852522,38.4956687948694));
#18599=CARTESIAN_POINT('Ctrl Pts',(5.4566127081494,4.00652780919873,38.5044182606229));
#18600=CARTESIAN_POINT('Ctrl Pts',(5.34244776448933,4.15337704569462,38.5131677263764));
#18601=CARTESIAN_POINT('Ctrl Pts',(5.22828631819406,4.30022178356479,38.5219169240959));
#18602=CARTESIAN_POINT('Ctrl Pts',(5.10806717843873,4.44235690972905,38.5306661218156));
#18603=CARTESIAN_POINT('Ctrl Pts',(4.98219864544516,4.57929969070866,38.5394153195352));
#18604=CARTESIAN_POINT('Ctrl Pts',(4.8563332994381,4.71623900430222,38.5481642957254));
#18605=CARTESIAN_POINT('Ctrl Pts',(4.72481904033422,4.84798602483837,38.5569132719156));
#18606=CARTESIAN_POINT('Ctrl Pts',(4.58810250736961,4.97409332259345,38.5656622481059));
#18607=CARTESIAN_POINT('Ctrl Pts',(4.45137708685396,5.1002088182235,38.574411793042));
#18608=CARTESIAN_POINT('Ctrl Pts',(4.30944892635796,5.22068366308144,38.5831613379782));
#18609=CARTESIAN_POINT('Ctrl Pts',(4.16280009466397,5.33510865605056,38.5919108829144));
#18610=CARTESIAN_POINT('Ctrl Pts',(4.01615988348529,5.44952692273083,38.6006599135227));
#18611=CARTESIAN_POINT('Ctrl Pts',(3.86479978231976,5.55789587288803,38.609408944131));
#18612=CARTESIAN_POINT('Ctrl Pts',(3.70923383580818,5.65984746714041,38.6181579747392));
#18613=CARTESIAN_POINT('Ctrl Pts',(3.55366577799287,5.76180044505539,38.6269071240872));
#18614=CARTESIAN_POINT('Ctrl Pts',(3.39389200026583,5.85733573571208,38.6356562734353));
#18615=CARTESIAN_POINT('Ctrl Pts',(3.2304551362578,5.9461288762207,38.6444054227833));
#18616=CARTESIAN_POINT('Ctrl Pts',(3.18695122151406,5.96976399206779,38.6467342868962));
#18617=CARTESIAN_POINT('Ctrl Pts',(3.14318791262581,5.99292165435376,38.6490631510091));
#18618=CARTESIAN_POINT('Ctrl Pts',(3.09917575053265,6.01559628526636,38.651392015122));
#18619=CARTESIAN_POINT('Origin',(0.,0.,-3.69717978381041));
#18620=CARTESIAN_POINT('',(3.09917575053253,6.01559628526642,41.0457515827422));
#18621=CARTESIAN_POINT('',(3.09917575053255,6.01559628526641,40.6512265384361));
#18622=CARTESIAN_POINT('',(3.09917575053259,6.01559628526639,-3.69717978381041));
#18623=CARTESIAN_POINT('',(-6.767,1.16999332856575E-12,39.69717978381));
#18624=CARTESIAN_POINT('Ctrl Pts',(-6.767,1.16999331250164E-12,39.69717978381));
#18625=CARTESIAN_POINT('Ctrl Pts',(-6.76700000000003,-0.186007249414499,
39.705929295616));
#18626=CARTESIAN_POINT('Ctrl Pts',(-6.75932637295445,-0.372014355526342,
39.7146788074219));
#18627=CARTESIAN_POINT('Ctrl Pts',(-6.74400518266938,-0.55738953715385,
39.7234283192278));
#18628=CARTESIAN_POINT('Ctrl Pts',(-6.72868405709659,-0.742763935810203,
39.7321777940784));
#18629=CARTESIAN_POINT('Ctrl Pts',(-6.70571545653008,-0.927506129693848,
39.7409272689289));
#18630=CARTESIAN_POINT('Ctrl Pts',(-6.6751773941567,-1.11098863924858,39.7496767437795));
#18631=CARTESIAN_POINT('Ctrl Pts',(-6.6446394582309,-1.29447038906552,39.7584261824015));
#18632=CARTESIAN_POINT('Ctrl Pts',(-6.60653217027145,-1.47669218228271,
39.7671756210234));
#18633=CARTESIAN_POINT('Ctrl Pts',(-6.56098496116697,-1.65703510504179,
39.7759250596454));
#18634=CARTESIAN_POINT('Ctrl Pts',(-6.51543793687492,-1.83737729604111,
39.7846744627657));
#18635=CARTESIAN_POINT('Ctrl Pts',(-6.46245112202602,-2.01584035397174,
39.7934238658859));
#18636=CARTESIAN_POINT('Ctrl Pts',(-6.40220448416191,-2.19181813638294,
39.8021732690062));
#18637=CARTESIAN_POINT('Ctrl Pts',(-6.34195808575127,-2.36779521936106,
39.8109226373515));
#18638=CARTESIAN_POINT('Ctrl Pts',(-6.27445201489165,-2.54128677545001,
39.8196720056967));
#18639=CARTESIAN_POINT('Ctrl Pts',(-6.19991555136103,-2.71170355238025,
39.828421374042));
#18640=CARTESIAN_POINT('Ctrl Pts',(-6.12537937788953,-2.88211966613253,
39.8371707083391));
#18641=CARTESIAN_POINT('Ctrl Pts',(-6.04381298133527,-3.04946076210623,
39.8459200426361));
#18642=CARTESIAN_POINT('Ctrl Pts',(-5.95549339426212,-3.2131584820703,39.8546693769332));
#18643=CARTESIAN_POINT('Ctrl Pts',(-5.86717414355061,-3.37685557859809,
39.8634186779087));
#18644=CARTESIAN_POINT('Ctrl Pts',(-5.77210188986133,-3.53690907467482,
39.8721679788843));
#18645=CARTESIAN_POINT('Ctrl Pts',(-5.67059953466958,-3.69277536785074,
39.8809172798599));
#18646=CARTESIAN_POINT('Ctrl Pts',(-5.56909755761669,-3.84864108035931,
39.8896665482406));
#18647=CARTESIAN_POINT('Ctrl Pts',(-5.4611656833799,-4.00031938104387,39.8984158166214));
#18648=CARTESIAN_POINT('Ctrl Pts',(-5.34717048686053,-4.14729511663298,
39.9071650850021));
#18649=CARTESIAN_POINT('Ctrl Pts',(-5.23317570555455,-4.29427031688116,
39.9159143215147));
#18650=CARTESIAN_POINT('Ctrl Pts',(-5.11311782178743,-4.43654275987201,
39.9246635580273));
#18651=CARTESIAN_POINT('Ctrl Pts',(-4.98740459171952,-4.57362924147717,
39.93341279454));
#18652=CARTESIAN_POINT('Ctrl Pts',(-4.86169180910768,-4.710715235145,39.9421619999111));
#18653=CARTESIAN_POINT('Ctrl Pts',(-4.7303239141537,-4.84261509316583,39.9509112052822));
#18654=CARTESIAN_POINT('Ctrl Pts',(-4.59374707237233,-4.96888084331579,
39.9596604106533));
#18655=CARTESIAN_POINT('Ctrl Pts',(-4.45717070537335,-5.09514615452783,
39.9684095856095));
#18656=CARTESIAN_POINT('Ctrl Pts',(-4.31538563819435,-5.21577720253694,
39.9771587605658));
#18657=CARTESIAN_POINT('Ctrl Pts',(-4.16887341290566,-5.33036429028714,
39.985907935522));
#18658=CARTESIAN_POINT('Ctrl Pts',(-4.02236168477252,-5.44495098921241,
39.9946570807899));
#18659=CARTESIAN_POINT('Ctrl Pts',(-3.87112305634348,-5.55349359238823,
40.0034062260578));
#18660=CARTESIAN_POINT('Ctrl Pts',(-3.71567117316636,-5.65562346102536,
40.0121553713258));
#18661=CARTESIAN_POINT('Ctrl Pts',(-3.56021980457203,-5.75775299158829,
40.0209044876319));
#18662=CARTESIAN_POINT('Ctrl Pts',(-3.40055544862289,-5.85346967275411,
40.0296536039381));
#18663=CARTESIAN_POINT('Ctrl Pts',(-3.23722036323303,-5.94244842803616,
40.0384027202442));
#18664=CARTESIAN_POINT('Ctrl Pts',(-3.07388580495955,-6.03142689616522,
40.0471518083152));
#18665=CARTESIAN_POINT('Ctrl Pts',(-2.90688079257624,-6.11366734484862,
40.0559008963861));
#18666=CARTESIAN_POINT('Ctrl Pts',(-2.73677251094541,-6.18889046787335,
40.0646499844571));
#18667=CARTESIAN_POINT('Ctrl Pts',(-2.56666476416557,-6.26411335438307,
40.0733990450193));
#18668=CARTESIAN_POINT('Ctrl Pts',(-2.39345402971991,-6.3323188435033,40.0821481055815));
#18669=CARTESIAN_POINT('Ctrl Pts',(-2.21772856473922,-6.39327529621084,
40.0908971661438));
#18670=CARTESIAN_POINT('Ctrl Pts',(-2.04200363768161,-6.45423156232116,
40.0996461999238));
#18671=CARTESIAN_POINT('Ctrl Pts',(-1.86376426619992,-6.50793874252085,
40.1083952337038));
#18672=CARTESIAN_POINT('Ctrl Pts',(-1.68361578194596,-6.55421443796147,
40.1171442674838));
#18673=CARTESIAN_POINT('Ctrl Pts',(-1.50346783419762,-6.60048999558704,
40.125893275208));
#18674=CARTESIAN_POINT('Ctrl Pts',(-1.32141106257128,-6.63933404145519,
40.1346422829322));
#18675=CARTESIAN_POINT('Ctrl Pts',(-1.13806375958912,-6.67061465527052,
40.1433912906565));
#18676=CARTESIAN_POINT('Ctrl Pts',(-0.954716987417324,-6.70189517852508,
40.1521402730514));
#18677=CARTESIAN_POINT('Ctrl Pts',(-0.770079973807532,-6.72561226535856,
40.1608892554463));
#18678=CARTESIAN_POINT('Ctrl Pts',(-0.584779770549598,-6.74168536939807,
40.1696382378412));
#18679=CARTESIAN_POINT('Ctrl Pts',(-0.391490647551099,-6.7584514394241,
40.1787644185172));
#18680=CARTESIAN_POINT('Ctrl Pts',(-0.197480213101576,-6.76689975924034,
40.1878905991933));
#18681=CARTESIAN_POINT('Ctrl Pts',(-0.00346532629509061,-6.76699911271708,
40.1970167798694));
#18682=CARTESIAN_POINT('Ctrl Pts',(0.184486595298722,-6.76709536139766,
40.2058577673993));
#18683=CARTESIAN_POINT('Ctrl Pts',(0.372442378187854,-6.75935659726755,
40.2146987549292));
#18684=CARTESIAN_POINT('Ctrl Pts',(0.559750217724665,-6.74380965728995,
40.2235397424591));
#18685=CARTESIAN_POINT('Ctrl Pts',(0.745129914460262,-6.72842275717225,
40.2322897210569));
#18686=CARTESIAN_POINT('Ctrl Pts',(0.929874656316616,-6.70538772273439,
40.2410396996547));
#18687=CARTESIAN_POINT('Ctrl Pts',(1.11335688290013,-6.67478280180703,40.2497896782524));
#18688=CARTESIAN_POINT('Ctrl Pts',(1.29683723119084,-6.64417819417979,40.2585395672774));
#18689=CARTESIAN_POINT('Ctrl Pts',(1.47905480730455,-6.60600390230026,40.2672894563023));
#18690=CARTESIAN_POINT('Ctrl Pts',(1.6593906480502,-6.56038959797081,40.2760393453272));
#18691=CARTESIAN_POINT('Ctrl Pts',(1.83972470264474,-6.51477574543197,40.2847891476882));
#18692=CARTESIAN_POINT('Ctrl Pts',(2.01817678126054,-6.46172209820035,40.2935389500491));
#18693=CARTESIAN_POINT('Ctrl Pts',(2.19414072347883,-6.40140886723945,40.3022887524101));
#18694=CARTESIAN_POINT('Ctrl Pts',(2.37010298132305,-6.34109621361297,40.3110384710156));
#18695=CARTESIAN_POINT('Ctrl Pts',(2.54357687927126,-6.27352420825885,40.3197881896211));
#18696=CARTESIAN_POINT('Ctrl Pts',(2.71397317790188,-6.19892237325401,40.3285379082266));
#18697=CARTESIAN_POINT('Ctrl Pts',(2.88436790207409,-6.12432122756865,40.3372875459848));
#18698=CARTESIAN_POINT('Ctrl Pts',(3.05168482126455,-6.04269049717317,40.3460371837431));
#18699=CARTESIAN_POINT('Ctrl Pts',(3.21535561997577,-5.95430745234828,40.3547868215013));
#18700=CARTESIAN_POINT('Ctrl Pts',(3.37902496075465,-5.8659251948141,40.3635363813204));
#18701=CARTESIAN_POINT('Ctrl Pts',(3.53904799385056,-5.77079087940121,40.3722859411394));
#18702=CARTESIAN_POINT('Ctrl Pts',(3.69488118815161,-5.66922763746909,40.3810355009584));
#18703=CARTESIAN_POINT('Ctrl Pts',(3.85071304611008,-5.56766526648931,40.3897849857458));
#18704=CARTESIAN_POINT('Ctrl Pts',(4.00235489706141,-5.45967423580587,40.3985344705333));
#18705=CARTESIAN_POINT('Ctrl Pts',(4.14929168607826,-5.34562133936195,40.4072839553207));
#18706=CARTESIAN_POINT('Ctrl Pts',(4.29622726385915,-5.23156938308401,40.416033367984));
#18707=CARTESIAN_POINT('Ctrl Pts',(4.43845763092212,-5.11145583677076,40.4247827806473));
#18708=CARTESIAN_POINT('Ctrl Pts',(4.57549970661095,-4.9856886620409,40.4335321933106));
#18709=CARTESIAN_POINT('Ctrl Pts',(4.71254069815417,-4.85992248226042,40.4422815367569));
#18710=CARTESIAN_POINT('Ctrl Pts',(4.84439326931427,-4.72850295733886,40.4510308802032));
#18711=CARTESIAN_POINT('Ctrl Pts',(4.97060959434801,-4.5918764422157,40.4597802236496));
#18712=CARTESIAN_POINT('Ctrl Pts',(5.09682496280611,-4.45525096256553,40.4685295007858));
#18713=CARTESIAN_POINT('Ctrl Pts',(5.21740397615928,-4.31341878218217,40.4772787779221));
#18714=CARTESIAN_POINT('Ctrl Pts',(5.33193710452017,-4.16686161438571,40.4860280550584));
#18715=CARTESIAN_POINT('Ctrl Pts',(5.44646940289463,-4.02030550864405,40.4947772687914));
#18716=CARTESIAN_POINT('Ctrl Pts',(5.55495572749743,-3.86902470980022,40.5035264825244));
#18717=CARTESIAN_POINT('Ctrl Pts',(5.65702762491531,-3.71353301465667,40.5122756962573));
#18718=CARTESIAN_POINT('Ctrl Pts',(5.75909881655234,-3.55804239466763,40.5210248494934));
#18719=CARTESIAN_POINT('Ctrl Pts',(5.85475551250867,-3.39834117619407,40.5297740027295));
#18720=CARTESIAN_POINT('Ctrl Pts',(5.94367283728183,-3.23497174691808,40.5385231559657));
#18721=CARTESIAN_POINT('Ctrl Pts',(6.03258957676403,-3.07160339300787,40.5472722516112));
#18722=CARTESIAN_POINT('Ctrl Pts',(6.11476689685378,-2.90456712829307,40.5560213472568));
#18723=CARTESIAN_POINT('Ctrl Pts',(6.18992570525356,-2.7344302447569,40.5647704429023));
#18724=CARTESIAN_POINT('Ctrl Pts',(6.26508404388792,-2.56429442462801,40.5735194838633));
#18725=CARTESIAN_POINT('Ctrl Pts',(6.33322384283407,-2.39105828655749,40.5822685248244));
#18726=CARTESIAN_POINT('Ctrl Pts',(6.39411368720122,-2.21531017131823,40.5910175657854));
#18727=CARTESIAN_POINT('Ctrl Pts',(6.45500317120969,-2.03956309619263,40.5997665549678));
#18728=CARTESIAN_POINT('Ctrl Pts',(6.50864269270143,-1.86130434438389,40.6085155441502));
#18729=CARTESIAN_POINT('Ctrl Pts',(6.55485008446394,-1.68113930719709,40.6172645333326));
#18730=CARTESIAN_POINT('Ctrl Pts',(6.60199664749458,-1.49731239211603,40.626191346862));
#18731=CARTESIAN_POINT('Ctrl Pts',(6.64140563640953,-1.31150116499434,40.6351181603913));
#18732=CARTESIAN_POINT('Ctrl Pts',(6.67293772282212,-1.12436255155423,40.6440449739207));
#18733=CARTESIAN_POINT('Ctrl Pts',(6.70384494949903,-0.94093239504902,40.6527948880762));
#18734=CARTESIAN_POINT('Ctrl Pts',(6.72718449348956,-0.756227260504442,
40.6615448022318));
#18735=CARTESIAN_POINT('Ctrl Pts',(6.74287707373951,-0.570874564539475,
40.6702947163873));
#18736=CARTESIAN_POINT('Ctrl Pts',(6.75856934538683,-0.38552551363027,40.6790444584713));
#18737=CARTESIAN_POINT('Ctrl Pts',(6.76661493004109,-0.199529212416038,
40.6877942005552));
#18738=CARTESIAN_POINT('Ctrl Pts',(6.76698649908907,-0.0135174385982532,
40.6965439426392));
#18739=CARTESIAN_POINT('Ctrl Pts',(6.76735806132384,0.172490924447966,40.7052935242851));
#18740=CARTESIAN_POINT('Ctrl Pts',(6.76005588896278,0.358514472903606,40.714043105931));
#18741=CARTESIAN_POINT('Ctrl Pts',(6.74510478454567,0.54392135966442,40.7227926875769));
#18742=CARTESIAN_POINT('Ctrl Pts',(6.73015393440664,0.72932509315264,40.7315421204159));
#18743=CARTESIAN_POINT('Ctrl Pts',(6.70755443556867,0.914111900258532,40.740291553255));
#18744=CARTESIAN_POINT('Ctrl Pts',(6.67738304682283,1.09765415591754,40.749040986094));
#18745=CARTESIAN_POINT('Ctrl Pts',(6.6472121311182,1.28119353391484,40.7577902817554));
#18746=CARTESIAN_POINT('Ctrl Pts',(6.60946960955449,1.46348811672858,40.7665395774167));
#18747=CARTESIAN_POINT('Ctrl Pts',(6.56428366991133,1.64391876348421,40.775288873078));
#18748=CARTESIAN_POINT('Ctrl Pts',(6.51909837867661,1.82434682109917,40.7840380431888));
#18749=CARTESIAN_POINT('Ctrl Pts',(6.46646995271858,2.00291071820648,40.7927872132997));
#18750=CARTESIAN_POINT('Ctrl Pts',(6.4065771328148,2.17900400212908,40.8015363834105));
#18751=CARTESIAN_POINT('Ctrl Pts',(6.34668509278983,2.35509499309866,40.8102854395963));
#18752=CARTESIAN_POINT('Ctrl Pts',(6.27952894037441,2.52871516398333,40.819034495782));
#18753=CARTESIAN_POINT('Ctrl Pts',(6.20533675061354,2.69927486771633,40.8277835519678));
#18754=CARTESIAN_POINT('Ctrl Pts',(6.12832117907822,2.87632521636124,40.8368655532501));
#18755=CARTESIAN_POINT('Ctrl Pts',(6.04372366625984,3.05007728920185,40.8459475545324));
#18756=CARTESIAN_POINT('Ctrl Pts',(5.95185378007773,3.2198952747837,40.8550295558146));
#18757=CARTESIAN_POINT('Ctrl Pts',(5.86334450817268,3.38350129286931,40.8637793361217));
#18758=CARTESIAN_POINT('Ctrl Pts',(5.76808562057143,3.54345567125145,40.8725291164289));
#18759=CARTESIAN_POINT('Ctrl Pts',(5.66640068804362,3.69921508465496,40.881278896736));
#18760=CARTESIAN_POINT('Ctrl Pts',(5.56471941107797,3.85496889852466,40.8900283624895));
#18761=CARTESIAN_POINT('Ctrl Pts',(5.45661270814982,4.00652780919816,40.898777828243));
#18762=CARTESIAN_POINT('Ctrl Pts',(5.34244776448978,4.15337704569404,40.9075272939964));
#18763=CARTESIAN_POINT('Ctrl Pts',(5.22828631819447,4.3002217835643,40.916276491716));
#18764=CARTESIAN_POINT('Ctrl Pts',(5.10806717843909,4.44235690972864,40.9250256894356));
#18765=CARTESIAN_POINT('Ctrl Pts',(4.98219864544546,4.57929969070834,40.9337748871553));
#18766=CARTESIAN_POINT('Ctrl Pts',(4.85633329943826,4.71623900430207,40.9425238633455));
#18767=CARTESIAN_POINT('Ctrl Pts',(4.72481904033422,4.84798602483838,40.9512728395357));
#18768=CARTESIAN_POINT('Ctrl Pts',(4.58810250736944,4.97409332259361,40.960021815726));
#18769=CARTESIAN_POINT('Ctrl Pts',(4.45137708685385,5.1002088182236,40.9687713606622));
#18770=CARTESIAN_POINT('Ctrl Pts',(4.30944892635792,5.22068366308147,40.9775209055984));
#18771=CARTESIAN_POINT('Ctrl Pts',(4.162800094664,5.33510865605054,40.9862704505345));
#18772=CARTESIAN_POINT('Ctrl Pts',(4.01615988348534,5.44952692273078,40.9950194811428));
#18773=CARTESIAN_POINT('Ctrl Pts',(3.86479978231984,5.55789587288798,41.0037685117511));
#18774=CARTESIAN_POINT('Ctrl Pts',(3.70923383580829,5.65984746714034,41.0125175423593));
#18775=CARTESIAN_POINT('Ctrl Pts',(3.5536657779929,5.76180044505538,41.0212666917074));
#18776=CARTESIAN_POINT('Ctrl Pts',(3.39389200026577,5.85733573571212,41.0300158410554));
#18777=CARTESIAN_POINT('Ctrl Pts',(3.23045513625766,5.94612887622078,41.0387649904034));
#18778=CARTESIAN_POINT('Ctrl Pts',(3.18695122151392,5.96976399206787,41.0410938545163));
#18779=CARTESIAN_POINT('Ctrl Pts',(3.14318791262567,5.99292165435383,41.0434227186293));
#18780=CARTESIAN_POINT('Ctrl Pts',(3.09917575053253,6.01559628526642,41.0457515827422));
#18781=CARTESIAN_POINT('Ctrl Pts',(3.09917575053254,6.01559628526642,39.0455765095776));
#18782=CARTESIAN_POINT('Ctrl Pts',(2.94385435927471,6.09561633091081,39.0537889104959));
#18783=CARTESIAN_POINT('Ctrl Pts',(2.78553706128792,6.16956278200781,39.0620013114142));
#18784=CARTESIAN_POINT('Ctrl Pts',(2.62474477414606,6.23722725821282,39.0702137123324));
#18785=CARTESIAN_POINT('Ctrl Pts',(2.46373037286765,6.30498520430357,39.0784374576402));
#18786=CARTESIAN_POINT('Ctrl Pts',(2.30023448502693,6.36644370565575,39.086661202948));
#18787=CARTESIAN_POINT('Ctrl Pts',(2.13479521821867,6.42144363646297,39.0948849482558));
#18788=CARTESIAN_POINT('Ctrl Pts',(1.9768168502074,6.47396320740453,39.1027378231369));
#18789=CARTESIAN_POINT('Ctrl Pts',(1.8170668025288,6.52059390228783,39.110590698018));
#18790=CARTESIAN_POINT('Ctrl Pts',(1.65602197365155,6.56124075330141,39.1184435728991));
#18791=CARTESIAN_POINT('Ctrl Pts',(1.47871771179268,6.60599139798894,39.1270892909515));
#18792=CARTESIAN_POINT('Ctrl Pts',(1.2994398801499,6.64359094358373,39.1357350090038));
#18793=CARTESIAN_POINT('Ctrl Pts',(1.1187787795732,6.67387616324851,39.1443807270562));
#18794=CARTESIAN_POINT('Ctrl Pts',(0.938349611031916,6.70412250286321,39.1530153457685));
#18795=CARTESIAN_POINT('Ctrl Pts',(0.756541014008898,6.72707319072024,39.1616499644808));
#18796=CARTESIAN_POINT('Ctrl Pts',(0.573955540286112,6.74261551905304,39.1702845831931));
#18797=CARTESIAN_POINT('Ctrl Pts',(0.384921856918772,6.75870674204548,39.1792241430956));
#18798=CARTESIAN_POINT('Ctrl Pts',(0.19505572705101,6.76685667977349,39.1881637029981));
#18799=CARTESIAN_POINT('Ctrl Pts',(0.0050371983657768,6.76699812521273,
39.1971032629005));
#18800=CARTESIAN_POINT('Ctrl Pts',(-0.177990118787014,6.76713436655428,
39.205713916171));
#18801=CARTESIAN_POINT('Ctrl Pts',(-0.361158472792682,6.75984085858258,
39.2143245694415));
#18802=CARTESIAN_POINT('Ctrl Pts',(-0.543854620886027,6.74511016598995,
39.2229352227119));
#18803=CARTESIAN_POINT('Ctrl Pts',(-0.726377834852708,6.73039341698335,
39.231537725423));
#18804=CARTESIAN_POINT('Ctrl Pts',(-0.908429431051354,6.70825354324155,
39.2401402281341));
#18805=CARTESIAN_POINT('Ctrl Pts',(-1.08939709403731,6.67873513260581,39.2487427308452));
#18806=CARTESIAN_POINT('Ctrl Pts',(-1.27016108156082,6.64924994434713,39.2573355516126));
#18807=CARTESIAN_POINT('Ctrl Pts',(-1.44984326925202,6.61240283520988,39.26592837238));
#18808=CARTESIAN_POINT('Ctrl Pts',(-1.62783717121543,6.56829012331287,39.2745211931475));
#18809=CARTESIAN_POINT('Ctrl Pts',(-1.6488145610587,6.56309123984383,39.2755338961059));
#18810=CARTESIAN_POINT('Ctrl Pts',(-1.66976850853207,6.55779149843397,39.2765465990642));
#18811=CARTESIAN_POINT('Ctrl Pts',(-1.69069802736641,6.5523911040367,39.2775593020226));
#18812=CARTESIAN_POINT('Ctrl Pts',(-1.86833610740447,6.50655556907902,39.2861545597827));
#18813=CARTESIAN_POINT('Ctrl Pts',(-2.04400450180928,6.45351909298188,39.2947498175428));
#18814=CARTESIAN_POINT('Ctrl Pts',(-2.21712304950587,6.39348530797951,39.3033450753028));
#18815=CARTESIAN_POINT('Ctrl Pts',(-2.39040371538069,6.33339530388341,39.3119483821573));
#18816=CARTESIAN_POINT('Ctrl Pts',(-2.5611294798661,6.26629501151802,39.3205516890117));
#18817=CARTESIAN_POINT('Ctrl Pts',(-2.7287399612937,6.19243629144773,39.3291549958662));
#18818=CARTESIAN_POINT('Ctrl Pts',(-2.903299631403,6.11551536323158,39.3381149988061));
#18819=CARTESIAN_POINT('Ctrl Pts',(-3.07447984919786,6.03126381812536,39.3470750017461));
#18820=CARTESIAN_POINT('Ctrl Pts',(-3.24167696116458,5.94001847467285,39.3560350046861));
#18821=CARTESIAN_POINT('Ctrl Pts',(-3.40265718392653,5.85216590627502,39.3646618478909));
#18822=CARTESIAN_POINT('Ctrl Pts',(-3.55994493731526,5.75783045377207,39.3732886910956));
#18823=CARTESIAN_POINT('Ctrl Pts',(-3.71303159681705,5.65735674684196,39.3819155343004));
#18824=CARTESIAN_POINT('Ctrl Pts',(-3.86626456846748,5.55678701244616,39.3905506225865));
#18825=CARTESIAN_POINT('Ctrl Pts',(-4.01528818196723,5.45006748831492,39.3991857108726));
#18826=CARTESIAN_POINT('Ctrl Pts',(-4.15962561129012,5.33758407651807,39.4078207991588));
#18827=CARTESIAN_POINT('Ctrl Pts',(-4.30417741066163,5.2249336042812,39.4164687122839));
#18828=CARTESIAN_POINT('Ctrl Pts',(-4.44402888199815,5.10650233121538,39.4251166254091));
#18829=CARTESIAN_POINT('Ctrl Pts',(-4.57873775253373,4.98271508251499,39.4337645385342));
#18830=CARTESIAN_POINT('Ctrl Pts',(-4.59385003711008,4.96882803764671,39.4347347027381));
#18831=CARTESIAN_POINT('Ctrl Pts',(-4.60889763973489,4.95487362194797,39.435704866942));
#18832=CARTESIAN_POINT('Ctrl Pts',(-4.62387996649728,4.94085246242236,39.4366750311459));
#18833=CARTESIAN_POINT('Ctrl Pts',(-4.74854157233275,4.82418832274242,39.4447473572604));
#18834=CARTESIAN_POINT('Ctrl Pts',(-4.86898185269501,4.70261880533513,39.4528196833749));
#18835=CARTESIAN_POINT('Ctrl Pts',(-4.98478223331834,4.5764871994133,39.4608920094894));
#18836=CARTESIAN_POINT('Ctrl Pts',(-5.10045796800315,4.45049135981895,39.4689556466629));
#18837=CARTESIAN_POINT('Ctrl Pts',(-5.21150349247123,4.31994347684868,39.4770192838365));
#18838=CARTESIAN_POINT('Ctrl Pts',(-5.3175343112745,4.18522614065458,39.4850829210101));
#18839=CARTESIAN_POINT('Ctrl Pts',(-5.42347421070832,4.05062432196188,39.4931396437713));
#18840=CARTESIAN_POINT('Ctrl Pts',(-5.52440773430764,3.91186045804607,39.5011963665325));
#18841=CARTESIAN_POINT('Ctrl Pts',(-5.61998826768889,3.76935284512331,39.5092530892937));
#18842=CARTESIAN_POINT('Ctrl Pts',(-5.71550638463916,3.62693829316467,39.5173045508174));
#18843=CARTESIAN_POINT('Ctrl Pts',(-5.80567826454077,3.48078516888765,39.5253560123412));
#18844=CARTESIAN_POINT('Ctrl Pts',(-5.89019860143735,3.33134348808788,39.5334074738649));
#18845=CARTESIAN_POINT('Ctrl Pts',(-5.97468943816998,3.18195396697233,39.5414561251842));
#18846=CARTESIAN_POINT('Ctrl Pts',(-6.05353247338711,3.02927849746071,39.5495047765034));
#18847=CARTESIAN_POINT('Ctrl Pts',(-6.1264666303992,2.87379463890605,39.5575534278226));
#18848=CARTESIAN_POINT('Ctrl Pts',(-6.19938975985999,2.718334289312,39.565600862196));
#18849=CARTESIAN_POINT('Ctrl Pts',(-6.26640563102561,2.56006673359669,39.5736482965695));
#18850=CARTESIAN_POINT('Ctrl Pts',(-6.32729996666182,2.39949247381219,39.5816957309429));
#18851=CARTESIAN_POINT('Ctrl Pts',(-6.388197141872,2.23891072626247,39.5897435405776));
#18852=CARTESIAN_POINT('Ctrl Pts',(-6.44297208213749,2.07602240984482,39.5977913502123));
#18853=CARTESIAN_POINT('Ctrl Pts',(-6.49145938811474,1.91134612575982,39.6058391598469));
#18854=CARTESIAN_POINT('Ctrl Pts',(-6.53997991942607,1.74655699926286,39.6138924841449));
#18855=CARTESIAN_POINT('Ctrl Pts',(-6.58220410403456,1.57997781601481,39.6219458084428));
#18856=CARTESIAN_POINT('Ctrl Pts',(-6.61801684346878,1.4121409489012,39.6299991327407));
#18857=CARTESIAN_POINT('Ctrl Pts',(-6.65384226337064,1.24424465461178,39.6380553085356));
#18858=CARTESIAN_POINT('Ctrl Pts',(-6.68325165017052,1.07509015652775,39.6461114843305));
#18859=CARTESIAN_POINT('Ctrl Pts',(-6.70618148458003,0.90521759587185,39.6541676601254));
#18860=CARTESIAN_POINT('Ctrl Pts',(-6.72913758268588,0.735150464192443,
39.6622330634163));
#18861=CARTESIAN_POINT('Ctrl Pts',(-6.74559926635269,0.564363998166427,
39.6702984667071));
#18862=CARTESIAN_POINT('Ctrl Pts',(-6.75555504822545,0.393401817987186,
39.678363869998));
#18863=CARTESIAN_POINT('Ctrl Pts',(-6.76319043194,0.262285863155353,39.6845494664409));
#18864=CARTESIAN_POINT('Ctrl Pts',(-6.76700023386168,0.131066634845332,
39.6907350628838));
#18865=CARTESIAN_POINT('Ctrl Pts',(-6.76699999998923,-1.20737753336487E-5,
39.6969206593267));
#18866=CARTESIAN_POINT('',(-6.76699932393892,-0.00129874070200122,39.3028202161899));
#18867=CARTESIAN_POINT('Ctrl Pts',(3.09917575053265,6.01559628526636,38.651392015122));
#18868=CARTESIAN_POINT('Ctrl Pts',(2.93382384459268,6.10078395293758,38.6601414630345));
#18869=CARTESIAN_POINT('Ctrl Pts',(2.76495772122984,6.17915010267049,38.6688909109469));
#18870=CARTESIAN_POINT('Ctrl Pts',(2.59315093316708,6.25042856433179,38.6776403588593));
#18871=CARTESIAN_POINT('Ctrl Pts',(2.4213455324561,6.32170645041454,38.6863897361193));
#18872=CARTESIAN_POINT('Ctrl Pts',(2.24659977927579,6.38589665313462,38.6951391133793));
#18873=CARTESIAN_POINT('Ctrl Pts',(2.06950718689902,6.44278115439081,38.7038884906393));
#18874=CARTESIAN_POINT('Ctrl Pts',(1.89241596572834,6.49966521519732,38.712637800154));
#18875=CARTESIAN_POINT('Ctrl Pts',(1.71297821457159,6.54924360009556,38.7213871096686));
#18876=CARTESIAN_POINT('Ctrl Pts',(1.53180337335795,6.59134792173568,38.7301364191833));
#18877=CARTESIAN_POINT('Ctrl Pts',(1.35062987477735,6.63345193135314,38.7388856638594));
#18878=CARTESIAN_POINT('Ctrl Pts',(1.16771959102906,6.66808192368246,38.7476349085355));
#18879=CARTESIAN_POINT('Ctrl Pts',(0.983693746906403,6.69512028363175,38.7563841532117));
#18880=CARTESIAN_POINT('Ctrl Pts',(0.799669205419443,6.72215845218872,38.7651333359558));
#18881=CARTESIAN_POINT('Ctrl Pts',(0.614529402873063,6.74160505424583,38.7738825187));
#18882=CARTESIAN_POINT('Ctrl Pts',(0.428903127362849,6.75339404354125,38.7826317014442));
#18883=CARTESIAN_POINT('Ctrl Pts',(0.243278104163518,6.76518295330331,38.7913808251628));
#18884=CARTESIAN_POINT('Ctrl Pts',(0.0571669005387937,6.76931433552276,
38.8001299488814));
#18885=CARTESIAN_POINT('Ctrl Pts',(-0.128798404777798,6.76577415902472,
38.8088790726));
#18886=CARTESIAN_POINT('Ctrl Pts',(-0.314762517259266,6.7622340052344,38.8176281401992));
#18887=CARTESIAN_POINT('Ctrl Pts',(-0.500580446819561,6.75102239665088,
38.8263772077984));
#18888=CARTESIAN_POINT('Ctrl Pts',(-0.685621118842547,6.73217741012498,
38.8351262753976));
#18889=CARTESIAN_POINT('Ctrl Pts',(-0.870660665414616,6.71333253821771,
38.8438752897834));
#18890=CARTESIAN_POINT('Ctrl Pts',(-1.05492267885518,6.68685441030608,38.8526243041692));
#18891=CARTESIAN_POINT('Ctrl Pts',(-1.23778137635303,6.65283295028168,38.861373318555));
#18892=CARTESIAN_POINT('Ctrl Pts',(-1.42999922978899,6.61707018861854,38.8705701289224));
#18893=CARTESIAN_POINT('Ctrl Pts',(-1.62066601233749,6.572971729344,38.8797669392898));
#18894=CARTESIAN_POINT('Ctrl Pts',(-1.80906628500441,6.52070304311279,38.8889637496572));
#18895=CARTESIAN_POINT('Ctrl Pts',(-1.98831342545575,6.47097374915016,38.8977137473949));
#18896=CARTESIAN_POINT('Ctrl Pts',(-2.16550875896742,6.41384933989515,38.9064637451327));
#18897=CARTESIAN_POINT('Ctrl Pts',(-2.34005036714043,6.34952386240464,38.9152137428704));
#18898=CARTESIAN_POINT('Ctrl Pts',(-2.51458843547124,6.28519968948582,38.9239635631513));
#18899=CARTESIAN_POINT('Ctrl Pts',(-2.68647261718093,6.21367483971083,38.9327133834322));
#18900=CARTESIAN_POINT('Ctrl Pts',(-2.85511905908771,6.13519226743825,38.941463203713));
#18901=CARTESIAN_POINT('Ctrl Pts',(-3.02376230488915,6.05671118252921,38.9502128581716));
#18902=CARTESIAN_POINT('Ctrl Pts',(-3.18916767379927,5.9712727599262,38.9589625126301));
#18903=CARTESIAN_POINT('Ctrl Pts',(-3.35077334102802,5.87916720437988,38.9677121670886));
#18904=CARTESIAN_POINT('Ctrl Pts',(-3.51237616037378,5.78706327195637,38.9764616673571));
#18905=CARTESIAN_POINT('Ctrl Pts',(-3.67017916302305,5.68829258362295,38.9852111676255));
#18906=CARTESIAN_POINT('Ctrl Pts',(-3.82364636566463,5.58319061741042,38.9939606678939));
#18907=CARTESIAN_POINT('Ctrl Pts',(-3.97711106778813,5.47809036367691,39.0027100256024));
#18908=CARTESIAN_POINT('Ctrl Pts',(-4.12623987481956,5.36665920043203,39.0114593833108));
#18909=CARTESIAN_POINT('Ctrl Pts',(-4.27052628213971,5.249275595123,39.0202087410193));
#18910=CARTESIAN_POINT('Ctrl Pts',(-4.41481053025004,5.13189374643013,39.0289579677958));
#18911=CARTESIAN_POINT('Ctrl Pts',(-4.55425230136541,5.00855981477343,39.0377071945723));
#18912=CARTESIAN_POINT('Ctrl Pts',(-4.68837800630544,4.8796926819208,39.0464564213488));
#18913=CARTESIAN_POINT('Ctrl Pts',(-4.82250188228895,4.75082730631809,39.0552055288196));
#18914=CARTESIAN_POINT('Ctrl Pts',(-4.95130963052971,4.61642907903521,39.0639546362905));
#18915=CARTESIAN_POINT('Ctrl Pts',(-5.07436379033376,4.4769544473168,39.0727037437613));
#18916=CARTESIAN_POINT('Ctrl Pts',(-5.1974164356282,4.3374815322057,39.0814527435511));
#18917=CARTESIAN_POINT('Ctrl Pts',(-5.31471544462792,4.19293255254566,39.0902017433408));
#18918=CARTESIAN_POINT('Ctrl Pts',(-5.4258624527565,4.04379841779572,39.0989507431306));
#18919=CARTESIAN_POINT('Ctrl Pts',(-5.53702160019171,3.89464799484317,39.1077006984727));
#18920=CARTESIAN_POINT('Ctrl Pts',(-5.64202723081265,3.74091164443829,39.1164506538149));
#18921=CARTESIAN_POINT('Ctrl Pts',(-5.74052265232977,3.58311159163217,39.1252006091571));
#18922=CARTESIAN_POINT('Ctrl Pts',(-5.83901427066932,3.42531763191759,39.1339502266395));
#18923=CARTESIAN_POINT('Ctrl Pts',(-5.93099603115758,3.2634605269558,39.142699844122));
#18924=CARTESIAN_POINT('Ctrl Pts',(-6.01615550622775,3.09809004467035,39.1514494616044));
#18925=CARTESIAN_POINT('Ctrl Pts',(-6.10131214578811,2.93272506863801,39.1601987877555));
#18926=CARTESIAN_POINT('Ctrl Pts',(-6.17964682328752,2.76384720416884,39.1689481139066));
#18927=CARTESIAN_POINT('Ctrl Pts',(-6.25089348288561,2.59203002791599,39.1776974400577));
#18928=CARTESIAN_POINT('Ctrl Pts',(-6.32213814889322,2.42021765937049,39.1864465213892));
#18929=CARTESIAN_POINT('Ctrl Pts',(-6.38629508412572,2.24546640831952,39.1951956027208));
#18930=CARTESIAN_POINT('Ctrl Pts',(-6.44314639819796,2.06836976660091,39.2039446840524));
#18931=CARTESIAN_POINT('Ctrl Pts',(-6.50000285283688,1.89125711158319,39.2126945564868));
#18932=CARTESIAN_POINT('Ctrl Pts',(-6.5495522767324,1.71179891440291,39.2214444289211));
#18933=CARTESIAN_POINT('Ctrl Pts',(-6.59162635926378,1.53060476278461,39.2301943013555));
#18934=CARTESIAN_POINT('Ctrl Pts',(-6.63369752055195,1.34942319164708,39.2389435662781));
#18935=CARTESIAN_POINT('Ctrl Pts',(-6.66829431424256,1.16650618642698,39.2476928312006));
#18936=CARTESIAN_POINT('Ctrl Pts',(-6.69529923745421,0.982474997618313,
39.2564420961231));
#18937=CARTESIAN_POINT('Ctrl Pts',(-6.72230554731447,0.798434359177479,
39.2651918103028));
#18938=CARTESIAN_POINT('Ctrl Pts',(-6.74171916496706,0.613279706240057,
39.2739415244825));
#18939=CARTESIAN_POINT('Ctrl Pts',(-6.75347414817277,0.42763995365508,39.2826912386622));
#18940=CARTESIAN_POINT('Ctrl Pts',(-6.76248837758746,0.285283364198185,
39.2894008978381));
#18941=CARTESIAN_POINT('Ctrl Pts',(-6.76699999999998,0.142641701104637,
39.296110557014));
#18942=CARTESIAN_POINT('Ctrl Pts',(-6.767,9.97351951862395E-13,39.3028202161899));
#18943=CARTESIAN_POINT('Ctrl Pts',(-6.76699633264442,-0.00704513853499345,
39.3028202161899));
#18944=CARTESIAN_POINT('Ctrl Pts',(-6.76678563109908,-0.209428182884763,
39.3123086093829));
#18945=CARTESIAN_POINT('Ctrl Pts',(-6.75749211943877,-0.411404992939795,
39.3217970025758));
#18946=CARTESIAN_POINT('Ctrl Pts',(-6.73924769947695,-0.612233162361049,
39.3312853957688));
#18947=CARTESIAN_POINT('Ctrl Pts',(-6.72089665210696,-0.814235048855196,
39.3408292427814));
#18948=CARTESIAN_POINT('Ctrl Pts',(-6.69348987512733,-1.01507473245287,
39.350373089794));
#18949=CARTESIAN_POINT('Ctrl Pts',(-6.65721041637865,-1.214017492485,39.3599169368065));
#18950=CARTESIAN_POINT('Ctrl Pts',(-6.62065693333061,-1.41446289760368,
39.369532869955));
#18951=CARTESIAN_POINT('Ctrl Pts',(-6.57509630764718,-1.61298251877728,
39.3791488031034));
#18952=CARTESIAN_POINT('Ctrl Pts',(-6.52076377595837,-1.80884736176085,
39.3887647362518));
#18953=CARTESIAN_POINT('Ctrl Pts',(-6.48530923539211,-1.9366584135417,39.3950395863517));
#18954=CARTESIAN_POINT('Ctrl Pts',(-6.44612043584999,-2.06333947643613,
39.4013144364515));
#18955=CARTESIAN_POINT('Ctrl Pts',(-6.40327340508318,-2.18869337728117,
39.4075892865513));
#18956=CARTESIAN_POINT('Ctrl Pts',(-6.3470550497922,-2.35316662102052,39.4158223366834));
#18957=CARTESIAN_POINT('Ctrl Pts',(-6.28441350000255,-2.51571289750371,
39.4240553868154));
#18958=CARTESIAN_POINT('Ctrl Pts',(-6.2154978737592,-2.67579430848018,39.4322884369474));
#18959=CARTESIAN_POINT('Ctrl Pts',(-6.14666431543332,-2.83568508710315,
39.4405116827823));
#18960=CARTESIAN_POINT('Ctrl Pts',(-6.07157169842181,-2.9931165193161,39.4487349286171));
#18961=CARTESIAN_POINT('Ctrl Pts',(-5.99041885552366,-3.14756587466993,
39.456958174452));
#18962=CARTESIAN_POINT('Ctrl Pts',(-5.90934641027032,-3.30186221795454,
39.4651732735655));
#18963=CARTESIAN_POINT('Ctrl Pts',(-5.8222258612897,-3.45318205305921,39.473388372679));
#18964=CARTESIAN_POINT('Ctrl Pts',(-5.72930409986526,-3.60102256744763,
39.4816034717925));
#18965=CARTESIAN_POINT('Ctrl Pts',(-5.63645580371146,-3.74874619701559,
39.4898120759314));
#18966=CARTESIAN_POINT('Ctrl Pts',(-5.53781562029324,-3.89299568302011,
39.4980206800703));
#18967=CARTESIAN_POINT('Ctrl Pts',(-5.43367638296984,-4.03329269520027,
39.5062292842092));
#18968=CARTESIAN_POINT('Ctrl Pts',(-5.3295986488634,-4.17350684987348,39.5144330404582));
#18969=CARTESIAN_POINT('Ctrl Pts',(-5.22002854355738,-4.30977289408286,
39.5226367967072));
#18970=CARTESIAN_POINT('Ctrl Pts',(-5.10530228676486,-4.44164131383361,
39.5308405529561));
#18971=CARTESIAN_POINT('Ctrl Pts',(-4.99060997457976,-4.57347071704301,
39.5390418819204));
#18972=CARTESIAN_POINT('Ctrl Pts',(-4.87076478168693,-4.70090481521211,
39.5472432108847));
#18973=CARTESIAN_POINT('Ctrl Pts',(-4.74614345313542,-4.82352685514031,
39.555444539849));
#18974=CARTESIAN_POINT('Ctrl Pts',(-4.62153931105492,-4.9461319843185,39.5636447377717));
#18975=CARTESIAN_POINT('Ctrl Pts',(-4.49216059990032,-5.06392612520121,
39.5718449356944));
#18976=CARTESIAN_POINT('Ctrl Pts',(-4.35842120621914,-5.17652910637807,
39.5800451336172));
#18977=CARTESIAN_POINT('Ctrl Pts',(-4.22467602017784,-5.28913696448011,
39.588245686697));
#18978=CARTESIAN_POINT('Ctrl Pts',(-4.08657004939793,-5.39655298413444,
39.5964462397769));
#18979=CARTESIAN_POINT('Ctrl Pts',(-3.94455059937957,-5.49843701145464,
39.6046467928567));
#18980=CARTESIAN_POINT('Ctrl Pts',(-3.8024992616789,-5.6003439148351,39.6128491872099));
#18981=CARTESIAN_POINT('Ctrl Pts',(-3.65653298568674,-5.69671614316347,
39.6210515815632));
#18982=CARTESIAN_POINT('Ctrl Pts',(-3.50712844921679,-5.78725660746906,
39.6292539759164));
#18983=CARTESIAN_POINT('Ctrl Pts',(-3.35758419324149,-5.87788174302483,
39.6374640409502));
#18984=CARTESIAN_POINT('Ctrl Pts',(-3.20459555953907,-5.96266403254292,
39.6456741059841));
#18985=CARTESIAN_POINT('Ctrl Pts',(-3.04866507112388,-6.04135169346308,
39.6538841710179));
#18986=CARTESIAN_POINT('Ctrl Pts',(-2.8926599571431,-6.12007701290186,39.6620981652432));
#18987=CARTESIAN_POINT('Ctrl Pts',(-2.73371050698783,-6.19270173934441,
39.6703121594686));
#18988=CARTESIAN_POINT('Ctrl Pts',(-2.57233958649055,-6.25902213223229,
39.6785261536939));
#18989=CARTESIAN_POINT('Ctrl Pts',(-2.41074866368255,-6.3254329419043,39.6867513463291));
#18990=CARTESIAN_POINT('Ctrl Pts',(-2.24673000941149,-6.38552211770407,
39.6949765389643));
#18991=CARTESIAN_POINT('Ctrl Pts',(-2.08082318680931,-6.43913533521674,
39.7032017315995));
#18992=CARTESIAN_POINT('Ctrl Pts',(-1.93162353658767,-6.48734958689539,
39.7105986297193));
#18993=CARTESIAN_POINT('Ctrl Pts',(-1.78089722348275,-6.53032712087692,
39.7179955278392));
#18994=CARTESIAN_POINT('Ctrl Pts',(-1.62904318274137,-6.56799111667821,
39.725392425959));
#18995=CARTESIAN_POINT('Ctrl Pts',(-1.45154649068435,-6.61201519816949,
39.7340383924499));
#18996=CARTESIAN_POINT('Ctrl Pts',(-1.27210607238131,-6.6488791593914,39.7426843589408));
#18997=CARTESIAN_POINT('Ctrl Pts',(-1.0913129970232,-6.67842233933496,39.7513303254317));
#18998=CARTESIAN_POINT('Ctrl Pts',(-0.910751180586849,-6.70792772953506,
39.7599652325561));
#18999=CARTESIAN_POINT('Ctrl Pts',(-0.728840456798993,-6.7301309624288,
39.7686001396804));
#19000=CARTESIAN_POINT('Ctrl Pts',(-0.546183922364777,-6.744921950842,39.7772350468048));
#19001=CARTESIAN_POINT('Ctrl Pts',(-0.357463338412182,-6.76020398813249,
39.7861566258763));
#19002=CARTESIAN_POINT('Ctrl Pts',(-0.167946876348377,-6.76757305659514,
39.7950782049478));
#19003=CARTESIAN_POINT('Ctrl Pts',(0.0216892493982601,-6.76696524126292,
39.8039997840193));
#19004=CARTESIAN_POINT('Ctrl Pts',(0.204724993366466,-6.76637858125239,
39.812610842995));
#19005=CARTESIAN_POINT('Ctrl Pts',(0.387871866214309,-6.75836091852008,
39.8212219019707));
#19006=CARTESIAN_POINT('Ctrl Pts',(0.570516541991954,-6.74290737555497,
39.8298329609464));
#19007=CARTESIAN_POINT('Ctrl Pts',(0.752988975408527,-6.72746840599429,
39.838435899296));
#19008=CARTESIAN_POINT('Ctrl Pts',(0.934959853108263,-6.70460756267172,
39.8470388376455));
#19009=CARTESIAN_POINT('Ctrl Pts',(1.11581699663422,-6.6743719876871,39.8556417759951));
#19010=CARTESIAN_POINT('Ctrl Pts',(1.29647162199824,-6.64417026955187,39.8642350810438));
#19011=CARTESIAN_POINT('Ctrl Pts',(1.47601470102438,-6.60661034439889,39.8728283860926));
#19012=CARTESIAN_POINT('Ctrl Pts',(1.65384009905333,-6.56179106088904,39.8814216911414));
#19013=CARTESIAN_POINT('Ctrl Pts',(1.67365275909974,-6.55679745908892,39.8823791259819));
#19014=CARTESIAN_POINT('Ctrl Pts',(1.69344410338551,-6.55171379529251,39.8833365608225));
#19015=CARTESIAN_POINT('Ctrl Pts',(1.71321329922587,-6.54654024591277,39.884293995663));
#19016=CARTESIAN_POINT('Ctrl Pts',(1.8906992305479,-6.50009261914438,39.8928897532106));
#19017=CARTESIAN_POINT('Ctrl Pts',(2.06619101226672,-6.44645022952148,39.9014855107581));
#19018=CARTESIAN_POINT('Ctrl Pts',(2.23910910938076,-6.38581861598716,39.9100812683057));
#19019=CARTESIAN_POINT('Ctrl Pts',(2.41218854495864,-6.32513043109592,39.9186850459873));
#19020=CARTESIAN_POINT('Ctrl Pts',(2.58268921467238,-6.25744010679457,39.9272888236689));
#19021=CARTESIAN_POINT('Ctrl Pts',(2.75005151816753,-6.18300134622535,39.9358926013506));
#19022=CARTESIAN_POINT('Ctrl Pts',(2.92399130653878,-6.10563707727332,39.9448345150186));
#19023=CARTESIAN_POINT('Ctrl Pts',(3.09454072032255,-6.02098337137873,39.9537764286866));
#19024=CARTESIAN_POINT('Ctrl Pts',(3.26110085699704,-5.92937688129985,39.9627183423546));
#19025=CARTESIAN_POINT('Ctrl Pts',(3.4217988968878,-5.84099448866459,39.9713455446853));
#19026=CARTESIAN_POINT('Ctrl Pts',(3.57878345104977,-5.74614057350822,39.979972747016));
#19027=CARTESIAN_POINT('Ctrl Pts',(3.73154691430984,-5.64516134634828,39.9885999493467));
#19028=CARTESIAN_POINT('Ctrl Pts',(3.88445586138645,-5.54408595193051,39.9972353677672));
#19029=CARTESIAN_POINT('Ctrl Pts',(4.03313544439508,-5.43687377724324,40.0058707861876));
#19030=CARTESIAN_POINT('Ctrl Pts',(4.17710997963996,-5.32391220983144,40.0145062046081));
#19031=CARTESIAN_POINT('Ctrl Pts',(4.3212972167531,-5.21078375779389,40.0231543806292));
#19032=CARTESIAN_POINT('Ctrl Pts',(4.46076528075879,-5.09188913384303,40.0318025566503));
#19033=CARTESIAN_POINT('Ctrl Pts',(4.59507316255803,-4.96765454019691,40.0404507326715));
#19034=CARTESIAN_POINT('Ctrl Pts',(4.60928242719726,-4.95451099124939,40.0413656769032));
#19035=CARTESIAN_POINT('Ctrl Pts',(4.62343397034782,-4.94130770519692,40.042280621135));
#19036=CARTESIAN_POINT('Ctrl Pts',(4.6375272953042,-4.92804520934098,40.0431955653667));
#19037=CARTESIAN_POINT('Ctrl Pts',(4.76423620493021,-4.80880603802919,40.0514215579081));
#19038=CARTESIAN_POINT('Ctrl Pts',(4.88650968612764,-4.6845203573194,40.0596475504494));
#19039=CARTESIAN_POINT('Ctrl Pts',(5.00392275384399,-4.55555112731296,40.0678735429908));
#19040=CARTESIAN_POINT('Ctrl Pts',(5.12121272913508,-4.42671710487426,40.0760909116422));
#19041=CARTESIAN_POINT('Ctrl Pts',(5.2336521987825,-4.29320957372223,40.0843082802936));
#19042=CARTESIAN_POINT('Ctrl Pts',(5.34085104333207,-4.15543007797493,40.092525648945));
#19043=CARTESIAN_POINT('Ctrl Pts',(5.44795895377338,-4.01776745714017,40.1007360470074));
#19044=CARTESIAN_POINT('Ctrl Pts',(5.5498348741313,-3.87584037018802,40.1089464450698));
#19045=CARTESIAN_POINT('Ctrl Pts',(5.64612714378422,-3.73008542478896,40.1171568431322));
#19046=CARTESIAN_POINT('Ctrl Pts',(5.74235699334489,-3.58442496295718,40.1253619189209));
#19047=CARTESIAN_POINT('Ctrl Pts',(5.83301020523841,-3.43494188323044,40.1335669947097));
#19048=CARTESIAN_POINT('Ctrl Pts',(5.91777680708612,-3.28210399919224,40.1417720704985));
#19049=CARTESIAN_POINT('Ctrl Pts',(6.00250541339887,-3.12933462276243,40.149973468468));
#19050=CARTESIAN_POINT('Ctrl Pts',(6.0813524931119,-2.97321375059752,40.1581748664374));
#19051=CARTESIAN_POINT('Ctrl Pts',(6.15405259617078,-2.81423624515847,40.1663762644069));
#19052=CARTESIAN_POINT('Ctrl Pts',(6.22674700475229,-2.65527119216133,40.1745770199746));
#19053=CARTESIAN_POINT('Ctrl Pts',(6.29329523892015,-2.49345027353249,40.1827777755423));
#19054=CARTESIAN_POINT('Ctrl Pts',(6.3534786747419,-2.32929125048801,40.19097853111));
#19055=CARTESIAN_POINT('Ctrl Pts',(6.41366180486043,-2.16513306129323,40.1991792450218));
#19056=CARTESIAN_POINT('Ctrl Pts',(6.46748007667239,-1.99863712744613,40.2073799589336));
#19057=CARTESIAN_POINT('Ctrl Pts',(6.51476377714247,-1.8303392931455,40.2155806728454));
#19058=CARTESIAN_POINT('Ctrl Pts',(6.56205580641776,-1.66201181395955,40.223782831275));
#19059=CARTESIAN_POINT('Ctrl Pts',(6.60281087417786,-1.49188214698168,40.2319849897046));
#19060=CARTESIAN_POINT('Ctrl Pts',(6.63690970038484,-1.32049938619359,40.2401871481342));
#19061=CARTESIAN_POINT('Ctrl Pts',(6.67102071256402,-1.14905537797291,40.2483922377871));
#19062=CARTESIAN_POINT('Ctrl Pts',(6.69847067468287,-0.976357735117145,
40.25659732744));
#19063=CARTESIAN_POINT('Ctrl Pts',(6.71919177212339,-0.802963840673674,
40.264802417093));
#19064=CARTESIAN_POINT('Ctrl Pts',(6.73993654096788,-0.629371864206111,
40.2730168800907));
#19065=CARTESIAN_POINT('Ctrl Pts',(6.75393704542791,-0.455082403312534,
40.2812313430885));
#19066=CARTESIAN_POINT('Ctrl Pts',(6.76117745574585,-0.280657107364366,
40.2894458060863));
#19067=CARTESIAN_POINT('Ctrl Pts',(6.76842215577805,-0.10612846994128,40.2976651358938));
#19068=CARTESIAN_POINT('Ctrl Pts',(6.76889877690449,0.0685358051907464,
40.3058844657012));
#19069=CARTESIAN_POINT('Ctrl Pts',(6.76264362239255,0.242776103670322,40.3141037955087));
#19070=CARTESIAN_POINT('Ctrl Pts',(6.75637877589794,0.41728637692849,40.3223358606694));
#19071=CARTESIAN_POINT('Ctrl Pts',(6.74336133630555,0.591371003614929,40.3305679258301));
#19072=CARTESIAN_POINT('Ctrl Pts',(6.7236794379904,0.764476170423357,40.3387999909908));
#19073=CARTESIAN_POINT('Ctrl Pts',(6.7059879345467,0.920075523985483,40.346199562252));
#19074=CARTESIAN_POINT('Ctrl Pts',(6.68291247249063,1.07488344052355,40.3535991335132));
#19075=CARTESIAN_POINT('Ctrl Pts',(6.65455179220865,1.22850699827582,40.3609987047744));
#19076=CARTESIAN_POINT('Ctrl Pts',(6.62329196254614,1.39783460959325,40.3691546916866));
#19077=CARTESIAN_POINT('Ctrl Pts',(6.58551401471038,1.56624452008607,40.3773106785988));
#19078=CARTESIAN_POINT('Ctrl Pts',(6.5412795957629,1.73319077139706,40.385466665511));
#19079=CARTESIAN_POINT('Ctrl Pts',(6.49709959192488,1.89993165325244,40.3936126193103));
#19080=CARTESIAN_POINT('Ctrl Pts',(6.44647902008466,2.06521211056929,40.4017585731096));
#19081=CARTESIAN_POINT('Ctrl Pts',(6.38953102028647,2.22849328937669,40.4099045269089));
#19082=CARTESIAN_POINT('Ctrl Pts',(6.33264109914247,2.39160794519551,40.4180421730234));
#19083=CARTESIAN_POINT('Ctrl Pts',(6.26943671711267,2.55272703933819,40.4261798191378));
#19084=CARTESIAN_POINT('Ctrl Pts',(6.20008160138574,2.71132387149857,40.4343174652523));
#19085=CARTESIAN_POINT('Ctrl Pts',(6.13078264161349,2.86979228982207,40.4424485224182));
#19086=CARTESIAN_POINT('Ctrl Pts',(6.05534301075599,3.02574217942287,40.4505795795842));
#19087=CARTESIAN_POINT('Ctrl Pts',(5.97397561401119,3.17866392737573,40.4587106367501));
#19088=CARTESIAN_POINT('Ctrl Pts',(5.89265719347881,3.33149362951771,40.4668367997152));
#19089=CARTESIAN_POINT('Ctrl Pts',(5.80541828473356,3.4812984983562,40.4749629626803));
#19090=CARTESIAN_POINT('Ctrl Pts',(5.71251907108747,3.62759077935508,40.4830891256454));
#19091=CARTESIAN_POINT('Ctrl Pts',(5.61964970089293,3.77383606462138,40.4912126781175));
#19092=CARTESIAN_POINT('Ctrl Pts',(5.52112384099072,3.91657069984591,40.4993362305895));
#19093=CARTESIAN_POINT('Ctrl Pts',(5.4172466508149,4.0553332445355,40.5074597830616));
#19094=CARTESIAN_POINT('Ctrl Pts',(5.31338306991627,4.19407760950795,40.5155822712415));
#19095=CARTESIAN_POINT('Ctrl Pts',(5.20416977378661,4.32885062745309,40.5237047594214));
#19096=CARTESIAN_POINT('Ctrl Pts',(5.08995408415236,4.45922150394222,40.5318272476013));
#19097=CARTESIAN_POINT('Ctrl Pts',(4.97573163057727,4.58960010109476,40.5399502168012));
#19098=CARTESIAN_POINT('Ctrl Pts',(4.85650643522585,4.7155757632107,40.5480731860011));
#19099=CARTESIAN_POINT('Ctrl Pts',(4.73266474162749,4.83675236531249,40.556196155201));
#19100=CARTESIAN_POINT('Ctrl Pts',(4.60873588189369,4.95801425772165,40.5643248417632));
#19101=CARTESIAN_POINT('Ctrl Pts',(4.48018429332503,5.0744700849674,40.5724535283254));
#19102=CARTESIAN_POINT('Ctrl Pts',(4.34743209048359,5.1857615852094,40.5805822148876));
#19103=CARTESIAN_POINT('Ctrl Pts',(4.214633173298,5.29709224796119,40.5887137618639));
#19104=CARTESIAN_POINT('Ctrl Pts',(4.07763098363975,5.40325473622688,40.5968453088401));
#19105=CARTESIAN_POINT('Ctrl Pts',(3.93687887216083,5.50393257098356,40.6049768558163));
#19106=CARTESIAN_POINT('Ctrl Pts',(3.79596064724308,5.60472922414495,40.613117999517));
#19107=CARTESIAN_POINT('Ctrl Pts',(3.65128396189943,5.70002808697505,40.6212591432177));
#19108=CARTESIAN_POINT('Ctrl Pts',(3.50333000523339,5.78955679430053,40.6294002869184));
#19109=CARTESIAN_POINT('Ctrl Pts',(3.37110942337792,5.86956504850397,40.636675704091));
#19110=CARTESIAN_POINT('Ctrl Pts',(3.23627203569165,5.94496563415476,40.6439511212635));
#19111=CARTESIAN_POINT('Ctrl Pts',(3.09917575053255,6.01559628526641,40.6512265384361));
#19112=CARTESIAN_POINT('Origin',(0.,0.,-3.69717978381041));
#19113=CARTESIAN_POINT('',(3.09917575053267,6.01559628526634,43.0458827467338));
#19114=CARTESIAN_POINT('',(3.09917575053259,6.01559628526639,42.6516693621546));
#19115=CARTESIAN_POINT('',(3.09917575053259,6.01559628526639,-3.69717978381041));
#19116=CARTESIAN_POINT('',(-6.76699999999432,8.76508570167211E-6,41.6973687769752));
#19117=CARTESIAN_POINT('Ctrl Pts',(-6.76699999999432,8.76508570167208E-6,
41.6973687769752));
#19118=CARTESIAN_POINT('Ctrl Pts',(-6.76700022316934,-0.172291357653503,
41.7055020235368));
#19119=CARTESIAN_POINT('Ctrl Pts',(-6.76041552196173,-0.344817324618494,
41.7136352700984));
#19120=CARTESIAN_POINT('Ctrl Pts',(-6.74722008764693,-0.517020395007585,
41.72176851666));
#19121=CARTESIAN_POINT('Ctrl Pts',(-6.73403694439764,-0.68906306452083,
41.7298941873992));
#19122=CARTESIAN_POINT('Ctrl Pts',(-6.71425535454535,-0.860783072876566,
41.7380198581384));
#19123=CARTESIAN_POINT('Ctrl Pts',(-6.68790153363355,-1.03163078493329,
41.7461455288777));
#19124=CARTESIAN_POINT('Ctrl Pts',(-6.66156668084154,-1.2023555296268,41.7542653511786));
#19125=CARTESIAN_POINT('Ctrl Pts',(-6.62866907138239,-1.37220886699804,
41.7623851734795));
#19126=CARTESIAN_POINT('Ctrl Pts',(-6.58928681335984,-1.54064541387114,
41.7705049957804));
#19127=CARTESIAN_POINT('Ctrl Pts',(-6.54992456624683,-1.70899637478059,
41.7786206922379));
#19128=CARTESIAN_POINT('Ctrl Pts',(-6.50408431591424,-1.87593162239383,
41.7867363886954));
#19129=CARTESIAN_POINT('Ctrl Pts',(-6.45189541292007,-2.04091513315496,
41.7948520851529));
#19130=CARTESIAN_POINT('Ctrl Pts',(-6.39971417545145,-2.20587441107646,
41.8029665895739));
#19131=CARTESIAN_POINT('Ctrl Pts',(-6.34118624531644,-2.36888217105438,
41.8110810939949));
#19132=CARTESIAN_POINT('Ctrl Pts',(-6.27649113796564,-2.52941653253053,
41.8191955984159));
#19133=CARTESIAN_POINT('Ctrl Pts',(-6.21179847389791,-2.68994483124702,
41.8273097963835));
#19134=CARTESIAN_POINT('Ctrl Pts',(-6.14093923265554,-2.84799957658851,
41.8354239943512));
#19135=CARTESIAN_POINT('Ctrl Pts',(-6.06414141080024,-3.00307807920768,
41.8435381923188));
#19136=CARTESIAN_POINT('Ctrl Pts',(-5.98733176980108,-3.15818044832578,
41.8516536390572));
#19137=CARTESIAN_POINT('Ctrl Pts',(-5.90458189114834,-3.31030533361942,
41.8597690857956));
#19138=CARTESIAN_POINT('Ctrl Pts',(-5.81616610487774,-3.45897395776137,
41.867884532534));
#19139=CARTESIAN_POINT('Ctrl Pts',(-5.72771976377007,-3.60769395899081,
41.8760027838185));
#19140=CARTESIAN_POINT('Ctrl Pts',(-5.63360380397292,-3.75295500559633,
41.884121035103));
#19141=CARTESIAN_POINT('Ctrl Pts',(-5.53413627041377,-3.89430670857995,
41.8922392863876));
#19142=CARTESIAN_POINT('Ctrl Pts',(-5.43455819379238,-4.03581550252121,
41.9003665598759));
#19143=CARTESIAN_POINT('Ctrl Pts',(-5.32961687635012,-4.17340597521397,
41.9084938333642));
#19144=CARTESIAN_POINT('Ctrl Pts',(-5.21967164507103,-4.30665960085557,
41.9166211068525));
#19145=CARTESIAN_POINT('Ctrl Pts',(-5.10966031301768,-4.4399933406388,41.9247532665834));
#19146=CARTESIAN_POINT('Ctrl Pts',(-4.99463931697718,-4.56898476535065,
41.9328854263143));
#19147=CARTESIAN_POINT('Ctrl Pts',(-4.87500509432254,-4.69325199944871,
41.9410175860452));
#19148=CARTESIAN_POINT('Ctrl Pts',(-4.7551935351311,-4.8177034377021,41.9491618002619));
#19149=CARTESIAN_POINT('Ctrl Pts',(-4.63075535388932,-4.93741644373681,
41.9573060144786));
#19150=CARTESIAN_POINT('Ctrl Pts',(-4.5021211123992,-5.05204854383738,41.9654502286954));
#19151=CARTESIAN_POINT('Ctrl Pts',(-4.41221603767525,-5.13216723856375,
41.971142384837));
#19152=CARTESIAN_POINT('Ctrl Pts',(-4.32026191353386,-5.2098048226097,41.9768345409787));
#19153=CARTESIAN_POINT('Ctrl Pts',(-4.22641390799836,-5.28485709156625,
41.9825266971203));
#19154=CARTESIAN_POINT('Ctrl Pts',(-4.09197864337153,-5.39236786476217,
41.990680589287));
#19155=CARTESIAN_POINT('Ctrl Pts',(-3.95321822543893,-5.49492178816961,
41.9988344814538));
#19156=CARTESIAN_POINT('Ctrl Pts',(-3.81053623764059,-5.59214650931357,
42.0069883736205));
#19157=CARTESIAN_POINT('Ctrl Pts',(-3.66802836173056,-5.68925258913461,
42.0151323157607));
#19158=CARTESIAN_POINT('Ctrl Pts',(-3.52160874027091,-5.78104220769026,
42.0232762579009));
#19159=CARTESIAN_POINT('Ctrl Pts',(-3.37171526295274,-5.8671820481021,42.0314202000411));
#19160=CARTESIAN_POINT('Ctrl Pts',(-3.2219731479675,-5.95323490456083,42.039555918434));
#19161=CARTESIAN_POINT('Ctrl Pts',(-3.06876447530341,-6.03364915987303,
42.0476916368269));
#19162=CARTESIAN_POINT('Ctrl Pts',(-2.9125574550802,-6.10813376334022,42.0558273552198));
#19163=CARTESIAN_POINT('Ctrl Pts',(-2.75647531441785,-6.18255882015863,
42.06395656952));
#19164=CARTESIAN_POINT('Ctrl Pts',(-2.59739992743273,-6.25106350723082,
42.0720857838202));
#19165=CARTESIAN_POINT('Ctrl Pts',(-2.43582553294712,-6.31340185423381,
42.0802149981204));
#19166=CARTESIAN_POINT('Ctrl Pts',(-2.27434633594233,-6.37570347231318,
42.0883394227958));
#19167=CARTESIAN_POINT('Ctrl Pts',(-2.11037140391,-6.43184585425817,42.0964638474712));
#19168=CARTESIAN_POINT('Ctrl Pts',(-1.94441645063388,-6.48163047901563,
42.1045882721466));
#19169=CARTESIAN_POINT('Ctrl Pts',(-1.77745404455236,-6.53171732831587,
42.1127620172808));
#19170=CARTESIAN_POINT('Ctrl Pts',(-1.60848783736744,-6.57536881497801,
42.120935762415));
#19171=CARTESIAN_POINT('Ctrl Pts',(-1.43806066745962,-6.61243302549868,
42.1291095075492));
#19172=CARTESIAN_POINT('Ctrl Pts',(-1.26872486327763,-6.64925988766087,
42.1372309104114));
#19173=CARTESIAN_POINT('Ctrl Pts',(-1.09794711950863,-6.67958353688564,
42.1453523132735));
#19174=CARTESIAN_POINT('Ctrl Pts',(-0.926271973831232,-6.70330584342493,
42.1534737161357));
#19175=CARTESIAN_POINT('Ctrl Pts',(-0.754583555135203,-6.7270299840481,
42.161595746902));
#19176=CARTESIAN_POINT('Ctrl Pts',(-0.581997958867696,-6.74415171520996,
42.1697177776682));
#19177=CARTESIAN_POINT('Ctrl Pts',(-0.40906646848288,-6.75462461017361,
42.1778398084345));
#19178=CARTESIAN_POINT('Ctrl Pts',(-0.236088677797123,-6.76510030912736,
42.1859640137756));
#19179=CARTESIAN_POINT('Ctrl Pts',(-0.0627651737578177,-6.76892360518161,
42.1940882191167));
#19180=CARTESIAN_POINT('Ctrl Pts',(0.110351168858707,-6.76610017805911,
42.2022124244578));
#19181=CARTESIAN_POINT('Ctrl Pts',(0.285341376097719,-6.76324618929166,
42.2104245687003));
#19182=CARTESIAN_POINT('Ctrl Pts',(0.460119527330116,-6.7536007497577,42.2186367129428));
#19183=CARTESIAN_POINT('Ctrl Pts',(0.634119112966488,-6.73722360847334,
42.2268488571852));
#19184=CARTESIAN_POINT('Ctrl Pts',(0.806530274157802,-6.72099597243902,
42.2349860336017));
#19185=CARTESIAN_POINT('Ctrl Pts',(0.978176671386174,-6.69815913995813,
42.2431232100181));
#19186=CARTESIAN_POINT('Ctrl Pts',(1.14851704837981,-6.66882280388233,42.2512603864346));
#19187=CARTESIAN_POINT('Ctrl Pts',(1.32121144483127,-6.6390810542037,42.25951001459));
#19188=CARTESIAN_POINT('Ctrl Pts',(1.49256307573794,-6.60265892719256,42.2677596427455));
#19189=CARTESIAN_POINT('Ctrl Pts',(1.66202383692403,-6.55972299457045,42.276009270901));
#19190=CARTESIAN_POINT('Ctrl Pts',(1.83148459811012,-6.51678706194835,42.2842588990564));
#19191=CARTESIAN_POINT('Ctrl Pts',(1.99905413843699,-6.46733749329357,42.2925085272119));
#19192=CARTESIAN_POINT('Ctrl Pts',(2.16420575846851,-6.41159125607768,42.3007581553673));
#19193=CARTESIAN_POINT('Ctrl Pts',(2.32886169154851,-6.35601233591493,42.308983023045));
#19194=CARTESIAN_POINT('Ctrl Pts',(2.49160642798038,-6.2940085238898,42.3172078907226));
#19195=CARTESIAN_POINT('Ctrl Pts',(2.65190242788229,-6.22572907481461,42.3254327584002));
#19196=CARTESIAN_POINT('Ctrl Pts',(2.81201783639852,-6.15752655018127,42.3336483598437));
#19197=CARTESIAN_POINT('Ctrl Pts',(2.96968967474599,-6.08306260639842,42.3418639612873));
#19198=CARTESIAN_POINT('Ctrl Pts',(3.12439564138987,-6.00253620364459,42.3500795627308));
#19199=CARTESIAN_POINT('Ctrl Pts',(3.2789583979792,-5.92208434352658,42.358287559059));
#19200=CARTESIAN_POINT('Ctrl Pts',(3.4305604343155,-5.83558136539181,42.3664955553871));
#19201=CARTESIAN_POINT('Ctrl Pts',(3.57869944091381,-5.74327426748916,42.3747035517153));
#19202=CARTESIAN_POINT('Ctrl Pts',(3.72673107092835,-5.65103407715568,42.3829055985867));
#19203=CARTESIAN_POINT('Ctrl Pts',(3.87130436765057,-5.55299833564588,42.3911076454582));
#19204=CARTESIAN_POINT('Ctrl Pts',(4.0119415802419,-5.44945995092414,42.3993096923296));
#19205=CARTESIAN_POINT('Ctrl Pts',(4.15250509503649,-5.34597582318526,42.4075074411012));
#19206=CARTESIAN_POINT('Ctrl Pts',(4.28913634652938,-5.23699500890228,42.4157051898728));
#19207=CARTESIAN_POINT('Ctrl Pts',(4.42138647724192,-5.12285375731753,42.4239029386444));
#19208=CARTESIAN_POINT('Ctrl Pts',(4.5536113838977,-5.00873427588448,42.43209912386));
#19209=CARTESIAN_POINT('Ctrl Pts',(4.68145655881384,-4.88945654711756,42.4402953090756));
#19210=CARTESIAN_POINT('Ctrl Pts',(4.80450593516675,-4.76539733064804,42.4484914942913));
#19211=CARTESIAN_POINT('Ctrl Pts',(4.92754620860461,-4.64134729179927,42.4566870731716));
#19212=CARTESIAN_POINT('Ctrl Pts',(5.04579113671474,-4.51251672382981,42.464882652052));
#19213=CARTESIAN_POINT('Ctrl Pts',(5.15886131848055,-4.37931945588411,42.4730782309323));
#19214=CARTESIAN_POINT('Ctrl Pts',(5.27194370735004,-4.24610780790617,42.4812746946108));
#19215=CARTESIAN_POINT('Ctrl Pts',(5.37985000457132,-4.10852879433005,42.4894711582892));
#19216=CARTESIAN_POINT('Ctrl Pts',(5.48224090557458,-3.96702957554451,42.4976676219677));
#19217=CARTESIAN_POINT('Ctrl Pts',(5.58466148963133,-3.82548933623039,42.5058664617954));
#19218=CARTESIAN_POINT('Ctrl Pts',(5.6815632823423,-3.68002691864602,42.5140653016232));
#19219=CARTESIAN_POINT('Ctrl Pts',(5.77265011563406,-3.53111875224695,42.5222641414509));
#19220=CARTESIAN_POINT('Ctrl Pts',(5.86383209171485,-3.38205504703128,42.5304715452002));
#19221=CARTESIAN_POINT('Ctrl Pts',(5.94918678604182,-3.2295387088168,42.5386789489494));
#19222=CARTESIAN_POINT('Ctrl Pts',(6.02846336904168,-3.07407195883939,42.5468863526987));
#19223=CARTESIAN_POINT('Ctrl Pts',(6.10778241677463,-2.91852193264355,42.5550981527677));
#19224=CARTESIAN_POINT('Ctrl Pts',(6.18101671238073,-2.76001866955657,42.5633099528367));
#19225=CARTESIAN_POINT('Ctrl Pts',(6.24796353223583,-2.59908458882184,42.5715217529057));
#19226=CARTESIAN_POINT('Ctrl Pts',(6.31500890716424,-2.43791359063295,42.5797456418919));
#19227=CARTESIAN_POINT('Ctrl Pts',(6.37574818351,-2.27430495965851,42.587969530878));
#19228=CARTESIAN_POINT('Ctrl Pts',(6.43002808066008,-2.10879773376274,42.5961934198642));
#19229=CARTESIAN_POINT('Ctrl Pts',(6.48018176724473,-1.95587191829703,42.6037921511141));
#19230=CARTESIAN_POINT('Ctrl Pts',(6.52482129653724,-1.80132555495087,42.6113908823641));
#19231=CARTESIAN_POINT('Ctrl Pts',(6.56386471263037,-1.6455907857927,42.618989613614));
#19232=CARTESIAN_POINT('Ctrl Pts',(6.60612521175542,-1.47702384841073,42.6272144619361));
#19233=CARTESIAN_POINT('Ctrl Pts',(6.64194738592476,-1.30659134167416,42.6354393102581));
#19234=CARTESIAN_POINT('Ctrl Pts',(6.67116620613291,-1.13482617618305,42.6436641585801));
#19235=CARTESIAN_POINT('Ctrl Pts',(6.70035211947112,-0.963254456352035,
42.6518797438994));
#19236=CARTESIAN_POINT('Ctrl Pts',(6.72294942787765,-0.790353416846953,
42.6600953292186));
#19237=CARTESIAN_POINT('Ctrl Pts',(6.73884315648882,-0.616670018927359,
42.6683109145378));
#19238=CARTESIAN_POINT('Ctrl Pts',(6.75472217860409,-0.443147330570621,
42.676518897961));
#19239=CARTESIAN_POINT('Ctrl Pts',(6.76390994150824,-0.268844080524225,
42.6847268813842));
#19240=CARTESIAN_POINT('Ctrl Pts',(6.76634269161954,-0.0943163801617513,
42.6929348648074));
#19241=CARTESIAN_POINT('Ctrl Pts',(6.768773679333,0.0800848841803265,42.701136901984));
#19242=CARTESIAN_POINT('Ctrl Pts',(6.76445939649494,0.254709917682513,42.7093389391605));
#19243=CARTESIAN_POINT('Ctrl Pts',(6.75338798891608,0.428998451237325,42.7175409763371));
#19244=CARTESIAN_POINT('Ctrl Pts',(6.74232237874528,0.603195720719244,42.7257387186165));
#19245=CARTESIAN_POINT('Ctrl Pts',(6.72450671535754,0.777056484078363,42.733936460896));
#19246=CARTESIAN_POINT('Ctrl Pts',(6.69998122647779,0.950021349678609,42.7421342031754));
#19247=CARTESIAN_POINT('Ctrl Pts',(6.67546040071404,1.12295332887091,42.7503303867897));
#19248=CARTESIAN_POINT('Ctrl Pts',(6.64423233476188,1.29498939386639,42.7585265704041));
#19249=CARTESIAN_POINT('Ctrl Pts',(6.60638906358163,1.46557583924855,42.7667227540185));
#19250=CARTESIAN_POINT('Ctrl Pts',(6.56854857819412,1.6361497270883,42.7749183342793));
#19251=CARTESIAN_POINT('Ctrl Pts',(6.52409393423409,1.8052738573329,42.7831139145402));
#19252=CARTESIAN_POINT('Ctrl Pts',(6.47316817398407,1.9724053313961,42.7913094948011));
#19253=CARTESIAN_POINT('Ctrl Pts',(6.42223689724095,2.13955490984538,42.7995059628418));
#19254=CARTESIAN_POINT('Ctrl Pts',(6.36483321225574,2.30471105874899,42.8077024308825));
#19255=CARTESIAN_POINT('Ctrl Pts',(6.30114987824893,2.46734659337587,42.8158988989232));
#19256=CARTESIAN_POINT('Ctrl Pts',(6.23744805931675,2.63002933510593,42.8240977460966));
#19257=CARTESIAN_POINT('Ctrl Pts',(6.16746309147786,2.79018967117871,42.8322965932699));
#19258=CARTESIAN_POINT('Ctrl Pts',(6.091435676857,2.94732088424619,42.8404954404433));
#19259=CARTESIAN_POINT('Ctrl Pts',(6.01532880619455,3.1046163147116,42.8487028562093));
#19260=CARTESIAN_POINT('Ctrl Pts',(5.93316702881184,3.2588759740207,42.8569102719752));
#19261=CARTESIAN_POINT('Ctrl Pts',(5.8452372548959,3.40961734421579,42.8651176877412));
#19262=CARTESIAN_POINT('Ctrl Pts',(5.75726035371393,3.56043950648321,42.8733295023933));
#19263=CARTESIAN_POINT('Ctrl Pts',(5.66350948561644,3.70773931805832,42.8815413170454));
#19264=CARTESIAN_POINT('Ctrl Pts',(5.564314558757,3.85106381292298,42.8897531316975));
#19265=CARTESIAN_POINT('Ctrl Pts',(5.4649735522876,3.99459937489533,42.8979770394952));
#19266=CARTESIAN_POINT('Ctrl Pts',(5.36017268038438,4.13414763365764,42.9062009472928));
#19267=CARTESIAN_POINT('Ctrl Pts',(5.25028256087597,4.26928823470163,42.9144248550904));
#19268=CARTESIAN_POINT('Ctrl Pts',(5.14874611993157,4.39415565425196,42.9220235940139));
#19269=CARTESIAN_POINT('Ctrl Pts',(5.04286535323869,4.51526029391803,42.9296223329375));
#19270=CARTESIAN_POINT('Ctrl Pts',(4.93295950574095,4.63229959250479,42.9372210718611));
#19271=CARTESIAN_POINT('Ctrl Pts',(4.81503765735996,4.75787517139151,42.9453740260453));
#19272=CARTESIAN_POINT('Ctrl Pts',(4.69213232769796,4.87914231663287,42.9535269802296));
#19273=CARTESIAN_POINT('Ctrl Pts',(4.56459273787198,4.99567634433681,42.9616799344139));
#19274=CARTESIAN_POINT('Ctrl Pts',(4.43724053715183,5.11203915299198,42.9698209097702));
#19275=CARTESIAN_POINT('Ctrl Pts',(4.30526790901352,5.2236824543534,42.9779618851266));
#19276=CARTESIAN_POINT('Ctrl Pts',(4.16906305282286,5.3302159676309,42.986102860483));
#19277=CARTESIAN_POINT('Ctrl Pts',(4.03297357626649,5.43665923597774,42.9942369395892));
#19278=CARTESIAN_POINT('Ctrl Pts',(3.89265929133585,5.5380011053793,43.0023710186954));
#19279=CARTESIAN_POINT('Ctrl Pts',(3.74854431605663,5.6338889331047,43.0105050978017));
#19280=CARTESIAN_POINT('Ctrl Pts',(3.60454489032177,5.72969987919595,43.0186326551073));
#19281=CARTESIAN_POINT('Ctrl Pts',(3.45675114718345,5.82006529201822,43.0267602124129));
#19282=CARTESIAN_POINT('Ctrl Pts',(3.30561904837234,5.90467371723772,43.0348877697185));
#19283=CARTESIAN_POINT('Ctrl Pts',(3.23746843885906,5.94282653714844,43.038552762057));
#19284=CARTESIAN_POINT('Ctrl Pts',(3.16863942116908,5.97980928870432,43.0422177543954));
#19285=CARTESIAN_POINT('Ctrl Pts',(3.09917575053267,6.01559628526635,43.0458827467338));
#19286=CARTESIAN_POINT('Ctrl Pts',(3.09917575053253,6.01559628526642,41.0457515827422));
#19287=CARTESIAN_POINT('Ctrl Pts',(2.93382384459258,6.10078395293763,41.0545010306546));
#19288=CARTESIAN_POINT('Ctrl Pts',(2.76495772122977,6.17915010267052,41.063250478567));
#19289=CARTESIAN_POINT('Ctrl Pts',(2.59315093316703,6.25042856433181,41.0719999264794));
#19290=CARTESIAN_POINT('Ctrl Pts',(2.42134553245601,6.32170645041457,41.0807493037394));
#19291=CARTESIAN_POINT('Ctrl Pts',(2.24659977927567,6.38589665313466,41.0894986809994));
#19292=CARTESIAN_POINT('Ctrl Pts',(2.06950718689887,6.44278115439085,41.0982480582594));
#19293=CARTESIAN_POINT('Ctrl Pts',(1.89241596572834,6.49966521519732,41.1069973677741));
#19294=CARTESIAN_POINT('Ctrl Pts',(1.71297821457174,6.54924360009552,41.1157466772887));
#19295=CARTESIAN_POINT('Ctrl Pts',(1.53180337335825,6.59134792173561,41.1244959868034));
#19296=CARTESIAN_POINT('Ctrl Pts',(1.35062987477768,6.63345193135307,41.1332452314795));
#19297=CARTESIAN_POINT('Ctrl Pts',(1.16771959102943,6.66808192368239,41.1419944761556));
#19298=CARTESIAN_POINT('Ctrl Pts',(0.983693746906803,6.69512028363169,41.1507437208318));
#19299=CARTESIAN_POINT('Ctrl Pts',(0.799669205419937,6.72215845218866,41.1594929035759));
#19300=CARTESIAN_POINT('Ctrl Pts',(0.61452940287365,6.74160505424577,41.1682420863201));
#19301=CARTESIAN_POINT('Ctrl Pts',(0.428903127363531,6.7533940435412,41.1769912690643));
#19302=CARTESIAN_POINT('Ctrl Pts',(0.243278104164166,6.76518295330329,41.1857403927829));
#19303=CARTESIAN_POINT('Ctrl Pts',(0.0571669005394085,6.76931433552275,
41.1944895165015));
#19304=CARTESIAN_POINT('Ctrl Pts',(-0.128798404777218,6.76577415902474,
41.2032386402201));
#19305=CARTESIAN_POINT('Ctrl Pts',(-0.31476251725885,6.76223400523443,41.2119877078193));
#19306=CARTESIAN_POINT('Ctrl Pts',(-0.500580446819306,6.7510223966509,41.2207367754185));
#19307=CARTESIAN_POINT('Ctrl Pts',(-0.685621118842454,6.73217741012499,
41.2294858430177));
#19308=CARTESIAN_POINT('Ctrl Pts',(-0.870660665414367,6.71333253821773,
41.2382348574035));
#19309=CARTESIAN_POINT('Ctrl Pts',(-1.05492267885478,6.68685441030614,41.2469838717893));
#19310=CARTESIAN_POINT('Ctrl Pts',(-1.23778137635247,6.65283295028178,41.2557328861751));
#19311=CARTESIAN_POINT('Ctrl Pts',(-1.42999922978841,6.61707018861867,41.2649296965425));
#19312=CARTESIAN_POINT('Ctrl Pts',(-1.62066601233689,6.57297172934414,41.2741265069099));
#19313=CARTESIAN_POINT('Ctrl Pts',(-1.80906628500378,6.52070304311296,41.2833233172772));
#19314=CARTESIAN_POINT('Ctrl Pts',(-1.98831342545516,6.47097374915034,41.292073315015));
#19315=CARTESIAN_POINT('Ctrl Pts',(-2.16550875896686,6.41384933989534,41.3008233127528));
#19316=CARTESIAN_POINT('Ctrl Pts',(-2.34005036713991,6.34952386240483,41.3095733104905));
#19317=CARTESIAN_POINT('Ctrl Pts',(-2.51458843547069,6.28519968948604,41.3183231307714));
#19318=CARTESIAN_POINT('Ctrl Pts',(-2.68647261718036,6.21367483971107,41.3270729510523));
#19319=CARTESIAN_POINT('Ctrl Pts',(-2.85511905908713,6.13519226743852,41.3358227713331));
#19320=CARTESIAN_POINT('Ctrl Pts',(-3.02376230488867,6.05671118252946,41.3445724257917));
#19321=CARTESIAN_POINT('Ctrl Pts',(-3.18916767379888,5.97127275992642,41.3533220802502));
#19322=CARTESIAN_POINT('Ctrl Pts',(-3.35077334102772,5.87916720438005,41.3620717347087));
#19323=CARTESIAN_POINT('Ctrl Pts',(-3.51237616037362,5.78706327195647,41.3708212349772));
#19324=CARTESIAN_POINT('Ctrl Pts',(-3.67017916302304,5.68829258362296,41.3795707352456));
#19325=CARTESIAN_POINT('Ctrl Pts',(-3.82364636566475,5.58319061741033,41.3883202355141));
#19326=CARTESIAN_POINT('Ctrl Pts',(-3.97711106778817,5.47809036367688,41.3970695932225));
#19327=CARTESIAN_POINT('Ctrl Pts',(-4.12623987481952,5.36665920043206,41.4058189509309));
#19328=CARTESIAN_POINT('Ctrl Pts',(-4.27052628213961,5.24927559512309,41.4145683086394));
#19329=CARTESIAN_POINT('Ctrl Pts',(-4.41481053025001,5.13189374643016,41.4233175354159));
#19330=CARTESIAN_POINT('Ctrl Pts',(-4.55425230136545,5.00855981477339,41.4320667621924));
#19331=CARTESIAN_POINT('Ctrl Pts',(-4.68837800630555,4.87969268192069,41.4408159889689));
#19332=CARTESIAN_POINT('Ctrl Pts',(-4.8225018822889,4.75082730631813,41.4495650964398));
#19333=CARTESIAN_POINT('Ctrl Pts',(-4.95130963052951,4.61642907903541,41.4583142039106));
#19334=CARTESIAN_POINT('Ctrl Pts',(-5.07436379033342,4.47695444731718,41.4670633113814));
#19335=CARTESIAN_POINT('Ctrl Pts',(-5.19741643562785,4.33748153220611,41.4758123111712));
#19336=CARTESIAN_POINT('Ctrl Pts',(-5.31471544462757,4.1929325525461,41.4845613109609));
#19337=CARTESIAN_POINT('Ctrl Pts',(-5.42586245275615,4.0437984177962,41.4933103107507));
#19338=CARTESIAN_POINT('Ctrl Pts',(-5.53702160019143,3.89464799484357,41.5020602660928));
#19339=CARTESIAN_POINT('Ctrl Pts',(-5.64202723081243,3.74091164443862,41.510810221435));
#19340=CARTESIAN_POINT('Ctrl Pts',(-5.74052265232961,3.58311159163242,41.5195601767772));
#19341=CARTESIAN_POINT('Ctrl Pts',(-5.83901427066912,3.42531763191793,41.5283097942596));
#19342=CARTESIAN_POINT('Ctrl Pts',(-5.93099603115734,3.26346052695622,41.537059411742));
#19343=CARTESIAN_POINT('Ctrl Pts',(-6.01615550622749,3.09809004467086,41.5458090292245));
#19344=CARTESIAN_POINT('Ctrl Pts',(-6.101312145788,2.93272506863827,41.5545583553756));
#19345=CARTESIAN_POINT('Ctrl Pts',(-6.17964682328753,2.76384720416884,41.5633076815267));
#19346=CARTESIAN_POINT('Ctrl Pts',(-6.25089348288573,2.59203002791572,41.5720570076778));
#19347=CARTESIAN_POINT('Ctrl Pts',(-6.32213814889341,2.42021765937,41.5808060890094));
#19348=CARTESIAN_POINT('Ctrl Pts',(-6.38629508412598,2.24546640831882,41.5895551703409));
#19349=CARTESIAN_POINT('Ctrl Pts',(-6.44314639819826,2.06836976659998,41.5983042516725));
#19350=CARTESIAN_POINT('Ctrl Pts',(-6.50000285283712,1.89125711158234,41.6070541241069));
#19351=CARTESIAN_POINT('Ctrl Pts',(-6.5495522767326,1.71179891440215,41.6158039965413));
#19352=CARTESIAN_POINT('Ctrl Pts',(-6.59162635926394,1.53060476278394,41.6245538689757));
#19353=CARTESIAN_POINT('Ctrl Pts',(-6.63369752055211,1.3494231916463,41.6333031338982));
#19354=CARTESIAN_POINT('Ctrl Pts',(-6.66829431424271,1.1665061864261,41.6420523988207));
#19355=CARTESIAN_POINT('Ctrl Pts',(-6.69529923745435,0.982474997617332,
41.6508016637432));
#19356=CARTESIAN_POINT('Ctrl Pts',(-6.72230554731459,0.79843435917646,41.6595513779229));
#19357=CARTESIAN_POINT('Ctrl Pts',(-6.74171916496715,0.613279706239005,
41.6683010921026));
#19358=CARTESIAN_POINT('Ctrl Pts',(-6.75347414817284,0.427639953653992,
41.6770508062823));
#19359=CARTESIAN_POINT('Ctrl Pts',(-6.76248837758748,0.285283364197565,
41.6837604654582));
#19360=CARTESIAN_POINT('Ctrl Pts',(-6.76699999999997,0.142641701104487,
41.6904701246341));
#19361=CARTESIAN_POINT('Ctrl Pts',(-6.767,1.31890318194932E-12,41.69717978381));
#19362=CARTESIAN_POINT('',(-6.76699997529837,-0.000578197107039292,41.3028202161655));
#19363=CARTESIAN_POINT('Ctrl Pts',(3.09917575053255,6.01559628526641,40.6512265384361));
#19364=CARTESIAN_POINT('Ctrl Pts',(2.94551530212736,6.09476062956918,40.6593809815982));
#19365=CARTESIAN_POINT('Ctrl Pts',(2.78901715297729,6.16793186163224,40.6675354247604));
#19366=CARTESIAN_POINT('Ctrl Pts',(2.63020092619897,6.23492839476302,40.6756898679225));
#19367=CARTESIAN_POINT('Ctrl Pts',(2.60999793920778,6.24345101310468,40.6767271933423));
#19368=CARTESIAN_POINT('Ctrl Pts',(2.58975745831133,6.25187377711503,40.6777645187622));
#19369=CARTESIAN_POINT('Ctrl Pts',(2.56948056803328,6.26019637156051,40.6788018441821));
#19370=CARTESIAN_POINT('Ctrl Pts',(2.40868055201595,6.3261963006319,40.6870280535191));
#19371=CARTESIAN_POINT('Ctrl Pts',(2.24511120123291,6.38608902214036,40.695254262856));
#19372=CARTESIAN_POINT('Ctrl Pts',(2.0792765258894,6.43963493754773,40.703480472193));
#19373=CARTESIAN_POINT('Ctrl Pts',(1.91362815869939,6.49312069641301,40.7116974397362));
#19374=CARTESIAN_POINT('Ctrl Pts',(1.74571987291272,6.54027373847451,40.7199144072794));
#19375=CARTESIAN_POINT('Ctrl Pts',(1.57607673768459,6.58090199873312,40.7281313748226));
#19376=CARTESIAN_POINT('Ctrl Pts',(1.40659014051535,6.62149276929909,40.736340760166));
#19377=CARTESIAN_POINT('Ctrl Pts',(1.23537222860056,6.65557066558009,40.7445501455093));
#19378=CARTESIAN_POINT('Ctrl Pts',(1.06296444828513,6.68299301074615,40.7527595308527));
#19379=CARTESIAN_POINT('Ctrl Pts',(0.890681164586124,6.71039555408435,40.7609629881533));
#19380=CARTESIAN_POINT('Ctrl Pts',(0.717210076635454,6.73115206294866,40.7691664454539));
#19381=CARTESIAN_POINT('Ctrl Pts',(0.543104165577543,6.74517063278108,40.7773699027545));
#19382=CARTESIAN_POINT('Ctrl Pts',(0.369089052147779,6.75918189181697,40.7855690818863));
#19383=CARTESIAN_POINT('Ctrl Pts',(0.194440131780878,6.76646218339899,40.7937682610182));
#19384=CARTESIAN_POINT('Ctrl Pts',(0.019716964911336,6.76697127534133,40.80196744015));
#19385=CARTESIAN_POINT('Ctrl Pts',(-0.154973280348247,6.76748027135979,
40.8101650743798));
#19386=CARTESIAN_POINT('Ctrl Pts',(-0.329737385997837,6.76122060181682,
40.8183627086096));
#19387=CARTESIAN_POINT('Ctrl Pts',(-0.504014009278662,6.7482041224648,40.8265603428394));
#19388=CARTESIAN_POINT('Ctrl Pts',(-0.678278053081919,6.73518858265651,
40.834757385355));
#19389=CARTESIAN_POINT('Ctrl Pts',(-0.852054326845273,6.71541723018181,
40.8429544278706));
#19390=CARTESIAN_POINT('Ctrl Pts',(-1.0247848860671,6.68895394940707,40.8511514703862));
#19391=CARTESIAN_POINT('Ctrl Pts',(-1.19753437089774,6.66248776912398,40.859349411029));
#19392=CARTESIAN_POINT('Ctrl Pts',(-1.36923755830116,6.62932825409143,40.8675473516718));
#19393=CARTESIAN_POINT('Ctrl Pts',(-1.53934494120944,6.58959074237338,40.8757452923147));
#19394=CARTESIAN_POINT('Ctrl Pts',(-1.70950187915898,6.54984165447327,40.8839456211506));
#19395=CARTESIAN_POINT('Ctrl Pts',(-1.87806173743238,6.50351083446698,40.8921459499866));
#19396=CARTESIAN_POINT('Ctrl Pts',(-2.04448840290889,6.45076399896718,40.9003462788226));
#19397=CARTESIAN_POINT('Ctrl Pts',(-2.2110884892894,6.39796219989608,40.908555152614));
#19398=CARTESIAN_POINT('Ctrl Pts',(-2.37555059960082,6.33873113691363,40.9167640264054));
#19399=CARTESIAN_POINT('Ctrl Pts',(-2.53735596045524,6.27328572041337,40.9249729001968));
#19400=CARTESIAN_POINT('Ctrl Pts',(-2.69924816046197,6.20780518008,40.9331861796003));
#19401=CARTESIAN_POINT('Ctrl Pts',(-2.85848044179878,6.13610378456785,40.9413994590037));
#19402=CARTESIAN_POINT('Ctrl Pts',(-3.01455711976554,6.05844323004441,40.9496127384071));
#19403=CARTESIAN_POINT('Ctrl Pts',(-3.17086208440454,5.98066908475399,40.9578380310226));
#19404=CARTESIAN_POINT('Ctrl Pts',(-3.32400190709226,5.89691853377205,40.966063323638));
#19405=CARTESIAN_POINT('Ctrl Pts',(-3.47350736005325,5.80749822381858,40.9742886162535));
#19406=CARTESIAN_POINT('Ctrl Pts',(-3.60871708299939,5.72662829502928,40.9817274053655));
#19407=CARTESIAN_POINT('Ctrl Pts',(-3.74095446105745,5.64112172591948,40.9891661944776));
#19408=CARTESIAN_POINT('Ctrl Pts',(-3.86989548350949,5.55123391208773,40.9966049835897));
#19409=CARTESIAN_POINT('Ctrl Pts',(-4.01161479509416,5.45243805291246,41.0047809701915));
#19410=CARTESIAN_POINT('Ctrl Pts',(-4.14975890089944,5.3480648934046,41.0129569567933));
#19411=CARTESIAN_POINT('Ctrl Pts',(-4.28385665501696,5.2384025388726,41.0211329433951));
#19412=CARTESIAN_POINT('Ctrl Pts',(-4.41780315719193,5.12886387503369,41.0292997081135));
#19413=CARTESIAN_POINT('Ctrl Pts',(-4.54771211508459,5.014048121242,41.0374664728319));
#19414=CARTESIAN_POINT('Ctrl Pts',(-4.67314066217522,4.89428701155997,41.0456332375503));
#19415=CARTESIAN_POINT('Ctrl Pts',(-4.79845377853718,4.77463611691651,41.0537924864708));
#19416=CARTESIAN_POINT('Ctrl Pts',(-4.9192944328203,4.65004917789119,41.0619517353913));
#19417=CARTESIAN_POINT('Ctrl Pts',(-5.03525220343385,4.52089861065415,41.0701109843119));
#19418=CARTESIAN_POINT('Ctrl Pts',(-5.15112732565981,4.39184009491207,41.0782644177639));
#19419=CARTESIAN_POINT('Ctrl Pts',(-5.26212625302865,4.25822469807299,41.0864178512159));
#19420=CARTESIAN_POINT('Ctrl Pts',(-5.3678748597193,4.1204621695137,41.0945712846679));
#19421=CARTESIAN_POINT('Ctrl Pts',(-5.47357003594037,3.98276924675653,41.1027205985216));
#19422=CARTESIAN_POINT('Ctrl Pts',(-5.57401995448648,3.84093365376934,41.1108699123753));
#19423=CARTESIAN_POINT('Ctrl Pts',(-5.66889028254878,3.69539875580755,41.119019226229));
#19424=CARTESIAN_POINT('Ctrl Pts',(-5.76374507207625,3.549887694583,41.1271672053304));
#19425=CARTESIAN_POINT('Ctrl Pts',(-5.85302188730736,3.4006788359124,41.1353151844317));
#19426=CARTESIAN_POINT('Ctrl Pts',(-5.93642918259666,3.24824530477838,41.143463163533));
#19427=CARTESIAN_POINT('Ctrl Pts',(-6.01983274651937,3.0958185930165,41.1516107781207));
#19428=CARTESIAN_POINT('Ctrl Pts',(-6.09736713816796,2.94016781481091,41.1597583927084));
#19429=CARTESIAN_POINT('Ctrl Pts',(-6.16878639378154,2.7817914062517,41.1679060072961));
#19430=CARTESIAN_POINT('Ctrl Pts',(-6.24021587719233,2.62339231694936,41.1760547886861));
#19431=CARTESIAN_POINT('Ctrl Pts',(-6.30552833107212,2.46226715157735,41.184203570076));
#19432=CARTESIAN_POINT('Ctrl Pts',(-6.36452564273323,2.29893504540496,41.192352351466));
#19433=CARTESIAN_POINT('Ctrl Pts',(-6.42354249184777,2.13554885043892,41.2005038313931));
#19434=CARTESIAN_POINT('Ctrl Pts',(-6.47623991082771,1.96995460122454,41.2086553113202));
#19435=CARTESIAN_POINT('Ctrl Pts',(-6.52246942850797,1.80268731458867,41.2168067912473));
#19436=CARTESIAN_POINT('Ctrl Pts',(-6.56874694125375,1.63524637257448,41.2249667339668));
#19437=CARTESIAN_POINT('Ctrl Pts',(-6.60854304531649,1.46612927504205,41.2331266766864));
#19438=CARTESIAN_POINT('Ctrl Pts',(-6.64176006570574,1.2958827993289,41.2412866194059));
#19439=CARTESIAN_POINT('Ctrl Pts',(-6.67499648835186,1.12553688164852,41.249451328396));
#19440=CARTESIAN_POINT('Ctrl Pts',(-6.70164611365765,0.954060629730198,
41.2576160373861));
#19441=CARTESIAN_POINT('Ctrl Pts',(-6.72166310516942,0.782006458160169,
41.2657807463761));
#19442=CARTESIAN_POINT('Ctrl Pts',(-6.74170705281312,0.609720587688462,
41.2739564504737));
#19443=CARTESIAN_POINT('Ctrl Pts',(-6.75510049993274,0.436855604788317,
41.2821321545712));
#19444=CARTESIAN_POINT('Ctrl Pts',(-6.76184969379621,0.263965373691635,
41.2903078586687));
#19445=CARTESIAN_POINT('Ctrl Pts',(-6.76529275408913,0.175766471457374,
41.294478644501));
#19446=CARTESIAN_POINT('Ctrl Pts',(-6.76700750622803,0.0875609516987905,
41.2986494303332));
#19447=CARTESIAN_POINT('Ctrl Pts',(-6.76699997529837,-0.000578197106943801,
41.3028202161655));
#19448=CARTESIAN_POINT('Ctrl Pts',(-6.76699997529832,-0.000578197623143367,
41.3028202161899));
#19449=CARTESIAN_POINT('Ctrl Pts',(-6.76699300077022,-0.0822053604272126,
41.3066828517924));
#19450=CARTESIAN_POINT('Ctrl Pts',(-6.76550913867493,-0.163818062147753,
41.3105454873949));
#19451=CARTESIAN_POINT('Ctrl Pts',(-6.7625496072816,-0.245380946806069,
41.3144081229974));
#19452=CARTESIAN_POINT('Ctrl Pts',(-6.75630316093462,-0.417529207869196,
41.3225606792107));
#19453=CARTESIAN_POINT('Ctrl Pts',(-6.74346931326276,-0.589708059610257,
41.3307132354239));
#19454=CARTESIAN_POINT('Ctrl Pts',(-6.72403209526724,-0.761368098764339,
41.3388657916372));
#19455=CARTESIAN_POINT('Ctrl Pts',(-6.70461739575737,-0.932829265624681,
41.3470089029176));
#19456=CARTESIAN_POINT('Ctrl Pts',(-6.67861459501554,-1.1037724568311,41.3551520141979));
#19457=CARTESIAN_POINT('Ctrl Pts',(-6.64605970415537,-1.27364807101581,
41.3632951254782));
#19458=CARTESIAN_POINT('Ctrl Pts',(-6.61353568466071,-1.44336259443845,
41.3714305147556));
#19459=CARTESIAN_POINT('Ctrl Pts',(-6.5744720131826,-1.61201119977722,41.3795659040329));
#19460=CARTESIAN_POINT('Ctrl Pts',(-6.52895649381364,-1.77904921289118,
41.3877012933103));
#19461=CARTESIAN_POINT('Ctrl Pts',(-6.48347457229122,-1.94596392481888,
41.3958306773489));
#19462=CARTESIAN_POINT('Ctrl Pts',(-6.43155038157621,-2.11127006057263,
41.4039600613875));
#19463=CARTESIAN_POINT('Ctrl Pts',(-6.37332281721652,-2.27443295516646,
41.4120894454261));
#19464=CARTESIAN_POINT('Ctrl Pts',(-6.31512600368384,-2.43750968105306,
41.4202145362182));
#19465=CARTESIAN_POINT('Ctrl Pts',(-6.25063256875132,-2.59844507643375,
41.4283396270104));
#19466=CARTESIAN_POINT('Ctrl Pts',(-6.18003129058261,-2.75671947202101,
41.4364647178026));
#19467=CARTESIAN_POINT('Ctrl Pts',(-6.10916051203007,-2.91559803528723,
41.4446208238277));
#19468=CARTESIAN_POINT('Ctrl Pts',(-6.03213527368781,-3.07179488638972,
41.4527769298528));
#19469=CARTESIAN_POINT('Ctrl Pts',(-5.94919558390946,-3.2248040102295,41.4609330358779));
#19470=CARTESIAN_POINT('Ctrl Pts',(-5.86658971138256,-3.37719730001799,
41.4690563150513));
#19471=CARTESIAN_POINT('Ctrl Pts',(-5.7781171026914,-3.52642816140395,41.4771795942247));
#19472=CARTESIAN_POINT('Ctrl Pts',(-5.68406107456446,-3.67202106483896,
41.4853028733981));
#19473=CARTESIAN_POINT('Ctrl Pts',(-5.5899925220826,-3.81763335519935,41.4934272342548));
#19474=CARTESIAN_POINT('Ctrl Pts',(-5.49033926782225,-3.95960641541173,
41.5015515951115));
#19475=CARTESIAN_POINT('Ctrl Pts',(-5.38542804251937,-4.09749359961013,
41.5096759559682));
#19476=CARTESIAN_POINT('Ctrl Pts',(-5.28048288749987,-4.23542537839859,
41.5178029443536));
#19477=CARTESIAN_POINT('Ctrl Pts',(-5.17027659660184,-4.36926835880579,
41.525929932739));
#19478=CARTESIAN_POINT('Ctrl Pts',(-5.05517623096443,-4.4986089265341,41.5340569211244));
#19479=CARTESIAN_POINT('Ctrl Pts',(-4.93933175456783,-4.62878566630681,
41.5422364495645));
#19480=CARTESIAN_POINT('Ctrl Pts',(-4.81852995461568,-4.75440129564737,
41.5504159780046));
#19481=CARTESIAN_POINT('Ctrl Pts',(-4.69318208614446,-4.87507240010779,
41.5585955064446));
#19482=CARTESIAN_POINT('Ctrl Pts',(-4.56842452119599,-4.9951752254349,41.5667365148483));
#19483=CARTESIAN_POINT('Ctrl Pts',(-4.43916392892557,-5.11037980130094,
41.574877523252));
#19484=CARTESIAN_POINT('Ctrl Pts',(-4.30583804466706,-5.22034938802929,
41.5830185316556));
#19485=CARTESIAN_POINT('Ctrl Pts',(-4.17156589227026,-5.33109947373337,
41.5912173201139));
#19486=CARTESIAN_POINT('Ctrl Pts',(-4.03317083000002,-5.43653975866168,
41.5994161085721));
#19487=CARTESIAN_POINT('Ctrl Pts',(-3.891128225651,-5.53637156733018,41.6076148970304));
#19488=CARTESIAN_POINT('Ctrl Pts',(-3.74908562130194,-5.63620337599872,
41.6158136854886));
#19489=CARTESIAN_POINT('Ctrl Pts',(-3.60339582188938,-5.73042656113058,
41.6240124739468));
#19490=CARTESIAN_POINT('Ctrl Pts',(-3.45455747197761,-5.81879039601907,
41.6322112624051));
#19491=CARTESIAN_POINT('Ctrl Pts',(-3.30509714590246,-5.90752349191479,
41.6404443125371));
#19492=CARTESIAN_POINT('Ctrl Pts',(-3.15199735783756,-5.99062409752655,
41.6486773626691));
#19493=CARTESIAN_POINT('Ctrl Pts',(-2.99572046393637,-6.06777948692542,
41.6569104128011));
#19494=CARTESIAN_POINT('Ctrl Pts',(-2.83962967179355,-6.14484299611554,
41.665133658636));
#19495=CARTESIAN_POINT('Ctrl Pts',(-2.68036962560976,-6.21597522979205,
41.6733569044708));
#19496=CARTESIAN_POINT('Ctrl Pts',(-2.5184306862568,-6.28090724963521,41.6815801503057));
#19497=CARTESIAN_POINT('Ctrl Pts',(-2.35665217885975,-6.34577494170775,
41.6897952494192));
#19498=CARTESIAN_POINT('Ctrl Pts',(-2.19220039386249,-6.40445452045606,
41.6980103485327));
#19499=CARTESIAN_POINT('Ctrl Pts',(-2.02558935548251,-6.45672337667922,
41.7062254476462));
#19500=CARTESIAN_POINT('Ctrl Pts',(-1.85911004216774,-6.50895090839855,
41.7144340517851));
#19501=CARTESIAN_POINT('Ctrl Pts',(-1.69047521596552,-6.55477770611507,
41.722642655924));
#19502=CARTESIAN_POINT('Ctrl Pts',(-1.52021799328566,-6.5940295914479,41.7308512600629));
#19503=CARTESIAN_POINT('Ctrl Pts',(-1.35006132220516,-6.63325829515127,
41.7390550163119));
#19504=CARTESIAN_POINT('Ctrl Pts',(-1.17828451153328,-6.66591974179152,
41.7472587725609));
#19505=CARTESIAN_POINT('Ctrl Pts',(-1.00543501373014,-6.69188982524111,
41.7554625288098));
#19506=CARTESIAN_POINT('Ctrl Pts',(-0.832636657736434,-6.71785222479762,
41.7636638577741));
#19507=CARTESIAN_POINT('Ctrl Pts',(-0.658766600006017,-6.73712714789639,
41.7718651867384));
#19508=CARTESIAN_POINT('Ctrl Pts',(-0.484381893107001,-6.74964170764864,
41.7800665157027));
#19509=CARTESIAN_POINT('Ctrl Pts',(-0.310021235523848,-6.76215454152363,
41.7882667136254));
#19510=CARTESIAN_POINT('Ctrl Pts',(-0.135146427312531,-6.7679088424695,
41.7964669115481));
#19511=CARTESIAN_POINT('Ctrl Pts',(0.039680932635225,-6.76688365672007,
41.8046671094709));
#19512=CARTESIAN_POINT('Ctrl Pts',(0.214515864495584,-6.76585842656903,
41.8128676625507));
#19513=CARTESIAN_POINT('Ctrl Pts',(0.389302985699496,-6.75805312679117,
41.8210682156306));
#19514=CARTESIAN_POINT('Ctrl Pts',(0.563481212773167,-6.74349893770672,
41.8292687687104));
#19515=CARTESIAN_POINT('Ctrl Pts',(0.737698548151672,-6.72894148076456,
41.8374711630636));
#19516=CARTESIAN_POINT('Ctrl Pts',(0.911306360135065,-6.70763214623251,
41.8456735574168));
#19517=CARTESIAN_POINT('Ctrl Pts',(1.08374913724422,-6.67965394369517,41.85387595177));
#19518=CARTESIAN_POINT('Ctrl Pts',(1.25635317866392,-6.65164957662013,41.8620860168039));
#19519=CARTESIAN_POINT('Ctrl Pts',(1.42778965433692,-6.61696393885949,41.8702960818377));
#19520=CARTESIAN_POINT('Ctrl Pts',(1.59751276324409,-6.57573128794602,41.8785061468715));
#19521=CARTESIAN_POINT('Ctrl Pts',(1.76731709862022,-6.53447890381731,41.8867201410968));
#19522=CARTESIAN_POINT('Ctrl Pts',(1.93540608788346,-6.48667335723624,41.8949341353222));
#19523=CARTESIAN_POINT('Ctrl Pts',(2.10124960291294,-6.43249866741208,41.9031481295475));
#19524=CARTESIAN_POINT('Ctrl Pts',(2.26731921788926,-6.37825011944226,41.9113733221827));
#19525=CARTESIAN_POINT('Ctrl Pts',(2.43113690442495,-6.31761519901466,41.9195985148178));
#19526=CARTESIAN_POINT('Ctrl Pts',(2.59219187337344,-6.25082636869852,41.927823707453));
#19527=CARTESIAN_POINT('Ctrl Pts',(2.73702826199803,-6.19076331664487,41.935220605573));
#19528=CARTESIAN_POINT('Ctrl Pts',(2.87963046621809,-6.12572408816284,41.9426175036929));
#19529=CARTESIAN_POINT('Ctrl Pts',(3.01964500430957,-6.05590893656338,41.9500144018129));
#19530=CARTESIAN_POINT('Ctrl Pts',(3.18330293023272,-5.97430453273133,41.9586603683038));
#19531=CARTESIAN_POINT('Ctrl Pts',(3.34379671844566,-5.88598941906037,41.9673063347946));
#19532=CARTESIAN_POINT('Ctrl Pts',(3.50057226502568,-5.79122463882493,41.9759523012855));
#19533=CARTESIAN_POINT('Ctrl Pts',(3.6571472743686,-5.69658107562633,41.9845872084099));
#19534=CARTESIAN_POINT('Ctrl Pts',(3.81001326636679,-5.59550445384675,41.9932221155342));
#19535=CARTESIAN_POINT('Ctrl Pts',(3.95863978141795,-5.4883021127645,42.0018570226586));
#19536=CARTESIAN_POINT('Ctrl Pts',(4.1122005768098,-5.37754074048316,42.0107786017301));
#19537=CARTESIAN_POINT('Ctrl Pts',(4.26123526340441,-5.26024003820608,42.0197001808016));
#19538=CARTESIAN_POINT('Ctrl Pts',(4.40518767082388,-5.13678991052012,42.028621759873));
#19539=CARTESIAN_POINT('Ctrl Pts',(4.54412974150958,-5.01763652729729,42.0372328188487));
#19540=CARTESIAN_POINT('Ctrl Pts',(4.67833706471288,-4.89275476582606,42.0458438778244));
#19541=CARTESIAN_POINT('Ctrl Pts',(4.8073396277206,-4.76253868265101,42.0544549368001));
#19542=CARTESIAN_POINT('Ctrl Pts',(4.93622053535602,-4.63244539925378,42.0630578751496));
#19543=CARTESIAN_POINT('Ctrl Pts',(5.05990625479924,-4.49702803960598,42.0716608134992));
#19544=CARTESIAN_POINT('Ctrl Pts',(5.17796138381624,-4.35671951216828,42.0802637518487));
#19545=CARTESIAN_POINT('Ctrl Pts',(5.29588431839897,-4.2165680978231,42.0888570568975));
#19546=CARTESIAN_POINT('Ctrl Pts',(5.40818904485295,-4.07153667495343,42.0974503619462));
#19547=CARTESIAN_POINT('Ctrl Pts',(5.51447829534973,-3.92209359017818,42.106043666995));
#19548=CARTESIAN_POINT('Ctrl Pts',(5.52632065763324,-3.90544318439959,42.1070011018355));
#19549=CARTESIAN_POINT('Ctrl Pts',(5.53808838564072,-3.88873804974682,42.107958536676));
#19550=CARTESIAN_POINT('Ctrl Pts',(5.54978095996358,-3.87197886053446,42.1089159715166));
#19551=CARTESIAN_POINT('Ctrl Pts',(5.65475576318882,-3.7215164780681,42.1175117290641));
#19552=CARTESIAN_POINT('Ctrl Pts',(5.75354654205222,-3.56687090449153,42.1261074866117));
#19553=CARTESIAN_POINT('Ctrl Pts',(5.84584546916468,-3.40857444551924,42.1347032441592));
#19554=CARTESIAN_POINT('Ctrl Pts',(5.93823051431431,-3.25013029056863,42.1433070218408));
#19555=CARTESIAN_POINT('Ctrl Pts',(6.02411146370063,-3.08802871466845,42.1519107995225));
#19556=CARTESIAN_POINT('Ctrl Pts',(6.10322690035181,-2.92282575649355,42.1605145772041));
#19557=CARTESIAN_POINT('Ctrl Pts',(6.18545164284543,-2.75113017760155,42.1694564908721));
#19558=CARTESIAN_POINT('Ctrl Pts',(6.26036818667169,-2.57608485797007,42.1783984045401));
#19559=CARTESIAN_POINT('Ctrl Pts',(6.32773899548431,-2.39833446479578,42.1873403182082));
#19560=CARTESIAN_POINT('Ctrl Pts',(6.39273868351397,-2.22684001034127,42.1959675205389));
#19561=CARTESIAN_POINT('Ctrl Pts',(6.45071468212739,-2.05282794452216,42.2045947228696));
#19562=CARTESIAN_POINT('Ctrl Pts',(6.50150514702655,-1.87689099928241,42.2132219252003));
#19563=CARTESIAN_POINT('Ctrl Pts',(6.55234398206938,-1.70078650103176,42.2218573436207));
#19564=CARTESIAN_POINT('Ctrl Pts',(6.59598354837541,-1.52275375950016,42.2304927620411));
#19565=CARTESIAN_POINT('Ctrl Pts',(6.63231300466784,-1.34339614712631,42.2391281804615));
#19566=CARTESIAN_POINT('Ctrl Pts',(6.66869613255724,-1.1637735594276,42.2477763564827));
#19567=CARTESIAN_POINT('Ctrl Pts',(6.69774751649917,-0.982822489873342,
42.2564245325038));
#19568=CARTESIAN_POINT('Ctrl Pts',(6.7194078817565,-0.801153367707252,42.2650727085249));
#19569=CARTESIAN_POINT('Ctrl Pts',(6.7216994662713,-0.781933463415356,42.2659876527567));
#19570=CARTESIAN_POINT('Ctrl Pts',(6.72390837236021,-0.762705523586282,
42.2669025969886));
#19571=CARTESIAN_POINT('Ctrl Pts',(6.72603456392106,-0.743470271725283,
42.2678175412204));
#19572=CARTESIAN_POINT('Ctrl Pts',(6.74515052237273,-0.570531820575015,
42.2760435337617));
#19573=CARTESIAN_POINT('Ctrl Pts',(6.75761744990937,-0.396628656856025,
42.2842695263031));
#19574=CARTESIAN_POINT('Ctrl Pts',(6.76334725359576,-0.222312679077808,
42.2924955188444));
#19575=CARTESIAN_POINT('Ctrl Pts',(6.76907105032358,-0.0481794490710688,
42.3007128874958));
#19576=CARTESIAN_POINT('Ctrl Pts',(6.76807177658168,0.126365378010484,42.3089302561473));
#19577=CARTESIAN_POINT('Ctrl Pts',(6.76031290176944,0.300763146295607,42.3171476247987));
#19578=CARTESIAN_POINT('Ctrl Pts',(6.75256060861734,0.475012977300236,42.3253580228611));
#19579=CARTESIAN_POINT('Ctrl Pts',(6.73806015026366,0.649115642033112,42.3335684209235));
#19580=CARTESIAN_POINT('Ctrl Pts',(6.71682701035082,0.822510737329076,42.3417788189858));
#19581=CARTESIAN_POINT('Ctrl Pts',(6.6956076345185,0.995793431724204,42.3499838947746));
#19582=CARTESIAN_POINT('Ctrl Pts',(6.66766431401944,1.16836911596368,42.3581889705634));
#19583=CARTESIAN_POINT('Ctrl Pts',(6.63306450304007,1.33968067035015,42.3663940463522));
#19584=CARTESIAN_POINT('Ctrl Pts',(6.5984802009793,1.51091543654391,42.3745954443217));
#19585=CARTESIAN_POINT('Ctrl Pts',(6.5572454235981,1.68088685131457,42.3827968422912));
#19586=CARTESIAN_POINT('Ctrl Pts',(6.50947905684096,1.84904608069918,42.3909982402606));
#19587=CARTESIAN_POINT('Ctrl Pts',(6.46171643154333,2.01719213845294,42.3991989958284));
#19588=CARTESIAN_POINT('Ctrl Pts',(6.40742332536684,2.1835259467978,42.4073997513961));
#19589=CARTESIAN_POINT('Ctrl Pts',(6.34676911807194,2.34751161059713,42.4156005069638));
#19590=CARTESIAN_POINT('Ctrl Pts',(6.28611521887159,2.51149644142721,42.4238012208756));
#19591=CARTESIAN_POINT('Ctrl Pts',(6.21910040623486,2.6731328149813,42.4320019347873));
#19592=CARTESIAN_POINT('Ctrl Pts',(6.14594301737774,2.83190279267241,42.4402026486991));
#19593=CARTESIAN_POINT('Ctrl Pts',(6.07277274218481,2.99070073696103,42.4484048071287));
#19594=CARTESIAN_POINT('Ctrl Pts',(5.99345788507549,3.14663095396814,42.4566069655583));
#19595=CARTESIAN_POINT('Ctrl Pts',(5.90826376476316,3.29919812772539,42.464809123988));
#19596=CARTESIAN_POINT('Ctrl Pts',(5.82303919844145,3.45181982474768,42.4730142136409));
#19597=CARTESIAN_POINT('Ctrl Pts',(5.731931358044,3.60107577165232,42.4812193032938));
#19598=CARTESIAN_POINT('Ctrl Pts',(5.63525011239159,3.74649772064399,42.4894243929467));
#19599=CARTESIAN_POINT('Ctrl Pts',(5.53845841984662,3.89208579701919,42.4976388559445));
#19600=CARTESIAN_POINT('Ctrl Pts',(5.43608080059845,4.03383082649398,42.5058533189423));
#19601=CARTESIAN_POINT('Ctrl Pts',(5.32846946003411,4.17129502834358,42.5140677819401));
#19602=CARTESIAN_POINT('Ctrl Pts',(5.22079436315163,4.30884067338809,42.5222871117476));
#19603=CARTESIAN_POINT('Ctrl Pts',(5.10787959512425,4.44210016211765,42.530506441555));
#19604=CARTESIAN_POINT('Ctrl Pts',(4.99011572398894,4.57067107339812,42.5387257713625));
#19605=CARTESIAN_POINT('Ctrl Pts',(4.87216938487518,4.69944119751054,42.5469578365232));
#19606=CARTESIAN_POINT('Ctrl Pts',(4.74935917990521,4.8235079720207,42.5551899016839));
#19607=CARTESIAN_POINT('Ctrl Pts',(4.62211136750552,4.94250700620407,42.5634219668446));
#19608=CARTESIAN_POINT('Ctrl Pts',(4.50773189682578,5.04947188272816,42.5708215381057));
#19609=CARTESIAN_POINT('Ctrl Pts',(4.3897675643863,5.15234259889075,42.5782211093669));
#19610=CARTESIAN_POINT('Ctrl Pts',(4.26854835633068,5.25088410933499,42.5856206806281));
#19611=CARTESIAN_POINT('Ctrl Pts',(4.13492892115702,5.35950601157244,42.5937771976381));
#19612=CARTESIAN_POINT('Ctrl Pts',(3.99694264807765,5.46320145068243,42.6019337146481));
#19613=CARTESIAN_POINT('Ctrl Pts',(3.85499061912882,5.56159476467217,42.6100902316581));
#19614=CARTESIAN_POINT('Ctrl Pts',(3.71323923686838,5.65984900144858,42.6182352195753));
#19615=CARTESIAN_POINT('Ctrl Pts',(3.56753356038438,5.75281583359409,42.6263802074924));
#19616=CARTESIAN_POINT('Ctrl Pts',(3.41830902533422,5.84015859436357,42.6345251954095));
#19617=CARTESIAN_POINT('Ctrl Pts',(3.31360945068443,5.90144040635399,42.6402399176579));
#19618=CARTESIAN_POINT('Ctrl Pts',(3.20717838310867,5.95995439641602,42.6459546399062));
#19619=CARTESIAN_POINT('Ctrl Pts',(3.09917575053259,6.01559628526639,42.6516693621546));
#19620=CARTESIAN_POINT('Origin',(0.,0.,-3.69717978381041));
#19621=CARTESIAN_POINT('',(3.09917575053261,6.01559628526638,45.0457515827422));
#19622=CARTESIAN_POINT('',(3.09917575053253,6.01559628526642,44.6513725725535));
#19623=CARTESIAN_POINT('',(3.09917575053259,6.01559628526639,-3.69717978381041));
#19624=CARTESIAN_POINT('',(-6.7672120803281,0.000214420623927318,43.6968126146988));
#19625=CARTESIAN_POINT('Ctrl Pts',(-6.767,1.46149302575801E-12,43.69717978381));
#19626=CARTESIAN_POINT('Ctrl Pts',(-6.76700000000004,-0.186007249414336,
43.705929295616));
#19627=CARTESIAN_POINT('Ctrl Pts',(-6.75932637295445,-0.372014355526311,
43.7146788074219));
#19628=CARTESIAN_POINT('Ctrl Pts',(-6.74400518266937,-0.557389537153946,
43.7234283192279));
#19629=CARTESIAN_POINT('Ctrl Pts',(-6.72868405709656,-0.742763935810554,
43.7321777940784));
#19630=CARTESIAN_POINT('Ctrl Pts',(-6.70571545653,-0.92750612969445,43.740927268929));
#19631=CARTESIAN_POINT('Ctrl Pts',(-6.67517739415656,-1.11098863924943,
43.7496767437795));
#19632=CARTESIAN_POINT('Ctrl Pts',(-6.64463945823074,-1.29447038906637,
43.7584261824015));
#19633=CARTESIAN_POINT('Ctrl Pts',(-6.60653217027127,-1.47669218228355,
43.7671756210235));
#19634=CARTESIAN_POINT('Ctrl Pts',(-6.56098496116676,-1.65703510504262,
43.7759250596455));
#19635=CARTESIAN_POINT('Ctrl Pts',(-6.51543793687472,-1.83737729604181,
43.7846744627657));
#19636=CARTESIAN_POINT('Ctrl Pts',(-6.46245112202584,-2.01584035397232,
43.793423865886));
#19637=CARTESIAN_POINT('Ctrl Pts',(-6.40220448416175,-2.19181813638339,
43.8021732690062));
#19638=CARTESIAN_POINT('Ctrl Pts',(-6.34195808575108,-2.36779521936157,
43.8109226373515));
#19639=CARTESIAN_POINT('Ctrl Pts',(-6.27445201489142,-2.54128677545057,
43.8196720056968));
#19640=CARTESIAN_POINT('Ctrl Pts',(-6.19991555136076,-2.71170355238086,
43.8284213740421));
#19641=CARTESIAN_POINT('Ctrl Pts',(-6.1253793778893,-2.88211966613302,43.8371707083391));
#19642=CARTESIAN_POINT('Ctrl Pts',(-6.04381298133508,-3.0494607621066,43.8459200426362));
#19643=CARTESIAN_POINT('Ctrl Pts',(-5.95549339426198,-3.21315848207055,
43.8546693769332));
#19644=CARTESIAN_POINT('Ctrl Pts',(-5.86717414355047,-3.37685557859834,
43.8634186779088));
#19645=CARTESIAN_POINT('Ctrl Pts',(-5.77210188986118,-3.53690907467507,
43.8721679788843));
#19646=CARTESIAN_POINT('Ctrl Pts',(-5.67059953466942,-3.69277536785098,
43.8809172798599));
#19647=CARTESIAN_POINT('Ctrl Pts',(-5.56909755761632,-3.84864108035987,
43.8896665482406));
#19648=CARTESIAN_POINT('Ctrl Pts',(-5.46116568337928,-4.00031938104473,
43.8984158166214));
#19649=CARTESIAN_POINT('Ctrl Pts',(-5.34717048685965,-4.14729511663412,
43.9071650850022));
#19650=CARTESIAN_POINT('Ctrl Pts',(-5.23317570555368,-4.29427031688222,
43.9159143215148));
#19651=CARTESIAN_POINT('Ctrl Pts',(-5.11311782178657,-4.436542759873,43.9246635580274));
#19652=CARTESIAN_POINT('Ctrl Pts',(-4.98740459171868,-4.57362924147809,
43.93341279454));
#19653=CARTESIAN_POINT('Ctrl Pts',(-4.86169180910655,-4.71071523514618,
43.9421619999112));
#19654=CARTESIAN_POINT('Ctrl Pts',(-4.73032391415227,-4.84261509316725,
43.9509112052823));
#19655=CARTESIAN_POINT('Ctrl Pts',(-4.59374707237057,-4.96888084331742,
43.9596604106534));
#19656=CARTESIAN_POINT('Ctrl Pts',(-4.45717070537163,-5.09514615452933,
43.9684095856097));
#19657=CARTESIAN_POINT('Ctrl Pts',(-4.31538563819269,-5.21577720253831,
43.9771587605659));
#19658=CARTESIAN_POINT('Ctrl Pts',(-4.16887341290407,-5.33036429028838,
43.9859079355221));
#19659=CARTESIAN_POINT('Ctrl Pts',(-4.02236168477094,-5.44495098921357,
43.99465708079));
#19660=CARTESIAN_POINT('Ctrl Pts',(-3.87112305634193,-5.55349359238931,
44.0034062260579));
#19661=CARTESIAN_POINT('Ctrl Pts',(-3.71567117316484,-5.65562346102636,
44.0121553713259));
#19662=CARTESIAN_POINT('Ctrl Pts',(-3.56021980457064,-5.75775299158915,
44.020904487632));
#19663=CARTESIAN_POINT('Ctrl Pts',(-3.40055544862164,-5.85346967275483,
44.0296536039382));
#19664=CARTESIAN_POINT('Ctrl Pts',(-3.23722036323193,-5.94244842803676,
44.0384027202443));
#19665=CARTESIAN_POINT('Ctrl Pts',(-3.07388580495827,-6.03142689616588,
44.0471518083153));
#19666=CARTESIAN_POINT('Ctrl Pts',(-2.90688079257477,-6.11366734484932,
44.0559008963862));
#19667=CARTESIAN_POINT('Ctrl Pts',(-2.73677251094374,-6.18889046787408,
44.0646499844572));
#19668=CARTESIAN_POINT('Ctrl Pts',(-2.56666476416412,-6.26411335438365,
44.0733990450194));
#19669=CARTESIAN_POINT('Ctrl Pts',(-2.39345402971868,-6.33231884350375,
44.0821481055816));
#19670=CARTESIAN_POINT('Ctrl Pts',(-2.21772856473822,-6.39327529621118,
44.0908971661438));
#19671=CARTESIAN_POINT('Ctrl Pts',(-2.04200363768048,-6.45423156232152,
44.0996461999238));
#19672=CARTESIAN_POINT('Ctrl Pts',(-1.86376426619866,-6.50793874252121,
44.1083952337038));
#19673=CARTESIAN_POINT('Ctrl Pts',(-1.68361578194456,-6.55421443796182,
44.1171442674838));
#19674=CARTESIAN_POINT('Ctrl Pts',(-1.50346783419641,-6.60048999558731,
44.1258932752081));
#19675=CARTESIAN_POINT('Ctrl Pts',(-1.32141106257024,-6.63933404145539,
44.1346422829323));
#19676=CARTESIAN_POINT('Ctrl Pts',(-1.13806375958828,-6.67061465527067,
44.1433912906565));
#19677=CARTESIAN_POINT('Ctrl Pts',(-0.954716987416852,-6.70189517852514,
44.1521402730514));
#19678=CARTESIAN_POINT('Ctrl Pts',(-0.77007997380744,-6.72561226535856,
44.1608892554463));
#19679=CARTESIAN_POINT('Ctrl Pts',(-0.58477977054989,-6.74168536939804,
44.1696382378412));
#19680=CARTESIAN_POINT('Ctrl Pts',(-0.391490647551392,-6.75845143942408,
44.1787644185172));
#19681=CARTESIAN_POINT('Ctrl Pts',(-0.197480213101866,-6.76689975924034,
44.1878905991933));
#19682=CARTESIAN_POINT('Ctrl Pts',(-0.00346532629538061,-6.76699911271708,
44.1970167798693));
#19683=CARTESIAN_POINT('Ctrl Pts',(0.184486595298432,-6.76709536139767,
44.2058577673993));
#19684=CARTESIAN_POINT('Ctrl Pts',(0.372442378187562,-6.75935659726757,
44.2146987549292));
#19685=CARTESIAN_POINT('Ctrl Pts',(0.559750217724375,-6.74380965728998,
44.2235397424591));
#19686=CARTESIAN_POINT('Ctrl Pts',(0.745129914460036,-6.72842275717228,
44.2322897210569));
#19687=CARTESIAN_POINT('Ctrl Pts',(0.929874656316456,-6.70538772273441,
44.2410396996547));
#19688=CARTESIAN_POINT('Ctrl Pts',(1.11335688290003,-6.67478280180705,44.2497896782524));
#19689=CARTESIAN_POINT('Ctrl Pts',(1.29683723119081,-6.6441781941798,44.2585395672774));
#19690=CARTESIAN_POINT('Ctrl Pts',(1.47905480730458,-6.60600390230025,44.2672894563023));
#19691=CARTESIAN_POINT('Ctrl Pts',(1.65939064805029,-6.56038959797078,44.2760393453272));
#19692=CARTESIAN_POINT('Ctrl Pts',(1.8397247026449,-6.51477574543193,44.2847891476882));
#19693=CARTESIAN_POINT('Ctrl Pts',(2.01817678126076,-6.46172209820029,44.2935389500492));
#19694=CARTESIAN_POINT('Ctrl Pts',(2.1941407234791,-6.40140886723935,44.3022887524101));
#19695=CARTESIAN_POINT('Ctrl Pts',(2.37010298132326,-6.34109621361289,44.3110384710156));
#19696=CARTESIAN_POINT('Ctrl Pts',(2.54357687927141,-6.27352420825879,44.3197881896211));
#19697=CARTESIAN_POINT('Ctrl Pts',(2.71397317790197,-6.19892237325397,44.3285379082266));
#19698=CARTESIAN_POINT('Ctrl Pts',(2.88436790207423,-6.12432122756859,44.3372875459848));
#19699=CARTESIAN_POINT('Ctrl Pts',(3.05168482126474,-6.04269049717307,44.3460371837431));
#19700=CARTESIAN_POINT('Ctrl Pts',(3.21535561997602,-5.95430745234814,44.3547868215014));
#19701=CARTESIAN_POINT('Ctrl Pts',(3.3790249607549,-5.86592519481396,44.3635363813204));
#19702=CARTESIAN_POINT('Ctrl Pts',(3.5390479938508,-5.77079087940106,44.3722859411394));
#19703=CARTESIAN_POINT('Ctrl Pts',(3.69488118815184,-5.66922763746894,44.3810355009584));
#19704=CARTESIAN_POINT('Ctrl Pts',(3.85071304611026,-5.56766526648918,44.3897849857458));
#19705=CARTESIAN_POINT('Ctrl Pts',(4.00235489706154,-5.45967423580577,44.3985344705333));
#19706=CARTESIAN_POINT('Ctrl Pts',(4.14929168607833,-5.34562133936189,44.4072839553207));
#19707=CARTESIAN_POINT('Ctrl Pts',(4.29622726385928,-5.2315693830839,44.416033367984));
#19708=CARTESIAN_POINT('Ctrl Pts',(4.43845763092229,-5.11145583677061,44.4247827806473));
#19709=CARTESIAN_POINT('Ctrl Pts',(4.57549970661116,-4.9856886620407,44.4335321933106));
#19710=CARTESIAN_POINT('Ctrl Pts',(4.71254069815443,-4.85992248226018,44.4422815367569));
#19711=CARTESIAN_POINT('Ctrl Pts',(4.84439326931456,-4.72850295733857,44.4510308802033));
#19712=CARTESIAN_POINT('Ctrl Pts',(4.97060959434834,-4.59187644221535,44.4597802236496));
#19713=CARTESIAN_POINT('Ctrl Pts',(5.09682496280656,-4.45525096256503,44.4685295007859));
#19714=CARTESIAN_POINT('Ctrl Pts',(5.21740397615984,-4.31341878218151,44.4772787779222));
#19715=CARTESIAN_POINT('Ctrl Pts',(5.33193710452082,-4.16686161438488,44.4860280550585));
#19716=CARTESIAN_POINT('Ctrl Pts',(5.44646940289518,-4.0203055086433,44.4947772687914));
#19717=CARTESIAN_POINT('Ctrl Pts',(5.55495572749788,-3.86902470979956,44.5035264825244));
#19718=CARTESIAN_POINT('Ctrl Pts',(5.65702762491568,-3.71353301465611,44.5122756962573));
#19719=CARTESIAN_POINT('Ctrl Pts',(5.75909881655263,-3.55804239466717,44.5210248494935));
#19720=CARTESIAN_POINT('Ctrl Pts',(5.85475551250888,-3.39834117619372,44.5297740027296));
#19721=CARTESIAN_POINT('Ctrl Pts',(5.94367283728196,-3.23497174691783,44.5385231559657));
#19722=CARTESIAN_POINT('Ctrl Pts',(6.03258957676404,-3.07160339300784,44.5472722516112));
#19723=CARTESIAN_POINT('Ctrl Pts',(6.11476689685368,-2.90456712829328,44.5560213472568));
#19724=CARTESIAN_POINT('Ctrl Pts',(6.18992570525336,-2.73443024475734,44.5647704429023));
#19725=CARTESIAN_POINT('Ctrl Pts',(6.26508404388763,-2.56429442462869,44.5735194838633));
#19726=CARTESIAN_POINT('Ctrl Pts',(6.33322384283372,-2.39105828655842,44.5822685248243));
#19727=CARTESIAN_POINT('Ctrl Pts',(6.39411368720081,-2.21531017131941,44.5910175657854));
#19728=CARTESIAN_POINT('Ctrl Pts',(6.45500317120933,-2.03956309619377,44.5997665549678));
#19729=CARTESIAN_POINT('Ctrl Pts',(6.50864269270112,-1.86130434438497,44.6085155441502));
#19730=CARTESIAN_POINT('Ctrl Pts',(6.55485008446368,-1.68113930719811,44.6172645333326));
#19731=CARTESIAN_POINT('Ctrl Pts',(6.60199664749434,-1.49731239211706,44.6261913468619));
#19732=CARTESIAN_POINT('Ctrl Pts',(6.64140563640933,-1.31150116499538,44.6351181603913));
#19733=CARTESIAN_POINT('Ctrl Pts',(6.67293772282195,-1.12436255155527,44.6440449739207));
#19734=CARTESIAN_POINT('Ctrl Pts',(6.7038449494989,-0.940932395050006,44.6527948880762));
#19735=CARTESIAN_POINT('Ctrl Pts',(6.72718449348945,-0.756227260505368,
44.6615448022317));
#19736=CARTESIAN_POINT('Ctrl Pts',(6.74287707373944,-0.570874564540339,
44.6702947163872));
#19737=CARTESIAN_POINT('Ctrl Pts',(6.75856934538678,-0.385525513631136,
44.6790444584712));
#19738=CARTESIAN_POINT('Ctrl Pts',(6.76661493004107,-0.199529212416906,
44.6877942005552));
#19739=CARTESIAN_POINT('Ctrl Pts',(6.76698649908907,-0.0135174385991209,
44.6965439426392));
#19740=CARTESIAN_POINT('Ctrl Pts',(6.76735806132386,0.172490924447099,44.7052935242851));
#19741=CARTESIAN_POINT('Ctrl Pts',(6.76005588896282,0.35851447290274,44.714043105931));
#19742=CARTESIAN_POINT('Ctrl Pts',(6.74510478454574,0.543921359663555,44.7227926875769));
#19743=CARTESIAN_POINT('Ctrl Pts',(6.73015393440673,0.729325093151777,44.7315421204159));
#19744=CARTESIAN_POINT('Ctrl Pts',(6.70755443556879,0.914111900257673,44.740291553255));
#19745=CARTESIAN_POINT('Ctrl Pts',(6.67738304682297,1.09765415591669,44.749040986094));
#19746=CARTESIAN_POINT('Ctrl Pts',(6.64721213111835,1.28119353391405,44.7577902817553));
#19747=CARTESIAN_POINT('Ctrl Pts',(6.60946960955465,1.46348811672786,44.7665395774167));
#19748=CARTESIAN_POINT('Ctrl Pts',(6.5642836699115,1.64391876348355,44.775288873078));
#19749=CARTESIAN_POINT('Ctrl Pts',(6.51909837867681,1.82434682109845,44.7840380431888));
#19750=CARTESIAN_POINT('Ctrl Pts',(6.46646995271882,2.00291071820571,44.7927872132996));
#19751=CARTESIAN_POINT('Ctrl Pts',(6.40657713281508,2.17900400212826,44.8015363834105));
#19752=CARTESIAN_POINT('Ctrl Pts',(6.34668509279017,2.35509499309773,44.8102854395962));
#19753=CARTESIAN_POINT('Ctrl Pts',(6.27952894037483,2.52871516398229,44.819034495782));
#19754=CARTESIAN_POINT('Ctrl Pts',(6.20533675061404,2.69927486771518,44.8277835519678));
#19755=CARTESIAN_POINT('Ctrl Pts',(6.12832117907873,2.87632521636016,44.83686555325));
#19756=CARTESIAN_POINT('Ctrl Pts',(6.04372366626035,3.05007728920084,44.8459475545323));
#19757=CARTESIAN_POINT('Ctrl Pts',(5.95185378007824,3.21989527478277,44.8550295558146));
#19758=CARTESIAN_POINT('Ctrl Pts',(5.86334450817324,3.38350129286833,44.8637793361217));
#19759=CARTESIAN_POINT('Ctrl Pts',(5.76808562057205,3.54345567125044,44.8725291164288));
#19760=CARTESIAN_POINT('Ctrl Pts',(5.66640068804431,3.69921508465391,44.8812788967359));
#19761=CARTESIAN_POINT('Ctrl Pts',(5.56471941107868,3.85496889852363,44.8900283624894));
#19762=CARTESIAN_POINT('Ctrl Pts',(5.45661270815056,4.00652780919715,44.8987778282429));
#19763=CARTESIAN_POINT('Ctrl Pts',(5.34244776449055,4.15337704569305,44.9075272939964));
#19764=CARTESIAN_POINT('Ctrl Pts',(5.22828631819535,4.30022178356323,44.916276491716));
#19765=CARTESIAN_POINT('Ctrl Pts',(5.10806717844008,4.4423569097275,44.9250256894356));
#19766=CARTESIAN_POINT('Ctrl Pts',(4.98219864544657,4.57929969070713,44.9337748871552));
#19767=CARTESIAN_POINT('Ctrl Pts',(4.85633329943962,4.71623900430066,44.9425238633454));
#19768=CARTESIAN_POINT('Ctrl Pts',(4.72481904033584,4.84798602483679,44.9512728395357));
#19769=CARTESIAN_POINT('Ctrl Pts',(4.58810250737134,4.97409332259185,44.9600218157259));
#19770=CARTESIAN_POINT('Ctrl Pts',(4.45137708685576,5.10020881822193,44.9687713606621));
#19771=CARTESIAN_POINT('Ctrl Pts',(4.30944892635983,5.2206836630799,44.9775209055983));
#19772=CARTESIAN_POINT('Ctrl Pts',(4.1628000946659,5.33510865604906,44.9862704505344));
#19773=CARTESIAN_POINT('Ctrl Pts',(4.01615988348713,5.44952692272947,44.9950194811427));
#19774=CARTESIAN_POINT('Ctrl Pts',(3.8647997823215,5.55789587288682,45.003768511751));
#19775=CARTESIAN_POINT('Ctrl Pts',(3.70923383580982,5.65984746713934,45.0125175423593));
#19776=CARTESIAN_POINT('Ctrl Pts',(3.55366577799451,5.76180044505438,45.0212666917073));
#19777=CARTESIAN_POINT('Ctrl Pts',(3.39389200026746,5.85733573571114,45.0300158410553));
#19778=CARTESIAN_POINT('Ctrl Pts',(3.23045513625943,5.94612887621981,45.0387649904033));
#19779=CARTESIAN_POINT('Ctrl Pts',(3.18695122151514,5.96976399206722,45.0410938545163));
#19780=CARTESIAN_POINT('Ctrl Pts',(3.14318791262633,5.99292165435349,45.0434227186292));
#19781=CARTESIAN_POINT('Ctrl Pts',(3.09917575053261,6.01559628526638,45.0457515827422));
#19782=CARTESIAN_POINT('Ctrl Pts',(3.09917575053267,6.01559628526635,43.0458827467338));
#19783=CARTESIAN_POINT('Ctrl Pts',(2.94523624461966,6.09490439723907,43.0540047924677));
#19784=CARTESIAN_POINT('Ctrl Pts',(2.78817827432546,6.16833687487766,43.0621268382015));
#19785=CARTESIAN_POINT('Ctrl Pts',(2.62849662845226,6.2356470774263,43.0702488839354));
#19786=CARTESIAN_POINT('Ctrl Pts',(2.46882253523766,6.30295409632176,43.0783705455109));
#19787=CARTESIAN_POINT('Ctrl Pts',(2.30652534672956,6.36413926578448,43.0864922070864));
#19788=CARTESIAN_POINT('Ctrl Pts',(2.14212130073705,6.41900345325726,43.0946138686619));
#19789=CARTESIAN_POINT('Ctrl Pts',(1.97771293322712,6.47386908288762,43.1027357437231));
#19790=CARTESIAN_POINT('Ctrl Pts',(1.81119794486564,6.52241328294052,43.1108576187842));
#19791=CARTESIAN_POINT('Ctrl Pts',(1.64310903459608,6.56448640035371,43.1189794938454));
#19792=CARTESIAN_POINT('Ctrl Pts',(1.4749836981359,6.60656863534277,43.1271031289808));
#19793=CARTESIAN_POINT('Ctrl Pts',(1.30528411553005,6.64217690616454,43.1352267641163));
#19794=CARTESIAN_POINT('Ctrl Pts',(1.13455446400562,6.67121242115741,43.1433503992517));
#19795=CARTESIAN_POINT('Ctrl Pts',(0.963755300768497,6.70025975781312,43.151477341884));
#19796=CARTESIAN_POINT('Ctrl Pts',(0.791925593920185,6.72272894853215,43.1596042845164));
#19797=CARTESIAN_POINT('Ctrl Pts',(0.619615901835754,6.73857293009375,43.1677312271487));
#19798=CARTESIAN_POINT('Ctrl Pts',(0.447103370332945,6.75443556286392,43.1758677366504));
#19799=CARTESIAN_POINT('Ctrl Pts',(0.274110089669046,6.76365737737787,43.1840042461521));
#19800=CARTESIAN_POINT('Ctrl Pts',(0.101188800426362,6.76624340581007,43.1921407556538));
#19801=CARTESIAN_POINT('Ctrl Pts',(-0.0718453686045659,6.76883112235334,
43.2002825765169));
#19802=CARTESIAN_POINT('Ctrl Pts',(-0.244807087985825,6.76477443114987,
43.2084243973801));
#19803=CARTESIAN_POINT('Ctrl Pts',(-0.417147791540064,6.75413034520457,
43.2165662182432));
#19804=CARTESIAN_POINT('Ctrl Pts',(-0.589746847604112,6.74347030292243,
43.2247202443476));
#19805=CARTESIAN_POINT('Ctrl Pts',(-0.761722665787755,6.72620317980963,
43.232874270452));
#19806=CARTESIAN_POINT('Ctrl Pts',(-0.932534917209093,6.70243743933398,
43.2410282965563));
#19807=CARTESIAN_POINT('Ctrl Pts',(-1.03325554186012,6.68842380620121,43.2458363744068));
#19808=CARTESIAN_POINT('Ctrl Pts',(-1.13357182950383,6.67215159794002,43.2506444522573));
#19809=CARTESIAN_POINT('Ctrl Pts',(-1.23337550007314,6.65365116878089,43.2554525301078));
#19810=CARTESIAN_POINT('Ctrl Pts',(-1.40424649873686,6.62197711523061,43.2636843021386));
#19811=CARTESIAN_POINT('Ctrl Pts',(-1.57414743562728,6.58367018517124,43.2719160741694));
#19812=CARTESIAN_POINT('Ctrl Pts',(-1.74252458728602,6.53879935941635,43.2801478462002));
#19813=CARTESIAN_POINT('Ctrl Pts',(-1.91070067979916,6.49398211391152,43.2883697886726));
#19814=CARTESIAN_POINT('Ctrl Pts',(-2.07735626741041,6.44261667123134,43.296591731145));
#19815=CARTESIAN_POINT('Ctrl Pts',(-2.24194537073223,6.38482340825902,43.3048136736174));
#19816=CARTESIAN_POINT('Ctrl Pts',(-2.40637091509038,6.32708757682991,43.3130274456073));
#19817=CARTESIAN_POINT('Ctrl Pts',(-2.56873372905258,6.26293676385857,43.3212412175972));
#19818=CARTESIAN_POINT('Ctrl Pts',(-2.72850052018119,6.19254179730513,43.329454989587));
#19819=CARTESIAN_POINT('Ctrl Pts',(-2.88814054352925,6.12220268599925,43.3376622443174));
#19820=CARTESIAN_POINT('Ctrl Pts',(-3.04518832035738,6.04562943313532,43.3458694990477));
#19821=CARTESIAN_POINT('Ctrl Pts',(-3.19912807143316,5.96304189005648,43.354076753778));
#19822=CARTESIAN_POINT('Ctrl Pts',(-3.35297650216819,5.88050333966812,43.3622791397899));
#19823=CARTESIAN_POINT('Ctrl Pts',(-3.50372026521591,5.79195777549586,43.3704815258019));
#19824=CARTESIAN_POINT('Ctrl Pts',(-3.65086575693661,5.69767217597043,43.3786839118138));
#19825=CARTESIAN_POINT('Ctrl Pts',(-3.79796732929761,5.60341471840921,43.3868838496125));
#19826=CARTESIAN_POINT('Ctrl Pts',(-3.94147246628386,5.50342082804556,43.3950837874112));
#19827=CARTESIAN_POINT('Ctrl Pts',(-4.08091406165074,5.39800235470691,43.4032837252099));
#19828=CARTESIAN_POINT('Ctrl Pts',(-4.22033615948397,5.29259862159139,43.4114825164456));
#19829=CARTESIAN_POINT('Ctrl Pts',(-4.3556955610149,5.18177203157267,43.4196813076814));
#19830=CARTESIAN_POINT('Ctrl Pts',(-4.48655593213868,5.06587651525294,43.4278800989172));
#19831=CARTESIAN_POINT('Ctrl Pts',(-4.61742174435583,4.94997618006924,43.4360792310536));
#19832=CARTESIAN_POINT('Ctrl Pts',(-4.74378788509258,4.82900673628776,43.44427836319));
#19833=CARTESIAN_POINT('Ctrl Pts',(-4.86525273595378,4.70336101264769,43.4524774953264));
#19834=CARTESIAN_POINT('Ctrl Pts',(-4.98674467152199,4.57768727203325,43.4606784557374));
#19835=CARTESIAN_POINT('Ctrl Pts',(-5.10333289138271,4.44733543237846,43.4688794161483));
#19836=CARTESIAN_POINT('Ctrl Pts',(-5.21465409925935,4.31273366034557,43.4770803765593));
#19837=CARTESIAN_POINT('Ctrl Pts',(-5.32607964190557,4.17800573405026,43.4852890232443));
#19838=CARTESIAN_POINT('Ctrl Pts',(-5.43222808109294,4.03902019373569,43.4934976699294));
#19839=CARTESIAN_POINT('Ctrl Pts',(-5.53277717272509,3.89623738457658,43.5017063166144));
#19840=CARTESIAN_POINT('Ctrl Pts',(-5.6333742693174,3.75338640689447,43.5099188823379));
#19841=CARTESIAN_POINT('Ctrl Pts',(-5.72836649351828,3.60673484638128,43.5181314480614));
#19842=CARTESIAN_POINT('Ctrl Pts',(-5.81747616663442,3.45677017613849,43.5263440137849));
#19843=CARTESIAN_POINT('Ctrl Pts',(-5.90670811108098,3.30659973272758,43.5345678483337));
#19844=CARTESIAN_POINT('Ctrl Pts',(-5.99004120164727,3.15310740915804,43.5427916828824));
#19845=CARTESIAN_POINT('Ctrl Pts',(-6.06724421044289,2.99680441317869,43.5510155174312));
#19846=CARTESIAN_POINT('Ctrl Pts',(-6.13817925295864,2.85319136184688,43.5585716744057));
#19847=CARTESIAN_POINT('Ctrl Pts',(-6.20393965309091,2.70720593898942,43.5661278313801));
#19848=CARTESIAN_POINT('Ctrl Pts',(-6.26438279490053,2.55925715764443,43.5736839883546));
#19849=CARTESIAN_POINT('Ctrl Pts',(-6.33711745157415,2.38122200767981,43.582776740102));
#19850=CARTESIAN_POINT('Ctrl Pts',(-6.40230502939274,2.19997039809362,43.5918694918494));
#19851=CARTESIAN_POINT('Ctrl Pts',(-6.45968401808883,2.01612781996773,43.6009622435968));
#19852=CARTESIAN_POINT('Ctrl Pts',(-6.51689443909958,1.83282533358212,43.6100282827069));
#19853=CARTESIAN_POINT('Ctrl Pts',(-6.56634198463486,1.64694728694844,43.619094321817));
#19854=CARTESIAN_POINT('Ctrl Pts',(-6.60781461466737,1.45913502397426,43.6281603609271));
#19855=CARTESIAN_POINT('Ctrl Pts',(-6.64920538668722,1.27169346183549,43.6372085056344));
#19856=CARTESIAN_POINT('Ctrl Pts',(-6.68265259622375,1.08232552107935,43.6462566503418));
#19857=CARTESIAN_POINT('Ctrl Pts',(-6.70799399247436,0.891686938856826,
43.6553047950491));
#19858=CARTESIAN_POINT('Ctrl Pts',(-6.73325265009385,0.701670783874526,
43.6643233979309));
#19859=CARTESIAN_POINT('Ctrl Pts',(-6.75045826143766,0.510392489687212,
43.6733420008127));
#19860=CARTESIAN_POINT('Ctrl Pts',(-6.75949971433177,0.318516266380099,
43.6823606036945));
#19861=CARTESIAN_POINT('Ctrl Pts',(-6.76445195659145,0.213420597264003,
43.6873003303997));
#19862=CARTESIAN_POINT('Ctrl Pts',(-6.76695579227593,0.108145788607282,
43.6922400571048));
#19863=CARTESIAN_POINT('Ctrl Pts',(-6.76699941967512,0.00280251968678848,
43.69717978381));
#19864=CARTESIAN_POINT('',(-6.76699727772403,0.00606986618896983,43.3028202161432));
#19865=CARTESIAN_POINT('Ctrl Pts',(3.09917575053259,6.01559628526639,42.6516693621546));
#19866=CARTESIAN_POINT('Ctrl Pts',(2.94547762866111,6.09478003856665,42.6598019609222));
#19867=CARTESIAN_POINT('Ctrl Pts',(2.78859575421918,6.16814523834569,42.6679345596898));
#19868=CARTESIAN_POINT('Ctrl Pts',(2.62901526227188,6.23542843361557,42.6760671584574));
#19869=CARTESIAN_POINT('Ctrl Pts',(2.46953836527548,6.30266795061861,42.6841944777817));
#19870=CARTESIAN_POINT('Ctrl Pts',(2.30736667512768,6.36383318397364,42.692321797106));
#19871=CARTESIAN_POINT('Ctrl Pts',(2.14300853510284,6.41870730119986,42.7004491164302));
#19872=CARTESIAN_POINT('Ctrl Pts',(1.97197764007607,6.47580924565839,42.7089063957471));
#19873=CARTESIAN_POINT('Ctrl Pts',(1.79857940220122,6.52609835618054,42.717363675064));
#19874=CARTESIAN_POINT('Ctrl Pts',(1.62340864502557,6.56938607262933,42.7258209543809));
#19875=CARTESIAN_POINT('Ctrl Pts',(1.45515793721862,6.61096372548239,42.7339441323253));
#19876=CARTESIAN_POINT('Ctrl Pts',(1.28527245991803,6.64608247726379,42.7420673102697));
#19877=CARTESIAN_POINT('Ctrl Pts',(1.11429343029639,6.67462651773103,42.750190488214));
#19878=CARTESIAN_POINT('Ctrl Pts',(0.943309450257023,6.70317138464421,42.7583139013517));
#19879=CARTESIAN_POINT('Ctrl Pts',(0.771232215586851,6.72514110037779,42.7664373144894));
#19880=CARTESIAN_POINT('Ctrl Pts',(0.598611430890102,6.74047130064417,42.7745607276271));
#19881=CARTESIAN_POINT('Ctrl Pts',(0.425952807857227,6.75580486127803,42.7826859214104));
#19882=CARTESIAN_POINT('Ctrl Pts',(0.252750761859558,6.76449597610237,42.7908111151937));
#19883=CARTESIAN_POINT('Ctrl Pts',(0.0795583495546547,6.76653230754248,
42.7989363089769));
#19884=CARTESIAN_POINT('Ctrl Pts',(-0.0937049778566374,6.76856947277582,
42.8070648296899));
#19885=CARTESIAN_POINT('Ctrl Pts',(-0.266958298377293,6.76394642463658,
42.8151933504029));
#19886=CARTESIAN_POINT('Ctrl Pts',(-0.439650370402464,6.75270290711838,
42.8233218711159));
#19887=CARTESIAN_POINT('Ctrl Pts',(-0.612534460621611,6.7414468878107,42.8314594300195));
#19888=CARTESIAN_POINT('Ctrl Pts',(-0.784855691413282,6.72355572461415,
42.8395969889231));
#19889=CARTESIAN_POINT('Ctrl Pts',(-0.956068947050589,6.6991209250532,42.8477345478267));
#19890=CARTESIAN_POINT('Ctrl Pts',(-1.12739465151351,6.67467007729256,42.8558774512869));
#19891=CARTESIAN_POINT('Ctrl Pts',(-1.29761057262233,6.64366709610046,42.8640203547472));
#19892=CARTESIAN_POINT('Ctrl Pts',(-1.46618386057521,6.60625414943967,42.8721632582074));
#19893=CARTESIAN_POINT('Ctrl Pts',(-1.63498327105339,6.56879101742578,42.880317084477));
#19894=CARTESIAN_POINT('Ctrl Pts',(-1.80213529769376,6.52490084712561,42.8884709107467));
#19895=CARTESIAN_POINT('Ctrl Pts',(-1.96712352916672,6.47477521007476,42.8966247370163));
#19896=CARTESIAN_POINT('Ctrl Pts',(-2.01298210917268,6.46084275855065,42.8988910980228));
#19897=CARTESIAN_POINT('Ctrl Pts',(-2.05867364890705,6.44642885910712,42.9011574590293));
#19898=CARTESIAN_POINT('Ctrl Pts',(-2.10418736768364,6.43153827024924,42.9034238200358));
#19899=CARTESIAN_POINT('Ctrl Pts',(-2.26938848846164,6.37748990781063,42.9116500293728));
#19900=CARTESIAN_POINT('Ctrl Pts',(-2.4327367662887,6.31699684427263,42.9198762387097));
#19901=CARTESIAN_POINT('Ctrl Pts',(-2.59369317001151,6.2502035758714,42.9281024480467));
#19902=CARTESIAN_POINT('Ctrl Pts',(-2.75446874610995,6.18348534684587,42.9363194155899));
#19903=CARTESIAN_POINT('Ctrl Pts',(-2.91285747074717,6.1104811434104,42.9445363831331));
#19904=CARTESIAN_POINT('Ctrl Pts',(-3.06833511080451,6.03138530089102,42.9527533506763));
#19905=CARTESIAN_POINT('Ctrl Pts',(-3.22366928400182,5.95236244399301,42.9609627360197));
#19906=CARTESIAN_POINT('Ctrl Pts',(-3.37609740464669,5.86725930414412,42.969172121363));
#19907=CARTESIAN_POINT('Ctrl Pts',(-3.5251148041122,5.77631843113146,42.9773815067064));
#19908=CARTESIAN_POINT('Ctrl Pts',(-3.6740245972852,5.68544322702873,42.985584964007));
#19909=CARTESIAN_POINT('Ctrl Pts',(-3.81952827006225,5.58873887230033,42.9937884213076));
#19910=CARTESIAN_POINT('Ctrl Pts',(-3.96114530187512,5.4864940442356,43.0019918786082));
#19911=CARTESIAN_POINT('Ctrl Pts',(-4.10268847927094,5.38430253766812,43.0101910577401));
#19912=CARTESIAN_POINT('Ctrl Pts',(-4.24034876359638,5.2765765233987,43.0183902368719));
#19913=CARTESIAN_POINT('Ctrl Pts',(-4.37367413811537,5.16364827748568,43.0265894160038));
#19914=CARTESIAN_POINT('Ctrl Pts',(-4.50697439126041,5.05074130968799,43.0347870502336));
#19915=CARTESIAN_POINT('Ctrl Pts',(-4.63594108416167,4.9326342895393,43.0429846844634));
#19916=CARTESIAN_POINT('Ctrl Pts',(-4.76015462476693,4.80970029714014,43.0511823186932));
#19917=CARTESIAN_POINT('Ctrl Pts',(-4.88435919950286,4.68677517825113,43.0593793612088));
#19918=CARTESIAN_POINT('Ctrl Pts',(-5.00381104966564,4.55902403268096,43.0675764037244));
#19919=CARTESIAN_POINT('Ctrl Pts',(-5.11812691275048,4.42685733957841,43.07577344624));
#19920=CARTESIAN_POINT('Ctrl Pts',(-5.23245530110767,4.29467616533753,43.0839713868828));
#19921=CARTESIAN_POINT('Ctrl Pts',(-5.34164634656284,4.15807875103507,43.0921693275256));
#19922=CARTESIAN_POINT('Ctrl Pts',(-5.44535657900357,4.01750926912466,43.1003672681685));
#19923=CARTESIAN_POINT('Ctrl Pts',(-5.54909702391801,3.87689883704302,43.1085675970044));
#19924=CARTESIAN_POINT('Ctrl Pts',(-5.64735326259328,3.73231432104986,43.1167679258404));
#19925=CARTESIAN_POINT('Ctrl Pts',(-5.73982469281005,3.58422955400572,43.1249682546764));
#19926=CARTESIAN_POINT('Ctrl Pts',(-5.83239248065666,3.43599047879164,43.1331771284678));
#19927=CARTESIAN_POINT('Ctrl Pts',(-5.91916322694038,3.28424417030447,43.1413860022592));
#19928=CARTESIAN_POINT('Ctrl Pts',(-5.99988143240041,3.12949066097613,43.1495948760507));
#19929=CARTESIAN_POINT('Ctrl Pts',(-6.08064295843088,2.97465409714647,43.1578081554541));
#19930=CARTESIAN_POINT('Ctrl Pts',(-6.15534531468992,2.81680743893843,43.1660214348575));
#19931=CARTESIAN_POINT('Ctrl Pts',(-6.22378091914611,2.65647135698331,43.1742347142609));
#19932=CARTESIAN_POINT('Ctrl Pts',(-6.29231662142997,2.49590075830803,43.1824600068764));
#19933=CARTESIAN_POINT('Ctrl Pts',(-6.35456712612489,2.33283379430901,43.1906852994918));
#19934=CARTESIAN_POINT('Ctrl Pts',(-6.41037414202956,2.16780819243741,43.1989105921073));
#19935=CARTESIAN_POINT('Ctrl Pts',(-6.46084488412926,2.01856235915123,43.2063493812193));
#19936=CARTESIAN_POINT('Ctrl Pts',(-6.50604607878305,1.8677149212602,43.2137881703314));
#19937=CARTESIAN_POINT('Ctrl Pts',(-6.54589673199735,1.71567041532643,43.2212269594435));
#19938=CARTESIAN_POINT('Ctrl Pts',(-6.60234368379457,1.50030508991207,43.2317637245043));
#19939=CARTESIAN_POINT('Ctrl Pts',(-6.64818382531231,1.28205434231952,43.2423004895651));
#19940=CARTESIAN_POINT('Ctrl Pts',(-6.68317317027446,1.06183114294304,43.2528372546259));
#19941=CARTESIAN_POINT('Ctrl Pts',(-6.71756478004758,0.845370093325244,
43.2631940164525));
#19942=CARTESIAN_POINT('Ctrl Pts',(-6.7414732007806,0.627003238492665,43.2735507782791));
#19943=CARTESIAN_POINT('Ctrl Pts',(-6.75471215089131,0.40761839826148,43.2839075401057));
#19944=CARTESIAN_POINT('Ctrl Pts',(-6.76277078217368,0.27407748137766,43.2902117654515));
#19945=CARTESIAN_POINT('Ctrl Pts',(-6.76687700164212,0.140159793959005,
43.2965159907974));
#19946=CARTESIAN_POINT('Ctrl Pts',(-6.76699727772403,0.0060698661890735,
43.3028202161432));
#19947=CARTESIAN_POINT('Ctrl Pts',(-6.76699727772492,0.00606986519518309,
43.3028202161899));
#19948=CARTESIAN_POINT('Ctrl Pts',(-6.76715235655782,-0.166819977707758,
43.3109486158973));
#19949=CARTESIAN_POINT('Ctrl Pts',(-6.76067749336114,-0.339861581287961,
43.3190770156048));
#19950=CARTESIAN_POINT('Ctrl Pts',(-6.7475647088073,-0.512503171169026,
43.3272054153122));
#19951=CARTESIAN_POINT('Ctrl Pts',(-6.7344591306595,-0.685049882239841,
43.3353293478869));
#19952=CARTESIAN_POINT('Ctrl Pts',(-6.71472292397814,-0.85719665330725,
43.3434532804617));
#19953=CARTESIAN_POINT('Ctrl Pts',(-6.68840018265249,-1.02839291941074,
43.3515772130364));
#19954=CARTESIAN_POINT('Ctrl Pts',(-6.66208305724268,-1.19955266105763,
43.3596994123828));
#19955=CARTESIAN_POINT('Ctrl Pts',(-6.62918224502249,-1.36976193915329,
43.3678216117292));
#19956=CARTESIAN_POINT('Ctrl Pts',(-6.58979359439325,-1.53847631873022,
43.3759438110755));
#19957=CARTESIAN_POINT('Ctrl Pts',(-6.55040804042411,-1.70717743430651,
43.3840653718702));
#19958=CARTESIAN_POINT('Ctrl Pts',(-6.50453574599593,-1.87438352856006,
43.3921869326648));
#19959=CARTESIAN_POINT('Ctrl Pts',(-6.45232345152619,-2.03956149132238,
43.4003084934595));
#19960=CARTESIAN_POINT('Ctrl Pts',(-6.40010530233302,-2.2047579759922,43.4084309649495));
#19961=CARTESIAN_POINT('Ctrl Pts',(-6.34154584781495,-2.36792552707013,
43.4165534364394));
#19962=CARTESIAN_POINT('Ctrl Pts',(-6.27684134802887,-2.5285473481181,43.4246759079294));
#19963=CARTESIAN_POINT('Ctrl Pts',(-6.21211724954308,-2.68921782078769,
43.4328008396792));
#19964=CARTESIAN_POINT('Ctrl Pts',(-6.14124453662508,-2.84734068862425,
43.440925771429));
#19965=CARTESIAN_POINT('Ctrl Pts',(-6.06446711525331,-3.00242029169988,
43.4490507031788));
#19966=CARTESIAN_POINT('Ctrl Pts',(-5.98760984615137,-3.15766117597095,
43.4571840847742));
#19967=CARTESIAN_POINT('Ctrl Pts',(-5.90483576632286,-3.3098521457591,43.4653174663696));
#19968=CARTESIAN_POINT('Ctrl Pts',(-5.81643455838062,-3.45852252097274,
43.473450847965));
#19969=CARTESIAN_POINT('Ctrl Pts',(-5.72798356075828,-3.6072766309067,43.4815888104759));
#19970=CARTESIAN_POINT('Ctrl Pts',(-5.63389931864332,-3.75250588857054,
43.4897267729869));
#19971=CARTESIAN_POINT('Ctrl Pts',(-5.53451396175305,-3.89376992221684,
43.4978647354978));
#19972=CARTESIAN_POINT('Ctrl Pts',(-5.43498826531216,-4.03523343123478,
43.50601418942));
#19973=CARTESIAN_POINT('Ctrl Pts',(-5.33014672314952,-4.1727202412223,43.5141636433421));
#19974=CARTESIAN_POINT('Ctrl Pts',(-5.22036137774323,-4.30582350843213,
43.5223130972642));
#19975=CARTESIAN_POINT('Ctrl Pts',(-5.14529369791631,-4.39683523144351,
43.5278854311265));
#19976=CARTESIAN_POINT('Ctrl Pts',(-5.06791540253621,-4.48579821978216,
43.5334577649888));
#19977=CARTESIAN_POINT('Ctrl Pts',(-4.98835480509962,-4.57259284634436,
43.5390300988511));
#19978=CARTESIAN_POINT('Ctrl Pts',(-4.87195434184831,-4.69957699509482,
43.5471826550644));
#19979=CARTESIAN_POINT('Ctrl Pts',(-4.75051986269689,-4.82231220563415,
43.5553352112776));
#19980=CARTESIAN_POINT('Ctrl Pts',(-4.62439552489982,-4.94036992838457,
43.5634877674909));
#19981=CARTESIAN_POINT('Ctrl Pts',(-4.4984173051886,-5.05829087841713,43.5716308787712));
#19982=CARTESIAN_POINT('Ctrl Pts',(-4.3677603065204,-5.17154488040067,43.5797739900516));
#19983=CARTESIAN_POINT('Ctrl Pts',(-4.23280838067924,-5.27973694538389,
43.5879171013319));
#19984=CARTESIAN_POINT('Ctrl Pts',(-4.09798442793581,-5.38782641328581,
43.5960524906093));
#19985=CARTESIAN_POINT('Ctrl Pts',(-3.958873939743,-5.49086327361666,43.6041878798866));
#19986=CARTESIAN_POINT('Ctrl Pts',(-3.81589699596826,-5.58848987796886,
43.612323269164));
#19987=CARTESIAN_POINT('Ctrl Pts',(-3.67302559240245,-5.6860444180291,43.6204526532026));
#19988=CARTESIAN_POINT('Ctrl Pts',(-3.52629371683801,-5.77819644889409,
43.6285820372412));
#19989=CARTESIAN_POINT('Ctrl Pts',(-3.37615384738565,-5.864629075976,43.6367114212798));
#19990=CARTESIAN_POINT('Ctrl Pts',(-3.22609326899139,-5.95101605672506,
43.6448365120719));
#19991=CARTESIAN_POINT('Ctrl Pts',(-3.07262859721654,-6.03168946716792,
43.652961602864));
#19992=CARTESIAN_POINT('Ctrl Pts',(-2.91624055427901,-6.106376178191,43.6610866936562));
#19993=CARTESIAN_POINT('Ctrl Pts',(-2.75925554427864,-6.18134798458118,
43.6692427996813));
#19994=CARTESIAN_POINT('Ctrl Pts',(-2.59932511257514,-6.25028709286662,
43.6773989057064));
#19995=CARTESIAN_POINT('Ctrl Pts',(-2.43696012126463,-6.31296399224373,
43.6855550117315));
#19996=CARTESIAN_POINT('Ctrl Pts',(-2.27524861968018,-6.37538862843606,
43.6936782909049));
#19997=CARTESIAN_POINT('Ctrl Pts',(-2.11112247080499,-6.43160125810205,
43.7018015700783));
#19998=CARTESIAN_POINT('Ctrl Pts',(-1.94510573082439,-6.48142366273909,
43.7099248492517));
#19999=CARTESIAN_POINT('Ctrl Pts',(-1.77906688431242,-6.53125270165018,
43.7180492101083));
#20000=CARTESIAN_POINT('Ctrl Pts',(-1.61113729568207,-6.57468971550923,
43.726173570965));
#20001=CARTESIAN_POINT('Ctrl Pts',(-1.4418553344958,-6.6116066273173,43.7342979318217));
#20002=CARTESIAN_POINT('Ctrl Pts',(-1.27251862522095,-6.64853547855674,
43.7424249202071));
#20003=CARTESIAN_POINT('Ctrl Pts',(-1.101829029676,-6.67893995077014,43.7505519085925));
#20004=CARTESIAN_POINT('Ctrl Pts',(-0.930334193544025,-6.70274326588172,
43.758678896978));
#20005=CARTESIAN_POINT('Ctrl Pts',(-0.757730662821797,-6.7267004667154,
43.7668584254181));
#20006=CARTESIAN_POINT('Ctrl Pts',(-0.584311816093609,-6.7439708114104,
43.7750379538581));
#20007=CARTESIAN_POINT('Ctrl Pts',(-0.410639352460591,-6.75452917102375,
43.7832174822982));
#20008=CARTESIAN_POINT('Ctrl Pts',(-0.237784768448134,-6.76503780791782,
43.7913584907019));
#20009=CARTESIAN_POINT('Ctrl Pts',(-0.0646793178176682,-6.76889759763473,
43.7994994991056));
#20010=CARTESIAN_POINT('Ctrl Pts',(0.108125414811876,-6.76613611263266,
43.8076405075093));
#20011=CARTESIAN_POINT('Ctrl Pts',(0.28215661305668,-6.76335502824606,43.8158392959675));
#20012=CARTESIAN_POINT('Ctrl Pts',(0.455882432014132,-6.75385835649914,
43.8240380844258));
#20013=CARTESIAN_POINT('Ctrl Pts',(0.628747328436504,-6.73772704975379,
43.832236872884));
#20014=CARTESIAN_POINT('Ctrl Pts',(0.801612224858811,-6.72159574300845,
43.8404356613423));
#20015=CARTESIAN_POINT('Ctrl Pts',(0.973615839090478,-6.69882991421583,
43.8486344498006));
#20016=CARTESIAN_POINT('Ctrl Pts',(1.14421600706632,-6.66956210925224,43.8568332382588));
#20017=CARTESIAN_POINT('Ctrl Pts',(1.31552909102076,-6.64017199792715,43.8650662883908));
#20018=CARTESIAN_POINT('Ctrl Pts',(1.48595952790044,-6.60413421298527,43.8732993385228));
#20019=CARTESIAN_POINT('Ctrl Pts',(1.65495256627668,-6.56151057328831,43.8815323886548));
#20020=CARTESIAN_POINT('Ctrl Pts',(1.82374435992116,-6.51893769179429,43.8897556344897));
#20021=CARTESIAN_POINT('Ctrl Pts',(1.99110181962276,-6.46979465911976,43.8979788803245));
#20022=CARTESIAN_POINT('Ctrl Pts',(2.15647727562801,-6.4141947865418,43.9062021261594));
#20023=CARTESIAN_POINT('Ctrl Pts',(2.32168889514025,-6.35864999643107,43.9144172252729));
#20024=CARTESIAN_POINT('Ctrl Pts',(2.48492208423485,-6.29666121898922,43.9226323243864));
#20025=CARTESIAN_POINT('Ctrl Pts',(2.64564120766742,-6.22839237687319,43.9308474234999));
#20026=CARTESIAN_POINT('Ctrl Pts',(2.8062332642672,-6.16017750907809,43.9390560276388));
#20027=CARTESIAN_POINT('Ctrl Pts',(2.96431488602863,-6.08569260551714,43.9472646317776));
#20028=CARTESIAN_POINT('Ctrl Pts',(3.1193673147187,-6.00515083539661,43.9554732359165));
#20029=CARTESIAN_POINT('Ctrl Pts',(3.27432817155355,-5.92465663214993,43.9636769921655));
#20030=CARTESIAN_POINT('Ctrl Pts',(3.42626308224412,-5.83811285308669,43.9718807484144));
#20031=CARTESIAN_POINT('Ctrl Pts',(3.57467485037603,-5.74578007881342,43.9800845046634));
#20032=CARTESIAN_POINT('Ctrl Pts',(3.723042707207,-5.65347462348047,43.9882858336277));
#20033=CARTESIAN_POINT('Ctrl Pts',(3.86788919213928,-5.55538377050031,43.9964871625919));
#20034=CARTESIAN_POINT('Ctrl Pts',(4.00874301933719,-5.45181331346877,44.0046884915562));
#20035=CARTESIAN_POINT('Ctrl Pts',(4.14957742144741,-5.34825713979219,44.0128886894789));
#20036=CARTESIAN_POINT('Ctrl Pts',(4.28641997345309,-5.23922307866104,44.0210888874016));
#20037=CARTESIAN_POINT('Ctrl Pts',(4.41882960990569,-5.12505940244801,44.0292890853243));
#20038=CARTESIAN_POINT('Ctrl Pts',(4.55124498112526,-5.01089078171511,44.0374896384041));
#20039=CARTESIAN_POINT('Ctrl Pts',(4.67922678288968,-4.89159233721435,44.045690191484));
#20040=CARTESIAN_POINT('Ctrl Pts',(4.80236815335128,-4.76755169029948,44.0538907445638));
#20041=CARTESIAN_POINT('Ctrl Pts',(4.92553717279321,-4.64348319248939,44.062093138917));
#20042=CARTESIAN_POINT('Ctrl Pts',(5.04386334391571,-4.51467062575975,44.0702955332702));
#20043=CARTESIAN_POINT('Ctrl Pts',(5.15697765972981,-4.38153744900664,44.0784979276235));
#20044=CARTESIAN_POINT('Ctrl Pts',(5.27019775731346,-4.24827976932992,44.0867079926573));
#20045=CARTESIAN_POINT('Ctrl Pts',(5.37819602945704,-4.11069368038182,44.0949180576911));
#20046=CARTESIAN_POINT('Ctrl Pts',(5.48064409712424,-3.96923535213739,44.103128122725));
#20047=CARTESIAN_POINT('Ctrl Pts',(5.58314119461901,-3.8277093244468,44.1113421169503));
#20048=CARTESIAN_POINT('Ctrl Pts',(5.68008259290995,-3.682307660451,44.1195561111755));
#20049=CARTESIAN_POINT('Ctrl Pts',(5.77118411546925,-3.53351424298183,44.1277701054008));
#20050=CARTESIAN_POINT('Ctrl Pts',(5.8624098397462,-3.38451797052729,44.135995298036));
#20051=CARTESIAN_POINT('Ctrl Pts',(5.9477796015865,-3.23212101596296,44.1442204906712));
#20052=CARTESIAN_POINT('Ctrl Pts',(6.02705536251554,-3.07683159389211,44.1524456833064));
#20053=CARTESIAN_POINT('Ctrl Pts',(6.09834788452548,-2.93718014922409,44.1598425814265));
#20054=CARTESIAN_POINT('Ctrl Pts',(6.16471252537249,-2.79518992302598,44.1672394795465));
#20055=CARTESIAN_POINT('Ctrl Pts',(6.22601009619027,-2.65124259209468,44.1746363776665));
#20056=CARTESIAN_POINT('Ctrl Pts',(6.29765860812913,-2.48298776696532,44.1832823441574));
#20057=CARTESIAN_POINT('Ctrl Pts',(6.36254645794287,-2.3116769900004,44.1919283106483));
#20058=CARTESIAN_POINT('Ctrl Pts',(6.42042117281807,-2.13786832233172,44.2005742771392));
#20059=CARTESIAN_POINT('Ctrl Pts',(6.47822185806526,-1.96428197957712,44.2092091842636));
#20060=CARTESIAN_POINT('Ctrl Pts',(6.52902720070417,-1.78820440536733,44.217844091388));
#20061=CARTESIAN_POINT('Ctrl Pts',(6.57263275044773,-1.61021356587936,44.2264789985124));
#20062=CARTESIAN_POINT('Ctrl Pts',(6.61768596924769,-1.42631357418107,44.2354005775839));
#20063=CARTESIAN_POINT('Ctrl Pts',(6.6550529727088,-1.24037137989682,44.2443221566554));
#20064=CARTESIAN_POINT('Ctrl Pts',(6.68456328737994,-1.05304447057679,44.2532437357268));
#20065=CARTESIAN_POINT('Ctrl Pts',(6.71304648054431,-0.872237569582721,
44.2618547947025));
#20066=CARTESIAN_POINT('Ctrl Pts',(6.73421058578448,-0.690141055066458,
44.2704658536782));
#20067=CARTESIAN_POINT('Ctrl Pts',(6.74795340358676,-0.507359697869109,
44.2790769126539));
#20068=CARTESIAN_POINT('Ctrl Pts',(6.76168326127738,-0.324750711930169,
44.2876798510034));
#20069=CARTESIAN_POINT('Ctrl Pts',(6.76800576214893,-0.141458474040101,
44.296282789353));
#20070=CARTESIAN_POINT('Ctrl Pts',(6.76687024857627,0.0419051182232875,
44.3048857277025));
#20071=CARTESIAN_POINT('Ctrl Pts',(6.76573600651614,0.225063385681669,44.3134790327512));
#20072=CARTESIAN_POINT('Ctrl Pts',(6.75716041240889,0.408292543811773,44.3220723378));
#20073=CARTESIAN_POINT('Ctrl Pts',(6.74114481887468,0.590978452195285,44.3306656428487));
#20074=CARTESIAN_POINT('Ctrl Pts',(6.7393604196064,0.611332652652995,44.3316230776892));
#20075=CARTESIAN_POINT('Ctrl Pts',(6.73748371635307,0.631680107803456,44.3325805125297));
#20076=CARTESIAN_POINT('Ctrl Pts',(6.735514751076,0.652019967514503,44.3335379473702));
#20077=CARTESIAN_POINT('Ctrl Pts',(6.71783757094296,0.834629263971174,44.3421337049178));
#20078=CARTESIAN_POINT('Ctrl Pts',(6.69274026974788,1.01641209288584,44.3507294624654));
#20079=CARTESIAN_POINT('Ctrl Pts',(6.66033376041236,1.19676363577414,44.359325220013));
#20080=CARTESIAN_POINT('Ctrl Pts',(6.62789701470164,1.37728345278487,44.3679289976947));
#20081=CARTESIAN_POINT('Ctrl Pts',(6.58813750239558,1.55636901769334,44.3765327753764));
#20082=CARTESIAN_POINT('Ctrl Pts',(6.54121685482633,1.73342754626088,44.385136553058));
#20083=CARTESIAN_POINT('Ctrl Pts',(6.49245218477855,1.91744462982725,44.3940784667261));
#20084=CARTESIAN_POINT('Ctrl Pts',(6.43595222804921,2.09927176573737,44.4030203803941));
#20085=CARTESIAN_POINT('Ctrl Pts',(6.37195427288985,2.27826419543494,44.4119622940621));
#20086=CARTESIAN_POINT('Ctrl Pts',(6.31020873067017,2.45095697284283,44.4205894963928));
#20087=CARTESIAN_POINT('Ctrl Pts',(6.24148413654294,2.62101092201237,44.4292166987236));
#20088=CARTESIAN_POINT('Ctrl Pts',(6.16604171145989,2.78786990595631,44.4378439010543));
#20089=CARTESIAN_POINT('Ctrl Pts',(6.09052743901424,2.95488779754286,44.4464793194748));
#20090=CARTESIAN_POINT('Ctrl Pts',(6.00828269922023,3.11870437662215,44.4551147378952));
#20091=CARTESIAN_POINT('Ctrl Pts',(5.91961443617632,3.27878848464077,44.4637501563157));
#20092=CARTESIAN_POINT('Ctrl Pts',(5.83081517840424,3.43910909412556,44.4723983323368));
#20093=CARTESIAN_POINT('Ctrl Pts',(5.73557358823278,3.59568595059942,44.4810465083579));
#20094=CARTESIAN_POINT('Ctrl Pts',(5.63424043766182,3.74801596723072,44.489694684379));
#20095=CARTESIAN_POINT('Ctrl Pts',(5.62351977455632,3.76413190540057,44.4906096286107));
#20096=CARTESIAN_POINT('Ctrl Pts',(5.61273096715472,3.78020033939302,44.4915245728425));
#20097=CARTESIAN_POINT('Ctrl Pts',(5.60187445720227,3.79622069507883,44.4924395170742));
#20098=CARTESIAN_POINT('Ctrl Pts',(5.50426680375573,3.94025495035235,44.5006655086577));
#20099=CARTESIAN_POINT('Ctrl Pts',(5.40097240507913,4.08071133054436,44.5088915002412));
#20100=CARTESIAN_POINT('Ctrl Pts',(5.29228213753906,4.21711261133551,44.5171174918247));
#20101=CARTESIAN_POINT('Ctrl Pts',(5.18370187668307,4.35337583880372,44.5253351577864));
#20102=CARTESIAN_POINT('Ctrl Pts',(5.06973684219314,4.48559186080498,44.5335528237481));
#20103=CARTESIAN_POINT('Ctrl Pts',(4.95072157811933,4.61331170158094,44.5417704897098));
#20104=CARTESIAN_POINT('Ctrl Pts',(4.83180519152927,4.74092543313991,44.5499813284621));
#20105=CARTESIAN_POINT('Ctrl Pts',(4.70784717391219,4.86405016171377,44.5581921672144));
#20106=CARTESIAN_POINT('Ctrl Pts',(4.57922282039794,4.98226929833653,44.5664030059667));
#20107=CARTESIAN_POINT('Ctrl Pts',(4.45069209100074,5.10040238467422,44.5746078681484));
#20108=CARTESIAN_POINT('Ctrl Pts',(4.31750205727295,5.21363675318523,44.5828127303301));
#20109=CARTESIAN_POINT('Ctrl Pts',(4.18006535127247,5.32159211694127,44.5910175925118));
#20110=CARTESIAN_POINT('Ctrl Pts',(4.0426867279238,5.42950185726825,44.5992189872053));
#20111=CARTESIAN_POINT('Ctrl Pts',(3.90106528814467,5.5321368156678,44.6074203818988));
#20112=CARTESIAN_POINT('Ctrl Pts',(3.7556474699345,5.62915633834899,44.6156217765923));
#20113=CARTESIAN_POINT('Ctrl Pts',(3.61025764095278,5.72615718724166,44.6238215927261));
#20114=CARTESIAN_POINT('Ctrl Pts',(3.46107318584336,5.81754455327705,44.6320214088599));
#20115=CARTESIAN_POINT('Ctrl Pts',(3.30857042086482,5.90302047854981,44.6402212249937));
#20116=CARTESIAN_POINT('Ctrl Pts',(3.23943832861813,5.94176816651244,44.643938340847));
#20117=CARTESIAN_POINT('Ctrl Pts',(3.16962471935677,5.9793016728163,44.6476554567003));
#20118=CARTESIAN_POINT('Ctrl Pts',(3.09917575053253,6.01559628526642,44.6513725725535));
#20119=CARTESIAN_POINT('Origin',(0.,0.,-3.69717978381041));
#20120=CARTESIAN_POINT('',(3.09917575053261,6.01559628526638,47.0456199604263));
#20121=CARTESIAN_POINT('',(3.09917575053265,6.01559628526636,46.6512392818024));
#20122=CARTESIAN_POINT('',(3.09917575053259,6.01559628526639,-3.69717978381041));
#20123=CARTESIAN_POINT('',(-6.76766674060731,-0.00120259113188305,45.6960259323079));
#20124=CARTESIAN_POINT('Ctrl Pts',(-6.76699874733023,-0.0041174787364938,
45.69717978381));
#20125=CARTESIAN_POINT('Ctrl Pts',(-6.76687707323121,-0.204086568634054,
45.7065548943844));
#20126=CARTESIAN_POINT('Ctrl Pts',(-6.7578875822965,-0.403727183863877,
45.7159300049587));
#20127=CARTESIAN_POINT('Ctrl Pts',(-6.74014155289775,-0.602312914439911,
45.7253051155331));
#20128=CARTESIAN_POINT('Ctrl Pts',(-6.72232161735131,-0.801725686716585,
45.734719270239));
#20129=CARTESIAN_POINT('Ctrl Pts',(-6.69567215036646,-1.00007463449364,
45.744133424945));
#20130=CARTESIAN_POINT('Ctrl Pts',(-6.66035568938451,-1.19664158831433,
45.7535475796509));
#20131=CARTESIAN_POINT('Ctrl Pts',(-6.62485099266477,-1.39425623843718,
45.7630119115351));
#20132=CARTESIAN_POINT('Ctrl Pts',(-6.58058674220859,-1.59006971430474,
45.7724762434192));
#20133=CARTESIAN_POINT('Ctrl Pts',(-6.52777710226088,-1.78337183537215,
45.7819405753034));
#20134=CARTESIAN_POINT('Ctrl Pts',(-6.49176167599389,-1.91520114334412,
45.788395115563));
#20135=CARTESIAN_POINT('Ctrl Pts',(-6.45177276579902,-2.04586281575445,
45.7948496558226));
#20136=CARTESIAN_POINT('Ctrl Pts',(-6.40789099875665,-2.1751372251087,45.8013041960823));
#20137=CARTESIAN_POINT('Ctrl Pts',(-6.34911231426086,-2.3482975199864,45.8099499141346));
#20138=CARTESIAN_POINT('Ctrl Pts',(-6.28325801214895,-2.51922872732067,
45.818595632187));
#20139=CARTESIAN_POINT('Ctrl Pts',(-6.21051183233006,-2.6873466059458,45.8272413502393));
#20140=CARTESIAN_POINT('Ctrl Pts',(-6.13785904378099,-2.85524865547579,
45.8358759689516));
#20141=CARTESIAN_POINT('Ctrl Pts',(-6.05833214096519,-3.02034429973347,
45.8445105876639));
#20142=CARTESIAN_POINT('Ctrl Pts',(-5.97216393053393,-3.18206646486675,
45.8531452063762));
#20143=CARTESIAN_POINT('Ctrl Pts',(-5.88295259364632,-3.34950002863337,
45.8620847662787));
#20144=CARTESIAN_POINT('Ctrl Pts',(-5.78662237322204,-3.51331717483302,
45.8710243261811));
#20145=CARTESIAN_POINT('Ctrl Pts',(-5.6834863835324,-3.67291049825636,45.8799638860836));
#20146=CARTESIAN_POINT('Ctrl Pts',(-5.58414500021901,-3.82663202227688,
45.888574539354));
#20147=CARTESIAN_POINT('Ctrl Pts',(-5.47848986391709,-3.97643467025301,
45.8971851926245));
#20148=CARTESIAN_POINT('Ctrl Pts',(-5.36684796464517,-4.12179959779512,
45.905795845895));
#20149=CARTESIAN_POINT('Ctrl Pts',(-5.2553117419003,-4.2670269277077,45.914398348606));
#20150=CARTESIAN_POINT('Ctrl Pts',(-5.13780023956334,-4.40782467096363,
45.9230008513171));
#20151=CARTESIAN_POINT('Ctrl Pts',(-5.01468361606663,-4.54370303065165,
45.9316033540281));
#20152=CARTESIAN_POINT('Ctrl Pts',(-4.8917055578514,-4.67942846198098,45.9401961747955));
#20153=CARTESIAN_POINT('Ctrl Pts',(-4.76313516799962,-4.81024532969496,
45.9487889955629));
#20154=CARTESIAN_POINT('Ctrl Pts',(-4.62938286366172,-4.93569684053176,
45.9573818163304));
#20155=CARTESIAN_POINT('Ctrl Pts',(-4.61361954705468,-4.95048187092014,
45.9583945192888));
#20156=CARTESIAN_POINT('Ctrl Pts',(-4.59778430079689,-4.96519241644914,
45.9594072222473));
#20157=CARTESIAN_POINT('Ctrl Pts',(-4.581877832874,-4.9798277605373,45.9604199252057));
#20158=CARTESIAN_POINT('Ctrl Pts',(-4.44687260680354,-5.10404439661381,
45.9690151829658));
#20159=CARTESIAN_POINT('Ctrl Pts',(-4.30689265901136,-5.22269458332118,
45.9776104407259));
#20160=CARTESIAN_POINT('Ctrl Pts',(-4.1624241898148,-5.33540194025198,45.986205698486));
#20161=CARTESIAN_POINT('Ctrl Pts',(-4.01782043202398,-5.44821484284245,
45.9948090053404));
#20162=CARTESIAN_POINT('Ctrl Pts',(-3.86872000361035,-5.55507361946534,
46.0034123121948));
#20163=CARTESIAN_POINT('Ctrl Pts',(-3.7156388435457,-5.65564470103404,46.0120156190493));
#20164=CARTESIAN_POINT('Ctrl Pts',(-3.5562108855009,-5.76038549451955,46.0209756219892));
#20165=CARTESIAN_POINT('Ctrl Pts',(-3.392465403019,-5.85830590497551,46.0299356249292));
#20166=CARTESIAN_POINT('Ctrl Pts',(-3.22501316908197,-5.94908220310057,
46.0388956278692));
#20167=CARTESIAN_POINT('Ctrl Pts',(-3.06378731054833,-6.03648316668055,
46.0475224710739));
#20168=CARTESIAN_POINT('Ctrl Pts',(-2.89912567226049,-6.11726162817497,
46.0561493142787));
#20169=CARTESIAN_POINT('Ctrl Pts',(-2.73159394639005,-6.1911778775969,46.0647761574835));
#20170=CARTESIAN_POINT('Ctrl Pts',(-2.56390210253855,-6.26516477226864,
46.0734112457696));
#20171=CARTESIAN_POINT('Ctrl Pts',(-2.39333497820425,-6.33227624899114,
46.0820463340558));
#20172=CARTESIAN_POINT('Ctrl Pts',(-2.22047563376888,-6.39232171905003,
46.0906814223419));
#20173=CARTESIAN_POINT('Ctrl Pts',(-2.04735955851763,-6.45245636868187,
46.0993293354671));
#20174=CARTESIAN_POINT('Ctrl Pts',(-1.87194475060178,-6.505503947692,46.1079772485922));
#20175=CARTESIAN_POINT('Ctrl Pts',(-1.69482816952968,-6.55132402463568,
46.1166251617174));
#20176=CARTESIAN_POINT('Ctrl Pts',(-1.67495838541209,-6.5564643397412,46.1175953259213));
#20177=CARTESIAN_POINT('Ctrl Pts',(-1.65506719264996,-6.56151374690653,
46.1185654901251));
#20178=CARTESIAN_POINT('Ctrl Pts',(-1.63515544032632,-6.5664720882656,46.119535654329));
#20179=CARTESIAN_POINT('Ctrl Pts',(-1.46635125143795,-6.60850700200626,
46.1277603338477));
#20180=CARTESIAN_POINT('Ctrl Pts',(-1.29570268034101,-6.64408396036139,
46.1359850133665));
#20181=CARTESIAN_POINT('Ctrl Pts',(-1.12374468653719,-6.67304180111884,
46.1442096928853));
#20182=CARTESIAN_POINT('Ctrl Pts',(-0.951967440038932,-6.70196920390959,
46.1524257273355));
#20183=CARTESIAN_POINT('Ctrl Pts',(-0.778883862167657,-6.72429128480226,
46.1606417617856));
#20184=CARTESIAN_POINT('Ctrl Pts',(-0.605042517849,-6.73989707277455,46.1688577962357));
#20185=CARTESIAN_POINT('Ctrl Pts',(-0.431349079722954,-6.75548958316498,
46.1770668403903));
#20186=CARTESIAN_POINT('Ctrl Pts',(-0.256899514153053,-6.7643771494694,
46.1852758845449));
#20187=CARTESIAN_POINT('Ctrl Pts',(-0.0822510853937956,-6.76650011150163,
46.1934849286995));
#20188=CARTESIAN_POINT('Ctrl Pts',(0.0922837230030589,-6.76862169240654,
46.2016886323276));
#20189=CARTESIAN_POINT('Ctrl Pts',(0.267016779777068,-6.76398743074585,
46.2098923359556));
#20190=CARTESIAN_POINT('Ctrl Pts',(0.441387114435408,-6.75258960808447,
46.2180960395836));
#20191=CARTESIAN_POINT('Ctrl Pts',(0.61567891936995,-6.74119691856611,46.2262960485776));
#20192=CARTESIAN_POINT('Ctrl Pts',(0.789607970726171,-6.72304675994468,
46.2344960575716));
#20193=CARTESIAN_POINT('Ctrl Pts',(0.962614622985368,-6.69818349163523,
46.2426960665655));
#20194=CARTESIAN_POINT('Ctrl Pts',(1.1356074412675,-6.67332221144519,46.2508954198695));
#20195=CARTESIAN_POINT('Ctrl Pts',(1.30767765162365,-6.64174893307519,46.2590947731734));
#20196=CARTESIAN_POINT('Ctrl Pts',(1.4782716717604,-6.6035597873019,46.2672941264774));
#20197=CARTESIAN_POINT('Ctrl Pts',(1.64886457967465,-6.56537089051054,46.2754934263239));
#20198=CARTESIAN_POINT('Ctrl Pts',(1.81798096644585,-6.52056628949023,46.2836927261705));
#20199=CARTESIAN_POINT('Ctrl Pts',(1.98507849305553,-6.46929303528665,46.2918920260171));
#20200=CARTESIAN_POINT('Ctrl Pts',(2.15220524336969,-6.41801081389811,46.3000927598401));
#20201=CARTESIAN_POINT('Ctrl Pts',(2.31731208732258,-6.36025779056477,46.3082934936631));
#20202=CARTESIAN_POINT('Ctrl Pts',(2.47987281956919,-6.296230602413,46.3164942274862));
#20203=CARTESIAN_POINT('Ctrl Pts',(2.64249147251195,-6.23218060125307,46.3246978832461));
#20204=CARTESIAN_POINT('Ctrl Pts',(2.80256187322549,-6.16185211335252,46.3329015390061));
#20205=CARTESIAN_POINT('Ctrl Pts',(2.95957868273731,-6.08548954651036,46.3411051947661));
#20206=CARTESIAN_POINT('Ctrl Pts',(3.11677536509815,-6.00903950143897,46.3493182483411));
#20207=CARTESIAN_POINT('Ctrl Pts',(3.27091114488567,-5.92654172444302,46.3575313019161));
#20208=CARTESIAN_POINT('Ctrl Pts',(3.42150521013566,-5.83828665766033,46.3657443554912));
#20209=CARTESIAN_POINT('Ctrl Pts',(3.57218838527274,-5.74997936837454,46.3739622689142));
#20210=CARTESIAN_POINT('Ctrl Pts',(3.71932536677659,-5.6559081912402,46.3821801823373));
#20211=CARTESIAN_POINT('Ctrl Pts',(3.86246525736947,-5.5564063148418,46.3903980957604));
#20212=CARTESIAN_POINT('Ctrl Pts',(4.00582839790815,-5.4567492490799,46.3986288263564));
#20213=CARTESIAN_POINT('Ctrl Pts',(4.14518170305987,-5.35164477300992,46.4068595569524));
#20214=CARTESIAN_POINT('Ctrl Pts',(4.28010718289921,-5.24146654123582,46.4150902875484));
#20215=CARTESIAN_POINT('Ctrl Pts',(4.40402009935294,-5.14028101241576,46.4226492292242));
#20216=CARTESIAN_POINT('Ctrl Pts',(4.52419874326469,-5.03481675630696,46.4302081709001));
#20217=CARTESIAN_POINT('Ctrl Pts',(4.6403480297744,-4.92538923970166,46.437767112576));
#20218=CARTESIAN_POINT('Ctrl Pts',(4.76563921444728,-4.80734888316323,46.4459210047427));
#20219=CARTESIAN_POINT('Ctrl Pts',(4.88662865956076,-4.68433134391698,46.4540748969094));
#20220=CARTESIAN_POINT('Ctrl Pts',(5.00289112422744,-4.55668403547211,46.4622287890761));
#20221=CARTESIAN_POINT('Ctrl Pts',(5.11901171620532,-4.42919249240618,46.4703727312163));
#20222=CARTESIAN_POINT('Ctrl Pts',(5.23041656606654,-4.29708269318446,46.4785166733565));
#20223=CARTESIAN_POINT('Ctrl Pts',(5.33671427509191,-4.16074148993064,46.4866606154968));
#20224=CARTESIAN_POINT('Ctrl Pts',(5.44290464476189,-4.02453796393255,46.4947963338897));
#20225=CARTESIAN_POINT('Ctrl Pts',(5.54399791740909,-3.88411182654212,46.5029320522826));
#20226=CARTESIAN_POINT('Ctrl Pts',(5.63964029380605,-3.7398858747934,46.5110677706755));
#20227=CARTESIAN_POINT('Ctrl Pts',(5.7352062089921,-3.59577522435077,46.5191969849757));
#20228=CARTESIAN_POINT('Ctrl Pts',(5.82532970345467,-3.447871111354,46.5273261992759));
#20229=CARTESIAN_POINT('Ctrl Pts',(5.90969796537712,-3.29662842280072,46.5354554135761));
#20230=CARTESIAN_POINT('Ctrl Pts',(5.9940165186433,-3.14547484442522,46.5435798382515));
#20231=CARTESIAN_POINT('Ctrl Pts',(6.07258641453862,-2.99098692630713,46.551704262927));
#20232=CARTESIAN_POINT('Ctrl Pts',(6.14513881239261,-2.83364746862166,46.5598286876024));
#20233=CARTESIAN_POINT('Ctrl Pts',(6.21813164974716,-2.67535285970467,46.5680024327366));
#20234=CARTESIAN_POINT('Ctrl Pts',(6.28503348242055,-2.51417228940198,46.5761761778708));
#20235=CARTESIAN_POINT('Ctrl Pts',(6.34561781566061,-2.35062194696865,46.5843499230049));
#20236=CARTESIAN_POINT('Ctrl Pts',(6.40581418455886,-2.18811893306995,46.5924713258671));
#20237=CARTESIAN_POINT('Ctrl Pts',(6.45977362134892,-2.02327676416144,46.6005927287292));
#20238=CARTESIAN_POINT('Ctrl Pts',(6.5073226460148,-1.85662085000221,46.6087141315914));
#20239=CARTESIAN_POINT('Ctrl Pts',(6.55487534692094,-1.68995205088511,46.6168361623577));
#20240=CARTESIAN_POINT('Ctrl Pts',(6.59601654801478,-1.52146957912764,46.6249581931239));
#20241=CARTESIAN_POINT('Ctrl Pts',(6.63062301652858,-1.35171277003713,46.6330802238902));
#20242=CARTESIAN_POINT('Ctrl Pts',(6.66523875050299,-1.18191051062781,46.6412044292313));
#20243=CARTESIAN_POINT('Ctrl Pts',(6.69331619506547,-1.01083359297957,46.6493286345724));
#20244=CARTESIAN_POINT('Ctrl Pts',(6.7147834865773,-0.839030230914723,46.6574528399135));
#20245=CARTESIAN_POINT('Ctrl Pts',(6.73648314666556,-0.665367216333993,
46.665664984156));
#20246=CARTESIAN_POINT('Ctrl Pts',(6.75142866861152,-0.490962319540475,
46.6738771283984));
#20247=CARTESIAN_POINT('Ctrl Pts',(6.75959981342889,-0.316384832588614,
46.6820892726408));
#20248=CARTESIAN_POINT('Ctrl Pts',(6.76769636469985,-0.143401045683258,
46.6902264490573));
#20249=CARTESIAN_POINT('Ctrl Pts',(6.76914176934004,0.0297518272489233,
46.6983636254738));
#20250=CARTESIAN_POINT('Ctrl Pts',(6.76396877858226,0.20252249841538,46.7065008018902));
#20251=CARTESIAN_POINT('Ctrl Pts',(6.75872429965996,0.377680774497899,46.7147504300456));
#20252=CARTESIAN_POINT('Ctrl Pts',(6.7466771868812,0.552445816264765,46.7230000582011));
#20253=CARTESIAN_POINT('Ctrl Pts',(6.7279155491853,0.7262515838404,46.7312496863565));
#20254=CARTESIAN_POINT('Ctrl Pts',(6.7091539114894,0.900057351416098,46.7394993145119));
#20255=CARTESIAN_POINT('Ctrl Pts',(6.68367786756759,1.07290347336076,46.7477489426673));
#20256=CARTESIAN_POINT('Ctrl Pts',(6.6516284246408,1.24423804013162,46.7559985708227));
#20257=CARTESIAN_POINT('Ctrl Pts',(6.61967322770685,1.41506877298592,46.764223939761));
#20258=CARTESIAN_POINT('Ctrl Pts',(6.58108788452275,1.58490752284196,46.7724493086992));
#20259=CARTESIAN_POINT('Ctrl Pts',(6.535944853491,1.75320103585543,46.7806746776375));
#20260=CARTESIAN_POINT('Ctrl Pts',(6.4908532574364,1.92130279893985,46.7888906747712));
#20261=CARTESIAN_POINT('Ctrl Pts',(6.43921894433532,2.08786248769128,46.7971066719049));
#20262=CARTESIAN_POINT('Ctrl Pts',(6.38116573048613,2.25233499286172,46.8053226690386));
#20263=CARTESIAN_POINT('Ctrl Pts',(6.32316699653763,2.41665314920023,46.8135309558893));
#20264=CARTESIAN_POINT('Ctrl Pts',(6.25876147769551,2.5788876867241,46.82173924274));
#20265=CARTESIAN_POINT('Ctrl Pts',(6.18812335874269,2.73850658151175,46.8299475295907));
#20266=CARTESIAN_POINT('Ctrl Pts',(6.1175373414047,2.8980077438017,46.8381497621324));
#20267=CARTESIAN_POINT('Ctrl Pts',(6.04072802571354,3.05489677954035,46.8463519946741));
#20268=CARTESIAN_POINT('Ctrl Pts',(5.95791849285489,3.20865956943048,46.8545542272158));
#20269=CARTESIAN_POINT('Ctrl Pts',(5.875152242314,3.36234199164185,46.862752172671));
#20270=CARTESIAN_POINT('Ctrl Pts',(5.78639219198939,3.51290110800492,46.8709501181261));
#20271=CARTESIAN_POINT('Ctrl Pts',(5.69190839107925,3.6598453338306,46.8791480635812));
#20272=CARTESIAN_POINT('Ctrl Pts',(5.59745048915356,3.80674928072823,46.887343761895));
#20273=CARTESIAN_POINT('Ctrl Pts',(5.49727215463076,3.95004000869569,46.8955394602087));
#20274=CARTESIAN_POINT('Ctrl Pts',(5.39168806620751,4.08925284088861,46.9037351585224));
#20275=CARTESIAN_POINT('Ctrl Pts',(5.28611371010395,4.2284528409985,46.9119301013894));
#20276=CARTESIAN_POINT('Ctrl Pts',(5.17513480943015,4.36357540829451,46.9201250442564));
#20277=CARTESIAN_POINT('Ctrl Pts',(5.05910785515908,4.49418699097709,46.9283199871233));
#20278=CARTESIAN_POINT('Ctrl Pts',(4.94307048684747,4.62481029674872,46.9365156655303));
#20279=CARTESIAN_POINT('Ctrl Pts',(4.82198440133823,4.75092154380613,46.9447113439373));
#20280=CARTESIAN_POINT('Ctrl Pts',(4.69624467744004,4.87212222030771,46.9529070223443));
#20281=CARTESIAN_POINT('Ctrl Pts',(4.57041656617863,4.9934080934988,46.9611084618138));
#20282=CARTESIAN_POINT('Ctrl Pts',(4.43992853930252,5.10977625015996,46.9693099012832));
#20283=CARTESIAN_POINT('Ctrl Pts',(4.30521122796165,5.2208663344921,46.9775113407527));
#20284=CARTESIAN_POINT('Ctrl Pts',(4.17044471281827,5.33199699307943,46.9857157756947));
#20285=CARTESIAN_POINT('Ctrl Pts',(4.03144611770919,5.43784551698511,46.9939202106367));
#20286=CARTESIAN_POINT('Ctrl Pts',(3.88867705369091,5.53809351420665,47.0021246455787));
#20287=CARTESIAN_POINT('Ctrl Pts',(3.74574858479657,5.63845344057532,47.0103382409571));
#20288=CARTESIAN_POINT('Ctrl Pts',(3.59904153553808,5.73320014918724,47.0185518363356));
#20289=CARTESIAN_POINT('Ctrl Pts',(3.44904507755022,5.82205951988011,47.026765431714));
#20290=CARTESIAN_POINT('Ctrl Pts',(3.33427144539633,5.89005254359641,47.0330502746181));
#20291=CARTESIAN_POINT('Ctrl Pts',(3.2175724536714,5.95459947399275,47.0393351175222));
#20292=CARTESIAN_POINT('Ctrl Pts',(3.09917575053261,6.01559628526638,47.0456199604263));
#20293=CARTESIAN_POINT('Ctrl Pts',(3.09917575053261,6.01559628526638,45.0457515827422));
#20294=CARTESIAN_POINT('Ctrl Pts',(2.93382384459261,6.10078395293761,45.0545010306546));
#20295=CARTESIAN_POINT('Ctrl Pts',(2.76495772122974,6.17915010267054,45.063250478567));
#20296=CARTESIAN_POINT('Ctrl Pts',(2.59315093316695,6.25042856433184,45.0719999264794));
#20297=CARTESIAN_POINT('Ctrl Pts',(2.42134553245605,6.32170645041456,45.0807493037394));
#20298=CARTESIAN_POINT('Ctrl Pts',(2.24659977927582,6.3858966531346,45.0894986809994));
#20299=CARTESIAN_POINT('Ctrl Pts',(2.06950718689915,6.44278115439076,45.0982480582594));
#20300=CARTESIAN_POINT('Ctrl Pts',(1.89241596572862,6.49966521519724,45.1069973677741));
#20301=CARTESIAN_POINT('Ctrl Pts',(1.71297821457202,6.54924360009545,45.1157466772887));
#20302=CARTESIAN_POINT('Ctrl Pts',(1.53180337335854,6.59134792173554,45.1244959868034));
#20303=CARTESIAN_POINT('Ctrl Pts',(1.3506298747779,6.63345193135303,45.1332452314795));
#20304=CARTESIAN_POINT('Ctrl Pts',(1.16771959102959,6.66808192368237,45.1419944761556));
#20305=CARTESIAN_POINT('Ctrl Pts',(0.9836937469069,6.69512028363167,45.1507437208318));
#20306=CARTESIAN_POINT('Ctrl Pts',(0.799669205419907,6.72215845218867,45.1594929035759));
#20307=CARTESIAN_POINT('Ctrl Pts',(0.614529402873492,6.74160505424579,45.1682420863201));
#20308=CARTESIAN_POINT('Ctrl Pts',(0.428903127363245,6.75339404354122,45.1769912690643));
#20309=CARTESIAN_POINT('Ctrl Pts',(0.243278104163816,6.76518295330331,45.1857403927829));
#20310=CARTESIAN_POINT('Ctrl Pts',(0.0571669005389931,6.76931433552276,
45.1944895165015));
#20311=CARTESIAN_POINT('Ctrl Pts',(-0.128798404777697,6.76577415902473,
45.2032386402201));
#20312=CARTESIAN_POINT('Ctrl Pts',(-0.314762517259329,6.7622340052344,45.2119877078193));
#20313=CARTESIAN_POINT('Ctrl Pts',(-0.500580446819786,6.75102239665087,
45.2207367754185));
#20314=CARTESIAN_POINT('Ctrl Pts',(-0.685621118842932,6.73217741012494,
45.2294858430178));
#20315=CARTESIAN_POINT('Ctrl Pts',(-0.870660665414716,6.71333253821769,
45.2382348574035));
#20316=CARTESIAN_POINT('Ctrl Pts',(-1.054922678855,6.6868544103061,45.2469838717893));
#20317=CARTESIAN_POINT('Ctrl Pts',(-1.23778137635256,6.65283295028177,45.2557328861751));
#20318=CARTESIAN_POINT('Ctrl Pts',(-1.4299992297885,6.61707018861865,45.2649296965425));
#20319=CARTESIAN_POINT('Ctrl Pts',(-1.62066601233698,6.57297172934412,45.2741265069099));
#20320=CARTESIAN_POINT('Ctrl Pts',(-1.80906628500387,6.52070304311294,45.2833233172773));
#20321=CARTESIAN_POINT('Ctrl Pts',(-1.98831342545531,6.4709737491503,45.292073315015));
#20322=CARTESIAN_POINT('Ctrl Pts',(-2.16550875896707,6.41384933989527,45.3008233127528));
#20323=CARTESIAN_POINT('Ctrl Pts',(-2.34005036714018,6.34952386240473,45.3095733104906));
#20324=CARTESIAN_POINT('Ctrl Pts',(-2.51458843547096,6.28519968948593,45.3183231307714));
#20325=CARTESIAN_POINT('Ctrl Pts',(-2.68647261718063,6.21367483971096,45.3270729510523));
#20326=CARTESIAN_POINT('Ctrl Pts',(-2.85511905908739,6.1351922674384,45.3358227713331));
#20327=CARTESIAN_POINT('Ctrl Pts',(-3.02376230488893,6.05671118252933,45.3445724257917));
#20328=CARTESIAN_POINT('Ctrl Pts',(-3.18916767379913,5.97127275992628,45.3533220802502));
#20329=CARTESIAN_POINT('Ctrl Pts',(-3.35077334102797,5.87916720437991,45.3620717347087));
#20330=CARTESIAN_POINT('Ctrl Pts',(-3.51237616037376,5.78706327195638,45.3708212349772));
#20331=CARTESIAN_POINT('Ctrl Pts',(-3.67017916302306,5.68829258362294,45.3795707352456));
#20332=CARTESIAN_POINT('Ctrl Pts',(-3.82364636566466,5.58319061741039,45.3883202355141));
#20333=CARTESIAN_POINT('Ctrl Pts',(-3.97711106778793,5.47809036367705,45.3970695932225));
#20334=CARTESIAN_POINT('Ctrl Pts',(-4.12623987481914,5.36665920043235,45.4058189509309));
#20335=CARTESIAN_POINT('Ctrl Pts',(-4.27052628213908,5.24927559512352,45.4145683086394));
#20336=CARTESIAN_POINT('Ctrl Pts',(-4.41481053024965,5.13189374643048,45.4233175354159));
#20337=CARTESIAN_POINT('Ctrl Pts',(-4.55425230136524,5.00855981477359,45.4320667621924));
#20338=CARTESIAN_POINT('Ctrl Pts',(-4.68837800630548,4.87969268192076,45.4408159889689));
#20339=CARTESIAN_POINT('Ctrl Pts',(-4.82250188228864,4.75082730631839,45.4495650964398));
#20340=CARTESIAN_POINT('Ctrl Pts',(-4.95130963052908,4.61642907903586,45.4583142039106));
#20341=CARTESIAN_POINT('Ctrl Pts',(-5.07436379033284,4.47695444731783,45.4670633113814));
#20342=CARTESIAN_POINT('Ctrl Pts',(-5.19741643562712,4.33748153220697,45.4758123111711));
#20343=CARTESIAN_POINT('Ctrl Pts',(-5.31471544462671,4.19293255254718,45.4845613109609));
#20344=CARTESIAN_POINT('Ctrl Pts',(-5.42586245275517,4.04379841779751,45.4933103107506));
#20345=CARTESIAN_POINT('Ctrl Pts',(-5.53702160019041,3.89464799484502,45.5020602660928));
#20346=CARTESIAN_POINT('Ctrl Pts',(-5.64202723081139,3.7409116444402,45.5108102214349));
#20347=CARTESIAN_POINT('Ctrl Pts',(-5.74052265232854,3.58311159163414,45.5195601767771));
#20348=CARTESIAN_POINT('Ctrl Pts',(-5.83901427066817,3.42531763191956,45.5283097942595));
#20349=CARTESIAN_POINT('Ctrl Pts',(-5.93099603115649,3.26346052695777,45.537059411742));
#20350=CARTESIAN_POINT('Ctrl Pts',(-6.01615550622674,3.09809004467232,45.5458090292244));
#20351=CARTESIAN_POINT('Ctrl Pts',(-6.10131214578726,2.93272506863981,45.5545583553755));
#20352=CARTESIAN_POINT('Ctrl Pts',(-6.1796468232868,2.76384720417045,45.5633076815266));
#20353=CARTESIAN_POINT('Ctrl Pts',(-6.25089348288503,2.59203002791741,45.5720570076777));
#20354=CARTESIAN_POINT('Ctrl Pts',(-6.32213814889273,2.42021765937177,45.5808060890093));
#20355=CARTESIAN_POINT('Ctrl Pts',(-6.38629508412533,2.24546640832067,45.5895551703409));
#20356=CARTESIAN_POINT('Ctrl Pts',(-6.44314639819764,2.06836976660191,45.5983042516724));
#20357=CARTESIAN_POINT('Ctrl Pts',(-6.50000285283656,1.89125711158428,45.6070541241068));
#20358=CARTESIAN_POINT('Ctrl Pts',(-6.54955227673208,1.71179891440411,45.6158039965412));
#20359=CARTESIAN_POINT('Ctrl Pts',(-6.59162635926348,1.53060476278591,45.6245538689756));
#20360=CARTESIAN_POINT('Ctrl Pts',(-6.63369752055166,1.34942319164848,45.6333031338981));
#20361=CARTESIAN_POINT('Ctrl Pts',(-6.66829431424229,1.16650618642847,45.6420523988206));
#20362=CARTESIAN_POINT('Ctrl Pts',(-6.69529923745398,0.982474997619904,
45.6508016637431));
#20363=CARTESIAN_POINT('Ctrl Pts',(-6.72230554731428,0.798434359179042,
45.6595513779228));
#20364=CARTESIAN_POINT('Ctrl Pts',(-6.74171916496692,0.613279706241595,
45.6683010921025));
#20365=CARTESIAN_POINT('Ctrl Pts',(-6.75347414817267,0.427639953656586,
45.6770508062822));
#20366=CARTESIAN_POINT('Ctrl Pts',(-6.76248837758742,0.285283364199395,
45.6837604654581));
#20367=CARTESIAN_POINT('Ctrl Pts',(-6.76699999999997,0.142641701105548,
45.6904701246341));
#20368=CARTESIAN_POINT('Ctrl Pts',(-6.767,1.61040289520569E-12,45.69717978381));
#20369=CARTESIAN_POINT('',(-6.76699973265636,-0.0019021642129279,45.3028202162182));
#20370=CARTESIAN_POINT('Ctrl Pts',(3.09917575053253,6.01559628526642,44.6513725725535));
#20371=CARTESIAN_POINT('Ctrl Pts',(2.9437420728611,6.0956741797613,44.6595737570002));
#20372=CARTESIAN_POINT('Ctrl Pts',(2.7852141545089,6.16971810297613,44.6677749414468));
#20373=CARTESIAN_POINT('Ctrl Pts',(2.62410422784775,6.23749677365781,44.6759761258935));
#20374=CARTESIAN_POINT('Ctrl Pts',(2.46295268942282,6.30529295033736,44.6841794285569));
#20375=CARTESIAN_POINT('Ctrl Pts',(2.2992181444318,6.36682051187649,44.6923827312203));
#20376=CARTESIAN_POINT('Ctrl Pts',(2.13343179158499,6.42189674400441,44.7005860338837));
#20377=CARTESIAN_POINT('Ctrl Pts',(1.96757257393781,6.47699718270055,44.7087929419827));
#20378=CARTESIAN_POINT('Ctrl Pts',(1.79966009172503,6.5256405308075,44.7169998500816));
#20379=CARTESIAN_POINT('Ctrl Pts',(1.63023969950547,6.56769423178,44.7252067581806));
#20380=CARTESIAN_POINT('Ctrl Pts',(1.46062126562505,6.60979709085371,44.7334232596331));
#20381=CARTESIAN_POINT('Ctrl Pts',(1.28949174912264,6.64529483190286,44.7416397610855));
#20382=CARTESIAN_POINT('Ctrl Pts',(1.11740662978061,6.67410603929263,44.749856262538));
#20383=CARTESIAN_POINT('Ctrl Pts',(0.94520687225507,6.70293643988453,44.7580782375887));
#20384=CARTESIAN_POINT('Ctrl Pts',(0.772050597385722,6.72507138328482,44.7663002126393));
#20385=CARTESIAN_POINT('Ctrl Pts',(0.598497247238427,6.74048144015307,44.77452218769));
#20386=CARTESIAN_POINT('Ctrl Pts',(0.424697225229204,6.75591339937825,44.7827558486568));
#20387=CARTESIAN_POINT('Ctrl Pts',(0.250499357361747,6.76460136413436,44.7909895096236));
#20388=CARTESIAN_POINT('Ctrl Pts',(0.0764629357328109,6.76656799415029,
44.7992231705904));
#20389=CARTESIAN_POINT('Ctrl Pts',(-0.00117737115148329,6.7674453378496,
44.8028963325542));
#20390=CARTESIAN_POINT('Ctrl Pts',(-0.0787856135802052,6.7669857002162,
44.806569494518));
#20391=CARTESIAN_POINT('Ctrl Pts',(-0.156312583787009,6.76519440786071,
44.8102426564818));
#20392=CARTESIAN_POINT('Ctrl Pts',(-0.328444383897077,6.76121723221653,
44.8183981148886));
#20393=CARTESIAN_POINT('Ctrl Pts',(-0.500705055019613,6.75065976822586,
44.8265535732954));
#20394=CARTESIAN_POINT('Ctrl Pts',(-0.672545883368081,6.73349619698153,
44.8347090317022));
#20395=CARTESIAN_POINT('Ctrl Pts',(-0.844177558840259,6.71635351605952,
44.842854563844));
#20396=CARTESIAN_POINT('Ctrl Pts',(-1.01539004901787,6.69262076879519,44.8510000959859));
#20397=CARTESIAN_POINT('Ctrl Pts',(-1.18563345689058,6.66232409192931,44.8591456281278));
#20398=CARTESIAN_POINT('Ctrl Pts',(-1.35570545493074,6.63205791931833,44.8672829589283));
#20399=CARTESIAN_POINT('Ctrl Pts',(-1.52480995599806,6.59524103781933,44.8754202897289));
#20400=CARTESIAN_POINT('Ctrl Pts',(-1.69240100768474,6.55195145198647,44.8835576205294));
#20401=CARTESIAN_POINT('Ctrl Pts',(-1.8598585398467,6.5086963548979,44.8916884683314));
#20402=CARTESIAN_POINT('Ctrl Pts',(-2.0258046712114,6.45897891227745,44.8998193161334));
#20403=CARTESIAN_POINT('Ctrl Pts',(-2.18970248843383,6.40292839348893,44.9079501639354));
#20404=CARTESIAN_POINT('Ctrl Pts',(-2.35350415809935,6.34691075567793,44.9160762419292));
#20405=CARTESIAN_POINT('Ctrl Pts',(-2.51525956162403,6.28456755838002,44.924202319923));
#20406=CARTESIAN_POINT('Ctrl Pts',(-2.67444583368734,6.216078223661,44.9323283979168));
#20407=CARTESIAN_POINT('Ctrl Pts',(-2.83419655119693,6.14734603827024,44.940483289499));
#20408=CARTESIAN_POINT('Ctrl Pts',(-2.99135952598779,6.07242414824676,44.9486381810812));
#20409=CARTESIAN_POINT('Ctrl Pts',(-3.14542489990301,5.99154330695107,44.9567930726634));
#20410=CARTESIAN_POINT('Ctrl Pts',(-3.29888947272746,5.91097787265721,44.9649161630197));
#20411=CARTESIAN_POINT('Ctrl Pts',(-3.44928024226919,5.82450006568852,44.973039253376));
#20412=CARTESIAN_POINT('Ctrl Pts',(-3.59611672016378,5.73238462901422,44.9811623437323));
#20413=CARTESIAN_POINT('Ctrl Pts',(-3.74296472832917,5.64026195901517,44.9892860719508));
#20414=CARTESIAN_POINT('Ctrl Pts',(-3.88625757899098,5.5425009718914,44.9974098001692));
#20415=CARTESIAN_POINT('Ctrl Pts',(-4.02554283308931,5.43942036424501,45.0055335283877));
#20416=CARTESIAN_POINT('Ctrl Pts',(-4.16486552335506,5.3363120512761,45.013659440048));
#20417=CARTESIAN_POINT('Ctrl Pts',(-4.3001781783461,5.22788148837119,45.0217853517083));
#20418=CARTESIAN_POINT('Ctrl Pts',(-4.4310606155373,5.11448832449877,45.0299112633685));
#20419=CARTESIAN_POINT('Ctrl Pts',(-4.56278005952017,5.00036999955564,45.0380891410786));
#20420=CARTESIAN_POINT('Ctrl Pts',(-4.69001214174115,4.88122562657827,45.0462670187887));
#20421=CARTESIAN_POINT('Ctrl Pts',(-4.81236605622012,4.75745961001672,45.0544448964988));
#20422=CARTESIAN_POINT('Ctrl Pts',(-4.93413600200223,4.634284301809,45.0625837429722));
#20423=CARTESIAN_POINT('Ctrl Pts',(-5.0510740412375,4.50653168095525,45.0707225894456));
#20424=CARTESIAN_POINT('Ctrl Pts',(-5.16283553362158,4.37463349925161,45.0788614359191));
#20425=CARTESIAN_POINT('Ctrl Pts',(-5.27540098316419,4.24178650695932,45.0870588292475));
#20426=CARTESIAN_POINT('Ctrl Pts',(-5.38271489711704,4.10473438413423,45.0952562225759));
#20427=CARTESIAN_POINT('Ctrl Pts',(-5.48446984907871,3.96394746112339,45.1034536159043));
#20428=CARTESIAN_POINT('Ctrl Pts',(-5.58622480104038,3.82316053811254,45.1116510092327));
#20429=CARTESIAN_POINT('Ctrl Pts',(-5.68242063563078,3.67863915864375,45.1198484025611));
#20430=CARTESIAN_POINT('Ctrl Pts',(-5.77279741327199,3.53087793973684,45.1280457958895));
#20431=CARTESIAN_POINT('Ctrl Pts',(-5.86662260470627,3.37747874790526,45.1365559687278));
#20432=CARTESIAN_POINT('Ctrl Pts',(-5.95443936757663,3.22015832143925,45.1450661415661));
#20433=CARTESIAN_POINT('Ctrl Pts',(-6.03591757032215,3.05940976076699,45.1535763144045));
#20434=CARTESIAN_POINT('Ctrl Pts',(-6.11728481284174,2.89888011381656,45.1620748977542));
#20435=CARTESIAN_POINT('Ctrl Pts',(-6.19233055395715,2.73493192385575,45.170573481104));
#20436=CARTESIAN_POINT('Ctrl Pts',(-6.26076857721881,2.56808602319111,45.1790720644537));
#20437=CARTESIAN_POINT('Ctrl Pts',(-6.32912168482866,2.40144713944094,45.1875601030404));
#20438=CARTESIAN_POINT('Ctrl Pts',(-6.39088329399675,2.23191800921721,45.196048141627));
#20439=CARTESIAN_POINT('Ctrl Pts',(-6.44581345317645,2.06004318567584,45.2045361802136));
#20440=CARTESIAN_POINT('Ctrl Pts',(-6.50066071850216,1.8884277345219,45.2130114096942));
#20441=CARTESIAN_POINT('Ctrl Pts',(-6.5486969998166,1.71447395817075,45.2214866391749));
#20442=CARTESIAN_POINT('Ctrl Pts',(-6.58973080093811,1.53874525869867,45.2299618686555));
#20443=CARTESIAN_POINT('Ctrl Pts',(-6.6307281949429,1.36317247398701,45.2384295785142));
#20444=CARTESIAN_POINT('Ctrl Pts',(-6.66473541712651,1.18582821850764,45.246897288373));
#20445=CARTESIAN_POINT('Ctrl Pts',(-6.69161067495236,1.00729120658509,45.2553649982317));
#20446=CARTESIAN_POINT('Ctrl Pts',(-6.71845848019703,0.82893656693392,45.2638240584807));
#20447=CARTESIAN_POINT('Ctrl Pts',(-6.73818880400721,0.649391920275191,
45.2722831187297));
#20448=CARTESIAN_POINT('Ctrl Pts',(-6.7507108406708,0.469246359229067,45.2807421789787));
#20449=CARTESIAN_POINT('Ctrl Pts',(-6.76160495827098,0.312520502252987,
45.2881015247158));
#20450=CARTESIAN_POINT('Ctrl Pts',(-6.76704393253596,0.155340131828287,
45.2954608704528));
#20451=CARTESIAN_POINT('Ctrl Pts',(-6.76699973265654,-0.00190216360935057,
45.3028202161899));
#20452=CARTESIAN_POINT('Ctrl Pts',(-6.76699973265637,-0.00190216421283039,
45.3028202162181));
#20453=CARTESIAN_POINT('Ctrl Pts',(-6.7669471825227,-0.188850661127842,
45.3115698889445));
#20454=CARTESIAN_POINT('Ctrl Pts',(-6.75914331389005,-0.375595569033888,
45.3203195616709));
#20455=CARTESIAN_POINT('Ctrl Pts',(-6.7436639021329,-0.561503495153537,
45.3290692343973));
#20456=CARTESIAN_POINT('Ctrl Pts',(-6.72815474027868,-0.747768720306037,
45.3378357232415));
#20457=CARTESIAN_POINT('Ctrl Pts',(-6.7049405837135,-0.933193474538999,
45.3466022120858));
#20458=CARTESIAN_POINT('Ctrl Pts',(-6.67414848370708,-1.11715308594232,
45.3553687009301));
#20459=CARTESIAN_POINT('Ctrl Pts',(-6.64326641890751,-1.30165016924219,
45.3641608026866));
#20460=CARTESIAN_POINT('Ctrl Pts',(-6.60476215828831,-1.48467327101841,
45.3729529044431));
#20461=CARTESIAN_POINT('Ctrl Pts',(-6.55881366539612,-1.66560868832183,
45.3817450061997));
#20462=CARTESIAN_POINT('Ctrl Pts',(-6.51279361530138,-1.84682588270842,
45.3905508002052));
#20463=CARTESIAN_POINT('Ctrl Pts',(-6.45930625285953,-2.02594863342554,
45.3993565942107));
#20464=CARTESIAN_POINT('Ctrl Pts',(-6.3985786005201,-2.202380732972,45.4081623882163));
#20465=CARTESIAN_POINT('Ctrl Pts',(-6.33770714788192,-2.37923061564765,
45.4169890339386));
#20466=CARTESIAN_POINT('Ctrl Pts',(-6.26956121274525,-2.55337684513432,
45.4258156796609));
#20467=CARTESIAN_POINT('Ctrl Pts',(-6.19441589284408,-2.72424315113036,
45.4346423253833));
#20468=CARTESIAN_POINT('Ctrl Pts',(-6.16261354068299,-2.79655571088655,
45.4383778620213));
#20469=CARTESIAN_POINT('Ctrl Pts',(-6.12955809997296,-2.86828112775628,
45.4421133986592));
#20470=CARTESIAN_POINT('Ctrl Pts',(-6.09527282366468,-2.93937717979418,
45.4458489352972));
#20471=CARTESIAN_POINT('Ctrl Pts',(-6.01977160329613,-3.09594114165299,
45.454075136316));
#20472=CARTESIAN_POINT('Ctrl Pts',(-5.93812869545449,-3.24981306424306,
45.4623013373349));
#20473=CARTESIAN_POINT('Ctrl Pts',(-5.85055888297444,-3.40047787183639,
45.4705275383537));
#20474=CARTESIAN_POINT('Ctrl Pts',(-5.76308743672242,-3.55097343927262,
45.4787444989695));
#20475=CARTESIAN_POINT('Ctrl Pts',(-5.66970252156123,-3.69826875805281,
45.4869614595852));
#20476=CARTESIAN_POINT('Ctrl Pts',(-5.57066635348732,-3.84187003659993,
45.495178420201));
#20477=CARTESIAN_POINT('Ctrl Pts',(-5.47172155432969,-3.98533883129341,
45.5033878000026));
#20478=CARTESIAN_POINT('Ctrl Pts',(-5.36713608794945,-4.12512007963921,
45.5115971798042));
#20479=CARTESIAN_POINT('Ctrl Pts',(-5.25721736041371,-4.26074578276676,
45.5198065596057));
#20480=CARTESIAN_POINT('Ctrl Pts',(-5.14737798735698,-4.39627357257915,
45.5280100127461));
#20481=CARTESIAN_POINT('Ctrl Pts',(-5.03221324714273,-4.52765151525559,
45.5362134658865));
#20482=CARTESIAN_POINT('Ctrl Pts',(-4.91207305886323,-4.65444167053258,
45.5444169190269));
#20483=CARTESIAN_POINT('Ctrl Pts',(-4.79199550449857,-4.78116572499931,
45.5526160953771));
#20484=CARTESIAN_POINT('Ctrl Pts',(-4.66694791567108,-4.90330649724465,
45.5608152717272));
#20485=CARTESIAN_POINT('Ctrl Pts',(-4.53731963983386,-5.02046008708146,
45.5690144480774));
#20486=CARTESIAN_POINT('Ctrl Pts',(-4.40771575551302,-5.13759163270232,
45.5772120816287));
#20487=CARTESIAN_POINT('Ctrl Pts',(-4.27353316267407,-5.24973762029901,
45.5854097151801));
#20488=CARTESIAN_POINT('Ctrl Pts',(-4.13519734668707,-5.35653170474629,
45.5936073487315));
#20489=CARTESIAN_POINT('Ctrl Pts',(-3.99687149427392,-5.46331809739851,
45.601804391852));
#20490=CARTESIAN_POINT('Ctrl Pts',(-3.85439329783237,-5.56475313470061,
45.6100014349726));
#20491=CARTESIAN_POINT('Ctrl Pts',(-3.708220487231,-5.66051144492088,45.6181984780932));
#20492=CARTESIAN_POINT('Ctrl Pts',(-3.56203163799523,-5.75628026210563,
45.6263964206244));
#20493=CARTESIAN_POINT('Ctrl Pts',(-3.41214766704513,-5.84637091467463,
45.6345943631556));
#20494=CARTESIAN_POINT('Ctrl Pts',(-3.25905441604444,-5.93050194446147,
45.6427923056867));
#20495=CARTESIAN_POINT('Ctrl Pts',(-3.10591654252586,-6.01465749615478,
45.6509926376952));
#20496=CARTESIAN_POINT('Ctrl Pts',(-2.94956783998034,-6.09284979233589,
45.6591929697036));
#20497=CARTESIAN_POINT('Ctrl Pts',(-2.79051785633367,-6.16484380122343,
45.667393301712));
#20498=CARTESIAN_POINT('Ctrl Pts',(-2.63130209961605,-6.23691284732676,
45.6756021806828));
#20499=CARTESIAN_POINT('Ctrl Pts',(-2.46937976411834,-6.30277055134834,
45.6838110596535));
#20500=CARTESIAN_POINT('Ctrl Pts',(-2.3052803772165,-6.36223006361925,45.6920199386243));
#20501=CARTESIAN_POINT('Ctrl Pts',(-2.14109289795754,-6.42172149513548,
45.7002332243117));
#20502=CARTESIAN_POINT('Ctrl Pts',(-1.97472637884107,-6.47480777878317,
45.708446509999));
#20503=CARTESIAN_POINT('Ctrl Pts',(-1.80672444073288,-6.52135229804819,
45.7166597956864));
#20504=CARTESIAN_POINT('Ctrl Pts',(-1.63847673649504,-6.56796490620842,
45.7248850963985));
#20505=CARTESIAN_POINT('Ctrl Pts',(-1.46858918126387,-6.60801654307638,
45.7331103971106));
#20506=CARTESIAN_POINT('Ctrl Pts',(-1.29761575748285,-6.64142171119499,
45.7413356978227));
#20507=CARTESIAN_POINT('Ctrl Pts',(-1.14299091982237,-6.67163265616605,
45.7487744901168));
#20508=CARTESIAN_POINT('Ctrl Pts',(-0.987478236060209,-6.69640808578942,
45.7562132824109));
#20509=CARTESIAN_POINT('Ctrl Pts',(-0.831489413486529,-6.71572143222602,
45.7636520747049));
#20510=CARTESIAN_POINT('Ctrl Pts',(-0.660533215975414,-6.73688792488581,
45.7718046309182));
#20511=CARTESIAN_POINT('Ctrl Pts',(-0.488500868444045,-6.75155544123094,
45.7799571871314));
#20512=CARTESIAN_POINT('Ctrl Pts',(-0.315932268866136,-6.75962098060898,
45.7881097433447));
#20513=CARTESIAN_POINT('Ctrl Pts',(-0.14356359417106,-6.76767717586521,
45.796252854625));
#20514=CARTESIAN_POINT('Ctrl Pts',(0.0293397344602783,-6.76914660243042,
45.8043959659054));
#20515=CARTESIAN_POINT('Ctrl Pts',(0.202229370063513,-6.76397754888969,
45.8125390771857));
#20516=CARTESIAN_POINT('Ctrl Pts',(0.374955056748411,-6.75881339709297,
45.820674466463));
#20517=CARTESIAN_POINT('Ctrl Pts',(0.547666713371004,-6.74702330894105,
45.8288098557404));
#20518=CARTESIAN_POINT('Ctrl Pts',(0.719812633999018,-6.7286074912968,45.8369452450177));
#20519=CARTESIAN_POINT('Ctrl Pts',(0.891831482975453,-6.71020526751731,
45.8450746290563));
#20520=CARTESIAN_POINT('Ctrl Pts',(1.06328506552707,-6.68518709153682,45.8532040130949));
#20521=CARTESIAN_POINT('Ctrl Pts',(1.23362344560039,-6.6536052027803,45.8613333971335));
#20522=CARTESIAN_POINT('Ctrl Pts',(1.40387186748705,-6.62203999288054,45.8694584879256));
#20523=CARTESIAN_POINT('Ctrl Pts',(1.5730059011896,-6.58391804016423,45.8775835787178));
#20524=CARTESIAN_POINT('Ctrl Pts',(1.74048249575696,-6.53934321487744,45.8857086695099));
#20525=CARTESIAN_POINT('Ctrl Pts',(1.90859838479267,-6.49459823781926,45.893864775535));
#20526=CARTESIAN_POINT('Ctrl Pts',(2.07504378685537,-6.44335107430534,45.9020208815601));
#20527=CARTESIAN_POINT('Ctrl Pts',(2.23928099763713,-6.38575834287685,45.9101769875852));
#20528=CARTESIAN_POINT('Ctrl Pts',(2.40285718334811,-6.32839741177661,45.9183002667586));
#20529=CARTESIAN_POINT('Ctrl Pts',(2.56424257946716,-6.26474203966973,45.926423545932));
#20530=CARTESIAN_POINT('Ctrl Pts',(2.72292270399433,-6.19499644455687,45.9345468251054));
#20531=CARTESIAN_POINT('Ctrl Pts',(2.881623958121,-6.12524156222864,45.9426711859621));
#20532=CARTESIAN_POINT('Ctrl Pts',(3.03761888820817,-6.04939498882009,45.9507955468188));
#20533=CARTESIAN_POINT('Ctrl Pts',(3.19041463624472,-5.96770839173929,45.9589199076755));
#20534=CARTESIAN_POINT('Ctrl Pts',(3.3432598005035,-5.88599537610242,45.9670468960609));
#20535=CARTESIAN_POINT('Ctrl Pts',(3.49290339993014,-5.79843874809302,45.9751738844463));
#20536=CARTESIAN_POINT('Ctrl Pts',(3.6388787853827,-5.70533523864214,45.9833008728317));
#20537=CARTESIAN_POINT('Ctrl Pts',(3.78579788508253,-5.61162982560273,45.9914804012718));
#20538=CARTESIAN_POINT('Ctrl Pts',(3.9290008603406,-5.51230576465283,45.9996599297119));
#20539=CARTESIAN_POINT('Ctrl Pts',(4.06804386164321,-5.40770821510804,46.0078394581519));
#20540=CARTESIAN_POINT('Ctrl Pts',(4.20643206462738,-5.30360324914469,46.0159804665556));
#20541=CARTESIAN_POINT('Ctrl Pts',(4.34069914794465,-5.19427463737249,46.0241214749593));
#20542=CARTESIAN_POINT('Ctrl Pts',(4.47044314019526,-5.0801010944942,46.032262483363));
#20543=CARTESIAN_POINT('Ctrl Pts',(4.60110797843696,-4.96511721544986,46.0404612718212));
#20544=CARTESIAN_POINT('Ctrl Pts',(4.72718501160129,-4.845219639765,46.0486600602795));
#20545=CARTESIAN_POINT('Ctrl Pts',(4.84830387431723,-4.72083028102902,46.0568588487377));
#20546=CARTESIAN_POINT('Ctrl Pts',(4.96942273703317,-4.59644092229304,46.0650576371959));
#20547=CARTESIAN_POINT('Ctrl Pts',(5.08558322879314,-4.46756009973438,46.0732564256542));
#20548=CARTESIAN_POINT('Ctrl Pts',(5.19645862884004,-4.33464032172843,46.0814552141124));
#20549=CARTESIAN_POINT('Ctrl Pts',(5.30779736280562,-4.20116508920697,46.0896882642445));
#20550=CARTESIAN_POINT('Ctrl Pts',(5.41415293398444,-4.06320223827321,46.0979213143765));
#20551=CARTESIAN_POINT('Ctrl Pts',(5.51514317079271,-3.92115860501186,46.1061543645085));
#20552=CARTESIAN_POINT('Ctrl Pts',(5.61601314375281,-3.77928412388327,46.1143776103433));
#20553=CARTESIAN_POINT('Ctrl Pts',(5.71153029948196,-3.63333882611836,46.1226008561782));
#20554=CARTESIAN_POINT('Ctrl Pts',(5.80135125192717,-3.48376414984756,46.1308241020131));
#20555=CARTESIAN_POINT('Ctrl Pts',(5.89108321928234,-3.33433765633003,46.1390392011266));
#20556=CARTESIAN_POINT('Ctrl Pts',(5.97513003871564,-3.18128924995496,46.1472543002401));
#20557=CARTESIAN_POINT('Ctrl Pts',(6.0531903082959,-3.02509108814142,46.1554693993536));
#20558=CARTESIAN_POINT('Ctrl Pts',(6.13118886231285,-2.86901641882408,46.1636780034925));
#20559=CARTESIAN_POINT('Ctrl Pts',(6.20321013436888,-2.7097972730889,46.1718866076314));
#20560=CARTESIAN_POINT('Ctrl Pts',(6.26899750750128,-2.54793234818798,46.1800952117703));
#20561=CARTESIAN_POINT('Ctrl Pts',(6.33474602750618,-2.38616301850946,46.1882989680192));
#20562=CARTESIAN_POINT('Ctrl Pts',(6.39426784844422,-2.2217513534322,46.1965027242682));
#20563=CARTESIAN_POINT('Ctrl Pts',(6.44735351411134,-2.05521815486243,46.2047064805171));
#20564=CARTESIAN_POINT('Ctrl Pts',(6.50042347306808,-1.88873422926848,46.2129078094814));
#20565=CARTESIAN_POINT('Ctrl Pts',(6.54706095771878,-1.72013036021124,46.2211091384457));
#20566=CARTESIAN_POINT('Ctrl Pts',(6.58710555702563,-1.54994496050733,46.22931046741));
#20567=CARTESIAN_POINT('Ctrl Pts',(6.62714463379993,-1.37978303099479,46.2375106653327));
#20568=CARTESIAN_POINT('Ctrl Pts',(6.66059255326884,-1.20804035368517,46.2457108632554));
#20569=CARTESIAN_POINT('Ctrl Pts',(6.68733945682799,-1.03526807598394,46.2539110611781));
#20570=CARTESIAN_POINT('Ctrl Pts',(6.71408751881694,-0.862488315377161,
46.262111614258));
#20571=CARTESIAN_POINT('Ctrl Pts',(6.73413393181892,-0.68867921961648,46.2703121673378));
#20572=CARTESIAN_POINT('Ctrl Pts',(6.74742039178061,-0.514399705076941,
46.2785127204177));
#20573=CARTESIAN_POINT('Ctrl Pts',(6.76070983495631,-0.34008105949039,46.2867151147709));
#20574=CARTESIAN_POINT('Ctrl Pts',(6.76723627480314,-0.165292141927449,
46.2949175091241));
#20575=CARTESIAN_POINT('Ctrl Pts',(6.76699346374685,0.00940540309585271,
46.3031199034773));
#20576=CARTESIAN_POINT('Ctrl Pts',(6.76675042561955,0.18426632103387,46.3113299685111));
#20577=CARTESIAN_POINT('Ctrl Pts',(6.75972548939747,0.359035336963717,46.3195400335449));
#20578=CARTESIAN_POINT('Ctrl Pts',(6.74596454714927,0.533152256494463,46.3277500985788));
#20579=CARTESIAN_POINT('Ctrl Pts',(6.73219701915824,0.707352505294048,46.3359640928041));
#20580=CARTESIAN_POINT('Ctrl Pts',(6.71168709957096,0.880899679843116,46.3441780870294));
#20581=CARTESIAN_POINT('Ctrl Pts',(6.68453229939796,1.05324115866476,46.3523920812547));
#20582=CARTESIAN_POINT('Ctrl Pts',(6.65734047818814,1.2258175963221,46.3606172738899));
#20583=CARTESIAN_POINT('Ctrl Pts',(6.62348574094907,1.39718470157754,46.3688424665251));
#20584=CARTESIAN_POINT('Ctrl Pts',(6.58311649814029,1.56680125475861,46.3770676591603));
#20585=CARTESIAN_POINT('Ctrl Pts',(6.54681252454595,1.71933705774644,46.3844645572802));
#20586=CARTESIAN_POINT('Ctrl Pts',(6.50524075859181,1.87045713637758,46.3918614554002));
#20587=CARTESIAN_POINT('Ctrl Pts',(6.45854278735461,2.01978069698413,46.3992583535202));
#20588=CARTESIAN_POINT('Ctrl Pts',(6.40395921895036,2.19431960239687,46.4079043200111));
#20589=CARTESIAN_POINT('Ctrl Pts',(6.3422476711174,2.366800036713,46.416550286502));
#20590=CARTESIAN_POINT('Ctrl Pts',(6.27357789492636,2.53663347693185,46.4251962529929));
#20591=CARTESIAN_POINT('Ctrl Pts',(6.20499595671444,2.70624967709252,46.4338311601173));
#20592=CARTESIAN_POINT('Ctrl Pts',(6.12947365207117,2.87322535340952,46.4424660672416));
#20593=CARTESIAN_POINT('Ctrl Pts',(6.0472301950042,3.03698797637222,46.451100974366));
#20594=CARTESIAN_POINT('Ctrl Pts',(5.96225632154287,3.20618738624136,46.4600225534375));
#20595=CARTESIAN_POINT('Ctrl Pts',(5.87010742063523,3.37195642021525,46.468944132509));
#20596=CARTESIAN_POINT('Ctrl Pts',(5.77108014181708,3.53368405445713,46.4778657115805));
#20597=CARTESIAN_POINT('Ctrl Pts',(5.67549955778911,3.68978267615799,46.4864767705563));
#20598=CARTESIAN_POINT('Ctrl Pts',(5.57351148267702,3.8421161671724,46.495087829532));
#20599=CARTESIAN_POINT('Ctrl Pts',(5.46543034541433,3.99015790908383,46.5036988885077));
#20600=CARTESIAN_POINT('Ctrl Pts',(5.35745113365368,4.13806004079822,46.5123018268572));
#20601=CARTESIAN_POINT('Ctrl Pts',(5.24339049506426,4.28167824720971,46.5209047652068));
#20602=CARTESIAN_POINT('Ctrl Pts',(5.123606713071,4.42051391240586,46.5295077035563));
#20603=CARTESIAN_POINT('Ctrl Pts',(5.00395706120337,4.55919411377457,46.5381010086051));
#20604=CARTESIAN_POINT('Ctrl Pts',(4.87859724969166,4.69310222727563,46.5466943136539));
#20605=CARTESIAN_POINT('Ctrl Pts',(4.74792660553026,4.82177166075893,46.5552876187026));
#20606=CARTESIAN_POINT('Ctrl Pts',(4.73336775691013,4.83610754175304,46.5562450535432));
#20607=CARTESIAN_POINT('Ctrl Pts',(4.71874302327827,4.85037842513139,46.5572024883837));
#20608=CARTESIAN_POINT('Ctrl Pts',(4.70405298792322,4.86458369100693,46.5581599232242));
#20609=CARTESIAN_POINT('Ctrl Pts',(4.57214264457756,4.99214100817269,46.5667572856872));
#20610=CARTESIAN_POINT('Ctrl Pts',(4.43511836880952,5.1142549251199,46.5753546481503));
#20611=CARTESIAN_POINT('Ctrl Pts',(4.29345710661388,5.23053678637927,46.5839520106134));
#20612=CARTESIAN_POINT('Ctrl Pts',(4.15168870009091,5.34690659646538,46.5925558756206));
#20613=CARTESIAN_POINT('Ctrl Pts',(4.00527654830392,5.45743535961786,46.6011597406278));
#20614=CARTESIAN_POINT('Ctrl Pts',(3.85472814895607,5.56177668534487,46.6097636056351));
#20615=CARTESIAN_POINT('Ctrl Pts',(3.70396633532926,5.66626592316454,46.6183796673024));
#20616=CARTESIAN_POINT('Ctrl Pts',(3.54905680859,5.76455002212831,46.6269957289696));
#20617=CARTESIAN_POINT('Ctrl Pts',(3.39053480736998,5.85632672585919,46.6356117906369));
#20618=CARTESIAN_POINT('Ctrl Pts',(3.29469437704921,5.91181377946244,46.6408209543587));
#20619=CARTESIAN_POINT('Ctrl Pts',(3.19753396979732,5.96492310283268,46.6460301180806));
#20620=CARTESIAN_POINT('Ctrl Pts',(3.09917575053265,6.01559628526636,46.6512392818024));
#20621=CARTESIAN_POINT('Origin',(0.,0.,-3.69717978381041));
#20622=CARTESIAN_POINT('',(3.0991757505326,6.01559628526639,49.0457515827422));
#20623=CARTESIAN_POINT('',(3.09917575053255,6.01559628526641,48.6513920151221));
#20624=CARTESIAN_POINT('',(3.09917575053259,6.01559628526639,-3.69717978381041));
#20625=CARTESIAN_POINT('',(-6.76699998408371,-0.000464124033430669,47.6972016155329));
#20626=CARTESIAN_POINT('Ctrl Pts',(-6.76699998408371,-0.000464124033430669,
47.6972016155329));
#20627=CARTESIAN_POINT('Ctrl Pts',(-6.76698722651986,-0.186471372351812,
47.7059511273078));
#20628=CARTESIAN_POINT('Ctrl Pts',(-6.75930084199275,-0.372477951060072,
47.7147006390827));
#20629=CARTESIAN_POINT('Ctrl Pts',(-6.74396693763965,-0.557852080773529,
47.7234501508577));
#20630=CARTESIAN_POINT('Ctrl Pts',(-6.72863309805146,-0.743225427533112,
47.7321996256778));
#20631=CARTESIAN_POINT('Ctrl Pts',(-6.70565182690122,-0.927966045015493,
47.7409491004979));
#20632=CARTESIAN_POINT('Ctrl Pts',(-6.67510118041105,-1.11144645902309,
47.749698575318));
#20633=CARTESIAN_POINT('Ctrl Pts',(-6.64455066041847,-1.29492611331422,
47.7584480139102));
#20634=CARTESIAN_POINT('Ctrl Pts',(-6.60643087487681,-1.47714529186708,
47.7671974525023));
#20635=CARTESIAN_POINT('Ctrl Pts',(-6.56087129712167,-1.65748508970822,
47.7759468910945));
#20636=CARTESIAN_POINT('Ctrl Pts',(-6.51531190422601,-1.8378241558147,47.7846962941855));
#20637=CARTESIAN_POINT('Ctrl Pts',(-6.46231284972204,-2.01628357860759,
47.7934456972765));
#20638=CARTESIAN_POINT('Ctrl Pts',(-6.40205414272168,-2.19225722798676,
47.8021951003675));
#20639=CARTESIAN_POINT('Ctrl Pts',(-6.34179567521861,-2.36823017796141,
47.8109444686842));
#20640=CARTESIAN_POINT('Ctrl Pts',(-6.27427770580163,-2.5417171031626,47.8196938370009));
#20641=CARTESIAN_POINT('Ctrl Pts',(-6.19972955465985,-2.71212876705314,
47.8284432053175));
#20642=CARTESIAN_POINT('Ctrl Pts',(-6.12518169361748,-2.88253976779748,
47.8371925395866));
#20643=CARTESIAN_POINT('Ctrl Pts',(-6.04360382045395,-3.0498752686225,47.8459418738556));
#20644=CARTESIAN_POINT('Ctrl Pts',(-5.95527300671056,-3.21356693030418,
47.8546912081246));
#20645=CARTESIAN_POINT('Ctrl Pts',(-5.86694252936545,-3.377257968584,47.8634405090728));
#20646=CARTESIAN_POINT('Ctrl Pts',(-5.77185929899606,-3.53730494329142,
47.872189810021));
#20647=CARTESIAN_POINT('Ctrl Pts',(-5.67034625435664,-3.69316427412912,
47.8809391109691));
#20648=CARTESIAN_POINT('Ctrl Pts',(-5.56883358788884,-3.84902302433627,
47.8896883793231));
#20649=CARTESIAN_POINT('Ctrl Pts',(-5.46089131148301,-4.00069392176395,
47.898437647677));
#20650=CARTESIAN_POINT('Ctrl Pts',(-5.34688603536768,-4.14766183828794,
47.907186916031));
#20651=CARTESIAN_POINT('Ctrl Pts',(-5.23288117449473,-4.29462921950947,
47.9159361525174));
#20652=CARTESIAN_POINT('Ctrl Pts',(-5.11281353374605,-4.43689342767989,
47.9246853890038));
#20653=CARTESIAN_POINT('Ctrl Pts',(-4.98709090241752,-4.57397128664188,
47.9334346254902));
#20654=CARTESIAN_POINT('Ctrl Pts',(-4.86136871856977,-4.71104865770678,
47.9421838308358));
#20655=CARTESIAN_POINT('Ctrl Pts',(-4.72999177811196,-4.84293950531728,
47.9509330361813));
#20656=CARTESIAN_POINT('Ctrl Pts',(-4.59340627727753,-4.96919588785424,
47.9596822415268));
#20657=CARTESIAN_POINT('Ctrl Pts',(-4.4568212512464,-5.09545183149432,47.968431416458));
#20658=CARTESIAN_POINT('Ctrl Pts',(-4.31502791149598,-5.21607315474496,
47.9771805913893));
#20659=CARTESIAN_POINT('Ctrl Pts',(-4.16850782818983,-5.33065019358053,
47.9859297663205));
#20660=CARTESIAN_POINT('Ctrl Pts',(-4.02198824205588,-5.44522684363309,
47.994678911564));
#20661=CARTESIAN_POINT('Ctrl Pts',(-3.87074217018864,-5.55375907379691,
48.0034280568075));
#20662=CARTESIAN_POINT('Ctrl Pts',(-3.7152832834129,-5.65587828051423,48.012177202051));
#20663=CARTESIAN_POINT('Ctrl Pts',(-3.55982491123215,-5.75799714919987,
48.0209263183334));
#20664=CARTESIAN_POINT('Ctrl Pts',(-3.40015399154343,-5.85370287959801,
48.0296754346158));
#20665=CARTESIAN_POINT('Ctrl Pts',(-3.23681280454993,-5.94267043241518,
48.0384245508981));
#20666=CARTESIAN_POINT('Ctrl Pts',(-3.07347214468129,-6.03163769812162,
48.0471736389459));
#20667=CARTESIAN_POINT('Ctrl Pts',(-2.90646149284465,-6.11386669270314,
48.0559227269936));
#20668=CARTESIAN_POINT('Ctrl Pts',(-2.73634805305211,-6.18907814884882,
48.0646718150414));
#20669=CARTESIAN_POINT('Ctrl Pts',(-2.56623514811494,-6.2642893685214,48.073420875581));
#20670=CARTESIAN_POINT('Ctrl Pts',(-2.39301973680805,-6.33248297804565,
48.0821699361207));
#20671=CARTESIAN_POINT('Ctrl Pts',(-2.21729009214273,-6.39342737874497,
48.0909189966604));
#20672=CARTESIAN_POINT('Ctrl Pts',(-2.04156098540153,-6.45437159288803,
48.0996680304184));
#20673=CARTESIAN_POINT('Ctrl Pts',(-1.86331793141591,-6.50806654872686,
48.1084170641764));
#20674=CARTESIAN_POINT('Ctrl Pts',(-1.68316627434103,-6.55432988892998,
48.1171660979344));
#20675=CARTESIAN_POINT('Ctrl Pts',(-1.50301515376888,-6.60059309135803,
48.1259151056372));
#20676=CARTESIAN_POINT('Ctrl Pts',(-1.32095571900333,-6.63942465117082,
48.13466411334));
#20677=CARTESIAN_POINT('Ctrl Pts',(-1.13760627160799,-6.67069269047812,
48.1434131210429));
#20678=CARTESIAN_POINT('Ctrl Pts',(-0.954257355016002,-6.7019606392633,
48.152162103417));
#20679=CARTESIAN_POINT('Ctrl Pts',(-0.769618715712151,-6.72566506319355,
48.1609110857912));
#20680=CARTESIAN_POINT('Ctrl Pts',(-0.584317411004386,-6.74172545890124,
48.1696600681653));
#20681=CARTESIAN_POINT('Ctrl Pts',(-0.391031954869637,-6.75847785530213,
48.1787860214422));
#20682=CARTESIAN_POINT('Ctrl Pts',(-0.197025793659618,-6.76691286680797,
48.187911974719));
#20683=CARTESIAN_POINT('Ctrl Pts',(-0.003015734995512,-6.76699932801404,
48.1970379279958));
#20684=CARTESIAN_POINT('Ctrl Pts',(0.184931509335365,-6.76708308730742,
48.2058786952328));
#20685=CARTESIAN_POINT('Ctrl Pts',(0.372882094257411,-6.75933222422522,
48.2147194624697));
#20686=CARTESIAN_POINT('Ctrl Pts',(0.560184265596068,-6.74377361635002,
48.2235602297067));
#20687=CARTESIAN_POINT('Ctrl Pts',(0.745562970101919,-6.72837478487249,
48.2323102082334));
#20688=CARTESIAN_POINT('Ctrl Pts',(0.930306227486469,-6.70532786008224,
48.2410601867601));
#20689=CARTESIAN_POINT('Ctrl Pts',(1.1137864824089,-6.67471113019906,48.2498101652868));
#20690=CARTESIAN_POINT('Ctrl Pts',(1.29726485910632,-6.64409471372894,48.258560054243));
#20691=CARTESIAN_POINT('Ctrl Pts',(1.47947997644983,-6.60590869441571,48.2673099431992));
#20692=CARTESIAN_POINT('Ctrl Pts',(1.65981287961014,-6.56028278389585,48.2760598321554));
#20693=CARTESIAN_POINT('Ctrl Pts',(1.84014399669517,-6.51465732526974,48.2848096344498));
#20694=CARTESIAN_POINT('Ctrl Pts',(2.01859265899936,-6.46159219320578,48.2935594367442));
#20695=CARTESIAN_POINT('Ctrl Pts',(2.19455271771757,-6.40126763767603,48.3023092390387));
#20696=CARTESIAN_POINT('Ctrl Pts',(2.37051109214448,-6.34094365957348,48.3110589575799));
#20697=CARTESIAN_POINT('Ctrl Pts',(2.54398063950056,-6.2733604900174,48.3198086761212));
#20698=CARTESIAN_POINT('Ctrl Pts',(2.71437213515056,-6.19874768900285,48.3285583946625));
#20699=CARTESIAN_POINT('Ctrl Pts',(2.88476205643078,-6.12413557738972,48.3373080323588));
#20700=CARTESIAN_POINT('Ctrl Pts',(3.05207372035493,-6.04249407926827,48.3460576700551));
#20701=CARTESIAN_POINT('Ctrl Pts',(3.21573882928381,-5.95410050148941,48.3548073077514));
#20702=CARTESIAN_POINT('Ctrl Pts',(3.37940248037333,-5.86570771107224,48.3635568675107));
#20703=CARTESIAN_POINT('Ctrl Pts',(3.53941938927846,-5.77056309755689,48.37230642727));
#20704=CARTESIAN_POINT('Ctrl Pts',(3.69524604569606,-5.66898982727678,48.3810559870293));
#20705=CARTESIAN_POINT('Ctrl Pts',(3.85107136586769,-5.56741742800858,48.3898054717593));
#20706=CARTESIAN_POINT('Ctrl Pts',(4.00270626535449,-5.45941663879865,48.3985549564893));
#20707=CARTESIAN_POINT('Ctrl Pts',(4.14963571284667,-5.34535428673044,48.4073044412193));
#20708=CARTESIAN_POINT('Ctrl Pts',(4.2965639492015,-5.23129287487658,48.4160538538275));
#20709=CARTESIAN_POINT('Ctrl Pts',(4.43878658479358,-5.11117017589603,48.4248032664356));
#20710=CARTESIAN_POINT('Ctrl Pts',(4.57582056523246,-4.98539418248905,48.4335526790438));
#20711=CARTESIAN_POINT('Ctrl Pts',(4.71285346162535,-4.85961918406859,48.4423020224372));
#20712=CARTESIAN_POINT('Ctrl Pts',(4.84469757387159,-4.7281911745026,48.4510513658306));
#20713=CARTESIAN_POINT('Ctrl Pts',(4.97090510496334,-4.59155653754252,48.4598007092241));
#20714=CARTESIAN_POINT('Ctrl Pts',(5.0971116795788,-4.45492293608158,48.4685499863098));
#20715=CARTESIAN_POINT('Ctrl Pts',(5.21768156407691,-4.31308299669927,48.4772992633954));
#20716=CARTESIAN_POINT('Ctrl Pts',(5.33220525957991,-4.16651845906247,48.4860485404811));
#20717=CARTESIAN_POINT('Ctrl Pts',(5.44672812519458,-4.01995498349585,48.4947977541657));
#20718=CARTESIAN_POINT('Ctrl Pts',(5.55520471305057,-3.86866720398892,48.5035469678503));
#20719=CARTESIAN_POINT('Ctrl Pts',(5.65726660280775,-3.713168941047,48.512296181535));
#20720=CARTESIAN_POINT('Ctrl Pts',(5.75932778687966,-3.5576717532648,48.521045334725));
#20721=CARTESIAN_POINT('Ctrl Pts',(5.85497420437281,-3.397964379865,48.529794487915));
#20722=CARTESIAN_POINT('Ctrl Pts',(5.94388101469654,-3.23458922942776,48.5385436411051));
#20723=CARTESIAN_POINT('Ctrl Pts',(6.03278723982154,-3.07121515435168,48.5472927367068));
#20724=CARTESIAN_POINT('Ctrl Pts',(6.11495380958366,-2.90417360223718,48.5560418323085));
#20725=CARTESIAN_POINT('Ctrl Pts',(6.19010166819865,-2.73403188301899,48.5647909279102));
#20726=CARTESIAN_POINT('Ctrl Pts',(6.26524905713621,-2.56389122719403,48.5735399688297));
#20727=CARTESIAN_POINT('Ctrl Pts',(6.33337770694414,-2.3906507051453,48.5822890097492));
#20728=CARTESIAN_POINT('Ctrl Pts',(6.39425624059827,-2.21489867252887,48.5910380506687));
#20729=CARTESIAN_POINT('Ctrl Pts',(6.45513441397643,-2.03914768000375,48.5997870398119));
#20730=CARTESIAN_POINT('Ctrl Pts',(6.50876246327865,-1.86088547739572,48.608536028955));
#20731=CARTESIAN_POINT('Ctrl Pts',(6.55495826025521,-1.68071746772384,48.6172850180981));
#20732=CARTESIAN_POINT('Ctrl Pts',(6.6020907396664,-1.49689630731125,48.6262114048615));
#20733=CARTESIAN_POINT('Ctrl Pts',(6.64148625753709,-1.3110915225784,48.6351377916249));
#20734=CARTESIAN_POINT('Ctrl Pts',(6.67300554640953,-1.12395995372949,48.6440641783884));
#20735=CARTESIAN_POINT('Ctrl Pts',(6.70390170574978,-0.940527935572548,
48.6528140924137));
#20736=CARTESIAN_POINT('Ctrl Pts',(6.72723010571988,-0.755821395994563,
48.6615640064391));
#20737=CARTESIAN_POINT('Ctrl Pts',(6.74291150312266,-0.570467756368566,
48.6703139204645));
#20738=CARTESIAN_POINT('Ctrl Pts',(6.75859259215796,-0.385117761636668,
48.6790636624268));
#20739=CARTESIAN_POINT('Ctrl Pts',(6.76662695537733,-0.199120977954146,
48.6878134043892));
#20740=CARTESIAN_POINT('Ctrl Pts',(6.76698730228438,-0.0131091846437382,
48.6965631463516));
#20741=CARTESIAN_POINT('Ctrl Pts',(6.76734764258434,0.172899198075617,48.7053127278843));
#20742=CARTESIAN_POINT('Ctrl Pts',(6.76003424758483,0.35892230324573,48.7140623094171));
#20743=CARTESIAN_POINT('Ctrl Pts',(6.74507195794377,0.544328285284334,48.7228118909499));
#20744=CARTESIAN_POINT('Ctrl Pts',(6.73010992275648,0.729731114246022,48.7315613236843));
#20745=CARTESIAN_POINT('Ctrl Pts',(6.70749927628582,0.914516555404612,48.7403107564188));
#20746=CARTESIAN_POINT('Ctrl Pts',(6.67731681518376,1.09805698834996,48.7490601891532));
#20747=CARTESIAN_POINT('Ctrl Pts',(6.64713482726716,1.28159454384065,48.7578094847184));
#20748=CARTESIAN_POINT('Ctrl Pts',(6.60938130876791,1.46388684739616,48.7665587802837));
#20749=CARTESIAN_POINT('Ctrl Pts',(6.56418448481257,1.64431476589672,48.7753080758489));
#20750=CARTESIAN_POINT('Ctrl Pts',(6.51898830937794,1.82474009547105,48.7840572458721));
#20751=CARTESIAN_POINT('Ctrl Pts',(6.46634911184241,2.00330081555438,48.7928064158953));
#20752=CARTESIAN_POINT('Ctrl Pts',(6.40644566956322,2.17939048427185,48.8015555859186));
#20753=CARTESIAN_POINT('Ctrl Pts',(6.34654300724299,2.35547786025438,48.8103046420252));
#20754=CARTESIAN_POINT('Ctrl Pts',(6.27937638173278,2.52909397798304,48.8190536981319));
#20755=CARTESIAN_POINT('Ctrl Pts',(6.20517390364207,2.699649204167,48.8278027542386));
#20756=CARTESIAN_POINT('Ctrl Pts',(6.12815443731935,2.87667930932306,48.8368839554263));
#20757=CARTESIAN_POINT('Ctrl Pts',(6.04355456528832,3.05041126288029,48.8459651566139));
#20758=CARTESIAN_POINT('Ctrl Pts',(5.95168380961829,3.22020943889175,48.8550463578016));
#20759=CARTESIAN_POINT('Ctrl Pts',(5.86316590408054,3.38381078074475,48.8637961378925));
#20760=CARTESIAN_POINT('Ctrl Pts',(5.76789857594155,3.54376012680152,48.8725459179834));
#20761=CARTESIAN_POINT('Ctrl Pts',(5.6662054246254,3.69951416890729,48.8812956980743));
#20762=CARTESIAN_POINT('Ctrl Pts',(5.56451592882081,3.85526261220236,48.8900451636413));
#20763=CARTESIAN_POINT('Ctrl Pts',(5.45640122875607,4.00681581333296,48.8987946292084));
#20764=CARTESIAN_POINT('Ctrl Pts',(5.34222853680848,4.1536590207321,48.9075440947754));
#20765=CARTESIAN_POINT('Ctrl Pts',(5.2280593420745,4.30049773018996,48.9162932923383));
#20766=CARTESIAN_POINT('Ctrl Pts',(5.10783270268491,4.44262650838489,48.9250424899013));
#20767=CARTESIAN_POINT('Ctrl Pts',(4.98195694431792,4.57956264341503,48.9337916874642));
#20768=CARTESIAN_POINT('Ctrl Pts',(4.85608437269241,4.71649531169298,48.9425406635275));
#20769=CARTESIAN_POINT('Ctrl Pts',(4.72456316218971,4.8482353889234,48.9512896395909));
#20770=CARTESIAN_POINT('Ctrl Pts',(4.58783997564082,4.97433546897594,48.9600386156542));
#20771=CARTESIAN_POINT('Ctrl Pts',(4.45110790519902,5.10044374266142,48.9687881602017));
#20772=CARTESIAN_POINT('Ctrl Pts',(4.30917339295186,5.22091109149112,48.9775377047492));
#20773=CARTESIAN_POINT('Ctrl Pts',(4.16251852921304,5.33532833984546,48.9862872492967));
#20774=CARTESIAN_POINT('Ctrl Pts',(4.01587228434862,5.44973886392304,48.9950362796354));
#20775=CARTESIAN_POINT('Ctrl Pts',(3.86450646904683,5.55809982276747,49.003785309974));
#20776=CARTESIAN_POINT('Ctrl Pts',(3.708935147323,5.6600432041595,49.0125343403127));
#20777=CARTESIAN_POINT('Ctrl Pts',(3.55336172014134,5.76198796522413,49.0212834890583));
#20778=CARTESIAN_POINT('Ctrl Pts',(3.39358291230957,5.85751481797819,49.0300326378038));
#20779=CARTESIAN_POINT('Ctrl Pts',(3.23014137446734,5.94629932823384,49.0387817865494));
#20780=CARTESIAN_POINT('Ctrl Pts',(3.18674080140078,5.96987533391392,49.041105051947));
#20781=CARTESIAN_POINT('Ctrl Pts',(3.14308210500722,5.9929761653931,49.0434283173446));
#20782=CARTESIAN_POINT('Ctrl Pts',(3.0991757505326,6.01559628526638,49.0457515827422));
#20783=CARTESIAN_POINT('Ctrl Pts',(3.09917575053261,6.01559628526638,47.0456199604263));
#20784=CARTESIAN_POINT('Ctrl Pts',(2.94420070234753,6.0954378983828,47.0538464887508));
#20785=CARTESIAN_POINT('Ctrl Pts',(2.78631654012032,6.16919515578224,47.0620730170753));
#20786=CARTESIAN_POINT('Ctrl Pts',(2.62604879104489,6.23667834243932,47.0702995453998));
#20787=CARTESIAN_POINT('Ctrl Pts',(2.60052446512196,6.24742575020221,47.071609706623));
#20788=CARTESIAN_POINT('Ctrl Pts',(2.57493971154706,6.25801412625621,47.0729198678462));
#20789=CARTESIAN_POINT('Ctrl Pts',(2.54929668466128,6.26844282207113,47.0742300290694));
#20790=CARTESIAN_POINT('Ctrl Pts',(2.38831649159949,6.33391143750199,47.0824548773914));
#20791=CARTESIAN_POINT('Ctrl Pts',(2.22458678934626,6.39326674151772,47.0906797257135));
#20792=CARTESIAN_POINT('Ctrl Pts',(2.05861209918271,6.44627064472929,47.0989045740355));
#20793=CARTESIAN_POINT('Ctrl Pts',(1.89282433332024,6.4992148537938,47.1071201593547));
#20794=CARTESIAN_POINT('Ctrl Pts',(1.72479695279772,6.54582179752411,47.1153357446739));
#20795=CARTESIAN_POINT('Ctrl Pts',(1.55505540613306,6.58590097738011,47.1235513299931));
#20796=CARTESIAN_POINT('Ctrl Pts',(1.38547092162903,6.62594307189839,47.1317593134164));
#20797=CARTESIAN_POINT('Ctrl Pts',(1.21417577674592,6.65946934970275,47.1399672968396));
#20798=CARTESIAN_POINT('Ctrl Pts',(1.041711658641,6.68633874555062,47.1481752802628));
#20799=CARTESIAN_POINT('Ctrl Pts',(0.869372481601259,6.71318867595272,47.1563773174394));
#20800=CARTESIAN_POINT('Ctrl Pts',(0.695866371181164,6.73339127501541,47.1645793546159));
#20801=CARTESIAN_POINT('Ctrl Pts',(0.521746405112546,6.74685628191028,47.1727813917924));
#20802=CARTESIAN_POINT('Ctrl Pts',(0.347717614848954,6.76031423801786,47.1809791340718));
#20803=CARTESIAN_POINT('Ctrl Pts',(0.173075966149704,6.76704160281862,47.1891768763513));
#20804=CARTESIAN_POINT('Ctrl Pts',(-0.00161903260454401,6.76699980631989,
47.1973746186307));
#20805=CARTESIAN_POINT('Ctrl Pts',(-0.176280815995487,6.76695801776807,
47.205570802245));
#20806=CARTESIAN_POINT('Ctrl Pts',(-0.350995570826527,6.76014962539898,
47.2137669858594));
#20807=CARTESIAN_POINT('Ctrl Pts',(-0.525202157850227,6.7465881520506,47.2219631694738));
#20808=CARTESIAN_POINT('Ctrl Pts',(-0.699395920838457,6.73302767701587,
47.2301587497346));
#20809=CARTESIAN_POINT('Ctrl Pts',(-0.873081232707041,6.71271513798809,
47.2383543299955));
#20810=CARTESIAN_POINT('Ctrl Pts',(-1.04570050552152,6.68571607628922,47.2465499102564));
#20811=CARTESIAN_POINT('Ctrl Pts',(-1.21833847718382,6.65871408993809,47.2547463782971));
#20812=CARTESIAN_POINT('Ctrl Pts',(-1.38990982513253,6.62502419332592,47.2629428463378));
#20813=CARTESIAN_POINT('Ctrl Pts',(-1.55986555218957,6.58476335634716,47.2711393143786));
#20814=CARTESIAN_POINT('Ctrl Pts',(-1.72987061113206,6.54449083313086,47.2793381615519));
#20815=CARTESIAN_POINT('Ctrl Pts',(-1.89825876600454,6.49764365313928,47.2875370087253));
#20816=CARTESIAN_POINT('Ctrl Pts',(-2.06449456563181,6.44438912453902,47.2957358558987));
#20817=CARTESIAN_POINT('Ctrl Pts',(-2.23090409783499,6.39107893977773,47.3039432716647));
#20818=CARTESIAN_POINT('Ctrl Pts',(-2.39515643856376,6.33134813769041,47.3121506874306));
#20819=CARTESIAN_POINT('Ctrl Pts',(-2.55673362096148,6.26541317005074,47.3203581031966));
#20820=CARTESIAN_POINT('Ctrl Pts',(-2.71839740304603,6.19944286358745,47.3285699178487));
#20821=CARTESIAN_POINT('Ctrl Pts',(-2.87738284207945,6.12726191087421,47.3367817325009));
#20822=CARTESIAN_POINT('Ctrl Pts',(-3.03319520514806,6.04913347905854,47.344993547153));
#20823=CARTESIAN_POINT('Ctrl Pts',(-3.18923702560847,5.97088999124964,47.3532174549506));
#20824=CARTESIAN_POINT('Ctrl Pts',(-3.34209611727311,5.8866816937324,47.3614413627483));
#20825=CARTESIAN_POINT('Ctrl Pts',(-3.49130433125497,5.79681663213184,47.3696652705459));
#20826=CARTESIAN_POINT('Ctrl Pts',(-3.6291699653541,5.71378297486666,47.3772640094694));
#20827=CARTESIAN_POINT('Ctrl Pts',(-3.76391883116865,5.6259205046909,47.3848627483929));
#20828=CARTESIAN_POINT('Ctrl Pts',(-3.89520661056735,5.53350291054341,47.3924614873164));
#20829=CARTESIAN_POINT('Ctrl Pts',(-4.03509486809112,5.43503116954024,47.4005580089596));
#20830=CARTESIAN_POINT('Ctrl Pts',(-4.17148000542102,5.33108698804352,47.4086545306027));
#20831=CARTESIAN_POINT('Ctrl Pts',(-4.30389637344467,5.22195030679628,47.4167510522459));
#20832=CARTESIAN_POINT('Ctrl Pts',(-4.43615862108418,5.11294065053463,47.424838150288));
#20833=CARTESIAN_POINT('Ctrl Pts',(-4.5644610092719,4.99875075525649,47.4329252483302));
#20834=CARTESIAN_POINT('Ctrl Pts',(-4.68836577643363,4.87970443227517,47.4410123463723));
#20835=CARTESIAN_POINT('Ctrl Pts',(-4.8121531637216,4.76077088657177,47.4490917831874));
#20836=CARTESIAN_POINT('Ctrl Pts',(-4.93155095663324,4.63699032549633,47.4571712200025));
#20837=CARTESIAN_POINT('Ctrl Pts',(-5.0461535513924,4.50872746301768,47.4652506568177));
#20838=CARTESIAN_POINT('Ctrl Pts',(-5.16067237307605,4.38055835910084,47.4733241876647));
#20839=CARTESIAN_POINT('Ctrl Pts',(-5.27040272860054,4.24791375180502,47.4813977185117));
#20840=CARTESIAN_POINT('Ctrl Pts',(-5.37497511899457,4.11119586862379,47.4894712493587));
#20841=CARTESIAN_POINT('Ctrl Pts',(-5.47949367726756,3.9745483655267,47.4975406240868));
#20842=CARTESIAN_POINT('Ctrl Pts',(-5.57885933259808,3.8338320556282,47.5056099988149));
#20843=CARTESIAN_POINT('Ctrl Pts',(-5.67274227269699,3.68948290517203,47.513679373543));
#20844=CARTESIAN_POINT('Ctrl Pts',(-5.76661107747611,3.54515548839186,47.5217475333199));
#20845=CARTESIAN_POINT('Ctrl Pts',(-5.8549986018577,3.39719662643701,47.5298156930968));
#20846=CARTESIAN_POINT('Ctrl Pts',(-5.93761777482627,3.24607211257962,47.5378838528736));
#20847=CARTESIAN_POINT('Ctrl Pts',(-6.0202340176665,3.09495295842514,47.5459517265094));
#20848=CARTESIAN_POINT('Ctrl Pts',(-6.09708213755128,2.94066870104229,47.5540196001451));
#20849=CARTESIAN_POINT('Ctrl Pts',(-6.16792066567482,2.78371041273002,47.5620874737809));
#20850=CARTESIAN_POINT('Ctrl Pts',(-6.23877054869785,2.62672696514868,47.5701566406379));
#20851=CARTESIAN_POINT('Ctrl Pts',(-6.30360876960811,2.46706897157694,47.578225807495));
#20852=CARTESIAN_POINT('Ctrl Pts',(-6.3622417676081,2.30524807569663,47.5862949743521));
#20853=CARTESIAN_POINT('Ctrl Pts',(-6.42089564396256,2.14336955775808,47.5943670145217));
#20854=CARTESIAN_POINT('Ctrl Pts',(-6.47333977272037,1.97932695298936,47.6024390546912));
#20855=CARTESIAN_POINT('Ctrl Pts',(-6.51943030803423,1.81364755635838,47.6105110948607));
#20856=CARTESIAN_POINT('Ctrl Pts',(-6.56557201593449,1.6477842121299,47.6185920971127));
#20857=CARTESIAN_POINT('Ctrl Pts',(-6.60534594483719,1.48028080479,47.6266730993646));
#20858=CARTESIAN_POINT('Ctrl Pts',(-6.63865911135347,1.31167610454852,47.6347541016165));
#20859=CARTESIAN_POINT('Ctrl Pts',(-6.67199286151105,1.14296722631874,47.6428400969828));
#20860=CARTESIAN_POINT('Ctrl Pts',(-6.69885784039119,0.973156065076676,
47.6509260923491));
#20861=CARTESIAN_POINT('Ctrl Pts',(-6.71921295318792,0.802786577934436,
47.6590120877154));
#20862=CARTESIAN_POINT('Ctrl Pts',(-6.73959751400368,0.632170614933792,
47.6671097812014));
#20863=CARTESIAN_POINT('Ctrl Pts',(-6.75345337276775,0.460995081396149,
47.6752074746874));
#20864=CARTESIAN_POINT('Ctrl Pts',(-6.7607915301348,0.289804910340657,47.6833051681734));
#20865=CARTESIAN_POINT('Ctrl Pts',(-6.76494034071624,0.193018270645183,
47.6878834014736));
#20866=CARTESIAN_POINT('Ctrl Pts',(-6.76700672276788,0.0962268956752369,
47.6924616347738));
#20867=CARTESIAN_POINT('Ctrl Pts',(-6.76699998356599,-0.000471612025413017,
47.697039868074));
#20868=CARTESIAN_POINT('',(-6.767,1.57869390845534E-12,47.3028202161899));
#20869=CARTESIAN_POINT('Ctrl Pts',(3.09917575053265,6.01559628526636,46.6512392818024));
#20870=CARTESIAN_POINT('Ctrl Pts',(2.93619253716553,6.09956362593521,46.6598710590822));
#20871=CARTESIAN_POINT('Ctrl Pts',(2.76991958324212,6.17683924023712,46.6685028363621));
#20872=CARTESIAN_POINT('Ctrl Pts',(2.60092745572062,6.24719660088257,46.6771346136419));
#20873=CARTESIAN_POINT('Ctrl Pts',(2.43165828803,6.31766930308491,46.6857805415752));
#20874=CARTESIAN_POINT('Ctrl Pts',(2.25966132069246,6.3812009694572,46.6944264695086));
#20875=CARTESIAN_POINT('Ctrl Pts',(2.08552446834769,6.43761420806832,46.7030723974419));
#20876=CARTESIAN_POINT('Ctrl Pts',(1.99160676613167,6.46803971348879,46.7077354292705));
#20877=CARTESIAN_POINT('Ctrl Pts',(1.89706683779563,6.49639548331203,46.7123984610992));
#20878=CARTESIAN_POINT('Ctrl Pts',(1.80199820030188,6.52265984749387,46.7170614929278));
#20879=CARTESIAN_POINT('Ctrl Pts',(1.63428887905408,6.56899246365482,46.7252874854692));
#20880=CARTESIAN_POINT('Ctrl Pts',(1.46457135062787,6.60891357559464,46.7335134780105));
#20881=CARTESIAN_POINT('Ctrl Pts',(1.29337652475002,6.64224857749434,46.7417394705518));
#20882=CARTESIAN_POINT('Ctrl Pts',(1.12236117451943,6.67554863195325,46.7499568392032));
#20883=CARTESIAN_POINT('Ctrl Pts',(0.949871959778354,6.70227625823853,46.7581742078546));
#20884=CARTESIAN_POINT('Ctrl Pts',(0.776454648957584,6.72230668581196,46.766391576506));
#20885=CARTESIAN_POINT('Ctrl Pts',(0.603184443719548,6.74232012207289,46.7746019745684));
#20886=CARTESIAN_POINT('Ctrl Pts',(0.428988064300652,6.75564763335025,46.7828123726308));
#20887=CARTESIAN_POINT('Ctrl Pts',(0.254421263079605,6.76221552606045,46.7910227706932));
#20888=CARTESIAN_POINT('Ctrl Pts',(0.079967622301007,6.76877916122775,46.799227846482));
#20889=CARTESIAN_POINT('Ctrl Pts',(-0.0948556052224034,6.76859189268669,
46.8074329222707));
#20890=CARTESIAN_POINT('Ctrl Pts',(-0.26948765704395,6.76163185944791,46.8156379980595));
#20891=CARTESIAN_POINT('Ctrl Pts',(-0.444041432302684,6.75467494595418,
46.823839396029));
#20892=CARTESIAN_POINT('Ctrl Pts',(-0.618403845327353,6.74095133021332,
46.8320407939985));
#20893=CARTESIAN_POINT('Ctrl Pts',(-0.792014147959577,6.72049124613907,
46.840242191968));
#20894=CARTESIAN_POINT('Ctrl Pts',(-0.965610851987389,6.70003276466896,
46.8484429475357));
#20895=CARTESIAN_POINT('Ctrl Pts',(-1.13845520640495,6.67283889913459,46.8566437031034));
#20896=CARTESIAN_POINT('Ctrl Pts',(-1.30999122033133,6.63899179112724,46.8648444586711));
#20897=CARTESIAN_POINT('Ctrl Pts',(-1.48152636293633,6.6051448550471,46.8730451725829));
#20898=CARTESIAN_POINT('Ctrl Pts',(-1.65175282648683,6.56464481213974,46.8812458864946));
#20899=CARTESIAN_POINT('Ctrl Pts',(-1.82012457539106,6.51762499151781,46.8894466004064));
#20900=CARTESIAN_POINT('Ctrl Pts',(-1.98852598220045,6.47059688857186,46.897648758836));
#20901=CARTESIAN_POINT('Ctrl Pts',(-2.15507167829978,6.41704681625701,46.9058509172656));
#20902=CARTESIAN_POINT('Ctrl Pts',(-2.31923050400422,6.35715808119449,46.9140530756952));
#20903=CARTESIAN_POINT('Ctrl Pts',(-2.48344799550768,6.29724794356357,46.9222581653482));
#20904=CARTESIAN_POINT('Ctrl Pts',(-2.64527658093408,6.23099475339782,46.9304632550011));
#20905=CARTESIAN_POINT('Ctrl Pts',(-2.80420475171964,6.15863010014671,46.938668344654));
#20906=CARTESIAN_POINT('Ctrl Pts',(-2.96331447915035,6.08618277883488,46.9468828076518));
#20907=CARTESIAN_POINT('Ctrl Pts',(-3.11951684590354,6.00761019503864,46.9550972706496));
#20908=CARTESIAN_POINT('Ctrl Pts',(-3.27232370178156,5.92319057525238,46.9633117336474));
#20909=CARTESIAN_POINT('Ctrl Pts',(-3.4252210908921,5.83872093950955,46.9715310634548));
#20910=CARTESIAN_POINT('Ctrl Pts',(-3.57471865275116,5.74839754733832,46.9797503932623));
#20911=CARTESIAN_POINT('Ctrl Pts',(-3.72035705695915,5.65254211560907,46.9879697230698));
#20912=CARTESIAN_POINT('Ctrl Pts',(-3.86622111904454,5.55653816169999,46.9962017882305));
#20913=CARTESIAN_POINT('Ctrl Pts',(-4.00821378275411,5.45498524724284,47.0044338533911));
#20914=CARTESIAN_POINT('Ctrl Pts',(-4.14590759872467,5.34824636519645,47.0126659185518));
#20915=CARTESIAN_POINT('Ctrl Pts',(-4.26967668747936,5.25230179373944,47.0200654898131));
#20916=CARTESIAN_POINT('Ctrl Pts',(-4.38997275868149,5.15216776742733,47.0274650610743));
#20917=CARTESIAN_POINT('Ctrl Pts',(-4.50651135356984,5.04813276570121,47.0348646323356));
#20918=CARTESIAN_POINT('Ctrl Pts',(-4.63308913785861,4.93513569361889,47.0429016378944));
#20919=CARTESIAN_POINT('Ctrl Pts',(-4.75564675297842,4.81716699154376,47.0509386434532));
#20920=CARTESIAN_POINT('Ctrl Pts',(-4.87375585167972,4.69454927529978,47.058975649012));
#20921=CARTESIAN_POINT('Ctrl Pts',(-4.99172100065018,4.57208100382716,47.06700285918));
#20922=CARTESIAN_POINT('Ctrl Pts',(-5.10524816249726,4.44497525956722,47.0750300693479));
#20923=CARTESIAN_POINT('Ctrl Pts',(-5.21394127849122,4.31359540806105,47.0830572795159));
#20924=CARTESIAN_POINT('Ctrl Pts',(-5.32252614494393,4.18234640024746,47.0910764952326));
#20925=CARTESIAN_POINT('Ctrl Pts',(-5.42628630775912,4.0468320435427,47.0990957109493));
#20926=CARTESIAN_POINT('Ctrl Pts',(-5.5248619918402,3.90745300305961,47.107114926666));
#20927=CARTESIAN_POINT('Ctrl Pts',(-5.62495660593286,3.76592630304417,47.1152577086306));
#20928=CARTESIAN_POINT('Ctrl Pts',(-5.71970536117816,3.62041510074397,47.1234004905953));
#20929=CARTESIAN_POINT('Ctrl Pts',(-5.80877294194265,3.47137521869287,47.1315432725599));
#20930=CARTESIAN_POINT('Ctrl Pts',(-5.89637343232061,3.32479027003381,47.1395519294362));
#20931=CARTESIAN_POINT('Ctrl Pts',(-5.97847825535804,3.17479232576088,47.1475605863125));
#20932=CARTESIAN_POINT('Ctrl Pts',(-6.05481135274774,3.0218452115615,47.1555692431888));
#20933=CARTESIAN_POINT('Ctrl Pts',(-6.13112427005438,2.86893853179454,47.1635757828267));
#20934=CARTESIAN_POINT('Ctrl Pts',(-6.20166832973967,2.71308457008167,47.1715823224647));
#20935=CARTESIAN_POINT('Ctrl Pts',(-6.26621333059703,2.55477190673612,47.1795888621026));
#20936=CARTESIAN_POINT('Ctrl Pts',(-6.33075423601889,2.39646928846443,47.1875948937188));
#20937=CARTESIAN_POINT('Ctrl Pts',(-6.38929669877065,2.2357086280691,47.1956009253349));
#20938=CARTESIAN_POINT('Ctrl Pts',(-6.44165866722065,2.07299845996594,47.2036069569511));
#20939=CARTESIAN_POINT('Ctrl Pts',(-6.49558069562354,1.90544054406604,47.2118515183566));
#20940=CARTESIAN_POINT('Ctrl Pts',(-6.54294808136012,1.73581554642876,47.2200960797621));
#20941=CARTESIAN_POINT('Ctrl Pts',(-6.58361741644066,1.56469508657096,47.2283406411677));
#20942=CARTESIAN_POINT('Ctrl Pts',(-6.62314407831425,1.39838254315073,47.2363535577872));
#20943=CARTESIAN_POINT('Ctrl Pts',(-6.65634397652307,1.23065782574296,47.2443664744068));
#20944=CARTESIAN_POINT('Ctrl Pts',(-6.68313760284297,1.0620549804348,47.2523793910263));
#20945=CARTESIAN_POINT('Ctrl Pts',(-6.71109309146522,0.886140945230387,
47.2607397748249));
#20946=CARTESIAN_POINT('Ctrl Pts',(-6.73207423179778,0.709271383199012,
47.2691001586234));
#20947=CARTESIAN_POINT('Ctrl Pts',(-6.74605103415646,0.532056805760918,
47.2774605424219));
#20948=CARTESIAN_POINT('Ctrl Pts',(-6.76002783651515,0.35484222832276,47.2858209262205));
#20949=CARTESIAN_POINT('Ctrl Pts',(-6.76700033878351,0.177283097596419,
47.294181310019));
#20950=CARTESIAN_POINT('Ctrl Pts',(-6.76699999998765,-1.29310941174092E-5,
47.3025416938175));
#20951=CARTESIAN_POINT('Ctrl Pts',(-6.767,1.57869394139717E-12,47.3028202161899));
#20952=CARTESIAN_POINT('Ctrl Pts',(-6.76700000000004,-0.186007249414218,
47.3115697279959));
#20953=CARTESIAN_POINT('Ctrl Pts',(-6.75932637295446,-0.372014355526194,
47.3203192398018));
#20954=CARTESIAN_POINT('Ctrl Pts',(-6.74400518266938,-0.557389537153829,
47.3290687516078));
#20955=CARTESIAN_POINT('Ctrl Pts',(-6.72868405709658,-0.742763935810309,
47.3378182264583));
#20956=CARTESIAN_POINT('Ctrl Pts',(-6.70571545653005,-0.927506129694079,
47.3465677013089));
#20957=CARTESIAN_POINT('Ctrl Pts',(-6.67517739415664,-1.11098863924893,
47.3553171761594));
#20958=CARTESIAN_POINT('Ctrl Pts',(-6.64463945823081,-1.294470389066,47.3640666147814));
#20959=CARTESIAN_POINT('Ctrl Pts',(-6.60653217027132,-1.47669218228331,
47.3728160534034));
#20960=CARTESIAN_POINT('Ctrl Pts',(-6.56098496116679,-1.65703510504251,
47.3815654920254));
#20961=CARTESIAN_POINT('Ctrl Pts',(-6.51543793687479,-1.83737729604157,
47.3903148951456));
#20962=CARTESIAN_POINT('Ctrl Pts',(-6.46245112202595,-2.01584035397196,
47.3990642982659));
#20963=CARTESIAN_POINT('Ctrl Pts',(-6.40220448416191,-2.19181813638292,
47.4078137013861));
#20964=CARTESIAN_POINT('Ctrl Pts',(-6.34195808575127,-2.36779521936104,
47.4165630697314));
#20965=CARTESIAN_POINT('Ctrl Pts',(-6.27445201489166,-2.54128677544999,
47.4253124380766));
#20966=CARTESIAN_POINT('Ctrl Pts',(-6.19991555136104,-2.71170355238023,
47.4340618064219));
#20967=CARTESIAN_POINT('Ctrl Pts',(-6.12537937788949,-2.88211966613263,
47.442811140719));
#20968=CARTESIAN_POINT('Ctrl Pts',(-6.04381298133517,-3.04946076210644,
47.451560475016));
#20969=CARTESIAN_POINT('Ctrl Pts',(-5.95549339426195,-3.21315848207062,
47.4603098093131));
#20970=CARTESIAN_POINT('Ctrl Pts',(-5.86717414355043,-3.37685557859841,
47.4690591102887));
#20971=CARTESIAN_POINT('Ctrl Pts',(-5.77210188986114,-3.53690907467513,
47.4778084112642));
#20972=CARTESIAN_POINT('Ctrl Pts',(-5.67059953466938,-3.69277536785104,
47.4865577122398));
#20973=CARTESIAN_POINT('Ctrl Pts',(-5.56909755761628,-3.84864108035993,
47.4953069806206));
#20974=CARTESIAN_POINT('Ctrl Pts',(-5.46116568337924,-4.00031938104479,
47.5040562490013));
#20975=CARTESIAN_POINT('Ctrl Pts',(-5.3471704868596,-4.14729511663418,47.5128055173821));
#20976=CARTESIAN_POINT('Ctrl Pts',(-5.23317570555375,-4.29427031688213,
47.5215547538947));
#20977=CARTESIAN_POINT('Ctrl Pts',(-5.11311782178677,-4.43654275987276,
47.5303039904073));
#20978=CARTESIAN_POINT('Ctrl Pts',(-4.98740459171902,-4.57362924147772,
47.5390532269199));
#20979=CARTESIAN_POINT('Ctrl Pts',(-4.86169180910708,-4.71071523514563,
47.547802432291));
#20980=CARTESIAN_POINT('Ctrl Pts',(-4.73032391415299,-4.84261509316654,
47.5565516376621));
#20981=CARTESIAN_POINT('Ctrl Pts',(-4.5937470723715,-4.96888084331656,47.5653008430333));
#20982=CARTESIAN_POINT('Ctrl Pts',(-4.45717070537264,-5.09514615452845,
47.5740500179895));
#20983=CARTESIAN_POINT('Ctrl Pts',(-4.31538563819377,-5.21577720253742,
47.5827991929457));
#20984=CARTESIAN_POINT('Ctrl Pts',(-4.16887341290522,-5.33036429028748,
47.5915483679019));
#20985=CARTESIAN_POINT('Ctrl Pts',(-4.02236168477222,-5.44495098921262,
47.6002975131699));
#20986=CARTESIAN_POINT('Ctrl Pts',(-3.87112305634334,-5.55349359238832,
47.6090466584378));
#20987=CARTESIAN_POINT('Ctrl Pts',(-3.71567117316639,-5.65562346102535,
47.6177958037057));
#20988=CARTESIAN_POINT('Ctrl Pts',(-3.56021980457248,-5.757752991588,47.6265449200118));
#20989=CARTESIAN_POINT('Ctrl Pts',(-3.40055544862379,-5.85346967275357,
47.635294036318));
#20990=CARTESIAN_POINT('Ctrl Pts',(-3.2372203632344,-5.94244842803541,47.6440431526241));
#20991=CARTESIAN_POINT('Ctrl Pts',(-3.07388580496105,-6.03142689616445,
47.652792240695));
#20992=CARTESIAN_POINT('Ctrl Pts',(-2.90688079257788,-6.11366734484783,
47.661541328766));
#20993=CARTESIAN_POINT('Ctrl Pts',(-2.73677251094719,-6.18889046787256,
47.6702904168369));
#20994=CARTESIAN_POINT('Ctrl Pts',(-2.56666476416749,-6.26411335438228,
47.6790394773991));
#20995=CARTESIAN_POINT('Ctrl Pts',(-2.39345402972197,-6.33231884350251,
47.6877885379614));
#20996=CARTESIAN_POINT('Ctrl Pts',(-2.21772856474142,-6.39327529621007,
47.6965375985236));
#20997=CARTESIAN_POINT('Ctrl Pts',(-2.04200363768377,-6.45423156232048,
47.7052866323036));
#20998=CARTESIAN_POINT('Ctrl Pts',(-1.86376426620204,-6.50793874252024,
47.7140356660836));
#20999=CARTESIAN_POINT('Ctrl Pts',(-1.68361578194803,-6.55421443796093,
47.7227846998636));
#21000=CARTESIAN_POINT('Ctrl Pts',(-1.50346783419996,-6.6004899955865,47.7315337075878));
#21001=CARTESIAN_POINT('Ctrl Pts',(-1.32141106257388,-6.63933404145467,
47.740282715312));
#21002=CARTESIAN_POINT('Ctrl Pts',(-1.13806375959199,-6.67061465527003,
47.7490317230363));
#21003=CARTESIAN_POINT('Ctrl Pts',(-0.954716987420964,-6.70189517852454,
47.7577807054311));
#21004=CARTESIAN_POINT('Ctrl Pts',(-0.770079973811953,-6.72561226535803,
47.766529687826));
#21005=CARTESIAN_POINT('Ctrl Pts',(-0.584779770554797,-6.74168536939762,
47.7752786702209));
#21006=CARTESIAN_POINT('Ctrl Pts',(-0.391490647556247,-6.7584514394238,
47.7844048508969));
#21007=CARTESIAN_POINT('Ctrl Pts',(-0.197480213106664,-6.7668997592402,
47.793531031573));
#21008=CARTESIAN_POINT('Ctrl Pts',(-0.00346532630011522,-6.76699911271707,
47.802657212249));
#21009=CARTESIAN_POINT('Ctrl Pts',(0.184486595293761,-6.7670953613978,47.811498199779));
#21010=CARTESIAN_POINT('Ctrl Pts',(0.372442378182964,-6.75935659726783,
47.8203391873089));
#21011=CARTESIAN_POINT('Ctrl Pts',(0.559750217719851,-6.74380965729035,
47.8291801748388));
#21012=CARTESIAN_POINT('Ctrl Pts',(0.745129914455523,-6.72842275717278,
47.8379301534366));
#21013=CARTESIAN_POINT('Ctrl Pts',(0.92987465631196,-6.70538772273504,47.8466801320344));
#21014=CARTESIAN_POINT('Ctrl Pts',(1.11335688289556,-6.67478280180779,47.8554301106321));
#21015=CARTESIAN_POINT('Ctrl Pts',(1.29683723118635,-6.64417819418067,47.8641799996571));
#21016=CARTESIAN_POINT('Ctrl Pts',(1.47905480730015,-6.60600390230124,47.872929888682));
#21017=CARTESIAN_POINT('Ctrl Pts',(1.65939064804589,-6.5603895979719,47.8816797777069));
#21018=CARTESIAN_POINT('Ctrl Pts',(1.8397247026404,-6.51477574543319,47.8904295800679));
#21019=CARTESIAN_POINT('Ctrl Pts',(2.01817678125617,-6.46172209820172,47.8991793824288));
#21020=CARTESIAN_POINT('Ctrl Pts',(2.19414072347444,-6.40140886724095,47.9079291847898));
#21021=CARTESIAN_POINT('Ctrl Pts',(2.37010298131865,-6.34109621361461,47.9166789033953));
#21022=CARTESIAN_POINT('Ctrl Pts',(2.54357687926684,-6.27352420826064,47.9254286220008));
#21023=CARTESIAN_POINT('Ctrl Pts',(2.71397317789746,-6.19892237325595,47.9341783406062));
#21024=CARTESIAN_POINT('Ctrl Pts',(2.88436790206983,-6.12432122757066,47.9429279783645));
#21025=CARTESIAN_POINT('Ctrl Pts',(3.05168482126046,-6.04269049717523,47.9516776161228));
#21026=CARTESIAN_POINT('Ctrl Pts',(3.21535561997186,-5.95430745235039,47.9604272538811));
#21027=CARTESIAN_POINT('Ctrl Pts',(3.37902496075074,-5.86592519481635,47.9691768137001));
#21028=CARTESIAN_POINT('Ctrl Pts',(3.53904799384665,-5.7707908794036,47.9779263735191));
#21029=CARTESIAN_POINT('Ctrl Pts',(3.69488118814772,-5.66922763747163,47.9866759333381));
#21030=CARTESIAN_POINT('Ctrl Pts',(3.85071304610632,-5.56766526649191,47.9954254181255));
#21031=CARTESIAN_POINT('Ctrl Pts',(4.00235489705778,-5.45967423580853,48.004174902913));
#21032=CARTESIAN_POINT('Ctrl Pts',(4.14929168607474,-5.34562133936468,48.0129243877004));
#21033=CARTESIAN_POINT('Ctrl Pts',(4.29622726385572,-5.23156938308683,48.0216738003637));
#21034=CARTESIAN_POINT('Ctrl Pts',(4.43845763091876,-5.11145583677367,48.030423213027));
#21035=CARTESIAN_POINT('Ctrl Pts',(4.57549970660767,-4.9856886620439,48.0391726256903));
#21036=CARTESIAN_POINT('Ctrl Pts',(4.71254069815098,-4.85992248226352,48.0479219691366));
#21037=CARTESIAN_POINT('Ctrl Pts',(4.84439326931116,-4.72850295734205,48.0566713125829));
#21038=CARTESIAN_POINT('Ctrl Pts',(4.970609594345,-4.59187644221896,48.0654206560293));
#21039=CARTESIAN_POINT('Ctrl Pts',(5.09682496280332,-4.45525096256874,48.0741699331656));
#21040=CARTESIAN_POINT('Ctrl Pts',(5.2174039761567,-4.31341878218531,48.0829192103019));
#21041=CARTESIAN_POINT('Ctrl Pts',(5.33193710451779,-4.16686161438876,48.0916684874381));
#21042=CARTESIAN_POINT('Ctrl Pts',(5.4464694028923,-4.02030550864721,48.1004177011711));
#21043=CARTESIAN_POINT('Ctrl Pts',(5.55495572749514,-3.8690247098035,48.1091669149041));
#21044=CARTESIAN_POINT('Ctrl Pts',(5.65702762491308,-3.71353301466007,48.117916128637));
#21045=CARTESIAN_POINT('Ctrl Pts',(5.7590988165501,-3.55804239467125,48.1266652818732));
#21046=CARTESIAN_POINT('Ctrl Pts',(5.85475551250643,-3.39834117619792,48.1354144351093));
#21047=CARTESIAN_POINT('Ctrl Pts',(5.94367283727961,-3.23497174692215,48.1441635883454));
#21048=CARTESIAN_POINT('Ctrl Pts',(6.0325895767618,-3.07160339301223,48.1529126839909));
#21049=CARTESIAN_POINT('Ctrl Pts',(6.11476689685156,-2.90456712829773,48.1616617796364));
#21050=CARTESIAN_POINT('Ctrl Pts',(6.18992570525137,-2.73443024476185,48.170410875282));
#21051=CARTESIAN_POINT('Ctrl Pts',(6.26508404388581,-2.56429442463313,48.179159916243));
#21052=CARTESIAN_POINT('Ctrl Pts',(6.33322384283207,-2.39105828656279,48.187908957204));
#21053=CARTESIAN_POINT('Ctrl Pts',(6.39411368719933,-2.2153101713237,48.196657998165));
#21054=CARTESIAN_POINT('Ctrl Pts',(6.45500317120803,-2.03956309619792,48.2054069873475));
#21055=CARTESIAN_POINT('Ctrl Pts',(6.50864269269998,-1.86130434438897,48.2141559765299));
#21056=CARTESIAN_POINT('Ctrl Pts',(6.55485008446269,-1.68113930720195,48.2229049657123));
#21057=CARTESIAN_POINT('Ctrl Pts',(6.60199664749348,-1.49731239212087,48.2318317792417));
#21058=CARTESIAN_POINT('Ctrl Pts',(6.64140563640859,-1.31150116499914,48.240758592771));
#21059=CARTESIAN_POINT('Ctrl Pts',(6.67293772282132,-1.12436255155899,48.2496854063004));
#21060=CARTESIAN_POINT('Ctrl Pts',(6.70384494949837,-0.940932395053742,
48.2584353204559));
#21061=CARTESIAN_POINT('Ctrl Pts',(6.72718449348903,-0.756227260509118,
48.2671852346114));
#21062=CARTESIAN_POINT('Ctrl Pts',(6.74287707373912,-0.570874564544097,
48.275935148767));
#21063=CARTESIAN_POINT('Ctrl Pts',(6.75856934538656,-0.385525513634903,
48.284684890851));
#21064=CARTESIAN_POINT('Ctrl Pts',(6.76661493004096,-0.199529212420676,
48.2934346329349));
#21065=CARTESIAN_POINT('Ctrl Pts',(6.76698649908906,-0.0135174386028909,
48.3021843750189));
#21066=CARTESIAN_POINT('Ctrl Pts',(6.76735806132396,0.172490924443328,48.3109339566648));
#21067=CARTESIAN_POINT('Ctrl Pts',(6.76005588896302,0.358514472898973,48.3196835383107));
#21068=CARTESIAN_POINT('Ctrl Pts',(6.74510478454604,0.543921359659797,48.3284331199566));
#21069=CARTESIAN_POINT('Ctrl Pts',(6.73015393440714,0.729325093148028,48.3371825527956));
#21070=CARTESIAN_POINT('Ctrl Pts',(6.7075544355693,0.914111900253936,48.3459319856347));
#21071=CARTESIAN_POINT('Ctrl Pts',(6.67738304682358,1.09765415591297,48.3546814184737));
#21072=CARTESIAN_POINT('Ctrl Pts',(6.64721213111906,1.28119353391034,48.3634307141351));
#21073=CARTESIAN_POINT('Ctrl Pts',(6.60946960955546,1.46348811672417,48.3721800097964));
#21074=CARTESIAN_POINT('Ctrl Pts',(6.56428366991241,1.64391876347989,48.3809293054577));
#21075=CARTESIAN_POINT('Ctrl Pts',(6.51909837867783,1.82434682109482,48.3896784755685));
#21076=CARTESIAN_POINT('Ctrl Pts',(6.46646995271994,2.00291071820211,48.3984276456794));
#21077=CARTESIAN_POINT('Ctrl Pts',(6.40657713281629,2.17900400212469,48.4071768157902));
#21078=CARTESIAN_POINT('Ctrl Pts',(6.34668509279148,2.35509499309419,48.415925871976));
#21079=CARTESIAN_POINT('Ctrl Pts',(6.27952894037623,2.52871516397879,48.4246749281617));
#21080=CARTESIAN_POINT('Ctrl Pts',(6.20533675061554,2.69927486771173,48.4334239843475));
#21081=CARTESIAN_POINT('Ctrl Pts',(6.12832117908028,2.87632521635686,48.4425059856298));
#21082=CARTESIAN_POINT('Ctrl Pts',(6.04372366626194,3.05007728919771,48.4515879869121));
#21083=CARTESIAN_POINT('Ctrl Pts',(5.95185378007985,3.21989527477979,48.4606699881943));
#21084=CARTESIAN_POINT('Ctrl Pts',(5.86334450817496,3.38350129286534,48.4694197685014));
#21085=CARTESIAN_POINT('Ctrl Pts',(5.76808562057389,3.54345567124744,48.4781695488086));
#21086=CARTESIAN_POINT('Ctrl Pts',(5.66640068804626,3.69921508465091,48.4869193291157));
#21087=CARTESIAN_POINT('Ctrl Pts',(5.56471941108072,3.85496889852069,48.4956687948692));
#21088=CARTESIAN_POINT('Ctrl Pts',(5.45661270815268,4.00652780919426,48.5044182606226));
#21089=CARTESIAN_POINT('Ctrl Pts',(5.34244776449275,4.15337704569023,48.5131677263761));
#21090=CARTESIAN_POINT('Ctrl Pts',(5.22828631819766,4.30022178356042,48.5219169240957));
#21091=CARTESIAN_POINT('Ctrl Pts',(5.10806717844251,4.4423569097247,48.5306661218153));
#21092=CARTESIAN_POINT('Ctrl Pts',(4.98219864544912,4.57929969070436,48.5394153195349));
#21093=CARTESIAN_POINT('Ctrl Pts',(4.85633329944224,4.71623900429795,48.5481642957252));
#21094=CARTESIAN_POINT('Ctrl Pts',(4.72481904033855,4.84798602483416,48.5569132719154));
#21095=CARTESIAN_POINT('Ctrl Pts',(4.58810250737412,4.97409332258929,48.5656622481056));
#21096=CARTESIAN_POINT('Ctrl Pts',(4.45137708685855,5.1002088182195,48.5744117930418));
#21097=CARTESIAN_POINT('Ctrl Pts',(4.30944892636264,5.22068366307758,48.583161337978));
#21098=CARTESIAN_POINT('Ctrl Pts',(4.16280009466872,5.33510865604686,48.5919108829142));
#21099=CARTESIAN_POINT('Ctrl Pts',(4.01615988349011,5.44952692272727,48.6006599135224));
#21100=CARTESIAN_POINT('Ctrl Pts',(3.86479978232465,5.55789587288463,48.6094089441307));
#21101=CARTESIAN_POINT('Ctrl Pts',(3.70923383581313,5.65984746713717,48.618157974739));
#21102=CARTESIAN_POINT('Ctrl Pts',(3.55366577799788,5.7618004450523,48.626907124087));
#21103=CARTESIAN_POINT('Ctrl Pts',(3.39389200027089,5.85733573570915,48.635656273435));
#21104=CARTESIAN_POINT('Ctrl Pts',(3.23045513626291,5.94612887621792,48.6444054227831));
#21105=CARTESIAN_POINT('Ctrl Pts',(3.18695122151745,5.969763992066,48.6467342868961));
#21106=CARTESIAN_POINT('Ctrl Pts',(3.14318791262746,5.99292165435291,48.6490631510091));
#21107=CARTESIAN_POINT('Ctrl Pts',(3.09917575053254,6.01559628526641,48.6513920151221));
#21108=CARTESIAN_POINT('Origin',(0.,0.,-3.69717978381041));
#21109=CARTESIAN_POINT('',(3.0991757505326,6.01559628526638,51.0457515827422));
#21110=CARTESIAN_POINT('',(3.09917575053255,6.01559628526641,50.6515095859174));
#21111=CARTESIAN_POINT('',(3.09917575053259,6.01559628526639,-3.69717978381041));
#21112=CARTESIAN_POINT('',(-6.767,6.11874741909821E-10,49.6971797837813));
#21113=CARTESIAN_POINT('Ctrl Pts',(-6.767,1.9002451714841E-12,49.69717978381));
#21114=CARTESIAN_POINT('Ctrl Pts',(-6.76700000000005,-0.186007249413768,
49.705929295616));
#21115=CARTESIAN_POINT('Ctrl Pts',(-6.75932637295449,-0.372014355525611,
49.7146788074219));
#21116=CARTESIAN_POINT('Ctrl Pts',(-6.74400518266944,-0.55738953715312,
49.7234283192279));
#21117=CARTESIAN_POINT('Ctrl Pts',(-6.72868405709666,-0.7427639358096,49.7321777940784));
#21118=CARTESIAN_POINT('Ctrl Pts',(-6.70571545653015,-0.927506129693374,
49.7409272689289));
#21119=CARTESIAN_POINT('Ctrl Pts',(-6.67517739415676,-1.11098863924823,
49.7496767437795));
#21120=CARTESIAN_POINT('Ctrl Pts',(-6.64463945823095,-1.2944703890653,49.7584261824015));
#21121=CARTESIAN_POINT('Ctrl Pts',(-6.60653217027148,-1.47669218228261,
49.7671756210235));
#21122=CARTESIAN_POINT('Ctrl Pts',(-6.56098496116696,-1.65703510504182,
49.7759250596455));
#21123=CARTESIAN_POINT('Ctrl Pts',(-6.515437936875,-1.83737729604082,49.7846744627657));
#21124=CARTESIAN_POINT('Ctrl Pts',(-6.4624511220262,-2.01584035397116,49.7934238658859));
#21125=CARTESIAN_POINT('Ctrl Pts',(-6.40220448416221,-2.19181813638206,
49.8021732690062));
#21126=CARTESIAN_POINT('Ctrl Pts',(-6.34195808575155,-2.36779521936031,
49.8109226373514));
#21127=CARTESIAN_POINT('Ctrl Pts',(-6.2744520148919,-2.54128677544938,49.8196720056967));
#21128=CARTESIAN_POINT('Ctrl Pts',(-6.19991555136125,-2.71170355237975,
49.828421374042));
#21129=CARTESIAN_POINT('Ctrl Pts',(-6.12537937788979,-2.88211966613198,
49.8371707083391));
#21130=CARTESIAN_POINT('Ctrl Pts',(-6.04381298133557,-3.04946076210563,
49.8459200426361));
#21131=CARTESIAN_POINT('Ctrl Pts',(-5.95549339426247,-3.21315848206964,
49.8546693769332));
#21132=CARTESIAN_POINT('Ctrl Pts',(-5.86717414355095,-3.3768555785975,49.8634186779087));
#21133=CARTESIAN_POINT('Ctrl Pts',(-5.77210188986166,-3.5369090746743,49.8721679788843));
#21134=CARTESIAN_POINT('Ctrl Pts',(-5.67059953466988,-3.69277536785027,
49.8809172798599));
#21135=CARTESIAN_POINT('Ctrl Pts',(-5.56909755761694,-3.84864108035896,
49.8896665482406));
#21136=CARTESIAN_POINT('Ctrl Pts',(-5.46116568338008,-4.00031938104363,
49.8984158166214));
#21137=CARTESIAN_POINT('Ctrl Pts',(-5.34717048686063,-4.14729511663284,
49.9071650850021));
#21138=CARTESIAN_POINT('Ctrl Pts',(-5.23317570555455,-4.29427031688118,
49.9159143215148));
#21139=CARTESIAN_POINT('Ctrl Pts',(-5.1131178217873,-4.43654275987217,49.9246635580274));
#21140=CARTESIAN_POINT('Ctrl Pts',(-4.98740459171925,-4.57362924147747,
49.93341279454));
#21141=CARTESIAN_POINT('Ctrl Pts',(-4.86169180910732,-4.71071523514538,
49.9421619999111));
#21142=CARTESIAN_POINT('Ctrl Pts',(-4.73032391415324,-4.84261509316629,
49.9509112052823));
#21143=CARTESIAN_POINT('Ctrl Pts',(-4.59374707237176,-4.96888084331632,
49.9596604106534));
#21144=CARTESIAN_POINT('Ctrl Pts',(-4.4571707053729,-5.09514615452822,49.9684095856096));
#21145=CARTESIAN_POINT('Ctrl Pts',(-4.31538563819403,-5.2157772025372,49.9771587605658));
#21146=CARTESIAN_POINT('Ctrl Pts',(-4.1688734129055,-5.33036429028727,49.985907935522));
#21147=CARTESIAN_POINT('Ctrl Pts',(-4.02236168477225,-5.44495098921261,
49.99465708079));
#21148=CARTESIAN_POINT('Ctrl Pts',(-3.8711230563431,-5.55349359238849,50.0034062260579));
#21149=CARTESIAN_POINT('Ctrl Pts',(-3.71567117316588,-5.65562346102568,
50.0121553713258));
#21150=CARTESIAN_POINT('Ctrl Pts',(-3.56021980457148,-5.75775299158864,
50.020904487632));
#21151=CARTESIAN_POINT('Ctrl Pts',(-3.40055544862227,-5.85346967275447,
50.0296536039382));
#21152=CARTESIAN_POINT('Ctrl Pts',(-3.23722036323235,-5.94244842803653,
50.0384027202443));
#21153=CARTESIAN_POINT('Ctrl Pts',(-3.07388580495869,-6.03142689616566,
50.0471518083153));
#21154=CARTESIAN_POINT('Ctrl Pts',(-2.9068807925752,-6.11366734484912,50.0559008963862));
#21155=CARTESIAN_POINT('Ctrl Pts',(-2.73677251094418,-6.18889046787389,
50.0646499844572));
#21156=CARTESIAN_POINT('Ctrl Pts',(-2.56666476416444,-6.26411335438353,
50.0733990450194));
#21157=CARTESIAN_POINT('Ctrl Pts',(-2.39345402971889,-6.33231884350368,
50.0821481055816));
#21158=CARTESIAN_POINT('Ctrl Pts',(-2.21772856473831,-6.39327529621115,
50.0908971661439));
#21159=CARTESIAN_POINT('Ctrl Pts',(-2.04200363768051,-6.45423156232151,
50.0996461999239));
#21160=CARTESIAN_POINT('Ctrl Pts',(-1.86376426619863,-6.50793874252122,
50.1083952337039));
#21161=CARTESIAN_POINT('Ctrl Pts',(-1.68361578194447,-6.55421443796185,
50.1171442674839));
#21162=CARTESIAN_POINT('Ctrl Pts',(-1.50346783419613,-6.60048999558738,
50.1258932752081));
#21163=CARTESIAN_POINT('Ctrl Pts',(-1.32141106256977,-6.63933404145549,
50.1346422829323));
#21164=CARTESIAN_POINT('Ctrl Pts',(-1.13806375958761,-6.67061465527078,
50.1433912906566));
#21165=CARTESIAN_POINT('Ctrl Pts',(-0.954716987415931,-6.70189517852527,
50.1521402730515));
#21166=CARTESIAN_POINT('Ctrl Pts',(-0.770079973806263,-6.7256122653587,
50.1608892554464));
#21167=CARTESIAN_POINT('Ctrl Pts',(-0.584779770548455,-6.74168536939817,
50.1696382378413));
#21168=CARTESIAN_POINT('Ctrl Pts',(-0.391490647549954,-6.75845143942417,
50.1787644185173));
#21169=CARTESIAN_POINT('Ctrl Pts',(-0.197480213100428,-6.76689975924038,
50.1878905991934));
#21170=CARTESIAN_POINT('Ctrl Pts',(-0.00346532629394415,-6.76699911271708,
50.1970167798694));
#21171=CARTESIAN_POINT('Ctrl Pts',(0.184486595299868,-6.76709536139763,
50.2058577673994));
#21172=CARTESIAN_POINT('Ctrl Pts',(0.372442378188994,-6.75935659726749,
50.2146987549293));
#21173=CARTESIAN_POINT('Ctrl Pts',(0.559750217725802,-6.74380965728986,
50.2235397424592));
#21174=CARTESIAN_POINT('Ctrl Pts',(0.745129914461395,-6.72842275717213,
50.232289721057));
#21175=CARTESIAN_POINT('Ctrl Pts',(0.92987465631775,-6.70538772273423,50.2410396996547));
#21176=CARTESIAN_POINT('Ctrl Pts',(1.11335688290126,-6.67478280180684,50.2497896782525));
#21177=CARTESIAN_POINT('Ctrl Pts',(1.29683723119203,-6.64417819417956,50.2585395672775));
#21178=CARTESIAN_POINT('Ctrl Pts',(1.47905480730579,-6.60600390229998,50.2672894563024));
#21179=CARTESIAN_POINT('Ctrl Pts',(1.65939064805149,-6.56038959797048,50.2760393453273));
#21180=CARTESIAN_POINT('Ctrl Pts',(1.83972470264602,-6.51477574543161,50.2847891476883));
#21181=CARTESIAN_POINT('Ctrl Pts',(2.01817678126181,-6.46172209819996,50.2935389500492));
#21182=CARTESIAN_POINT('Ctrl Pts',(2.19414072348009,-6.40140886723902,50.3022887524102));
#21183=CARTESIAN_POINT('Ctrl Pts',(2.37010298132424,-6.34109621361252,50.3110384710157));
#21184=CARTESIAN_POINT('Ctrl Pts',(2.54357687927237,-6.27352420825839,50.3197881896212));
#21185=CARTESIAN_POINT('Ctrl Pts',(2.71397317790293,-6.19892237325356,50.3285379082266));
#21186=CARTESIAN_POINT('Ctrl Pts',(2.88436790207529,-6.12432122756809,50.3372875459849));
#21187=CARTESIAN_POINT('Ctrl Pts',(3.0516848212659,-6.04269049717249,50.3460371837432));
#21188=CARTESIAN_POINT('Ctrl Pts',(3.21535561997727,-5.95430745234747,50.3547868215015));
#21189=CARTESIAN_POINT('Ctrl Pts',(3.37902496075602,-5.86592519481331,50.3635363813205));
#21190=CARTESIAN_POINT('Ctrl Pts',(3.53904799385179,-5.77079087940045,50.3722859411395));
#21191=CARTESIAN_POINT('Ctrl Pts',(3.69488118815271,-5.66922763746837,50.3810355009585));
#21192=CARTESIAN_POINT('Ctrl Pts',(3.85071304611117,-5.56766526648856,50.3897849857459));
#21193=CARTESIAN_POINT('Ctrl Pts',(4.00235489706248,-5.45967423580509,50.3985344705334));
#21194=CARTESIAN_POINT('Ctrl Pts',(4.1492916860793,-5.34562133936114,50.4072839553208));
#21195=CARTESIAN_POINT('Ctrl Pts',(4.29622726386022,-5.23156938308313,50.4160333679841));
#21196=CARTESIAN_POINT('Ctrl Pts',(4.43845763092321,-5.11145583676981,50.4247827806474));
#21197=CARTESIAN_POINT('Ctrl Pts',(4.57549970661206,-4.98568866203988,50.4335321933107));
#21198=CARTESIAN_POINT('Ctrl Pts',(4.71254069815535,-4.85992248225929,50.442281536757));
#21199=CARTESIAN_POINT('Ctrl Pts',(4.8443932693155,-4.7285029573376,50.4510308802033));
#21200=CARTESIAN_POINT('Ctrl Pts',(4.9706095943493,-4.59187644221431,50.4597802236497));
#21201=CARTESIAN_POINT('Ctrl Pts',(5.09682496280745,-4.45525096256402,50.468529500786));
#21202=CARTESIAN_POINT('Ctrl Pts',(5.21740397616065,-4.31341878218052,50.4772787779223));
#21203=CARTESIAN_POINT('Ctrl Pts',(5.33193710452157,-4.16686161438392,50.4860280550586));
#21204=CARTESIAN_POINT('Ctrl Pts',(5.44646940289602,-4.02030550864217,50.4947772687915));
#21205=CARTESIAN_POINT('Ctrl Pts',(5.5549557274988,-3.86902470979825,50.5035264825245));
#21206=CARTESIAN_POINT('Ctrl Pts',(5.65702762491666,-3.71353301465461,50.5122756962575));
#21207=CARTESIAN_POINT('Ctrl Pts',(5.75909881655357,-3.55804239466565,50.5210248494936));
#21208=CARTESIAN_POINT('Ctrl Pts',(5.85475551250977,-3.39834117619217,50.5297740027297));
#21209=CARTESIAN_POINT('Ctrl Pts',(5.94367283728282,-3.23497174691626,50.5385231559658));
#21210=CARTESIAN_POINT('Ctrl Pts',(6.03258957676485,-3.07160339300625,50.5472722516113));
#21211=CARTESIAN_POINT('Ctrl Pts',(6.11476689685444,-2.90456712829166,50.5560213472569));
#21212=CARTESIAN_POINT('Ctrl Pts',(6.18992570525408,-2.73443024475571,50.5647704429024));
#21213=CARTESIAN_POINT('Ctrl Pts',(6.26508404388836,-2.56429442462692,50.5735194838634));
#21214=CARTESIAN_POINT('Ctrl Pts',(6.33322384283444,-2.39105828655651,50.5822685248245));
#21215=CARTESIAN_POINT('Ctrl Pts',(6.39411368720152,-2.21531017131736,50.5910175657855));
#21216=CARTESIAN_POINT('Ctrl Pts',(6.45500317121003,-2.03956309619158,50.5997665549679));
#21217=CARTESIAN_POINT('Ctrl Pts',(6.50864269270179,-1.86130434438265,50.6085155441503));
#21218=CARTESIAN_POINT('Ctrl Pts',(6.55485008446431,-1.68113930719564,50.6172645333327));
#21219=CARTESIAN_POINT('Ctrl Pts',(6.60199664749489,-1.49731239211464,50.6261913468621));
#21220=CARTESIAN_POINT('Ctrl Pts',(6.6414056364098,-1.311501164993,50.6351181603914));
#21221=CARTESIAN_POINT('Ctrl Pts',(6.67293772282234,-1.12436255155295,50.6440449739208));
#21222=CARTESIAN_POINT('Ctrl Pts',(6.70384494949923,-0.940932395047674,
50.6527948880763));
#21223=CARTESIAN_POINT('Ctrl Pts',(6.72718449348972,-0.756227260503029,
50.6615448022319));
#21224=CARTESIAN_POINT('Ctrl Pts',(6.74287707373963,-0.570874564537995,
50.6702947163874));
#21225=CARTESIAN_POINT('Ctrl Pts',(6.75856934538691,-0.385525513628787,
50.6790444584714));
#21226=CARTESIAN_POINT('Ctrl Pts',(6.76661493004114,-0.199529212414554,
50.6877942005553));
#21227=CARTESIAN_POINT('Ctrl Pts',(6.76698649908907,-0.0135174385967701,
50.6965439426393));
#21228=CARTESIAN_POINT('Ctrl Pts',(6.7673580613238,0.172490924449449,50.7052935242852));
#21229=CARTESIAN_POINT('Ctrl Pts',(6.7600558889627,0.358514472905087,50.7140431059311));
#21230=CARTESIAN_POINT('Ctrl Pts',(6.74510478454555,0.543921359665896,50.722792687577));
#21231=CARTESIAN_POINT('Ctrl Pts',(6.73015393440647,0.729325093154176,50.7315421204161));
#21232=CARTESIAN_POINT('Ctrl Pts',(6.70755443556846,0.914111900260126,50.7402915532551));
#21233=CARTESIAN_POINT('Ctrl Pts',(6.67738304682256,1.09765415591919,50.7490409860941));
#21234=CARTESIAN_POINT('Ctrl Pts',(6.64721213111787,1.28119353391654,50.7577902817555));
#21235=CARTESIAN_POINT('Ctrl Pts',(6.6094696095541,1.46348811673033,50.7665395774168));
#21236=CARTESIAN_POINT('Ctrl Pts',(6.56428366991088,1.64391876348601,50.7752888730781));
#21237=CARTESIAN_POINT('Ctrl Pts',(6.51909837867613,1.8243468211009,50.784038043189));
#21238=CARTESIAN_POINT('Ctrl Pts',(6.46646995271807,2.00291071820813,50.7927872132998));
#21239=CARTESIAN_POINT('Ctrl Pts',(6.40657713281426,2.17900400213066,50.8015363834106));
#21240=CARTESIAN_POINT('Ctrl Pts',(6.34668509278925,2.35509499310022,50.8102854395964));
#21241=CARTESIAN_POINT('Ctrl Pts',(6.27952894037379,2.52871516398488,50.8190344957822));
#21242=CARTESIAN_POINT('Ctrl Pts',(6.20533675061288,2.69927486771786,50.8277835519679));
#21243=CARTESIAN_POINT('Ctrl Pts',(6.12832117907754,2.87632521636268,50.8368655532502));
#21244=CARTESIAN_POINT('Ctrl Pts',(6.04372366625915,3.05007728920321,50.8459475545325));
#21245=CARTESIAN_POINT('Ctrl Pts',(5.95185378007704,3.21989527478499,50.8550295558147));
#21246=CARTESIAN_POINT('Ctrl Pts',(5.86334450817198,3.38350129287052,50.8637793361218));
#21247=CARTESIAN_POINT('Ctrl Pts',(5.76808562057073,3.54345567125259,50.872529116429));
#21248=CARTESIAN_POINT('Ctrl Pts',(5.66640068804293,3.69921508465602,50.8812788967361));
#21249=CARTESIAN_POINT('Ctrl Pts',(5.56471941107724,3.85496889852571,50.8900283624896));
#21250=CARTESIAN_POINT('Ctrl Pts',(5.45661270814907,4.00652780919919,50.8987778282431));
#21251=CARTESIAN_POINT('Ctrl Pts',(5.342447764489,4.15337704569505,50.9075272939965));
#21252=CARTESIAN_POINT('Ctrl Pts',(5.2282863181937,4.30022178356523,50.9162764917161));
#21253=CARTESIAN_POINT('Ctrl Pts',(5.10806717843834,4.4423569097295,50.9250256894357));
#21254=CARTESIAN_POINT('Ctrl Pts',(4.98219864544473,4.57929969070913,50.9337748871553));
#21255=CARTESIAN_POINT('Ctrl Pts',(4.85633329943768,4.71623900430265,50.9425238633456));
#21256=CARTESIAN_POINT('Ctrl Pts',(4.72481904033381,4.84798602483877,50.9512728395358));
#21257=CARTESIAN_POINT('Ctrl Pts',(4.58810250736921,4.97409332259381,50.9600218157261));
#21258=CARTESIAN_POINT('Ctrl Pts',(4.45137708685352,5.10020881822388,50.9687713606622));
#21259=CARTESIAN_POINT('Ctrl Pts',(4.30944892635749,5.22068366308183,50.9775209055984));
#21260=CARTESIAN_POINT('Ctrl Pts',(4.16280009466346,5.33510865605096,50.9862704505346));
#21261=CARTESIAN_POINT('Ctrl Pts',(4.01615988348459,5.44952692273135,50.9950194811429));
#21262=CARTESIAN_POINT('Ctrl Pts',(3.86479978231886,5.55789587288866,51.0037685117512));
#21263=CARTESIAN_POINT('Ctrl Pts',(3.70923383580707,5.65984746714114,51.0125175423594));
#21264=CARTESIAN_POINT('Ctrl Pts',(3.55366577799171,5.7618004450561,51.0212666917075));
#21265=CARTESIAN_POINT('Ctrl Pts',(3.39389200026462,5.85733573571278,51.0300158410555));
#21266=CARTESIAN_POINT('Ctrl Pts',(3.23045513625655,5.94612887622138,51.0387649904035));
#21267=CARTESIAN_POINT('Ctrl Pts',(3.1869512215132,5.96976399206825,51.0410938545164));
#21268=CARTESIAN_POINT('Ctrl Pts',(3.14318791262535,5.99292165435399,51.0434227186293));
#21269=CARTESIAN_POINT('Ctrl Pts',(3.0991757505326,6.01559628526638,51.0457515827422));
#21270=CARTESIAN_POINT('Ctrl Pts',(3.0991757505326,6.01559628526638,49.0457515827422));
#21271=CARTESIAN_POINT('Ctrl Pts',(2.93382384459263,6.1007839529376,49.0545010306546));
#21272=CARTESIAN_POINT('Ctrl Pts',(2.76495772122979,6.17915010267052,49.063250478567));
#21273=CARTESIAN_POINT('Ctrl Pts',(2.59315093316703,6.25042856433181,49.0719999264794));
#21274=CARTESIAN_POINT('Ctrl Pts',(2.42134553245604,6.32170645041456,49.0807493037394));
#21275=CARTESIAN_POINT('Ctrl Pts',(2.24659977927573,6.38589665313464,49.0894986809994));
#21276=CARTESIAN_POINT('Ctrl Pts',(2.06950718689896,6.44278115439082,49.0982480582595));
#21277=CARTESIAN_POINT('Ctrl Pts',(1.8924159657284,6.4996652151973,49.1069973677741));
#21278=CARTESIAN_POINT('Ctrl Pts',(1.71297821457178,6.54924360009551,49.1157466772888));
#21279=CARTESIAN_POINT('Ctrl Pts',(1.53180337335826,6.5913479217356,49.1244959868034));
#21280=CARTESIAN_POINT('Ctrl Pts',(1.3506298747776,6.63345193135309,49.1332452314795));
#21281=CARTESIAN_POINT('Ctrl Pts',(1.16771959102925,6.66808192368243,49.1419944761557));
#21282=CARTESIAN_POINT('Ctrl Pts',(0.983693746906534,6.69512028363173,49.1507437208318));
#21283=CARTESIAN_POINT('Ctrl Pts',(0.79966920541951,6.72215845218871,49.159492903576));
#21284=CARTESIAN_POINT('Ctrl Pts',(0.614529402873065,6.74160505424583,49.1682420863201));
#21285=CARTESIAN_POINT('Ctrl Pts',(0.428903127362787,6.75339404354125,49.1769912690643));
#21286=CARTESIAN_POINT('Ctrl Pts',(0.24327810416352,6.76518295330331,49.1857403927829));
#21287=CARTESIAN_POINT('Ctrl Pts',(0.0571669005388619,6.76931433552276,
49.1944895165015));
#21288=CARTESIAN_POINT('Ctrl Pts',(-0.128798404777666,6.76577415902473,
49.2032386402201));
#21289=CARTESIAN_POINT('Ctrl Pts',(-0.314762517259134,6.76223400523441,
49.2119877078193));
#21290=CARTESIAN_POINT('Ctrl Pts',(-0.50058044681943,6.75102239665089,49.2207367754186));
#21291=CARTESIAN_POINT('Ctrl Pts',(-0.685621118842415,6.732177410125,49.2294858430178));
#21292=CARTESIAN_POINT('Ctrl Pts',(-0.870660665414357,6.71333253821774,
49.2382348574035));
#21293=CARTESIAN_POINT('Ctrl Pts',(-1.0549226788548,6.68685441030613,49.2469838717893));
#21294=CARTESIAN_POINT('Ctrl Pts',(-1.23778137635252,6.65283295028177,49.2557328861751));
#21295=CARTESIAN_POINT('Ctrl Pts',(-1.42999922977601,6.61707018862097,49.2649296965419));
#21296=CARTESIAN_POINT('Ctrl Pts',(-1.62066601231224,6.57297172934985,49.2741265069087));
#21297=CARTESIAN_POINT('Ctrl Pts',(-1.80906628496722,6.5207030431231,49.2833233172755));
#21298=CARTESIAN_POINT('Ctrl Pts',(-1.98831342541891,6.47097374916148,49.2920733150132));
#21299=CARTESIAN_POINT('Ctrl Pts',(-2.16550875893095,6.41384933990746,49.300823312751));
#21300=CARTESIAN_POINT('Ctrl Pts',(-2.34005036710439,6.34952386241792,49.3095733104888));
#21301=CARTESIAN_POINT('Ctrl Pts',(-2.5145884354355,6.28519968950012,49.3183231307696));
#21302=CARTESIAN_POINT('Ctrl Pts',(-2.68647261714554,6.21367483972613,49.3270729510505));
#21303=CARTESIAN_POINT('Ctrl Pts',(-2.85511905905272,6.13519226745454,49.3358227713314));
#21304=CARTESIAN_POINT('Ctrl Pts',(-3.02376230485472,6.0567111825464,49.3445724257899));
#21305=CARTESIAN_POINT('Ctrl Pts',(-3.18916767376544,5.97127275994428,49.3533220802484));
#21306=CARTESIAN_POINT('Ctrl Pts',(-3.35077334099482,5.8791672043988,49.362071734707));
#21307=CARTESIAN_POINT('Ctrl Pts',(-3.51237616034115,5.78706327197617,49.3708212349754));
#21308=CARTESIAN_POINT('Ctrl Pts',(-3.67017916299103,5.68829258364361,49.3795707352439));
#21309=CARTESIAN_POINT('Ctrl Pts',(-3.82364636563326,5.5831906174319,49.3883202355123));
#21310=CARTESIAN_POINT('Ctrl Pts',(-3.9771110677573,5.47809036369929,49.3970695932207));
#21311=CARTESIAN_POINT('Ctrl Pts',(-4.12623987478931,5.36665920045529,49.4058189509292));
#21312=CARTESIAN_POINT('Ctrl Pts',(-4.27052628211007,5.24927559514712,49.4145683086376));
#21313=CARTESIAN_POINT('Ctrl Pts',(-4.41481053022136,5.13189374645482,49.4233175354141));
#21314=CARTESIAN_POINT('Ctrl Pts',(-4.5542523013377,5.00855981479864,49.4320667621907));
#21315=CARTESIAN_POINT('Ctrl Pts',(-4.68837800627872,4.87969268194648,49.4408159889672));
#21316=CARTESIAN_POINT('Ctrl Pts',(-4.82250188226293,4.75082730634451,49.449565096438));
#21317=CARTESIAN_POINT('Ctrl Pts',(-4.95130963050442,4.61642907906233,49.4583142039089));
#21318=CARTESIAN_POINT('Ctrl Pts',(-5.07436379030924,4.47695444734459,49.4670633113798));
#21319=CARTESIAN_POINT('Ctrl Pts',(-5.1974164356044,4.33748153223421,49.4758123111695));
#21320=CARTESIAN_POINT('Ctrl Pts',(-5.31471544460488,4.19293255257486,49.4845613109592));
#21321=CARTESIAN_POINT('Ctrl Pts',(-5.42586245273424,4.04379841782559,49.493310310749));
#21322=CARTESIAN_POINT('Ctrl Pts',(-5.53702160017027,3.89464799487365,49.5020602660911));
#21323=CARTESIAN_POINT('Ctrl Pts',(-5.64202723079206,3.74091164446935,49.5108102214333));
#21324=CARTESIAN_POINT('Ctrl Pts',(-5.74052265231004,3.58311159166377,49.5195601767754));
#21325=CARTESIAN_POINT('Ctrl Pts',(-5.8390142706505,3.42531763194968,49.5283097942579));
#21326=CARTESIAN_POINT('Ctrl Pts',(-5.93099603113968,3.26346052698834,49.5370594117404));
#21327=CARTESIAN_POINT('Ctrl Pts',(-6.01615550621079,3.0980900447033,49.5458090292228));
#21328=CARTESIAN_POINT('Ctrl Pts',(-6.10131214577217,2.9327250686712,49.5545583553739));
#21329=CARTESIAN_POINT('Ctrl Pts',(-6.1796468232726,2.76384720420222,49.563307681525));
#21330=CARTESIAN_POINT('Ctrl Pts',(-6.25089348287171,2.59203002794952,49.5720570076761));
#21331=CARTESIAN_POINT('Ctrl Pts',(-6.32213814888022,2.42021765940446,49.5808060890077));
#21332=CARTESIAN_POINT('Ctrl Pts',(-6.38629508411364,2.24546640835389,49.5895551703392));
#21333=CARTESIAN_POINT('Ctrl Pts',(-6.44314639818681,2.06836976663565,49.5983042516708));
#21334=CARTESIAN_POINT('Ctrl Pts',(-6.50000285282666,1.89125711161829,49.6070541241052));
#21335=CARTESIAN_POINT('Ctrl Pts',(-6.54955227672314,1.71179891443835,49.6158039965396));
#21336=CARTESIAN_POINT('Ctrl Pts',(-6.59162635925548,1.53060476282034,49.624553868974));
#21337=CARTESIAN_POINT('Ctrl Pts',(-6.63369752054463,1.34942319168304,49.6333031338965));
#21338=CARTESIAN_POINT('Ctrl Pts',(-6.66829431423623,1.16650618646313,49.642052398819));
#21339=CARTESIAN_POINT('Ctrl Pts',(-6.69529923744888,0.982474997654602,
49.6508016637415));
#21340=CARTESIAN_POINT('Ctrl Pts',(-6.72230554731013,0.798434359213978,
49.6595513779212));
#21341=CARTESIAN_POINT('Ctrl Pts',(-6.74171916496372,0.613279706276726,
49.6683010921009));
#21342=CARTESIAN_POINT('Ctrl Pts',(-6.75347414817044,0.427639953691877,
49.6770508062806));
#21343=CARTESIAN_POINT('Ctrl Pts',(-6.76248837757382,0.285283364425952,
49.6837604654475));
#21344=CARTESIAN_POINT('Ctrl Pts',(-6.76699999998711,0.142641701524115,
49.6904701246144));
#21345=CARTESIAN_POINT('Ctrl Pts',(-6.767,6.11779405774452E-10,49.6971797837813));
#21346=CARTESIAN_POINT('',(-6.76699999998378,1.48178903510378E-5,49.3031392543722));
#21347=CARTESIAN_POINT('Ctrl Pts',(3.09917575053254,6.01559628526641,48.6513920151221));
#21348=CARTESIAN_POINT('Ctrl Pts',(2.9338238445926,6.10078395293762,48.6601414630345));
#21349=CARTESIAN_POINT('Ctrl Pts',(2.76495772122978,6.17915010267052,48.6688909109469));
#21350=CARTESIAN_POINT('Ctrl Pts',(2.59315093316705,6.2504285643318,48.6776403588593));
#21351=CARTESIAN_POINT('Ctrl Pts',(2.42134553245609,6.32170645041454,48.6863897361193));
#21352=CARTESIAN_POINT('Ctrl Pts',(2.24659977927581,6.38589665313461,48.6951391133793));
#21353=CARTESIAN_POINT('Ctrl Pts',(2.06950718689908,6.44278115439079,48.7038884906393));
#21354=CARTESIAN_POINT('Ctrl Pts',(1.89241596572848,6.49966521519728,48.712637800154));
#21355=CARTESIAN_POINT('Ctrl Pts',(1.71297821457183,6.5492436000955,48.7213871096686));
#21356=CARTESIAN_POINT('Ctrl Pts',(1.53180337335827,6.5913479217356,48.7301364191833));
#21357=CARTESIAN_POINT('Ctrl Pts',(1.35062987477764,6.63345193135308,48.7388856638594));
#21358=CARTESIAN_POINT('Ctrl Pts',(1.16771959102932,6.66808192368241,48.7476349085356));
#21359=CARTESIAN_POINT('Ctrl Pts',(0.983693746906633,6.69512028363171,48.7563841532117));
#21360=CARTESIAN_POINT('Ctrl Pts',(0.799669205419703,6.72215845218869,48.7651333359559));
#21361=CARTESIAN_POINT('Ctrl Pts',(0.614529402873353,6.7416050542458,48.7738825187));
#21362=CARTESIAN_POINT('Ctrl Pts',(0.42890312736317,6.75339404354123,48.7826317014442));
#21363=CARTESIAN_POINT('Ctrl Pts',(0.243278104163996,6.76518295330329,48.7913808251628));
#21364=CARTESIAN_POINT('Ctrl Pts',(0.0571669005394296,6.76931433552275,
48.8001299488814));
#21365=CARTESIAN_POINT('Ctrl Pts',(-0.128798404777005,6.76577415902474,
48.8088790726));
#21366=CARTESIAN_POINT('Ctrl Pts',(-0.314762517258572,6.76223400523444,
48.8176281401992));
#21367=CARTESIAN_POINT('Ctrl Pts',(-0.500580446818966,6.75102239665093,
48.8263772077984));
#21368=CARTESIAN_POINT('Ctrl Pts',(-0.68562111884205,6.73217741012503,48.8351262753976));
#21369=CARTESIAN_POINT('Ctrl Pts',(-0.870660665413836,6.7133325382178,48.8438752897834));
#21370=CARTESIAN_POINT('Ctrl Pts',(-1.05492267885412,6.68685441030623,48.8526243041692));
#21371=CARTESIAN_POINT('Ctrl Pts',(-1.23778137635169,6.65283295028193,48.8613733185549));
#21372=CARTESIAN_POINT('Ctrl Pts',(-1.4299992297877,6.61707018861882,48.8705701289223));
#21373=CARTESIAN_POINT('Ctrl Pts',(-1.62066601233624,6.57297172934431,48.8797669392897));
#21374=CARTESIAN_POINT('Ctrl Pts',(-1.8090662850032,6.52070304311312,48.8889637496571));
#21375=CARTESIAN_POINT('Ctrl Pts',(-1.98831342545458,6.47097374915052,48.8977137473949));
#21376=CARTESIAN_POINT('Ctrl Pts',(-2.16550875896629,6.41384933989553,48.9064637451326));
#21377=CARTESIAN_POINT('Ctrl Pts',(-2.34005036713935,6.34952386240504,48.9152137428704));
#21378=CARTESIAN_POINT('Ctrl Pts',(-2.51458843547014,6.28519968948626,48.9239635631513));
#21379=CARTESIAN_POINT('Ctrl Pts',(-2.68647261717981,6.21367483971131,48.9327133834321));
#21380=CARTESIAN_POINT('Ctrl Pts',(-2.85511905908659,6.13519226743878,48.941463203713));
#21381=CARTESIAN_POINT('Ctrl Pts',(-3.02376230488808,6.05671118252975,48.9502128581715));
#21382=CARTESIAN_POINT('Ctrl Pts',(-3.18916767379824,5.97127275992676,48.9589625126301));
#21383=CARTESIAN_POINT('Ctrl Pts',(-3.35077334102703,5.87916720438044,48.9677121670886));
#21384=CARTESIAN_POINT('Ctrl Pts',(-3.51237616037283,5.78706327195694,48.9764616673571));
#21385=CARTESIAN_POINT('Ctrl Pts',(-3.67017916302215,5.68829258362353,48.9852111676255));
#21386=CARTESIAN_POINT('Ctrl Pts',(-3.82364636566377,5.583190617411,48.9939606678939));
#21387=CARTESIAN_POINT('Ctrl Pts',(-3.97711106778711,5.47809036367765,49.0027100256024));
#21388=CARTESIAN_POINT('Ctrl Pts',(-4.12623987481839,5.36665920043293,49.0114593833108));
#21389=CARTESIAN_POINT('Ctrl Pts',(-4.2705262821384,5.24927559512408,49.0202087410192));
#21390=CARTESIAN_POINT('Ctrl Pts',(-4.41481053024908,5.13189374643098,49.0289579677958));
#21391=CARTESIAN_POINT('Ctrl Pts',(-4.55425230136478,5.00855981477402,49.0377071945723));
#21392=CARTESIAN_POINT('Ctrl Pts',(-4.68837800630512,4.87969268192111,49.0464564213488));
#21393=CARTESIAN_POINT('Ctrl Pts',(-4.82250188228871,4.75082730631834,49.0552055288197));
#21394=CARTESIAN_POINT('Ctrl Pts',(-4.95130963052954,4.61642907903539,49.0639546362905));
#21395=CARTESIAN_POINT('Ctrl Pts',(-5.07436379033366,4.47695444731691,49.0727037437614));
#21396=CARTESIAN_POINT('Ctrl Pts',(-5.19741643562795,4.33748153220598,49.0814527435511));
#21397=CARTESIAN_POINT('Ctrl Pts',(-5.31471544462755,4.19293255254612,49.0902017433408));
#21398=CARTESIAN_POINT('Ctrl Pts',(-5.42586245275602,4.04379841779637,49.0989507431306));
#21399=CARTESIAN_POINT('Ctrl Pts',(-5.53702160019123,3.89464799484385,49.1077006984727));
#21400=CARTESIAN_POINT('Ctrl Pts',(-5.64202723081217,3.74091164443901,49.1164506538149));
#21401=CARTESIAN_POINT('Ctrl Pts',(-5.74052265232929,3.58311159163293,49.125200609157));
#21402=CARTESIAN_POINT('Ctrl Pts',(-5.83901427066885,3.42531763191839,49.1339502266395));
#21403=CARTESIAN_POINT('Ctrl Pts',(-5.93099603115712,3.26346052695664,49.1426998441219));
#21404=CARTESIAN_POINT('Ctrl Pts',(-6.0161555062273,3.09809004467122,49.1514494616044));
#21405=CARTESIAN_POINT('Ctrl Pts',(-6.10131214578779,2.9327250686387,49.1601987877555));
#21406=CARTESIAN_POINT('Ctrl Pts',(-6.17964682328731,2.76384720416932,49.1689481139066));
#21407=CARTESIAN_POINT('Ctrl Pts',(-6.2508934828855,2.59203002791627,49.1776974400577));
#21408=CARTESIAN_POINT('Ctrl Pts',(-6.3221381488933,2.42021765937033,49.1864465213893));
#21409=CARTESIAN_POINT('Ctrl Pts',(-6.38629508412596,2.24546640831891,49.1951956027209));
#21410=CARTESIAN_POINT('Ctrl Pts',(-6.44314639819831,2.06836976659982,49.2039446840524));
#21411=CARTESIAN_POINT('Ctrl Pts',(-6.50000285283717,1.89125711158218,49.2126945564868));
#21412=CARTESIAN_POINT('Ctrl Pts',(-6.54955227673264,1.71179891440199,49.2214444289212));
#21413=CARTESIAN_POINT('Ctrl Pts',(-6.59162635926397,1.53060476278377,49.2301943013556));
#21414=CARTESIAN_POINT('Ctrl Pts',(-6.6336975205521,1.34942319164633,49.2389435662781));
#21415=CARTESIAN_POINT('Ctrl Pts',(-6.66829431424267,1.16650618642632,49.2476928312006));
#21416=CARTESIAN_POINT('Ctrl Pts',(-6.69529923745429,0.982474997617739,
49.2564420961231));
#21417=CARTESIAN_POINT('Ctrl Pts',(-6.72230554731453,0.798434359176932,
49.2651918103028));
#21418=CARTESIAN_POINT('Ctrl Pts',(-6.7417191649671,0.61327970623954,49.2739415244825));
#21419=CARTESIAN_POINT('Ctrl Pts',(-6.7534741481728,0.427639953654592,49.2826912386622));
#21420=CARTESIAN_POINT('Ctrl Pts',(-6.76248837758746,0.285283364198101,
49.2894008978381));
#21421=CARTESIAN_POINT('Ctrl Pts',(-6.76699999999996,0.14264170110496,49.296110557014));
#21422=CARTESIAN_POINT('Ctrl Pts',(-6.767,1.72760381084485E-12,49.3028202161899));
#21423=CARTESIAN_POINT('Ctrl Pts',(-6.76699999998378,1.48178903510378E-5,
49.3031392543722));
#21424=CARTESIAN_POINT('Ctrl Pts',(-6.76700037226677,-0.169998519403827,
49.3111672172146));
#21425=CARTESIAN_POINT('Ctrl Pts',(-6.76058934995979,-0.34027818884635,
49.3191951800569));
#21426=CARTESIAN_POINT('Ctrl Pts',(-6.74773259984795,-0.510287919658342,
49.3272231428992));
#21427=CARTESIAN_POINT('Ctrl Pts',(-6.73488877417485,-0.680126745666957,
49.3352430355128));
#21428=CARTESIAN_POINT('Ctrl Pts',(-6.71561214204822,-0.849695800879844,
49.3432629281264));
#21429=CARTESIAN_POINT('Ctrl Pts',(-6.68992035983133,-1.01845695987328,
49.3512828207401));
#21430=CARTESIAN_POINT('Ctrl Pts',(-6.66424869218064,-1.18708599266867,
49.3592964344331));
#21431=CARTESIAN_POINT('Ctrl Pts',(-6.63217192635893,-1.35490801784299,
49.3673100481261));
#21432=CARTESIAN_POINT('Ctrl Pts',(-6.59375966618062,-1.52138833459762,
49.3753236618191));
#21433=CARTESIAN_POINT('Ctrl Pts',(-6.55342219520463,-1.69621259419569,
49.3837389153931));
#21434=CARTESIAN_POINT('Ctrl Pts',(-6.50609782033658,-1.86955676459864,
49.3921541689672));
#21435=CARTESIAN_POINT('Ctrl Pts',(-6.4519283527089,-2.04081099847856,49.4005694225413));
#21436=CARTESIAN_POINT('Ctrl Pts',(-6.40038451205324,-2.20376443570606,
49.4085767836673));
#21437=CARTESIAN_POINT('Ctrl Pts',(-6.34264360673731,-2.36482535153571,
49.4165841447933));
#21438=CARTESIAN_POINT('Ctrl Pts',(-6.27887940922215,-2.52348219023754,
49.4245915059194));
#21439=CARTESIAN_POINT('Ctrl Pts',(-6.21511890076893,-2.68212984988709,
49.4325984037815));
#21440=CARTESIAN_POINT('Ctrl Pts',(-6.14533593344823,-2.83837335948393,
49.4406053016436));
#21441=CARTESIAN_POINT('Ctrl Pts',(-6.06975281374618,-2.99172020416688,
49.4486121995057));
#21442=CARTESIAN_POINT('Ctrl Pts',(-5.99415888392195,-3.14508898097084,
49.4566202425382));
#21443=CARTESIAN_POINT('Ctrl Pts',(-5.91276331761375,-3.29555993067592,
49.4646282855706));
#21444=CARTESIAN_POINT('Ctrl Pts',(-5.82583475976305,-3.4426644262746,49.472636328603));
#21445=CARTESIAN_POINT('Ctrl Pts',(-5.73887630095644,-3.58981952164332,
49.4806471261749));
#21446=CARTESIAN_POINT('Ctrl Pts',(-5.64638125516209,-3.73360553489412,
49.4886579237468));
#21447=CARTESIAN_POINT('Ctrl Pts',(-5.54866191440153,-3.87358231610869,
49.4966687213186));
#21448=CARTESIAN_POINT('Ctrl Pts',(-5.45083898367368,-4.01370748340604,
49.504688010948));
#21449=CARTESIAN_POINT('Ctrl Pts',(-5.34778091813517,-4.15001504905328,
49.5127073005773));
#21450=CARTESIAN_POINT('Ctrl Pts',(-5.23984105520187,-4.28209699986127,
49.5207265902067));
#21451=CARTESIAN_POINT('Ctrl Pts',(-5.13183455085293,-4.41426049726332,
49.5287508308967));
#21452=CARTESIAN_POINT('Ctrl Pts',(-5.01894049648163,-4.54219290453409,
49.5367750715868));
#21453=CARTESIAN_POINT('Ctrl Pts',(-4.90154905527637,-4.66552310665367,
49.5447993122769));
#21454=CARTESIAN_POINT('Ctrl Pts',(-4.78399975275928,-4.78901915619189,
49.5528343435079));
#21455=CARTESIAN_POINT('Ctrl Pts',(-4.66194126130477,-4.90790038788604,
49.560869374739));
#21456=CARTESIAN_POINT('Ctrl Pts',(-4.53579723218991,-5.0218355676444,49.5689044059701));
#21457=CARTESIAN_POINT('Ctrl Pts',(-4.49191601804543,-5.06146973865232,
49.5716995198457));
#21458=CARTESIAN_POINT('Ctrl Pts',(-4.44754067122288,-5.10050576622392,
49.5744946337214));
#21459=CARTESIAN_POINT('Ctrl Pts',(-4.40268982281328,-5.13893095148168,
49.577289747597));
#21460=CARTESIAN_POINT('Ctrl Pts',(-4.27069073999476,-5.25201887269187,
49.585515956934));
#21461=CARTESIAN_POINT('Ctrl Pts',(-4.13414715702875,-5.36017579829563,
49.5937421662709));
#21462=CARTESIAN_POINT('Ctrl Pts',(-3.99346254917625,-5.46301618781482,
49.6019683756079));
#21463=CARTESIAN_POINT('Ctrl Pts',(-3.85293599445357,-5.56574104056219,
49.6101853431511));
#21464=CARTESIAN_POINT('Ctrl Pts',(-3.70827796566465,-5.66316104117019,
49.6184023106943));
#21465=CARTESIAN_POINT('Ctrl Pts',(-3.55992683843884,-5.75492918331432,
49.6266192782375));
#21466=CARTESIAN_POINT('Ctrl Pts',(-3.41171260208985,-5.84661264648313,
49.6348286635809));
#21467=CARTESIAN_POINT('Ctrl Pts',(-3.2598123571534,-5.93265445006514,49.6430380489243));
#21468=CARTESIAN_POINT('Ctrl Pts',(-3.10469551541618,-6.01274935088389,
49.6512474342676));
#21469=CARTESIAN_POINT('Ctrl Pts',(-2.94969068441236,-6.09278641472968,
49.6594508915682));
#21470=CARTESIAN_POINT('Ctrl Pts',(-2.79147420044349,-6.16688496542816,
49.6676543488688));
#21471=CARTESIAN_POINT('Ctrl Pts',(-2.63054234718681,-6.23478435550556,
49.6758578061694));
#21472=CARTESIAN_POINT('Ctrl Pts',(-2.46969442118183,-6.30264833550667,
49.6840569853013));
#21473=CARTESIAN_POINT('Ctrl Pts',(-2.30613427663016,-6.3643194563415,49.6922561644331));
#21474=CARTESIAN_POINT('Ctrl Pts',(-2.14038064566728,-6.41958407466192,
49.7004553435649));
#21475=CARTESIAN_POINT('Ctrl Pts',(-1.97465824626051,-6.47483827993728,
49.7086529777947));
#21476=CARTESIAN_POINT('Ctrl Pts',(-1.8067435215996,-6.52368826794435,49.7168506120245));
#21477=CARTESIAN_POINT('Ctrl Pts',(-1.63717322747893,-6.56596929807216,
49.7250482462543));
#21478=CARTESIAN_POINT('Ctrl Pts',(-1.46761517312772,-6.60824727630894,
49.7332452887699));
#21479=CARTESIAN_POINT('Ctrl Pts',(-1.2964021351184,-6.64395715333708,49.7414423312855));
#21480=CARTESIAN_POINT('Ctrl Pts',(-1.12408395493887,-6.67298465922476,
49.7496393738011));
#21481=CARTESIAN_POINT('Ctrl Pts',(-0.951746894333704,-6.70201534557585,
49.757837314444));
#21482=CARTESIAN_POINT('Ctrl Pts',(-0.778304804087646,-6.72436214250033,
49.7660352550868));
#21483=CARTESIAN_POINT('Ctrl Pts',(-0.604315646037443,-6.73996228475756,
49.7742331957296));
#21484=CARTESIAN_POINT('Ctrl Pts',(-0.430275802121834,-6.75556697158941,
49.7824335245656));
#21485=CARTESIAN_POINT('Ctrl Pts',(-0.255688930114081,-6.76442105687205,
49.7906338534016));
#21486=CARTESIAN_POINT('Ctrl Pts',(-0.0811160685115168,-6.7665138131411,
49.7988341822376));
#21487=CARTESIAN_POINT('Ctrl Pts',(0.0936387025426088,-6.76860875011647,
49.807043056029));
#21488=CARTESIAN_POINT('Ctrl Pts',(0.268379074897014,-6.76392827796832,
49.8152519298204));
#21489=CARTESIAN_POINT('Ctrl Pts',(0.442545051686371,-6.75251381910677,
49.8234608036118));
#21490=CARTESIAN_POINT('Ctrl Pts',(0.616804501434506,-6.74109323423105,
49.8316740830152));
#21491=CARTESIAN_POINT('Ctrl Pts',(0.79048858467799,-6.72293149516101,49.8398873624187));
#21492=CARTESIAN_POINT('Ctrl Pts',(0.963044560249353,-6.6981216900691,49.8481006418221));
#21493=CARTESIAN_POINT('Ctrl Pts',(1.1358529260556,-6.67327559673789,49.8563259344376));
#21494=CARTESIAN_POINT('Ctrl Pts',(1.30752953393986,-6.6417620696749,49.864551227053));
#21495=CARTESIAN_POINT('Ctrl Pts',(1.47753267223525,-6.60372517617726,49.8727765196685));
#21496=CARTESIAN_POINT('Ctrl Pts',(1.63128008929183,-6.56932537516913,49.8802153087805));
#21497=CARTESIAN_POINT('Ctrl Pts',(1.78365876575744,-6.52959079986507,49.8876540978925));
#21498=CARTESIAN_POINT('Ctrl Pts',(1.93428095369982,-6.48466238073765,49.8950928870045));
#21499=CARTESIAN_POINT('Ctrl Pts',(2.10084682581374,-6.43497819133045,49.9033190880233));
#21500=CARTESIAN_POINT('Ctrl Pts',(2.26572998687126,-6.37880278601693,49.9115452890422));
#21501=CARTESIAN_POINT('Ctrl Pts',(2.42838779218591,-6.31626643918403,49.919771490061));
#21502=CARTESIAN_POINT('Ctrl Pts',(2.59086288573823,-6.25380033875656,49.9279884506768));
#21503=CARTESIAN_POINT('Ctrl Pts',(2.75111726945716,-6.18498765233058,49.9362054112926));
#21504=CARTESIAN_POINT('Ctrl Pts',(2.9086217813601,-6.11000886521432,49.9444223719083));
#21505=CARTESIAN_POINT('Ctrl Pts',(3.06598098254605,-6.03509925212478,49.9526317517099));
#21506=CARTESIAN_POINT('Ctrl Pts',(3.22059504262432,-5.95403502084389,49.9608411315115));
#21507=CARTESIAN_POINT('Ctrl Pts',(3.37195308983396,-5.86704536883423,49.9690505113131));
#21508=CARTESIAN_POINT('Ctrl Pts',(3.52320186595561,-5.78011851793818,49.9772539644535));
#21509=CARTESIAN_POINT('Ctrl Pts',(3.67119900159623,-5.68727494490937,49.9854574175939));
#21510=CARTESIAN_POINT('Ctrl Pts',(3.81545655206118,-5.58879059361983,49.9936608707343));
#21511=CARTESIAN_POINT('Ctrl Pts',(3.95963889525941,-5.49035758618611,50.0018600470844));
#21512=CARTESIAN_POINT('Ctrl Pts',(4.10008524173568,-5.38628986074918,50.0100592234346));
#21513=CARTESIAN_POINT('Ctrl Pts',(4.23633499460492,-5.27690769423587,50.0182583997847));
#21514=CARTESIAN_POINT('Ctrl Pts',(4.3725591100272,-5.16754610962774,50.0264560333361));
#21515=CARTESIAN_POINT('Ctrl Pts',(4.50458792147498,-5.05287229525539,50.0346536668875));
#21516=CARTESIAN_POINT('Ctrl Pts',(4.63199217272379,-4.93324817050851,50.0428513004388));
#21517=CARTESIAN_POINT('Ctrl Pts',(4.75938724773965,-4.81363266163453,50.0510483435594));
#21518=CARTESIAN_POINT('Ctrl Pts',(4.88215816381982,-4.68906779733273,50.05924538668));
#21519=CARTESIAN_POINT('Ctrl Pts',(4.9999109985639,-4.55995383819176,50.0674424298005));
#21520=CARTESIAN_POINT('Ctrl Pts',(5.11767675359486,-4.43082571217832,50.0756403723317));
#21521=CARTESIAN_POINT('Ctrl Pts',(5.23042308858188,-4.29714776195844,50.0838383148629));
#21522=CARTESIAN_POINT('Ctrl Pts',(5.33779497401187,-4.15935497588432,50.0920362573941));
#21523=CARTESIAN_POINT('Ctrl Pts',(5.44519815542578,-4.02152202696123,50.1002365894025));
#21524=CARTESIAN_POINT('Ctrl Pts',(5.54722354658387,-3.87957213605305,50.1084369214109));
#21525=CARTESIAN_POINT('Ctrl Pts',(5.64355819131297,-3.7339710686164,50.1166372534193));
#21526=CARTESIAN_POINT('Ctrl Pts',(5.7399932427791,-3.58821824551458,50.1248461323901));
#21527=CARTESIAN_POINT('Ctrl Pts',(5.83072549980653,-3.43880694257282,50.1330550113609));
#21528=CARTESIAN_POINT('Ctrl Pts',(5.91548640475926,-3.28623030159306,50.1412638903316));
#21529=CARTESIAN_POINT('Ctrl Pts',(6.00029281133168,-3.13357175393362,50.149477176019));
#21530=CARTESIAN_POINT('Ctrl Pts',(6.07912131368349,-2.97774480051613,50.1576904617064));
#21531=CARTESIAN_POINT('Ctrl Pts',(6.15175071231138,-2.8192644738613,50.1659037473938));
#21532=CARTESIAN_POINT('Ctrl Pts',(6.22448635879819,-2.66055231002063,50.1741290481059));
#21533=CARTESIAN_POINT('Ctrl Pts',(6.29100464202356,-2.49917934749279,50.1823543488179));
#21534=CARTESIAN_POINT('Ctrl Pts',(6.35113318783342,-2.33567896561169,50.19057964953));
#21535=CARTESIAN_POINT('Ctrl Pts',(6.40551220434368,-2.18781259289312,50.1980184418241));
#21536=CARTESIAN_POINT('Ctrl Pts',(6.45466563267677,-2.0382065863057,50.2054572341182));
#21537=CARTESIAN_POINT('Ctrl Pts',(6.49850187116025,-1.88726321177699,50.2128960264123));
#21538=CARTESIAN_POINT('Ctrl Pts',(6.54654426625421,-1.72183658105326,50.2210485826255));
#21539=CARTESIAN_POINT('Ctrl Pts',(6.58834100216934,-1.55431554506159,50.2292011388388));
#21540=CARTESIAN_POINT('Ctrl Pts',(6.62370465993362,-1.38521679818492,50.237353695052));
#21541=CARTESIAN_POINT('Ctrl Pts',(6.6590273480479,-1.21631395628283,50.2454968063324));
#21542=CARTESIAN_POINT('Ctrl Pts',(6.6879317196072,-1.04583739610205,50.2536399176127));
#21543=CARTESIAN_POINT('Ctrl Pts',(6.71027965269082,-0.874320297536072,
50.2617830288931));
#21544=CARTESIAN_POINT('Ctrl Pts',(6.73260639352983,-0.702965846329679,
50.2699184181704));
#21545=CARTESIAN_POINT('Ctrl Pts',(6.7483890269995,-0.530573181193096,50.2780538074478));
#21546=CARTESIAN_POINT('Ctrl Pts',(6.75754015748445,-0.357687041958609,
50.2861891967251));
#21547=CARTESIAN_POINT('Ctrl Pts',(6.76668453294861,-0.184928520778165,
50.2943185807637));
#21548=CARTESIAN_POINT('Ctrl Pts',(6.76920713324293,-0.0116776143251095,
50.3024479648023));
#21549=CARTESIAN_POINT('Ctrl Pts',(6.76507221624997,0.161514423265437,50.3105773488409));
#21550=CARTESIAN_POINT('Ctrl Pts',(6.76093948296706,0.334614995611171,50.318702439633));
#21551=CARTESIAN_POINT('Ctrl Pts',(6.75015624322899,0.507656396368457,50.3268275304251));
#21552=CARTESIAN_POINT('Ctrl Pts',(6.73273882396683,0.680085971219667,50.3349526212172));
#21553=CARTESIAN_POINT('Ctrl Pts',(6.71525491863941,0.853173747139149,50.3431087272423));
#21554=CARTESIAN_POINT('Ctrl Pts',(6.69108607376356,1.02564464489716,50.3512648332674));
#21555=CARTESIAN_POINT('Ctrl Pts',(6.66030154434002,1.19694291361867,50.3594209392925));
#21556=CARTESIAN_POINT('Ctrl Pts',(6.62964091707995,1.36755173778832,50.367544218466));
#21557=CARTESIAN_POINT('Ctrl Pts',(6.59241784662351,1.53699699592338,50.3756674976394));
#21558=CARTESIAN_POINT('Ctrl Pts',(6.54875227082131,1.70473830701746,50.3837907768128));
#21559=CARTESIAN_POINT('Ctrl Pts',(6.50508088057863,1.87250195428485,50.3919151376695));
#21560=CARTESIAN_POINT('Ctrl Pts',(6.45496536843223,2.03856084851579,50.4000394985262));
#21561=CARTESIAN_POINT('Ctrl Pts',(6.39857595315297,2.20238842435493,50.4081638593829));
#21562=CARTESIAN_POINT('Ctrl Pts',(6.34216830077025,2.36626898425916,50.4162908477683));
#21563=CARTESIAN_POINT('Ctrl Pts',(6.2794828237427,2.5279164430318,50.4244178361537));
#21564=CARTESIAN_POINT('Ctrl Pts',(6.21073839413157,2.68682295651575,50.4325448245392));
#21565=CARTESIAN_POINT('Ctrl Pts',(6.14154953960981,2.84675678251727,50.4407243529792));
#21566=CARTESIAN_POINT('Ctrl Pts',(6.06622326924259,3.00391375563312,50.4489038814193));
#21567=CARTESIAN_POINT('Ctrl Pts',(5.98502988923725,3.15780085264045,50.4570834098594));
#21568=CARTESIAN_POINT('Ctrl Pts',(5.90421887503382,3.31096324569722,50.465224418263));
#21569=CARTESIAN_POINT('Ctrl Pts',(5.81759613095532,3.46088620999193,50.4733654266667));
#21570=CARTESIAN_POINT('Ctrl Pts',(5.72547174231819,3.60711274122614,50.4815064350704));
#21571=CARTESIAN_POINT('Ctrl Pts',(5.63269350934899,3.75437710174812,50.4897052235287));
#21572=CARTESIAN_POINT('Ctrl Pts',(5.53433546335785,3.89789205475113,50.4979040119869));
#21573=CARTESIAN_POINT('Ctrl Pts',(5.43075535893094,4.03722494189299,50.5061028004452));
#21574=CARTESIAN_POINT('Ctrl Pts',(5.32717525450403,4.17655782903485,50.5143015889034));
#21575=CARTESIAN_POINT('Ctrl Pts',(5.21837337498346,4.31170840166453,50.5225003773617));
#21576=CARTESIAN_POINT('Ctrl Pts',(5.10474461150638,4.44228223453852,50.5306991658199));
#21577=CARTESIAN_POINT('Ctrl Pts',(4.99061989257435,4.57342598301052,50.5389337395295));
#21578=CARTESIAN_POINT('Ctrl Pts',(4.87127132453099,4.70036077080625,50.5471683132391));
#21579=CARTESIAN_POINT('Ctrl Pts',(4.74704009445691,4.82264443450049,50.5554028869487));
#21580=CARTESIAN_POINT('Ctrl Pts',(4.62299741549927,4.94474250298411,50.5636249626892));
#21581=CARTESIAN_POINT('Ctrl Pts',(4.49408709554759,5.06220326617622,50.5718470384298));
#21582=CARTESIAN_POINT('Ctrl Pts',(4.36069029164882,5.17461778108487,50.5800691141703));
#21583=CARTESIAN_POINT('Ctrl Pts',(4.22740969371894,5.28693436832779,50.5882840274133));
#21584=CARTESIAN_POINT('Ctrl Pts',(4.08965066291297,5.39421322799149,50.5964989406564));
#21585=CARTESIAN_POINT('Ctrl Pts',(3.94783148302989,5.49608183905572,50.6047138538994));
#21586=CARTESIAN_POINT('Ctrl Pts',(3.80613172030727,5.5978646728627,50.612921849872));
#21587=CARTESIAN_POINT('Ctrl Pts',(3.66037890926252,5.69424612619518,50.6211298458447));
#21588=CARTESIAN_POINT('Ctrl Pts',(3.51102457414039,5.78489372761353,50.6293378418173));
#21589=CARTESIAN_POINT('Ctrl Pts',(3.37654407855222,5.86651395211287,50.636728423184));
#21590=CARTESIAN_POINT('Ctrl Pts',(3.23914426110165,5.94348589201141,50.6441190045507));
#21591=CARTESIAN_POINT('Ctrl Pts',(3.09917575053255,6.01559628526641,50.6515095859174));
#21592=CARTESIAN_POINT('Origin',(0.,0.,-3.69717978381041));
#21593=CARTESIAN_POINT('',(3.09917575053258,6.01559628526639,53.0455807084606));
#21594=CARTESIAN_POINT('',(3.09917575053253,6.01559628526642,52.6511649350805));
#21595=CARTESIAN_POINT('',(3.09917575053259,6.01559628526639,-3.69717978381041));
#21596=CARTESIAN_POINT('',(-6.76699995210602,-0.000805106932658668,51.69717978381));
#21597=CARTESIAN_POINT('Ctrl Pts',(-6.76699995210602,-0.000805106932658668,
51.69717978381));
#21598=CARTESIAN_POINT('Ctrl Pts',(-6.76697776002256,-0.187331668327564,
51.7059085008878));
#21599=CARTESIAN_POINT('Ctrl Pts',(-6.75923913773472,-0.373667474836227,
51.7146372179655));
#21600=CARTESIAN_POINT('Ctrl Pts',(-6.74385683031687,-0.55918159142499,
51.7233659350433));
#21601=CARTESIAN_POINT('Ctrl Pts',(-6.72844715360874,-0.745025787862566,
51.7321101828724));
#21602=CARTESIAN_POINT('Ctrl Pts',(-6.70536664484977,-0.930045094505219,
51.7408544307015));
#21603=CARTESIAN_POINT('Ctrl Pts',(-6.67473938789428,-1.11361712616714,
51.7495986785305));
#21604=CARTESIAN_POINT('Ctrl Pts',(-6.64402544099753,-1.29770875541049,
51.7583676768076));
#21605=CARTESIAN_POINT('Ctrl Pts',(-6.60572205444346,-1.48034463564412,
51.7671366750847));
#21606=CARTESIAN_POINT('Ctrl Pts',(-6.56000430699961,-1.66091315009141,
51.7759056733618));
#21607=CARTESIAN_POINT('Ctrl Pts',(-6.51422000550895,-1.84174452887551,
51.7846874371918));
#21608=CARTESIAN_POINT('Ctrl Pts',(-6.46099986358177,-2.02050226191529,
51.7934692010217));
#21609=CARTESIAN_POINT('Ctrl Pts',(-6.40056811135066,-2.19659209958543,
51.8022509648517));
#21610=CARTESIAN_POINT('Ctrl Pts',(-6.33999002914278,-2.37310832273842,
51.8110539929219));
#21611=CARTESIAN_POINT('Ctrl Pts',(-6.27216550584455,-2.54694346518936,
51.8198570209921));
#21612=CARTESIAN_POINT('Ctrl Pts',(-6.19736705102892,-2.71752288579529,
51.8286600490622));
#21613=CARTESIAN_POINT('Ctrl Pts',(-6.14343480472519,-2.84051648705539,
51.8350073336321));
#21614=CARTESIAN_POINT('Ctrl Pts',(-6.08587786014791,-2.96181796013422,
51.8413546182019));
#21615=CARTESIAN_POINT('Ctrl Pts',(-6.0248127130065,-3.08122066285349,51.8477019027718));
#21616=CARTESIAN_POINT('Ctrl Pts',(-5.94639478163091,-3.23455383875197,
51.8558528849461));
#21617=CARTESIAN_POINT('Ctrl Pts',(-5.86199628252426,-3.38513229218628,
51.8640038671204));
#21618=CARTESIAN_POINT('Ctrl Pts',(-5.77183468666551,-3.5324514646071,51.8721548492947));
#21619=CARTESIAN_POINT('Ctrl Pts',(-5.68177782185669,-3.67959951215535,
51.8802963633477));
#21620=CARTESIAN_POINT('Ctrl Pts',(-5.5859713748947,-3.82349550620328,51.8884378774007));
#21621=CARTESIAN_POINT('Ctrl Pts',(-5.48468001845993,-3.96365665706635,
51.8965793914538));
#21622=CARTESIAN_POINT('Ctrl Pts',(-5.38348500590702,-4.10368449280921,
51.9047131616569));
#21623=CARTESIAN_POINT('Ctrl Pts',(-5.27681568289663,-4.23998426334832,
51.9128469318599));
#21624=CARTESIAN_POINT('Ctrl Pts',(-5.1649815891154,-4.3720995167195,51.920980702063));
#21625=CARTESIAN_POINT('Ctrl Pts',(-5.05323034599209,-4.50411689443139,
51.929108446481));
#21626=CARTESIAN_POINT('Ctrl Pts',(-4.93632218602984,-4.63195564968424,
51.937236190899));
#21627=CARTESIAN_POINT('Ctrl Pts',(-4.81460873288302,-4.75518998035269,
51.945363935317));
#21628=CARTESIAN_POINT('Ctrl Pts',(-4.69295986003724,-4.87835892375318,
51.953487367211));
#21629=CARTESIAN_POINT('Ctrl Pts',(-4.56651102810959,-4.99692804838911,
51.9616107991051));
#21630=CARTESIAN_POINT('Ctrl Pts',(-4.43565274173749,-5.11050621315704,
51.9697342309991));
#21631=CARTESIAN_POINT('Ctrl Pts',(-4.303964341867,-5.22480487312867,51.9779091947499));
#21632=CARTESIAN_POINT('Ctrl Pts',(-4.16781059763206,-5.33404875060903,
51.9860841585008));
#21633=CARTESIAN_POINT('Ctrl Pts',(-4.02762598954331,-5.43787806854432,
51.9942591222516));
#21634=CARTESIAN_POINT('Ctrl Pts',(-3.88835665086666,-5.54102948182173,
52.0023807114246));
#21635=CARTESIAN_POINT('Ctrl Pts',(-3.74510924011445,-5.63883662977525,
52.0105023005976));
#21636=CARTESIAN_POINT('Ctrl Pts',(-3.59834138050517,-5.73098842341739,
52.0186238897707));
#21637=CARTESIAN_POINT('Ctrl Pts',(-3.45155414452848,-5.82315238298616,
52.0267465511601));
#21638=CARTESIAN_POINT('Ctrl Pts',(-3.30124584393747,-5.90965930647105,
52.0348692125494));
#21639=CARTESIAN_POINT('Ctrl Pts',(-3.14790123780602,-5.99024263256667,
52.0429918739388));
#21640=CARTESIAN_POINT('Ctrl Pts',(-2.99450718569254,-6.07085194276305,
52.051117154481));
#21641=CARTESIAN_POINT('Ctrl Pts',(-2.83807520224387,-6.14553368188226,
52.0592424350233));
#21642=CARTESIAN_POINT('Ctrl Pts',(-2.67911263257415,-6.21406827303833,
52.0673677155656));
#21643=CARTESIAN_POINT('Ctrl Pts',(-2.51841819869326,-6.28334953434384,
52.0755815193533));
#21644=CARTESIAN_POINT('Ctrl Pts',(-2.35513806783831,-6.3463487670734,52.0837953231411));
#21645=CARTESIAN_POINT('Ctrl Pts',(-2.18981398807035,-6.40289026125323,
52.0920091269288));
#21646=CARTESIAN_POINT('Ctrl Pts',(-2.02598866772291,-6.45891917373793,
52.100148467784));
#21647=CARTESIAN_POINT('Ctrl Pts',(-1.86015667324503,-6.50860690949064,
52.1082878086392));
#21648=CARTESIAN_POINT('Ctrl Pts',(-1.69285694530543,-6.5518336641532,52.1164271494943));
#21649=CARTESIAN_POINT('Ctrl Pts',(-1.52326139969761,-6.5956536101396,52.1246781847484));
#21650=CARTESIAN_POINT('Ctrl Pts',(-1.35215792933208,-6.63283388052945,
52.1329292200024));
#21651=CARTESIAN_POINT('Ctrl Pts',(-1.18011453005237,-6.66330388740895,
52.1411802552564));
#21652=CARTESIAN_POINT('Ctrl Pts',(-1.00807113077267,-6.69377389428846,
52.1494312905105));
#21653=CARTESIAN_POINT('Ctrl Pts',(-0.835088192012403,-6.71753365186203,
52.1576823257645));
#21654=CARTESIAN_POINT('Ctrl Pts',(-0.661734484834696,-6.73456728168786,
52.1659333610185));
#21655=CARTESIAN_POINT('Ctrl Pts',(-0.488785496707557,-6.75156114406595,
52.1741651330494));
#21656=CARTESIAN_POINT('Ctrl Pts',(-0.314927570707862,-6.76191347781179,
52.1823969050802));
#21657=CARTESIAN_POINT('Ctrl Pts',(-0.140711821677379,-6.76553687324519,
52.190628677111));
#21658=CARTESIAN_POINT('Ctrl Pts',(0.0332958963387049,-6.76915594198233,
52.1988506195834));
#21659=CARTESIAN_POINT('Ctrl Pts',(0.207660231874101,-6.76606206461893,
52.2070725620558));
#21660=CARTESIAN_POINT('Ctrl Pts',(0.381823245449463,-6.75621935769069,
52.2152945045282));
#21661=CARTESIAN_POINT('Ctrl Pts',(0.555813186072828,-6.74638643186528,
52.2235082765181));
#21662=CARTESIAN_POINT('Ctrl Pts',(0.729601847885147,-6.72981805269848,
52.231722048508));
#21663=CARTESIAN_POINT('Ctrl Pts',(0.902629477736182,-6.70653032692179,
52.2399358204979));
#21664=CARTESIAN_POINT('Ctrl Pts',(1.07551981792611,-6.68326107891067,52.2481430752283));
#21665=CARTESIAN_POINT('Ctrl Pts',(1.24764997537319,-6.65328315106042,52.2563503299586));
#21666=CARTESIAN_POINT('Ctrl Pts',(1.41846341614987,-6.61666460817264,52.264557584689));
#21667=CARTESIAN_POINT('Ctrl Pts',(1.58917552675394,-6.58006778818474,52.2727599707009));
#21668=CARTESIAN_POINT('Ctrl Pts',(1.75857212732575,-6.53683827572664,52.2809623567129));
#21669=CARTESIAN_POINT('Ctrl Pts',(1.92610490867979,-6.48709556587227,52.2891647427249));
#21670=CARTESIAN_POINT('Ctrl Pts',(2.09358768556224,-6.43736770301023,52.2973646805236));
#21671=CARTESIAN_POINT('Ctrl Pts',(2.25920740719941,-6.38113061332355,52.3055646183223));
#21672=CARTESIAN_POINT('Ctrl Pts',(2.4224287672088,-6.31855425455849,52.313764556121));
#21673=CARTESIAN_POINT('Ctrl Pts',(2.58562730465929,-6.25598664558351,52.3219633473567));
#21674=CARTESIAN_POINT('Ctrl Pts',(2.74642781353569,-6.18708166040106,52.3301621385925));
#21675=CARTESIAN_POINT('Ctrl Pts',(2.90431287157553,-6.11205822485362,52.3383609298282));
#21676=CARTESIAN_POINT('Ctrl Pts',(3.06220449437847,-6.0370316698781,52.3465600619647));
#21677=CARTESIAN_POINT('Ctrl Pts',(3.21718010105147,-5.95588631147893,52.3547591941011));
#21678=CARTESIAN_POINT('Ctrl Pts',(3.36874482540485,-5.86888808048919,52.3629583262375));
#21679=CARTESIAN_POINT('Ctrl Pts',(3.52034334625225,-5.78187045029421,52.3711592866484));
#21680=CARTESIAN_POINT('Ctrl Pts',(3.66852915914536,-5.68899752652939,52.3793602470593));
#21681=CARTESIAN_POINT('Ctrl Pts',(3.81283440679735,-5.59057982559433,52.3875612074702));
#21682=CARTESIAN_POINT('Ctrl Pts',(3.95727490320491,-5.49206988358146,52.3957698541553));
#21683=CARTESIAN_POINT('Ctrl Pts',(4.09782727131412,-5.38800498374804,52.4039785008403));
#21684=CARTESIAN_POINT('Ctrl Pts',(4.23405416241301,-5.27873795047198,52.4121871475253));
#21685=CARTESIAN_POINT('Ctrl Pts',(4.37034609205585,-5.1694187500453,52.4203997132489));
#21686=CARTESIAN_POINT('Ctrl Pts',(4.50230815666514,-5.05489269901851,52.4286122789724));
#21687=CARTESIAN_POINT('Ctrl Pts',(4.62953829304672,-4.93555105263983,52.4368248446959));
#21688=CARTESIAN_POINT('Ctrl Pts',(4.75694300753476,-4.81604565230128,52.4450486792446));
#21689=CARTESIAN_POINT('Ctrl Pts',(4.87960256561733,-4.69171170605568,52.4532725137934));
#21690=CARTESIAN_POINT('Ctrl Pts',(4.99715294271958,-4.56297616332466,52.4614963483422));
#21691=CARTESIAN_POINT('Ctrl Pts',(5.10515962701359,-4.44469241584614,52.4690525053167));
#21692=CARTESIAN_POINT('Ctrl Pts',(5.20885338823642,-4.32269332652127,52.4766086622911));
#21693=CARTESIAN_POINT('Ctrl Pts',(5.30798369569739,-4.1973322582577,52.4841648192656));
#21694=CARTESIAN_POINT('Ctrl Pts',(5.42140811126335,-4.05389473378399,52.492810537318));
#21695=CARTESIAN_POINT('Ctrl Pts',(5.52911641506232,-3.90572865115852,52.5014562553704));
#21696=CARTESIAN_POINT('Ctrl Pts',(5.63071799218921,-3.75330572861268,52.5101019734228));
#21697=CARTESIAN_POINT('Ctrl Pts',(5.73218913359683,-3.60107848603656,52.5187365921351));
#21698=CARTESIAN_POINT('Ctrl Pts',(5.82756901293679,-3.44460555341883,52.5273712108475));
#21699=CARTESIAN_POINT('Ctrl Pts',(5.91650808941616,-3.284390510867,52.5360058295599));
#21700=CARTESIAN_POINT('Ctrl Pts',(6.00858814857537,-3.11851729539922,52.5449453894623));
#21701=CARTESIAN_POINT('Ctrl Pts',(6.09376395189131,-2.94863306633431,52.5538849493647));
#21702=CARTESIAN_POINT('Ctrl Pts',(6.17169573986025,-2.77533073607288,52.5628245092671));
#21703=CARTESIAN_POINT('Ctrl Pts',(6.24676024105247,-2.60840459058642,52.5714351625376));
#21704=CARTESIAN_POINT('Ctrl Pts',(6.31510408129153,-2.43830767506642,52.5800458158081));
#21705=CARTESIAN_POINT('Ctrl Pts',(6.37646938595806,-2.26559642697891,52.5886564690786));
#21706=CARTESIAN_POINT('Ctrl Pts',(6.43777660425816,-2.09304866164275,52.5972589717897));
#21707=CARTESIAN_POINT('Ctrl Pts',(6.49211835510333,-1.91789178395019,52.6058614745008));
#21708=CARTESIAN_POINT('Ctrl Pts',(6.53928460601878,-1.74070268612588,52.6144639772119));
#21709=CARTESIAN_POINT('Ctrl Pts',(6.58639777226828,-1.56371301106435,52.6230567979794));
#21710=CARTESIAN_POINT('Ctrl Pts',(6.62635147144205,-1.38469597291436,52.6316496187469));
#21711=CARTESIAN_POINT('Ctrl Pts',(6.65898525322215,-1.20424432627685,52.6402424395144));
#21712=CARTESIAN_POINT('Ctrl Pts',(6.66283129263544,-1.18297728006574,52.6412551424725));
#21713=CARTESIAN_POINT('Ctrl Pts',(6.66657571754772,-1.16169032500973,52.6422678454306));
#21714=CARTESIAN_POINT('Ctrl Pts',(6.67021831111871,-1.14038444483285,52.6432805483887));
#21715=CARTESIAN_POINT('Ctrl Pts',(6.70113461328505,-0.959552019630638,
52.6518758061487));
#21716=CARTESIAN_POINT('Ctrl Pts',(6.72467477233005,-0.777568192048651,
52.6604710639087));
#21717=CARTESIAN_POINT('Ctrl Pts',(6.74078702283454,-0.595045639245815,
52.6690663216688));
#21718=CARTESIAN_POINT('Ctrl Pts',(6.75691436177832,-0.412352161812903,
52.6776696285232));
#21719=CARTESIAN_POINT('Ctrl Pts',(6.76559988104457,-0.229119256336365,
52.6862729353776));
#21720=CARTESIAN_POINT('Ctrl Pts',(6.7668439141714,-0.0459613015649521,
52.694876242232));
#21721=CARTESIAN_POINT('Ctrl Pts',(6.76813952534306,0.144790445526304,52.703836245172));
#21722=CARTESIAN_POINT('Ctrl Pts',(6.76136345946303,0.335460513310029,52.712796248112));
#21723=CARTESIAN_POINT('Ctrl Pts',(6.74657584249044,0.525360258798081,52.7217562510521));
#21724=CARTESIAN_POINT('Ctrl Pts',(6.7323380733906,0.708198963194397,52.7303830942568));
#21725=CARTESIAN_POINT('Ctrl Pts',(6.71067387788064,0.890323309720602,52.7390099374615));
#21726=CARTESIAN_POINT('Ctrl Pts',(6.68168941773004,1.07112815526175,52.7476367806663));
#21727=CARTESIAN_POINT('Ctrl Pts',(6.65267725576229,1.25210580453098,52.7562718689524));
#21728=CARTESIAN_POINT('Ctrl Pts',(6.61633092131939,1.43176113616266,52.7649069572385));
#21729=CARTESIAN_POINT('Ctrl Pts',(6.57280725018437,1.60950111895699,52.7735420455246));
#21730=CARTESIAN_POINT('Ctrl Pts',(6.52921893766329,1.78750508129504,52.7821899586497));
#21731=CARTESIAN_POINT('Ctrl Pts',(6.47843206682968,1.96358771594611,52.7908378717748));
#21732=CARTESIAN_POINT('Ctrl Pts',(6.42065313210189,2.13717157879993,52.7994857849));
#21733=CARTESIAN_POINT('Ctrl Pts',(6.41417121520304,2.15664504571831,52.8004559491041));
#21734=CARTESIAN_POINT('Ctrl Pts',(6.40760134973931,2.17608708599836,52.8014261133082));
#21735=CARTESIAN_POINT('Ctrl Pts',(6.40094386457128,2.19549690106985,52.8023962775123));
#21736=CARTESIAN_POINT('Ctrl Pts',(6.34449558867436,2.36007114624046,52.8106222209846));
#21737=CARTESIAN_POINT('Ctrl Pts',(6.28162179823061,2.52268390004036,52.818848164457));
#21738=CARTESIAN_POINT('Ctrl Pts',(6.21247796981053,2.68279825455043,52.8270741079293));
#21739=CARTESIAN_POINT('Ctrl Pts',(6.14340912648672,2.84273896825175,52.8352911305307));
#21740=CARTESIAN_POINT('Ctrl Pts',(6.06808392849906,3.00018635222957,52.8435081531322));
#21741=CARTESIAN_POINT('Ctrl Pts',(5.98670738887978,3.15461941285036,52.8517251757336));
#21742=CARTESIAN_POINT('Ctrl Pts',(5.90541625048179,3.30889040253464,52.8599335749189));
#21743=CARTESIAN_POINT('Ctrl Pts',(5.81808659401201,3.46015305840489,52.8681419741042));
#21744=CARTESIAN_POINT('Ctrl Pts',(5.72497110107103,3.60790727318505,52.8763503732895));
#21745=CARTESIAN_POINT('Ctrl Pts',(5.63191132478228,3.75557307764873,52.8845538608913));
#21746=CARTESIAN_POINT('Ctrl Pts',(5.53307279596194,3.89973431912708,52.8927573484931));
#21747=CARTESIAN_POINT('Ctrl Pts',(5.42875384719854,4.03991592320027,52.9009608360948));
#21748=CARTESIAN_POINT('Ctrl Pts',(5.32447839363699,4.18003907933818,52.9091609032983));
#21749=CARTESIAN_POINT('Ctrl Pts',(5.21472728457515,4.31618561582027,52.9173609705019));
#21750=CARTESIAN_POINT('Ctrl Pts',(5.09984188074631,4.44790982275787,52.9255610377054));
#21751=CARTESIAN_POINT('Ctrl Pts',(4.98498353674963,4.57960300369207,52.9337591734848));
#21752=CARTESIAN_POINT('Ctrl Pts',(4.86499354277201,4.70687566058062,52.9419573092641));
#21753=CARTESIAN_POINT('Ctrl Pts',(4.74025324529591,4.8293154970929,52.9501554450435));
#21754=CARTESIAN_POINT('Ctrl Pts',(4.61548608009013,4.95178170584009,52.9583553466139));
#21755=CARTESIAN_POINT('Ctrl Pts',(4.48596681833585,5.06941275856206,52.9665552481843));
#21756=CARTESIAN_POINT('Ctrl Pts',(4.35211370372905,5.18183319972901,52.9747551497547));
#21757=CARTESIAN_POINT('Ctrl Pts',(4.2182492492111,5.29426316505099,52.9829557460131));
#21758=CARTESIAN_POINT('Ctrl Pts',(4.08005048847611,5.40148141307023,52.9911563422715));
#21759=CARTESIAN_POINT('Ctrl Pts',(3.93796841058711,5.50315307775624,52.9993569385299));
#21760=CARTESIAN_POINT('Ctrl Pts',(3.79578526474136,5.60489706505721,53.0075633681596));
#21761=CARTESIAN_POINT('Ctrl Pts',(3.64971357664433,5.70108638035999,53.0157697977892));
#21762=CARTESIAN_POINT('Ctrl Pts',(3.50023361237609,5.79142932779056,53.0239762274189));
#21763=CARTESIAN_POINT('Ctrl Pts',(3.36905853787642,5.87070913574167,53.0311777210994));
#21764=CARTESIAN_POINT('Ctrl Pts',(3.23525936987647,5.94548734957398,53.03837921478));
#21765=CARTESIAN_POINT('Ctrl Pts',(3.09917575053258,6.01559628526639,53.0455807084606));
#21766=CARTESIAN_POINT('Ctrl Pts',(3.0991757505326,6.01559628526638,51.0457515827422));
#21767=CARTESIAN_POINT('Ctrl Pts',(2.93382384459266,6.10078395293759,51.0545010306546));
#21768=CARTESIAN_POINT('Ctrl Pts',(2.76495772122985,6.17915010267049,51.063250478567));
#21769=CARTESIAN_POINT('Ctrl Pts',(2.59315093316712,6.25042856433177,51.0719999264794));
#21770=CARTESIAN_POINT('Ctrl Pts',(2.42134553245628,6.32170645041447,51.0807493037394));
#21771=CARTESIAN_POINT('Ctrl Pts',(2.24659977927612,6.38589665313449,51.0894986809994));
#21772=CARTESIAN_POINT('Ctrl Pts',(2.06950718689951,6.44278115439065,51.0982480582594));
#21773=CARTESIAN_POINT('Ctrl Pts',(1.89241596572898,6.49966521519713,51.1069973677741));
#21774=CARTESIAN_POINT('Ctrl Pts',(1.71297821457239,6.54924360009535,51.1157466772887));
#21775=CARTESIAN_POINT('Ctrl Pts',(1.53180337335891,6.59134792173545,51.1244959868034));
#21776=CARTESIAN_POINT('Ctrl Pts',(1.35062987477834,6.63345193135294,51.1332452314795));
#21777=CARTESIAN_POINT('Ctrl Pts',(1.16771959103009,6.66808192368228,51.1419944761557));
#21778=CARTESIAN_POINT('Ctrl Pts',(0.983693746907472,6.69512028363159,51.1507437208318));
#21779=CARTESIAN_POINT('Ctrl Pts',(0.799669205420609,6.72215845218858,51.1594929035759));
#21780=CARTESIAN_POINT('Ctrl Pts',(0.614529402874324,6.74160505424571,51.1682420863201));
#21781=CARTESIAN_POINT('Ctrl Pts',(0.428903127364207,6.75339404354116,51.1769912690643));
#21782=CARTESIAN_POINT('Ctrl Pts',(0.243278104164781,6.76518295330327,51.1857403927829));
#21783=CARTESIAN_POINT('Ctrl Pts',(0.0571669005399603,6.76931433552275,
51.1944895165015));
#21784=CARTESIAN_POINT('Ctrl Pts',(-0.12879840477673,6.76577415902474,51.2032386402201));
#21785=CARTESIAN_POINT('Ctrl Pts',(-0.314762517258233,6.76223400523445,
51.2119877078193));
#21786=CARTESIAN_POINT('Ctrl Pts',(-0.500580446818562,6.75102239665096,
51.2207367754185));
#21787=CARTESIAN_POINT('Ctrl Pts',(-0.685621118841584,6.73217741012508,
51.2294858430177));
#21788=CARTESIAN_POINT('Ctrl Pts',(-0.870660665413498,6.71333253821785,
51.2382348574035));
#21789=CARTESIAN_POINT('Ctrl Pts',(-1.05492267885391,6.68685441030627,51.2469838717893));
#21790=CARTESIAN_POINT('Ctrl Pts',(-1.23778137635161,6.65283295028194,51.2557328861751));
#21791=CARTESIAN_POINT('Ctrl Pts',(-1.42999922978755,6.61707018861885,51.2649296965425));
#21792=CARTESIAN_POINT('Ctrl Pts',(-1.62066601233603,6.57297172934436,51.2741265069099));
#21793=CARTESIAN_POINT('Ctrl Pts',(-1.80906628500293,6.5207030431132,51.2833233172772));
#21794=CARTESIAN_POINT('Ctrl Pts',(-1.98831342545431,6.4709737491506,51.292073315015));
#21795=CARTESIAN_POINT('Ctrl Pts',(-2.16550875896602,6.41384933989562,51.3008233127528));
#21796=CARTESIAN_POINT('Ctrl Pts',(-2.34005036713908,6.34952386240514,51.3095733104905));
#21797=CARTESIAN_POINT('Ctrl Pts',(-2.51458843546987,6.28519968948637,51.3183231307714));
#21798=CARTESIAN_POINT('Ctrl Pts',(-2.68647261717955,6.21367483971142,51.3270729510523));
#21799=CARTESIAN_POINT('Ctrl Pts',(-2.85511905908633,6.1351922674389,51.3358227713331));
#21800=CARTESIAN_POINT('Ctrl Pts',(-3.02376230488782,6.05671118252988,51.3445724257917));
#21801=CARTESIAN_POINT('Ctrl Pts',(-3.18916767379798,5.97127275992689,51.3533220802502));
#21802=CARTESIAN_POINT('Ctrl Pts',(-3.35077334102678,5.87916720438059,51.3620717347087));
#21803=CARTESIAN_POINT('Ctrl Pts',(-3.51237616037259,5.78706327195709,51.3708212349772));
#21804=CARTESIAN_POINT('Ctrl Pts',(-3.67017916302191,5.68829258362369,51.3795707352456));
#21805=CARTESIAN_POINT('Ctrl Pts',(-3.82364636566354,5.58319061741116,51.3883202355141));
#21806=CARTESIAN_POINT('Ctrl Pts',(-3.97711106778698,5.47809036367774,51.3970695932225));
#21807=CARTESIAN_POINT('Ctrl Pts',(-4.12623987481836,5.36665920043295,51.4058189509309));
#21808=CARTESIAN_POINT('Ctrl Pts',(-4.27052628213847,5.24927559512402,51.4145683086394));
#21809=CARTESIAN_POINT('Ctrl Pts',(-4.41481053024885,5.13189374643116,51.4233175354159));
#21810=CARTESIAN_POINT('Ctrl Pts',(-4.55425230136427,5.00855981477447,51.4320667621924));
#21811=CARTESIAN_POINT('Ctrl Pts',(-4.68837800630435,4.87969268192185,51.4408159889689));
#21812=CARTESIAN_POINT('Ctrl Pts',(-4.82250188228773,4.75082730631932,51.4495650964397));
#21813=CARTESIAN_POINT('Ctrl Pts',(-4.95130963052837,4.61642907903663,51.4583142039106));
#21814=CARTESIAN_POINT('Ctrl Pts',(-5.07436379033232,4.47695444731843,51.4670633113814));
#21815=CARTESIAN_POINT('Ctrl Pts',(-5.19741643562648,4.33748153220773,51.4758123111711));
#21816=CARTESIAN_POINT('Ctrl Pts',(-5.31471544462597,4.19293255254811,51.4845613109609));
#21817=CARTESIAN_POINT('Ctrl Pts',(-5.42586245275435,4.04379841779862,51.4933103107506));
#21818=CARTESIAN_POINT('Ctrl Pts',(-5.53702160018961,3.89464799484615,51.5020602660927));
#21819=CARTESIAN_POINT('Ctrl Pts',(-5.64202723081062,3.74091164444135,51.5108102214349));
#21820=CARTESIAN_POINT('Ctrl Pts',(-5.74052265232781,3.58311159163531,51.519560176777));
#21821=CARTESIAN_POINT('Ctrl Pts',(-5.83901427066747,3.42531763192076,51.5283097942595));
#21822=CARTESIAN_POINT('Ctrl Pts',(-5.93099603115583,3.26346052695898,51.537059411742));
#21823=CARTESIAN_POINT('Ctrl Pts',(-6.0161555062261,3.09809004467355,51.5458090292244));
#21824=CARTESIAN_POINT('Ctrl Pts',(-6.10131214578663,2.93272506864111,51.5545583553755));
#21825=CARTESIAN_POINT('Ctrl Pts',(-6.17964682328618,2.76384720417183,51.5633076815266));
#21826=CARTESIAN_POINT('Ctrl Pts',(-6.25089348288442,2.59203002791887,51.5720570076777));
#21827=CARTESIAN_POINT('Ctrl Pts',(-6.32213814889222,2.42021765937313,51.5808060890093));
#21828=CARTESIAN_POINT('Ctrl Pts',(-6.38629508412489,2.24546640832192,51.5895551703408));
#21829=CARTESIAN_POINT('Ctrl Pts',(-6.44314639819727,2.06836976660304,51.5983042516724));
#21830=CARTESIAN_POINT('Ctrl Pts',(-6.50000285283626,1.89125711158531,51.6070541241068));
#21831=CARTESIAN_POINT('Ctrl Pts',(-6.54955227673185,1.71179891440502,51.6158039965412));
#21832=CARTESIAN_POINT('Ctrl Pts',(-6.59162635926329,1.5306047627867,51.6245538689756));
#21833=CARTESIAN_POINT('Ctrl Pts',(-6.63369752055148,1.34942319164934,51.6333031338981));
#21834=CARTESIAN_POINT('Ctrl Pts',(-6.66829431424213,1.1665061864294,51.6420523988206));
#21835=CARTESIAN_POINT('Ctrl Pts',(-6.69529923745383,0.982474997620903,
51.6508016637431));
#21836=CARTESIAN_POINT('Ctrl Pts',(-6.72230554731416,0.798434359180046,
51.6595513779228));
#21837=CARTESIAN_POINT('Ctrl Pts',(-6.74171916496683,0.613279706242597,
51.6683010921025));
#21838=CARTESIAN_POINT('Ctrl Pts',(-6.75347414817261,0.427639953657591,
51.6770508062822));
#21839=CARTESIAN_POINT('Ctrl Pts',(-6.76248837758738,0.285283364200273,
51.6837604654581));
#21840=CARTESIAN_POINT('Ctrl Pts',(-6.76699999999995,0.142641701106303,
51.6904701246341));
#21841=CARTESIAN_POINT('Ctrl Pts',(-6.767,2.23847959696427E-12,51.69717978381));
#21842=CARTESIAN_POINT('',(-6.76699991050681,0.00110054571900286,51.3028202161511));
#21843=CARTESIAN_POINT('Ctrl Pts',(3.09917575053255,6.01559628526641,50.6515095859174));
#21844=CARTESIAN_POINT('Ctrl Pts',(2.94372576997178,6.09568257884875,50.6597176158886));
#21845=CARTESIAN_POINT('Ctrl Pts',(2.78510729620925,6.1697715374377,50.6679256458599));
#21846=CARTESIAN_POINT('Ctrl Pts',(2.6238253565943,6.23761408698012,50.6761336758311));
#21847=CARTESIAN_POINT('Ctrl Pts',(2.46269641988174,6.30539227651415,50.6843339191127));
#21848=CARTESIAN_POINT('Ctrl Pts',(2.29890939798744,6.36693576138702,50.6925341623944));
#21849=CARTESIAN_POINT('Ctrl Pts',(2.13298918365071,6.42204376677932,50.700734405676));
#21850=CARTESIAN_POINT('Ctrl Pts',(1.96706474179028,6.47715317628262,50.7089348578937));
#21851=CARTESIAN_POINT('Ctrl Pts',(1.79900733918795,6.52582666653708,50.7171353101114));
#21852=CARTESIAN_POINT('Ctrl Pts',(1.62935819918338,6.5679129758816,50.7253357623291));
#21853=CARTESIAN_POINT('Ctrl Pts',(1.45967399289318,6.61000798441873,50.7335379095711));
#21854=CARTESIAN_POINT('Ctrl Pts',(1.28839774159573,6.64551301394018,50.741740056813));
#21855=CARTESIAN_POINT('Ctrl Pts',(1.11608211499278,6.67432765996645,50.7499422040549));
#21856=CARTESIAN_POINT('Ctrl Pts',(0.943531307150705,6.70318163303631,50.7581555458193));
#21857=CARTESIAN_POINT('Ctrl Pts',(0.769938641694908,6.72532690243689,50.7663688875837));
#21858=CARTESIAN_POINT('Ctrl Pts',(0.595864882246309,6.74071465366289,50.7745822293481));
#21859=CARTESIAN_POINT('Ctrl Pts',(0.421786699118565,6.75610279593274,50.7827957798354));
#21860=CARTESIAN_POINT('Ctrl Pts',(0.247227757010974,6.76473308307763,50.7910093303228));
#21861=CARTESIAN_POINT('Ctrl Pts',(0.0727493048034127,6.76660893939133,
50.7992228808101));
#21862=CARTESIAN_POINT('Ctrl Pts',(-0.101971380471242,6.76848740000614,
50.8074478343876));
#21863=CARTESIAN_POINT('Ctrl Pts',(-0.276610994058523,6.76359269692049,
50.8156727879652));
#21864=CARTESIAN_POINT('Ctrl Pts',(-0.450610895119438,6.75198036291573,
50.8238977415427));
#21865=CARTESIAN_POINT('Ctrl Pts',(-0.624115081960255,6.7404011116832,50.832099262771));
#21866=CARTESIAN_POINT('Ctrl Pts',(-0.79698285563322,6.72214256066124,50.8403007839993));
#21867=CARTESIAN_POINT('Ctrl Pts',(-0.968670483191178,6.69731039261241,
50.8485023052276));
#21868=CARTESIAN_POINT('Ctrl Pts',(-1.14966196433778,6.67113255476139,50.8571482717184));
#21869=CARTESIAN_POINT('Ctrl Pts',(-1.32975286856129,6.63759031909408,50.8657942382093));
#21870=CARTESIAN_POINT('Ctrl Pts',(-1.50833518579757,6.59675783755058,50.8744402047002));
#21871=CARTESIAN_POINT('Ctrl Pts',(-1.68668907197277,6.55597758630193,50.8830751118246));
#21872=CARTESIAN_POINT('Ctrl Pts',(-1.86353792321638,6.50792575185398,50.8917100189489));
#21873=CARTESIAN_POINT('Ctrl Pts',(-2.03828166633691,6.45272786104255,50.9003449260733));
#21874=CARTESIAN_POINT('Ctrl Pts',(-2.21882676069068,6.39569744480726,50.9092665051448));
#21875=CARTESIAN_POINT('Ctrl Pts',(-2.3971242476004,6.33103834858026,50.9181880842163));
#21876=CARTESIAN_POINT('Ctrl Pts',(-2.57252375267655,6.25894644024975,50.9271096632879));
#21877=CARTESIAN_POINT('Ctrl Pts',(-2.74181838879493,6.18936372744451,50.9357207222635));
#21878=CARTESIAN_POINT('Ctrl Pts',(-2.90841303997573,6.11285698168042,50.9443317812392));
#21879=CARTESIAN_POINT('Ctrl Pts',(-3.07173784346953,6.0296530265843,50.9529428402149));
#21880=CARTESIAN_POINT('Ctrl Pts',(-3.23490862413441,5.9465275366586,50.9615457785645));
#21881=CARTESIAN_POINT('Ctrl Pts',(-3.39481543420343,5.85671756737965,50.970148716914));
#21882=CARTESIAN_POINT('Ctrl Pts',(-3.55090909497626,5.76049768676413,50.9787516552636));
#21883=CARTESIAN_POINT('Ctrl Pts',(-3.7068279669575,5.66438555015677,50.9873449603123));
#21884=CARTESIAN_POINT('Ctrl Pts',(-3.85894194881801,5.56187798104296,50.995938265361));
#21885=CARTESIAN_POINT('Ctrl Pts',(-4.00672696246917,5.45329515506199,51.0045315704097));
#21886=CARTESIAN_POINT('Ctrl Pts',(-4.02319263198647,5.44119725092621,51.0054890052503));
#21887=CARTESIAN_POINT('Ctrl Pts',(-4.03960458966874,5.42902397727664,51.0064464400909));
#21888=CARTESIAN_POINT('Ctrl Pts',(-4.05596213087828,5.4167758115766,51.0074038749316));
#21889=CARTESIAN_POINT('Ctrl Pts',(-4.20281855634457,5.30681296262605,51.0159996324792));
#21890=CARTESIAN_POINT('Ctrl Pts',(-4.34511433100738,5.19093896239823,51.0245953900268));
#21891=CARTESIAN_POINT('Ctrl Pts',(-4.48239025425366,5.06956276305677,51.0331911475744));
#21892=CARTESIAN_POINT('Ctrl Pts',(-4.61979426060219,4.94807331559589,51.041794925256));
#21893=CARTESIAN_POINT('Ctrl Pts',(-4.75216883799272,4.82107162412226,51.0503987029375));
#21894=CARTESIAN_POINT('Ctrl Pts',(-4.87909141508808,4.68900372821496,51.0590024806191));
#21895=CARTESIAN_POINT('Ctrl Pts',(-5.01100216045051,4.55174544851197,51.0679443942871));
#21896=CARTESIAN_POINT('Ctrl Pts',(-5.1370234511554,4.40901497961087,51.0768863079551));
#21897=CARTESIAN_POINT('Ctrl Pts',(-5.25672760455551,4.2613500080965,51.0858282216231));
#21898=CARTESIAN_POINT('Ctrl Pts',(-5.37221876109697,4.11888211657855,51.0944554239538));
#21899=CARTESIAN_POINT('Ctrl Pts',(-5.48182972798825,3.97182141005477,51.1030826262846));
#21900=CARTESIAN_POINT('Ctrl Pts',(-5.58522098140526,3.82067999037744,51.1117098286153));
#21901=CARTESIAN_POINT('Ctrl Pts',(-5.68871069916511,3.66939463163297,51.1203452470357));
#21902=CARTESIAN_POINT('Ctrl Pts',(-5.78596871565353,3.5140210591272,51.1289806654561));
#21903=CARTESIAN_POINT('Ctrl Pts',(-5.8767006022561,3.35509746973807,51.1376160838765));
#21904=CARTESIAN_POINT('Ctrl Pts',(-5.96756653229802,3.1959390933814,51.1462642598976));
#21905=CARTESIAN_POINT('Ctrl Pts',(-6.05188692151583,3.03322048828594,51.1549124359188));
#21906=CARTESIAN_POINT('Ctrl Pts',(-6.12941409520859,2.86750272004374,51.16356061194));
#21907=CARTESIAN_POINT('Ctrl Pts',(-6.13761617622538,2.84997040851603,51.1644755561717));
#21908=CARTESIAN_POINT('Ctrl Pts',(-6.14574226703425,2.8324045443392,51.1653905004034));
#21909=CARTESIAN_POINT('Ctrl Pts',(-6.15379210651178,2.81480580321864,51.1663054446351));
#21910=CARTESIAN_POINT('Ctrl Pts',(-6.23137319601528,2.64519627077582,51.175123306225));
#21911=CARTESIAN_POINT('Ctrl Pts',(-6.30201094808761,2.47221860160181,51.1839411678148));
#21912=CARTESIAN_POINT('Ctrl Pts',(-6.36542467166714,2.29644458877878,51.1927590294046));
#21913=CARTESIAN_POINT('Ctrl Pts',(-6.43138349855206,2.11361590394177,51.2019307949668));
#21914=CARTESIAN_POINT('Ctrl Pts',(-6.48952626910946,1.92776199853278,51.211102560529));
#21915=CARTESIAN_POINT('Ctrl Pts',(-6.539590179954,1.73955433322712,51.2202743260912));
#21916=CARTESIAN_POINT('Ctrl Pts',(-6.587510676453,1.5594045084487,51.2290534157008));
#21917=CARTESIAN_POINT('Ctrl Pts',(-6.62802949287413,1.37709857063926,51.2378325053105));
#21918=CARTESIAN_POINT('Ctrl Pts',(-6.66096483337967,1.1932461977645,51.2466115949201));
#21919=CARTESIAN_POINT('Ctrl Pts',(-6.69384701086094,1.00969059267806,51.2553765136438));
#21920=CARTESIAN_POINT('Ctrl Pts',(-6.71917007219714,0.824593800378376,
51.2641414323675));
#21921=CARTESIAN_POINT('Ctrl Pts',(-6.73680234476203,0.638579022211728,
51.2729063510912));
#21922=CARTESIAN_POINT('Ctrl Pts',(-6.75439619629057,0.452969573563714,
51.2816521709007));
#21923=CARTESIAN_POINT('Ctrl Pts',(-6.76433266229265,0.266446403454901,
51.2903979907102));
#21924=CARTESIAN_POINT('Ctrl Pts',(-6.76653133397799,0.0796411093222789,
51.2991438105197));
#21925=CARTESIAN_POINT('Ctrl Pts',(-6.76683941292852,0.0534658602596612,
51.3003692790635));
#21926=CARTESIAN_POINT('Ctrl Pts',(-6.76699565200429,0.0272850882396232,
51.3015947476073));
#21927=CARTESIAN_POINT('Ctrl Pts',(-6.76699991050681,0.00110054571902172,
51.3028202161511));
#21928=CARTESIAN_POINT('Ctrl Pts',(-6.76699991050694,0.0011005448889491,
51.3028202161899));
#21929=CARTESIAN_POINT('Ctrl Pts',(-6.7670293195252,-0.179728811491938,
51.3112832507402));
#21930=CARTESIAN_POINT('Ctrl Pts',(-6.75980613686487,-0.360470594821842,
51.3197462852904));
#21931=CARTESIAN_POINT('Ctrl Pts',(-6.74537751872907,-0.540528565225264,
51.3282093198407));
#21932=CARTESIAN_POINT('Ctrl Pts',(-6.73093802421214,-0.720722264434683,
51.3366787338785));
#21933=CARTESIAN_POINT('Ctrl Pts',(-6.70928228373777,-0.900230799662108,
51.3451481479163));
#21934=CARTESIAN_POINT('Ctrl Pts',(-6.68050916102434,-1.07846481141938,
51.3536175619541));
#21935=CARTESIAN_POINT('Ctrl Pts',(-6.65171094590499,-1.25685425712857,
51.3620943619812));
#21936=CARTESIAN_POINT('Ctrl Pts',(-6.61578301640392,-1.43396664259712,
51.3705711620082));
#21937=CARTESIAN_POINT('Ctrl Pts',(-6.57287508846235,-1.60922405881562,
51.3790479620353));
#21938=CARTESIAN_POINT('Ctrl Pts',(-6.52855870350362,-1.79023431721328,
51.3878030138692));
#21939=CARTESIAN_POINT('Ctrl Pts',(-6.4767964103259,-1.96926538920702,51.3965580657032));
#21940=CARTESIAN_POINT('Ctrl Pts',(-6.41780797571549,-2.14570030219569,
51.4053131175372));
#21941=CARTESIAN_POINT('Ctrl Pts',(-6.36053538499355,-2.31700311142258,
51.4138135041595));
#21942=CARTESIAN_POINT('Ctrl Pts',(-6.29645132653337,-2.48585841071289,
51.4223138907819));
#21943=CARTESIAN_POINT('Ctrl Pts',(-6.22580501065645,-2.65172415030015,
51.4308142774042));
#21944=CARTESIAN_POINT('Ctrl Pts',(-6.15198392877506,-2.82504370973367,
51.439696661844));
#21945=CARTESIAN_POINT('Ctrl Pts',(-6.07099737519763,-2.99509844173543,
51.4485790462838));
#21946=CARTESIAN_POINT('Ctrl Pts',(-5.98318190989025,-3.16130087672182,
51.4574614307236));
#21947=CARTESIAN_POINT('Ctrl Pts',(-5.89536644458283,-3.32750331170826,
51.4663438151633));
#21948=CARTESIAN_POINT('Ctrl Pts',(-5.80072232668789,-3.48985314242165,
51.4752261996031));
#21949=CARTESIAN_POINT('Ctrl Pts',(-5.69963587399677,-3.64779932340708,
51.4841085840429));
#21950=CARTESIAN_POINT('Ctrl Pts',(-5.60682224202642,-3.79281933670102,
51.4922640424497));
#21951=CARTESIAN_POINT('Ctrl Pts',(-5.50831883497746,-3.93453128983594,
51.5004195008565));
#21952=CARTESIAN_POINT('Ctrl Pts',(-5.40438862416666,-4.07245289708525,
51.5085749592633));
#21953=CARTESIAN_POINT('Ctrl Pts',(-5.30058491008398,-4.21020663560882,
51.5167204914052));
#21954=CARTESIAN_POINT('Ctrl Pts',(-5.19136775760629,-4.34417892263188,
51.5248660235471));
#21955=CARTESIAN_POINT('Ctrl Pts',(-5.0770451485939,-4.47391345011716,51.5330115556889));
#21956=CARTESIAN_POINT('Ctrl Pts',(-4.96283764547294,-4.60351735419761,
51.5411488864895));
#21957=CARTESIAN_POINT('Ctrl Pts',(-4.84353515935554,-4.7288917209991,51.54928621729));
#21958=CARTESIAN_POINT('Ctrl Pts',(-4.71948794390356,-4.84961055625593,
51.5574235480906));
#21959=CARTESIAN_POINT('Ctrl Pts',(-4.59553955667126,-4.9702332150083,51.5655543958926));
#21960=CARTESIAN_POINT('Ctrl Pts',(-4.46685422751048,-5.08620747368003,
51.5736852436946));
#21961=CARTESIAN_POINT('Ctrl Pts',(-4.33382132026465,-5.19714169173976,
51.5818160914966));
#21962=CARTESIAN_POINT('Ctrl Pts',(-4.20086645426036,-5.30801083233643,
51.5899421694904));
#21963=CARTESIAN_POINT('Ctrl Pts',(-4.06356936929772,-5.41384558692698,
51.5980682474842));
#21964=CARTESIAN_POINT('Ctrl Pts',(-3.92235498716737,-5.5142923711609,51.6061943254779));
#21965=CARTESIAN_POINT('Ctrl Pts',(-3.7806398846293,-5.61509532134616,51.6143492170601));
#21966=CARTESIAN_POINT('Ctrl Pts',(-3.63497992465894,-5.71047176661043,
51.6225041086423));
#21967=CARTESIAN_POINT('Ctrl Pts',(-3.48583713478017,-5.80010590160107,
51.6306590002245));
#21968=CARTESIAN_POINT('Ctrl Pts',(-3.33727594963583,-5.88939049480482,
51.6387820905808));
#21969=CARTESIAN_POINT('Ctrl Pts',(-3.18525937398488,-5.97297730829069,
51.6469051809371));
#21970=CARTESIAN_POINT('Ctrl Pts',(-3.03027176795098,-6.05059848381623,
51.6550282712934));
#21971=CARTESIAN_POINT('Ctrl Pts',(-2.87527199158271,-6.12822575451082,
51.6631519995118));
#21972=CARTESIAN_POINT('Ctrl Pts',(-2.71730104721002,-6.19988629028897,
51.6712757277303));
#21973=CARTESIAN_POINT('Ctrl Pts',(-2.55686628275255,-6.26535903297833,
51.6793994559487));
#21974=CARTESIAN_POINT('Ctrl Pts',(-2.39638839770137,-6.33084937299796,
51.687525367609));
#21975=CARTESIAN_POINT('Ctrl Pts',(-2.23344571254812,-6.39014847019056,
51.6956512792693));
#21976=CARTESIAN_POINT('Ctrl Pts',(-2.06856381296008,-6.44308410248633,
51.7037771909296));
#21977=CARTESIAN_POINT('Ctrl Pts',(-1.90262747648431,-6.49635826365341,
51.7119550686397));
#21978=CARTESIAN_POINT('Ctrl Pts',(-1.73472739414795,-6.54318717256633,
51.7201329463498));
#21979=CARTESIAN_POINT('Ctrl Pts',(-1.56541213514596,-6.5834469578738,51.7283108240599));
#21980=CARTESIAN_POINT('Ctrl Pts',(-1.39690498115332,-6.62351459195772,
51.7364496705333));
#21981=CARTESIAN_POINT('Ctrl Pts',(-1.22699650039423,-6.65707566049365,
51.7445885170068));
#21982=CARTESIAN_POINT('Ctrl Pts',(-1.05623464916449,-6.6840599463129,51.7527273634802));
#21983=CARTESIAN_POINT('Ctrl Pts',(-0.884244421238745,-6.71123834380065,
51.7609247568086));
#21984=CARTESIAN_POINT('Ctrl Pts',(-0.711388874229226,-6.73174493705477,
51.769122150137));
#21985=CARTESIAN_POINT('Ctrl Pts',(-0.538229598620791,-6.74556134796568,
51.7773195434654));
#21986=CARTESIAN_POINT('Ctrl Pts',(-0.365070323012357,-6.75937775887658,
51.7855169367938));
#21987=CARTESIAN_POINT('Ctrl Pts',(-0.19160769323252,-6.76650403322454,
51.7937143301222));
#21988=CARTESIAN_POINT('Ctrl Pts',(-0.0183993852529096,-6.76697498610881,
51.8019117234507));
#21989=CARTESIAN_POINT('Ctrl Pts',(0.155417795802133,-6.7674475945172,51.8101379327876));
#21990=CARTESIAN_POINT('Ctrl Pts',(0.329496174290599,-6.76121953317085,
51.8183641421246));
#21991=CARTESIAN_POINT('Ctrl Pts',(0.50327859407008,-6.74825900931128,51.8265903514616));
#21992=CARTESIAN_POINT('Ctrl Pts',(0.676865776745864,-6.73531304604503,
51.8348073190048));
#21993=CARTESIAN_POINT('Ctrl Pts',(0.850157308409486,-6.71564970794485,
51.843024286548));
#21994=CARTESIAN_POINT('Ctrl Pts',(1.02259445868563,-6.68928916799576,51.8512412540912));
#21995=CARTESIAN_POINT('Ctrl Pts',(1.19487249272749,-6.66295295221258,51.8594506394346));
#21996=CARTESIAN_POINT('Ctrl Pts',(1.36629736317955,-6.62993189581132,51.8676600247779));
#21997=CARTESIAN_POINT('Ctrl Pts',(1.53631380092767,-6.59029808924294,51.8758694101213));
#21998=CARTESIAN_POINT('Ctrl Pts',(1.70620746886125,-6.55069290246655,51.8840728674219));
#21999=CARTESIAN_POINT('Ctrl Pts',(1.87469438199783,-6.50448455780097,51.8922763247225));
#22000=CARTESIAN_POINT('Ctrl Pts',(2.04122773926517,-6.45179651852524,51.9004797820231));
#22001=CARTESIAN_POINT('Ctrl Pts',(2.207674248052,-6.39913595648427,51.9086789611549));
#22002=CARTESIAN_POINT('Ctrl Pts',(2.37216888947289,-6.34000253974969,51.9168781402868));
#22003=CARTESIAN_POINT('Ctrl Pts',(2.53417825948068,-6.27457006887129,51.9250773194186));
#22004=CARTESIAN_POINT('Ctrl Pts',(2.69615710343171,-6.20914992688054,51.9332749536484));
#22005=CARTESIAN_POINT('Ctrl Pts',(2.85565127420781,-6.13743322328416,51.9414725878783));
#22006=CARTESIAN_POINT('Ctrl Pts',(3.01214536417536,-6.05964267140208,51.9496702221081));
#22007=CARTESIAN_POINT('Ctrl Pts',(3.16862815822796,-5.9818577345273,51.9578672646236));
#22008=CARTESIAN_POINT('Ctrl Pts',(3.32211098116247,-5.89799998136302,51.9660643071392));
#22009=CARTESIAN_POINT('Ctrl Pts',(3.47210119730316,-5.80833902898978,51.9742613496548));
#22010=CARTESIAN_POINT('Ctrl Pts',(3.62210784745626,-5.71866825271441,51.9824592902976));
#22011=CARTESIAN_POINT('Ctrl Pts',(3.76862082048467,-5.6231931945263,51.9906572309405));
#22012=CARTESIAN_POINT('Ctrl Pts',(3.91117470277814,-5.52222794208536,51.9988551715833));
#22013=CARTESIAN_POINT('Ctrl Pts',(4.05377011333156,-5.42123327682745,52.0070555004193));
#22014=CARTESIAN_POINT('Ctrl Pts',(4.19240384319343,-5.31474543879705,52.0152558292553));
#22015=CARTESIAN_POINT('Ctrl Pts',(4.3266418856865,-5.20312012094889,52.0234561580913));
#22016=CARTESIAN_POINT('Ctrl Pts',(4.46101980770262,-5.09137848662344,52.0316650318827));
#22017=CARTESIAN_POINT('Ctrl Pts',(4.59099261521088,-4.97448890685478,52.0398739056741));
#22018=CARTESIAN_POINT('Ctrl Pts',(4.71616091591607,-4.85284609432297,52.0480827794655));
#22019=CARTESIAN_POINT('Ctrl Pts',(4.84139639306712,-4.73113799743591,52.0562960588689));
#22020=CARTESIAN_POINT('Ctrl Pts',(4.96182197592798,-4.60467184176375,52.0645093382723));
#22021=CARTESIAN_POINT('Ctrl Pts',(5.07707730261945,-4.47387696111844,52.0727226176757));
#22022=CARTESIAN_POINT('Ctrl Pts',(5.19250120834156,-4.3428907724024,52.0809479102911));
#22023=CARTESIAN_POINT('Ctrl Pts',(5.30273951858665,-4.20756348381302,52.0891732029066));
#22024=CARTESIAN_POINT('Ctrl Pts',(5.40747332910717,-4.06835608016243,52.097398495522));
#22025=CARTESIAN_POINT('Ctrl Pts',(5.50219247963385,-3.94245970577029,52.1048372846341));
#22026=CARTESIAN_POINT('Ctrl Pts',(5.5924099379874,-3.81339031464735,52.1122760737462));
#22027=CARTESIAN_POINT('Ctrl Pts',(5.67792195915921,-3.68150665158949,52.1197148628583));
#22028=CARTESIAN_POINT('Ctrl Pts',(5.77248561260963,-3.53566281772527,52.1279410638772));
#22029=CARTESIAN_POINT('Ctrl Pts',(5.86155858299504,-3.38596933453658,52.136167264896));
#22030=CARTESIAN_POINT('Ctrl Pts',(5.94481231055862,-3.23287729309831,52.1443934659149));
#22031=CARTESIAN_POINT('Ctrl Pts',(6.02797252010593,-3.07995721830275,52.1526104265306));
#22032=CARTESIAN_POINT('Ctrl Pts',(6.10532633338411,-2.92364649926657,52.1608273871464));
#22033=CARTESIAN_POINT('Ctrl Pts',(6.17658801737508,-2.76442570231478,52.1690443477622));
#22034=CARTESIAN_POINT('Ctrl Pts',(6.24778395666923,-2.60535179949229,52.1772537275638));
#22035=CARTESIAN_POINT('Ctrl Pts',(6.31289881449309,-2.44337349088994,52.1854631073653));
#22036=CARTESIAN_POINT('Ctrl Pts',(6.3716923719208,-2.27899655936693,52.1936724871669));
#22037=CARTESIAN_POINT('Ctrl Pts',(6.43044348405991,-2.11473829775612,52.2018759403073));
#22038=CARTESIAN_POINT('Ctrl Pts',(6.4828822653894,-1.9480851987053,52.2100793934477));
#22039=CARTESIAN_POINT('Ctrl Pts',(6.52881626566073,-1.77956375812836,52.2182828465881));
#22040=CARTESIAN_POINT('Ctrl Pts',(6.57472631868904,-1.61113017456074,52.2264820229382));
#22041=CARTESIAN_POINT('Ctrl Pts',(6.61413825245348,-1.44083053512187,52.2346811992884));
#22042=CARTESIAN_POINT('Ctrl Pts',(6.64690918518168,-1.26920734474215,52.2428803756385));
#22043=CARTESIAN_POINT('Ctrl Pts',(6.67967395156445,-1.09761644785506,52.2510780091899));
#22044=CARTESIAN_POINT('Ctrl Pts',(6.70580013268361,-0.924702846842289,
52.2592756427412));
#22045=CARTESIAN_POINT('Ctrl Pts',(6.72519570953941,-0.751020418093132,
52.2674732762926));
#22046=CARTESIAN_POINT('Ctrl Pts',(6.74458988943764,-0.577350498741494,
52.2756703194132));
#22047=CARTESIAN_POINT('Ctrl Pts',(6.75725438983026,-0.402912218299536,
52.2838673625338));
#22048=CARTESIAN_POINT('Ctrl Pts',(6.76314895297657,-0.228265722025817,
52.2920644056544));
#22049=CARTESIAN_POINT('Ctrl Pts',(6.76904416289669,-0.0536000628765411,
52.3002623481856));
#22050=CARTESIAN_POINT('Ctrl Pts',(6.76816794355004,0.1212734990702,52.3084602907168));
#22051=CARTESIAN_POINT('Ctrl Pts',(6.76053216405729,0.295793608360497,52.316658233248));
#22052=CARTESIAN_POINT('Ctrl Pts',(6.75289415894258,0.470364585513826,52.3248585652564));
#22053=CARTESIAN_POINT('Ctrl Pts',(6.73849268490011,0.644581546556523,52.3330588972648));
#22054=CARTESIAN_POINT('Ctrl Pts',(6.71739159661993,0.817886995654062,52.3412592292732));
#22055=CARTESIAN_POINT('Ctrl Pts',(6.69626851530248,0.991373075871156,52.3494681082439));
#22056=CARTESIAN_POINT('Ctrl Pts',(6.6684319125601,1.16394538958286,52.3576769872147));
#22057=CARTESIAN_POINT('Ctrl Pts',(6.63399719299451,1.33505439714681,52.3658858661855));
#22058=CARTESIAN_POINT('Ctrl Pts',(6.59954398807276,1.50625525999478,52.3740991518728));
#22059=CARTESIAN_POINT('Ctrl Pts',(6.55848568943385,1.67599090241361,52.3823124375602));
#22060=CARTESIAN_POINT('Ctrl Pts',(6.51098794669323,1.84372583591367,52.3905257232476));
#22061=CARTESIAN_POINT('Ctrl Pts',(6.46342072060891,2.01170614494867,52.3987510239597));
#22062=CARTESIAN_POINT('Ctrl Pts',(6.40939533595326,2.17767955502114,52.4069763246718));
#22063=CARTESIAN_POINT('Ctrl Pts',(6.34912650578597,2.34112827788783,52.4152016253839));
#22064=CARTESIAN_POINT('Ctrl Pts',(6.29462061899694,2.48894793125848,52.4226404176779));
#22065=CARTESIAN_POINT('Ctrl Pts',(6.23500890614251,2.63470272676859,52.430079209972));
#22066=CARTESIAN_POINT('Ctrl Pts',(6.17048252953134,2.77802706119803,52.437518002266));
#22067=CARTESIAN_POINT('Ctrl Pts',(6.09974706525856,2.93514286205176,52.4456725966223));
#22068=CARTESIAN_POINT('Ctrl Pts',(6.02289617693403,3.08980105830553,52.4538271909787));
#22069=CARTESIAN_POINT('Ctrl Pts',(5.9401224555034,3.24148642039794,52.461981785335));
#22070=CARTESIAN_POINT('Ctrl Pts',(5.85747523226454,3.39293997070648,52.4701239175062));
#22071=CARTESIAN_POINT('Ctrl Pts',(5.76892338489564,3.54142942142937,52.4782660496774));
#22072=CARTESIAN_POINT('Ctrl Pts',(5.67470749145207,3.68645953273026,52.4864081818485));
#22073=CARTESIAN_POINT('Ctrl Pts',(5.58057537657762,3.83136068049049,52.4945430738805));
#22074=CARTESIAN_POINT('Ctrl Pts',(5.48078943761993,3.97280830693704,52.5026779659125));
#22075=CARTESIAN_POINT('Ctrl Pts',(5.37563639108518,4.11033117775693,52.5108128579445));
#22076=CARTESIAN_POINT('Ctrl Pts',(5.27055683700799,4.2477579325433,52.5189420644236));
#22077=CARTESIAN_POINT('Ctrl Pts',(5.16011786372585,4.38126510315289,52.5270712709028));
#22078=CARTESIAN_POINT('Ctrl Pts',(5.04464975887452,4.51040993816386,52.5352004773819));
#22079=CARTESIAN_POINT('Ctrl Pts',(4.92924038507035,4.63948908567258,52.5433255490671));
#22080=CARTESIAN_POINT('Ctrl Pts',(4.80880721628425,4.76421004385035,52.5514506207524));
#22081=CARTESIAN_POINT('Ctrl Pts',(4.68372110033272,4.88416273831023,52.5595756924376));
#22082=CARTESIAN_POINT('Ctrl Pts',(4.55865929744746,5.00409211749017,52.5676991848477));
#22083=CARTESIAN_POINT('Ctrl Pts',(4.42894660773446,5.11925482125234,52.5758226772577));
#22084=CARTESIAN_POINT('Ctrl Pts',(4.29499117035121,5.22927718204009,52.5839461696677));
#22085=CARTESIAN_POINT('Ctrl Pts',(4.16105365691941,5.3392848212496,52.5920685751111));
#22086=CARTESIAN_POINT('Ctrl Pts',(4.0228748111491,5.44415325782776,52.6001909805546));
#22087=CARTESIAN_POINT('Ctrl Pts',(3.8808961193363,5.54354889136196,52.608313385998));
#22088=CARTESIAN_POINT('Ctrl Pts',(3.73886862973991,5.64297868697044,52.6164385830954));
#22089=CARTESIAN_POINT('Ctrl Pts',(3.59303898458832,5.73693171154433,52.6245637801929));
#22090=CARTESIAN_POINT('Ctrl Pts',(3.4438782889268,5.82511728045527,52.6326889772903));
#22091=CARTESIAN_POINT('Ctrl Pts',(3.33081901237669,5.89195926305005,52.638847629887));
#22092=CARTESIAN_POINT('Ctrl Pts',(3.21584661904426,5.95548860693522,52.6450062824837));
#22093=CARTESIAN_POINT('Ctrl Pts',(3.09917575053253,6.01559628526642,52.6511649350805));
#22094=CARTESIAN_POINT('Origin',(0.,0.,-3.69717978381041));
#22095=CARTESIAN_POINT('',(3.09917575053258,6.01559628526639,55.0458595242204));
#22096=CARTESIAN_POINT('',(3.09917575053251,6.01559628526643,54.6513758699904));
#22097=CARTESIAN_POINT('',(3.09917575053259,6.01559628526639,-3.69717978381041));
#22098=CARTESIAN_POINT('',(-6.76699752191952,-0.00579122915657409,53.6971797837779));
#22099=CARTESIAN_POINT('Ctrl Pts',(-6.76699752191893,-0.00579122983738126,
53.69717978381));
#22100=CARTESIAN_POINT('Ctrl Pts',(-6.76677989625174,-0.260084772302621,
53.7091640693841));
#22101=CARTESIAN_POINT('Ctrl Pts',(-6.75222508869606,-0.513791481686647,
53.7211483549582));
#22102=CARTESIAN_POINT('Ctrl Pts',(-6.72355008369308,-0.765613004115478,
53.7331326405323));
#22103=CARTESIAN_POINT('Ctrl Pts',(-6.70444183559884,-0.933420058570815,
53.7411186444391));
#22104=CARTESIAN_POINT('Ctrl Pts',(-6.6790643925138,-1.10039086166875,53.7491046483459));
#22105=CARTESIAN_POINT('Ctrl Pts',(-6.64749262677839,-1.26614800751213,
53.7570906522527));
#22106=CARTESIAN_POINT('Ctrl Pts',(-6.61497661658581,-1.43686259753244,
53.7653155005748));
#22107=CARTESIAN_POINT('Ctrl Pts',(-6.57583454917597,-1.60656341094717,
53.7735403488968));
#22108=CARTESIAN_POINT('Ctrl Pts',(-6.53014070694439,-1.77469753690816,
53.7817651972189));
#22109=CARTESIAN_POINT('Ctrl Pts',(-6.4844983261104,-1.94264230656458,53.7899807825381));
#22110=CARTESIAN_POINT('Ctrl Pts',(-6.43231895666366,-2.10902355915417,
53.7981963678573));
#22111=CARTESIAN_POINT('Ctrl Pts',(-6.37372820420558,-2.27329667639628,
53.8064119531765));
#22112=CARTESIAN_POINT('Ctrl Pts',(-6.31519166587682,-2.43741779142559,
53.8146199365997));
#22113=CARTESIAN_POINT('Ctrl Pts',(-6.25025567892752,-2.59943432009761,
53.822827920023));
#22114=CARTESIAN_POINT('Ctrl Pts',(-6.17909617111013,-2.7588148738493,53.8310359034462));
#22115=CARTESIAN_POINT('Ctrl Pts',(-6.10798821456512,-2.91807996488083,
53.8392379406227));
#22116=CARTESIAN_POINT('Ctrl Pts',(-6.03066586312489,-3.07471255832712,
53.8474399777993));
#22117=CARTESIAN_POINT('Ctrl Pts',(-5.94735388331155,-3.22819931024387,
53.8556420149758));
#22118=CARTESIAN_POINT('Ctrl Pts',(-5.86408552880434,-3.38160569068759,
53.8638397572552));
#22119=CARTESIAN_POINT('Ctrl Pts',(-5.77483396487451,-3.53186919668161,
53.8720374995346));
#22120=CARTESIAN_POINT('Ctrl Pts',(-5.67987084575693,-3.67849917432647,
53.880235241814));
#22121=CARTESIAN_POINT('Ctrl Pts',(-5.58492578230503,-3.82510127270745,
53.8884314254284));
#22122=CARTESIAN_POINT('Ctrl Pts',(-5.48427151635331,-3.96807091461804,
53.8966276090427));
#22123=CARTESIAN_POINT('Ctrl Pts',(-5.37822431914769,-4.10694438395851,
53.9048237926571));
#22124=CARTESIAN_POINT('Ctrl Pts',(-5.27218492849548,-4.24580763027392,
53.913019372918));
#22125=CARTESIAN_POINT('Ctrl Pts',(-5.16075361427734,-4.3805750188078,53.9212149531789));
#22126=CARTESIAN_POINT('Ctrl Pts',(-5.04428838637792,-4.51081408118899,
53.9294105334398));
#22127=CARTESIAN_POINT('Ctrl Pts',(-4.92781054247369,-4.64106725161484,
53.9376070014805));
#22128=CARTESIAN_POINT('Ctrl Pts',(-4.80629793773614,-4.76679085107235,
53.9458034695212));
#22129=CARTESIAN_POINT('Ctrl Pts',(-4.68014708707251,-4.8875875688694,53.9539999375619));
#22130=CARTESIAN_POINT('Ctrl Pts',(-4.55395961946476,-5.00841934950307,
53.9621987847353));
#22131=CARTESIAN_POINT('Ctrl Pts',(-4.42313148335591,-5.12432115180538,
53.9703976319087));
#22132=CARTESIAN_POINT('Ctrl Pts',(-4.28809409074618,-5.23493439012446,
53.9785964790821));
#22133=CARTESIAN_POINT('Ctrl Pts',(-4.1529155709298,-5.34566323003388,53.9868038948481));
#22134=CARTESIAN_POINT('Ctrl Pts',(-4.01351928378293,-5.45109223592226,
53.9950113106141));
#22135=CARTESIAN_POINT('Ctrl Pts',(-3.87036839545008,-5.55090420413658,
54.0032187263801));
#22136=CARTESIAN_POINT('Ctrl Pts',(-3.72714078327598,-5.65076966805529,
54.0114305410322));
#22137=CARTESIAN_POINT('Ctrl Pts',(-3.58015486006431,-5.74501189923058,
54.0196423556844));
#22138=CARTESIAN_POINT('Ctrl Pts',(-3.42990038334897,-5.83335858320938,
54.0278541703365));
#22139=CARTESIAN_POINT('Ctrl Pts',(-3.27942463407448,-5.92183537111111,
54.0360780781341));
#22140=CARTESIAN_POINT('Ctrl Pts',(-3.12567102790622,-6.00439909114341,
54.0443019859317));
#22141=CARTESIAN_POINT('Ctrl Pts',(-2.96915255132073,-6.08082413221971,
54.0525258937293));
#22142=CARTESIAN_POINT('Ctrl Pts',(-2.82453236958644,-6.15143945873337,
54.0601246326527));
#22143=CARTESIAN_POINT('Ctrl Pts',(-2.67755213333043,-6.21681438246504,
54.0677233715761));
#22144=CARTESIAN_POINT('Ctrl Pts',(-2.52862869857054,-6.27680857639975,
54.0753221104995));
#22145=CARTESIAN_POINT('Ctrl Pts',(-2.36888215716391,-6.34116288706281,
54.0834730926737));
#22146=CARTESIAN_POINT('Ctrl Pts',(-2.20642631344928,-6.39951591725883,
54.091624074848));
#22147=CARTESIAN_POINT('Ctrl Pts',(-2.04175619711414,-6.45162930053688,
54.0997750570223));
#22148=CARTESIAN_POINT('Ctrl Pts',(-1.87727736038111,-6.50368214929027,
54.1079165710753));
#22149=CARTESIAN_POINT('Ctrl Pts',(-1.71058971603811,-6.54950966947025,
54.1160580851284));
#22150=CARTESIAN_POINT('Ctrl Pts',(-1.54220965914812,-6.5889208803286,54.1241995991814));
#22151=CARTESIAN_POINT('Ctrl Pts',(-1.37398975796036,-6.62829460497709,
54.1323333693845));
#22152=CARTESIAN_POINT('Ctrl Pts',(-1.20408100262226,-6.66126408753093,
54.1404671395875));
#22153=CARTESIAN_POINT('Ctrl Pts',(-1.0330163950658,-6.68768765176165,54.1486009097906));
#22154=CARTESIAN_POINT('Ctrl Pts',(-0.862078518229963,-6.71409164048003,
54.1567286542086));
#22155=CARTESIAN_POINT('Ctrl Pts',(-0.689986854089072,-6.73395931129053,
54.1648563986266));
#22156=CARTESIAN_POINT('Ctrl Pts',(-0.51728608276181,-6.74719972348388,
54.1729841430445));
#22157=CARTESIAN_POINT('Ctrl Pts',(-0.344676945247087,-6.76043311040781,
54.1811075749386));
#22158=CARTESIAN_POINT('Ctrl Pts',(-0.171459708007611,-6.76704621375931,
54.1892310068326));
#22159=CARTESIAN_POINT('Ctrl Pts',(0.00181431908837062,-6.76699975677894,
54.1973544387267));
#22160=CARTESIAN_POINT('Ctrl Pts',(0.176187528458872,-6.76695300509376,
54.2055294024775));
#22161=CARTESIAN_POINT('Ctrl Pts',(0.350617878930557,-6.76016185860829,
54.2137043662283));
#22162=CARTESIAN_POINT('Ctrl Pts',(0.524541422292644,-6.74663955583068,
54.2218793299792));
#22163=CARTESIAN_POINT('Ctrl Pts',(0.697329413745348,-6.73320554056402,
54.2300009191522));
#22164=CARTESIAN_POINT('Ctrl Pts',(0.869616829378833,-6.71312805834558,
54.2381225083252));
#22165=CARTESIAN_POINT('Ctrl Pts',(1.04085417149711,-6.68647228317572,54.2462440974982));
#22166=CARTESIAN_POINT('Ctrl Pts',(1.21211412045663,-6.65981298889682,54.2543667588876));
#22167=CARTESIAN_POINT('Ctrl Pts',(1.38232335810515,-6.62657372812762,54.2624894202769));
#22168=CARTESIAN_POINT('Ctrl Pts',(1.55094109439532,-6.58687108737645,54.2706120816663));
#22169=CARTESIAN_POINT('Ctrl Pts',(1.71961320148922,-6.54715564450533,54.2787373622085));
#22170=CARTESIAN_POINT('Ctrl Pts',(1.88669242926656,-6.500972755372,54.2868626427508));
#22171=CARTESIAN_POINT('Ctrl Pts',(2.05165174144156,-6.44848929066645,54.294987923293));
#22172=CARTESIAN_POINT('Ctrl Pts',(2.21840825109433,-6.39543402950303,54.3032017270808));
#22173=CARTESIAN_POINT('Ctrl Pts',(2.3829980164088,-6.33594021797138,54.3114155308686));
#22174=CARTESIAN_POINT('Ctrl Pts',(2.54489678858769,-6.27023040529103,54.3196293346564));
#22175=CARTESIAN_POINT('Ctrl Pts',(2.7053278537605,-6.20511629047262,54.3277686755115));
#22176=CARTESIAN_POINT('Ctrl Pts',(2.86311620993667,-6.13389862319921,54.3359080163667));
#22177=CARTESIAN_POINT('Ctrl Pts',(3.01777638448957,-6.05684032257885,54.3440473572218));
#22178=CARTESIAN_POINT('Ctrl Pts',(3.17455892687851,-5.97872456770946,54.3522983924759));
#22179=CARTESIAN_POINT('Ctrl Pts',(3.32812646607889,-5.89460690617624,54.36054942773));
#22180=CARTESIAN_POINT('Ctrl Pts',(3.47800386231351,-5.80480646824098,54.3688004629841));
#22181=CARTESIAN_POINT('Ctrl Pts',(3.62788125854819,-5.71500603030568,54.3770514982382));
#22182=CARTESIAN_POINT('Ctrl Pts',(3.77406822709501,-5.61952308203906,54.3853025334923));
#22183=CARTESIAN_POINT('Ctrl Pts',(3.91612491505882,-5.51871856952821,54.3935535687464));
#22184=CARTESIAN_POINT('Ctrl Pts',(4.05784995134361,-5.41814939958594,54.4017853407773));
#22185=CARTESIAN_POINT('Ctrl Pts',(4.19590651381752,-5.31196967080089,54.4100171128081));
#22186=CARTESIAN_POINT('Ctrl Pts',(4.32982117865205,-5.20047474379947,54.418248884839));
#22187=CARTESIAN_POINT('Ctrl Pts',(4.4635759359942,-5.08911295288297,54.4264708273114));
#22188=CARTESIAN_POINT('Ctrl Pts',(4.59319837135361,-4.97244882885405,54.4346927697838));
#22189=CARTESIAN_POINT('Ctrl Pts',(4.71824369305165,-4.85082111121182,54.4429147122562));
#22190=CARTESIAN_POINT('Ctrl Pts',(4.84316475206892,-4.72931426003662,54.4511284842461));
#22191=CARTESIAN_POINT('Ctrl Pts',(4.96351750059756,-4.60285388646279,54.459342256236));
#22192=CARTESIAN_POINT('Ctrl Pts',(5.07888986678513,-4.47181917356542,54.4675560282259));
#22193=CARTESIAN_POINT('Ctrl Pts',(5.1941706901766,-4.34088843083354,54.4757632829563));
#22194=CARTESIAN_POINT('Ctrl Pts',(5.30447876646133,-4.2053908457353,54.4839705376866));
#22195=CARTESIAN_POINT('Ctrl Pts',(5.40943852255572,-4.06574272067111,54.492177792417));
#22196=CARTESIAN_POINT('Ctrl Pts',(5.51433601428634,-3.92617743785032,54.500380178429));
#22197=CARTESIAN_POINT('Ctrl Pts',(5.61389129159109,-3.78246680569833,54.5085825644409));
#22198=CARTESIAN_POINT('Ctrl Pts',(5.70776871342452,-3.63506056538984,54.5167849504529));
#22199=CARTESIAN_POINT('Ctrl Pts',(5.80161811512457,-3.48769832226867,54.5249848882516));
#22200=CARTESIAN_POINT('Ctrl Pts',(5.88979284162434,-3.33664296798299,54.5331848260503));
#22201=CARTESIAN_POINT('Ctrl Pts',(5.97200015707509,-3.18237381900605,54.541384763849));
#22202=CARTESIAN_POINT('Ctrl Pts',(6.05419597782134,-3.02812624083786,54.5495835550848));
#22203=CARTESIAN_POINT('Ctrl Pts',(6.13042588011323,-2.87066607878234,54.5577823463206));
#22204=CARTESIAN_POINT('Ctrl Pts',(6.20044273888851,-2.710497895547,54.5659811375563));
#22205=CARTESIAN_POINT('Ctrl Pts',(6.27046250892149,-2.55032305261763,54.5741802696928));
#22206=CARTESIAN_POINT('Ctrl Pts',(6.33426857712661,-2.38744029259166,54.5823794018292));
#22207=CARTESIAN_POINT('Ctrl Pts',(6.39166166953295,-2.22237487886794,54.5905785339656));
#22208=CARTESIAN_POINT('Ctrl Pts',(6.4490675596751,-2.05727265821384,54.5987794943765));
#22209=CARTESIAN_POINT('Ctrl Pts',(6.50005750820112,-1.88998715298163,54.6069804547875));
#22210=CARTESIAN_POINT('Ctrl Pts',(6.54448186788967,-1.72105958085806,54.6151814151984));
#22211=CARTESIAN_POINT('Ctrl Pts',(6.58894786389753,-1.55197368293349,54.6233900618834));
#22212=CARTESIAN_POINT('Ctrl Pts',(6.62683588539739,-1.3812429903637,54.6315987085685));
#22213=CARTESIAN_POINT('Ctrl Pts',(6.65804706090852,-1.20942066078247,54.6398073552535));
#22214=CARTESIAN_POINT('Ctrl Pts',(6.68927313751141,-1.03751629839533,54.6480199209771));
#22215=CARTESIAN_POINT('Ctrl Pts',(6.7138159620467,-0.864519614543845,54.6562324867006));
#22216=CARTESIAN_POINT('Ctrl Pts',(6.73162850336684,-0.690989647288,54.6644450524241));
#22217=CARTESIAN_POINT('Ctrl Pts',(6.74946548606402,-0.517221571876593,
54.6726688869729));
#22218=CARTESIAN_POINT('Ctrl Pts',(6.76055370632946,-0.342919108470499,
54.6808927215216));
#22219=CARTESIAN_POINT('Ctrl Pts',(6.76489825762268,-0.16864330408773,54.6891165560704));
#22220=CARTESIAN_POINT('Ctrl Pts',(6.76889008301258,-0.00851662268189041,
54.6966727130446));
#22221=CARTESIAN_POINT('Ctrl Pts',(6.76718940853875,0.151587348590576,54.7042288700189));
#22222=CARTESIAN_POINT('Ctrl Pts',(6.75983876983123,0.311237539327512,54.7117850269931));
#22223=CARTESIAN_POINT('Ctrl Pts',(6.75142820477987,0.493908510937084,54.7204307450454));
#22224=CARTESIAN_POINT('Ctrl Pts',(6.73560133324951,0.676401735153858,54.7290764630978));
#22225=CARTESIAN_POINT('Ctrl Pts',(6.71237252634239,0.858104928085077,54.7377221811502));
#22226=CARTESIAN_POINT('Ctrl Pts',(6.68917354048944,1.03957485114661,54.7463567998625));
#22227=CARTESIAN_POINT('Ctrl Pts',(6.65859160637791,1.22025646429683,54.7549914185748));
#22228=CARTESIAN_POINT('Ctrl Pts',(6.62069299883697,1.39954035852889,54.7636260372871));
#22229=CARTESIAN_POINT('Ctrl Pts',(6.58145595970188,1.58515586344356,54.7725655971896));
#22230=CARTESIAN_POINT('Ctrl Pts',(6.53437600806887,1.76927280158388,54.781505157092));
#22231=CARTESIAN_POINT('Ctrl Pts',(6.4795853778515,1.95122072845004,54.7904447169945));
#22232=CARTESIAN_POINT('Ctrl Pts',(6.42681061886781,2.1264743794821,54.799055370265));
#22233=CARTESIAN_POINT('Ctrl Pts',(6.3668825032131,2.29971543155046,54.8076660235354));
#22234=CARTESIAN_POINT('Ctrl Pts',(6.29997117461289,2.47035467069948,54.8162766768059));
#22235=CARTESIAN_POINT('Ctrl Pts',(6.23312318206175,2.6408323883924,54.824879179517));
#22236=CARTESIAN_POINT('Ctrl Pts',(6.15930526625744,2.80871292030108,54.8334816822281));
#22237=CARTESIAN_POINT('Ctrl Pts',(6.0787371052689,2.97342297781985,54.8420841849391));
#22238=CARTESIAN_POINT('Ctrl Pts',(5.99825962212379,3.13794765748433,54.8506770057066));
#22239=CARTESIAN_POINT('Ctrl Pts',(5.91104718384051,3.29930870803239,54.859269826474));
#22240=CARTESIAN_POINT('Ctrl Pts',(5.81736730544237,3.45695337451494,54.8678626472414));
#22241=CARTESIAN_POINT('Ctrl Pts',(5.80632670625338,3.47553251452534,54.8688753501998));
#22242=CARTESIAN_POINT('Ctrl Pts',(5.79519633069773,3.49406005925568,54.8698880531582));
#22243=CARTESIAN_POINT('Ctrl Pts',(5.78397666006704,3.51253512378164,54.8709007561166));
#22244=CARTESIAN_POINT('Ctrl Pts',(5.68875035480715,3.6693411648995,54.8794960138767));
#22245=CARTESIAN_POINT('Ctrl Pts',(5.58719985117846,3.8221801252544,54.8880912716368));
#22246=CARTESIAN_POINT('Ctrl Pts',(5.47968778795488,3.97055547077964,54.8966865293968));
#22247=CARTESIAN_POINT('Ctrl Pts',(5.37207504424347,4.11906976352366,54.9052898362513));
#22248=CARTESIAN_POINT('Ctrl Pts',(5.25848977672164,4.26311185076452,54.9138931431057));
#22249=CARTESIAN_POINT('Ctrl Pts',(5.13933507636798,4.40221807420007,54.9224964499602));
#22250=CARTESIAN_POINT('Ctrl Pts',(5.015240180819,4.5470916898964,54.9314564529002));
#22251=CARTESIAN_POINT('Ctrl Pts',(4.88510444856113,4.68661115451239,54.9404164558401));
#22252=CARTESIAN_POINT('Ctrl Pts',(4.74942480987268,4.82029594271616,54.9493764587801));
#22253=CARTESIAN_POINT('Ctrl Pts',(4.6187901463701,4.94900993024758,54.9580033019849));
#22254=CARTESIAN_POINT('Ctrl Pts',(4.48301667055892,5.07231515410789,54.9666301451896));
#22255=CARTESIAN_POINT('Ctrl Pts',(4.34258132168731,5.18982431923591,54.9752569883944));
#22256=CARTESIAN_POINT('Ctrl Pts',(4.20201175212178,5.30744579342153,54.9838920766805));
#22257=CARTESIAN_POINT('Ctrl Pts',(4.05677165544218,5.41925996304238,54.9925271649667));
#22258=CARTESIAN_POINT('Ctrl Pts',(3.90736828990719,5.52492190415645,55.0011622532529));
#22259=CARTESIAN_POINT('Ctrl Pts',(3.75774303039178,5.63074077445756,55.009810166378));
#22260=CARTESIAN_POINT('Ctrl Pts',(3.60394239921484,5.73038898730998,55.0184580795032));
#22261=CARTESIAN_POINT('Ctrl Pts',(3.44650092837927,5.82356594799792,55.0271059926284));
#22262=CARTESIAN_POINT('Ctrl Pts',(3.42883839211303,5.83401898453647,55.0280761568322));
#22263=CARTESIAN_POINT('Ctrl Pts',(3.41113005765446,5.84439062630108,55.029046321036));
#22264=CARTESIAN_POINT('Ctrl Pts',(3.39337669691533,5.85468048597291,55.0300164852398));
#22265=CARTESIAN_POINT('Ctrl Pts',(3.29673766573511,5.91069253260895,55.0352974982333));
#22266=CARTESIAN_POINT('Ctrl Pts',(3.19862976534322,5.96435855979782,55.0405785112269));
#22267=CARTESIAN_POINT('Ctrl Pts',(3.09917575053258,6.01559628526639,55.0458595242204));
#22268=CARTESIAN_POINT('Ctrl Pts',(3.09917575053258,6.01559628526639,53.0455807084606));
#22269=CARTESIAN_POINT('Ctrl Pts',(2.94389790458265,6.09559389679854,53.0537979533555));
#22270=CARTESIAN_POINT('Ctrl Pts',(2.785645637837,6.16951112027455,53.0620151982504));
#22271=CARTESIAN_POINT('Ctrl Pts',(2.62494151830489,6.23714446084739,53.0702324431454));
#22272=CARTESIAN_POINT('Ctrl Pts',(2.46067861284263,6.30627553888669,53.078631658581));
#22273=CARTESIAN_POINT('Ctrl Pts',(2.29385438133757,6.3688410547015,53.0870308740166));
#22274=CARTESIAN_POINT('Ctrl Pts',(2.12504217396318,6.42467779416819,53.0954300894522));
#22275=CARTESIAN_POINT('Ctrl Pts',(1.95622996658878,6.48051453363488,53.1038293048877));
#22276=CARTESIAN_POINT('Ctrl Pts',(1.78543017853457,6.5296224489739,53.1122285203233));
#22277=CARTESIAN_POINT('Ctrl Pts',(1.61322576824907,6.57189406645126,53.1206277357589));
#22278=CARTESIAN_POINT('Ctrl Pts',(1.44605108355753,6.61293101963649,53.1287816279257));
#22279=CARTESIAN_POINT('Ctrl Pts',(1.27703569613876,6.64765218906878,53.1369355200924));
#22280=CARTESIAN_POINT('Ctrl Pts',(1.10670232505557,6.6758893762342,53.1450894122591));
#22281=CARTESIAN_POINT('Ctrl Pts',(0.936576808273544,6.70409210614225,53.1532333543993));
#22282=CARTESIAN_POINT('Ctrl Pts',(0.765136865949179,6.72582654422594,53.1613772965395));
#22283=CARTESIAN_POINT('Ctrl Pts',(0.592919935417015,6.74097433240812,53.1695212386797));
#22284=CARTESIAN_POINT('Ctrl Pts',(0.420876909425892,6.75610682436395,53.1776569570726));
#22285=CARTESIAN_POINT('Ctrl Pts',(0.248058818721434,6.76466587584156,53.1857926754655));
#22286=CARTESIAN_POINT('Ctrl Pts',(0.0750128443173994,6.76658422493856,
53.1939283938584));
#22287=CARTESIAN_POINT('Ctrl Pts',(-0.0978947886393597,6.76850104041312,
53.2020576081586));
#22288=CARTESIAN_POINT('Ctrl Pts',(-0.271029578634426,6.76378772005493,
53.2101868224589));
#22289=CARTESIAN_POINT('Ctrl Pts',(-0.443839678090963,6.75242884747052,
53.2183160367591));
#22290=CARTESIAN_POINT('Ctrl Pts',(-0.616547960138858,6.74107666738254,
53.2264404614345));
#22291=CARTESIAN_POINT('Ctrl Pts',(-0.788931568674309,6.72308675649276,
53.2345648861099));
#22292=CARTESIAN_POINT('Ctrl Pts',(-0.960439117220119,6.69849577906215,
53.2426893107854));
#22293=CARTESIAN_POINT('Ctrl Pts',(-1.13298782637896,6.67375551865623,53.2508630559196));
#22294=CARTESIAN_POINT('Ctrl Pts',(-1.30464942893307,6.6423337798946,53.2590368010538));
#22295=CARTESIAN_POINT('Ctrl Pts',(-1.47486751946542,6.60432091891558,53.2672105461879));
#22296=CARTESIAN_POINT('Ctrl Pts',(-1.64399558315513,6.56655148117496,53.2753319490501));
#22297=CARTESIAN_POINT('Ctrl Pts',(-1.81169821212646,6.5222751928793,53.2834533519123));
#22298=CARTESIAN_POINT('Ctrl Pts',(-1.97744006838208,6.47163192525325,53.2915747547744));
#22299=CARTESIAN_POINT('Ctrl Pts',(-2.14319473892537,6.42098474215639,53.2996967855407));
#22300=CARTESIAN_POINT('Ctrl Pts',(-2.30698798475606,6.36396970609436,53.3078188163069));
#22301=CARTESIAN_POINT('Ctrl Pts',(-2.4683000816797,6.30077643681951,53.3159408470732));
#22302=CARTESIAN_POINT('Ctrl Pts',(-2.62965536795347,6.23756624831614,53.3240650524143));
#22303=CARTESIAN_POINT('Ctrl Pts',(-2.78852784195636,6.16817466633816,53.3321892577554));
#22304=CARTESIAN_POINT('Ctrl Pts',(-2.94441823979469,6.09283925843809,53.3403134630965));
#22305=CARTESIAN_POINT('Ctrl Pts',(-3.10199604332251,6.01668839687522,53.348525607339));
#22306=CARTESIAN_POINT('Ctrl Pts',(-3.25652648989856,5.93446444821664,53.3567377515815));
#22307=CARTESIAN_POINT('Ctrl Pts',(-3.40752067337968,5.84645977156177,53.3649498958239));
#22308=CARTESIAN_POINT('Ctrl Pts',(-3.55713644638242,5.75925848061124,53.3730870722404));
#22309=CARTESIAN_POINT('Ctrl Pts',(-3.70327997723185,5.6663818151341,53.3812242486569));
#22310=CARTESIAN_POINT('Ctrl Pts',(-3.84550626848677,5.56815683498848,53.3893614250733));
#22311=CARTESIAN_POINT('Ctrl Pts',(-3.98969805648939,5.46857443437359,53.3976110532288));
#22312=CARTESIAN_POINT('Ctrl Pts',(-4.12986322942873,5.36349504988159,53.4058606813842));
#22313=CARTESIAN_POINT('Ctrl Pts',(-4.26557448679539,5.25330022915122,53.4141103095397));
#22314=CARTESIAN_POINT('Ctrl Pts',(-4.4012857441621,5.14310540842081,53.4223599376951));
#22315=CARTESIAN_POINT('Ctrl Pts',(-4.53254283863639,5.02779545292852,53.4306095658506));
#22316=CARTESIAN_POINT('Ctrl Pts',(-4.6589590763726,4.90778863895802,53.4388591940061));
#22317=CARTESIAN_POINT('Ctrl Pts',(-4.783286477857,4.78976475525007,53.4469725095907));
#22318=CARTESIAN_POINT('Ctrl Pts',(-4.90332457913685,4.66682505072133,53.4550858251754));
#22319=CARTESIAN_POINT('Ctrl Pts',(-5.01865373847193,4.53931753166946,53.4631991407601));
#22320=CARTESIAN_POINT('Ctrl Pts',(-5.13385069024837,4.41195618083645,53.4713031556471));
#22321=CARTESIAN_POINT('Ctrl Pts',(-5.24434919911163,4.28003770958282,53.479407170534));
#22322=CARTESIAN_POINT('Ctrl Pts',(-5.34976387157572,4.14394926590363,53.487511185421));
#22323=CARTESIAN_POINT('Ctrl Pts',(-5.45508038457376,4.00798754432729,53.4956076540551));
#22324=CARTESIAN_POINT('Ctrl Pts',(-5.55532226046852,3.86786387087928,53.5037041226892));
#22325=CARTESIAN_POINT('Ctrl Pts',(-5.65014210968964,3.72400095868837,53.5118005913233));
#22326=CARTESIAN_POINT('Ctrl Pts',(-5.74488807005004,3.5802501524201,53.5198907507422));
#22327=CARTESIAN_POINT('Ctrl Pts',(-5.83422021707111,3.43276621887143,53.527980910161));
#22328=CARTESIAN_POINT('Ctrl Pts',(-5.91783259522884,3.28200340871961,53.5360710695798));
#22329=CARTESIAN_POINT('Ctrl Pts',(-6.00140935231352,3.13130482749169,53.5441577823778));
#22330=CARTESIAN_POINT('Ctrl Pts',(-6.07927101126975,2.97733047237376,53.5522444951759));
#22331=CARTESIAN_POINT('Ctrl Pts',(-6.15115588124769,2.82056205827704,53.5603312079739));
#22332=CARTESIAN_POINT('Ctrl Pts',(-6.22302411160969,2.66382993229214,53.5684160488927));
#22333=CARTESIAN_POINT('Ctrl Pts',(-6.28891815330792,2.50430537076334,53.5765008898115));
#22334=CARTESIAN_POINT('Ctrl Pts',(-6.34862312441312,2.3424929934083,53.5845857307303));
#22335=CARTESIAN_POINT('Ctrl Pts',(-6.40832589041272,2.18068659232917,53.5926702730487));
#22336=CARTESIAN_POINT('Ctrl Pts',(-6.46183991417272,2.01659289092625,53.6007548153671));
#22337=CARTESIAN_POINT('Ctrl Pts',(-6.50899918430194,1.85073461597192,53.6088393576855));
#22338=CARTESIAN_POINT('Ctrl Pts',(-6.55618318282665,1.68478937171109,53.6169281392078));
#22339=CARTESIAN_POINT('Ctrl Pts',(-6.59700566875786,1.51707806119666,53.6250169207301));
#22340=CARTESIAN_POINT('Ctrl Pts',(-6.6313509400887,1.34813712558655,53.6331057022524));
#22341=CARTESIAN_POINT('Ctrl Pts',(-6.66570576845019,1.17914917990377,53.6411967345862));
#22342=CARTESIAN_POINT('Ctrl Pts',(-6.69357972811641,1.00893129170854,53.64928776692));
#22343=CARTESIAN_POINT('Ctrl Pts',(-6.71490866735369,0.838027797330332,
53.6573787992538));
#22344=CARTESIAN_POINT('Ctrl Pts',(-6.73625802014904,0.666960734179693,
53.6654775753744));
#22345=CARTESIAN_POINT('Ctrl Pts',(-6.75104980613574,0.495207122242946,
53.673576351495));
#22346=CARTESIAN_POINT('Ctrl Pts',(-6.7592718950147,0.323314783553781,53.6816751276156));
#22347=CARTESIAN_POINT('Ctrl Pts',(-6.76451880553983,0.213622011517981,
53.6868433463364));
#22348=CARTESIAN_POINT('Ctrl Pts',(-6.76709137289696,0.103872766967097,
53.6920115650572));
#22349=CARTESIAN_POINT('Ctrl Pts',(-6.76699752191952,-0.00579122915667694,
53.697179783778));
#22350=CARTESIAN_POINT('',(-6.76699862526772,-0.00431342378654712,53.3028202162263));
#22351=CARTESIAN_POINT('Ctrl Pts',(3.09917575053253,6.01559628526642,52.6511649350805));
#22352=CARTESIAN_POINT('Ctrl Pts',(2.94515939621147,6.09494398877942,52.6592949270191));
#22353=CARTESIAN_POINT('Ctrl Pts',(2.78818271189624,6.16832714753178,52.6674249189578));
#22354=CARTESIAN_POINT('Ctrl Pts',(2.6287573478755,6.23553717060452,52.6755549108964));
#22355=CARTESIAN_POINT('Ctrl Pts',(2.46914177694221,6.30282738048479,52.6836946025505));
#22356=CARTESIAN_POINT('Ctrl Pts',(2.30707202997899,6.36392960719194,52.6918342942046));
#22357=CARTESIAN_POINT('Ctrl Pts',(2.14307717840784,6.41868438290804,52.6999739858587));
#22358=CARTESIAN_POINT('Ctrl Pts',(1.97896652703362,6.47347782198572,52.7081194250999));
#22359=CARTESIAN_POINT('Ctrl Pts',(1.81292841243395,6.52191477893482,52.7162648643411));
#22360=CARTESIAN_POINT('Ctrl Pts',(1.64550328180379,6.5638866496591,52.7244103035823));
#22361=CARTESIAN_POINT('Ctrl Pts',(1.47784304389534,6.60591745951787,52.7325671810827));
#22362=CARTESIAN_POINT('Ctrl Pts',(1.30879225749729,6.64146498483198,52.7407240585831));
#22363=CARTESIAN_POINT('Ctrl Pts',(1.13889846745706,6.67047219324269,52.7488809360836));
#22364=CARTESIAN_POINT('Ctrl Pts',(1.09418564949929,6.67810633942793,52.7510276712803));
#22365=CARTESIAN_POINT('Ctrl Pts',(1.04941445079136,6.6852877556321,52.753174406477));
#22366=CARTESIAN_POINT('Ctrl Pts',(1.0045948586897,6.69201600191558,52.7553211416737));
#22367=CARTESIAN_POINT('Ctrl Pts',(0.832705028385672,6.71781983139463,52.7635541918057));
#22368=CARTESIAN_POINT('Ctrl Pts',(0.659569085890686,6.73703443976784,52.7717872419377));
#22369=CARTESIAN_POINT('Ctrl Pts',(0.485733193020823,6.7495445968745,52.7800202920697));
#22370=CARTESIAN_POINT('Ctrl Pts',(0.312104311977997,6.76203985630706,52.7882435379046));
#22371=CARTESIAN_POINT('Ctrl Pts',(0.137777494084929,6.76784653707539,52.7964667837394));
#22372=CARTESIAN_POINT('Ctrl Pts',(-0.0366916789560165,6.76690052540271,
52.8046900295743));
#22373=CARTESIAN_POINT('Ctrl Pts',(-0.21098800641131,6.76595545093823,52.8129051286877));
#22374=CARTESIAN_POINT('Ctrl Pts',(-0.385426052436014,6.75827100888565,
52.8211202278012));
#22375=CARTESIAN_POINT('Ctrl Pts',(-0.559445794775028,6.74383491810917,
52.8293353269147));
#22376=CARTESIAN_POINT('Ctrl Pts',(-0.733327954622235,6.72941024071209,
52.8375439310536));
#22377=CARTESIAN_POINT('Ctrl Pts',(-0.906792114155987,6.70824457619736,
52.8457525351925));
#22378=CARTESIAN_POINT('Ctrl Pts',(-1.07927883681853,6.6803776983338,52.8539611393313));
#22379=CARTESIAN_POINT('Ctrl Pts',(-1.2516636911726,6.65252727826866,52.8621648955804));
#22380=CARTESIAN_POINT('Ctrl Pts',(-1.42307190598866,6.61798358599597,52.8703686518295));
#22381=CARTESIAN_POINT('Ctrl Pts',(-1.59294965437233,6.57683817640628,52.8785724080786));
#22382=CARTESIAN_POINT('Ctrl Pts',(-1.76277714020926,6.53570494070689,52.8867737370429));
#22383=CARTESIAN_POINT('Ctrl Pts',(-1.93107471304449,6.48797395901418,52.8949750660072));
#22384=CARTESIAN_POINT('Ctrl Pts',(-2.0972989744039,6.433787843251,52.9031763949714));
#22385=CARTESIAN_POINT('Ctrl Pts',(-2.26350031185091,6.37960920027044,52.9113765928942));
#22386=CARTESIAN_POINT('Ctrl Pts',(-2.42762856652253,6.31897730647894,52.9195767908169));
#22387=CARTESIAN_POINT('Ctrl Pts',(-2.589155718125,6.25208458574423,52.9277769887396));
#22388=CARTESIAN_POINT('Ctrl Pts',(-2.75068986559701,6.18518896783253,52.9359775418194));
#22389=CARTESIAN_POINT('Ctrl Pts',(-2.90962235449856,6.11203211979522,52.9441780948992));
#22390=CARTESIAN_POINT('Ctrl Pts',(-3.06544530637694,6.03285455432266,52.9523786479791));
#22391=CARTESIAN_POINT('Ctrl Pts',(-3.22130324524423,5.95365921108004,52.9605810423323));
#22392=CARTESIAN_POINT('Ctrl Pts',(-3.37404993715094,5.86844062019941,52.9687834366855));
#22393=CARTESIAN_POINT('Ctrl Pts',(-3.5232022135851,5.77748519359323,52.9769858310388));
#22394=CARTESIAN_POINT('Ctrl Pts',(-3.67249397361664,5.68644470767448,52.9851958960726));
#22395=CARTESIAN_POINT('Ctrl Pts',(-3.81818429606853,5.5896568540881,52.9934059611064));
#22396=CARTESIAN_POINT('Ctrl Pts',(-3.95981833588254,5.48745184460041,53.0016160261403));
#22397=CARTESIAN_POINT('Ctrl Pts',(-4.1015201592352,5.38519792160845,53.0098300203656));
#22398=CARTESIAN_POINT('Ctrl Pts',(-4.23916154734745,5.27752189422133,53.0180440145909));
#22399=CARTESIAN_POINT('Ctrl Pts',(-4.37232094003325,5.1647941485936,53.0262580088162));
#22400=CARTESIAN_POINT('Ctrl Pts',(-4.50566187332155,5.05191271750331,53.0344832014514));
#22401=CARTESIAN_POINT('Ctrl Pts',(-4.63450833501256,4.93396604605028,53.0427083940865));
#22402=CARTESIAN_POINT('Ctrl Pts',(-4.7584749478192,4.81136209102756,53.0509335867217));
#22403=CARTESIAN_POINT('Ctrl Pts',(-4.86995785720111,4.70110461687214,53.0583304848416));
#22404=CARTESIAN_POINT('Ctrl Pts',(-4.97749464124063,4.58708124221604,53.0657273829615));
#22405=CARTESIAN_POINT('Ctrl Pts',(-5.08083346162143,4.46961075880976,53.0731242810814));
#22406=CARTESIAN_POINT('Ctrl Pts',(-5.2016224685459,4.33230376245259,53.0817702475723));
#22407=CARTESIAN_POINT('Ctrl Pts',(-5.31694983733856,4.1899752222184,53.0904162140632));
#22408=CARTESIAN_POINT('Ctrl Pts',(-5.42640085573318,4.0430759024409,53.0990621805541));
#22409=CARTESIAN_POINT('Ctrl Pts',(-5.53571187139551,3.89636448686419,53.1076970876785));
#22410=CARTESIAN_POINT('Ctrl Pts',(-5.63916134397898,3.74509419367296,53.1163319948028));
#22411=CARTESIAN_POINT('Ctrl Pts',(-5.73637392148778,3.58974974515981,53.1249669019272));
#22412=CARTESIAN_POINT('Ctrl Pts',(-5.83681387810786,3.4292479863373,53.1338884809987));
#22413=CARTESIAN_POINT('Ctrl Pts',(-5.93059546957259,3.26439712748198,53.1428100600702));
#22414=CARTESIAN_POINT('Ctrl Pts',(-6.01735067509065,3.0957680554244,53.1517316391417));
#22415=CARTESIAN_POINT('Ctrl Pts',(-6.10108632156991,2.93300820395935,53.1603426981174));
#22416=CARTESIAN_POINT('Ctrl Pts',(-6.17827625866201,2.76672900032398,53.1689537570931));
#22417=CARTESIAN_POINT('Ctrl Pts',(-6.24863382533625,2.59747267875211,53.1775648160689));
#22418=CARTESIAN_POINT('Ctrl Pts',(-6.31892504157508,2.42837597370996,53.1861677544182));
#22419=CARTESIAN_POINT('Ctrl Pts',(-6.38239661685956,2.25630802893954,53.1947706927676));
#22420=CARTESIAN_POINT('Ctrl Pts',(-6.43880859873856,2.0818340060654,53.2033736311169));
#22421=CARTESIAN_POINT('Ctrl Pts',(-6.49515741224976,1.90755535372928,53.2119669361657));
#22422=CARTESIAN_POINT('Ctrl Pts',(-6.54446230921303,1.73087628779443,53.2205602412146));
#22423=CARTESIAN_POINT('Ctrl Pts',(-6.58653202175268,1.55238040648114,53.2291535462634));
#22424=CARTESIAN_POINT('Ctrl Pts',(-6.59121927634099,1.53249304362142,53.230110981104));
#22425=CARTESIAN_POINT('Ctrl Pts',(-6.59581676624511,1.51258314576003,53.2310684159446));
#22426=CARTESIAN_POINT('Ctrl Pts',(-6.60032426476746,1.4926515333198,53.2320258507851));
#22427=CARTESIAN_POINT('Ctrl Pts',(-6.63752498744106,1.32815444404714,53.2399276321848));
#22428=CARTESIAN_POINT('Ctrl Pts',(-6.66857070888122,1.16227112455706,53.2478294135844));
#22429=CARTESIAN_POINT('Ctrl Pts',(-6.69337176356371,0.995521689732583,
53.255731194984));
#22430=CARTESIAN_POINT('Ctrl Pts',(-6.71818808436948,0.828669613409205,
53.2636378402723));
#22431=CARTESIAN_POINT('Ctrl Pts',(-6.73675200528878,0.660950739777101,
53.2715444855606));
#22432=CARTESIAN_POINT('Ctrl Pts',(-6.74902561190871,0.492891762763725,
53.2794511308489));
#22433=CARTESIAN_POINT('Ctrl Pts',(-6.76111767498075,0.327318609509081,
53.2872408259626));
#22434=CARTESIAN_POINT('Ctrl Pts',(-6.76710426439709,0.16141570621137,53.2950305210762));
#22435=CARTESIAN_POINT('Ctrl Pts',(-6.76699862526822,-0.00431342301278818,
53.3028202161899));
#22436=CARTESIAN_POINT('Ctrl Pts',(-6.76699862526772,-0.00431342378654577,
53.3028202162263));
#22437=CARTESIAN_POINT('Ctrl Pts',(-6.7668657739302,-0.212733663223811,
53.3126165032661));
#22438=CARTESIAN_POINT('Ctrl Pts',(-6.75710010762463,-0.420817753426841,
53.3224127903059));
#22439=CARTESIAN_POINT('Ctrl Pts',(-6.73781830924752,-0.627768613080422,
53.3322090773457));
#22440=CARTESIAN_POINT('Ctrl Pts',(-6.71837254760011,-0.836479284711892,
53.3420886673653));
#22441=CARTESIAN_POINT('Ctrl Pts',(-6.68924817378419,-1.04403733784282,
53.3519682573849));
#22442=CARTESIAN_POINT('Ctrl Pts',(-6.65061516021554,-1.2496427452321,53.3618478474045));
#22443=CARTESIAN_POINT('Ctrl Pts',(-6.61271103871109,-1.45136897944904,
53.3715410384327));
#22444=CARTESIAN_POINT('Ctrl Pts',(-6.5656539155427,-1.65121560294499,53.3812342294609));
#22445=CARTESIAN_POINT('Ctrl Pts',(-6.50965016194429,-1.84844360722711,
53.3909274204891));
#22446=CARTESIAN_POINT('Ctrl Pts',(-6.46212335079957,-2.01581842605051,
53.3991534130305));
#22447=CARTESIAN_POINT('Ctrl Pts',(-6.40807475476983,-2.18157874669713,
53.4073794055718));
#22448=CARTESIAN_POINT('Ctrl Pts',(-6.34763095885382,-2.34518020847024,
53.4156053981132));
#22449=CARTESIAN_POINT('Ctrl Pts',(-6.28725053044514,-2.50861015525707,
53.4238227667646));
#22450=CARTESIAN_POINT('Ctrl Pts',(-6.22048837652145,-2.66988541688268,
53.432040135416));
#22451=CARTESIAN_POINT('Ctrl Pts',(-6.14752138460948,-2.82847482325177,
53.4402575040674));
#22452=CARTESIAN_POINT('Ctrl Pts',(-6.0746162887784,-2.98692970217952,53.4484679021298));
#22453=CARTESIAN_POINT('Ctrl Pts',(-5.99551698666296,-3.14270293981774,
53.4566783001921));
#22454=CARTESIAN_POINT('Ctrl Pts',(-5.9104491970952,-3.29528136713038,53.4648886982545));
#22455=CARTESIAN_POINT('Ctrl Pts',(-5.82543655151031,-3.44776088765088,
53.4730937740433));
#22456=CARTESIAN_POINT('Ctrl Pts',(-5.7344632990645,-3.59704941129093,53.4812988498321));
#22457=CARTESIAN_POINT('Ctrl Pts',(-5.63780205186725,-3.74265641275839,
53.4895039256209));
#22458=CARTESIAN_POINT('Ctrl Pts',(-5.54118413182602,-3.88819814776742,
53.4977053235904));
#22459=CARTESIAN_POINT('Ctrl Pts',(-5.43888349427051,-4.03006135039806,
53.5059067215598));
#22460=CARTESIAN_POINT('Ctrl Pts',(-5.33121725879015,-4.16778256865422,
53.5141081195293));
#22461=CARTESIAN_POINT('Ctrl Pts',(-5.22355945662589,-4.30549299943778,
53.522308875097));
#22462=CARTESIAN_POINT('Ctrl Pts',(-5.11053710730422,-4.43906180466784,
53.5305096306648));
#22463=CARTESIAN_POINT('Ctrl Pts',(-4.99250921412986,-4.5680565612554,53.5387103862325));
#22464=CARTESIAN_POINT('Ctrl Pts',(-4.87448192048102,-4.69705066261098,
53.5469111001442));
#22465=CARTESIAN_POINT('Ctrl Pts',(-4.75144937475753,-4.82147049648515,
53.555111814056));
#22466=CARTESIAN_POINT('Ctrl Pts',(-4.62380914846253,-4.94091873628723,
53.5633125279678));
#22467=CARTESIAN_POINT('Ctrl Pts',(-4.496146438932,-5.06038801634432,53.5715146863974));
#22468=CARTESIAN_POINT('Ctrl Pts',(-4.36387469348221,-5.1748837127253,53.579716844827));
#22469=CARTESIAN_POINT('Ctrl Pts',(-4.22742646181163,-5.28404717143733,
53.5879190032566));
#22470=CARTESIAN_POINT('Ctrl Pts',(-4.09092946733719,-5.39324964213406,
53.5961240929096));
#22471=CARTESIAN_POINT('Ctrl Pts',(-3.95025329303532,-5.49711585537118,
53.6043291825625));
#22472=CARTESIAN_POINT('Ctrl Pts',(-3.80586153818101,-5.59532902984217,
53.6125342722155));
#22473=CARTESIAN_POINT('Ctrl Pts',(-3.6613048328186,-5.69365440125299,53.6207487352133));
#22474=CARTESIAN_POINT('Ctrl Pts',(-3.51302436353896,-5.78631363033407,
53.628963198211));
#22475=CARTESIAN_POINT('Ctrl Pts',(-3.36151144712169,-5.87303412137797,
53.6371776612088));
#22476=CARTESIAN_POINT('Ctrl Pts',(-3.20990876409008,-5.95980599157196,
53.6453969910163));
#22477=CARTESIAN_POINT('Ctrl Pts',(-3.05507013350502,-6.04063194441922,
53.6536163208237));
#22478=CARTESIAN_POINT('Ctrl Pts',(-2.89750906385215,-6.11528660202403,
53.6618356506312));
#22479=CARTESIAN_POINT('Ctrl Pts',(-2.73970386287458,-6.19005693249459,
53.6700677157919));
#22480=CARTESIAN_POINT('Ctrl Pts',(-2.5791681224417,-6.25863671833393,53.6782997809526));
#22481=CARTESIAN_POINT('Ctrl Pts',(-2.4164340604615,-6.32084926504671,53.6865318461133));
#22482=CARTESIAN_POINT('Ctrl Pts',(-2.27015700060778,-6.37677036913779,
53.6939314173744));
#22483=CARTESIAN_POINT('Ctrl Pts',(-2.12210415199189,-6.4275475489319,53.7013309886355));
#22484=CARTESIAN_POINT('Ctrl Pts',(-1.97266978345942,-6.47308758827085,
53.7087305598966));
#22485=CARTESIAN_POINT('Ctrl Pts',(-1.80797027127025,-6.5232796715102,53.7168860183034));
#22486=CARTESIAN_POINT('Ctrl Pts',(-1.64108525912738,-6.56726366386642,
53.7250414767102));
#22487=CARTESIAN_POINT('Ctrl Pts',(-1.47252769844495,-6.60484300928587,
53.7331969351169));
#22488=CARTESIAN_POINT('Ctrl Pts',(-1.30417529447042,-6.64237661570222,
53.7413424672588));
#22489=CARTESIAN_POINT('Ctrl Pts',(-1.13415474695746,-6.67352101341617,
53.7494879994007));
#22490=CARTESIAN_POINT('Ctrl Pts',(-0.962996420609403,-6.6981286113282,
53.7576335315426));
#22491=CARTESIAN_POINT('Ctrl Pts',(-0.792010425280498,-6.72271143304315,
53.7657708623432));
#22492=CARTESIAN_POINT('Ctrl Pts',(-0.619889290828873,-6.7407705061041,
53.7739081931437));
#22493=CARTESIAN_POINT('Ctrl Pts',(-0.447175898437896,-6.75220872869436,
53.7820455239443));
#22494=CARTESIAN_POINT('Ctrl Pts',(-0.274600106533052,-6.7636378384708,
53.7901763717463));
#22495=CARTESIAN_POINT('Ctrl Pts',(-0.101433359209004,-6.76845657656059,
53.7983072195483));
#22496=CARTESIAN_POINT('Ctrl Pts',(0.0717739725180646,-6.76661935510407,
53.8064380673503));
#22497=CARTESIAN_POINT('Ctrl Pts',(0.244879695437417,-6.76478321141879,
53.8145641453441));
#22498=CARTESIAN_POINT('Ctrl Pts',(0.418025590781101,-6.75629888797378,
53.8226902233378));
#22499=CARTESIAN_POINT('Ctrl Pts',(0.590658902779662,-6.74117282530029,
53.8308163013316));
#22500=CARTESIAN_POINT('Ctrl Pts',(0.763904340972275,-6.72599312837124,
53.8389711929138));
#22501=CARTESIAN_POINT('Ctrl Pts',(0.936633182670272,-6.7041244865418,53.8471260844961));
#22502=CARTESIAN_POINT('Ctrl Pts',(1.10828892944676,-6.67562616155711,53.8552809760782));
#22503=CARTESIAN_POINT('Ctrl Pts',(1.27927527882838,-6.64723897007574,53.8634040664345));
#22504=CARTESIAN_POINT('Ctrl Pts',(1.44919652710337,-6.61227378673521,53.8715271567908));
#22505=CARTESIAN_POINT('Ctrl Pts',(1.61751027262617,-6.57084085318986,53.8796502471471));
#22506=CARTESIAN_POINT('Ctrl Pts',(1.78583723491278,-6.52940466614138,53.8877739753655));
#22507=CARTESIAN_POINT('Ctrl Pts',(1.95255608777658,-6.48149980465698,53.895897703584));
#22508=CARTESIAN_POINT('Ctrl Pts',(2.11713728372672,-6.42728704212394,53.9040214318024));
#22509=CARTESIAN_POINT('Ctrl Pts',(2.28176271472091,-6.37305970864356,53.9121473434627));
#22510=CARTESIAN_POINT('Ctrl Pts',(2.44424899745888,-6.31252121266928,53.920273255123));
#22511=CARTESIAN_POINT('Ctrl Pts',(2.60408437468839,-6.2458813284839,53.9283991667834));
#22512=CARTESIAN_POINT('Ctrl Pts',(2.76494191577037,-6.17881527531186,53.9365770444934));
#22513=CARTESIAN_POINT('Ctrl Pts',(2.92311418135037,-6.10556966957484,53.9447549222035));
#22514=CARTESIAN_POINT('Ctrl Pts',(3.07810327724429,-6.02640599483788,53.9529327999136));
#22515=CARTESIAN_POINT('Ctrl Pts',(3.23235264379837,-5.947620151151,53.961071646387));
#22516=CARTESIAN_POINT('Ctrl Pts',(3.38344887013187,-5.86297283847708,53.9692104928605));
#22517=CARTESIAN_POINT('Ctrl Pts',(3.53092932571211,-5.77276598320305,53.9773493393339));
#22518=CARTESIAN_POINT('Ctrl Pts',(3.67947068308868,-5.68191022421886,53.9855467326623));
#22519=CARTESIAN_POINT('Ctrl Pts',(3.82434373903263,-5.58541484526097,53.9937441259907));
#22520=CARTESIAN_POINT('Ctrl Pts',(3.9651091049225,-5.48363007377966,54.0019415193191));
#22521=CARTESIAN_POINT('Ctrl Pts',(4.10587447081243,-5.38184530229831,54.0101389126475));
#22522=CARTESIAN_POINT('Ctrl Pts',(4.24253189133332,-5.27477141597334,54.0183363059759));
#22523=CARTESIAN_POINT('Ctrl Pts',(4.3746794556649,-5.16279659295071,54.0265336993043));
#22524=CARTESIAN_POINT('Ctrl Pts',(4.50729155368351,-5.05042814876937,54.0347599086413));
#22525=CARTESIAN_POINT('Ctrl Pts',(4.63575678636189,-4.93278991264607,54.0429861179783));
#22526=CARTESIAN_POINT('Ctrl Pts',(4.7596304403996,-4.81021902524423,54.0512123273153));
#22527=CARTESIAN_POINT('Ctrl Pts',(4.88336492769362,-4.68778584098357,54.0594292948585));
#22528=CARTESIAN_POINT('Ctrl Pts',(5.00251785559057,-4.56043129027937,54.0676462624017));
#22529=CARTESIAN_POINT('Ctrl Pts',(5.11667701461948,-4.42853308986901,54.0758632299448));
#22530=CARTESIAN_POINT('Ctrl Pts',(5.23073083338146,-4.29675659841091,54.0840726152882));
#22531=CARTESIAN_POINT('Ctrl Pts',(5.33979982704329,-4.16044507653162,54.0922820006316));
#22532=CARTESIAN_POINT('Ctrl Pts',(5.44350809155414,-4.02001351455249,54.100491385975));
#22533=CARTESIAN_POINT('Ctrl Pts',(5.54714146775072,-3.87968335898484,54.1086948432756));
#22534=CARTESIAN_POINT('Ctrl Pts',(5.64542161299945,-3.73523937653856,54.1168983005762));
#22535=CARTESIAN_POINT('Ctrl Pts',(5.73801238649264,-3.58713016943309,54.1251017578768));
#22536=CARTESIAN_POINT('Ctrl Pts',(5.83055487315543,-3.43909820246606,54.1333009370086));
#22537=CARTESIAN_POINT('Ctrl Pts',(5.91741370930256,-3.28740512215544,54.1415001161405));
#22538=CARTESIAN_POINT('Ctrl Pts',(5.99829559759164,-3.13252915771151,54.1496992952724));
#22539=CARTESIAN_POINT('Ctrl Pts',(6.07916224598982,-2.97768237523713,54.1578969295022));
#22540=CARTESIAN_POINT('Ctrl Pts',(6.15405401841697,-2.81965421790738,54.166094563732));
#22541=CARTESIAN_POINT('Ctrl Pts',(6.22272303809128,-2.65894847471853,54.1742921979618));
#22542=CARTESIAN_POINT('Ctrl Pts',(6.29138710116054,-2.49825433144625,54.1824892404774));
#22543=CARTESIAN_POINT('Ctrl Pts',(6.3538291642663,-2.33488331670718,54.190686282993));
#22544=CARTESIAN_POINT('Ctrl Pts',(6.4098491032884,-2.16936015291905,54.1988833255086));
#22545=CARTESIAN_POINT('Ctrl Pts',(6.46587518026003,-2.0038188532164,54.2070812661514));
#22546=CARTESIAN_POINT('Ctrl Pts',(6.51547761625543,-1.83612527449301,54.2152792067943));
#22547=CARTESIAN_POINT('Ctrl Pts',(6.55850584910796,-1.66682033441422,54.2234771474371));
#22548=CARTESIAN_POINT('Ctrl Pts',(6.60154661678304,-1.49746607305868,54.2316774762731));
#22549=CARTESIAN_POINT('Ctrl Pts',(6.63800927819798,-1.32649986287014,54.2398778051091));
#22550=CARTESIAN_POINT('Ctrl Pts',(6.66779416029866,-1.15447392170076,54.2480781339451));
#22551=CARTESIAN_POINT('Ctrl Pts',(6.69761007901933,-0.982268725037,54.2562870077365));
#22552=CARTESIAN_POINT('Ctrl Pts',(6.72073425528281,-0.809001945121539,
54.2644958815279));
#22553=CARTESIAN_POINT('Ctrl Pts',(6.73711866972606,-0.635233051744458,
54.2727047553193));
#22554=CARTESIAN_POINT('Ctrl Pts',(6.7535118775038,-0.461370898519205,54.2809180347227));
#22555=CARTESIAN_POINT('Ctrl Pts',(6.76315809274141,-0.287006452402152,
54.2891313141262));
#22556=CARTESIAN_POINT('Ctrl Pts',(6.76606145846543,-0.112700223019793,
54.2973445935296));
#22557=CARTESIAN_POINT('Ctrl Pts',(6.76896907081815,0.0618609566189891,
54.3055698861451));
#22558=CARTESIAN_POINT('Ctrl Pts',(6.76511413205971,0.236363390784799,54.3137951787605));
#22559=CARTESIAN_POINT('Ctrl Pts',(6.75455286888362,0.410249364967281,54.3220204713759));
#22560=CARTESIAN_POINT('Ctrl Pts',(6.74500147500663,0.567508340660824,54.329459260488));
#22561=CARTESIAN_POINT('Ctrl Pts',(6.72996565522437,0.724262994944808,54.3368980496));
#22562=CARTESIAN_POINT('Ctrl Pts',(6.70952298555752,0.880108121923286,54.3443368387121));
#22563=CARTESIAN_POINT('Ctrl Pts',(6.68691590961242,1.05245364619639,54.3525632236772));
#22564=CARTESIAN_POINT('Ctrl Pts',(6.65763248579208,1.22416845318491,54.3607896086424));
#22565=CARTESIAN_POINT('Ctrl Pts',(6.62171517814278,1.39469605991898,54.3690159936076));
#22566=CARTESIAN_POINT('Ctrl Pts',(6.58583838831994,1.56503129677822,54.3772330984997));
#22567=CARTESIAN_POINT('Ctrl Pts',(6.54334269003506,1.73418165247868,54.3854502033918));
#22568=CARTESIAN_POINT('Ctrl Pts',(6.49432226520474,1.90159599170432,54.393667308284));
#22569=CARTESIAN_POINT('Ctrl Pts',(6.44534730067471,2.06885507511243,54.4018767928412));
#22570=CARTESIAN_POINT('Ctrl Pts',(6.38985976052621,2.2343810063116,54.4100862773984));
#22571=CARTESIAN_POINT('Ctrl Pts',(6.32800482632947,2.39763298232881,54.4182957619556));
#22572=CARTESIAN_POINT('Ctrl Pts',(6.26619484386969,2.56076631849977,54.4264992804472));
#22573=CARTESIAN_POINT('Ctrl Pts',(6.19802681108652,2.72162865713693,54.4347027989389));
#22574=CARTESIAN_POINT('Ctrl Pts',(6.12369570284242,2.87969441764041,54.4429063174306));
#22575=CARTESIAN_POINT('Ctrl Pts',(6.04940370234929,3.03767701516481,54.4511055198133));
#22576=CARTESIAN_POINT('Ctrl Pts',(5.96895523867511,3.1928656420963,54.4593047221961));
#22577=CARTESIAN_POINT('Ctrl Pts',(5.88259339742212,3.34475468765733,54.4675039245789));
#22578=CARTESIAN_POINT('Ctrl Pts',(5.79625018319389,3.49661097290464,54.4757013585099));
#22579=CARTESIAN_POINT('Ctrl Pts',(5.70399630503805,3.64516878067554,54.483898792441));
#22580=CARTESIAN_POINT('Ctrl Pts',(5.6061209149474,3.7899468712621,54.492096226372));
#22581=CARTESIAN_POINT('Ctrl Pts',(5.50825324360556,3.93471354421126,54.5002930138287));
#22582=CARTESIAN_POINT('Ctrl Pts',(5.40476514373408,4.07570079626699,54.5084898012854));
#22583=CARTESIAN_POINT('Ctrl Pts',(5.29598922111453,4.21245619203793,54.516686588742));
#22584=CARTESIAN_POINT('Ctrl Pts',(5.18720210735474,4.34922565754762,54.5248842195048));
#22585=CARTESIAN_POINT('Ctrl Pts',(5.07312631060924,4.48176211890996,54.5330818502675));
#22586=CARTESIAN_POINT('Ctrl Pts',(4.95413488642051,4.60964603057016,54.5412794810303));
#22587=CARTESIAN_POINT('Ctrl Pts',(4.83510959399437,4.73756634151469,54.5494794450646));
#22588=CARTESIAN_POINT('Ctrl Pts',(4.7111661317907,4.86083120287225,54.5576794090989));
#22589=CARTESIAN_POINT('Ctrl Pts',(4.582714608375,4.97905772392592,54.5658793731332));
#22590=CARTESIAN_POINT('Ctrl Pts',(4.45414192612709,5.09739575932248,54.5740870715878));
#22591=CARTESIAN_POINT('Ctrl Pts',(4.32105295405945,5.2106857196889,54.5822947700423));
#22592=CARTESIAN_POINT('Ctrl Pts',(4.18389174031732,5.31858429521471,54.5905024684969));
#22593=CARTESIAN_POINT('Ctrl Pts',(4.04665726739587,5.4265405004514,54.5987145507655));
#22594=CARTESIAN_POINT('Ctrl Pts',(3.9053465066936,5.52909937007814,54.6069266330341));
#22595=CARTESIAN_POINT('Ctrl Pts',(3.76043261936165,5.6259608526225,54.6151387153027));
#22596=CARTESIAN_POINT('Ctrl Pts',(3.61533942837926,5.72294218301393,54.6233609584769));
#22597=CARTESIAN_POINT('Ctrl Pts',(3.46663451090963,5.81421185833465,54.6315832016511));
#22598=CARTESIAN_POINT('Ctrl Pts',(3.31481654211206,5.89951525908191,54.6398054448253));
#22599=CARTESIAN_POINT('Ctrl Pts',(3.24360327303733,5.93952853339006,54.6436622532137));
#22600=CARTESIAN_POINT('Ctrl Pts',(3.17170535883719,5.97822974792016,54.647519061602));
#22601=CARTESIAN_POINT('Ctrl Pts',(3.09917575053251,6.01559628526643,54.6513758699904));
#22602=CARTESIAN_POINT('Origin',(0.,0.,-3.69717978381041));
#22603=CARTESIAN_POINT('',(3.09917575053258,6.01559628526639,57.0458946091258));
#22604=CARTESIAN_POINT('',(3.09917575053263,6.01559628526637,56.6515777772535));
#22605=CARTESIAN_POINT('',(3.09917575053259,6.01559628526639,-3.69717978381041));
#22606=CARTESIAN_POINT('',(-6.76699940565952,0.00283616003333658,55.6971797838559));
#22607=CARTESIAN_POINT('Ctrl Pts',(-6.76699940565952,0.00283616003323741,
55.6971797838558));
#22608=CARTESIAN_POINT('Ctrl Pts',(-6.76707134889961,-0.168818421231435,
55.7052944011409));
#22609=CARTESIAN_POINT('Ctrl Pts',(-6.76060770170997,-0.340730811922388,
55.7134090184261));
#22610=CARTESIAN_POINT('Ctrl Pts',(-6.74757589657687,-0.512355852835504,
55.7215236357112));
#22611=CARTESIAN_POINT('Ctrl Pts',(-6.7345577476259,-0.683801045846384,
55.7296297495932));
#22612=CARTESIAN_POINT('Ctrl Pts',(-6.71498516853079,-0.854959123553571,
55.7377358634753));
#22613=CARTESIAN_POINT('Ctrl Pts',(-6.68887757730892,-1.02528325636085,
55.7458419773573));
#22614=CARTESIAN_POINT('Ctrl Pts',(-6.66279174601455,-1.19546542889505,
55.7539413350262));
#22615=CARTESIAN_POINT('Ctrl Pts',(-6.63018180148919,-1.36481467740047,
55.7620406926952));
#22616=CARTESIAN_POINT('Ctrl Pts',(-6.59111909538432,-1.53278767951083,
55.7701400503641));
#22617=CARTESIAN_POINT('Ctrl Pts',(-6.5520805758803,-1.70065667715348,55.7782343931237));
#22618=CARTESIAN_POINT('Ctrl Pts',(-6.50659733355476,-1.86715076671615,
55.7863287358832));
#22619=CARTESIAN_POINT('Ctrl Pts',(-6.45479207658211,-2.03173528002365,
55.7944230786428));
#22620=CARTESIAN_POINT('Ctrl Pts',(-6.40300243503939,-2.19627018334781,
55.8025149815603));
#22621=CARTESIAN_POINT('Ctrl Pts',(-6.34489467906279,-2.35889630336945,
55.8106068844779));
#22622=CARTESIAN_POINT('Ctrl Pts',(-6.28064183324126,-2.51909252758604,
55.8186987873954));
#22623=CARTESIAN_POINT('Ctrl Pts',(-6.21639767769422,-2.67926708507111,
55.8267895958734));
#22624=CARTESIAN_POINT('Ctrl Pts',(-6.14601022330997,-2.83701205795902,
55.8348804043514));
#22625=CARTESIAN_POINT('Ctrl Pts',(-6.06970120868306,-2.9918249008442,55.8429712128293));
#22626=CARTESIAN_POINT('Ctrl Pts',(-5.99338771118787,-3.14664683840301,
55.851062496612));
#22627=CARTESIAN_POINT('Ctrl Pts',(-5.91115212404481,-3.2985359716822,55.8591537803946));
#22628=CARTESIAN_POINT('Ctrl Pts',(-5.82326280444565,-3.44701309982422,
55.8672450641772));
#22629=CARTESIAN_POINT('Ctrl Pts',(-5.7353512698158,-3.59552775725847,55.8753383931243));
#22630=CARTESIAN_POINT('Ctrl Pts',(-5.64178334607896,-3.74062837509862,
55.8834317220714));
#22631=CARTESIAN_POINT('Ctrl Pts',(-5.54287143362222,-3.88186363366036,
55.8915250510186));
#22632=CARTESIAN_POINT('Ctrl Pts',(-5.44386021068177,-4.02324069659627,
55.8996265059072));
#22633=CARTESIAN_POINT('Ctrl Pts',(-5.3394944940311,-4.16074434571123,55.9077279607958));
#22634=CARTESIAN_POINT('Ctrl Pts',(-5.2301283013377,-4.2939546983575,55.9158294156844));
#22635=CARTESIAN_POINT('Ctrl Pts',(-5.12070475684185,-4.42723490672098,
55.9239351189886));
#22636=CARTESIAN_POINT('Ctrl Pts',(-5.00627575655876,-4.55621705729177,
55.9320408222929));
#22637=CARTESIAN_POINT('Ctrl Pts',(-4.88723282960504,-4.68051752151733,
55.9401465255971));
#22638=CARTESIAN_POINT('Ctrl Pts',(-4.76801861168757,-4.80499684178127,
55.9482638922043));
#22639=CARTESIAN_POINT('Ctrl Pts',(-4.64417746908534,-4.92478076149952,
55.9563812588116));
#22640=CARTESIAN_POINT('Ctrl Pts',(-4.51613550604893,-5.03952468899639,
55.9644986254188));
#22641=CARTESIAN_POINT('Ctrl Pts',(-4.40986072031907,-5.1347621097556,55.9712360369394));
#22642=CARTESIAN_POINT('Ctrl Pts',(-4.30069266936053,-5.22652816319539,
55.9779734484599));
#22643=CARTESIAN_POINT('Ctrl Pts',(-4.18888991287168,-5.31464865234212,
55.9847108599805));
#22644=CARTESIAN_POINT('Ctrl Pts',(-4.05240415550037,-5.42222374332229,
55.9929357083025));
#22645=CARTESIAN_POINT('Ctrl Pts',(-3.91158021645315,-5.52468878958651,
56.0011605566246));
#22646=CARTESIAN_POINT('Ctrl Pts',(-3.76683671702674,-5.62167503038545,
56.0093854049466));
#22647=CARTESIAN_POINT('Ctrl Pts',(-3.62225623087324,-5.71855204317344,
56.0176009902658));
#22648=CARTESIAN_POINT('Ctrl Pts',(-3.4737652696585,-5.80996233934751,56.025816575585));
#22649=CARTESIAN_POINT('Ctrl Pts',(-3.32181576814251,-5.89557707120514,
56.0340321609042));
#22650=CARTESIAN_POINT('Ctrl Pts',(-3.17000686577554,-5.98111258359629,
56.0422401443274));
#22651=CARTESIAN_POINT('Ctrl Pts',(-3.01474610696026,-6.06086303648539,
56.0504481277507));
#22652=CARTESIAN_POINT('Ctrl Pts',(-2.85651474687221,-6.13454256655715,
56.0586561111739));
#22653=CARTESIAN_POINT('Ctrl Pts',(-2.69839801697386,-6.20816871973508,
56.0668581483504));
#22654=CARTESIAN_POINT('Ctrl Pts',(-2.53731529618713,-6.27573255936942,
56.075060185527));
#22655=CARTESIAN_POINT('Ctrl Pts',(-2.37377288303919,-6.33699386931594,
56.0832622227036));
#22656=CARTESIAN_POINT('Ctrl Pts',(-2.21031610689051,-6.39822310052121,
56.0914599649829));
#22657=CARTESIAN_POINT('Ctrl Pts',(-2.04440253943738,-6.45315625109748,
56.0996577072623));
#22658=CARTESIAN_POINT('Ctrl Pts',(-1.87655900350602,-6.5016009802479,56.1078554495417));
#22659=CARTESIAN_POINT('Ctrl Pts',(-1.70874738024495,-6.55003649843492,
56.116051633156));
#22660=CARTESIAN_POINT('Ctrl Pts',(-1.53900686205038,-6.59198594712425,
56.1242478167704));
#22661=CARTESIAN_POINT('Ctrl Pts',(-1.36788029639942,-6.6273065792011,56.1324440003847));
#22662=CARTESIAN_POINT('Ctrl Pts',(-1.1967663280512,-6.66262461118665,56.1406395806456));
#22663=CARTESIAN_POINT('Ctrl Pts',(-1.02426686668324,-6.6913147249621,56.1488351609065));
#22664=CARTESIAN_POINT('Ctrl Pts',(-0.850935785196513,-6.71328513393197,
56.1570307411674));
#22665=CARTESIAN_POINT('Ctrl Pts',(-0.677585927756354,-6.73525792282916,
56.1652272092081));
#22666=CARTESIAN_POINT('Ctrl Pts',(-0.503404626776022,-6.75050951157719,
56.1734236772488));
#22667=CARTESIAN_POINT('Ctrl Pts',(-0.328951775392259,-6.75899990601171,
56.1816201452895));
#22668=CARTESIAN_POINT('Ctrl Pts',(-0.154448286773356,-6.76749276489491,
56.1898189924629));
#22669=CARTESIAN_POINT('Ctrl Pts',(0.0203265509343518,-6.76922050292508,
56.1980178396363));
#22670=CARTESIAN_POINT('Ctrl Pts',(0.194811887535325,-6.76419524618228,
56.2062166868096));
#22671=CARTESIAN_POINT('Ctrl Pts',(0.369479578280686,-6.75916473755751,
56.2144241025756));
#22672=CARTESIAN_POINT('Ctrl Pts',(0.543856804288456,-6.7473671444689,56.2226315183416));
#22673=CARTESIAN_POINT('Ctrl Pts',(0.717385873467032,-6.72886665855031,
56.2308389341075));
#22674=CARTESIAN_POINT('Ctrl Pts',(0.891007948123133,-6.71035625702198,
56.2390507487596));
#22675=CARTESIAN_POINT('Ctrl Pts',(1.06378060499883,-6.68513585267878,56.2472625634118));
#22676=CARTESIAN_POINT('Ctrl Pts',(1.23515550778358,-6.6533209656225,56.2554743780639));
#22677=CARTESIAN_POINT('Ctrl Pts',(1.40678278616593,-6.62145922630837,56.2636982858615));
#22678=CARTESIAN_POINT('Ctrl Pts',(1.57700784678693,-6.58298367547638,56.2719221936591));
#22679=CARTESIAN_POINT('Ctrl Pts',(1.745295437402,-6.53806032674705,56.2801461014567));
#22680=CARTESIAN_POINT('Ctrl Pts',(1.90079006314705,-6.49655198217838,56.2877448403802));
#22681=CARTESIAN_POINT('Ctrl Pts',(2.05463055554878,-6.44953950084289,56.2953435793037));
#22682=CARTESIAN_POINT('Ctrl Pts',(2.20641016366796,-6.39719025742261,56.3029423182272));
#22683=CARTESIAN_POINT('Ctrl Pts',(2.36922045267152,-6.34103649898305,56.3110933004015));
#22684=CARTESIAN_POINT('Ctrl Pts',(2.53014140601998,-6.27857511840655,56.3192442825758));
#22685=CARTESIAN_POINT('Ctrl Pts',(2.68864296595399,-6.20995072457311,56.3273952647501));
#22686=CARTESIAN_POINT('Ctrl Pts',(2.84696041163582,-6.1414060443334,56.3355367788031));
#22687=CARTESIAN_POINT('Ctrl Pts',(3.00286372596184,-6.06671274500468,56.3436782928561));
#22688=CARTESIAN_POINT('Ctrl Pts',(3.15583778969361,-5.98606522225926,56.3518198069092));
#22689=CARTESIAN_POINT('Ctrl Pts',(3.30866635122605,-5.90549440788939,56.3599535771122));
#22690=CARTESIAN_POINT('Ctrl Pts',(3.45857088775684,-5.81898081446106,56.3680873473153));
#22691=CARTESIAN_POINT('Ctrl Pts',(3.60505606954399,-5.72676695312845,56.3762211175183));
#22692=CARTESIAN_POINT('Ctrl Pts',(3.75143272991933,-5.63462140709091,56.3843488619363));
#22693=CARTESIAN_POINT('Ctrl Pts',(3.89439477132242,-5.53678419572485,56.3924766063543));
#22694=CARTESIAN_POINT('Ctrl Pts',(4.03347131311705,-5.43354379445513,56.4006043507722));
#22695=CARTESIAN_POINT('Ctrl Pts',(4.17247406187973,-5.330358171814,56.4087277826663));
#22696=CARTESIAN_POINT('Ctrl Pts',(4.3075951238005,-5.22177528624459,56.4168512145604));
#22697=CARTESIAN_POINT('Ctrl Pts',(4.43839248785028,-5.10812696825306,56.4249746464545));
#22698=CARTESIAN_POINT('Ctrl Pts',(4.57001957893041,-4.99375771003405,56.4331496102053));
#22699=CARTESIAN_POINT('Ctrl Pts',(4.69726761262311,-4.87425873615773,56.4413245739561));
#22700=CARTESIAN_POINT('Ctrl Pts',(4.81971946900952,-4.75000981473203,56.449499537707));
#22701=CARTESIAN_POINT('Ctrl Pts',(4.94137183363872,-4.62657211815382,56.45762112688));
#22702=CARTESIAN_POINT('Ctrl Pts',(5.05829022241523,-4.49844659671581,56.465742716053));
#22703=CARTESIAN_POINT('Ctrl Pts',(5.17010247939526,-4.3660427566105,56.473864305226));
#22704=CARTESIAN_POINT('Ctrl Pts',(5.2819294978866,-4.23362143648254,56.4819869666154));
#22705=CARTESIAN_POINT('Ctrl Pts',(5.38864880570886,-4.09692095230147,56.4901096280048));
#22706=CARTESIAN_POINT('Ctrl Pts',(5.48992853191956,-3.95638391898657,56.4982322893941));
#22707=CARTESIAN_POINT('Ctrl Pts',(5.59124091578664,-3.81580156949327,56.5063575699364));
#22708=CARTESIAN_POINT('Ctrl Pts',(5.68711001143615,-3.67138050419232,56.5144828504786));
#22709=CARTESIAN_POINT('Ctrl Pts',(5.77724730308799,-3.52359228614244,56.5226081310208));
#22710=CARTESIAN_POINT('Ctrl Pts',(5.8683666218291,-3.37419394612263,56.5308219348086));
#22711=CARTESIAN_POINT('Ctrl Pts',(5.95362831122039,-3.22135498257339,56.5390357385963));
#22712=CARTESIAN_POINT('Ctrl Pts',(6.03278246772727,-3.06558717003488,56.5472495423841));
#22713=CARTESIAN_POINT('Ctrl Pts',(6.11121904553692,-2.91123148376901,56.5553888832393));
#22714=CARTESIAN_POINT('Ctrl Pts',(6.18365827760207,-2.7540001919264,56.5635282240944));
#22715=CARTESIAN_POINT('Ctrl Pts',(6.24990600766964,-2.59441012472874,56.5716675649496));
#22716=CARTESIAN_POINT('Ctrl Pts',(6.31706284088456,-2.43263003785449,56.5799186002037));
#22717=CARTESIAN_POINT('Ctrl Pts',(6.377856874295,-2.26842633637579,56.5881696354577));
#22718=CARTESIAN_POINT('Ctrl Pts',(6.4321386101332,-2.10235151676254,56.5964206707118));
#22719=CARTESIAN_POINT('Ctrl Pts',(6.48642034597141,-1.9362766971493,56.6046717059658));
#22720=CARTESIAN_POINT('Ctrl Pts',(6.53418974372113,-1.76833114698214,56.6129227412199));
#22721=CARTESIAN_POINT('Ctrl Pts',(6.57535136644329,-1.59907579801969,56.621173776474));
#22722=CARTESIAN_POINT('Ctrl Pts',(6.61641689146346,-1.43021559990437,56.6294055485048));
#22723=CARTESIAN_POINT('Ctrl Pts',(6.65103383186121,-1.25952460223781,56.6376373205357));
#22724=CARTESIAN_POINT('Ctrl Pts',(6.67903840006713,-1.08753622947872,56.6458690925665));
#22725=CARTESIAN_POINT('Ctrl Pts',(6.70700952802003,-0.915753228023974,
56.6540910350389));
#22726=CARTESIAN_POINT('Ctrl Pts',(6.72838394919001,-0.742676286453013,
56.6623129775113));
#22727=CARTESIAN_POINT('Ctrl Pts',(6.74304793715289,-0.568852808077908,
56.6705349199837));
#22728=CARTESIAN_POINT('Ctrl Pts',(6.75769735290761,-0.395202065244957,
56.6787486919736));
#22729=CARTESIAN_POINT('Ctrl Pts',(6.76564958570011,-0.220806617608481,
56.6869624639635));
#22730=CARTESIAN_POINT('Ctrl Pts',(6.76684213195596,-0.0462229508549047,
56.6951762359534));
#22731=CARTESIAN_POINT('Ctrl Pts',(6.76803373197987,0.12822219159306,56.7033834906838));
#22732=CARTESIAN_POINT('Ctrl Pts',(6.76247632597551,0.302854899009995,56.7115907454141));
#22733=CARTESIAN_POINT('Ctrl Pts',(6.75015930678691,0.477114591055564,56.7197980001445));
#22734=CARTESIAN_POINT('Ctrl Pts',(6.7378495943166,0.651270908537818,56.7280003861565));
#22735=CARTESIAN_POINT('Ctrl Pts',(6.71878828214661,0.82505429500201,56.7362027721684));
#22736=CARTESIAN_POINT('Ctrl Pts',(6.69301683849192,0.997905105540422,56.7444051581804));
#22737=CARTESIAN_POINT('Ctrl Pts',(6.66725308698803,1.17070432430472,56.7526050959791));
#22738=CARTESIAN_POINT('Ctrl Pts',(6.63478324245407,1.34257116708588,56.7608050337778));
#22739=CARTESIAN_POINT('Ctrl Pts',(6.59570056008811,1.51295179092179,56.7690049715765));
#22740=CARTESIAN_POINT('Ctrl Pts',(6.55662334248996,1.68330859114856,56.7772037628122));
#22741=CARTESIAN_POINT('Ctrl Pts',(6.51093520792635,1.85217923690409,56.785402554048));
#22742=CARTESIAN_POINT('Ctrl Pts',(6.45878040288734,2.01902072977927,56.7936013452837));
#22743=CARTESIAN_POINT('Ctrl Pts',(6.40662342928366,2.185869159821,56.8018004774201));
#22744=CARTESIAN_POINT('Ctrl Pts',(6.34799935640286,2.35068792675093,56.8099996095566));
#22745=CARTESIAN_POINT('Ctrl Pts',(6.28310213308798,2.51294977768862,56.818198741693));
#22746=CARTESIAN_POINT('Ctrl Pts',(6.21819043873685,2.67524781040739,56.8263997021039));
#22747=CARTESIAN_POINT('Ctrl Pts',(6.14700294099896,2.83498745882719,56.8346006625148));
#22748=CARTESIAN_POINT('Ctrl Pts',(6.06978151960589,2.99166196356654,56.8428016229257));
#22749=CARTESIAN_POINT('Ctrl Pts',(5.99248772315154,3.14848331003294,56.8510102696108));
#22750=CARTESIAN_POINT('Ctrl Pts',(5.9091488628883,3.30223345126376,56.8592189162958));
#22751=CARTESIAN_POINT('Ctrl Pts',(5.82005298481939,3.45242990571784,56.8674275629809));
#22752=CARTESIAN_POINT('Ctrl Pts',(5.73091456987614,3.60269806817737,56.8756401287044));
#22753=CARTESIAN_POINT('Ctrl Pts',(5.63601385153254,3.74940886027348,56.8838526944278));
#22754=CARTESIAN_POINT('Ctrl Pts',(5.53568187272827,3.89210935148895,56.8920652601513));
#22755=CARTESIAN_POINT('Ctrl Pts',(5.43521222397096,4.03500564837034,56.9002890947001));
#22756=CARTESIAN_POINT('Ctrl Pts',(5.3292966380478,4.17388036182298,56.9085129292489));
#22757=CARTESIAN_POINT('Ctrl Pts',(5.21830683100648,4.30831322183881,56.9167367637976));
#22758=CARTESIAN_POINT('Ctrl Pts',(5.11632807649764,4.43183173218608,56.9242929207721));
#22759=CARTESIAN_POINT('Ctrl Pts',(5.01006618032121,4.55160060682997,56.9318490777466));
#22760=CARTESIAN_POINT('Ctrl Pts',(4.89983590488299,4.66732226284189,56.939405234721));
#22761=CARTESIAN_POINT('Ctrl Pts',(4.77037908012015,4.80322828397848,56.9482793492547));
#22762=CARTESIAN_POINT('Ctrl Pts',(4.63514552804324,4.9338696802297,56.9571534637885));
#22763=CARTESIAN_POINT('Ctrl Pts',(4.494581686238,5.0587572056518,56.9660275783222));
#22764=CARTESIAN_POINT('Ctrl Pts',(4.35783563105977,5.18025272130586,56.9746606673165));
#22765=CARTESIAN_POINT('Ctrl Pts',(4.21604527949635,5.29630258905356,56.9832937563108));
#22766=CARTESIAN_POINT('Ctrl Pts',(4.0696609981487,5.40649131693998,56.9919268453051));
#22767=CARTESIAN_POINT('Ctrl Pts',(3.91714640520632,5.52129455145204,57.0009214726086));
#22768=CARTESIAN_POINT('Ctrl Pts',(3.75964502175002,5.62973490596909,57.009916099912));
#22769=CARTESIAN_POINT('Ctrl Pts',(3.59770745665002,5.73138639915028,57.0189107272154));
#22770=CARTESIAN_POINT('Ctrl Pts',(3.43576989154996,5.83303789233151,57.0279053545189));
#22771=CARTESIAN_POINT('Ctrl Pts',(3.26939643015181,5.92790027351654,57.0368999818223));
#22772=CARTESIAN_POINT('Ctrl Pts',(3.09917575053259,6.01559628526639,57.0458946091257));
#22773=CARTESIAN_POINT('Ctrl Pts',(3.09917575053258,6.01559628526639,55.0458595242204));
#22774=CARTESIAN_POINT('Ctrl Pts',(2.94439360812047,6.09533851523518,55.0540784634639));
#22775=CARTESIAN_POINT('Ctrl Pts',(2.78634971423239,6.16919687680001,55.0622974027074));
#22776=CARTESIAN_POINT('Ctrl Pts',(2.62553110980132,6.23689629474993,55.0705163419508));
#22777=CARTESIAN_POINT('Ctrl Pts',(2.46486086366275,6.30453325866921,55.0787276990629));
#22778=CARTESIAN_POINT('Ctrl Pts',(2.30142133292268,6.36602245613136,55.0869390561749));
#22779=CARTESIAN_POINT('Ctrl Pts',(2.13572376068943,6.42113486994524,55.0951504132869));
#22780=CARTESIAN_POINT('Ctrl Pts',(1.97014586454737,6.47620747847909,55.1033558396958));
#22781=CARTESIAN_POINT('Ctrl Pts',(1.80231351396567,6.52491236430631,55.1115612661046));
#22782=CARTESIAN_POINT('Ctrl Pts',(1.63275760578661,6.5670687220971,55.1197666925134));
#22783=CARTESIAN_POINT('Ctrl Pts',(1.46329021233422,6.60920307264244,55.1279678353731));
#22784=CARTESIAN_POINT('Ctrl Pts',(1.29210140067427,6.64479561916022,55.1361689782327));
#22785=CARTESIAN_POINT('Ctrl Pts',(1.11973698256718,6.67371546365826,55.1443701210923));
#22786=CARTESIAN_POINT('Ctrl Pts',(0.941198440117324,6.7036712221684,55.1528650303588));
#22787=CARTESIAN_POINT('Ctrl Pts',(0.761398889731606,6.72646726241169,55.1613599396252));
#22788=CARTESIAN_POINT('Ctrl Pts',(0.580956816055468,6.74201588383465,55.1698548488916));
#22789=CARTESIAN_POINT('Ctrl Pts',(0.40679692454045,6.75702317212979,55.1780540035906));
#22790=CARTESIAN_POINT('Ctrl Pts',(0.232038878029628,6.76527918081022,55.1862531582896));
#22791=CARTESIAN_POINT('Ctrl Pts',(0.0572440019946399,6.76675787391833,
55.1944523129886));
#22792=CARTESIAN_POINT('Ctrl Pts',(-0.117571233752477,6.76823673926126,
55.2026524227065));
#22793=CARTESIAN_POINT('Ctrl Pts',(-0.292422949038723,6.76293671292917,
55.2108525324245));
#22794=CARTESIAN_POINT('Ctrl Pts',(-0.466749923568456,6.75088390574515,
55.2190526421425));
#22795=CARTESIAN_POINT('Ctrl Pts',(-0.641128828132783,6.73882750816615,
55.2272551945804));
#22796=CARTESIAN_POINT('Ctrl Pts',(-0.814982323011746,6.72001434722957,
55.2354577470184));
#22797=CARTESIAN_POINT('Ctrl Pts',(-0.98775435508373,6.69452241269033,55.2436602994563));
#22798=CARTESIAN_POINT('Ctrl Pts',(-1.16060919733535,6.6690182597865,55.2518667834035));
#22799=CARTESIAN_POINT('Ctrl Pts',(-1.33238119003697,6.6368290086569,55.2600732673507));
#22800=CARTESIAN_POINT('Ctrl Pts',(-1.50252445657173,6.5980837564708,55.2682797512978));
#22801=CARTESIAN_POINT('Ctrl Pts',(-1.67286916646132,6.55929263133455,55.2764959514195));
#22802=CARTESIAN_POINT('Ctrl Pts',(-1.84158094989867,6.51393008400835,55.2847121515411));
#22803=CARTESIAN_POINT('Ctrl Pts',(-2.00812818465421,6.46217534534598,55.2929283516627));
#22804=CARTESIAN_POINT('Ctrl Pts',(-2.17479235022103,6.41038427030379,55.3011503202797));
#22805=CARTESIAN_POINT('Ctrl Pts',(-2.33928860165323,6.35219217846584,55.3093722888966));
#22806=CARTESIAN_POINT('Ctrl Pts',(-2.5011054099358,6.28782639140028,55.3175942575136));
#22807=CARTESIAN_POINT('Ctrl Pts',(-2.66314387204506,6.22337243720819,55.325827488439));
#22808=CARTESIAN_POINT('Ctrl Pts',(-2.82249523650154,6.15272804690666,55.3340607193644));
#22809=CARTESIAN_POINT('Ctrl Pts',(-2.97867190289986,6.07616677642039,55.3422939502898));
#22810=CARTESIAN_POINT('Ctrl Pts',(-3.01631912457594,6.05771127222588,55.3442786146888));
#22811=CARTESIAN_POINT('Ctrl Pts',(-3.05378200236287,6.03891215075457,55.3462632790878));
#22812=CARTESIAN_POINT('Ctrl Pts',(-3.09105396253018,6.01977361706622,55.3482479434869));
#22813=CARTESIAN_POINT('Ctrl Pts',(-3.2441839043967,5.94114393035398,55.3564018356536));
#22814=CARTESIAN_POINT('Ctrl Pts',(-3.39456247297689,5.85653868877348,55.3645557278203));
#22815=CARTESIAN_POINT('Ctrl Pts',(-3.54168471217314,5.76617363591828,55.3727096199871));
#22816=CARTESIAN_POINT('Ctrl Pts',(-3.68862742113394,5.67591885367413,55.3808535621273));
#22817=CARTESIAN_POINT('Ctrl Pts',(-3.83232140220006,5.57991843998532,55.3889975042675));
#22818=CARTESIAN_POINT('Ctrl Pts',(-3.9722832661189,5.47843542023741,55.3971414464077));
#22819=CARTESIAN_POINT('Ctrl Pts',(-4.11210379664129,5.37705487797486,55.4052771648006));
#22820=CARTESIAN_POINT('Ctrl Pts',(-4.24819941893756,5.27020296442739,55.4134128831935));
#22821=CARTESIAN_POINT('Ctrl Pts',(-4.38011288995688,5.15818767313032,55.4215486015864));
#22822=CARTESIAN_POINT('Ctrl Pts',(-4.51192090287179,5.04626193235598,55.4296778158867));
#22823=CARTESIAN_POINT('Ctrl Pts',(-4.63955314418621,4.9291812683987,55.4378070301869));
#22824=CARTESIAN_POINT('Ctrl Pts',(-4.76258284177514,4.80729587972584,55.4459362444871));
#22825=CARTESIAN_POINT('Ctrl Pts',(-4.88554005190463,4.68548230430085,55.4540606691626));
#22826=CARTESIAN_POINT('Ctrl Pts',(-5.00389985955734,4.55886989843988,55.462185093838));
#22827=CARTESIAN_POINT('Ctrl Pts',(-5.11726998927648,4.42784788095191,55.4703095185134));
#22828=CARTESIAN_POINT('Ctrl Pts',(-5.23132834825853,4.29603047594216,55.4784832636476));
#22829=CARTESIAN_POINT('Ctrl Pts',(-5.34033596388518,4.15974998873474,55.4866570087817));
#22830=CARTESIAN_POINT('Ctrl Pts',(-5.4439319762056,4.01943946819033,55.4948307539159));
#22831=CARTESIAN_POINT('Ctrl Pts',(-5.54686458997772,3.88002745516137,55.5029521567781));
#22832=CARTESIAN_POINT('Ctrl Pts',(-5.64445450512135,3.7366371837638,55.5110735596402));
#22833=CARTESIAN_POINT('Ctrl Pts',(-5.73638923462593,3.58972527484593,55.5191949625024));
#22834=CARTESIAN_POINT('Ctrl Pts',(-5.82833107203969,3.44280200747288,55.5273169932686));
#22835=CARTESIAN_POINT('Ctrl Pts',(-5.91461665870489,3.29235687046016,55.5354390240349));
#22836=CARTESIAN_POINT('Ctrl Pts',(-5.99497791594782,3.13887380875657,55.5435610548012));
#22837=CARTESIAN_POINT('Ctrl Pts',(-6.07536068893902,2.98534965383178,55.5516852601423));
#22838=CARTESIAN_POINT('Ctrl Pts',(-6.14981580447394,2.82878627875354,55.5598094654834));
#22839=CARTESIAN_POINT('Ctrl Pts',(-6.2181220707769,2.66969041518249,55.5679336708245));
#22840=CARTESIAN_POINT('Ctrl Pts',(-6.28716770514826,2.50887244897422,55.5761458150669));
#22841=CARTESIAN_POINT('Ctrl Pts',(-6.3499304463994,2.34546720131573,55.5843579593094));
#22842=CARTESIAN_POINT('Ctrl Pts',(-6.40623284922578,2.18001598193695,55.5925701035518));
#22843=CARTESIAN_POINT('Ctrl Pts',(-6.46202127316779,2.01607514983982,55.6007072799682));
#22844=CARTESIAN_POINT('Ctrl Pts',(-6.51146677541545,1.85012591390681,55.6088444563847));
#22845=CARTESIAN_POINT('Ctrl Pts',(-6.55444781601728,1.68270699383651,55.6169816328011));
#22846=CARTESIAN_POINT('Ctrl Pts',(-6.59802283326526,1.51297442739444,55.6252312609565));
#22847=CARTESIAN_POINT('Ctrl Pts',(-6.63495332642006,1.34173164236327,55.6334808891119));
#22848=CARTESIAN_POINT('Ctrl Pts',(-6.66516684415941,1.16954689496323,55.6417305172673));
#22849=CARTESIAN_POINT('Ctrl Pts',(-6.69538036189876,0.9973621475632,55.6499801454227));
#22850=CARTESIAN_POINT('Ctrl Pts',(-6.71887691516152,0.824235827583319,
55.6582297735781));
#22851=CARTESIAN_POINT('Ctrl Pts',(-6.73563879448179,0.650737297434142,
55.6664794017335));
#22852=CARTESIAN_POINT('Ctrl Pts',(-6.7564314932459,0.435516640819393,55.6767128624256));
#22853=CARTESIAN_POINT('Ctrl Pts',(-6.76690867697218,0.219312224909553,
55.6869463231178));
#22854=CARTESIAN_POINT('Ctrl Pts',(-6.76699940565911,0.00283616100313801,
55.69717978381));
#22855=CARTESIAN_POINT('',(-6.76699999332355,-0.000300597867382727,55.3028202161605));
#22856=CARTESIAN_POINT('Ctrl Pts',(3.09917575053251,6.01559628526643,54.6513758699904));
#22857=CARTESIAN_POINT('Ctrl Pts',(3.03170056831351,6.05035883224919,54.6549639060335));
#22858=CARTESIAN_POINT('Ctrl Pts',(2.96367868074345,6.08396626315161,54.6585519420766));
#22859=CARTESIAN_POINT('Ctrl Pts',(2.8951533392384,6.11640222208258,54.6621399781197));
#22860=CARTESIAN_POINT('Ctrl Pts',(2.73945348228504,6.19010158723388,54.6702925343329));
#22861=CARTESIAN_POINT('Ctrl Pts',(2.58069410409827,6.25796707530155,54.6784450905462));
#22862=CARTESIAN_POINT('Ctrl Pts',(2.41935558589252,6.31973160419101,54.6865976467594));
#22863=CARTESIAN_POINT('Ctrl Pts',(2.25820398224972,6.38142457738471,54.6947407580398));
#22864=CARTESIAN_POINT('Ctrl Pts',(2.09447952438987,6.43703053178444,54.7028838693201));
#22865=CARTESIAN_POINT('Ctrl Pts',(1.92868669728718,6.48632843939524,54.7110269806005));
#22866=CARTESIAN_POINT('Ctrl Pts',(1.76305108929455,6.5355795984627,54.7191623698778));
#22867=CARTESIAN_POINT('Ctrl Pts',(1.5953513649588,6.57853451633816,54.7272977591551));
#22868=CARTESIAN_POINT('Ctrl Pts',(1.42611147686499,6.61502041233086,54.7354331484325));
#22869=CARTESIAN_POINT('Ctrl Pts',(1.25699651529884,6.65147937580579,54.7435625324711));
#22870=CARTESIAN_POINT('Ctrl Pts',(1.08634400956924,6.68147874892201,54.7516919165097));
#22871=CARTESIAN_POINT('Ctrl Pts',(0.914692545464687,6.7048957148692,54.7598213005483));
#22872=CARTESIAN_POINT('Ctrl Pts',(0.743131733005261,6.72830031397467,54.7679463913404));
#22873=CARTESIAN_POINT('Ctrl Pts',(0.570573374236173,6.74512937973692,54.7760714821325));
#22874=CARTESIAN_POINT('Ctrl Pts',(0.397565704887895,6.75531128152486,54.7841965729247));
#22875=CARTESIAN_POINT('Ctrl Pts',(0.22389762775997,6.76553204983922,54.7923526789498));
#22876=CARTESIAN_POINT('Ctrl Pts',(0.049777168539924,6.76905473590006,54.8005087849749));
#22877=CARTESIAN_POINT('Ctrl Pts',(-0.124235975849758,6.76585947402876,
54.808664891));
#22878=CARTESIAN_POINT('Ctrl Pts',(-0.297548748803826,6.76267707250862,
54.8167881701735));
#22879=CARTESIAN_POINT('Ctrl Pts',(-0.470754701295699,6.75283072801071,
54.8249114493468));
#22880=CARTESIAN_POINT('Ctrl Pts',(-0.643301263867664,6.7363530551706,54.8330347285203));
#22881=CARTESIAN_POINT('Ctrl Pts',(-0.815870802472411,6.71987318818912,
54.8411590893769));
#22882=CARTESIAN_POINT('Ctrl Pts',(-0.987780412063691,6.69676026883925,
54.8492834502336));
#22883=CARTESIAN_POINT('Ctrl Pts',(-1.15848317996609,6.66709874846141,54.8574078110903));
#22884=CARTESIAN_POINT('Ctrl Pts',(-1.32924115546454,6.63742763514459,54.8655347994757));
#22885=CARTESIAN_POINT('Ctrl Pts',(-1.49879115180774,6.60120376597276,54.8736617878611));
#22886=CARTESIAN_POINT('Ctrl Pts',(-1.66659701485307,6.5585626009121,54.8817887762466));
#22887=CARTESIAN_POINT('Ctrl Pts',(-1.83548772369796,6.5156457655741,54.8899683046866));
#22888=CARTESIAN_POINT('Ctrl Pts',(-2.00261130556678,6.46622846506356,54.8981478331267));
#22889=CARTESIAN_POINT('Ctrl Pts',(-2.16743807252027,6.41049929426637,54.9063273615668));
#22890=CARTESIAN_POINT('Ctrl Pts',(-2.33148861709045,6.35503257010073,54.9144683699705));
#22891=CARTESIAN_POINT('Ctrl Pts',(-2.49326361463911,6.29331348729231,54.9226093783741));
#22892=CARTESIAN_POINT('Ctrl Pts',(-2.65226262308908,6.22557563428191,54.9307503867778));
#22893=CARTESIAN_POINT('Ctrl Pts',(-2.81239011230343,6.15735701812156,54.9389491752361));
#22894=CARTESIAN_POINT('Ctrl Pts',(-2.96970172158162,6.08303404365845,54.9471479636944));
#22895=CARTESIAN_POINT('Ctrl Pts',(-3.12371347702433,6.00289122952071,54.9553467521526));
#22896=CARTESIAN_POINT('Ctrl Pts',(-3.27772523246704,5.92274841538296,54.9635455406109));
#22897=CARTESIAN_POINT('Ctrl Pts',(-3.42843684358858,5.83678600183742,54.9717443290691));
#22898=CARTESIAN_POINT('Ctrl Pts',(-3.5753961880223,5.74533124359907,54.9799431175274));
#22899=CARTESIAN_POINT('Ctrl Pts',(-3.72296965649872,5.6534943077859,54.9881761676594));
#22900=CARTESIAN_POINT('Ctrl Pts',(-3.86721823322404,5.55583365106446,54.9964092177914));
#22901=CARTESIAN_POINT('Ctrl Pts',(-4.00765146065182,5.45261577318037,55.0046422679234));
#22902=CARTESIAN_POINT('Ctrl Pts',(-4.14791745369263,5.34952081192255,55.0128655137583));
#22903=CARTESIAN_POINT('Ctrl Pts',(-4.28437685887732,5.24088201721773,55.0210887595931));
#22904=CARTESIAN_POINT('Ctrl Pts',(-4.41656519971276,5.12701090662837,55.029312005428));
#22905=CARTESIAN_POINT('Ctrl Pts',(-4.54862258233521,5.01325260747955,55.0375271045415));
#22906=CARTESIAN_POINT('Ctrl Pts',(-4.67641705782021,4.89427254786337,55.045742203655));
#22907=CARTESIAN_POINT('Ctrl Pts',(-4.79951438540531,4.77042457903775,55.0539573027685));
#22908=CARTESIAN_POINT('Ctrl Pts',(-4.9225143904864,4.64667452618382,55.0621659069074));
#22909=CARTESIAN_POINT('Ctrl Pts',(-5.04082439311391,4.51806448273646,55.0703745110463));
#22910=CARTESIAN_POINT('Ctrl Pts',(-5.15404435826846,4.38498754308391,55.0785831151852));
#22911=CARTESIAN_POINT('Ctrl Pts',(-5.26719745725208,4.25198919686126,55.0867868714341));
#22912=CARTESIAN_POINT('Ctrl Pts',(-5.37526627585814,4.11452948193927,55.0949906276831));
#22913=CARTESIAN_POINT('Ctrl Pts',(-5.47788863137583,3.97303726917373,55.1031943839321));
#22914=CARTESIAN_POINT('Ctrl Pts',(-5.58048062352503,3.83158692038776,55.1113957128964));
#22915=CARTESIAN_POINT('Ctrl Pts',(-5.67762914942449,3.68610673771275,55.1195970418606));
#22916=CARTESIAN_POINT('Ctrl Pts',(-5.76901307699329,3.53705769213345,55.1277983708249));
#22917=CARTESIAN_POINT('Ctrl Pts',(-5.86038440184607,3.38802920184045,55.1359985687476));
#22918=CARTESIAN_POINT('Ctrl Pts',(-5.94599252382731,3.23543313381405,55.1441987666703));
#22919=CARTESIAN_POINT('Ctrl Pts',(-6.02556032163339,3.07975840129666,55.152398964593));
#22920=CARTESIAN_POINT('Ctrl Pts',(-6.1051315655844,2.92407692638214,55.1605995176729));
#22921=CARTESIAN_POINT('Ctrl Pts',(-6.17866180104383,2.7653168403509,55.1688000707527));
#22922=CARTESIAN_POINT('Ctrl Pts',(-6.24592042595145,2.6039905976563,55.1770006238325));
#22923=CARTESIAN_POINT('Ctrl Pts',(-6.31319415246435,2.44262813231754,55.1852030181858));
#22924=CARTESIAN_POINT('Ctrl Pts',(-6.3741933259118,2.27869869335459,55.193405412539));
#22925=CARTESIAN_POINT('Ctrl Pts',(-6.42873592055473,2.11273364714281,55.2016078068922));
#22926=CARTESIAN_POINT('Ctrl Pts',(-6.4833295221116,1.9466133944381,55.209817871926));
#22927=CARTESIAN_POINT('Ctrl Pts',(-6.53145436936603,1.77845407196468,55.2180279369598));
#22928=CARTESIAN_POINT('Ctrl Pts',(-6.57297840188812,1.60880201650555,55.2262380019937));
#22929=CARTESIAN_POINT('Ctrl Pts',(-6.61452230707553,1.43906876858232,55.234451996219));
#22930=CARTESIAN_POINT('Ctrl Pts',(-6.64945902734759,1.26784171414278,55.2426659904443));
#22931=CARTESIAN_POINT('Ctrl Pts',(-6.67770789282387,1.09567618305674,55.2508799846696));
#22932=CARTESIAN_POINT('Ctrl Pts',(-6.70599527091237,0.923275933010371,
55.2591051773048));
#22933=CARTESIAN_POINT('Ctrl Pts',(-6.727576527936,0.749935004945466,55.26733036994));
#22934=CARTESIAN_POINT('Ctrl Pts',(-6.74242290182665,0.576213860405586,
55.2755555625752));
#22935=CARTESIAN_POINT('Ctrl Pts',(-6.75577421406819,0.419986807201015,
55.2829524606951));
#22936=CARTESIAN_POINT('Ctrl Pts',(-6.76367947340974,0.263452476255881,
55.290349358815));
#22937=CARTESIAN_POINT('Ctrl Pts',(-6.76615373703693,0.107016852790295,
55.2977462569349));
#22938=CARTESIAN_POINT('Ctrl Pts',(-6.76671948376637,0.0712474459374166,
55.2994375766768));
#22939=CARTESIAN_POINT('Ctrl Pts',(-6.76700158246802,0.0354739095168925,
55.3011288964187));
#22940=CARTESIAN_POINT('Ctrl Pts',(-6.76699999332355,-0.000300597867481069,
55.3028202161605));
#22941=CARTESIAN_POINT('Ctrl Pts',(-6.76699999332352,-0.000300598487863234,
55.3028202161898));
#22942=CARTESIAN_POINT('Ctrl Pts',(-6.7669919378939,-0.181642469414841,
55.3113935581795));
#22943=CARTESIAN_POINT('Ctrl Pts',(-6.75969016719996,-0.363162940377724,
55.3199669001692));
#22944=CARTESIAN_POINT('Ctrl Pts',(-6.74507751209151,-0.544259456396834,
55.3285402421589));
#22945=CARTESIAN_POINT('Ctrl Pts',(-6.73048339037461,-0.725126285708546,
55.3371027104845));
#22946=CARTESIAN_POINT('Ctrl Pts',(-6.70859689518945,-0.905569919651554,
55.34566517881));
#22947=CARTESIAN_POINT('Ctrl Pts',(-6.67945284379024,-1.08498788361092,
55.3542276471356));
#22948=CARTESIAN_POINT('Ctrl Pts',(-6.65035580230743,-1.26411644293771,
55.3627763040348));
#22949=CARTESIAN_POINT('Ctrl Pts',(-6.61402461003255,-1.44222232324766,
55.3713249609339));
#22950=CARTESIAN_POINT('Ctrl Pts',(-6.57054578095658,-1.61870847911341,
55.3798736178331));
#22951=CARTESIAN_POINT('Ctrl Pts',(-6.52710837203152,-1.79502650526263,
55.3884141308456));
#22952=CARTESIAN_POINT('Ctrl Pts',(-6.47653697394261,-1.96972757813517,
55.396954643858));
#22953=CARTESIAN_POINT('Ctrl Pts',(-6.4189693188722,-2.14222358389066,55.4054951568705));
#22954=CARTESIAN_POINT('Ctrl Pts',(-6.36146978187363,-2.31451548031953,
55.4140255641512));
#22955=CARTESIAN_POINT('Ctrl Pts',(-6.29699060257995,-2.48460721701655,
55.4225559714319));
#22956=CARTESIAN_POINT('Ctrl Pts',(-6.22571961560228,-2.65192463465782,
55.4310863787127));
#22957=CARTESIAN_POINT('Ctrl Pts',(-6.15453154832205,-2.81904738809932,
55.4396068613548));
#22958=CARTESIAN_POINT('Ctrl Pts',(-6.07656756443147,-2.98340197460336,
55.4481273439968));
#22959=CARTESIAN_POINT('Ctrl Pts',(-5.99206411720368,-3.14443263806367,
55.4566478266389));
#22960=CARTESIAN_POINT('Ctrl Pts',(-5.90681411731338,-3.30688594017953,
55.4652435841865));
#22961=CARTESIAN_POINT('Ctrl Pts',(-5.81500381503648,-3.46577502039305,
55.4738393417341));
#22962=CARTESIAN_POINT('Ctrl Pts',(-5.71696406270463,-3.62058157009945,
55.4824350992816));
#22963=CARTESIAN_POINT('Ctrl Pts',(-5.61883283595042,-3.77553255958026,
55.4910388769632));
#22964=CARTESIAN_POINT('Ctrl Pts',(-5.51446072094989,-3.92639315744197,
55.4996426546449));
#22965=CARTESIAN_POINT('Ctrl Pts',(-5.40422100295438,-4.07267533093748,
55.5082464323265));
#22966=CARTESIAN_POINT('Ctrl Pts',(-5.28964876764329,-4.22470652176681,
55.5171883459945));
#22967=CARTESIAN_POINT('Ctrl Pts',(-5.16873863590604,-4.37179184566761,
55.5261302596625));
#22968=CARTESIAN_POINT('Ctrl Pts',(-5.04195356579148,-4.51342367171558,
55.5350721733305));
#22969=CARTESIAN_POINT('Ctrl Pts',(-4.9196307059426,-4.65007075478422,55.5436993756612));
#22970=CARTESIAN_POINT('Ctrl Pts',(-4.79183963920985,-4.78164149138373,
55.5523265779919));
#22971=CARTESIAN_POINT('Ctrl Pts',(-4.65903206133329,-4.90771935337266,
55.5609537803227));
#22972=CARTESIAN_POINT('Ctrl Pts',(-4.52609800456668,-5.03391728522732,
55.5695891987431));
#22973=CARTESIAN_POINT('Ctrl Pts',(-4.38813812777909,-5.15461169769776,
55.5782246171636));
#22974=CARTESIAN_POINT('Ctrl Pts',(-4.24563705091085,-5.26942644240652,
55.586860035584));
#22975=CARTESIAN_POINT('Ctrl Pts',(-4.10292544899946,-5.38441080954632,
55.5955082116051));
#22976=CARTESIAN_POINT('Ctrl Pts',(-3.95565948263147,-5.49349796567173,
55.6041563876262));
#22977=CARTESIAN_POINT('Ctrl Pts',(-3.8043537739338,-5.59635429210443,55.6128045636474));
#22978=CARTESIAN_POINT('Ctrl Pts',(-3.78834620365939,-5.60723610144071,
55.6137195078791));
#22979=CARTESIAN_POINT('Ctrl Pts',(-3.77229344066174,-5.61804821207019,
55.6146344521109));
#22980=CARTESIAN_POINT('Ctrl Pts',(-3.75619611061305,-5.62879025889359,
55.6155493963426));
#22981=CARTESIAN_POINT('Ctrl Pts',(-3.61146978487512,-5.72536881962095,
55.6237753888839));
#22982=CARTESIAN_POINT('Ctrl Pts',(-3.4628263023278,-5.81648879399469,55.6320013814253));
#22983=CARTESIAN_POINT('Ctrl Pts',(-3.31071505867864,-5.90181792333841,
55.6402273739666));
#22984=CARTESIAN_POINT('Ctrl Pts',(-3.1587632840073,-5.98705759611923,55.6484447426181));
#22985=CARTESIAN_POINT('Ctrl Pts',(-3.00335129777346,-6.06651833953246,
55.6566621112695));
#22986=CARTESIAN_POINT('Ctrl Pts',(-2.84495823010512,-6.13991055870989,
55.6648794799209));
#22987=CARTESIAN_POINT('Ctrl Pts',(-2.68669952332861,-6.21324052109687,
55.6730898779833));
#22988=CARTESIAN_POINT('Ctrl Pts',(-2.52546509477776,-6.28051206195501,
55.6813002760457));
#22989=CARTESIAN_POINT('Ctrl Pts',(-2.36175956934444,-6.34148095767937,
55.6895106741081));
#22990=CARTESIAN_POINT('Ctrl Pts',(-2.19816016368635,-6.40241033118543,
55.6977157498968));
#22991=CARTESIAN_POINT('Ctrl Pts',(-2.03209318647946,-6.45704507317781,
55.7059208256856));
#22992=CARTESIAN_POINT('Ctrl Pts',(-1.86408427121,-6.50518860832086,55.7141259014744));
#22993=CARTESIAN_POINT('Ctrl Pts',(-1.69615066376803,-6.55331056374575,
55.7223272994439));
#22994=CARTESIAN_POINT('Ctrl Pts',(-1.52627719615885,-6.59494701060637,
55.7305286974133));
#22995=CARTESIAN_POINT('Ctrl Pts',(-1.35500582168781,-6.62995084621237,
55.7387300953828));
#22996=CARTESIAN_POINT('Ctrl Pts',(-1.1837478626166,-6.66495194002658,55.7469308509505));
#22997=CARTESIAN_POINT('Ctrl Pts',(-1.01109256379185,-6.69332137718182,
55.7551316065182));
#22998=CARTESIAN_POINT('Ctrl Pts',(-0.837593635799518,-6.71496283692383,
55.763332362086));
#22999=CARTESIAN_POINT('Ctrl Pts',(-0.66409558909929,-6.73660418673752,
55.7715330759977));
#23000=CARTESIAN_POINT('Ctrl Pts',(-0.489754277252908,-6.75151758179396,
55.7797337899095));
#23001=CARTESIAN_POINT('Ctrl Pts',(-0.315130006418644,-6.75965842917041,
55.7879345038213));
#23002=CARTESIAN_POINT('Ctrl Pts',(-0.140474976326381,-6.7678007105195,
55.7961366622509));
#23003=CARTESIAN_POINT('Ctrl Pts',(0.03446275406608,-6.76916805074496,55.8043388206805));
#23004=CARTESIAN_POINT('Ctrl Pts',(0.209121334914704,-6.76376797852229,
55.8125409791101));
#23005=CARTESIAN_POINT('Ctrl Pts',(0.383842333883037,-6.75836597646398,
55.8207460687631));
#23006=CARTESIAN_POINT('Ctrl Pts',(0.5582836266049,-6.7461917552627,55.828951158416));
#23007=CARTESIAN_POINT('Ctrl Pts',(0.731886885323504,-6.72730485314078,
55.8371562480689));
#23008=CARTESIAN_POINT('Ctrl Pts',(0.905688465239941,-6.7083963749662,55.8453707110667));
#23009=CARTESIAN_POINT('Ctrl Pts',(1.07864974189527,-6.68275993446701,55.8535851740645));
#23010=CARTESIAN_POINT('Ctrl Pts',(1.25021994594242,-6.65050667895069,55.8617996370623));
#23011=CARTESIAN_POINT('Ctrl Pts',(1.42189179991283,-6.61823431439988,55.8700189668697));
#23012=CARTESIAN_POINT('Ctrl Pts',(1.5921705896081,-6.57933739993316,55.8782382966772));
#23013=CARTESIAN_POINT('Ctrl Pts',(1.76051927672503,-6.53397741626642,55.8864576264847));
#23014=CARTESIAN_POINT('Ctrl Pts',(1.92912880992589,-6.4885471500551,55.8946896916454));
#23015=CARTESIAN_POINT('Ctrl Pts',(2.09580192228886,-6.43663390899524,55.9029217568061));
#23016=CARTESIAN_POINT('Ctrl Pts',(2.26001890768737,-6.37844836436696,55.9111538219667));
#23017=CARTESIAN_POINT('Ctrl Pts',(2.40762892559136,-6.32614701890327,55.918553393228));
#23018=CARTESIAN_POINT('Ctrl Pts',(2.55325456856072,-6.26877855995937,55.9259529644892));
#23019=CARTESIAN_POINT('Ctrl Pts',(2.69653527350191,-6.20652773447118,55.9333525357504));
#23020=CARTESIAN_POINT('Ctrl Pts',(2.85445250794638,-6.13791781098557,55.9415079941572));
#23021=CARTESIAN_POINT('Ctrl Pts',(3.01000707065127,-6.06316503924268,55.9496634525639));
#23022=CARTESIAN_POINT('Ctrl Pts',(3.16268103959137,-5.9824524771877,55.9578189109707));
#23023=CARTESIAN_POINT('Ctrl Pts',(3.31516918424258,-5.90183815293024,55.9659644431126));
#23024=CARTESIAN_POINT('Ctrl Pts',(3.46478339452723,-5.81527864642458,55.9741099752545));
#23025=CARTESIAN_POINT('Ctrl Pts',(3.61102424978326,-5.7230055798922,55.9822555073964));
#23026=CARTESIAN_POINT('Ctrl Pts',(3.75711786221345,-5.63082541863613,55.990392838197));
#23027=CARTESIAN_POINT('Ctrl Pts',(3.89984457457807,-5.53294334355425,55.9985301689975));
#23028=CARTESIAN_POINT('Ctrl Pts',(4.03872818351032,-5.42963752562908,56.0066674997981));
#23029=CARTESIAN_POINT('Ctrl Pts',(4.17750114409153,-5.32641401128526,56.0147983476001));
#23030=CARTESIAN_POINT('Ctrl Pts',(4.31243680575048,-5.21777557504684,56.0229291954021));
#23031=CARTESIAN_POINT('Ctrl Pts',(4.44308667312931,-5.10404445661093,56.0310600432041));
#23032=CARTESIAN_POINT('Ctrl Pts',(4.57365989723239,-4.99038005638641,56.0391861211979));
#23033=CARTESIAN_POINT('Ctrl Pts',(4.69995205900485,-4.87162916294331,56.0473121991917));
#23034=CARTESIAN_POINT('Ctrl Pts',(4.82154659059871,-4.74815516539698,56.0554382771855));
#23035=CARTESIAN_POINT('Ctrl Pts',(4.9435722741931,-4.62424335160712,56.0635931687677));
#23036=CARTESIAN_POINT('Ctrl Pts',(5.06086665791248,-4.49557510456205,56.0717480603499));
#23037=CARTESIAN_POINT('Ctrl Pts',(5.17304458199475,-4.36255644693508,56.0799029519321));
#23038=CARTESIAN_POINT('Ctrl Pts',(5.28478505139497,-4.23005651556423,56.0880260422884));
#23039=CARTESIAN_POINT('Ctrl Pts',(5.39144866997132,-4.09324033547733,56.0961491326447));
#23040=CARTESIAN_POINT('Ctrl Pts',(5.49269407084485,-3.95254359167686,56.104272223001));
#23041=CARTESIAN_POINT('Ctrl Pts',(5.59394742196961,-3.81183579972556,56.1123959512194));
#23042=CARTESIAN_POINT('Ctrl Pts',(5.68978149420295,-3.6672471340104,56.1205196794378));
#23043=CARTESIAN_POINT('Ctrl Pts',(5.77989747702832,-3.51924340662048,56.1286434076563));
#23044=CARTESIAN_POINT('Ctrl Pts',(5.87003768063073,-3.3711998997689,56.1367693193166));
#23045=CARTESIAN_POINT('Ctrl Pts',(5.95445654445746,-3.21973981590843,56.1448952309769));
#23046=CARTESIAN_POINT('Ctrl Pts',(6.03290057877024,-3.06535472770669,56.1530211426372));
#23047=CARTESIAN_POINT('Ctrl Pts',(6.11184627083669,-2.9099823308176,56.1611990203473));
#23048=CARTESIAN_POINT('Ctrl Pts',(6.18474027868607,-2.75164772317277,56.1693768980574));
#23049=CARTESIAN_POINT('Ctrl Pts',(6.2513732005971,-2.59087284652419,56.1775547757674));
#23050=CARTESIAN_POINT('Ctrl Pts',(6.31768809802375,-2.43086531349166,56.1856936222409));
#23051=CARTESIAN_POINT('Ctrl Pts',(6.37780147487082,-2.26844111862139,56.1938324687143));
#23052=CARTESIAN_POINT('Ctrl Pts',(6.43155700025837,-2.10413011775119,56.2019713151877));
#23053=CARTESIAN_POINT('Ctrl Pts',(6.48569921643279,-1.93863714442772,56.2101687085161));
#23054=CARTESIAN_POINT('Ctrl Pts',(6.53339166227497,-1.77123048055735,56.2183661018445));
#23055=CARTESIAN_POINT('Ctrl Pts',(6.57452702349717,-1.602461674208,56.2265634951729));
#23056=CARTESIAN_POINT('Ctrl Pts',(6.61566238471935,-1.43369286785871,56.2347608885013));
#23057=CARTESIAN_POINT('Ctrl Pts',(6.65024064706947,-1.26356229597695,56.2429582818297));
#23058=CARTESIAN_POINT('Ctrl Pts',(6.6782076362055,-1.09262608779333,56.251155675158));
#23059=CARTESIAN_POINT('Ctrl Pts',(6.70627293671529,-0.921088993566183,
56.259381884495));
#23060=CARTESIAN_POINT('Ctrl Pts',(6.72776404513952,-0.748230083283909,
56.267608093832));
#23061=CARTESIAN_POINT('Ctrl Pts',(6.7425611068047,-0.574594396948484,56.275834303169));
#23062=CARTESIAN_POINT('Ctrl Pts',(6.757341544605,-0.401153782868209,56.2840512707122));
#23063=CARTESIAN_POINT('Ctrl Pts',(6.76544288077921,-0.226938484562735,
56.2922682382554));
#23064=CARTESIAN_POINT('Ctrl Pts',(6.76679631720286,-0.0525033474156623,
56.3004852057985));
#23065=CARTESIAN_POINT('Ctrl Pts',(6.7681485047442,0.12177082985688,56.3086945911419));
#23066=CARTESIAN_POINT('Ctrl Pts',(6.76276519031299,0.296264085603788,56.3169039764853));
#23067=CARTESIAN_POINT('Ctrl Pts',(6.75062938420426,0.470416748339141,56.3251133618287));
#23068=CARTESIAN_POINT('Ctrl Pts',(6.73850234142858,0.644443654468779,56.3333168191293));
#23069=CARTESIAN_POINT('Ctrl Pts',(6.71963254398363,0.818130101146211,56.3415202764299));
#23070=CARTESIAN_POINT('Ctrl Pts',(6.69405506783194,0.990916620525424,56.3497237337305));
#23071=CARTESIAN_POINT('Ctrl Pts',(6.66849093053905,1.16361303034995,56.3579229128623));
#23072=CARTESIAN_POINT('Ctrl Pts',(6.63622613578524,1.33541009391742,56.3661220919942));
#23073=CARTESIAN_POINT('Ctrl Pts',(6.59734758540405,1.50575357790155,56.374321271126));
#23074=CARTESIAN_POINT('Ctrl Pts',(6.55847636057965,1.67606496550217,56.3825189053559));
#23075=CARTESIAN_POINT('Ctrl Pts',(6.51299393603396,1.84492296840324,56.3907165395857));
#23076=CARTESIAN_POINT('Ctrl Pts',(6.461038363333,2.01178335502092,56.3989141738155));
#23077=CARTESIAN_POINT('Ctrl Pts',(6.40908654084219,2.17863169747312,56.4071112163311));
#23078=CARTESIAN_POINT('Ctrl Pts',(6.35066260651705,2.34348236808057,56.4153082588467));
#23079=CARTESIAN_POINT('Ctrl Pts',(6.28595453639365,2.50580617095419,56.4235053013623));
#23080=CARTESIAN_POINT('Ctrl Pts',(6.22123937638624,2.66814775919728,56.4317032420051));
#23081=CARTESIAN_POINT('Ctrl Pts',(6.15023884166485,2.82796159486556,56.4399011826479));
#23082=CARTESIAN_POINT('Ctrl Pts',(6.07318913700969,2.98473829775871,56.4480991232908));
#23083=CARTESIAN_POINT('Ctrl Pts',(5.9961169865251,3.14156067224979,56.4562994521267));
#23084=CARTESIAN_POINT('Ctrl Pts',(5.91299231413938,3.29534382979463,56.4644997809627));
#23085=CARTESIAN_POINT('Ctrl Pts',(5.82409738891453,3.44560279260959,56.4727001097987));
#23086=CARTESIAN_POINT('Ctrl Pts',(5.73510983287103,3.59601832916258,56.4809089835901));
#23087=CARTESIAN_POINT('Ctrl Pts',(5.64034019428901,3.7429020251711,56.4891178573815));
#23088=CARTESIAN_POINT('Ctrl Pts',(5.54011476302192,3.88579688256432,56.4973267311729));
#23089=CARTESIAN_POINT('Ctrl Pts',(5.4398355418715,4.02876843005117,56.5055400105764));
#23090=CARTESIAN_POINT('Ctrl Pts',(5.33409490781192,4.16774658605689,56.5137532899798));
#23091=CARTESIAN_POINT('Ctrl Pts',(5.22325952987308,4.30230739064401,56.5219665693832));
#23092=CARTESIAN_POINT('Ctrl Pts',(5.11226203777377,4.43706501155704,56.5301918619987));
#23093=CARTESIAN_POINT('Ctrl Pts',(4.99615514830823,4.56739210122478,56.5384171546141));
#23094=CARTESIAN_POINT('Ctrl Pts',(4.87534336262341,4.69290060586455,56.5466424472295));
#23095=CARTESIAN_POINT('Ctrl Pts',(4.76608361491862,4.8064079716734,56.5540812363416));
#23096=CARTESIAN_POINT('Ctrl Pts',(4.6529763248279,4.91597456532653,56.5615200254537));
#23097=CARTESIAN_POINT('Ctrl Pts',(4.53634333548057,5.02134226503642,56.5689588145658));
#23098=CARTESIAN_POINT('Ctrl Pts',(4.4073677887153,5.13786038531722,56.5771848053285));
#23099=CARTESIAN_POINT('Ctrl Pts',(4.2737198578081,5.24956897061698,56.5854107960912));
#23100=CARTESIAN_POINT('Ctrl Pts',(4.13579271193453,5.35607203498135,56.5936367868539));
#23101=CARTESIAN_POINT('Ctrl Pts',(3.99800205900093,5.46246970373067,56.6018546371621));
#23102=CARTESIAN_POINT('Ctrl Pts',(3.85594090032626,5.56367188666554,56.6100724874703));
#23103=CARTESIAN_POINT('Ctrl Pts',(3.71003847747409,5.65932005594857,56.6182903377784));
#23104=CARTESIAN_POINT('Ctrl Pts',(3.5642860834826,5.75486987192408,56.6264997378176));
#23105=CARTESIAN_POINT('Ctrl Pts',(3.41470059302471,5.84487685720998,56.6347091378568));
#23106=CARTESIAN_POINT('Ctrl Pts',(3.26174323667611,5.92902353326394,56.642918537896));
#23107=CARTESIAN_POINT('Ctrl Pts',(3.20796365254908,5.95860938223443,56.6458049510152));
#23108=CARTESIAN_POINT('Ctrl Pts',(3.15376751463628,5.98747114796232,56.6486913641344));
#23109=CARTESIAN_POINT('Ctrl Pts',(3.09917575053263,6.01559628526637,56.6515777772535));
#23110=CARTESIAN_POINT('Origin',(0.,0.,-3.69717978381041));
#23111=CARTESIAN_POINT('',(3.09917575053261,6.01559628526638,59.0457515827422));
#23112=CARTESIAN_POINT('',(3.09917575053263,6.01559628526637,58.651392015122));
#23113=CARTESIAN_POINT('',(3.09917575053259,6.01559628526639,-3.69717978381041));
#23114=CARTESIAN_POINT('',(-6.76699881114908,0.0028363625950735,57.69717978381));
#23115=CARTESIAN_POINT('Ctrl Pts',(-6.767,2.48324459799684E-12,57.69717978381));
#23116=CARTESIAN_POINT('Ctrl Pts',(-6.76700000000007,-0.186007249413249,
57.7059292956159));
#23117=CARTESIAN_POINT('Ctrl Pts',(-6.75932637295451,-0.37201435552516,
57.7146788074219));
#23118=CARTESIAN_POINT('Ctrl Pts',(-6.74400518266947,-0.557389537152733,
57.7234283192279));
#23119=CARTESIAN_POINT('Ctrl Pts',(-6.72868405709669,-0.742763935809343,
57.7321777940784));
#23120=CARTESIAN_POINT('Ctrl Pts',(-6.70571545653017,-0.927506129693245,
57.740927268929));
#23121=CARTESIAN_POINT('Ctrl Pts',(-6.67517739415676,-1.11098863924823,
57.7496767437795));
#23122=CARTESIAN_POINT('Ctrl Pts',(-6.64463945823093,-1.29447038906542,
57.7584261824015));
#23123=CARTESIAN_POINT('Ctrl Pts',(-6.60653217027143,-1.47669218228286,
57.7671756210235));
#23124=CARTESIAN_POINT('Ctrl Pts',(-6.56098496116687,-1.65703510504219,
57.7759250596455));
#23125=CARTESIAN_POINT('Ctrl Pts',(-6.51543793687486,-1.83737729604131,
57.7846744627658));
#23126=CARTESIAN_POINT('Ctrl Pts',(-6.46245112202601,-2.01584035397176,
57.793423865886));
#23127=CARTESIAN_POINT('Ctrl Pts',(-6.40220448416196,-2.19181813638278,
57.8021732690062));
#23128=CARTESIAN_POINT('Ctrl Pts',(-6.34195808575139,-2.36779521936072,
57.8109226373515));
#23129=CARTESIAN_POINT('Ctrl Pts',(-6.27445201489185,-2.54128677544949,
57.8196720056968));
#23130=CARTESIAN_POINT('Ctrl Pts',(-6.19991555136133,-2.71170355237957,
57.828421374042));
#23131=CARTESIAN_POINT('Ctrl Pts',(-6.12537937788982,-2.88211966613192,
57.8371707083391));
#23132=CARTESIAN_POINT('Ctrl Pts',(-6.04381298133555,-3.04946076210568,
57.8459200426362));
#23133=CARTESIAN_POINT('Ctrl Pts',(-5.95549339426238,-3.21315848206981,
57.8546693769332));
#23134=CARTESIAN_POINT('Ctrl Pts',(-5.86717414355101,-3.37685557859738,
57.8634186779088));
#23135=CARTESIAN_POINT('Ctrl Pts',(-5.77210188986189,-3.5369090746739,57.8721679788843));
#23136=CARTESIAN_POINT('Ctrl Pts',(-5.67059953467031,-3.69277536784962,
57.8809172798599));
#23137=CARTESIAN_POINT('Ctrl Pts',(-5.56909755761735,-3.84864108035837,
57.8896665482406));
#23138=CARTESIAN_POINT('Ctrl Pts',(-5.46116568338046,-4.00031938104311,
57.8984158166214));
#23139=CARTESIAN_POINT('Ctrl Pts',(-5.34717048686099,-4.14729511663238,
57.9071650850021));
#23140=CARTESIAN_POINT('Ctrl Pts',(-5.23317570555503,-4.29427031688057,
57.9159143215147));
#23141=CARTESIAN_POINT('Ctrl Pts',(-5.11311782178793,-4.43654275987144,
57.9246635580274));
#23142=CARTESIAN_POINT('Ctrl Pts',(-4.98740459172003,-4.57362924147661,
57.93341279454));
#23143=CARTESIAN_POINT('Ctrl Pts',(-4.86169180910817,-4.7107152351445,57.9421619999111));
#23144=CARTESIAN_POINT('Ctrl Pts',(-4.73032391415416,-4.84261509316539,
57.9509112052822));
#23145=CARTESIAN_POINT('Ctrl Pts',(-4.59374707237275,-4.9688808433154,57.9596604106533));
#23146=CARTESIAN_POINT('Ctrl Pts',(-4.45717070537378,-5.09514615452746,
57.9684095856096));
#23147=CARTESIAN_POINT('Ctrl Pts',(-4.31538563819479,-5.21577720253658,
57.9771587605658));
#23148=CARTESIAN_POINT('Ctrl Pts',(-4.16887341290611,-5.33036429028679,
57.985907935522));
#23149=CARTESIAN_POINT('Ctrl Pts',(-4.02236168477283,-5.44495098921219,
57.99465708079));
#23150=CARTESIAN_POINT('Ctrl Pts',(-3.87112305634363,-5.55349359238812,
58.0034062260579));
#23151=CARTESIAN_POINT('Ctrl Pts',(-3.71567117316636,-5.65562346102536,
58.0121553713258));
#23152=CARTESIAN_POINT('Ctrl Pts',(-3.56021980457208,-5.75775299158826,
58.020904487632));
#23153=CARTESIAN_POINT('Ctrl Pts',(-3.400555448623,-5.85346967275404,58.0296536039381));
#23154=CARTESIAN_POINT('Ctrl Pts',(-3.2372203632332,-5.94244842803607,58.0384027202443));
#23155=CARTESIAN_POINT('Ctrl Pts',(-3.07388580495989,-6.03142689616504,
58.0471518083152));
#23156=CARTESIAN_POINT('Ctrl Pts',(-2.90688079257676,-6.11366734484836,
58.0559008963862));
#23157=CARTESIAN_POINT('Ctrl Pts',(-2.73677251094612,-6.18889046787303,
58.0646499844571));
#23158=CARTESIAN_POINT('Ctrl Pts',(-2.56666476416658,-6.26411335438264,
58.0733990450193));
#23159=CARTESIAN_POINT('Ctrl Pts',(-2.39345402972123,-6.33231884350279,
58.0821481055815));
#23160=CARTESIAN_POINT('Ctrl Pts',(-2.21772856474086,-6.39327529621027,
58.0908971661437));
#23161=CARTESIAN_POINT('Ctrl Pts',(-2.04200363768338,-6.45423156232059,
58.0996461999237));
#23162=CARTESIAN_POINT('Ctrl Pts',(-1.86376426620184,-6.50793874252029,
58.1083952337037));
#23163=CARTESIAN_POINT('Ctrl Pts',(-1.68361578194802,-6.55421443796094,
58.1171442674837));
#23164=CARTESIAN_POINT('Ctrl Pts',(-1.50346783420026,-6.60048999558642,
58.1258932752079));
#23165=CARTESIAN_POINT('Ctrl Pts',(-1.3214110625745,-6.63933404145454,58.1346422829321));
#23166=CARTESIAN_POINT('Ctrl Pts',(-1.13806375959293,-6.67061465526987,
58.1433912906564));
#23167=CARTESIAN_POINT('Ctrl Pts',(-0.954716987421843,-6.70189517852442,
58.1521402730512));
#23168=CARTESIAN_POINT('Ctrl Pts',(-0.77007997381277,-6.72561226535794,
58.1608892554461));
#23169=CARTESIAN_POINT('Ctrl Pts',(-0.584779770555553,-6.74168536939755,
58.169638237841));
#23170=CARTESIAN_POINT('Ctrl Pts',(-0.391490647557006,-6.75845143942376,
58.178764418517));
#23171=CARTESIAN_POINT('Ctrl Pts',(-0.197480213107425,-6.76689975924017,
58.1878905991931));
#23172=CARTESIAN_POINT('Ctrl Pts',(-0.00346532630087703,-6.76699911271707,
58.1970167798691));
#23173=CARTESIAN_POINT('Ctrl Pts',(0.184486595292999,-6.76709536139782,
58.2058577673991));
#23174=CARTESIAN_POINT('Ctrl Pts',(0.3724423781822,-6.75935659726787,58.214698754929));
#23175=CARTESIAN_POINT('Ctrl Pts',(0.559750217719087,-6.74380965729041,
58.2235397424589));
#23176=CARTESIAN_POINT('Ctrl Pts',(0.745129914454696,-6.72842275717287,
58.2322897210567));
#23177=CARTESIAN_POINT('Ctrl Pts',(0.929874656311072,-6.70538772273516,
58.2410396996545));
#23178=CARTESIAN_POINT('Ctrl Pts',(1.11335688289461,-6.67478280180795,58.2497896782522));
#23179=CARTESIAN_POINT('Ctrl Pts',(1.29683723118535,-6.64417819418086,58.2585395672772));
#23180=CARTESIAN_POINT('Ctrl Pts',(1.47905480729908,-6.60600390230148,58.2672894563021));
#23181=CARTESIAN_POINT('Ctrl Pts',(1.65939064804477,-6.56038959797218,58.276039345327));
#23182=CARTESIAN_POINT('Ctrl Pts',(1.83972470263941,-6.51477574543348,58.284789147688));
#23183=CARTESIAN_POINT('Ctrl Pts',(2.01817678125532,-6.46172209820199,58.2935389500489));
#23184=CARTESIAN_POINT('Ctrl Pts',(2.19414072347371,-6.4014088672412,58.3022887524099));
#23185=CARTESIAN_POINT('Ctrl Pts',(2.37010298131792,-6.34109621361488,58.3110384710154));
#23186=CARTESIAN_POINT('Ctrl Pts',(2.54357687926612,-6.27352420826093,58.3197881896209));
#23187=CARTESIAN_POINT('Ctrl Pts',(2.71397317789675,-6.19892237325626,58.3285379082263));
#23188=CARTESIAN_POINT('Ctrl Pts',(2.88436790206907,-6.12432122757102,58.3372875459846));
#23189=CARTESIAN_POINT('Ctrl Pts',(3.05168482125965,-6.04269049717564,58.3460371837429));
#23190=CARTESIAN_POINT('Ctrl Pts',(3.21535561997101,-5.95430745235085,58.3547868215011));
#23191=CARTESIAN_POINT('Ctrl Pts',(3.37902496075002,-5.86592519481678,58.3635363813202));
#23192=CARTESIAN_POINT('Ctrl Pts',(3.53904799384605,-5.77079087940398,58.3722859411392));
#23193=CARTESIAN_POINT('Ctrl Pts',(3.69488118814723,-5.66922763747195,58.3810355009582));
#23194=CARTESIAN_POINT('Ctrl Pts',(3.85071304610573,-5.56766526649232,58.3897849857456));
#23195=CARTESIAN_POINT('Ctrl Pts',(4.00235489705709,-5.45967423580903,58.3985344705331));
#23196=CARTESIAN_POINT('Ctrl Pts',(4.14929168607398,-5.34562133936527,58.4072839553205));
#23197=CARTESIAN_POINT('Ctrl Pts',(4.29622726385506,-5.23156938308737,58.4160333679838));
#23198=CARTESIAN_POINT('Ctrl Pts',(4.43845763091822,-5.11145583677415,58.4247827806471));
#23199=CARTESIAN_POINT('Ctrl Pts',(4.57549970660723,-4.98568866204431,58.4335321933104));
#23200=CARTESIAN_POINT('Ctrl Pts',(4.71254069815065,-4.85992248226385,58.4422815367567));
#23201=CARTESIAN_POINT('Ctrl Pts',(4.84439326931092,-4.72850295734229,58.451030880203));
#23202=CARTESIAN_POINT('Ctrl Pts',(4.97060959434485,-4.59187644221912,58.4597802236494));
#23203=CARTESIAN_POINT('Ctrl Pts',(5.09682496280305,-4.45525096256904,58.4685295007857));
#23204=CARTESIAN_POINT('Ctrl Pts',(5.21740397615631,-4.31341878218577,58.477278777922));
#23205=CARTESIAN_POINT('Ctrl Pts',(5.3319371045173,-4.16686161438938,58.4860280550582));
#23206=CARTESIAN_POINT('Ctrl Pts',(5.44646940289187,-4.0203055086478,58.4947772687912));
#23207=CARTESIAN_POINT('Ctrl Pts',(5.55495572749476,-3.86902470980404,58.5035264825242));
#23208=CARTESIAN_POINT('Ctrl Pts',(5.65702762491275,-3.71353301466057,58.5122756962571));
#23209=CARTESIAN_POINT('Ctrl Pts',(5.75909881654979,-3.55804239467176,58.5210248494933));
#23210=CARTESIAN_POINT('Ctrl Pts',(5.85475551250613,-3.39834117619844,58.5297740027294));
#23211=CARTESIAN_POINT('Ctrl Pts',(5.94367283727932,-3.23497174692268,58.5385231559655));
#23212=CARTESIAN_POINT('Ctrl Pts',(6.03258957676171,-3.07160339301243,58.547272251611));
#23213=CARTESIAN_POINT('Ctrl Pts',(6.11476689685164,-2.90456712829758,58.5560213472566));
#23214=CARTESIAN_POINT('Ctrl Pts',(6.18992570525159,-2.73443024476135,58.5647704429021));
#23215=CARTESIAN_POINT('Ctrl Pts',(6.26508404388607,-2.56429442463251,58.5735194838632));
#23216=CARTESIAN_POINT('Ctrl Pts',(6.33322384283236,-2.39105828656204,58.5822685248242));
#23217=CARTESIAN_POINT('Ctrl Pts',(6.39411368719963,-2.21531017132282,58.5910175657852));
#23218=CARTESIAN_POINT('Ctrl Pts',(6.45500317120822,-2.03956309619727,58.5997665549676));
#23219=CARTESIAN_POINT('Ctrl Pts',(6.50864269270009,-1.86130434438857,58.60851554415));
#23220=CARTESIAN_POINT('Ctrl Pts',(6.55485008446273,-1.6811393072018,58.6172645333324));
#23221=CARTESIAN_POINT('Ctrl Pts',(6.60199664749351,-1.49731239212072,58.6261913468618));
#23222=CARTESIAN_POINT('Ctrl Pts',(6.64140563640862,-1.31150116499899,58.6351181603912));
#23223=CARTESIAN_POINT('Ctrl Pts',(6.67293772282135,-1.12436255155884,58.6440449739205));
#23224=CARTESIAN_POINT('Ctrl Pts',(6.7038449494984,-0.940932395053588,58.6527948880761));
#23225=CARTESIAN_POINT('Ctrl Pts',(6.72718449348905,-0.756227260508963,
58.6615448022316));
#23226=CARTESIAN_POINT('Ctrl Pts',(6.74287707373913,-0.570874564543943,
58.6702947163871));
#23227=CARTESIAN_POINT('Ctrl Pts',(6.75856934538658,-0.385525513634686,
58.6790444584711));
#23228=CARTESIAN_POINT('Ctrl Pts',(6.76661493004097,-0.199529212420397,
58.6877942005551));
#23229=CARTESIAN_POINT('Ctrl Pts',(6.76698649908906,-0.013517438602549,
58.6965439426391));
#23230=CARTESIAN_POINT('Ctrl Pts',(6.76735806132395,0.172490924443669,58.705293524285));
#23231=CARTESIAN_POINT('Ctrl Pts',(6.760055888963,0.358514472899315,58.7140431059309));
#23232=CARTESIAN_POINT('Ctrl Pts',(6.74510478454601,0.543921359660137,58.7227926875768));
#23233=CARTESIAN_POINT('Ctrl Pts',(6.7301539344071,0.72932509314843,58.7315421204158));
#23234=CARTESIAN_POINT('Ctrl Pts',(6.70755443556924,0.914111900254398,58.7402915532548));
#23235=CARTESIAN_POINT('Ctrl Pts',(6.6773830468235,1.09765415591349,58.7490409860939));
#23236=CARTESIAN_POINT('Ctrl Pts',(6.64721213111895,1.28119353391093,58.7577902817552));
#23237=CARTESIAN_POINT('Ctrl Pts',(6.60946960955533,1.46348811672481,58.7665395774165));
#23238=CARTESIAN_POINT('Ctrl Pts',(6.56428366991224,1.64391876348059,58.7752888730779));
#23239=CARTESIAN_POINT('Ctrl Pts',(6.51909837867765,1.82434682109545,58.7840380431887));
#23240=CARTESIAN_POINT('Ctrl Pts',(6.46646995271976,2.00291071820267,58.7927872132995));
#23241=CARTESIAN_POINT('Ctrl Pts',(6.40657713281612,2.17900400212519,58.8015363834103));
#23242=CARTESIAN_POINT('Ctrl Pts',(6.34668509279128,2.35509499309474,58.8102854395961));
#23243=CARTESIAN_POINT('Ctrl Pts',(6.27952894037599,2.5287151639794,58.8190344957819));
#23244=CARTESIAN_POINT('Ctrl Pts',(6.20533675061526,2.69927486771238,58.8277835519677));
#23245=CARTESIAN_POINT('Ctrl Pts',(6.12832117907998,2.87632521635751,58.8368655532499));
#23246=CARTESIAN_POINT('Ctrl Pts',(6.04372366626162,3.05007728919834,58.8459475545322));
#23247=CARTESIAN_POINT('Ctrl Pts',(5.95185378007951,3.21989527478042,58.8550295558145));
#23248=CARTESIAN_POINT('Ctrl Pts',(5.86334450817458,3.38350129286602,58.8637793361216));
#23249=CARTESIAN_POINT('Ctrl Pts',(5.76808562057345,3.54345567124816,58.8725291164287));
#23250=CARTESIAN_POINT('Ctrl Pts',(5.66640068804577,3.69921508465167,58.8812788967359));
#23251=CARTESIAN_POINT('Ctrl Pts',(5.56471941108017,3.85496889852148,58.8900283624894));
#23252=CARTESIAN_POINT('Ctrl Pts',(5.45661270815207,4.00652780919509,58.8987778282428));
#23253=CARTESIAN_POINT('Ctrl Pts',(5.34244776449207,4.15337704569109,58.9075272939963));
#23254=CARTESIAN_POINT('Ctrl Pts',(5.22828631819689,4.30022178356136,58.9162764917159));
#23255=CARTESIAN_POINT('Ctrl Pts',(5.10806717844163,4.44235690972572,58.9250256894355));
#23256=CARTESIAN_POINT('Ctrl Pts',(4.98219864544812,4.57929969070544,58.9337748871551));
#23257=CARTESIAN_POINT('Ctrl Pts',(4.85633329944126,4.71623900429896,58.9425238633454));
#23258=CARTESIAN_POINT('Ctrl Pts',(4.72481904033758,4.84798602483509,58.9512728395356));
#23259=CARTESIAN_POINT('Ctrl Pts',(4.58810250737318,4.97409332259016,58.9600218157258));
#23260=CARTESIAN_POINT('Ctrl Pts',(4.45137708685764,5.10020881822029,58.968771360662));
#23261=CARTESIAN_POINT('Ctrl Pts',(4.30944892636175,5.22068366307831,58.9775209055982));
#23262=CARTESIAN_POINT('Ctrl Pts',(4.16280009466787,5.33510865604752,58.9862704505343));
#23263=CARTESIAN_POINT('Ctrl Pts',(4.01615988348914,5.44952692272799,58.9950194811426));
#23264=CARTESIAN_POINT('Ctrl Pts',(3.86479978232355,5.5578958728854,59.0037685117509));
#23265=CARTESIAN_POINT('Ctrl Pts',(3.70923383581191,5.65984746713797,59.0125175423592));
#23266=CARTESIAN_POINT('Ctrl Pts',(3.55366577799669,5.76180044505304,59.0212666917072));
#23267=CARTESIAN_POINT('Ctrl Pts',(3.39389200026974,5.85733573570982,59.0300158410552));
#23268=CARTESIAN_POINT('Ctrl Pts',(3.2304551362618,5.94612887621853,59.0387649904032));
#23269=CARTESIAN_POINT('Ctrl Pts',(3.18695122151672,5.96976399206638,59.0410938545162));
#23270=CARTESIAN_POINT('Ctrl Pts',(3.14318791262713,5.99292165435308,59.0434227186292));
#23271=CARTESIAN_POINT('Ctrl Pts',(3.09917575053261,6.01559628526638,59.0457515827422));
#23272=CARTESIAN_POINT('Ctrl Pts',(3.09917575053259,6.01559628526639,57.0458946091257));
#23273=CARTESIAN_POINT('Ctrl Pts',(2.93318603311847,6.10111254710523,57.0546656682455));
#23274=CARTESIAN_POINT('Ctrl Pts',(2.76353838605607,6.17981426143319,57.0634367273652));
#23275=CARTESIAN_POINT('Ctrl Pts',(2.59080947744217,6.25139946344783,57.072207786485));
#23276=CARTESIAN_POINT('Ctrl Pts',(2.41808056882822,6.32298466546249,57.0809788456047));
#23277=CARTESIAN_POINT('Ctrl Pts',(2.2422706905842,6.38745318365418,57.0897499047244));
#23278=CARTESIAN_POINT('Ctrl Pts',(2.06398265584147,6.44455309516382,57.0985209638442));
#23279=CARTESIAN_POINT('Ctrl Pts',(1.88926810960206,6.50050853347528,57.1071162216042));
#23280=CARTESIAN_POINT('Ctrl Pts',(1.71237973373101,6.54932200570452,57.1157114793643));
#23281=CARTESIAN_POINT('Ctrl Pts',(1.53391690303733,6.59085638855653,57.1243067371243));
#23282=CARTESIAN_POINT('Ctrl Pts',(1.3552869494704,6.63242966659682,57.1329100439788));
#23283=CARTESIAN_POINT('Ctrl Pts',(1.17507989550135,6.66671017993159,57.1415133508332));
#23284=CARTESIAN_POINT('Ctrl Pts',(0.993904102582022,6.69361215151211,57.1501166576877));
#23285=CARTESIAN_POINT('Ctrl Pts',(0.805216698462053,6.72162948816315,57.1590766606277));
#23286=CARTESIAN_POINT('Ctrl Pts',(0.615478894157729,6.74164336922374,57.1680366635677));
#23287=CARTESIAN_POINT('Ctrl Pts',(0.425380962470535,6.75361681151423,57.1769966665077));
#23288=CARTESIAN_POINT('Ctrl Pts',(0.242351441030697,6.76514504537225,57.1856235097124));
#23289=CARTESIAN_POINT('Ctrl Pts',(0.0589883873994425,6.76922003344946,
57.1942503529171));
#23290=CARTESIAN_POINT('Ctrl Pts',(-0.124094149256997,6.76586207678816,
57.2028771961219));
#23291=CARTESIAN_POINT('Ctrl Pts',(-0.307351666537452,6.76250091076914,
57.2115122844079));
#23292=CARTESIAN_POINT('Ctrl Pts',(-0.49032782722238,6.7516926346868,57.220147372694));
#23293=CARTESIAN_POINT('Ctrl Pts',(-0.672413472376344,6.73350942096072,
57.2287824609801));
#23294=CARTESIAN_POINT('Ctrl Pts',(-0.854769551255752,6.71529920151311,
57.2374303741052));
#23295=CARTESIAN_POINT('Ctrl Pts',(-1.0362321690501,6.68969219430666,57.2460782872303));
#23296=CARTESIAN_POINT('Ctrl Pts',(-1.21620064023721,6.65681192483959,57.2547262003555));
#23297=CARTESIAN_POINT('Ctrl Pts',(-1.23639036301568,6.65312325914697,57.2556963645595));
#23298=CARTESIAN_POINT('Ctrl Pts',(-1.25656129563698,6.6493431084083,57.2566665287636));
#23299=CARTESIAN_POINT('Ctrl Pts',(-1.27671260132203,6.64547168631585,57.2576366929677));
#23300=CARTESIAN_POINT('Ctrl Pts',(-1.44754763156528,6.61265125668285,57.2658613724865));
#23301=CARTESIAN_POINT('Ctrl Pts',(-1.61734140890645,6.5731958646621,57.2740860520053));
#23302=CARTESIAN_POINT('Ctrl Pts',(-1.78554078892278,6.52718416249251,57.2823107315241));
#23303=CARTESIAN_POINT('Ctrl Pts',(-1.95356337236176,6.48122082382735,57.2905267659742));
#23304=CARTESIAN_POINT('Ctrl Pts',(-2.11999455290109,6.42871499207132,57.2987428004244));
#23305=CARTESIAN_POINT('Ctrl Pts',(-2.28428994028193,6.36979657985456,57.3069588348745));
#23306=CARTESIAN_POINT('Ctrl Pts',(-2.44844554327894,6.31092829609289,57.3151678790291));
#23307=CARTESIAN_POINT('Ctrl Pts',(-2.61046863671812,6.24565841824118,57.3233769231837));
#23308=CARTESIAN_POINT('Ctrl Pts',(-2.7698285067248,6.17416707283944,57.3315859673383));
#23309=CARTESIAN_POINT('Ctrl Pts',(-2.92908470258851,6.10272223728966,57.3397896709664));
#23310=CARTESIAN_POINT('Ctrl Pts',(-3.08568080036079,6.0250641425843,57.3479933745944));
#23311=CARTESIAN_POINT('Ctrl Pts',(-3.23910455825723,5.94142160267029,57.3561970782225));
#23312=CARTESIAN_POINT('Ctrl Pts',(-3.39245921996666,5.85781673215416,57.3643970872165));
#23313=CARTESIAN_POINT('Ctrl Pts',(-3.54264407412645,5.76823295714502,57.3725970962105));
#23314=CARTESIAN_POINT('Ctrl Pts',(-3.68916997333061,5.67294578749664,57.3807971052045));
#23315=CARTESIAN_POINT('Ctrl Pts',(-3.83568415601414,5.57766623721176,57.3889964585084));
#23316=CARTESIAN_POINT('Ctrl Pts',(-3.9785396615097,5.47668438860189,57.3971958118123));
#23317=CARTESIAN_POINT('Ctrl Pts',(-4.11727460720717,5.37032017749846,57.4053951651163));
#23318=CARTESIAN_POINT('Ctrl Pts',(-4.25600864839371,5.26395665985831,57.4135944649628));
#23319=CARTESIAN_POINT('Ctrl Pts',(-4.39062189811246,5.15221106689264,57.4217937648094));
#23320=CARTESIAN_POINT('Ctrl Pts',(-4.52068408089549,5.03544481061386,57.429993064656));
#23321=CARTESIAN_POINT('Ctrl Pts',(-4.65076901026754,4.91865813307208,57.438193798479));
#23322=CARTESIAN_POINT('Ctrl Pts',(-4.77630102015048,4.79684928233111,57.446394532302));
#23323=CARTESIAN_POINT('Ctrl Pts',(-4.89688531866907,4.67041788021194,57.454595266125));
#23324=CARTESIAN_POINT('Ctrl Pts',(-5.01751258160126,4.54394143034509,57.462798921885));
#23325=CARTESIAN_POINT('Ctrl Pts',(-5.13318837414066,4.41283940741912,57.471002577645));
#23326=CARTESIAN_POINT('Ctrl Pts',(-5.24355691907412,4.27754600634873,57.4792062334049));
#23327=CARTESIAN_POINT('Ctrl Pts',(-5.35405189827077,4.14209761799016,57.48741928698));
#23328=CARTESIAN_POINT('Ctrl Pts',(-5.45922725652506,4.00244853694774,57.4956323405549));
#23329=CARTESIAN_POINT('Ctrl Pts',(-5.55876882285838,3.85906441693031,57.50384539413));
#23330=CARTESIAN_POINT('Ctrl Pts',(-5.65836929016983,3.71559545331207,57.512063307553));
#23331=CARTESIAN_POINT('Ctrl Pts',(-5.75232912779609,3.56838734685494,57.5202812209761));
#23332=CARTESIAN_POINT('Ctrl Pts',(-5.84037927736495,3.41793196195098,57.5284991343992));
#23333=CARTESIAN_POINT('Ctrl Pts',(-5.92856675546629,3.2672419173978,57.5367298649952));
#23334=CARTESIAN_POINT('Ctrl Pts',(-6.0108259569123,3.11329478905805,57.5449605955912));
#23335=CARTESIAN_POINT('Ctrl Pts',(-6.08693469270373,2.95660532482097,57.5531913261871));
#23336=CARTESIAN_POINT('Ctrl Pts',(-6.15683146409667,2.81270479162234,57.5607502678629));
#23337=CARTESIAN_POINT('Ctrl Pts',(-6.22154127474536,2.66649174099346,57.5683092095387));
#23338=CARTESIAN_POINT('Ctrl Pts',(-6.28092899305939,2.51837645798755,57.5758681512144));
#23339=CARTESIAN_POINT('Ctrl Pts',(-6.35325564641545,2.33799096693271,57.5850739764228));
#23340=CARTESIAN_POINT('Ctrl Pts',(-6.4178787503003,2.15431021712131,57.5942798016312));
#23341=CARTESIAN_POINT('Ctrl Pts',(-6.47451834347859,1.96796880563672,57.6034856268395));
#23342=CARTESIAN_POINT('Ctrl Pts',(-6.53087849318174,1.7825467491239,57.6126460331519));
#23343=CARTESIAN_POINT('Ctrl Pts',(-6.57933360955935,1.59449040026369,57.6218064394644));
#23344=CARTESIAN_POINT('Ctrl Pts',(-6.61965344318901,1.40444910626052,57.6309668457768));
#23345=CARTESIAN_POINT('Ctrl Pts',(-6.65984329256155,1.21502047293069,57.6400977205039));
#23346=CARTESIAN_POINT('Ctrl Pts',(-6.69195011400064,1.02361985191255,57.6492285952309));
#23347=CARTESIAN_POINT('Ctrl Pts',(-6.71579294063093,0.830911655094422,
57.658359469958));
#23348=CARTESIAN_POINT('Ctrl Pts',(-6.73951276827878,0.63919759007472,57.6674432408614));
#23349=CARTESIAN_POINT('Ctrl Pts',(-6.75505355118757,0.446189597845692,
57.6765270117648));
#23350=CARTESIAN_POINT('Ctrl Pts',(-6.76228528965658,0.252560213205239,
57.6856107826683));
#23351=CARTESIAN_POINT('Ctrl Pts',(-6.76535537994889,0.170358720903004,
57.6894671163822));
#23352=CARTESIAN_POINT('Ctrl Pts',(-6.76692856984046,0.0880454475793552,
57.6933234500961));
#23353=CARTESIAN_POINT('Ctrl Pts',(-6.76699762229816,0.00567272518766376,
57.69717978381));
#23354=CARTESIAN_POINT('',(-6.76699917942892,0.00177812752557784,57.3028202161898));
#23355=CARTESIAN_POINT('Ctrl Pts',(3.09917575053263,6.01559628526637,56.6515777772535));
#23356=CARTESIAN_POINT('Ctrl Pts',(2.94405292266811,6.09551403301305,56.6597795375883));
#23357=CARTESIAN_POINT('Ctrl Pts',(2.78573390061559,6.16948079869564,56.6679812979231));
#23358=CARTESIAN_POINT('Ctrl Pts',(2.62471678447104,6.2372390367306,56.6761830582579));
#23359=CARTESIAN_POINT('Ctrl Pts',(2.46377224922607,6.3049667317153,56.6843811215253));
#23360=CARTESIAN_POINT('Ctrl Pts',(2.3001323728999,6.36649133592748,56.6925791847926));
#23361=CARTESIAN_POINT('Ctrl Pts',(2.13431734198294,6.42160248565036,56.7007772480599));
#23362=CARTESIAN_POINT('Ctrl Pts',(1.96851864043036,6.47670820806041,56.7089745039869));
#23363=CARTESIAN_POINT('Ctrl Pts',(1.80054554873222,6.52540161398418,56.7171717599139));
#23364=CARTESIAN_POINT('Ctrl Pts',(1.63093593018586,6.56752137351899,56.7253690158409));
#23365=CARTESIAN_POINT('Ctrl Pts',(1.46132768219545,6.60964079269878,56.7335662055288));
#23366=CARTESIAN_POINT('Ctrl Pts',(1.29008328168006,6.64518658412611,56.7417633952166));
#23367=CARTESIAN_POINT('Ctrl Pts',(1.11775327674701,6.6740479929591,56.7499605849045));
#23368=CARTESIAN_POINT('Ctrl Pts',(0.945393343640902,6.70291441408949,56.7581591981802));
#23369=CARTESIAN_POINT('Ctrl Pts',(0.771947784351753,6.72509408092856,56.766357811456));
#23370=CARTESIAN_POINT('Ctrl Pts',(0.597974857397319,6.74052780351218,56.7745564247317));
#23371=CARTESIAN_POINT('Ctrl Pts',(0.423940097438025,6.7559670115093,56.7827579519373));
#23372=CARTESIAN_POINT('Ctrl Pts',(0.24937795353745,6.76465546779899,56.7909594791428));
#23373=CARTESIAN_POINT('Ctrl Pts',(0.0748493465936413,6.76658603546238,
56.7991610063483));
#23374=CARTESIAN_POINT('Ctrl Pts',(-0.09986542506865,6.76851866240759,56.8073712818905));
#23375=CARTESIAN_POINT('Ctrl Pts',(-0.274546229425493,6.76367899881959,
56.8155815574327));
#23376=CARTESIAN_POINT('Ctrl Pts',(-0.448633668200303,6.75211202748867,
56.8237918329748));
#23377=CARTESIAN_POINT('Ctrl Pts',(-0.622824548304756,6.74053818315816,
56.8320069869955));
#23378=CARTESIAN_POINT('Ctrl Pts',(-0.796421004089131,6.72222910078704,
56.8402221410161));
#23379=CARTESIAN_POINT('Ctrl Pts',(-0.968871311662083,6.69728134256268,
56.8484372950367));
#23380=CARTESIAN_POINT('Ctrl Pts',(-1.14155771237634,6.67229942960303,56.8566636960162));
#23381=CARTESIAN_POINT('Ctrl Pts',(-1.31309447847888,6.64066075042655,56.8648900969957));
#23382=CARTESIAN_POINT('Ctrl Pts',(-1.4829415689939,6.60251265072244,56.8731164979752));
#23383=CARTESIAN_POINT('Ctrl Pts',(-1.57685225994353,6.58142006449818,56.8776649833079));
#23384=CARTESIAN_POINT('Ctrl Pts',(-1.6702466723437,6.55833834733766,56.8822134686406));
#23385=CARTESIAN_POINT('Ctrl Pts',(-1.76303592873773,6.53329880795145,56.8867619539734));
#23386=CARTESIAN_POINT('Ctrl Pts',(-1.92934835439208,6.48841875723844,56.8949145101866));
#23387=CARTESIAN_POINT('Ctrl Pts',(-2.09420608726525,6.43711385937417,56.9030670663999));
#23388=CARTESIAN_POINT('Ctrl Pts',(-2.25707025773122,6.37949236629884,56.9112196226131));
#23389=CARTESIAN_POINT('Ctrl Pts',(-2.41974574612937,6.32193762911238,56.9193627338935));
#23390=CARTESIAN_POINT('Ctrl Pts',(-2.58043192847426,6.25808098443318,56.9275058451738));
#23391=CARTESIAN_POINT('Ctrl Pts',(-2.73860145605382,6.18808137187124,56.9356489564542));
#23392=CARTESIAN_POINT('Ctrl Pts',(-2.89662099359569,6.11814813900132,56.9437843457315));
#23393=CARTESIAN_POINT('Ctrl Pts',(-3.05212829561936,6.04208368258898,56.9519197350089));
#23394=CARTESIAN_POINT('Ctrl Pts',(-3.20461248564616,5.96009629258125,56.9600551242862));
#23395=CARTESIAN_POINT('Ctrl Pts',(-3.35698411757205,5.8781694225849,56.9681845083248));
#23396=CARTESIAN_POINT('Ctrl Pts',(-3.50633676029002,5.7903284969734,56.9763138923634));
#23397=CARTESIAN_POINT('Ctrl Pts',(-3.65218080266926,5.69682932732008,56.9844432764019));
#23398=CARTESIAN_POINT('Ctrl Pts',(-3.79794782267948,5.60337953594392,56.9925683671941));
#23399=CARTESIAN_POINT('Ctrl Pts',(-3.94020962550192,5.50427764850932,57.0006934579862));
#23400=CARTESIAN_POINT('Ctrl Pts',(-4.07850245121144,5.39982469673436,57.0088185487783));
#23401=CARTESIAN_POINT('Ctrl Pts',(-4.21732317061703,5.29497302539824,57.0169746548035));
#23402=CARTESIAN_POINT('Ctrl Pts',(-4.35214422810211,5.18472953990045,57.0251307608286));
#23403=CARTESIAN_POINT('Ctrl Pts',(-4.48252671162608,5.06944210732884,57.0332868668537));
#23404=CARTESIAN_POINT('Ctrl Pts',(-4.61238442923383,4.95461868582334,57.0414101460271));
#23405=CARTESIAN_POINT('Ctrl Pts',(-4.73783897379996,4.83479210393786,57.0495334252005));
#23406=CARTESIAN_POINT('Ctrl Pts',(-4.85849089436494,4.71034555307495,57.0576567043739));
#23407=CARTESIAN_POINT('Ctrl Pts',(-4.97915888075271,4.58588243110217,57.0657810652306));
#23408=CARTESIAN_POINT('Ctrl Pts',(-5.09502271468609,4.45679837748956,57.0739054260873));
#23409=CARTESIAN_POINT('Ctrl Pts',(-5.20572086942813,4.32351237185699,57.082029786944));
#23410=CARTESIAN_POINT('Ctrl Pts',(-5.31645482545819,4.19018325971837,57.0901567753294));
#23411=CARTESIAN_POINT('Ctrl Pts',(-5.42201954189366,4.05264977069983,57.0982837637148));
#23412=CARTESIAN_POINT('Ctrl Pts',(-5.52209476250759,3.91136273361168,57.1064107521003));
#23413=CARTESIAN_POINT('Ctrl Pts',(-5.62281695802919,3.76916229191435,57.1145902805403));
#23414=CARTESIAN_POINT('Ctrl Pts',(-5.71797821649251,3.62315990804978,57.1227698089804));
#23415=CARTESIAN_POINT('Ctrl Pts',(-5.8072976639558,3.47384266227093,57.1309493374205));
#23416=CARTESIAN_POINT('Ctrl Pts',(-5.89619647734567,3.32522859954018,57.1390903458242));
#23417=CARTESIAN_POINT('Ctrl Pts',(-5.97930826431235,3.17333118059628,57.1472313542278));
#23418=CARTESIAN_POINT('Ctrl Pts',(-6.05640359250733,3.01865276649441,57.1553723626315));
#23419=CARTESIAN_POINT('Ctrl Pts',(-6.13404609766739,2.8628765366471,57.1635711510898));
#23420=CARTESIAN_POINT('Ctrl Pts',(-6.20558627238428,2.70428003495723,57.1717699395481));
#23421=CARTESIAN_POINT('Ctrl Pts',(-6.27084024999759,2.54339370900577,57.1799687280064));
#23422=CARTESIAN_POINT('Ctrl Pts',(-6.33609422761088,2.38250738305437,57.1881675164646));
#23423=CARTESIAN_POINT('Ctrl Pts',(-6.39506194283338,2.21933160411982,57.1963663049229));
#23424=CARTESIAN_POINT('Ctrl Pts',(-6.44761148990513,2.05440869235978,57.2045650933811));
#23425=CARTESIAN_POINT('Ctrl Pts',(-6.5133098196148,1.84821928755487,57.2148153569394));
#23426=CARTESIAN_POINT('Ctrl Pts',(-6.56914272493654,1.63878519480052,57.2250656204976));
#23427=CARTESIAN_POINT('Ctrl Pts',(-6.61484041058002,1.42694615965621,57.2353158840558));
#23428=CARTESIAN_POINT('Ctrl Pts',(-6.66019682625352,1.21668913682053,57.2454895987235));
#23429=CARTESIAN_POINT('Ctrl Pts',(-6.69556881076077,1.00406286086859,57.2556633133912));
#23430=CARTESIAN_POINT('Ctrl Pts',(-6.72073887317306,0.789910120596348,
57.2658370280589));
#23431=CARTESIAN_POINT('Ctrl Pts',(-6.74554717001033,0.578835365907071,
57.2758645174342));
#23432=CARTESIAN_POINT('Ctrl Pts',(-6.76044466374881,0.36627764876757,57.2858920068094));
#23433=CARTESIAN_POINT('Ctrl Pts',(-6.76526863623834,0.153066258626491,
57.2959194961847));
#23434=CARTESIAN_POINT('Ctrl Pts',(-6.76637522374717,0.104156970361828,
57.2982197361864));
#23435=CARTESIAN_POINT('Ctrl Pts',(-6.76695192245588,0.0552133810525768,
57.3005199761882));
#23436=CARTESIAN_POINT('Ctrl Pts',(-6.76699711774311,0.00624567502194366,
57.3028202161899));
#23437=CARTESIAN_POINT('Ctrl Pts',(-6.767,2.30894580037963E-12,57.3028202161898));
#23438=CARTESIAN_POINT('Ctrl Pts',(-6.76700000000006,-0.186007249413423,
57.3115697279958));
#23439=CARTESIAN_POINT('Ctrl Pts',(-6.7593263729545,-0.372014355525331,
57.3203192398017));
#23440=CARTESIAN_POINT('Ctrl Pts',(-6.74400518266946,-0.557389537152904,
57.3290687516077));
#23441=CARTESIAN_POINT('Ctrl Pts',(-6.72868405709669,-0.742763935809257,
57.3378182264582));
#23442=CARTESIAN_POINT('Ctrl Pts',(-6.70571545653021,-0.927506129692905,
57.3465677013088));
#23443=CARTESIAN_POINT('Ctrl Pts',(-6.67517739415685,-1.11098863924764,
57.3553171761593));
#23444=CARTESIAN_POINT('Ctrl Pts',(-6.64463945823106,-1.29447038906471,
57.3640666147813));
#23445=CARTESIAN_POINT('Ctrl Pts',(-6.60653217027161,-1.47669218228203,
57.3728160534033));
#23446=CARTESIAN_POINT('Ctrl Pts',(-6.56098496116711,-1.65703510504124,
57.3815654920253));
#23447=CARTESIAN_POINT('Ctrl Pts',(-6.51543793687511,-1.83737729604043,
57.3903148951455));
#23448=CARTESIAN_POINT('Ctrl Pts',(-6.46245112202627,-2.01584035397095,
57.3990642982657));
#23449=CARTESIAN_POINT('Ctrl Pts',(-6.40220448416222,-2.19181813638204,
57.407813701386));
#23450=CARTESIAN_POINT('Ctrl Pts',(-6.34195808575158,-2.36779521936023,
57.4165630697313));
#23451=CARTESIAN_POINT('Ctrl Pts',(-6.27445201489196,-2.54128677544924,
57.4253124380765));
#23452=CARTESIAN_POINT('Ctrl Pts',(-6.19991555136134,-2.71170355237955,
57.4340618064218));
#23453=CARTESIAN_POINT('Ctrl Pts',(-6.12537937788983,-2.8821196661319,57.4428111407189));
#23454=CARTESIAN_POINT('Ctrl Pts',(-6.04381298133556,-3.04946076210566,
57.4515604750159));
#23455=CARTESIAN_POINT('Ctrl Pts',(-5.95549339426239,-3.21315848206979,
57.460309809313));
#23456=CARTESIAN_POINT('Ctrl Pts',(-5.86717414355093,-3.37685557859754,
57.4690591102886));
#23457=CARTESIAN_POINT('Ctrl Pts',(-5.7721018898617,-3.53690907467422,57.4778084112641));
#23458=CARTESIAN_POINT('Ctrl Pts',(-5.67059953467,-3.69277536785009,57.4865577122397));
#23459=CARTESIAN_POINT('Ctrl Pts',(-5.56909755761692,-3.84864108035899,
57.4953069806205));
#23460=CARTESIAN_POINT('Ctrl Pts',(-5.46116568337991,-4.00031938104388,
57.5040562490012));
#23461=CARTESIAN_POINT('Ctrl Pts',(-5.34717048686029,-4.14729511663328,
57.512805517382));
#23462=CARTESIAN_POINT('Ctrl Pts',(-5.23317570555419,-4.2942703168816,57.5215547538946));
#23463=CARTESIAN_POINT('Ctrl Pts',(-5.11311782178693,-4.43654275987259,
57.5303039904072));
#23464=CARTESIAN_POINT('Ctrl Pts',(-4.98740459171888,-4.57362924147787,
57.5390532269199));
#23465=CARTESIAN_POINT('Ctrl Pts',(-4.86169180910706,-4.71071523514563,
57.547802432291));
#23466=CARTESIAN_POINT('Ctrl Pts',(-4.73032391415311,-4.84261509316641,
57.5565516376621));
#23467=CARTESIAN_POINT('Ctrl Pts',(-4.59374707237177,-4.96888084331631,
57.5653008430332));
#23468=CARTESIAN_POINT('Ctrl Pts',(-4.45717070537292,-5.0951461545282,57.5740500179894));
#23469=CARTESIAN_POINT('Ctrl Pts',(-4.31538563819405,-5.21577720253718,
57.5827991929457));
#23470=CARTESIAN_POINT('Ctrl Pts',(-4.16887341290552,-5.33036429028725,
57.5915483679019));
#23471=CARTESIAN_POINT('Ctrl Pts',(-4.02236168477258,-5.44495098921236,
57.6002975131698));
#23472=CARTESIAN_POINT('Ctrl Pts',(-3.87112305634375,-5.55349359238803,
57.6090466584377));
#23473=CARTESIAN_POINT('Ctrl Pts',(-3.71567117316686,-5.65562346102504,
57.6177958037056));
#23474=CARTESIAN_POINT('Ctrl Pts',(-3.56021980457275,-5.75775299158784,
57.6265449200117));
#23475=CARTESIAN_POINT('Ctrl Pts',(-3.40055544862384,-5.85346967275354,
57.6352940363179));
#23476=CARTESIAN_POINT('Ctrl Pts',(-3.23722036323423,-5.94244842803551,
57.6440431526241));
#23477=CARTESIAN_POINT('Ctrl Pts',(-3.07388580496088,-6.03142689616454,
57.652792240695));
#23478=CARTESIAN_POINT('Ctrl Pts',(-2.90688079257771,-6.11366734484792,
57.6615413287659));
#23479=CARTESIAN_POINT('Ctrl Pts',(-2.73677251094701,-6.18889046787264,
57.6702904168368));
#23480=CARTESIAN_POINT('Ctrl Pts',(-2.56666476416755,-6.26411335438225,
57.6790394773991));
#23481=CARTESIAN_POINT('Ctrl Pts',(-2.39345402972227,-6.33231884350239,
57.6877885379613));
#23482=CARTESIAN_POINT('Ctrl Pts',(-2.21772856474196,-6.39327529620988,
57.6965375985235));
#23483=CARTESIAN_POINT('Ctrl Pts',(-2.04200363768462,-6.4542315623202,57.7052866323035));
#23484=CARTESIAN_POINT('Ctrl Pts',(-1.86376426620321,-6.5079387425199,57.7140356660835));
#23485=CARTESIAN_POINT('Ctrl Pts',(-1.68361578194952,-6.55421443796055,
57.7227846998635));
#23486=CARTESIAN_POINT('Ctrl Pts',(-1.50346783420109,-6.60048999558625,
57.7315337075877));
#23487=CARTESIAN_POINT('Ctrl Pts',(-1.32141106257464,-6.63933404145453,
57.7402827153119));
#23488=CARTESIAN_POINT('Ctrl Pts',(-1.13806375959237,-6.67061465526997,
57.7490317230362));
#23489=CARTESIAN_POINT('Ctrl Pts',(-0.954716987420905,-6.70189517852456,
57.7577807054311));
#23490=CARTESIAN_POINT('Ctrl Pts',(-0.770079973811447,-6.7256122653581,
57.766529687826));
#23491=CARTESIAN_POINT('Ctrl Pts',(-0.584779770553844,-6.7416853693977,
57.7752786702208));
#23492=CARTESIAN_POINT('Ctrl Pts',(-0.391490647555292,-6.75845143942386,
57.7844048508969));
#23493=CARTESIAN_POINT('Ctrl Pts',(-0.197480213105708,-6.76689975924022,
57.793531031573));
#23494=CARTESIAN_POINT('Ctrl Pts',(-0.00346532629915959,-6.76699911271707,
57.802657212249));
#23495=CARTESIAN_POINT('Ctrl Pts',(0.184486595294652,-6.76709536139777,
57.8114981997789));
#23496=CARTESIAN_POINT('Ctrl Pts',(0.372442378183787,-6.75935659726778,
57.8203391873089));
#23497=CARTESIAN_POINT('Ctrl Pts',(0.559750217720607,-6.74380965729029,
57.8291801748388));
#23498=CARTESIAN_POINT('Ctrl Pts',(0.745129914456277,-6.7284227571727,57.8379301534366));
#23499=CARTESIAN_POINT('Ctrl Pts',(0.929874656312708,-6.70538772273493,
57.8466801320343));
#23500=CARTESIAN_POINT('Ctrl Pts',(1.1133568828963,-6.67478280180767,57.8554301106321));
#23501=CARTESIAN_POINT('Ctrl Pts',(1.29683723118703,-6.64417819418053,57.864179999657));
#23502=CARTESIAN_POINT('Ctrl Pts',(1.47905480730076,-6.60600390230111,57.872929888682));
#23503=CARTESIAN_POINT('Ctrl Pts',(1.65939064804643,-6.56038959797176,57.8816797777069));
#23504=CARTESIAN_POINT('Ctrl Pts',(1.839724702641,-6.51477574543303,57.8904295800679));
#23505=CARTESIAN_POINT('Ctrl Pts',(2.01817678125683,-6.46172209820151,57.8991793824288));
#23506=CARTESIAN_POINT('Ctrl Pts',(2.19414072347515,-6.40140886724071,57.9079291847898));
#23507=CARTESIAN_POINT('Ctrl Pts',(2.37010298131935,-6.34109621361435,57.9166789033953));
#23508=CARTESIAN_POINT('Ctrl Pts',(2.54357687926754,-6.27352420826035,57.9254286220007));
#23509=CARTESIAN_POINT('Ctrl Pts',(2.71397317789815,-6.19892237325565,57.9341783406062));
#23510=CARTESIAN_POINT('Ctrl Pts',(2.88436790207039,-6.12432122757039,57.9429279783645));
#23511=CARTESIAN_POINT('Ctrl Pts',(3.0516848212609,-6.04269049717501,57.9516776161227));
#23512=CARTESIAN_POINT('Ctrl Pts',(3.21535561997218,-5.95430745235022,57.960427253881));
#23513=CARTESIAN_POINT('Ctrl Pts',(3.37902496075111,-5.86592519481614,57.9691768137));
#23514=CARTESIAN_POINT('Ctrl Pts',(3.53904799384707,-5.77079087940335,57.977926373519));
#23515=CARTESIAN_POINT('Ctrl Pts',(3.69488118814818,-5.66922763747132,57.986675933338));
#23516=CARTESIAN_POINT('Ctrl Pts',(3.85071304610672,-5.56766526649163,57.9954254181255));
#23517=CARTESIAN_POINT('Ctrl Pts',(4.00235489705812,-5.45967423580828,58.0041749029129));
#23518=CARTESIAN_POINT('Ctrl Pts',(4.14929168607503,-5.34562133936446,58.0129243877004));
#23519=CARTESIAN_POINT('Ctrl Pts',(4.29622726385604,-5.23156938308656,58.0216738003637));
#23520=CARTESIAN_POINT('Ctrl Pts',(4.43845763091913,-5.11145583677336,58.030423213027));
#23521=CARTESIAN_POINT('Ctrl Pts',(4.57549970660807,-4.98568866204353,58.0391726256903));
#23522=CARTESIAN_POINT('Ctrl Pts',(4.71254069815142,-4.8599224822631,58.0479219691366));
#23523=CARTESIAN_POINT('Ctrl Pts',(4.84439326931163,-4.72850295734157,58.0566713125829));
#23524=CARTESIAN_POINT('Ctrl Pts',(4.9706095943455,-4.59187644221842,58.0654206560292));
#23525=CARTESIAN_POINT('Ctrl Pts',(5.09682496280371,-4.45525096256828,58.0741699331655));
#23526=CARTESIAN_POINT('Ctrl Pts',(5.217403976157,-4.31341878218494,58.0829192103018));
#23527=CARTESIAN_POINT('Ctrl Pts',(5.331937104518,-4.16686161438848,58.0916684874381));
#23528=CARTESIAN_POINT('Ctrl Pts',(5.44646940289262,-4.02030550864678,58.1004177011711));
#23529=CARTESIAN_POINT('Ctrl Pts',(5.55495572749556,-3.8690247098029,58.1091669149041));
#23530=CARTESIAN_POINT('Ctrl Pts',(5.65702762491359,-3.71353301465929,58.117916128637));
#23531=CARTESIAN_POINT('Ctrl Pts',(5.75909881655059,-3.55804239467046,58.1266652818731));
#23532=CARTESIAN_POINT('Ctrl Pts',(5.8547555125069,-3.39834117619712,58.1354144351092));
#23533=CARTESIAN_POINT('Ctrl Pts',(5.94367283728005,-3.23497174692134,58.1441635883454));
#23534=CARTESIAN_POINT('Ctrl Pts',(6.03258957676231,-3.07160339301124,58.1529126839909));
#23535=CARTESIAN_POINT('Ctrl Pts',(6.11476689685213,-2.90456712829655,58.1616617796364));
#23536=CARTESIAN_POINT('Ctrl Pts',(6.18992570525198,-2.73443024476048,58.170410875282));
#23537=CARTESIAN_POINT('Ctrl Pts',(6.26508404388646,-2.56429442463157,58.179159916243));
#23538=CARTESIAN_POINT('Ctrl Pts',(6.33322384283274,-2.39105828656103,58.1879089572041));
#23539=CARTESIAN_POINT('Ctrl Pts',(6.39411368720001,-2.21531017132174,58.1966579981651));
#23540=CARTESIAN_POINT('Ctrl Pts',(6.45500317120857,-2.03956309619618,58.2054069873475));
#23541=CARTESIAN_POINT('Ctrl Pts',(6.5086426927004,-1.86130434438747,58.2141559765299));
#23542=CARTESIAN_POINT('Ctrl Pts',(6.55485008446302,-1.68113930720069,58.2229049657123));
#23543=CARTESIAN_POINT('Ctrl Pts',(6.60199664749377,-1.4973123921196,58.2318317792417));
#23544=CARTESIAN_POINT('Ctrl Pts',(6.64140563640884,-1.31150116499787,58.240758592771));
#23545=CARTESIAN_POINT('Ctrl Pts',(6.67293772282154,-1.12436255155771,58.2496854063004));
#23546=CARTESIAN_POINT('Ctrl Pts',(6.70384494949855,-0.940932395052457,
58.2584353204559));
#23547=CARTESIAN_POINT('Ctrl Pts',(6.72718449348918,-0.75622726050783,58.2671852346114));
#23548=CARTESIAN_POINT('Ctrl Pts',(6.74287707373923,-0.570874564542807,
58.275935148767));
#23549=CARTESIAN_POINT('Ctrl Pts',(6.75856934538664,-0.38552551363361,58.284684890851));
#23550=CARTESIAN_POINT('Ctrl Pts',(6.766614930041,-0.199529212419383,58.2934346329349));
#23551=CARTESIAN_POINT('Ctrl Pts',(6.76698649908906,-0.0135174386015994,
58.3021843750189));
#23552=CARTESIAN_POINT('Ctrl Pts',(6.76735806132392,0.172490924444619,58.3109339566648));
#23553=CARTESIAN_POINT('Ctrl Pts',(6.76005588896295,0.358514472900262,58.3196835383107));
#23554=CARTESIAN_POINT('Ctrl Pts',(6.74510478454594,0.543921359661082,58.3284331199566));
#23555=CARTESIAN_POINT('Ctrl Pts',(6.730153934407,0.729325093149309,58.3371825527956));
#23556=CARTESIAN_POINT('Ctrl Pts',(6.70755443556913,0.914111900255213,58.3459319856347));
#23557=CARTESIAN_POINT('Ctrl Pts',(6.67738304682337,1.09765415591424,58.3546814184737));
#23558=CARTESIAN_POINT('Ctrl Pts',(6.6472121311188,1.28119353391173,58.3634307141351));
#23559=CARTESIAN_POINT('Ctrl Pts',(6.60946960955513,1.46348811672568,58.3721800097964));
#23560=CARTESIAN_POINT('Ctrl Pts',(6.56428366991201,1.64391876348151,58.3809293054577));
#23561=CARTESIAN_POINT('Ctrl Pts',(6.51909837867738,1.82434682109643,58.3896784755686));
#23562=CARTESIAN_POINT('Ctrl Pts',(6.46646995271944,2.0029107182037,58.3984276456794));
#23563=CARTESIAN_POINT('Ctrl Pts',(6.40657713281575,2.17900400212627,58.4071768157902));
#23564=CARTESIAN_POINT('Ctrl Pts',(6.3466850927909,2.35509499309575,58.415925871976));
#23565=CARTESIAN_POINT('Ctrl Pts',(6.27952894037561,2.52871516398034,58.4246749281618));
#23566=CARTESIAN_POINT('Ctrl Pts',(6.20533675061488,2.69927486771325,58.4334239843475));
#23567=CARTESIAN_POINT('Ctrl Pts',(6.1283211790796,2.87632521635831,58.4425059856298));
#23568=CARTESIAN_POINT('Ctrl Pts',(6.04372366626125,3.05007728919907,58.4515879869121));
#23569=CARTESIAN_POINT('Ctrl Pts',(5.95185378007915,3.21989527478108,58.4606699881943));
#23570=CARTESIAN_POINT('Ctrl Pts',(5.8633445081742,3.38350129286667,58.4694197685015));
#23571=CARTESIAN_POINT('Ctrl Pts',(5.76808562057306,3.5434556712488,58.4781695488086));
#23572=CARTESIAN_POINT('Ctrl Pts',(5.66640068804536,3.6992150846523,58.4869193291157));
#23573=CARTESIAN_POINT('Ctrl Pts',(5.56471941107977,3.85496889852205,58.4956687948692));
#23574=CARTESIAN_POINT('Ctrl Pts',(5.4566127081517,4.0065278091956,58.5044182606227));
#23575=CARTESIAN_POINT('Ctrl Pts',(5.34244776449173,4.15337704569154,58.5131677263762));
#23576=CARTESIAN_POINT('Ctrl Pts',(5.22828631819657,4.30022178356175,58.5219169240958));
#23577=CARTESIAN_POINT('Ctrl Pts',(5.10806717844134,4.44235690972605,58.5306661218153));
#23578=CARTESIAN_POINT('Ctrl Pts',(4.98219864544787,4.57929969070571,58.5394153195349));
#23579=CARTESIAN_POINT('Ctrl Pts',(4.85633329944113,4.71623900429909,58.5481642957252));
#23580=CARTESIAN_POINT('Ctrl Pts',(4.72481904033758,4.84798602483508,58.5569132719154));
#23581=CARTESIAN_POINT('Ctrl Pts',(4.58810250737332,4.97409332259002,58.5656622481056));
#23582=CARTESIAN_POINT('Ctrl Pts',(4.45137708685774,5.1002088182202,58.5744117930418));
#23583=CARTESIAN_POINT('Ctrl Pts',(4.30944892636181,5.22068366307826,58.583161337978));
#23584=CARTESIAN_POINT('Ctrl Pts',(4.16280009466788,5.33510865604752,58.5919108829141));
#23585=CARTESIAN_POINT('Ctrl Pts',(4.01615988348915,5.44952692272799,58.6006599135224));
#23586=CARTESIAN_POINT('Ctrl Pts',(3.86479978232356,5.55789587288539,58.6094089441307));
#23587=CARTESIAN_POINT('Ctrl Pts',(3.70923383581191,5.65984746713797,58.618157974739));
#23588=CARTESIAN_POINT('Ctrl Pts',(3.55366577799659,5.7618004450531,58.626907124087));
#23589=CARTESIAN_POINT('Ctrl Pts',(3.39389200026952,5.85733573570994,58.635656273435));
#23590=CARTESIAN_POINT('Ctrl Pts',(3.23045513626147,5.9461288762187,58.6444054227831));
#23591=CARTESIAN_POINT('Ctrl Pts',(3.18695122151651,5.9697639920665,58.6467342868961));
#23592=CARTESIAN_POINT('Ctrl Pts',(3.14318791262702,5.99292165435313,58.649063151009));
#23593=CARTESIAN_POINT('Ctrl Pts',(3.09917575053262,6.01559628526637,58.651392015122));
#23594=CARTESIAN_POINT('Origin',(0.,0.,-3.69717978381041));
#23595=CARTESIAN_POINT('',(3.09917575053255,6.01559628526641,61.0455262068868));
#23596=CARTESIAN_POINT('',(3.09917575053261,6.01559628526638,60.6511868721373));
#23597=CARTESIAN_POINT('',(3.09917575053259,6.01559628526639,-3.69717978381041));
#23598=CARTESIAN_POINT('',(-6.76765222831417,-0.00200817279939102,59.6960497532493));
#23599=CARTESIAN_POINT('Ctrl Pts',(-6.76699734633338,-0.0059928888702975,
59.69717978381));
#23600=CARTESIAN_POINT('Ctrl Pts',(-6.76681265505105,-0.214540960501165,
59.7069683551803));
#23601=CARTESIAN_POINT('Ctrl Pts',(-6.75698359187389,-0.422659502131963,
59.7167569265505));
#23602=CARTESIAN_POINT('Ctrl Pts',(-6.73765166604857,-0.629554625900658,
59.7265454979208));
#23603=CARTESIAN_POINT('Ctrl Pts',(-6.71817163684709,-0.838034789184822,
59.736409060292));
#23604=CARTESIAN_POINT('Ctrl Pts',(-6.6890426811903,-1.04527270412106,59.7462726226633));
#23605=CARTESIAN_POINT('Ctrl Pts',(-6.65045814561019,-1.25047808996683,
59.7561361850345));
#23606=CARTESIAN_POINT('Ctrl Pts',(-6.61153030721492,-1.45750927429865,
59.766087507662));
#23607=CARTESIAN_POINT('Ctrl Pts',(-6.56297792934071,-1.66247158939489,
59.7760388302894));
#23608=CARTESIAN_POINT('Ctrl Pts',(-6.50504769461876,-1.86457595467043,
59.7859901529169));
#23609=CARTESIAN_POINT('Ctrl Pts',(-6.47109324051564,-1.98303470816466,
59.7918228882587));
#23610=CARTESIAN_POINT('Ctrl Pts',(-6.43391797308779,-2.10051205147262,
59.7976556236004));
#23611=CARTESIAN_POINT('Ctrl Pts',(-6.39357906915677,-2.21685265329938,
59.8034883589422));
#23612=CARTESIAN_POINT('Ctrl Pts',(-6.33718716150031,-2.37949139247111,
59.8116422511089));
#23613=CARTESIAN_POINT('Ctrl Pts',(-6.27449306449052,-2.54024340953854,
59.8197961432757));
#23614=CARTESIAN_POINT('Ctrl Pts',(-6.20563962095389,-2.69857849521693,
59.8279500354424));
#23615=CARTESIAN_POINT('Ctrl Pts',(-6.13687019785494,-2.85672036785448,
59.8360939775826));
#23616=CARTESIAN_POINT('Ctrl Pts',(-6.06195653347624,-3.01245084821206,
59.8442379197229));
#23617=CARTESIAN_POINT('Ctrl Pts',(-5.98109130842289,-3.16525445427506,
59.8523818618631));
#23618=CARTESIAN_POINT('Ctrl Pts',(-5.90030774101968,-3.31790375935895,
59.860517580256));
#23619=CARTESIAN_POINT('Ctrl Pts',(-5.81358474718157,-3.46763175332366,
59.8686532986489));
#23620=CARTESIAN_POINT('Ctrl Pts',(-5.72116319629874,-3.61394253984714,
59.8767890170418));
#23621=CARTESIAN_POINT('Ctrl Pts',(-5.6288155317408,-3.76013635834526,59.884918231342));
#23622=CARTESIAN_POINT('Ctrl Pts',(-5.53077857539011,-3.90291810117333,
59.8930474456422));
#23623=CARTESIAN_POINT('Ctrl Pts',(-5.42733925560266,-4.04181612701448,
59.9011766599424));
#23624=CARTESIAN_POINT('Ctrl Pts',(-5.32396088088463,-4.18063231598893,
59.9093010846179));
#23625=CARTESIAN_POINT('Ctrl Pts',(-5.21518669939534,-4.31556905237643,
59.9174255092933));
#23626=CARTESIAN_POINT('Ctrl Pts',(-5.10134710952039,-4.44618338220411,
59.9255499339687));
#23627=CARTESIAN_POINT('Ctrl Pts',(-4.98681644045892,-4.5775906246284,59.9337236791029));
#23628=CARTESIAN_POINT('Ctrl Pts',(-4.86715886167765,-4.70462249188359,
59.9418974242371));
#23629=CARTESIAN_POINT('Ctrl Pts',(-4.7427525719935,-4.82686099249285,59.9500711693713));
#23630=CARTESIAN_POINT('Ctrl Pts',(-4.61914294378451,-4.94831671351384,
59.9581925722334));
#23631=CARTESIAN_POINT('Ctrl Pts',(-4.49084552583913,-5.06504003602356,
59.9663139750956));
#23632=CARTESIAN_POINT('Ctrl Pts',(-4.35826863593558,-5.17665756033951,
59.9744353779577));
#23633=CARTESIAN_POINT('Ctrl Pts',(-4.22568149588488,-5.28828371433481,
59.982557408724));
#23634=CARTESIAN_POINT('Ctrl Pts',(-4.08881450476893,-5.39480304807199,
59.9906794394903));
#23635=CARTESIAN_POINT('Ctrl Pts',(-3.94810925875312,-5.49588230231943,
59.9988014702565));
#23636=CARTESIAN_POINT('Ctrl Pts',(-3.80736634062081,-5.59698861930653,
60.0069256755977));
#23637=CARTESIAN_POINT('Ctrl Pts',(-3.66278341847713,-5.69265174318178,
60.0150498809388));
#23638=CARTESIAN_POINT('Ctrl Pts',(-3.51483122164988,-5.78258164519233,
60.0231740862799));
#23639=CARTESIAN_POINT('Ctrl Pts',(-3.36527754466686,-5.87348497616553,
60.0313862305223));
#23640=CARTESIAN_POINT('Ctrl Pts',(-3.21228155414851,-5.95853004384766,
60.0395983747647));
#23641=CARTESIAN_POINT('Ctrl Pts',(-3.05635434741772,-6.03746528793507,
60.0478105190072));
#23642=CARTESIAN_POINT('Ctrl Pts',(-2.90185058423,-6.11567994024203,60.0559476954236));
#23643=CARTESIAN_POINT('Ctrl Pts',(-2.74446925827017,-6.18789576148942,
60.0640848718401));
#23644=CARTESIAN_POINT('Ctrl Pts',(-2.58472673772144,-6.25391690793121,
60.0722220482565));
#23645=CARTESIAN_POINT('Ctrl Pts',(-2.42277665483177,-6.32085043384523,
60.0804716764119));
#23646=CARTESIAN_POINT('Ctrl Pts',(-2.25840000661337,-6.38141668080218,
60.0887213045673));
#23647=CARTESIAN_POINT('Ctrl Pts',(-2.09214928617978,-6.43546426952535,
60.0969709327227));
#23648=CARTESIAN_POINT('Ctrl Pts',(-1.92589856574613,-6.48951185824855,
60.1052205608782));
#23649=CARTESIAN_POINT('Ctrl Pts',(-1.75777416057214,-6.53704074493859,
60.1134701890336));
#23650=CARTESIAN_POINT('Ctrl Pts',(-1.58833733130281,-6.57795359682553,
60.121719817189));
#23651=CARTESIAN_POINT('Ctrl Pts',(-1.41940905063369,-6.61874365266129,
60.1299446848666));
#23652=CARTESIAN_POINT('Ctrl Pts',(-1.24867130851606,-6.65307942640394,
60.1381695525442));
#23653=CARTESIAN_POINT('Ctrl Pts',(-1.07665842662517,-6.68080052331882,
60.1463944202218));
#23654=CARTESIAN_POINT('Ctrl Pts',(-0.904839336499182,-6.7084903893152,
60.1546100216653));
#23655=CARTESIAN_POINT('Ctrl Pts',(-0.731748318183226,-6.72958036109917,
60.1628256231089));
#23656=CARTESIAN_POINT('Ctrl Pts',(-0.557933309136579,-6.74396021804369,
60.1710412245524));
#23657=CARTESIAN_POINT('Ctrl Pts',(-0.384279199229741,-6.75832676367162,
60.1792492208806));
#23658=CARTESIAN_POINT('Ctrl Pts',(-0.209902788589785,-6.76599553539176,
60.1874572172087));
#23659=CARTESIAN_POINT('Ctrl Pts',(-0.0353607199741979,-6.76690761127141,
60.1956652135368));
#23660=CARTESIAN_POINT('Ctrl Pts',(0.139054834150475,-6.76781902604502,
60.2038672604083));
#23661=CARTESIAN_POINT('Ctrl Pts',(0.313635449772633,-6.76198349800724,
60.2120693072797));
#23662=CARTESIAN_POINT('Ctrl Pts',(0.487820776911681,-6.74939403869809,
60.2202713541511));
#23663=CARTESIAN_POINT('Ctrl Pts',(0.661914826112078,-6.73681117661452,
60.2284691029227));
#23664=CARTESIAN_POINT('Ctrl Pts',(0.835613642499457,-6.71748145980735,
60.2366668516943));
#23665=CARTESIAN_POINT('Ctrl Pts',(1.00835820546982,-6.69144997212575,60.2448646004659));
#23666=CARTESIAN_POINT('Ctrl Pts',(1.18106982088387,-6.66542344942765,60.2530607856815));
#23667=CARTESIAN_POINT('Ctrl Pts',(1.35282719007815,-6.63269774918149,60.2612569708971));
#23668=CARTESIAN_POINT('Ctrl Pts',(1.52307742835258,-6.59336971109939,60.2694531561128));
#23669=CARTESIAN_POINT('Ctrl Pts',(1.69331507189868,-6.55404458241679,60.2776487349931));
#23670=CARTESIAN_POINT('Ctrl Pts',(1.86204545674993,-6.5081181685023,60.2858443138735));
#23671=CARTESIAN_POINT('Ctrl Pts',(2.02872694719519,-6.45573822066261,60.2940398927538));
#23672=CARTESIAN_POINT('Ctrl Pts',(2.19542643264329,-6.40335261786204,60.3022363564323));
#23673=CARTESIAN_POINT('Ctrl Pts',(2.36007624059371,-6.34451220064319,60.3104328201107));
#23674=CARTESIAN_POINT('Ctrl Pts',(2.52215087996938,-6.27941429901465,60.3186292837891));
#23675=CARTESIAN_POINT('Ctrl Pts',(2.68427250467484,-6.21429752554788,60.3268281236169));
#23676=CARTESIAN_POINT('Ctrl Pts',(2.84381714090245,-6.14291978804291,60.3350269634447));
#23677=CARTESIAN_POINT('Ctrl Pts',(3.00028018016918,-6.06552618001802,60.3432258032725));
#23678=CARTESIAN_POINT('Ctrl Pts',(3.15690664953161,-5.9880517321678,60.3514332070217));
#23679=CARTESIAN_POINT('Ctrl Pts',(3.31044476909495,-5.9045490189965,60.359640610771));
#23680=CARTESIAN_POINT('Ctrl Pts',(3.46041453008442,-5.81530913021661,60.3678480145202));
#23681=CARTESIAN_POINT('Ctrl Pts',(3.61046462281412,-5.7260214398298,60.3760598145893));
#23682=CARTESIAN_POINT('Ctrl Pts',(3.7569422457987,-5.63099064257468,60.3842716146583));
#23683=CARTESIAN_POINT('Ctrl Pts',(3.89939731408626,-5.53055056815294,60.3924834147273));
#23684=CARTESIAN_POINT('Ctrl Pts',(4.04206209613958,-5.42996263190717,60.4007073037134));
#23685=CARTESIAN_POINT('Ctrl Pts',(4.18069220397646,-5.32394972221459,60.4089311926996));
#23686=CARTESIAN_POINT('Ctrl Pts',(4.31487051633804,-5.2128860938291,60.4171550816857));
#23687=CARTESIAN_POINT('Ctrl Pts',(4.43884895730922,-5.11026522124924,60.4247538129358));
#23688=CARTESIAN_POINT('Ctrl Pts',(4.55902693142482,-5.0033329036962,60.4323525441859));
#23689=CARTESIAN_POINT('Ctrl Pts',(4.67510465874965,-4.8924110037626,60.439951275436));
#23690=CARTESIAN_POINT('Ctrl Pts',(4.80074690998782,-4.77234940761958,60.448176123758));
#23691=CARTESIAN_POINT('Ctrl Pts',(4.92193756477516,-4.64727625819529,60.45640097208));
#23692=CARTESIAN_POINT('Ctrl Pts',(5.03825283089154,-4.5175543618216,60.4646258204021));
#23693=CARTESIAN_POINT('Ctrl Pts',(5.15443710022891,-4.3879785610651,60.4728414057213));
#23694=CARTESIAN_POINT('Ctrl Pts',(5.26575667708866,-4.25376470329733,60.4810569910405));
#23695=CARTESIAN_POINT('Ctrl Pts',(5.37182261935113,-4.11531417345354,60.4892725763597));
#23696=CARTESIAN_POINT('Ctrl Pts',(5.47779041860503,-3.97699175213588,60.4974805597829));
#23697=CARTESIAN_POINT('Ctrl Pts',(5.5785140476264,-3.83444074891005,60.5056885432062));
#23698=CARTESIAN_POINT('Ctrl Pts',(5.67364301506104,-3.68809760413809,60.5138965266294));
#23699=CARTESIAN_POINT('Ctrl Pts',(5.76870306662689,-3.54186047717789,60.5220985638059));
#23700=CARTESIAN_POINT('Ctrl Pts',(5.85817633474329,-3.39183698016989,60.5303006009824));
#23701=CARTESIAN_POINT('Ctrl Pts',(5.94175401476835,-3.23849474725283,60.538502638159));
#23702=CARTESIAN_POINT('Ctrl Pts',(6.02528793035647,-3.08523281013342,60.5467003804384));
#23703=CARTESIAN_POINT('Ctrl Pts',(6.10293223666537,-2.92865591338539,60.5548981227178));
#23704=CARTESIAN_POINT('Ctrl Pts',(6.17442265531003,-2.76925872276215,60.5630958649972));
#23705=CARTESIAN_POINT('Ctrl Pts',(6.24589948123463,-2.60989183887696,60.5712920486115));
#23706=CARTESIAN_POINT('Ctrl Pts',(6.31122459774818,-2.44770605369602,60.5794882322259));
#23707=CARTESIAN_POINT('Ctrl Pts',(6.37018058473801,-2.28321885018212,60.5876844158402));
#23708=CARTESIAN_POINT('Ctrl Pts',(6.42913223174462,-2.11874375522138,60.5958799961011));
#23709=CARTESIAN_POINT('Ctrl Pts',(6.48171556105628,-1.95196791680613,60.604075576362));
#23710=CARTESIAN_POINT('Ctrl Pts',(6.52776206483786,-1.7834268767919,60.6122711566229));
#23711=CARTESIAN_POINT('Ctrl Pts',(6.57381355657095,-1.61486757970135,60.6204676246636));
#23712=CARTESIAN_POINT('Ctrl Pts',(6.61332671744159,-1.44454304626998,60.6286640927043));
#23713=CARTESIAN_POINT('Ctrl Pts',(6.64618347708717,-1.27300203805553,60.636860560745));
#23714=CARTESIAN_POINT('Ctrl Pts',(6.67904977383951,-1.1014112378066,60.6450594079184));
#23715=CARTESIAN_POINT('Ctrl Pts',(6.70525575336807,-0.928603611784166,
60.6532582550918));
#23716=CARTESIAN_POINT('Ctrl Pts',(6.72473481698215,-0.755136173989895,
60.6614571022652));
#23717=CARTESIAN_POINT('Ctrl Pts',(6.74423423811189,-0.581487445854731,
60.6696645180311));
#23718=CARTESIAN_POINT('Ctrl Pts',(6.75699265764824,-0.407177885348716,
60.6778719337971));
#23719=CARTESIAN_POINT('Ctrl Pts',(6.76299547117577,-0.232768676707155,
60.6860793495631));
#23720=CARTESIAN_POINT('Ctrl Pts',(6.76900150200023,-0.0582659908640812,
60.6942911642152));
#23721=CARTESIAN_POINT('Ctrl Pts',(6.76824471028132,0.116336091098023,60.7025029788674));
#23722=CARTESIAN_POINT('Ctrl Pts',(6.76076262469402,0.29047845452012,60.7107147935195));
#23723=CARTESIAN_POINT('Ctrl Pts',(6.75326952059825,0.464877269046196,60.7189387013171));
#23724=CARTESIAN_POINT('Ctrl Pts',(6.73903135900979,0.638814654417665,60.7271626091147));
#23725=CARTESIAN_POINT('Ctrl Pts',(6.71813749751791,0.811737374058775,60.7353865169123));
#23726=CARTESIAN_POINT('Ctrl Pts',(6.69883195537331,0.971514773420187,60.7429852558358));
#23727=CARTESIAN_POINT('Ctrl Pts',(6.67384477093599,1.1304257897702,60.7505839947593));
#23728=CARTESIAN_POINT('Ctrl Pts',(6.64328465932267,1.28804422874686,60.7581827336827));
#23729=CARTESIAN_POINT('Ctrl Pts',(6.61050133861164,1.45712920789633,60.7663342711601));
#23730=CARTESIAN_POINT('Ctrl Pts',(6.57120696873145,1.62522739997276,60.7744858086374));
#23731=CARTESIAN_POINT('Ctrl Pts',(6.5254704576766,1.79179360027598,60.7826373461148));
#23732=CARTESIAN_POINT('Ctrl Pts',(6.4797877416664,1.95816388628719,60.7907792957964));
#23733=CARTESIAN_POINT('Ctrl Pts',(6.42767806415106,2.12300541842217,60.7989212454781));
#23734=CARTESIAN_POINT('Ctrl Pts',(6.36926173053051,2.28578083113835,60.8070631951598));
#23735=CARTESIAN_POINT('Ctrl Pts',(6.31090181179256,2.4483990454268,60.8151972818499));
#23736=CARTESIAN_POINT('Ctrl Pts',(6.24624748588144,2.60895477103907,60.8233313685401));
#23737=CARTESIAN_POINT('Ctrl Pts',(6.17546947516548,2.76692351923566,60.8314654552303));
#23738=CARTESIAN_POINT('Ctrl Pts',(6.10474493038905,2.92477293732599,60.8395933974049));
#23739=CARTESIAN_POINT('Ctrl Pts',(6.02790606129483,3.08003893707896,60.8477213395795));
#23740=CARTESIAN_POINT('Ctrl Pts',(5.94517252486965,3.23221482106852,60.8558492817541));
#23741=CARTESIAN_POINT('Ctrl Pts',(5.86248222417664,3.38431117943829,60.8639729763461));
#23742=CARTESIAN_POINT('Ctrl Pts',(5.77390356492504,3.53332031724075,60.8720966709381));
#23743=CARTESIAN_POINT('Ctrl Pts',(5.67970318818474,3.67875803690921,60.8802203655301));
#23744=CARTESIAN_POINT('Ctrl Pts',(5.58552832753847,3.82415636180389,60.8883418596536));
#23745=CARTESIAN_POINT('Ctrl Pts',(5.48573497913876,3.96598488739328,60.8964633537772));
#23746=CARTESIAN_POINT('Ctrl Pts',(5.38063437906526,4.10378638318577,60.9045848479008));
#23747=CARTESIAN_POINT('Ctrl Pts',(5.27554223581709,4.24157679090475,60.9127056885356));
#23748=CARTESIAN_POINT('Ctrl Pts',(5.16514391309833,4.37534052320748,60.9208265291705));
#23749=CARTESIAN_POINT('Ctrl Pts',(5.04979236142588,4.50465160767011,60.9289473698053));
#23750=CARTESIAN_POINT('Ctrl Pts',(4.93442812738708,4.63397690928476,60.9370691032888));
#23751=CARTESIAN_POINT('Ctrl Pts',(4.81410982419634,4.75884831586788,60.9451908367723));
#23752=CARTESIAN_POINT('Ctrl Pts',(4.68922881402648,4.87887508855308,60.9533125702557));
#23753=CARTESIAN_POINT('Ctrl Pts',(4.56425269415373,4.99899327394125,60.9614404892726));
#23754=CARTESIAN_POINT('Ctrl Pts',(4.43470718941319,5.11425920068743,60.9695684082895));
#23755=CARTESIAN_POINT('Ctrl Pts',(4.30101898063026,5.22432050397544,60.9776963273064));
#23756=CARTESIAN_POINT('Ctrl Pts',(4.16727776249131,5.33442544820131,60.9858274691636));
#23757=CARTESIAN_POINT('Ctrl Pts',(4.02939085683188,5.43932143362197,60.9939586110208));
#23758=CARTESIAN_POINT('Ctrl Pts',(3.88781555167283,5.53869833410079,61.002089752878));
#23759=CARTESIAN_POINT('Ctrl Pts',(3.74607089457628,5.63819410891734,61.0102306211817));
#23760=CARTESIAN_POINT('Ctrl Pts',(3.60062932981021,5.73215740947761,61.0183714894854));
#23761=CARTESIAN_POINT('Ctrl Pts',(3.45197527296536,5.82032264697033,61.0265123577891));
#23762=CARTESIAN_POINT('Ctrl Pts',(3.33624290883387,5.88896235708532,61.0328503074883));
#23763=CARTESIAN_POINT('Ctrl Pts',(3.21856396001261,5.95408865972539,61.0391882571876));
#23764=CARTESIAN_POINT('Ctrl Pts',(3.09917575053255,6.01559628526641,61.0455262068868));
#23765=CARTESIAN_POINT('Ctrl Pts',(3.09917575053261,6.01559628526638,59.0457515827422));
#23766=CARTESIAN_POINT('Ctrl Pts',(2.93382384459273,6.10078395293755,59.0545010306546));
#23767=CARTESIAN_POINT('Ctrl Pts',(2.76495772122997,6.17915010267043,59.063250478567));
#23768=CARTESIAN_POINT('Ctrl Pts',(2.5931509331673,6.25042856433169,59.0719999264794));
#23769=CARTESIAN_POINT('Ctrl Pts',(2.42134553245641,6.32170645041442,59.0807493037394));
#23770=CARTESIAN_POINT('Ctrl Pts',(2.24659977927619,6.38589665313447,59.0894986809994));
#23771=CARTESIAN_POINT('Ctrl Pts',(2.06950718689952,6.44278115439065,59.0982480582594));
#23772=CARTESIAN_POINT('Ctrl Pts',(1.89241596572899,6.49966521519713,59.1069973677741));
#23773=CARTESIAN_POINT('Ctrl Pts',(1.7129782145724,6.54924360009535,59.1157466772888));
#23774=CARTESIAN_POINT('Ctrl Pts',(1.53180337335892,6.59134792173545,59.1244959868034));
#23775=CARTESIAN_POINT('Ctrl Pts',(1.35062987477835,6.63345193135294,59.1332452314795));
#23776=CARTESIAN_POINT('Ctrl Pts',(1.1677195910301,6.66808192368227,59.1419944761557));
#23777=CARTESIAN_POINT('Ctrl Pts',(0.983693746907481,6.69512028363159,59.1507437208318));
#23778=CARTESIAN_POINT('Ctrl Pts',(0.799669205420618,6.72215845218858,59.1594929035759));
#23779=CARTESIAN_POINT('Ctrl Pts',(0.614529402874333,6.74160505424571,59.1682420863201));
#23780=CARTESIAN_POINT('Ctrl Pts',(0.428903127364216,6.75339404354116,59.1769912690643));
#23781=CARTESIAN_POINT('Ctrl Pts',(0.243278104164918,6.76518295330326,59.1857403927829));
#23782=CARTESIAN_POINT('Ctrl Pts',(0.0571669005402259,6.76931433552275,
59.1944895165015));
#23783=CARTESIAN_POINT('Ctrl Pts',(-0.128798404776336,6.76577415902475,
59.2032386402201));
#23784=CARTESIAN_POINT('Ctrl Pts',(-0.314762517257839,6.76223400523447,
59.2119877078193));
#23785=CARTESIAN_POINT('Ctrl Pts',(-0.50058044681817,6.75102239665099,59.2207367754185));
#23786=CARTESIAN_POINT('Ctrl Pts',(-0.685621118841192,6.73217741012512,
59.2294858430177));
#23787=CARTESIAN_POINT('Ctrl Pts',(-0.870660665413108,6.7133325382179,59.2382348574035));
#23788=CARTESIAN_POINT('Ctrl Pts',(-1.05492267885353,6.68685441030633,59.2469838717893));
#23789=CARTESIAN_POINT('Ctrl Pts',(-1.23778137635122,6.65283295028201,59.2557328861751));
#23790=CARTESIAN_POINT('Ctrl Pts',(-1.42999922978717,6.61707018861893,59.2649296965425));
#23791=CARTESIAN_POINT('Ctrl Pts',(-1.62066601233565,6.57297172934445,59.2741265069099));
#23792=CARTESIAN_POINT('Ctrl Pts',(-1.80906628500255,6.5207030431133,59.2833233172772));
#23793=CARTESIAN_POINT('Ctrl Pts',(-1.98831342545394,6.47097374915072,59.292073315015));
#23794=CARTESIAN_POINT('Ctrl Pts',(-2.16550875896565,6.41384933989575,59.3008233127528));
#23795=CARTESIAN_POINT('Ctrl Pts',(-2.34005036713871,6.34952386240527,59.3095733104905));
#23796=CARTESIAN_POINT('Ctrl Pts',(-2.51458843546951,6.28519968948651,59.3183231307714));
#23797=CARTESIAN_POINT('Ctrl Pts',(-2.68647261717919,6.21367483971158,59.3270729510523));
#23798=CARTESIAN_POINT('Ctrl Pts',(-2.85511905908597,6.13519226743906,59.3358227713331));
#23799=CARTESIAN_POINT('Ctrl Pts',(-3.02376230488747,6.05671118253005,59.3445724257917));
#23800=CARTESIAN_POINT('Ctrl Pts',(-3.18916767379764,5.97127275992708,59.3533220802502));
#23801=CARTESIAN_POINT('Ctrl Pts',(-3.35077334102644,5.87916720438078,59.3620717347087));
#23802=CARTESIAN_POINT('Ctrl Pts',(-3.51237616037225,5.7870632719573,59.3708212349771));
#23803=CARTESIAN_POINT('Ctrl Pts',(-3.67017916302158,5.6882925836239,59.3795707352456));
#23804=CARTESIAN_POINT('Ctrl Pts',(-3.82364636566321,5.58319061741139,59.388320235514));
#23805=CARTESIAN_POINT('Ctrl Pts',(-3.97711106778666,5.47809036367798,59.3970695932225));
#23806=CARTESIAN_POINT('Ctrl Pts',(-4.12623987481805,5.36665920043319,59.4058189509309));
#23807=CARTESIAN_POINT('Ctrl Pts',(-4.27052628213816,5.24927559512427,59.4145683086394));
#23808=CARTESIAN_POINT('Ctrl Pts',(-4.4148105302487,5.1318937464313,59.4233175354159));
#23809=CARTESIAN_POINT('Ctrl Pts',(-4.55425230136426,5.00855981477448,59.4320667621924));
#23810=CARTESIAN_POINT('Ctrl Pts',(-4.68837800630449,4.87969268192172,59.4408159889689));
#23811=CARTESIAN_POINT('Ctrl Pts',(-4.82250188228786,4.75082730631919,59.4495650964398));
#23812=CARTESIAN_POINT('Ctrl Pts',(-4.95130963052849,4.6164290790365,59.4583142039106));
#23813=CARTESIAN_POINT('Ctrl Pts',(-5.07436379033244,4.47695444731829,59.4670633113814));
#23814=CARTESIAN_POINT('Ctrl Pts',(-5.19741643562668,4.33748153220749,59.4758123111712));
#23815=CARTESIAN_POINT('Ctrl Pts',(-5.31471544462624,4.19293255254776,59.4845613109609));
#23816=CARTESIAN_POINT('Ctrl Pts',(-5.42586245275469,4.04379841779816,59.4933103107506));
#23817=CARTESIAN_POINT('Ctrl Pts',(-5.53702160019002,3.89464799484558,59.5020602660928));
#23818=CARTESIAN_POINT('Ctrl Pts',(-5.64202723081108,3.74091164444066,59.510810221435));
#23819=CARTESIAN_POINT('Ctrl Pts',(-5.74052265232831,3.5831115916345,59.5195601767771));
#23820=CARTESIAN_POINT('Ctrl Pts',(-5.83901427066792,3.42531763191999,59.5283097942596));
#23821=CARTESIAN_POINT('Ctrl Pts',(-5.93099603115622,3.26346052695826,59.537059411742));
#23822=CARTESIAN_POINT('Ctrl Pts',(-6.01615550622645,3.09809004467287,59.5458090292245));
#23823=CARTESIAN_POINT('Ctrl Pts',(-6.10131214578696,2.93272506864043,59.5545583553756));
#23824=CARTESIAN_POINT('Ctrl Pts',(-6.17964682328649,2.76384720417114,59.5633076815266));
#23825=CARTESIAN_POINT('Ctrl Pts',(-6.25089348288471,2.59203002791816,59.5720570076777));
#23826=CARTESIAN_POINT('Ctrl Pts',(-6.32213814889247,2.42021765937248,59.5808060890093));
#23827=CARTESIAN_POINT('Ctrl Pts',(-6.3862950841251,2.24546640832132,59.5895551703409));
#23828=CARTESIAN_POINT('Ctrl Pts',(-6.44314639819745,2.0683697666025,59.5983042516725));
#23829=CARTESIAN_POINT('Ctrl Pts',(-6.50000285283642,1.89125711158476,59.6070541241069));
#23830=CARTESIAN_POINT('Ctrl Pts',(-6.54955227673199,1.71179891440447,59.6158039965413));
#23831=CARTESIAN_POINT('Ctrl Pts',(-6.59162635926342,1.53060476278615,59.6245538689757));
#23832=CARTESIAN_POINT('Ctrl Pts',(-6.63369752055164,1.34942319164859,59.6333031338982));
#23833=CARTESIAN_POINT('Ctrl Pts',(-6.6682943142423,1.16650618642847,59.6420523988207));
#23834=CARTESIAN_POINT('Ctrl Pts',(-6.695299237454,0.98247499761977,59.6508016637432));
#23835=CARTESIAN_POINT('Ctrl Pts',(-6.7223055473143,0.798434359178909,59.6595513779229));
#23836=CARTESIAN_POINT('Ctrl Pts',(-6.74171916496693,0.613279706241456,
59.6683010921026));
#23837=CARTESIAN_POINT('Ctrl Pts',(-6.75347414817268,0.427639953656448,
59.6770508062823));
#23838=CARTESIAN_POINT('Ctrl Pts',(-6.7624883775874,0.285283364199705,59.6837604654582));
#23839=CARTESIAN_POINT('Ctrl Pts',(-6.76699999999994,0.142641701106312,
59.6904701246341));
#23840=CARTESIAN_POINT('Ctrl Pts',(-6.767,2.82448417516006E-12,59.69717978381));
#23841=CARTESIAN_POINT('',(-6.76699904389988,-0.00254360543768349,59.3028202161898));
#23842=CARTESIAN_POINT('Ctrl Pts',(3.09917575053262,6.01559628526637,58.651392015122));
#23843=CARTESIAN_POINT('Ctrl Pts',(2.93382384459268,6.10078395293758,58.6601414630344));
#23844=CARTESIAN_POINT('Ctrl Pts',(2.76495772122987,6.17915010267048,58.6688909109468));
#23845=CARTESIAN_POINT('Ctrl Pts',(2.59315093316714,6.25042856433176,58.6776403588593));
#23846=CARTESIAN_POINT('Ctrl Pts',(2.42134553245624,6.32170645041448,58.6863897361193));
#23847=CARTESIAN_POINT('Ctrl Pts',(2.24659977927602,6.38589665313453,58.6951391133793));
#23848=CARTESIAN_POINT('Ctrl Pts',(2.06950718689935,6.4427811543907,58.7038884906393));
#23849=CARTESIAN_POINT('Ctrl Pts',(1.89241596572876,6.4996652151972,58.7126378001539));
#23850=CARTESIAN_POINT('Ctrl Pts',(1.7129782145721,6.54924360009543,58.7213871096686));
#23851=CARTESIAN_POINT('Ctrl Pts',(1.53180337335855,6.59134792173554,58.7301364191833));
#23852=CARTESIAN_POINT('Ctrl Pts',(1.35062987477805,6.633451931353,58.7388856638594));
#23853=CARTESIAN_POINT('Ctrl Pts',(1.16771959102986,6.66808192368232,58.7476349085355));
#23854=CARTESIAN_POINT('Ctrl Pts',(0.983693746907299,6.69512028363162,58.7563841532116));
#23855=CARTESIAN_POINT('Ctrl Pts',(0.799669205420246,6.72215845218863,58.7651333359558));
#23856=CARTESIAN_POINT('Ctrl Pts',(0.614529402873771,6.74160505424577,58.7738825186999));
#23857=CARTESIAN_POINT('Ctrl Pts',(0.428903127363461,6.75339404354121,58.7826317014441));
#23858=CARTESIAN_POINT('Ctrl Pts',(0.243278104164161,6.76518295330329,58.7913808251627));
#23859=CARTESIAN_POINT('Ctrl Pts',(0.0571669005394668,6.76931433552275,
58.8001299488813));
#23860=CARTESIAN_POINT('Ctrl Pts',(-0.128798404777095,6.76577415902474,
58.8088790726));
#23861=CARTESIAN_POINT('Ctrl Pts',(-0.314762517258661,6.76223400523443,
58.8176281401992));
#23862=CARTESIAN_POINT('Ctrl Pts',(-0.500580446819053,6.75102239665092,
58.8263772077984));
#23863=CARTESIAN_POINT('Ctrl Pts',(-0.685621118842137,6.73217741012502,
58.8351262753976));
#23864=CARTESIAN_POINT('Ctrl Pts',(-0.870660665413986,6.71333253821778,
58.8438752897834));
#23865=CARTESIAN_POINT('Ctrl Pts',(-1.05492267885434,6.6868544103062,58.8526243041691));
#23866=CARTESIAN_POINT('Ctrl Pts',(-1.23778137635196,6.65283295028188,58.8613733185549));
#23867=CARTESIAN_POINT('Ctrl Pts',(-1.42999922978791,6.61707018861877,58.8705701289223));
#23868=CARTESIAN_POINT('Ctrl Pts',(-1.62066601233639,6.57297172934427,58.8797669392897));
#23869=CARTESIAN_POINT('Ctrl Pts',(-1.80906628500328,6.5207030431131,58.8889637496571));
#23870=CARTESIAN_POINT('Ctrl Pts',(-1.98831342545466,6.47097374915049,58.8977137473948));
#23871=CARTESIAN_POINT('Ctrl Pts',(-2.16550875896637,6.4138493398955,58.9064637451326));
#23872=CARTESIAN_POINT('Ctrl Pts',(-2.34005036713942,6.34952386240501,58.9152137428704));
#23873=CARTESIAN_POINT('Ctrl Pts',(-2.51458843547009,6.28519968948628,58.9239635631512));
#23874=CARTESIAN_POINT('Ctrl Pts',(-2.68647261717965,6.21367483971138,58.9327133834321));
#23875=CARTESIAN_POINT('Ctrl Pts',(-2.85511905908631,6.1351922674389,58.9414632037129));
#23876=CARTESIAN_POINT('Ctrl Pts',(-3.02376230488786,6.05671118252986,58.9502128581715));
#23877=CARTESIAN_POINT('Ctrl Pts',(-3.18916767379808,5.97127275992684,58.95896251263));
#23878=CARTESIAN_POINT('Ctrl Pts',(-3.35077334102693,5.8791672043805,58.9677121670885));
#23879=CARTESIAN_POINT('Ctrl Pts',(-3.51237616037285,5.78706327195694,58.976461667357));
#23880=CARTESIAN_POINT('Ctrl Pts',(-3.67017916302227,5.68829258362346,58.9852111676254));
#23881=CARTESIAN_POINT('Ctrl Pts',(-3.823646365664,5.58319061741085,58.9939606678939));
#23882=CARTESIAN_POINT('Ctrl Pts',(-3.97711106778738,5.47809036367745,59.0027100256023));
#23883=CARTESIAN_POINT('Ctrl Pts',(-4.1262398748187,5.36665920043269,59.0114593833108));
#23884=CARTESIAN_POINT('Ctrl Pts',(-4.27052628213875,5.24927559512379,59.0202087410192));
#23885=CARTESIAN_POINT('Ctrl Pts',(-4.41481053024922,5.13189374643084,59.0289579677957));
#23886=CARTESIAN_POINT('Ctrl Pts',(-4.55425230136473,5.00855981477405,59.0377071945722));
#23887=CARTESIAN_POINT('Ctrl Pts',(-4.68837800630489,4.87969268192133,59.0464564213487));
#23888=CARTESIAN_POINT('Ctrl Pts',(-4.82250188228821,4.75082730631883,59.0552055288196));
#23889=CARTESIAN_POINT('Ctrl Pts',(-4.95130963052879,4.61642907903618,59.0639546362904));
#23890=CARTESIAN_POINT('Ctrl Pts',(-5.07436379033269,4.47695444731801,59.0727037437613));
#23891=CARTESIAN_POINT('Ctrl Pts',(-5.19741643562739,4.33748153220667,59.081452743551));
#23892=CARTESIAN_POINT('Ctrl Pts',(-5.31471544462736,4.19293255254638,59.0902017433408));
#23893=CARTESIAN_POINT('Ctrl Pts',(-5.42586245275617,4.04379841779617,59.0989507431306));
#23894=CARTESIAN_POINT('Ctrl Pts',(-5.53702160019137,3.89464799484365,59.1077006984727));
#23895=CARTESIAN_POINT('Ctrl Pts',(-5.64202723081231,3.7409116444388,59.1164506538149));
#23896=CARTESIAN_POINT('Ctrl Pts',(-5.74052265232942,3.58311159163272,59.125200609157));
#23897=CARTESIAN_POINT('Ctrl Pts',(-5.83901427066901,3.42531763191812,59.1339502266395));
#23898=CARTESIAN_POINT('Ctrl Pts',(-5.9309960311573,3.26346052695631,59.1426998441219));
#23899=CARTESIAN_POINT('Ctrl Pts',(-6.0161555062275,3.09809004467083,59.1514494616044));
#23900=CARTESIAN_POINT('Ctrl Pts',(-6.10131214578804,2.93272506863819,59.1601987877555));
#23901=CARTESIAN_POINT('Ctrl Pts',(-6.17964682328759,2.76384720416869,59.1689481139066));
#23902=CARTESIAN_POINT('Ctrl Pts',(-6.25089348288581,2.59203002791551,59.1776974400577));
#23903=CARTESIAN_POINT('Ctrl Pts',(-6.32213814889339,2.42021765937003,59.1864465213892));
#23904=CARTESIAN_POINT('Ctrl Pts',(-6.38629508412587,2.24546640831909,59.1951956027208));
#23905=CARTESIAN_POINT('Ctrl Pts',(-6.44314639819809,2.0683697666005,59.2039446840524));
#23906=CARTESIAN_POINT('Ctrl Pts',(-6.50000285283701,1.89125711158275,59.2126945564868));
#23907=CARTESIAN_POINT('Ctrl Pts',(-6.54955227673252,1.71179891440244,59.2214444289212));
#23908=CARTESIAN_POINT('Ctrl Pts',(-6.5916263592639,1.5306047627841,59.2301943013556));
#23909=CARTESIAN_POINT('Ctrl Pts',(-6.63369752055203,1.34942319164666,59.2389435662781));
#23910=CARTESIAN_POINT('Ctrl Pts',(-6.66829431424261,1.16650618642665,59.2476928312006));
#23911=CARTESIAN_POINT('Ctrl Pts',(-6.69529923745424,0.982474997618072,
59.2564420961231));
#23912=CARTESIAN_POINT('Ctrl Pts',(-6.7223055473145,0.798434359177204,59.2651918103028));
#23913=CARTESIAN_POINT('Ctrl Pts',(-6.74171916496709,0.613279706239749,
59.2739415244825));
#23914=CARTESIAN_POINT('Ctrl Pts',(-6.75347414817279,0.427639953654739,
59.2826912386622));
#23915=CARTESIAN_POINT('Ctrl Pts',(-6.76248837758744,0.285283364198505,
59.289400897838));
#23916=CARTESIAN_POINT('Ctrl Pts',(-6.76699999999995,0.142641701105622,
59.2961105570139));
#23917=CARTESIAN_POINT('Ctrl Pts',(-6.767,2.6471802258598E-12,59.3028202161898));
#23918=CARTESIAN_POINT('Ctrl Pts',(-6.76699808779975,-0.00508721087801415,
59.3028202161898));
#23919=CARTESIAN_POINT('Ctrl Pts',(-6.76685389172481,-0.196896551357745,
59.3117968853725));
#23920=CARTESIAN_POINT('Ctrl Pts',(-6.75855052427745,-0.388401106019233,
59.3207735545552));
#23921=CARTESIAN_POINT('Ctrl Pts',(-6.74218962523088,-0.578937006442967,
59.3297502237379));
#23922=CARTESIAN_POINT('Ctrl Pts',(-6.72574110339922,-0.770493345059413,
59.3387749685644));
#23923=CARTESIAN_POINT('Ctrl Pts',(-6.70114859654504,-0.961070402327572,
59.3477997133909));
#23924=CARTESIAN_POINT('Ctrl Pts',(-6.66856551188544,-1.15001000590954,
59.3568244582174));
#23925=CARTESIAN_POINT('Ctrl Pts',(-6.63589346638885,-1.33946546688962,
59.3658738430944));
#23926=CARTESIAN_POINT('Ctrl Pts',(-6.59518726618906,-1.52727431190146,
59.3749232279714));
#23927=CARTESIAN_POINT('Ctrl Pts',(-6.54665030744605,-1.71279267630867,
59.3839726128485));
#23928=CARTESIAN_POINT('Ctrl Pts',(-6.49792014969984,-1.89904948754086,
59.3930580183618));
#23929=CARTESIAN_POINT('Ctrl Pts',(-6.44129688469831,-2.08299734195364,
59.4021434238751));
#23930=CARTESIAN_POINT('Ctrl Pts',(-6.37703367310896,-2.26400762631985,
59.4112288293884));
#23931=CARTESIAN_POINT('Ctrl Pts',(-6.3346927207129,-2.38326945037125,59.4172149093372));
#23932=CARTESIAN_POINT('Ctrl Pts',(-6.28903618429288,-2.50125653358099,
59.423200989286));
#23933=CARTESIAN_POINT('Ctrl Pts',(-6.24014724426247,-2.61779513520891,
59.4291870692348));
#23934=CARTESIAN_POINT('Ctrl Pts',(-6.17290706410859,-2.7780783518929,59.4374201193668));
#23935=CARTESIAN_POINT('Ctrl Pts',(-6.09938911658582,-2.9360035466864,59.4456531694988));
#23936=CARTESIAN_POINT('Ctrl Pts',(-6.01977864578517,-3.09104416916823,
59.4538862196308));
#23937=CARTESIAN_POINT('Ctrl Pts',(-5.94026297881782,-3.24590016210093,
59.4621094654656));
#23938=CARTESIAN_POINT('Ctrl Pts',(-5.85466939759303,-3.39787810731453,
59.4703327113005));
#23939=CARTESIAN_POINT('Ctrl Pts',(-5.76323171819324,-3.54646995791751,
59.4785559571353));
#23940=CARTESIAN_POINT('Ctrl Pts',(-5.67188462556532,-3.69491459944695,
59.4867710562488));
#23941=CARTESIAN_POINT('Ctrl Pts',(-5.57470515147535,-3.83997952410623,
59.4949861553623));
#23942=CARTESIAN_POINT('Ctrl Pts',(-5.47197370948423,-3.98117981542073,
59.5032012544759));
#23943=CARTESIAN_POINT('Ctrl Pts',(-5.36932348843731,-4.12226847176974,
59.5114098586148));
#23944=CARTESIAN_POINT('Ctrl Pts',(-5.26113025220341,-4.25949829225545,
59.5196184627536));
#23945=CARTESIAN_POINT('Ctrl Pts',(-5.14771859082211,-4.39241190118874,
59.5278270668925));
#23946=CARTESIAN_POINT('Ctrl Pts',(-5.03437390882547,-4.5252470131524,59.5360308231415));
#23947=CARTESIAN_POINT('Ctrl Pts',(-4.91581717317682,-4.6537707199673,59.5442345793905));
#23948=CARTESIAN_POINT('Ctrl Pts',(-4.79241430671134,-4.77755733747158,
59.5524383356394));
#23949=CARTESIAN_POINT('Ctrl Pts',(-4.66904795204328,-4.90130732963617,
59.5606396646037));
#23950=CARTESIAN_POINT('Ctrl Pts',(-4.54083857255589,-5.02032276832821,
59.568840993568));
#23951=CARTESIAN_POINT('Ctrl Pts',(-4.4081903020088,-5.13421340238946,59.5770423225322));
#23952=CARTESIAN_POINT('Ctrl Pts',(-4.27556032492461,-5.24808832984497,
59.5852425204549));
#23953=CARTESIAN_POINT('Ctrl Pts',(-4.13849294721889,-5.35683962636661,
59.5934427183777));
#23954=CARTESIAN_POINT('Ctrl Pts',(-3.99742687846337,-5.46011605658145,
59.6016429163004));
#23955=CARTESIAN_POINT('Ctrl Pts',(-3.85635470002368,-5.56339695978102,
59.6098434693802));
#23956=CARTESIAN_POINT('Ctrl Pts',(-3.71128377457562,-5.66120231256384,
59.6180440224601));
#23957=CARTESIAN_POINT('Ctrl Pts',(-3.56268344058216,-5.75322307078404,
59.6262445755399));
#23958=CARTESIAN_POINT('Ctrl Pts',(-3.41404974129794,-5.84526449046085,
59.6344469698931));
#23959=CARTESIAN_POINT('Ctrl Pts',(-3.26188535965923,-5.93151854010717,
59.6426493642463));
#23960=CARTESIAN_POINT('Ctrl Pts',(-3.10668601908128,-6.01172113282418,
59.6508517585995));
#23961=CARTESIAN_POINT('Ctrl Pts',(-2.95134153983737,-6.09199872906422,
59.6590618236333));
#23962=CARTESIAN_POINT('Ctrl Pts',(-2.79295674983463,-6.16621339711428,
59.6672718886672));
#23963=CARTESIAN_POINT('Ctrl Pts',(-2.63205008647175,-6.23414800452348,
59.675481953701));
#23964=CARTESIAN_POINT('Ctrl Pts',(-2.47106641603435,-6.30211512423059,
59.6836959479263));
#23965=CARTESIAN_POINT('Ctrl Pts',(-2.30755880086754,-6.3637960643812,59.6919099421516));
#23966=CARTESIAN_POINT('Ctrl Pts',(-2.14206271716062,-6.41902300321089,
59.7001239363769));
#23967=CARTESIAN_POINT('Ctrl Pts',(-1.97634100717147,-6.47432523475208,
59.7083491290121));
#23968=CARTESIAN_POINT('Ctrl Pts',(-1.80862575487906,-6.52315577996311,
59.7165743216473));
#23969=CARTESIAN_POINT('Ctrl Pts',(-1.6394657449671,-6.56539725158192,59.7247995142825));
#23970=CARTESIAN_POINT('Ctrl Pts',(-1.48734051036217,-6.60338491653545,
59.7321964124025));
#23971=CARTESIAN_POINT('Ctrl Pts',(-1.33404717200257,-6.63604440680909,
59.7395933105225));
#23972=CARTESIAN_POINT('Ctrl Pts',(-1.17998895555638,-6.66332612624994,
59.7469902086425));
#23973=CARTESIAN_POINT('Ctrl Pts',(-0.999915882299108,-6.69521474067624,
59.7556361751334));
#23974=CARTESIAN_POINT('Ctrl Pts',(-0.818389007109079,-6.71982792700986,
59.7642821416243));
#23975=CARTESIAN_POINT('Ctrl Pts',(-0.636008931829445,-6.73704546805446,
59.7729281081152));
#23976=CARTESIAN_POINT('Ctrl Pts',(-0.453862145459705,-6.75424098552343,
59.7815630152395));
#23977=CARTESIAN_POINT('Ctrl Pts',(-0.270864637381904,-6.76405969304869,
59.7901979223639));
#23978=CARTESIAN_POINT('Ctrl Pts',(-0.0876255804028921,-6.76643264635503,
59.7988328294883));
#23979=CARTESIAN_POINT('Ctrl Pts',(0.101696865371653,-6.76888437979587,
59.8077544085598));
#23980=CARTESIAN_POINT('Ctrl Pts',(0.291276863503035,-6.76338739230685,
59.8166759876313));
#23981=CARTESIAN_POINT('Ctrl Pts',(0.480435422154191,-6.74992376291314,
59.8255975667027));
#23982=CARTESIAN_POINT('Ctrl Pts',(0.663010220993306,-6.7369287419861,59.8342086256784));
#23983=CARTESIAN_POINT('Ctrl Pts',(0.845192075588722,-6.71651228279546,
59.8428196846541));
#23984=CARTESIAN_POINT('Ctrl Pts',(1.02636874057709,-6.68871110217553,59.8514307436298));
#23985=CARTESIAN_POINT('Ctrl Pts',(1.20737454760633,-6.66093613935238,59.8600336819794));
#23986=CARTESIAN_POINT('Ctrl Pts',(1.38737675453623,-6.62579038585825,59.868636620329));
#23987=CARTESIAN_POINT('Ctrl Pts',(1.56576778775354,-6.58336238064057,59.8772395586785));
#23988=CARTESIAN_POINT('Ctrl Pts',(1.7439590642814,-6.54098188497372,59.8858328637273));
#23989=CARTESIAN_POINT('Ctrl Pts',(1.92054247025903,-6.4913354758701,59.894426168776));
#23990=CARTESIAN_POINT('Ctrl Pts',(2.09491996763691,-6.4345628700943,59.9030194738248));
#23991=CARTESIAN_POINT('Ctrl Pts',(2.11434847511248,-6.42823747253837,59.9039769086652));
#23992=CARTESIAN_POINT('Ctrl Pts',(2.13374960972759,-6.4218236654166,59.9049343435057));
#23993=CARTESIAN_POINT('Ctrl Pts',(2.15312255267417,-6.41532168119151,59.9058917783461));
#23994=CARTESIAN_POINT('Ctrl Pts',(2.32705096379606,-6.35694749465068,59.9144875358937));
#23995=CARTESIAN_POINT('Ctrl Pts',(2.49850201340885,-6.29153030270548,59.9230832934413));
#23996=CARTESIAN_POINT('Ctrl Pts',(2.66691143544978,-6.21931446346518,59.9316790509889));
#23997=CARTESIAN_POINT('Ctrl Pts',(2.83547798920735,-6.14703124439156,59.9402828286705));
#23998=CARTESIAN_POINT('Ctrl Pts',(3.00099697016294,-6.06793683674931,59.9488866063521));
#23999=CARTESIAN_POINT('Ctrl Pts',(3.16292726653382,-5.982322300463,59.9574903840337));
#24000=CARTESIAN_POINT('Ctrl Pts',(3.33122156515136,-5.89334303803536,59.9664322977018));
#24001=CARTESIAN_POINT('Ctrl Pts',(3.49563907118009,-5.79732097715773,59.9753742113698));
#24002=CARTESIAN_POINT('Ctrl Pts',(3.65560508503817,-5.69463260116428,59.9843161250378));
#24003=CARTESIAN_POINT('Ctrl Pts',(3.80994108277038,-5.59555835043932,59.9929433273685));
#24004=CARTESIAN_POINT('Ctrl Pts',(3.9601333743541,-5.49027924038039,60.0015705296993));
#24005=CARTESIAN_POINT('Ctrl Pts',(4.10569899548884,-5.37917510018422,60.01019773203));
#24006=CARTESIAN_POINT('Ctrl Pts',(4.2514032455969,-5.26796515030053,60.0188331504504));
#24007=CARTESIAN_POINT('Ctrl Pts',(4.39247179358532,-5.15091928931802,60.0274685688709));
#24008=CARTESIAN_POINT('Ctrl Pts',(4.52845631495592,-5.02845626445491,60.0361039872913));
#24009=CARTESIAN_POINT('Ctrl Pts',(4.66464173408752,-4.90581231791593,60.0447521633124));
#24010=CARTESIAN_POINT('Ctrl Pts',(4.7957278961417,-4.77773542460653,60.0534003393336));
#24011=CARTESIAN_POINT('Ctrl Pts',(4.92130370304089,-4.64468070618811,60.0620485153547));
#24012=CARTESIAN_POINT('Ctrl Pts',(4.93458914726629,-4.63060402148169,60.0629634595865));
#24013=CARTESIAN_POINT('Ctrl Pts',(4.94781295268266,-4.61647165060833,60.0638784038184));
#24014=CARTESIAN_POINT('Ctrl Pts',(4.96097465947815,-4.60228415333252,60.0647933480502));
#24015=CARTESIAN_POINT('Ctrl Pts',(5.07930766619511,-4.47472856829164,60.0730193405916));
#24016=CARTESIAN_POINT('Ctrl Pts',(5.19287330028552,-4.34243880531907,60.0812453331329));
#24017=CARTESIAN_POINT('Ctrl Pts',(5.30127216306996,-4.20580580306076,60.0894713256743));
#24018=CARTESIAN_POINT('Ctrl Pts',(5.40955738365779,-4.06931604284492,60.0976886943257));
#24019=CARTESIAN_POINT('Ctrl Pts',(5.51268639872425,-3.92849238907775,60.1059060629771));
#24020=CARTESIAN_POINT('Ctrl Pts',(5.61029721093421,-3.78376191177297,60.1141234316285));
#24021=CARTESIAN_POINT('Ctrl Pts',(5.7078252223249,-3.639154205725,60.1223338296909));
#24022=CARTESIAN_POINT('Ctrl Pts',(5.79984415439632,-3.49064657191445,60.1305442277533));
#24023=CARTESIAN_POINT('Ctrl Pts',(5.88603275743845,-3.33869845574014,60.1387546258157));
#24024=CARTESIAN_POINT('Ctrl Pts',(5.97216548994621,-3.18684883776797,60.1469597016045));
#24025=CARTESIAN_POINT('Ctrl Pts',(6.05247524563156,-3.03156349044571,60.1551647773933));
#24026=CARTESIAN_POINT('Ctrl Pts',(6.12668448284336,-2.87333016684238,60.163369853182));
#24027=CARTESIAN_POINT('Ctrl Pts',(6.20086045672258,-2.71516776928363,60.1715712511515));
#24028=CARTESIAN_POINT('Ctrl Pts',(6.26894120819666,-2.55406035175253,60.179772649121));
#24029=CARTESIAN_POINT('Ctrl Pts',(6.33069544938897,-2.39051963536923,60.1879740470905));
#24030=CARTESIAN_POINT('Ctrl Pts',(6.39244485347498,-2.22699172885638,60.1961748026582));
#24031=CARTESIAN_POINT('Ctrl Pts',(6.44786859971942,-2.06103123497598,60.2043755582259));
#24032=CARTESIAN_POINT('Ctrl Pts',(6.49678367114102,-1.89316954613037,60.2125763137936));
#24033=CARTESIAN_POINT('Ctrl Pts',(6.54569849409731,-1.72530870994231,60.2207770277054));
#24034=CARTESIAN_POINT('Ctrl Pts',(6.5881046068,-1.55554704178981,60.2289777416172));
#24035=CARTESIAN_POINT('Ctrl Pts',(6.62386901663486,-1.38443065931981,60.237178455529));
#24036=CARTESIAN_POINT('Ctrl Pts',(6.65963972620516,-1.2132841354902,60.2453806139586));
#24037=CARTESIAN_POINT('Ctrl Pts',(6.6887663287528,-1.04078277271815,60.2535827723882));
#24038=CARTESIAN_POINT('Ctrl Pts',(6.71116704694042,-0.86748248861922,60.2617849308178));
#24039=CARTESIAN_POINT('Ctrl Pts',(6.73357577052176,-0.694120271818259,
60.2699900204707));
#24040=CARTESIAN_POINT('Ctrl Pts',(6.74925377563276,-0.519958920123828,
60.2781951101237));
#24041=CARTESIAN_POINT('Ctrl Pts',(6.75817119392634,-0.345559131820007,
60.2864001997766));
#24042=CARTESIAN_POINT('Ctrl Pts',(6.76709879931602,-0.170960112377284,
60.2946146627744));
#24043=CARTESIAN_POINT('Ctrl Pts',(6.76925037003157,0.00387752958574603,
60.3028291257722));
#24044=CARTESIAN_POINT('Ctrl Pts',(6.76464819222189,0.17839236381944,60.31104358877));
#24045=CARTESIAN_POINT('Ctrl Pts',(6.76004328776732,0.353010592576657,60.3192629185774));
#24046=CARTESIAN_POINT('Ctrl Pts',(6.74867668177691,0.527305275350919,60.3274822483849));
#24047=CARTESIAN_POINT('Ctrl Pts',(6.73062253549272,0.700720546807031,60.3357015781924));
#24048=CARTESIAN_POINT('Ctrl Pts',(6.71254041540346,0.874404514712382,60.343933643353));
#24049=CARTESIAN_POINT('Ctrl Pts',(6.68775009868203,1.04720599381189,60.3521657085137));
#24050=CARTESIAN_POINT('Ctrl Pts',(6.65637706510546,1.2185784205943,60.3603977736744));
#24051=CARTESIAN_POINT('Ctrl Pts',(6.62817672981943,1.37262026300166,60.3677973449355));
#24052=CARTESIAN_POINT('Ctrl Pts',(6.59465848349134,1.5255074604202,60.3751969161967));
#24053=CARTESIAN_POINT('Ctrl Pts',(6.55594747915721,1.67685468974871,60.3825964874578));
#24054=CARTESIAN_POINT('Ctrl Pts',(6.51327697742987,1.84368224489941,60.3907529128389));
#24055=CARTESIAN_POINT('Ctrl Pts',(6.46416488242527,2.00915214045401,60.3989093382201));
#24056=CARTESIAN_POINT('Ctrl Pts',(6.40870973227483,2.17272376694459,60.4070657636012));
#24057=CARTESIAN_POINT('Ctrl Pts',(6.35332336696102,2.33609250429729,60.415212072007));
#24058=CARTESIAN_POINT('Ctrl Pts',(6.29160972490991,2.49756731724697,60.4233583804128));
#24059=CARTESIAN_POINT('Ctrl Pts',(6.22371824315168,2.65661819422004,60.4315046888185));
#24060=CARTESIAN_POINT('Ctrl Pts',(6.15589669331968,2.81550524012171,60.4396426060827));
#24061=CARTESIAN_POINT('Ctrl Pts',(6.08191011608718,2.97197298738088,60.4477805233468));
#24062=CARTESIAN_POINT('Ctrl Pts',(6.00195759739385,3.12550699872618,60.455918440611));
#24063=CARTESIAN_POINT('Ctrl Pts',(5.92202210112849,3.27900832164973,60.4640546252579));
#24064=CARTESIAN_POINT('Ctrl Pts',(5.83612332874608,3.42957681351207,60.4721908099048));
#24065=CARTESIAN_POINT('Ctrl Pts',(5.74450873561673,3.57671754356186,60.4803269945518));
#24066=CARTESIAN_POINT('Ctrl Pts',(5.65300859758315,3.72367444911626,60.4884530145758));
#24067=CARTESIAN_POINT('Ctrl Pts',(5.55580708295737,3.86721182911656,60.4965790345998));
#24068=CARTESIAN_POINT('Ctrl Pts',(5.45319686416382,4.00686073637129,60.5047050546238));
#24069=CARTESIAN_POINT('Ctrl Pts',(5.35062109290156,4.14646276174468,60.5128283466414));
#24070=CARTESIAN_POINT('Ctrl Pts',(5.24264044877855,4.28217861910984,60.5209516386591));
#24071=CARTESIAN_POINT('Ctrl Pts',(5.12959067261962,4.41356868433853,60.5290749306768));
#24072=CARTESIAN_POINT('Ctrl Pts',(5.01655734279137,4.54493963511576,60.5371970409287));
#24073=CARTESIAN_POINT('Ctrl Pts',(4.898456588398,4.67198577034943,60.5453191511807));
#24074=CARTESIAN_POINT('Ctrl Pts',(4.77566411355636,4.79430091613886,60.5534412614327));
#24075=CARTESIAN_POINT('Ctrl Pts',(4.65251851601471,4.91696781194059,60.5615867289914));
#24076=CARTESIAN_POINT('Ctrl Pts',(4.52465442212268,5.03487619368594,60.5697321965501));
#24077=CARTESIAN_POINT('Ctrl Pts',(4.39248754888795,5.14765404168387,60.5778776641088));
#24078=CARTESIAN_POINT('Ctrl Pts',(4.26062336331425,5.26017360663259,60.586004476974));
#24079=CARTESIAN_POINT('Ctrl Pts',(4.12447638791394,5.36758590235807,60.5941312898391));
#24080=CARTESIAN_POINT('Ctrl Pts',(3.98449184794063,5.46956247918375,60.6022581027042));
#24081=CARTESIAN_POINT('Ctrl Pts',(3.84402531667306,5.57189017922817,60.6104128976098));
#24082=CARTESIAN_POINT('Ctrl Pts',(3.69969504955309,5.66874444752584,60.6185676925152));
#24083=CARTESIAN_POINT('Ctrl Pts',(3.55197900450941,5.75983803170926,60.6267224874208));
#24084=CARTESIAN_POINT('Ctrl Pts',(3.40426295946573,5.85093161589267,60.6348772823263));
#24085=CARTESIAN_POINT('Ctrl Pts',(3.25316147405337,5.93626436243895,60.6430320772318));
#24086=CARTESIAN_POINT('Ctrl Pts',(3.0991757505326,6.01559628526638,60.6511868721373));
#24087=CARTESIAN_POINT('Origin',(0.,0.,-3.69717978381041));
#24088=CARTESIAN_POINT('',(3.09917575053259,6.01559628526639,63.0459622914914));
#24089=CARTESIAN_POINT('',(3.09917575053255,6.01559628526641,62.6516502284592));
#24090=CARTESIAN_POINT('',(3.09917575053259,6.01559628526639,-3.69717978381041));
#24091=CARTESIAN_POINT('',(-6.76699995039181,-0.000819388301575002,61.6971797837649));
#24092=CARTESIAN_POINT('Ctrl Pts',(-6.7669999503917,-0.000819389256966134,
61.69717978381));
#24093=CARTESIAN_POINT('Ctrl Pts',(-6.76698654599217,-0.11152082960351,
61.7024122253477));
#24094=CARTESIAN_POINT('Ctrl Pts',(-6.76425673829185,-0.222188623443844,
61.7076446668854));
#24095=CARTESIAN_POINT('Ctrl Pts',(-6.75881518896444,-0.332725474563706,
61.712877108423));
#24096=CARTESIAN_POINT('Ctrl Pts',(-6.75026182071719,-0.506474224346479,
61.7211017879418));
#24097=CARTESIAN_POINT('Ctrl Pts',(-6.73499304333732,-0.68012191140438,
61.7293264674606));
#24098=CARTESIAN_POINT('Ctrl Pts',(-6.71300920765678,-0.853109827581033,
61.7375511469794));
#24099=CARTESIAN_POINT('Ctrl Pts',(-6.69104847947462,-1.02591591388727,
61.7457671814295));
#24100=CARTESIAN_POINT('Ctrl Pts',(-6.66238679335155,-1.19806325767366,
61.7539832158797));
#24101=CARTESIAN_POINT('Ctrl Pts',(-6.62707648148646,-1.36899463422218,
61.7621992503298));
#24102=CARTESIAN_POINT('Ctrl Pts',(-6.59179621203621,-1.53978058041187,
61.7704082944844));
#24103=CARTESIAN_POINT('Ctrl Pts',(-6.54987865498482,-1.70935227077692,
61.778617338639));
#24104=CARTESIAN_POINT('Ctrl Pts',(-6.50142777761176,-1.87715898434261,
61.7868263827936));
#24105=CARTESIAN_POINT('Ctrl Pts',(-6.45300842074125,-2.04485652853454,
61.7950300864217));
#24106=CARTESIAN_POINT('Ctrl Pts',(-6.3980643089523,-2.21079103998572,61.8032337900497));
#24107=CARTESIAN_POINT('Ctrl Pts',(-6.33675020530368,-2.37442326378086,
61.8114374936778));
#24108=CARTESIAN_POINT('Ctrl Pts',(-6.27546371518033,-2.53798179388603,
61.8196375026718));
#24109=CARTESIAN_POINT('Ctrl Pts',(-6.20781307413923,-2.69923976711647,
61.8278375116657));
#24110=CARTESIAN_POINT('Ctrl Pts',(-6.13400251700446,-2.85767425039716,
61.8360375206597));
#24111=CARTESIAN_POINT('Ctrl Pts',(-6.06019786191762,-3.01609606492218,
61.8442368739637));
#24112=CARTESIAN_POINT('Ctrl Pts',(-5.98023441516054,-3.17169451087125,
61.8524362272676));
#24113=CARTESIAN_POINT('Ctrl Pts',(-5.89436422029642,-3.32396742440256,
61.8606355805715));
#24114=CARTESIAN_POINT('Ctrl Pts',(-5.80849458528061,-3.47623934515944,
61.8688348804181));
#24115=CARTESIAN_POINT('Ctrl Pts',(-5.71671845402208,-3.62518546386789,
61.8770341802647));
#24116=CARTESIAN_POINT('Ctrl Pts',(-5.61933336673632,-3.77032909882994,
61.8852334801113));
#24117=CARTESIAN_POINT('Ctrl Pts',(-5.52193124776209,-3.91549811797806,
61.8934342139343));
#24118=CARTESIAN_POINT('Ctrl Pts',(-5.41891841813569,-4.05686303072718,
61.9016349477573));
#24119=CARTESIAN_POINT('Ctrl Pts',(-5.31063522389015,-4.19397693350563,
61.9098356815803));
#24120=CARTESIAN_POINT('Ctrl Pts',(-5.20231344813795,-4.33113969022664,
61.9180393373403));
#24121=CARTESIAN_POINT('Ctrl Pts',(-5.08871778906956,-4.46404813854992,
61.9262429931003));
#24122=CARTESIAN_POINT('Ctrl Pts',(-4.97022829260731,-4.59228915894523,
61.9344466488602));
#24123=CARTESIAN_POINT('Ctrl Pts',(-4.85160305880967,-4.72067708767348,
61.9426597024353));
#24124=CARTESIAN_POINT('Ctrl Pts',(-4.72807303084948,-4.84438664272941,
61.9508727560103));
#24125=CARTESIAN_POINT('Ctrl Pts',(-4.60005523419539,-4.96304149109713,
61.9590858095853));
#24126=CARTESIAN_POINT('Ctrl Pts',(-4.47196168653879,-5.08176655020079,
61.9673037230084));
#24127=CARTESIAN_POINT('Ctrl Pts',(-4.33937534849418,-5.19543070751279,
61.9755216364315));
#24128=CARTESIAN_POINT('Ctrl Pts',(-4.20274552019563,-5.30369862383559,
61.9837395498546));
#24129=CARTESIAN_POINT('Ctrl Pts',(-4.06590259545257,-5.4121354015872,61.9919702804505));
#24130=CARTESIAN_POINT('Ctrl Pts',(-3.92500386664062,-5.51515890747701,
62.0002010110466));
#24131=CARTESIAN_POINT('Ctrl Pts',(-3.78052786042997,-5.61247700186939,
62.0084317416425));
#24132=CARTESIAN_POINT('Ctrl Pts',(-3.6478439277254,-5.70185203254728,62.0159906833184));
#24133=CARTESIAN_POINT('Ctrl Pts',(-3.51214333222039,-5.78641540611171,
62.0235496249942));
#24134=CARTESIAN_POINT('Ctrl Pts',(-3.37381337021396,-5.86597582188723,
62.0311085666701));
#24135=CARTESIAN_POINT('Ctrl Pts',(-3.2245957095948,-5.95179829264999,62.0392624588368));
#24136=CARTESIAN_POINT('Ctrl Pts',(-3.07185677620594,-6.0320639703605,62.0474163510036));
#24137=CARTESIAN_POINT('Ctrl Pts',(-2.91605207173513,-6.10646618879768,
62.0555702431703));
#24138=CARTESIAN_POINT('Ctrl Pts',(-2.76043749253325,-6.18077761574151,
62.0637141853105));
#24139=CARTESIAN_POINT('Ctrl Pts',(-2.60176491531566,-6.24923966991835,
62.0718581274507));
#24140=CARTESIAN_POINT('Ctrl Pts',(-2.44051781454467,-6.31158948260184,
62.0800020695909));
#24141=CARTESIAN_POINT('Ctrl Pts',(-2.27943354098797,-6.37387633448626,
62.0881377879838));
#24142=CARTESIAN_POINT('Ctrl Pts',(-2.11578025795185,-6.43006310150856,
62.0962735063767));
#24143=CARTESIAN_POINT('Ctrl Pts',(-1.95006498203012,-6.47993329949159,
62.1044092247696));
#24144=CARTESIAN_POINT('Ctrl Pts',(-1.78448218703509,-6.52976362879016,
62.1125384390698));
#24145=CARTESIAN_POINT('Ctrl Pts',(-1.61684102990984,-6.57328733880246,
62.12066765337));
#24146=CARTESIAN_POINT('Ctrl Pts',(-1.4476673996933,-6.6103364589002,62.1287968676703));
#24147=CARTESIAN_POINT('Ctrl Pts',(-1.27859344432647,-6.64736375014983,
62.1369212923457));
#24148=CARTESIAN_POINT('Ctrl Pts',(-1.1079891702708,-6.67792397036248,62.1450457170211));
#24149=CARTESIAN_POINT('Ctrl Pts',(-0.936394478055206,-6.70189931149877,
62.1531701416965));
#24150=CARTESIAN_POINT('Ctrl Pts',(-0.763758096208908,-6.72602019830394,
62.1613438868307));
#24151=CARTESIAN_POINT('Ctrl Pts',(-0.590119591330146,-6.74347588739461,
62.1695176319649));
#24152=CARTESIAN_POINT('Ctrl Pts',(-0.416038587367723,-6.75419876031355,
62.1776913770991));
#24153=CARTESIAN_POINT('Ctrl Pts',(-0.243072347214923,-6.76485296709205,
62.1858127799612));
#24154=CARTESIAN_POINT('Ctrl Pts',(-0.0696696296329457,-6.76886033584515,
62.1939341828234));
#24155=CARTESIAN_POINT('Ctrl Pts',(0.103616438768401,-6.76620666500935,
62.2020555856855));
#24156=CARTESIAN_POINT('Ctrl Pts',(0.276915904736252,-6.76355278900569,
62.2101776164518));
#24157=CARTESIAN_POINT('Ctrl Pts',(0.450098337609681,-6.75423685314459,
62.218299647218));
#24158=CARTESIAN_POINT('Ctrl Pts',(0.622611803962377,-6.73829678342879,
62.2264216779843));
#24159=CARTESIAN_POINT('Ctrl Pts',(0.795171458695426,-6.72235244595338,
62.2345458833254));
#24160=CARTESIAN_POINT('Ctrl Pts',(0.967061425990442,-6.69978047686512,
62.2426700886665));
#24161=CARTESIAN_POINT('Ctrl Pts',(1.13773612147734,-6.67067054484673,62.2507942940076));
#24162=CARTESIAN_POINT('Ctrl Pts',(1.31025825244533,-6.64124551795671,62.2590064382501));
#24163=CARTESIAN_POINT('Ctrl Pts',(1.48153827060829,-6.60514022707172,62.2672185824925));
#24164=CARTESIAN_POINT('Ctrl Pts',(1.65102533557588,-6.56249985457421,62.2754307267349));
#24165=CARTESIAN_POINT('Ctrl Pts',(1.81896517043931,-6.52024874168182,62.2835679031514));
#24166=CARTESIAN_POINT('Ctrl Pts',(1.98514431810167,-6.47158153011745,62.2917050795678));
#24167=CARTESIAN_POINT('Ctrl Pts',(2.14904449102325,-6.41668892619883,62.2998422559843));
#24168=CARTESIAN_POINT('Ctrl Pts',(2.31520968297819,-6.36103773374152,62.3080918841397));
#24169=CARTESIAN_POINT('Ctrl Pts',(2.47903208332613,-6.29898796424722,62.3163415122951));
#24170=CARTESIAN_POINT('Ctrl Pts',(2.63999528366881,-6.2307875828186,62.3245911404505));
#24171=CARTESIAN_POINT('Ctrl Pts',(2.80095848401154,-6.16258720138996,62.332840768606));
#24172=CARTESIAN_POINT('Ctrl Pts',(2.95906216307362,-6.08823642901855,62.3410903967614));
#24173=CARTESIAN_POINT('Ctrl Pts',(3.11381873017303,-6.00802978651268,62.3493400249168));
#24174=CARTESIAN_POINT('Ctrl Pts',(3.2681108100888,-5.92806387665025,62.3575648925944));
#24175=CARTESIAN_POINT('Ctrl Pts',(3.41953711714995,-5.84203832537791,62.365789760272));
#24176=CARTESIAN_POINT('Ctrl Pts',(3.56758905171279,-5.75018237607287,62.3740146279496));
#24177=CARTESIAN_POINT('Ctrl Pts',(3.71547418919984,-5.65842991277619,62.3822302293931));
#24178=CARTESIAN_POINT('Ctrl Pts',(3.85999222207756,-5.56086031861584,62.3904458308366));
#24179=CARTESIAN_POINT('Ctrl Pts',(4.00065716874635,-5.45774964780892,62.3986614322802));
#24180=CARTESIAN_POINT('Ctrl Pts',(4.14119190301844,-5.35473442571108,62.4068694286083));
#24181=CARTESIAN_POINT('Ctrl Pts',(4.27788036684366,-5.24618855289939,62.4150774249364));
#24182=CARTESIAN_POINT('Ctrl Pts',(4.41026364162656,-5.13243252379872,62.4232854212646));
#24183=CARTESIAN_POINT('Ctrl Pts',(4.54255096015806,-5.0187589492388,62.431487468136));
#24184=CARTESIAN_POINT('Ctrl Pts',(4.67053903420414,-4.89988297336291,62.4396895150074));
#24185=CARTESIAN_POINT('Ctrl Pts',(4.79380019810623,-4.77616673291843,62.4478915618789));
#24186=CARTESIAN_POINT('Ctrl Pts',(4.91699676974234,-4.65251532321265,62.4560893106504));
#24187=CARTESIAN_POINT('Ctrl Pts',(5.03547111325602,-4.5240289554722,62.464287059422));
#24188=CARTESIAN_POINT('Ctrl Pts',(5.1488307097639,-4.39110821116859,62.4724848081936));
#24189=CARTESIAN_POINT('Ctrl Pts',(5.26216868520536,-4.25821281882749,62.4806809934092));
#24190=CARTESIAN_POINT('Ctrl Pts',(5.37039361948129,-4.12088500325434,62.4888771786248));
#24191=CARTESIAN_POINT('Ctrl Pts',(5.47315156208715,-3.97956040014761,62.4970733638405));
#24192=CARTESIAN_POINT('Ctrl Pts',(5.57590190289238,-3.838246251916,62.5052689427208));
#24193=CARTESIAN_POINT('Ctrl Pts',(5.67318584573008,-3.69293619468311,62.5134645216012));
#24194=CARTESIAN_POINT('Ctrl Pts',(5.76469131545445,-3.54409692834776,62.5216601004815));
#24195=CARTESIAN_POINT('Ctrl Pts',(5.85620666414728,-3.39524159326349,62.5298565641599));
#24196=CARTESIAN_POINT('Ctrl Pts',(5.94194210886517,-3.24285659572238,62.5380530278384));
#24197=CARTESIAN_POINT('Ctrl Pts',(6.02163027224256,-3.08743548344123,62.5462494915168));
#24198=CARTESIAN_POINT('Ctrl Pts',(6.10134153716534,-2.93196931468335,62.5544483313446));
#24199=CARTESIAN_POINT('Ctrl Pts',(6.175001865117,-2.77346559723053,62.5626471711724));
#24200=CARTESIAN_POINT('Ctrl Pts',(6.24239096363938,-2.61244024947431,62.5708460110002));
#24201=CARTESIAN_POINT('Ctrl Pts',(6.30985045199229,-2.45124670616144,62.5790534147494));
#24202=CARTESIAN_POINT('Ctrl Pts',(6.37102548520224,-2.28752660178286,62.5872608184986));
#24203=CARTESIAN_POINT('Ctrl Pts',(6.42574450346411,-2.12181445376377,62.5954682222479));
#24204=CARTESIAN_POINT('Ctrl Pts',(6.48049283212787,-1.95601354154876,62.6036800223169));
#24205=CARTESIAN_POINT('Ctrl Pts',(6.52877815272834,-1.78821880302378,62.6118918223859));
#24206=CARTESIAN_POINT('Ctrl Pts',(6.57047952295643,-1.61897740515742,62.6201036224549));
#24207=CARTESIAN_POINT('Ctrl Pts',(6.6122422834284,-1.44948686030543,62.6283275114411));
#24208=CARTESIAN_POINT('Ctrl Pts',(6.64740165105475,-1.27854575147428,62.6365514004272));
#24209=CARTESIAN_POINT('Ctrl Pts',(6.67588807835824,-1.10671015412091,62.6447752894134));
#24210=CARTESIAN_POINT('Ctrl Pts',(6.70220904471821,-0.947937032830664,
62.6523740206634));
#24211=CARTESIAN_POINT('Ctrl Pts',(6.72283357712056,-0.788400533362211,
62.6599727519134));
#24212=CARTESIAN_POINT('Ctrl Pts',(6.7377463720338,-0.628540234309178,62.6675714831635));
#24213=CARTESIAN_POINT('Ctrl Pts',(6.75388794517058,-0.455507833351089,
62.6757963314855));
#24214=CARTESIAN_POINT('Ctrl Pts',(6.76338240844148,-0.281610384600581,
62.6840211798076));
#24215=CARTESIAN_POINT('Ctrl Pts',(6.76614767100241,-0.107399693615434,
62.6922460281296));
#24216=CARTESIAN_POINT('Ctrl Pts',(6.76890981926458,0.066614797505694,62.7004616134488));
#24217=CARTESIAN_POINT('Ctrl Pts',(6.76495785204496,0.240941472929343,62.708677198768));
#24218=CARTESIAN_POINT('Ctrl Pts',(6.75426128694405,0.41502224963117,62.7168927840872));
#24219=CARTESIAN_POINT('Ctrl Pts',(6.7435746193942,0.588941949075024,62.7251007675104));
#24220=CARTESIAN_POINT('Ctrl Pts',(6.72615580448716,0.762615847088591,62.7333087509337));
#24221=CARTESIAN_POINT('Ctrl Pts',(6.70202637679818,0.935484604203326,62.7415167343569));
#24222=CARTESIAN_POINT('Ctrl Pts',(6.67791442959404,1.10822812711328,62.7497187715335));
#24223=CARTESIAN_POINT('Ctrl Pts',(6.64710160215835,1.28016731702472,62.75792080871));
#24224=CARTESIAN_POINT('Ctrl Pts',(6.6096613572644,1.45074661546589,62.7661228458865));
#24225=CARTESIAN_POINT('Ctrl Pts',(6.57224071749989,1.6212365921295,62.7743205881659));
#24226=CARTESIAN_POINT('Ctrl Pts',(6.52819965053682,1.7903677463213,62.7825183304454));
#24227=CARTESIAN_POINT('Ctrl Pts',(6.47766296223122,1.95759330498904,62.7907160727248));
#24228=CARTESIAN_POINT('Ctrl Pts',(6.42713588264062,2.12478706848404,62.7989122563391));
#24229=CARTESIAN_POINT('Ctrl Pts',(6.37011573945722,2.29007561325848,62.8071084399534));
#24230=CARTESIAN_POINT('Ctrl Pts',(6.30677767904757,2.45292566276831,62.8153046235678));
#24231=CARTESIAN_POINT('Ctrl Pts',(6.2434442812029,2.6157637242423,62.8235002038287));
#24232=CARTESIAN_POINT('Ctrl Pts',(6.17379402159843,2.77616331319956,62.8316957840896));
#24233=CARTESIAN_POINT('Ctrl Pts',(6.09805081799695,2.93360958907737,62.8398913643505));
#24234=CARTESIAN_POINT('Ctrl Pts',(6.02229940957214,3.09107292019998,62.8480878323912));
#24235=CARTESIAN_POINT('Ctrl Pts',(5.94045389779311,3.24558197745001,62.8562843004319));
#24236=CARTESIAN_POINT('Ctrl Pts',(5.85278495040703,3.39664501004873,62.8644807684726));
#24237=CARTESIAN_POINT('Ctrl Pts',(5.76509055595571,3.54775189067987,62.872679615646));
#24238=CARTESIAN_POINT('Ctrl Pts',(5.67156953904491,3.69541044400648,62.8808784628194));
#24239=CARTESIAN_POINT('Ctrl Pts',(5.57253684130363,3.83915643759326,62.8890773099928));
#24240=CARTESIAN_POINT('Ctrl Pts',(5.47340064476296,3.98305265972167,62.8972847257588));
#24241=CARTESIAN_POINT('Ctrl Pts',(5.36874146302995,4.12302785692412,62.9054921415247));
#24242=CARTESIAN_POINT('Ctrl Pts',(5.2589162295534,4.25864873998078,62.9136995572907));
#24243=CARTESIAN_POINT('Ctrl Pts',(5.14903213361444,4.39434231106074,62.9219113719429));
#24244=CARTESIAN_POINT('Ctrl Pts',(5.03397670244471,4.52567664593781,62.930123186595));
#24245=CARTESIAN_POINT('Ctrl Pts',(4.914144874771,4.6522542008968,62.9383350012471));
#24246=CARTESIAN_POINT('Ctrl Pts',(4.79413657651372,4.7790181605483,62.9465589090448));
#24247=CARTESIAN_POINT('Ctrl Pts',(4.66933808116413,4.90101108999017,62.9547828168424));
#24248=CARTESIAN_POINT('Ctrl Pts',(4.54017960588137,5.0178738671213,62.96300672464));
#24249=CARTESIAN_POINT('Ctrl Pts',(4.42083956005578,5.12585291493526,62.9706054635635));
#24250=CARTESIAN_POINT('Ctrl Pts',(4.29777775434849,5.22945244427701,62.978204202487));
#24251=CARTESIAN_POINT('Ctrl Pts',(4.17135572179625,5.32842194671534,62.9858029414105));
#24252=CARTESIAN_POINT('Ctrl Pts',(4.03572133038419,5.43460334532583,62.9939553995587));
#24253=CARTESIAN_POINT('Ctrl Pts',(3.89581693059393,5.53576935291031,63.0021078577069));
#24254=CARTESIAN_POINT('Ctrl Pts',(3.75205217390674,5.63155338110913,63.0102603158551));
#24255=CARTESIAN_POINT('Ctrl Pts',(3.60847848010543,5.72721011265146,63.0184019394134));
#24256=CARTESIAN_POINT('Ctrl Pts',(3.46105494864114,5.8174989092354,63.0265435629716));
#24257=CARTESIAN_POINT('Ctrl Pts',(3.31022470676398,5.90209296696768,63.0346851865299));
#24258=CARTESIAN_POINT('Ctrl Pts',(3.24058550614499,5.94115053582307,63.0384442215171));
#24259=CARTESIAN_POINT('Ctrl Pts',(3.17022055591669,5.97899470370963,63.0422032565043));
#24260=CARTESIAN_POINT('Ctrl Pts',(3.09917575053259,6.01559628526639,63.0459622914914));
#24261=CARTESIAN_POINT('Ctrl Pts',(3.09917575053255,6.01559628526641,61.0455262068868));
#24262=CARTESIAN_POINT('Ctrl Pts',(2.94555351499629,6.09474094267679,61.0536815348355));
#24263=CARTESIAN_POINT('Ctrl Pts',(2.78910094792113,6.16789239804414,61.0618368627841));
#24264=CARTESIAN_POINT('Ctrl Pts',(2.630338046527,6.23487054885605,61.0699921907328));
#24265=CARTESIAN_POINT('Ctrl Pts',(2.5886648585963,6.25245143860753,61.0721328577983));
#24266=CARTESIAN_POINT('Ctrl Pts',(2.54683256238906,6.26960726075716,61.0742735248638));
#24267=CARTESIAN_POINT('Ctrl Pts',(2.50485070333391,6.28633533579045,61.0764141919293));
#24268=CARTESIAN_POINT('Ctrl Pts',(2.34341266435111,6.35066187325475,61.0846459639602));
#24269=CARTESIAN_POINT('Ctrl Pts',(2.17925810486761,6.40886006779471,61.092877735991));
#24270=CARTESIAN_POINT('Ctrl Pts',(2.01289222894281,6.46069298718502,61.1011095080218));
#24271=CARTESIAN_POINT('Ctrl Pts',(1.84672501049944,6.51246401288971,61.1093314504943));
#24272=CARTESIAN_POINT('Ctrl Pts',(1.67835207224814,6.55788479280917,61.1175533929666));
#24273=CARTESIAN_POINT('Ctrl Pts',(1.50829947536923,6.59676600256527,61.125775335439));
#24274=CARTESIAN_POINT('Ctrl Pts',(1.33841586675202,6.63560857446361,61.1339891074289));
#24275=CARTESIAN_POINT('Ctrl Pts',(1.166856270493,6.66792443889963,61.1422028794189));
#24276=CARTESIAN_POINT('Ctrl Pts',(0.994162919560558,6.69357371583901,61.1504166514088));
#24277=CARTESIAN_POINT('Ctrl Pts',(0.821606593053894,6.71920264122793,61.1586239061391));
#24278=CARTESIAN_POINT('Ctrl Pts',(0.647918656475359,6.73817546252874,61.1668311608695));
#24279=CARTESIAN_POINT('Ctrl Pts',(0.473652670493714,6.75040311001752,61.1750384155998));
#24280=CARTESIAN_POINT('Ctrl Pts',(0.299490062808121,6.76262350380526,61.1832408016118));
#24281=CARTESIAN_POINT('Ctrl Pts',(0.124750445316112,6.76810666999312,61.1914431876238));
#24282=CARTESIAN_POINT('Ctrl Pts',(-0.0500062489708984,6.7668152313377,
61.1996455736357));
#24283=CARTESIAN_POINT('Ctrl Pts',(-0.224710782623472,6.76552417814539,
61.2078455114344));
#24284=CARTESIAN_POINT('Ctrl Pts',(-0.399432025036917,6.75746254672673,
61.2160454492332));
#24285=CARTESIAN_POINT('Ctrl Pts',(-0.573608529755235,6.74264504883596,
61.2242453870319));
#24286=CARTESIAN_POINT('Ctrl Pts',(-0.747760680102598,6.72782962281384,
61.2324441782676));
#24287=CARTESIAN_POINT('Ctrl Pts',(-0.921367887376428,6.70626024126302,
61.2406429695034));
#24288=CARTESIAN_POINT('Ctrl Pts',(-1.09387229603085,6.67800362383671,61.2488417607391));
#24289=CARTESIAN_POINT('Ctrl Pts',(-1.26638387731199,6.64974583151771,61.2570408928756));
#24290=CARTESIAN_POINT('Ctrl Pts',(-1.4377922148764,6.61480030724318,61.265240025012));
#24291=CARTESIAN_POINT('Ctrl Pts',(-1.60754807733957,6.57328518923695,61.2734391571484));
#24292=CARTESIAN_POINT('Ctrl Pts',(-1.77734179262776,6.53176081402761,61.2816401175593));
#24293=CARTESIAN_POINT('Ctrl Pts',(-1.94548195082092,6.48366401253082,61.2898410779702));
#24294=CARTESIAN_POINT('Ctrl Pts',(-2.11143289407961,6.42916325300568,61.2980420383812));
#24295=CARTESIAN_POINT('Ctrl Pts',(-2.27753937332141,6.37461141314893,61.3062506850662));
#24296=CARTESIAN_POINT('Ctrl Pts',(-2.44145219723324,6.3136437355179,61.3144593317513));
#24297=CARTESIAN_POINT('Ctrl Pts',(-2.602653275827,6.24647780159563,61.3226679784363));
#24298=CARTESIAN_POINT('Ctrl Pts',(-2.76393131634332,6.17927980077003,61.3308805441598));
#24299=CARTESIAN_POINT('Ctrl Pts',(-2.9224947051069,6.10587779396102,61.3390931098833));
#24300=CARTESIAN_POINT('Ctrl Pts',(-3.07784858531042,6.02653607687722,61.3473056756068));
#24301=CARTESIAN_POINT('Ctrl Pts',(-3.23341563345513,5.94708549150858,61.3555295101556));
#24302=CARTESIAN_POINT('Ctrl Pts',(-3.38576405884343,5.86167908273416,61.3637533447044));
#24303=CARTESIAN_POINT('Ctrl Pts',(-3.53442564233534,5.7706259954014,61.3719771792532));
#24304=CARTESIAN_POINT('Ctrl Pts',(-3.67101767300739,5.68696533603261,61.3795333362275));
#24305=CARTESIAN_POINT('Ctrl Pts',(-3.80449737468062,5.59853828613694,61.3870894932019));
#24306=CARTESIAN_POINT('Ctrl Pts',(-3.93452598659682,5.50561479408016,61.3946456501763));
#24307=CARTESIAN_POINT('Ctrl Pts',(-4.08330409181379,5.39929218650467,61.4032913682287));
#24308=CARTESIAN_POINT('Ctrl Pts',(-4.22790301321821,5.2868403360242,61.4119370862811));
#24309=CARTESIAN_POINT('Ctrl Pts',(-4.36781656082279,5.16860401762431,61.4205828043335));
#24310=CARTESIAN_POINT('Ctrl Pts',(-4.50755048794591,5.0505194905613,61.4292174230459));
#24311=CARTESIAN_POINT('Ctrl Pts',(-4.64261080379205,4.92666549947308,61.4378520417583));
#24312=CARTESIAN_POINT('Ctrl Pts',(-4.77252193589838,4.7974288292135,61.4464866604707));
#24313=CARTESIAN_POINT('Ctrl Pts',(-4.90702102452552,4.66362802180546,61.4554262203731));
#24314=CARTESIAN_POINT('Ctrl Pts',(-5.03600031520607,4.52405756887495,61.4643657802755));
#24315=CARTESIAN_POINT('Ctrl Pts',(-5.15896883919704,4.37919279276375,61.4733053401779));
#24316=CARTESIAN_POINT('Ctrl Pts',(-5.2774130730106,4.23965791947924,61.4819159934485));
#24317=CARTESIAN_POINT('Ctrl Pts',(-5.39028068970313,4.09521158941102,61.490526646719));
#24318=CARTESIAN_POINT('Ctrl Pts',(-5.49716951174906,3.94631680926615,61.4991372999895));
#24319=CARTESIAN_POINT('Ctrl Pts',(-5.60395715637359,3.79756296799242,61.5077398027006));
#24320=CARTESIAN_POINT('Ctrl Pts',(-5.70477711225701,3.64436931869997,61.5163423054117));
#24321=CARTESIAN_POINT('Ctrl Pts',(-5.79926748747544,3.48723179738748,61.5249448081228));
#24322=CARTESIAN_POINT('Ctrl Pts',(-5.89365151567872,3.33027113119192,61.5335376288903));
#24323=CARTESIAN_POINT('Ctrl Pts',(-5.98172001818,3.16937570896732,61.5421304496577));
#24324=CARTESIAN_POINT('Ctrl Pts',(-6.063154334882,3.00507046696107,61.5507232704252));
#24325=CARTESIAN_POINT('Ctrl Pts',(-6.07275173900028,2.98570634787531,61.5517359733834));
#24326=CARTESIAN_POINT('Ctrl Pts',(-6.08225704614675,2.96629489997478,61.5527486763416));
#24327=CARTESIAN_POINT('Ctrl Pts',(-6.09166977497695,2.94683700815506,61.5537613792998));
#24328=CARTESIAN_POINT('Ctrl Pts',(-6.16973431150839,2.78546283769022,61.5621602388123));
#24329=CARTESIAN_POINT('Ctrl Pts',(-6.24135027080265,2.62105142964491,61.5705590983248));
#24330=CARTESIAN_POINT('Ctrl Pts',(-6.3063014248226,2.4541498200559,61.5789579578373));
#24331=CARTESIAN_POINT('Ctrl Pts',(-6.37129295259934,2.28714446411944,61.5873620380963));
#24332=CARTESIAN_POINT('Ctrl Pts',(-6.42961129234394,2.11764613002741,61.5957661183554));
#24333=CARTESIAN_POINT('Ctrl Pts',(-6.48108965391801,1.94621835822112,61.6041701986144));
#24334=CARTESIAN_POINT('Ctrl Pts',(-6.53263955916306,1.77455233928095,61.6125859587081));
#24335=CARTESIAN_POINT('Ctrl Pts',(-6.57733039319003,1.60095184351121,61.6210017188018));
#24336=CARTESIAN_POINT('Ctrl Pts',(-6.61504586263275,1.42599342048459,61.6294174788956));
#24337=CARTESIAN_POINT('Ctrl Pts',(-6.65278947490392,1.2509044455927,61.637839518728));
#24338=CARTESIAN_POINT('Ctrl Pts',(-6.68354728082114,1.07445584971838,61.6462615585603));
#24339=CARTESIAN_POINT('Ctrl Pts',(-6.70725467162531,0.89723116862962,61.6546835983928));
#24340=CARTESIAN_POINT('Ctrl Pts',(-6.7309994247517,0.719727185373209,61.6631189111732));
#24341=CARTESIAN_POINT('Ctrl Pts',(-6.74767152196744,0.54144500394835,61.6715542239536));
#24342=CARTESIAN_POINT('Ctrl Pts',(-6.7572583650388,0.362971607860936,61.6799895367341));
#24343=CARTESIAN_POINT('Ctrl Pts',(-6.76377067841043,0.241735172136537,
61.6857196190777));
#24344=CARTESIAN_POINT('Ctrl Pts',(-6.76701462962386,0.120410512533247,
61.6914497014212));
#24345=CARTESIAN_POINT('Ctrl Pts',(-6.76699995039181,-0.000819388301668836,
61.6971797837648));
#24346=CARTESIAN_POINT('',(-6.76699930182051,-0.00307394872789667,61.3028202161439));
#24347=CARTESIAN_POINT('Ctrl Pts',(3.0991757505326,6.01559628526638,60.6511868721373));
#24348=CARTESIAN_POINT('Ctrl Pts',(2.94429628532114,6.0953886549795,60.6593889979253));
#24349=CARTESIAN_POINT('Ctrl Pts',(2.78649934526633,6.16911017648326,60.6675911237134));
#24350=CARTESIAN_POINT('Ctrl Pts',(2.62631334247578,6.2365669424078,60.6757932495014));
#24351=CARTESIAN_POINT('Ctrl Pts',(2.46612733968517,6.30402370833236,60.6839953752894));
#24352=CARTESIAN_POINT('Ctrl Pts',(2.30355264512538,6.36521564451638,60.6921975010774));
#24353=CARTESIAN_POINT('Ctrl Pts',(2.13913066466676,6.42000070089423,60.7003996268654));
#24354=CARTESIAN_POINT('Ctrl Pts',(1.9742258990232,6.47494662027531,60.7086258362024));
#24355=CARTESIAN_POINT('Ctrl Pts',(1.80697223583982,6.52361162574131,60.7168520455394));
#24356=CARTESIAN_POINT('Ctrl Pts',(1.63788877021495,6.56579084165828,60.7250782548764));
#24357=CARTESIAN_POINT('Ctrl Pts',(1.46899526262028,6.60792267103311,60.7332952224196));
#24358=CARTESIAN_POINT('Ctrl Pts',(1.29827639086296,6.64358313425741,60.7415121899627));
#24359=CARTESIAN_POINT('Ctrl Pts',(1.12626903778939,6.67261620764427,60.7497291575059));
#24360=CARTESIAN_POINT('Ctrl Pts',(0.954420404354541,6.70162249078736,60.7579385428493));
#24361=CARTESIAN_POINT('Ctrl Pts',(0.781286008843523,6.7240135038616,60.7661479281927));
#24362=CARTESIAN_POINT('Ctrl Pts',(0.60741572512062,6.73968360806917,60.7743573135361));
#24363=CARTESIAN_POINT('Ctrl Pts',(0.433670994096106,6.75534239680738,60.7825607708367));
#24364=CARTESIAN_POINT('Ctrl Pts',(0.259191789036619,6.76428991136996,60.7907642281373));
#24365=CARTESIAN_POINT('Ctrl Pts',(0.0845360497352806,6.76647195045506,
60.7989676854379));
#24366=CARTESIAN_POINT('Ctrl Pts',(-0.0900286051981397,6.76865285158929,
60.8071668645697));
#24367=CARTESIAN_POINT('Ctrl Pts',(-0.264769253210243,6.76407530167798,
60.8153660437016));
#24368=CARTESIAN_POINT('Ctrl Pts',(-0.439124893712001,6.75273709896383,
60.8235652228334));
#24369=CARTESIAN_POINT('Ctrl Pts',(-0.613447681853623,6.74140103261141,
60.8317628570632));
#24370=CARTESIAN_POINT('Ctrl Pts',(-0.787385249069672,6.72330686788164,
60.8399604912931));
#24371=CARTESIAN_POINT('Ctrl Pts',(-0.960378348078167,6.69850449194017,
60.8481581255229));
#24372=CARTESIAN_POINT('Ctrl Pts',(-1.13335896025528,6.67370390626137,60.8563551680385));
#24373=CARTESIAN_POINT('Ctrl Pts',(-1.30539488482131,6.642196123723,60.8645522105541));
#24374=CARTESIAN_POINT('Ctrl Pts',(-1.47593379243997,6.60408270998583,60.8727492530697));
#24375=CARTESIAN_POINT('Ctrl Pts',(-1.64649138553442,6.56596512026747,60.8809471937125));
#24376=CARTESIAN_POINT('Ctrl Pts',(-1.81555128478065,6.52124053565646,60.8891451343553));
#24377=CARTESIAN_POINT('Ctrl Pts',(-1.98257306739036,6.47006128506202,60.8973430749982));
#24378=CARTESIAN_POINT('Ctrl Pts',(-2.14964350615569,6.41886712512138,60.9055434038341));
#24379=CARTESIAN_POINT('Ctrl Pts',(-2.31467430277852,6.36121465882843,60.9137437326701));
#24380=CARTESIAN_POINT('Ctrl Pts',(-2.4771418132325,6.29730556961747,60.9219440615061));
#24381=CARTESIAN_POINT('Ctrl Pts',(-2.63977861904817,6.23332988547721,60.9301529352975));
#24382=CARTESIAN_POINT('Ctrl Pts',(-2.79984646819465,6.16308468478895,60.9383618090889));
#24383=CARTESIAN_POINT('Ctrl Pts',(-2.95684235178738,6.08681955594845,60.9465706828803));
#24384=CARTESIAN_POINT('Ctrl Pts',(-3.1139224933389,6.01051349645464,60.9547839622838));
#24385=CARTESIAN_POINT('Ctrl Pts',(-3.26792706660759,5.9281812369788,60.9629972416872));
#24386=CARTESIAN_POINT('Ctrl Pts',(-3.41837927031567,5.84011747863655,60.9712105210906));
#24387=CARTESIAN_POINT('Ctrl Pts',(-3.56905153401845,5.75192491320662,60.9794358137061));
#24388=CARTESIAN_POINT('Ctrl Pts',(-3.71616074221359,5.65798428862504,60.9876611063215));
#24389=CARTESIAN_POINT('Ctrl Pts',(-3.85925953728978,5.55863335936433,60.9958863989369));
#24390=CARTESIAN_POINT('Ctrl Pts',(-3.98867520777543,5.46878237832146,61.003325188049));
#24391=CARTESIAN_POINT('Ctrl Pts',(-4.11481101145358,5.37450694914118,61.0107639771612));
#24392=CARTESIAN_POINT('Ctrl Pts',(-4.23736099882772,5.27608384747758,61.0182027662733));
#24393=CARTESIAN_POINT('Ctrl Pts',(-4.37105208055609,5.16871304140562,61.0263178202561));
#24394=CARTESIAN_POINT('Ctrl Pts',(-4.50087193157398,5.05608682975706,61.0344328742391));
#24395=CARTESIAN_POINT('Ctrl Pts',(-4.62637357311772,4.93851764823799,61.042547928222));
#24396=CARTESIAN_POINT('Ctrl Pts',(-4.75173320454199,4.82108150094307,61.0506537996972));
#24397=CARTESIAN_POINT('Ctrl Pts',(-4.87278408495042,4.69871376635119,61.0587596711725));
#24398=CARTESIAN_POINT('Ctrl Pts',(-4.98911012961864,4.57176870746286,61.0668655426477));
#24399=CARTESIAN_POINT('Ctrl Pts',(-5.10532954422664,4.4449400125351,61.0749639838904));
#24400=CARTESIAN_POINT('Ctrl Pts',(-5.21683249680145,4.31354261643889,61.0830624251331));
#24401=CARTESIAN_POINT('Ctrl Pts',(-5.32323783316524,4.17796935981563,61.0911608663758));
#24402=CARTESIAN_POINT('Ctrl Pts',(-5.42956848042597,4.04249126613515,61.0992536230792));
#24403=CARTESIAN_POINT('Ctrl Pts',(-5.53080840856302,3.90284343752029,61.1073463797826));
#24404=CARTESIAN_POINT('Ctrl Pts',(-5.62661508061142,3.75945364842235,61.1154391364861));
#24405=CARTESIAN_POINT('Ctrl Pts',(-5.72238045895121,3.61612566186951,61.1235284051241));
#24406=CARTESIAN_POINT('Ctrl Pts',(-5.81271703735493,3.469059231583,61.1316176737622));
#24407=CARTESIAN_POINT('Ctrl Pts',(-5.89732414460166,3.31871314420187,61.1397069424002));
#24408=CARTESIAN_POINT('Ctrl Pts',(-5.98191328451942,3.16839898460672,61.1477944931855));
#24409=CARTESIAN_POINT('Ctrl Pts',(-6.06077519345288,3.01480687577612,61.1558820439708));
#24410=CARTESIAN_POINT('Ctrl Pts',(-6.13365395582839,2.85842231836913,61.1639695947561));
#24411=CARTESIAN_POINT('Ctrl Pts',(-6.20653140322502,2.70204058266743,61.1720569996147));
#24412=CARTESIAN_POINT('Ctrl Pts',(-6.27342576295178,2.5428668337222,61.1801444044733));
#24413=CARTESIAN_POINT('Ctrl Pts',(-6.33412833012273,2.38140867923519,61.1882318093319));
#24414=CARTESIAN_POINT('Ctrl Pts',(-6.39484159834729,2.21992206182728,61.1963206398921));
#24415=CARTESIAN_POINT('Ctrl Pts',(-6.44936077169434,2.05615058330686,61.2044094704524));
#24416=CARTESIAN_POINT('Ctrl Pts',(-6.49752632398515,1.89061912322921,61.2124983010127));
#24417=CARTESIAN_POINT('Ctrl Pts',(-6.54573346668213,1.72494472861995,61.2205941161861));
#24418=CARTESIAN_POINT('Ctrl Pts',(-6.58757592708849,1.55750767229182,61.2286899313595));
#24419=CARTESIAN_POINT('Ctrl Pts',(-6.62294466919305,1.38884589094952,61.2367857465329));
#24420=CARTESIAN_POINT('Ctrl Pts',(-6.65832968734877,1.22010649452627,61.244885287253));
#24421=CARTESIAN_POINT('Ctrl Pts',(-6.68723498928914,1.05014161398107,61.2529848279732));
#24422=CARTESIAN_POINT('Ctrl Pts',(-6.70960323088031,0.879496153579135,
61.2610843686933));
#24423=CARTESIAN_POINT('Ctrl Pts',(-6.73200003672778,0.708632778834374,
61.2691942525312));
#24424=CARTESIAN_POINT('Ctrl Pts',(-6.74784307313428,0.537087455670259,
61.2773041363692));
#24425=CARTESIAN_POINT('Ctrl Pts',(-6.75712705912241,0.365407863729989,
61.2854140202071));
#24426=CARTESIAN_POINT('Ctrl Pts',(-6.76376911394562,0.242582897907103,
61.2912160855193));
#24427=CARTESIAN_POINT('Ctrl Pts',(-6.76705506770958,0.11968923497642,61.2970181508316));
#24428=CARTESIAN_POINT('Ctrl Pts',(-6.76699930182051,-0.00307394872799501,
61.3028202161439));
#24429=CARTESIAN_POINT('Ctrl Pts',(-6.76699930182007,-0.00307394969982656,
61.3028202161898));
#24430=CARTESIAN_POINT('Ctrl Pts',(-6.7668929816298,-0.237127439049988,
61.3138821126868));
#24431=CARTESIAN_POINT('Ctrl Pts',(-6.75464487673108,-0.470843644988345,
61.3249440091838));
#24432=CARTESIAN_POINT('Ctrl Pts',(-6.73035212995149,-0.703313021959266,
61.3360059056808));
#24433=CARTESIAN_POINT('Ctrl Pts',(-6.71244851064451,-0.874641660238803,
61.344158461894));
#24434=CARTESIAN_POINT('Ctrl Pts',(-6.68797057376292,-1.04555419704913,
61.3523110181073));
#24435=CARTESIAN_POINT('Ctrl Pts',(-6.65693963625638,-1.21550141062804,
61.3604635743205));
#24436=CARTESIAN_POINT('Ctrl Pts',(-6.62594464883903,-1.385251736263,61.3686066856009));
#24437=CARTESIAN_POINT('Ctrl Pts',(-6.58841183801031,-1.55403860890881,
61.3767497968813));
#24438=CARTESIAN_POINT('Ctrl Pts',(-6.54441439465594,-1.7213161333759,61.3848929081616));
#24439=CARTESIAN_POINT('Ctrl Pts',(-6.50045867348595,-1.88843503081411,
61.3930282974389));
#24440=CARTESIAN_POINT('Ctrl Pts',(-6.45005061682981,-2.05404707849207,
61.4011636867163));
#24441=CARTESIAN_POINT('Ctrl Pts',(-6.39331475531231,-2.21761480864147,
61.4092990759936));
#24442=CARTESIAN_POINT('Ctrl Pts',(-6.33662077407636,-2.3810617992373,61.4174284600322));
#24443=CARTESIAN_POINT('Ctrl Pts',(-6.27360840794948,-2.54246713314629,
61.4255578440708));
#24444=CARTESIAN_POINT('Ctrl Pts',(-6.20445248283445,-2.70130679269302,
61.4336872281094));
#24445=CARTESIAN_POINT('Ctrl Pts',(-6.13533307997369,-2.86006256669525,
61.4418123189015));
#24446=CARTESIAN_POINT('Ctrl Pts',(-6.06007672529144,-3.01625503039086,
61.4499374096936));
#24447=CARTESIAN_POINT('Ctrl Pts',(-5.97890699582596,-3.16937850930801,
61.4580625004858));
#24448=CARTESIAN_POINT('Ctrl Pts',(-5.89742742390638,-3.3230864937397,61.4662186065109));
#24449=CARTESIAN_POINT('Ctrl Pts',(-5.8099893722018,-3.47370166810867,61.474374712536));
#24450=CARTESIAN_POINT('Ctrl Pts',(-5.71686660431286,-3.62073545408835,
61.4825308185611));
#24451=CARTESIAN_POINT('Ctrl Pts',(-5.6241186387233,-3.7671774556707,61.4906540977345));
#24452=CARTESIAN_POINT('Ctrl Pts',(-5.52573184718002,-3.91006654457672,
61.4987773769079));
#24453=CARTESIAN_POINT('Ctrl Pts',(-5.42202113510328,-4.04894749416356,
61.5069006560813));
#24454=CARTESIAN_POINT('Ctrl Pts',(-5.31829661306878,-4.18784693692251,
61.515025016938));
#24455=CARTESIAN_POINT('Ctrl Pts',(-5.20924697736297,-4.32273688415053,
61.5231493777947));
#24456=CARTESIAN_POINT('Ctrl Pts',(-5.09522848922095,-4.45319386986814,
61.5312737386514));
#24457=CARTESIAN_POINT('Ctrl Pts',(-4.98117312594974,-4.58369304714854,
61.5394007270368));
#24458=CARTESIAN_POINT('Ctrl Pts',(-4.86214595082338,-4.70975613270178,
61.5475277154222));
#24459=CARTESIAN_POINT('Ctrl Pts',(-4.73854122315886,-4.83099535048671,
61.5556547038076));
#24460=CARTESIAN_POINT('Ctrl Pts',(-4.61413740500253,-4.95301836601139,
61.5638342322477));
#24461=CARTESIAN_POINT('Ctrl Pts',(-4.48509691070055,-5.07015466284871,
61.5720137606878));
#24462=CARTESIAN_POINT('Ctrl Pts',(-4.35185604424471,-5.18204959163561,
61.5801932891279));
#24463=CARTESIAN_POINT('Ctrl Pts',(-4.21924265198395,-5.29341757112954,
61.5883342975316));
#24464=CARTESIAN_POINT('Ctrl Pts',(-4.08246869228262,-5.39959326967789,
61.5964753059353));
#24465=CARTESIAN_POINT('Ctrl Pts',(-3.94199372397726,-5.50027040063704,
61.6046163143389));
#24466=CARTESIAN_POINT('Ctrl Pts',(-3.80052174757006,-5.60166207822643,
61.6128151027972));
#24467=CARTESIAN_POINT('Ctrl Pts',(-3.65529634943674,-5.6974766422748,61.6210138912555));
#24468=CARTESIAN_POINT('Ctrl Pts',(-3.50681205355254,-5.7874483342021,61.6292126797137));
#24469=CARTESIAN_POINT('Ctrl Pts',(-3.35832775766833,-5.8774200261294,61.637411468172));
#24470=CARTESIAN_POINT('Ctrl Pts',(-3.20658492023533,-5.96154872252506,
61.6456102566303));
#24471=CARTESIAN_POINT('Ctrl Pts',(-3.05209803754034,-6.03961808140568,
61.6538090450885));
#24472=CARTESIAN_POINT('Ctrl Pts',(-2.89696557419642,-6.11801368201303,
61.6620420952205));
#24473=CARTESIAN_POINT('Ctrl Pts',(-2.73858390273423,-6.19054299955712,
61.6702751453525));
#24474=CARTESIAN_POINT('Ctrl Pts',(-2.57743551803947,-6.2569253751622,61.6785081954846));
#24475=CARTESIAN_POINT('Ctrl Pts',(-2.41647903629973,-6.32322869956199,
61.6867314413194));
#24476=CARTESIAN_POINT('Ctrl Pts',(-2.25276272988472,-6.38339952299103,
61.6949546871543));
#24477=CARTESIAN_POINT('Ctrl Pts',(-2.08679406518591,-6.43720277212897,
61.7031779329891));
#24478=CARTESIAN_POINT('Ctrl Pts',(-1.92098982466843,-6.49095271870399,
61.7113930321026));
#24479=CARTESIAN_POINT('Ctrl Pts',(-1.75293800810747,-6.53834754438559,
61.7196081312162));
#24480=CARTESIAN_POINT('Ctrl Pts',(-1.5831665497045,-6.57920000272805,61.7278232303297));
#24481=CARTESIAN_POINT('Ctrl Pts',(-1.41352931503992,-6.6200201625338,61.7360318344686));
#24482=CARTESIAN_POINT('Ctrl Pts',(-1.24217549320595,-6.65430817414218,
61.7442404386074));
#24483=CARTESIAN_POINT('Ctrl Pts',(-1.06964878308494,-6.68192640492582,
61.7524490427463));
#24484=CARTESIAN_POINT('Ctrl Pts',(-0.897223964891428,-6.70952832475816,
61.7606527989953));
#24485=CARTESIAN_POINT('Ctrl Pts',(-0.72362799107796,-6.73046825448673,
61.7688565552442));
#24486=CARTESIAN_POINT('Ctrl Pts',(-0.549415468721582,-6.74465949049538,
61.7770603114932));
#24487=CARTESIAN_POINT('Ctrl Pts',(-0.375254491459373,-6.758846527675,61.7852616404575));
#24488=CARTESIAN_POINT('Ctrl Pts',(-0.200477685263298,-6.7662888157333,
61.7934629694218));
#24489=CARTESIAN_POINT('Ctrl Pts',(-0.0256457625954296,-6.76695140331752,
61.801664298386));
#24490=CARTESIAN_POINT('Ctrl Pts',(0.149162049081187,-6.76761389952458,
61.8098644963088));
#24491=CARTESIAN_POINT('Ctrl Pts',(0.324024603937487,-6.76149855526386,
61.8180646942315));
#24492=CARTESIAN_POINT('Ctrl Pts',(0.498380174682741,-6.74862254104371,
61.8262648921542));
#24493=CARTESIAN_POINT('Ctrl Pts',(0.67274329690716,-6.73574596915308,61.8344654452341));
#24494=CARTESIAN_POINT('Ctrl Pts',(0.846599033939123,-6.71610817028283,
61.8426659983139));
#24495=CARTESIAN_POINT('Ctrl Pts',(1.01938970737883,-6.68977829412082,61.8508665513937));
#24496=CARTESIAN_POINT('Ctrl Pts',(1.19221917757542,-6.66344250610151,61.8590689457469));
#24497=CARTESIAN_POINT('Ctrl Pts',(1.36398275375906,-6.63041170204703,61.8672713401002));
#24498=CARTESIAN_POINT('Ctrl Pts',(1.53413183069558,-6.59080636387132,61.8754737344534));
#24499=CARTESIAN_POINT('Ctrl Pts',(1.70444002692969,-6.55116398774215,61.8836837994872));
#24500=CARTESIAN_POINT('Ctrl Pts',(1.87313035797372,-6.50493487494192,61.891893864521));
#24501=CARTESIAN_POINT('Ctrl Pts',(2.03966738128879,-6.45228997904671,61.9001039295549));
#24502=CARTESIAN_POINT('Ctrl Pts',(2.20628410626878,-6.39961988823825,61.9083179237802));
#24503=CARTESIAN_POINT('Ctrl Pts',(2.37074513180857,-6.3405280133835,61.9165319180055));
#24504=CARTESIAN_POINT('Ctrl Pts',(2.53253402601486,-6.27523389261922,61.9247459122308));
#24505=CARTESIAN_POINT('Ctrl Pts',(2.69454349236949,-6.20985075422143,61.932971104866));
#24506=CARTESIAN_POINT('Ctrl Pts',(2.85387321990489,-6.13824861793555,61.9411962975012));
#24507=CARTESIAN_POINT('Ctrl Pts',(3.0100293556326,-6.06069404261839,61.9494214901364));
#24508=CARTESIAN_POINT('Ctrl Pts',(3.15046023403321,-5.99094937914409,61.9568183882563));
#24509=CARTESIAN_POINT('Ctrl Pts',(3.28832468724447,-5.91639146587919,61.9642152863762));
#24510=CARTESIAN_POINT('Ctrl Pts',(3.42328362396414,-5.83724406119009,61.9716121844961));
#24511=CARTESIAN_POINT('Ctrl Pts',(3.58103224042604,-5.74473152449021,61.980258150987));
#24512=CARTESIAN_POINT('Ctrl Pts',(3.73516901794116,-5.64573824605703,61.9889041174779));
#24513=CARTESIAN_POINT('Ctrl Pts',(3.88515882616753,-5.54056223640278,61.9975500839688));
#24514=CARTESIAN_POINT('Ctrl Pts',(4.03495677703869,-5.43552076116312,62.0061849910931));
#24515=CARTESIAN_POINT('Ctrl Pts',(4.18061808769504,-5.32431249906942,62.0148198982175));
#24516=CARTESIAN_POINT('Ctrl Pts',(4.3216343565494,-5.20728004703913,62.0234548053419));
#24517=CARTESIAN_POINT('Ctrl Pts',(4.46733225171322,-5.08636221206021,62.0323763844134));
#24518=CARTESIAN_POINT('Ctrl Pts',(4.60807109022155,-4.95922696164353,62.0412979634849));
#24519=CARTESIAN_POINT('Ctrl Pts',(4.74332241674989,-4.82630101120496,62.0502195425565));
#24520=CARTESIAN_POINT('Ctrl Pts',(4.87386625208897,-4.69800161605849,62.0588306015322));
#24521=CARTESIAN_POINT('Ctrl Pts',(4.99929785419993,-4.56430803677536,62.0674416605079));
#24522=CARTESIAN_POINT('Ctrl Pts',(5.11917500867218,-4.42564528973869,62.0760527194836));
#24523=CARTESIAN_POINT('Ctrl Pts',(5.23893911345366,-4.2871133080738,62.0846556578331));
#24524=CARTESIAN_POINT('Ctrl Pts',(5.35315901520982,-4.14362173155766,62.0932585961827));
#24525=CARTESIAN_POINT('Ctrl Pts',(5.46142966450565,-3.99563199252104,62.1018615345322));
#24526=CARTESIAN_POINT('Ctrl Pts',(5.56957907572101,-3.84780796775702,62.110454839581));
#24527=CARTESIAN_POINT('Ctrl Pts',(5.67179234487287,-3.69549607454804,62.1190481446298));
#24528=CARTESIAN_POINT('Ctrl Pts',(5.76770487186885,-3.5391905163498,62.1276414496785));
#24529=CARTESIAN_POINT('Ctrl Pts',(5.77839109730472,-3.52177551870455,62.1285988845191));
#24530=CARTESIAN_POINT('Ctrl Pts',(5.78899914961594,-3.50431097827565,62.1295563193596));
#24531=CARTESIAN_POINT('Ctrl Pts',(5.79952855630722,-3.48679760304167,62.1305137542002));
#24532=CARTESIAN_POINT('Ctrl Pts',(5.89406055285213,-3.32956421129886,62.1391095117478));
#24533=CARTESIAN_POINT('Ctrl Pts',(5.9821391368501,-3.16857652712314,62.1477052692953));
#24534=CARTESIAN_POINT('Ctrl Pts',(6.06349327923072,-3.00438650188751,62.1563010268429));
#24535=CARTESIAN_POINT('Ctrl Pts',(6.14492332779223,-2.84004328177587,62.1649048045245));
#24536=CARTESIAN_POINT('Ctrl Pts',(6.21961627579129,-2.67249203022544,62.1735085822061));
#24537=CARTESIAN_POINT('Ctrl Pts',(6.28734900686327,-2.5023052303617,62.1821123598877));
#24538=CARTESIAN_POINT('Ctrl Pts',(6.3577436934947,-2.32542994044489,62.1910542735557));
#24539=CARTESIAN_POINT('Ctrl Pts',(6.42061988745001,-2.14570810900155,62.1999961872238));
#24540=CARTESIAN_POINT('Ctrl Pts',(6.47578430699948,-1.96379902465076,62.2089381008918));
#24541=CARTESIAN_POINT('Ctrl Pts',(6.52900721057239,-1.78829224447416,62.2175653032225));
#24542=CARTESIAN_POINT('Ctrl Pts',(6.57505189391687,-1.61074984784267,62.2261925055532));
#24543=CARTESIAN_POINT('Ctrl Pts',(6.61379707200392,-1.43177417575271,62.2348197078839));
#24544=CARTESIAN_POINT('Ctrl Pts',(6.65257914894263,-1.25262805672969,62.2434551263043));
#24545=CARTESIAN_POINT('Ctrl Pts',(6.68404778913837,-1.07204623735428,62.2520905447247));
#24546=CARTESIAN_POINT('Ctrl Pts',(6.70813331464309,-0.890638216660103,
62.2607259631452));
#24547=CARTESIAN_POINT('Ctrl Pts',(6.73225442308106,-0.708962191454703,
62.2693741391663));
#24548=CARTESIAN_POINT('Ctrl Pts',(6.7489705878499,-0.52645782899367,62.2780223151874));
#24549=CARTESIAN_POINT('Ctrl Pts',(6.75826405733234,-0.343738172698098,
62.2866704912086));
#24550=CARTESIAN_POINT('Ctrl Pts',(6.75924727116554,-0.324407125879982,
62.2875854354403));
#24551=CARTESIAN_POINT('Ctrl Pts',(6.76014745201357,-0.305073667561077,
62.2885003796721));
#24552=CARTESIAN_POINT('Ctrl Pts',(6.76096461291053,-0.285738522029537,
62.2894153239038));
#24553=CARTESIAN_POINT('Ctrl Pts',(6.76831146445643,-0.111901956468381,
62.2976413164452));
#24554=CARTESIAN_POINT('Ctrl Pts',(6.76895917775932,0.0624463016276273,
62.3058673089865));
#24555=CARTESIAN_POINT('Ctrl Pts',(6.76285728096748,0.236749651034807,62.3140933015278));
#24556=CARTESIAN_POINT('Ctrl Pts',(6.75676178122574,0.410870265909723,62.3223106701793));
#24557=CARTESIAN_POINT('Ctrl Pts',(6.74393077494341,0.584945710722264,62.3305280388307));
#24558=CARTESIAN_POINT('Ctrl Pts',(6.72436569210212,0.758416138330427,62.3387454074821));
#24559=CARTESIAN_POINT('Ctrl Pts',(6.70481720583301,0.931739415298017,62.3469558055445));
#24560=CARTESIAN_POINT('Ctrl Pts',(6.67854605984623,1.10445834317808,62.3551662036068));
#24561=CARTESIAN_POINT('Ctrl Pts',(6.64560569714577,1.27601485808894,62.3633766016692));
#24562=CARTESIAN_POINT('Ctrl Pts',(6.61268668756626,1.4474601639325,62.371581677458));
#24563=CARTESIAN_POINT('Ctrl Pts',(6.57310714014275,1.61774420715714,62.3797867532467));
#24564=CARTESIAN_POINT('Ctrl Pts',(6.5269721262206,1.78631572336455,62.3879918290355));
#24565=CARTESIAN_POINT('Ctrl Pts',(6.48085779172285,1.95481167956599,62.396193227005));
#24566=CARTESIAN_POINT('Ctrl Pts',(6.42819393926824,2.12159629321306,62.4043946249745));
#24567=CARTESIAN_POINT('Ctrl Pts',(6.36913639184669,2.28613005361773,62.412596022944));
#24568=CARTESIAN_POINT('Ctrl Pts',(6.31008347030392,2.45065092636847,62.4207967785117));
#24569=CARTESIAN_POINT('Ctrl Pts',(6.24463796408132,2.61292095715668,62.4289975340794));
#24570=CARTESIAN_POINT('Ctrl Pts',(6.17300519655273,2.77241696779778,62.4371982896471));
#24571=CARTESIAN_POINT('Ctrl Pts',(6.10137279288451,2.93191216827505,62.4453990035588));
#24572=CARTESIAN_POINT('Ctrl Pts',(6.0235533363634,3.08863304931904,62.4535997174706));
#24573=CARTESIAN_POINT('Ctrl Pts',(5.93979977772341,3.24207766726169,62.4618004313824));
#24574=CARTESIAN_POINT('Ctrl Pts',(5.85603146628133,3.39554931376427,62.470002589812));
#24575=CARTESIAN_POINT('Ctrl Pts',(5.76632714190889,3.54574323282565,62.4782047482416));
#24576=CARTESIAN_POINT('Ctrl Pts',(5.67098509493223,3.69218323665774,62.4864069066712));
#24577=CARTESIAN_POINT('Ctrl Pts',(5.57560897535943,3.83867557407474,62.4946119963241));
#24578=CARTESIAN_POINT('Ctrl Pts',(5.47459131506278,3.98141102368854,62.5028170859771));
#24579=CARTESIAN_POINT('Ctrl Pts',(5.3682730167594,4.11994342406943,62.51102217563));
#24580=CARTESIAN_POINT('Ctrl Pts',(5.2618332623702,4.2586340813391,62.5192366386278));
#24581=CARTESIAN_POINT('Ctrl Pts',(5.150080990854,4.39311181226388,62.5274511016256));
#24582=CARTESIAN_POINT('Ctrl Pts',(5.03339727842801,4.52296372277222,62.5356655646233));
#24583=CARTESIAN_POINT('Ctrl Pts',(4.91664443459033,4.6528925664334,62.5438848944308));
#24584=CARTESIAN_POINT('Ctrl Pts',(4.79495457498674,4.77818986985511,62.5521042242383));
#24585=CARTESIAN_POINT('Ctrl Pts',(4.66874465285244,4.8984806181572,62.5603235540458));
#24586=CARTESIAN_POINT('Ctrl Pts',(4.5423391760957,5.01895774968075,62.5685556192064));
#24587=CARTESIAN_POINT('Ctrl Pts',(4.41139990957234,5.13441258701736,62.5767876843671));
#24588=CARTESIAN_POINT('Ctrl Pts',(4.27637683634421,5.24451047797397,62.5850197495278));
#24589=CARTESIAN_POINT('Ctrl Pts',(4.15500840293664,5.34347436782933,62.592419320789));
#24590=CARTESIAN_POINT('Ctrl Pts',(4.03034093818189,5.43811046666926,62.5998188920503));
#24591=CARTESIAN_POINT('Ctrl Pts',(3.90271960484759,5.52820664283982,62.6072184633115));
#24592=CARTESIAN_POINT('Ctrl Pts',(3.76207289121807,5.62749827973083,62.6153732549358));
#24593=CARTESIAN_POINT('Ctrl Pts',(3.6174051020321,5.72158092630715,62.6235280465601));
#24594=CARTESIAN_POINT('Ctrl Pts',(3.46914159230921,5.81010719458001,62.6316828381844));
#24595=CARTESIAN_POINT('Ctrl Pts',(3.34813153676848,5.88236076972154,62.6383386349427));
#24596=CARTESIAN_POINT('Ctrl Pts',(3.22472693851301,5.95091355411429,62.644994431701));
#24597=CARTESIAN_POINT('Ctrl Pts',(3.09917575053255,6.01559628526641,62.6516502284592));
#24598=CARTESIAN_POINT('Origin',(0.,0.,-3.69717978381041));
#24599=CARTESIAN_POINT('',(3.09917575053256,6.01559628526641,65.0457972463573));
#24600=CARTESIAN_POINT('',(3.09917575053261,6.01559628526638,64.6514343427993));
#24601=CARTESIAN_POINT('',(3.09917575053259,6.01559628526639,-3.69717978381041));
#24602=CARTESIAN_POINT('',(-6.76699856902015,0.00440078166664134,63.6971797838431));
#24603=CARTESIAN_POINT('Ctrl Pts',(-6.76699856902015,0.00440078166665036,
63.6971797838431));
#24604=CARTESIAN_POINT('Ctrl Pts',(-6.767108590525,-0.164777201310378,63.7051406601575));
#24605=CARTESIAN_POINT('Ctrl Pts',(-6.76087012901741,-0.334158426395189,
63.713101536472));
#24606=CARTESIAN_POINT('Ctrl Pts',(-6.74826403482701,-0.503211204426377,
63.7210624127865));
#24607=CARTESIAN_POINT('Ctrl Pts',(-6.73566544902183,-0.672163292001071,
63.7290185474795));
#24608=CARTESIAN_POINT('Ctrl Pts',(-6.71670680146507,-0.840786942478803,
63.7369746821726));
#24609=CARTESIAN_POINT('Ctrl Pts',(-6.69142101104761,-1.00855037202442,
63.7449308168656));
#24610=CARTESIAN_POINT('Ctrl Pts',(-6.66614483777729,-1.17624999476154,
63.7528839255383));
#24611=CARTESIAN_POINT('Ctrl Pts',(-6.63454636505756,-1.34308967047614,
63.7608370342109));
#24612=CARTESIAN_POINT('Ctrl Pts',(-6.59671034256163,-1.50854289178017,
63.7687901428835));
#24613=CARTESIAN_POINT('Ctrl Pts',(-6.57674288147224,-1.59585864382195,
63.7729872909315));
#24614=CARTESIAN_POINT('Ctrl Pts',(-6.55503909123649,-1.68278837295603,
63.7771844389794));
#24615=CARTESIAN_POINT('Ctrl Pts',(-6.53161718373125,-1.7692557659046,63.7813815870274));
#24616=CARTESIAN_POINT('Ctrl Pts',(-6.48365191542533,-1.94633065622099,
63.7899768447874));
#24617=CARTESIAN_POINT('Ctrl Pts',(-6.42850987667823,-2.12134953563729,
63.7985721025475));
#24618=CARTESIAN_POINT('Ctrl Pts',(-6.3664016514861,-2.29373473007561,63.8071673603075));
#24619=CARTESIAN_POINT('Ctrl Pts',(-6.30423526457459,-2.46628135593908,
63.815770667162));
#24620=CARTESIAN_POINT('Ctrl Pts',(-6.23508977348513,-2.63618908665449,
63.8243739740165));
#24621=CARTESIAN_POINT('Ctrl Pts',(-6.15922374956039,-2.80290060523939,
63.8329772808709));
#24622=CARTESIAN_POINT('Ctrl Pts',(-6.08021229397599,-2.97652404119465,
63.8419372838109));
#24623=CARTESIAN_POINT('Ctrl Pts',(-5.99391132970834,-3.14668024408994,
63.8508972867509));
#24624=CARTESIAN_POINT('Ctrl Pts',(-5.90066489955293,-3.3127696483734,63.8598572896909));
#24625=CARTESIAN_POINT('Ctrl Pts',(-5.81088565084752,-3.47268335133925,
63.8684841328956));
#24626=CARTESIAN_POINT('Ctrl Pts',(-5.71466832376391,-3.62882700613723,
63.8771109761004));
#24627=CARTESIAN_POINT('Ctrl Pts',(-5.61236363058181,-3.78069616315865,
63.8857378193051));
#24628=CARTESIAN_POINT('Ctrl Pts',(-5.50996115997395,-3.9327104687042,63.8943729075912));
#24629=CARTESIAN_POINT('Ctrl Pts',(-5.40145988802639,-4.0804418742919,63.9030079958773));
#24630=CARTESIAN_POINT('Ctrl Pts',(-5.28725141460612,-4.22341822209755,
63.9116430841634));
#24631=CARTESIAN_POINT('Ctrl Pts',(-5.17287331868323,-4.36660691847247,
63.9202909972886));
#24632=CARTESIAN_POINT('Ctrl Pts',(-5.05277127917993,-4.50502621113751,
63.9289389104137));
#24633=CARTESIAN_POINT('Ctrl Pts',(-4.92737540137381,-4.63823896041766,
63.9375868235388));
#24634=CARTESIAN_POINT('Ctrl Pts',(-4.91330789280599,-4.65318340296735,
63.9385569877428));
#24635=CARTESIAN_POINT('Ctrl Pts',(-4.89917379495111,-4.66806235925509,
63.9395271519469));
#24636=CARTESIAN_POINT('Ctrl Pts',(-4.8849737418991,-4.68287524294171,63.9404973161509));
#24637=CARTESIAN_POINT('Ctrl Pts',(-4.76459114582249,-4.80845318177368,
63.9487219956697));
#24638=CARTESIAN_POINT('Ctrl Pts',(-4.63920445119171,-4.92955161938866,
63.9569466751885));
#24639=CARTESIAN_POINT('Ctrl Pts',(-4.50918025965089,-5.0457489420278,63.9651713547073));
#24640=CARTESIAN_POINT('Ctrl Pts',(-4.37929273824527,-5.16182412813523,
63.9733873891574));
#24641=CARTESIAN_POINT('Ctrl Pts',(-4.24477769190263,-5.27300822111426,
63.9816034236076));
#24642=CARTESIAN_POINT('Ctrl Pts',(-4.10603999731073,-5.37891481067367,
63.9898194580577));
#24643=CARTESIAN_POINT('Ctrl Pts',(-3.96742034232716,-5.48473129370227,
63.9980285022123));
#24644=CARTESIAN_POINT('Ctrl Pts',(-3.82458547763046,-5.58527899973977,
64.0062375463669));
#24645=CARTESIAN_POINT('Ctrl Pts',(-3.6779750017535,-5.68021028540989,64.0144465905215));
#24646=CARTESIAN_POINT('Ctrl Pts',(-3.53145990569484,-5.77507981199545,
64.0226502941495));
#24647=CARTESIAN_POINT('Ctrl Pts',(-3.38117439093799,-5.86434000225391,
64.0308539977775));
#24648=CARTESIAN_POINT('Ctrl Pts',(-3.22758889044179,-5.94768517612497,
64.0390577014056));
#24649=CARTESIAN_POINT('Ctrl Pts',(-3.07407255897636,-6.03099281451985,
64.0472577103995));
#24650=CARTESIAN_POINT('Ctrl Pts',(-2.91725951703486,-6.1083905731466,64.0554577193934));
#24651=CARTESIAN_POINT('Ctrl Pts',(-2.75764684846178,-6.17961753340519,
64.0636577283874));
#24652=CARTESIAN_POINT('Ctrl Pts',(-2.59804694285403,-6.25083879820594,
64.0718570816913));
#24653=CARTESIAN_POINT('Ctrl Pts',(-2.43564818000986,-6.31589009354785,
64.0800564349952));
#24654=CARTESIAN_POINT('Ctrl Pts',(-2.27097012292736,-6.37455752980325,
64.0882557882992));
#24655=CARTESIAN_POINT('Ctrl Pts',(-2.10629313949679,-6.43322458356442,
64.0964550881457));
#24656=CARTESIAN_POINT('Ctrl Pts',(-1.93933722878695,-6.48550773980239,
64.1046543879924));
#24657=CARTESIAN_POINT('Ctrl Pts',(-1.77063959705818,-6.53124218026936,
64.1128536878389));
#24658=CARTESIAN_POINT('Ctrl Pts',(-1.60191246178225,-6.5769846192376,64.121054421662));
#24659=CARTESIAN_POINT('Ctrl Pts',(-1.43144334463502,-6.61617596679467,
64.129255155485));
#24660=CARTESIAN_POINT('Ctrl Pts',(-1.25978224665404,-6.64870195534552,
64.137455889308));
#24661=CARTESIAN_POINT('Ctrl Pts',(-1.08805998549927,-6.68123953296759,
64.145659545068));
#24662=CARTESIAN_POINT('Ctrl Pts',(-0.915145249504272,-6.70710695399991,
64.153863200828));
#24663=CARTESIAN_POINT('Ctrl Pts',(-0.74159586278167,-6.72624148959173,
64.162066856588));
#24664=CARTESIAN_POINT('Ctrl Pts',(-0.567847664080384,-6.74539794502408,
64.170279910163));
#24665=CARTESIAN_POINT('Ctrl Pts',(-0.393463718880097,-6.75780606641138,
64.1784929637381));
#24666=CARTESIAN_POINT('Ctrl Pts',(-0.219005651738879,-6.76345514692797,
64.1867060173131));
#24667=CARTESIAN_POINT('Ctrl Pts',(-0.0444443538451033,-6.76910757013225,
64.1949239307362));
#24668=CARTESIAN_POINT('Ctrl Pts',(0.13019079550207,-6.76799298229928,64.2031418441593));
#24669=CARTESIAN_POINT('Ctrl Pts',(0.304340682312922,-6.76015279036571,
64.2113597575824));
#24670=CARTESIAN_POINT('Ctrl Pts',(0.478762184203271,-6.75230037037736,
64.2195904881783));
#24671=CARTESIAN_POINT('Ctrl Pts',(0.652696554015657,-6.7377014134082,64.2278212187743));
#24672=CARTESIAN_POINT('Ctrl Pts',(0.825590936044537,-6.71644910695534,
64.2360519493703));
#24673=CARTESIAN_POINT('Ctrl Pts',(0.984373748163748,-6.69693140520583,
64.2436108910461));
#24674=CARTESIAN_POINT('Ctrl Pts',(1.14227931093385,-6.6718027559243,64.2511698327218));
#24675=CARTESIAN_POINT('Ctrl Pts',(1.29888976933328,-6.64117266505858,64.2587287743976));
#24676=CARTESIAN_POINT('Ctrl Pts',(1.46782675082405,-6.60813173569457,64.2668826665644));
#24677=CARTESIAN_POINT('Ctrl Pts',(1.63577890605571,-6.56858639027811,64.2750365587311));
#24678=CARTESIAN_POINT('Ctrl Pts',(1.80220123910377,-6.52260375109303,64.2831904508978));
#24679=CARTESIAN_POINT('Ctrl Pts',(1.96842049040956,-6.47667722357463,64.291334393038));
#24680=CARTESIAN_POINT('Ctrl Pts',(2.13311328691637,-6.42432913476805,64.2994783351782));
#24681=CARTESIAN_POINT('Ctrl Pts',(2.29574222967256,-6.36567801690425,64.3076222773184));
#24682=CARTESIAN_POINT('Ctrl Pts',(2.45820694983116,-6.30708612490004,64.3157579957113));
#24683=CARTESIAN_POINT('Ctrl Pts',(2.61861162384944,-6.24220399800913,64.3238937141042));
#24684=CARTESIAN_POINT('Ctrl Pts',(2.77643149132963,-6.1712006266166,64.3320294324971));
#24685=CARTESIAN_POINT('Ctrl Pts',(2.93412518986032,-6.10025401880475,64.3401586467973));
#24686=CARTESIAN_POINT('Ctrl Pts',(3.08923786441552,-6.0231960595287,64.3482878610975));
#24687=CARTESIAN_POINT('Ctrl Pts',(3.24126231487832,-5.94024474295038,64.3564170753977));
#24688=CARTESIAN_POINT('Ctrl Pts',(3.39319719455959,-5.85734230018304,64.3645415000731));
#24689=CARTESIAN_POINT('Ctrl Pts',(3.54204715351871,-5.76855358973366,64.3726659247485));
#24690=CARTESIAN_POINT('Ctrl Pts',(3.68732730335867,-5.67414366736565,64.3807903494239));
#24691=CARTESIAN_POINT('Ctrl Pts',(3.83348939671183,-5.57916061633067,64.3889640945581));
#24692=CARTESIAN_POINT('Ctrl Pts',(3.97603785477099,-5.47848803534081,64.3971378396923));
#24693=CARTESIAN_POINT('Ctrl Pts',(4.11450580585539,-5.37244180737049,64.4053115848265));
#24694=CARTESIAN_POINT('Ctrl Pts',(4.25208704869958,-5.26707466841282,64.4134329876886));
#24695=CARTESIAN_POINT('Ctrl Pts',(4.38563961262473,-5.15640274723064,64.4215543905508));
#24696=CARTESIAN_POINT('Ctrl Pts',(4.51473655633834,-5.04077799817272,64.4296757934129));
#24697=CARTESIAN_POINT('Ctrl Pts',(4.64384348114784,-4.92514430961807,64.4377978241792));
#24698=CARTESIAN_POINT('Ctrl Pts',(4.7684938269026,-4.80455727457664,64.4459198549454));
#24699=CARTESIAN_POINT('Ctrl Pts',(4.88829573248609,-4.67940742314219,64.4540418857117));
#24700=CARTESIAN_POINT('Ctrl Pts',(5.00812971357128,-4.55422406435866,64.4621660910528));
#24701=CARTESIAN_POINT('Ctrl Pts',(5.12311241673919,-4.42447572094981,64.4702902963939));
#24702=CARTESIAN_POINT('Ctrl Pts',(5.23289070154551,-4.29058782752184,64.478414501735));
#24703=CARTESIAN_POINT('Ctrl Pts',(5.34385726032461,-4.15525069029021,64.4866266459775));
#24704=CARTESIAN_POINT('Ctrl Pts',(5.44950583014637,-4.01568416011006,64.4948387902199));
#24705=CARTESIAN_POINT('Ctrl Pts',(5.54951570161092,-3.87235903262777,64.5030509344624));
#24706=CARTESIAN_POINT('Ctrl Pts',(5.64861259317411,-3.7303423055947,64.5111881108788));
#24707=CARTESIAN_POINT('Ctrl Pts',(5.74217316368213,-3.58463566111503,64.5193252872953));
#24708=CARTESIAN_POINT('Ctrl Pts',(5.82993113162976,-3.43572292253816,64.5274624637117));
#24709=CARTESIAN_POINT('Ctrl Pts',(5.91890187113345,-3.28475228383092,64.5357120918672));
#24710=CARTESIAN_POINT('Ctrl Pts',(6.00190826949739,-3.13048663444368,64.5439617200226));
#24711=CARTESIAN_POINT('Ctrl Pts',(6.07872300777909,-2.97345179794413,64.5522113481781));
#24712=CARTESIAN_POINT('Ctrl Pts',(6.15553774606078,-2.81641696144457,64.5604609763335));
#24713=CARTESIAN_POINT('Ctrl Pts',(6.22616072658722,-2.65661331534446,64.5687106044889));
#24714=CARTESIAN_POINT('Ctrl Pts',(6.29041691467294,-2.49458293900937,64.5769602326444));
#24715=CARTESIAN_POINT('Ctrl Pts',(6.35448024389379,-2.33303888150807,64.585185100322));
#24716=CARTESIAN_POINT('Ctrl Pts',(6.41240659834632,-2.16879863247724,64.5934099679995));
#24717=CARTESIAN_POINT('Ctrl Pts',(6.46396227940405,-2.00236875985461,64.6016348356771));
#24718=CARTESIAN_POINT('Ctrl Pts',(6.51545987721636,-1.83612638911222,64.6098504371206));
#24719=CARTESIAN_POINT('Ctrl Pts',(6.56060098822739,-1.66769964649672,64.6180660385642));
#24720=CARTESIAN_POINT('Ctrl Pts',(6.59919968439063,-1.49761561341308,64.6262816400077));
#24721=CARTESIAN_POINT('Ctrl Pts',(6.63776265005493,-1.32768902573478,64.6344896363359));
#24722=CARTESIAN_POINT('Ctrl Pts',(6.66979518313659,-1.15610855052929,64.642697632664));
#24723=CARTESIAN_POINT('Ctrl Pts',(6.69516092787743,-0.983417078265128,
64.6509056289921));
#24724=CARTESIAN_POINT('Ctrl Pts',(6.72050828659645,-0.810850779111668,
64.6591076758636));
#24725=CARTESIAN_POINT('Ctrl Pts',(6.73919843014089,-0.637175440410905,
64.667309722735));
#24726=CARTESIAN_POINT('Ctrl Pts',(6.75114590405125,-0.462944901918249,
64.6755117696065));
#24727=CARTESIAN_POINT('Ctrl Pts',(6.76308711715413,-0.288805665056759,
64.683709518378));
#24728=CARTESIAN_POINT('Ctrl Pts',(6.76829267512614,-0.114112165085269,
64.6919072671496));
#24729=CARTESIAN_POINT('Ctrl Pts',(6.76672886816929,0.0605757763829547,
64.7001050159211));
#24730=CARTESIAN_POINT('Ctrl Pts',(6.76516535947721,0.235230399634836,64.7083012011367));
#24731=CARTESIAN_POINT('Ctrl Pts',(6.75683505459466,0.409879108046038,64.7164973863524));
#24732=CARTESIAN_POINT('Ctrl Pts',(6.74175634871382,0.583960901582418,64.724693571568));
#24733=CARTESIAN_POINT('Ctrl Pts',(6.72667875832161,0.758029816940473,64.7328891504484));
#24734=CARTESIAN_POINT('Ctrl Pts',(6.70485379123764,0.931531543383801,64.7410847293287));
#24735=CARTESIAN_POINT('Ctrl Pts',(6.67635182832526,1.10390908340225,64.7492803082091));
#24736=CARTESIAN_POINT('Ctrl Pts',(6.64784678832906,1.27630523337192,64.7574767718875));
#24737=CARTESIAN_POINT('Ctrl Pts',(6.61266337489708,1.44757660101982,64.765673235566));
#24738=CARTESIAN_POINT('Ctrl Pts',(6.57092332096869,1.61717522549347,64.7738696992444));
#24739=CARTESIAN_POINT('Ctrl Pts',(6.52917116662659,1.78682301649487,64.7820685390722));
#24740=CARTESIAN_POINT('Ctrl Pts',(6.48085867143856,1.95479675006364,64.7902673789));
#24741=CARTESIAN_POINT('Ctrl Pts',(6.42615778718546,2.12056244760574,64.7984662187278));
#24742=CARTESIAN_POINT('Ctrl Pts',(6.37139976630256,2.28650129213487,64.806673622477));
#24743=CARTESIAN_POINT('Ctrl Pts',(6.31024013745913,2.45022715162502,64.8148810262263));
#24744=CARTESIAN_POINT('Ctrl Pts',(6.24289984237217,2.61122395786143,64.8230884299755));
#24745=CARTESIAN_POINT('Ctrl Pts',(6.17552347625953,2.77230700250717,64.8313002300446));
#24746=CARTESIAN_POINT('Ctrl Pts',(6.10195999499159,2.93065775459247,64.8395120301136));
#24747=CARTESIAN_POINT('Ctrl Pts',(6.02247685234882,3.08578378421474,64.8477238301826));
#24748=CARTESIAN_POINT('Ctrl Pts',(5.94287669941409,3.24113818102802,64.8559477191688));
#24749=CARTESIAN_POINT('Ctrl Pts',(5.85733964515753,3.39325805536864,64.8641716081549));
#24750=CARTESIAN_POINT('Ctrl Pts',(5.76617778938328,3.54167794995859,64.8723954971411));
#24751=CARTESIAN_POINT('Ctrl Pts',(5.68194581063761,3.67881536670334,64.8799942283911));
#24752=CARTESIAN_POINT('Ctrl Pts',(5.59291229325792,3.81279409181644,64.8875929596412));
#24753=CARTESIAN_POINT('Ctrl Pts',(5.49935390779853,3.94327219410239,64.8951916908913));
#24754=CARTESIAN_POINT('Ctrl Pts',(5.3980829195581,4.08450642230494,64.903416833077));
#24755=CARTESIAN_POINT('Ctrl Pts',(5.29122553709665,4.22203511372218,64.9116419752628));
#24756=CARTESIAN_POINT('Ctrl Pts',(5.17908162278455,4.35538776052551,64.9198671174485));
#24757=CARTESIAN_POINT('Ctrl Pts',(5.06705998759757,4.48859500269335,64.9280832911298));
#24758=CARTESIAN_POINT('Ctrl Pts',(4.94976352614232,4.61763499403864,64.9362994648111));
#24759=CARTESIAN_POINT('Ctrl Pts',(4.82753522675317,4.74206628322056,64.9445156384924));
#24760=CARTESIAN_POINT('Ctrl Pts',(4.7019751711756,4.86988937871769,64.9529557724812));
#24761=CARTESIAN_POINT('Ctrl Pts',(4.57121077534139,4.99284861819941,64.9613959064699));
#24762=CARTESIAN_POINT('Ctrl Pts',(4.43565908084522,5.11050071113539,64.9698360404586));
#24763=CARTESIAN_POINT('Ctrl Pts',(4.30393800121349,5.22482802190831,64.9780376609944));
#24764=CARTESIAN_POINT('Ctrl Pts',(4.16769680793882,5.33414380210309,64.9862392815301));
#24765=CARTESIAN_POINT('Ctrl Pts',(4.02735618745112,5.4380778901556,64.9944409020658));
#24766=CARTESIAN_POINT('Ctrl Pts',(3.88089364401347,5.54654577944627,65.0030002927811));
#24767=CARTESIAN_POINT('Ctrl Pts',(3.7299662655183,5.64915161858864,65.0115596834963));
#24768=CARTESIAN_POINT('Ctrl Pts',(3.57509119478739,5.74552103372303,65.0201190742116));
#24769=CARTESIAN_POINT('Ctrl Pts',(3.42021612405647,5.84189044885741,65.0286784649268));
#24770=CARTESIAN_POINT('Ctrl Pts',(3.26139372758728,5.93202318678242,65.0372378556421));
#24771=CARTESIAN_POINT('Ctrl Pts',(3.09917575053256,6.01559628526641,65.0457972463573));
#24772=CARTESIAN_POINT('Ctrl Pts',(3.09917575053259,6.01559628526639,63.0459622914914));
#24773=CARTESIAN_POINT('Ctrl Pts',(2.94550623433066,6.09476530120842,63.0540930631184));
#24774=CARTESIAN_POINT('Ctrl Pts',(2.78865426101915,6.168117870594,63.0622238347455));
#24775=CARTESIAN_POINT('Ctrl Pts',(2.6291048227603,6.23539067187763,63.0703546063725));
#24776=CARTESIAN_POINT('Ctrl Pts',(2.46965807767459,6.30262017336964,63.0784801446703));
#24777=CARTESIAN_POINT('Ctrl Pts',(2.30751766087169,6.36377755756109,63.0866056829681));
#24778=CARTESIAN_POINT('Ctrl Pts',(2.14319177109584,6.41864612144236,63.0947312212659));
#24779=CARTESIAN_POINT('Ctrl Pts',(1.97893710493117,6.47349090369515,63.1028532377195));
#24780=CARTESIAN_POINT('Ctrl Pts',(1.81249919881251,6.52205217898337,63.1109752541731));
#24781=CARTESIAN_POINT('Ctrl Pts',(1.64440476370505,6.56416193989028,63.1190972706267));
#24782=CARTESIAN_POINT('Ctrl Pts',(1.47631779800722,6.60626982961655,63.127218926172));
#24783=CARTESIAN_POINT('Ctrl Pts',(1.30657480222966,6.64192667751996,63.1353405817174));
#24784=CARTESIAN_POINT('Ctrl Pts',(1.13571641098715,6.67101470795969,63.1434622372628));
#24785=CARTESIAN_POINT('Ctrl Pts',(0.964853172710025,6.70010356358973,63.1515841232091));
#24786=CARTESIAN_POINT('Ctrl Pts',(0.792874836639891,6.72262316836435,63.1597060091555));
#24787=CARTESIAN_POINT('Ctrl Pts',(0.620330728893733,6.7385071630733,63.1678278951018));
#24788=CARTESIAN_POINT('Ctrl Pts',(0.447748870088166,6.7543946330538,63.1759515580419));
#24789=CARTESIAN_POINT('Ctrl Pts',(0.274601357510065,6.76364356823193,63.1840752209821));
#24790=CARTESIAN_POINT('Ctrl Pts',(0.101441073081922,6.76623962838237,63.1921988839222));
#24791=CARTESIAN_POINT('Ctrl Pts',(-0.0717900733916588,6.76883675091344,
63.200325871293));
#24792=CARTESIAN_POINT('Ctrl Pts',(-0.245033636566598,6.76477557157275,
63.2084528586638));
#24793=CARTESIAN_POINT('Ctrl Pts',(-0.417738348494154,6.75409384537981,
63.2165798460347));
#24794=CARTESIAN_POINT('Ctrl Pts',(-0.590646486797809,6.74339953733646,
63.2247164060661));
#24795=CARTESIAN_POINT('Ctrl Pts',(-0.763014140958481,6.72606913119763,
63.2328529660975));
#24796=CARTESIAN_POINT('Ctrl Pts',(-0.934295864837633,6.70219219635988,
63.240989526129));
#24797=CARTESIAN_POINT('Ctrl Pts',(-1.10568971810508,6.67829963051354,63.2491314127503));
#24798=CARTESIAN_POINT('Ctrl Pts',(-1.27599586574884,6.64785206168226,63.2572732993716));
#24799=CARTESIAN_POINT('Ctrl Pts',(-1.44468094551783,6.61098978713912,63.2654151859929));
#24800=CARTESIAN_POINT('Ctrl Pts',(-1.61361837281639,6.57407236780233,63.2735692526184));
#24801=CARTESIAN_POINT('Ctrl Pts',(-1.78092953606017,6.53072116885973,63.2817233192439));
#24802=CARTESIAN_POINT('Ctrl Pts',(-1.94609709820228,6.48112606607592,63.2898773858694));
#24803=CARTESIAN_POINT('Ctrl Pts',(-2.04168455420969,6.45242388240227,63.2945963904653));
#24804=CARTESIAN_POINT('Ctrl Pts',(-2.13655442647952,6.42163133589962,63.2993153950612));
#24805=CARTESIAN_POINT('Ctrl Pts',(-2.23060992106565,6.38879240389321,63.3040343996572));
#24806=CARTESIAN_POINT('Ctrl Pts',(-2.39467913819437,6.33150858555442,63.312266171688));
#24807=CARTESIAN_POINT('Ctrl Pts',(-2.55678115665872,6.26781647570823,63.3204979437188));
#24808=CARTESIAN_POINT('Ctrl Pts',(-2.71637917710084,6.19786843731076,63.3287297157497));
#24809=CARTESIAN_POINT('Ctrl Pts',(-2.87578662155742,6.12800392386127,63.3369516582221));
#24810=CARTESIAN_POINT('Ctrl Pts',(-3.03269569687596,6.05189849917589,63.3451736006945));
#24811=CARTESIAN_POINT('Ctrl Pts',(-3.18658507162592,5.96975414747465,63.3533955431669));
#24812=CARTESIAN_POINT('Ctrl Pts',(-3.340321520173,5.88769142599522,63.3616093151568));
#24813=CARTESIAN_POINT('Ctrl Pts',(-3.49104393031614,5.79960189629139,63.3698230871467));
#24814=CARTESIAN_POINT('Ctrl Pts',(-3.63825118030288,5.70573547836076,63.3780368591366));
#24815=CARTESIAN_POINT('Ctrl Pts',(-3.78534162794163,5.61194353922118,63.3862441138669));
#24816=CARTESIAN_POINT('Ctrl Pts',(-3.92892216999375,5.51238403337113,63.3944513685973));
#24817=CARTESIAN_POINT('Ctrl Pts',(-4.06851644748125,5.40735267174008,63.4026586233277));
#24818=CARTESIAN_POINT('Ctrl Pts',(-4.20802791466854,5.30238361695101,63.4108610093396));
#24819=CARTESIAN_POINT('Ctrl Pts',(-4.34355754257503,5.19194938769162,63.4190633953516));
#24820=CARTESIAN_POINT('Ctrl Pts',(-4.47465805488804,5.07638890273643,63.4272657813635));
#24821=CARTESIAN_POINT('Ctrl Pts',(-4.60571943687818,4.9608629097829,63.4354657191622));
#24822=CARTESIAN_POINT('Ctrl Pts',(-4.73235406559019,4.84021394268184,63.4436656569609));
#24823=CARTESIAN_POINT('Ctrl Pts',(-4.85414767600162,4.71482124152847,63.4518655947596));
#24824=CARTESIAN_POINT('Ctrl Pts',(-4.97592425652285,4.58944607351109,63.4600643859954));
#24825=CARTESIAN_POINT('Ctrl Pts',(-5.09286091665338,4.45932874893275,63.4682631772311));
#24826=CARTESIAN_POINT('Ctrl Pts',(-5.2045802034484,4.32488542112656,63.4764619684669));
#24827=CARTESIAN_POINT('Ctrl Pts',(-5.31630413546221,4.19043650325002,63.4846611006033));
#24828=CARTESIAN_POINT('Ctrl Pts',(-5.4228100328044,4.05166149943201,63.4928602327397));
#24829=CARTESIAN_POINT('Ctrl Pts',(-5.52376066847092,3.90900973105129,63.5010593648761));
#24830=CARTESIAN_POINT('Ctrl Pts',(-5.62473381450443,3.76632615362217,63.509260325287));
#24831=CARTESIAN_POINT('Ctrl Pts',(-5.72014902465459,3.61976438240121,63.517461285698));
#24832=CARTESIAN_POINT('Ctrl Pts',(-5.80971232107568,3.46980283969298,63.5256622461089));
#24833=CARTESIAN_POINT('Ctrl Pts',(-5.89935955986601,3.31970074691911,63.5338708927939));
#24834=CARTESIAN_POINT('Ctrl Pts',(-5.98314374290121,3.1661928245452,63.5420795394789));
#24835=CARTESIAN_POINT('Ctrl Pts',(-6.06081635948654,3.00978305805923,63.550288186164));
#24836=CARTESIAN_POINT('Ctrl Pts',(-6.13852605916045,2.85329861715798,63.5585007518875));
#24837=CARTESIAN_POINT('Ctrl Pts',(-6.21011822793787,2.69390989663681,63.566713317611));
#24838=CARTESIAN_POINT('Ctrl Pts',(-6.27539252680471,2.53214091916774,63.5749258833345));
#24839=CARTESIAN_POINT('Ctrl Pts',(-6.34075639142878,2.37014997131804,63.5831497178833));
#24840=CARTESIAN_POINT('Ctrl Pts',(-6.39978493946788,2.20577257659968,63.591373552432));
#24841=CARTESIAN_POINT('Ctrl Pts',(-6.45232735118248,2.03954915439232,63.5995973869808));
#24842=CARTESIAN_POINT('Ctrl Pts',(-6.50060394385643,1.88682109747779,63.6071535439552));
#24843=CARTESIAN_POINT('Ctrl Pts',(-6.54340536908842,1.73253496099723,63.6147097009296));
#24844=CARTESIAN_POINT('Ctrl Pts',(-6.58065285209234,1.57711668567957,63.622265857904));
#24845=CARTESIAN_POINT('Ctrl Pts',(-6.63190660814036,1.3632560506483,63.6326633772796));
#24846=CARTESIAN_POINT('Ctrl Pts',(-6.67274538650549,1.14683583986141,63.6430608966552));
#24847=CARTESIAN_POINT('Ctrl Pts',(-6.70296292886345,0.928750221686325,
63.6534584160308));
#24848=CARTESIAN_POINT('Ctrl Pts',(-6.732835253359,0.713156104972025,63.6637371497894));
#24849=CARTESIAN_POINT('Ctrl Pts',(-6.75232765311494,0.495934283327142,
63.674015883548));
#24850=CARTESIAN_POINT('Ctrl Pts',(-6.76128863461862,0.277965824116989,
63.6842946173066));
#24851=CARTESIAN_POINT('Ctrl Pts',(-6.76503305623774,0.186885867014341,
63.6885896728077));
#24852=CARTESIAN_POINT('Ctrl Pts',(-6.76693921015938,0.0956757623781489,
63.6928847283089));
#24853=CARTESIAN_POINT('Ctrl Pts',(-6.76699856901969,0.00440078236972949,
63.69717978381));
#24854=CARTESIAN_POINT('',(-6.76699754938808,0.00575904295465441,63.3028202162211));
#24855=CARTESIAN_POINT('Ctrl Pts',(3.09917575053255,6.01559628526641,62.6516502284592));
#24856=CARTESIAN_POINT('Ctrl Pts',(2.94565184939477,6.09469028176659,62.6597889318832));
#24857=CARTESIAN_POINT('Ctrl Pts',(2.78891768509697,6.16799628340453,62.6679276353073));
#24858=CARTESIAN_POINT('Ctrl Pts',(2.6294535729494,6.23524361253862,62.6760663387313));
#24859=CARTESIAN_POINT('Ctrl Pts',(2.47012263887975,6.30243477938065,62.6841982450343));
#24860=CARTESIAN_POINT('Ctrl Pts',(2.30806663153626,6.36357720714301,62.6923301513372));
#24861=CARTESIAN_POINT('Ctrl Pts',(2.1437899634967,6.418446353473,62.7004620576402));
#24862=CARTESIAN_POINT('Ctrl Pts',(1.97961598145489,6.47328120221768,62.7085888808542));
#24863=CARTESIAN_POINT('Ctrl Pts',(1.81322444865879,6.52185046297917,62.7167157040682));
#24864=CARTESIAN_POINT('Ctrl Pts',(1.6451392279764,6.56397790372372,62.7248425272822));
#24865=CARTESIAN_POINT('Ctrl Pts',(1.47262848185054,6.60721452027877,62.7331833220921));
#24866=CARTESIAN_POINT('Ctrl Pts',(1.29833399745046,6.64366528018179,62.7415241169019));
#24867=CARTESIAN_POINT('Ctrl Pts',(1.1228388075019,6.67319428852238,62.7498649117118));
#24868=CARTESIAN_POINT('Ctrl Pts',(0.951923374720132,6.70195270202436,62.7579880434916));
#24869=CARTESIAN_POINT('Ctrl Pts',(0.779869504139152,6.72414606989112,62.7661111752714));
#24870=CARTESIAN_POINT('Ctrl Pts',(0.607225751379997,6.73970072680242,62.7742343070512));
#24871=CARTESIAN_POINT('Ctrl Pts',(0.434573703316043,6.75525613109448,62.7823578291368));
#24872=CARTESIAN_POINT('Ctrl Pts',(0.261332080946672,6.76417215593664,62.7904813512224));
#24873=CARTESIAN_POINT('Ctrl Pts',(0.0880539029469755,6.76642708600158,
62.798604873308));
#24874=CARTESIAN_POINT('Ctrl Pts',(-0.0852655664839576,6.76868255340648,
62.8067303311933));
#24875=CARTESIAN_POINT('Ctrl Pts',(-0.258621243203989,6.76427376061019,
62.8148557890786));
#24876=CARTESIAN_POINT('Ctrl Pts',(-0.431460810487573,6.75323112065724,
62.8229812469639));
#24877=CARTESIAN_POINT('Ctrl Pts',(-0.612338934353396,6.74167490104499,
62.8314846099435));
#24878=CARTESIAN_POINT('Ctrl Pts',(-0.792651343496034,6.72285303507262,
62.8399879729232));
#24879=CARTESIAN_POINT('Ctrl Pts',(-0.97177279733705,6.69686095348826,62.8484913359028));
#24880=CARTESIAN_POINT('Ctrl Pts',(-1.14320331372459,6.67198489385139,62.8566295900056));
#24881=CARTESIAN_POINT('Ctrl Pts',(-1.31354266533925,6.64054162568567,62.8647678441084));
#24882=CARTESIAN_POINT('Ctrl Pts',(-1.4822551784215,6.60266677835878,62.8729060982112));
#24883=CARTESIAN_POINT('Ctrl Pts',(-1.65108271136965,6.56476610983,62.881049900574));
#24884=CARTESIAN_POINT('Ctrl Pts',(-1.81828084427154,6.52042522003151,62.8891937029369));
#24885=CARTESIAN_POINT('Ctrl Pts',(-1.98333029704277,6.46982920430147,62.8973375052997));
#24886=CARTESIAN_POINT('Ctrl Pts',(-2.14859502525585,6.4191671957465,62.9054919296951));
#24887=CARTESIAN_POINT('Ctrl Pts',(-2.31170513660626,6.36223389716979,62.9136463540905));
#24888=CARTESIAN_POINT('Ctrl Pts',(-2.47216188947549,6.29926222602496,62.9218007784858));
#24889=CARTESIAN_POINT('Ctrl Pts',(-2.49328755790541,6.29097140235257,62.9228743865636));
#24890=CARTESIAN_POINT('Ctrl Pts',(-2.51436726845114,6.28257597265725,62.9239479946414));
#24891=CARTESIAN_POINT('Ctrl Pts',(-2.53539991657681,6.27407652671071,62.9250216027191));
#24892=CARTESIAN_POINT('Ctrl Pts',(-2.69655645961628,6.20895199658447,62.9332478120561));
#24893=CARTESIAN_POINT('Ctrl Pts',(-2.85542747637427,6.13752321639356,62.9414740213931));
#24894=CARTESIAN_POINT('Ctrl Pts',(-3.01148497277787,6.05997089586519,62.94970023073));
#24895=CARTESIAN_POINT('Ctrl Pts',(-3.16736714526967,5.98250570204663,62.9579171982732));
#24896=CARTESIAN_POINT('Ctrl Pts',(-3.32044177330885,5.89893082506714,62.9661341658164));
#24897=CARTESIAN_POINT('Ctrl Pts',(-3.47019900586617,5.80947569576511,62.9743511333596));
#24898=CARTESIAN_POINT('Ctrl Pts',(-3.61981805006439,5.72010311110763,62.982560518703));
#24899=CARTESIAN_POINT('Ctrl Pts',(-3.76612548916819,5.62486126296155,62.9907699040464));
#24900=CARTESIAN_POINT('Ctrl Pts',(-3.90863426053248,5.52402635922311,62.9989792893898));
#24901=CARTESIAN_POINT('Ctrl Pts',(-4.05104012552073,5.42326426892922,63.0071827466903));
#24902=CARTESIAN_POINT('Ctrl Pts',(-4.18965249485716,5.31691737390216,63.0153862039909));
#24903=CARTESIAN_POINT('Ctrl Pts',(-4.32401152580629,5.20530626617631,63.0235896612915));
#24904=CARTESIAN_POINT('Ctrl Pts',(-4.45830048744434,5.09375336453734,63.0317888404233));
#24905=CARTESIAN_POINT('Ctrl Pts',(-4.58834025443122,4.97694194800198,63.0399880195552));
#24906=CARTESIAN_POINT('Ctrl Pts',(-4.7137023782453,4.85523417450947,63.0481871986871));
#24907=CARTESIAN_POINT('Ctrl Pts',(-4.8390408811333,4.73354933338466,63.0563848329169));
#24908=CARTESIAN_POINT('Ctrl Pts',(-4.95970323506052,4.6069702180812,63.0645824671467));
#24909=CARTESIAN_POINT('Ctrl Pts',(-5.07529610806809,4.47589749831572,63.0727801013765));
#24910=CARTESIAN_POINT('Ctrl Pts',(-5.19088063745551,4.34483423952268,63.0809771438921));
#24911=CARTESIAN_POINT('Ctrl Pts',(-5.30139617677094,4.20927829066182,63.0891741864077));
#24912=CARTESIAN_POINT('Ctrl Pts',(-5.40648817564024,4.06966517132089,63.0973712289233));
#24913=CARTESIAN_POINT('Ctrl Pts',(-5.5115916891486,3.9300367549574,63.1055691695661));
#24914=CARTESIAN_POINT('Ctrl Pts',(-5.61127026255347,3.78635056910221,63.1137671102089));
#24915=CARTESIAN_POINT('Ctrl Pts',(-5.70521133069505,3.63907305121907,63.1219650508518));
#24916=CARTESIAN_POINT('Ctrl Pts',(-5.79917976539459,3.49175262900442,63.1301653796878));
#24917=CARTESIAN_POINT('Ctrl Pts',(-5.88740717270984,3.34083909315635,63.1383657085238));
#24918=CARTESIAN_POINT('Ctrl Pts',(-5.96962576769131,3.18682556687935,63.1465660373598));
#24919=CARTESIAN_POINT('Ctrl Pts',(-6.05193003658202,3.0326515545119,63.1547749111512));
#24920=CARTESIAN_POINT('Ctrl Pts',(-6.12821281479293,2.87537141495665,63.1629837849426));
#24921=CARTESIAN_POINT('Ctrl Pts',(-6.19825309286485,2.71550135275079,63.171192658734));
#24922=CARTESIAN_POINT('Ctrl Pts',(-6.26833096078139,2.55554549004607,63.1794059381374));
#24923=CARTESIAN_POINT('Ctrl Pts',(-6.33215951868453,2.3929972672502,63.1876192175408));
#24924=CARTESIAN_POINT('Ctrl Pts',(-6.38956696334292,2.22839023085202,63.1958324969443));
#24925=CARTESIAN_POINT('Ctrl Pts',(-6.44705837541194,2.06354243079159,63.2040577895597));
#24926=CARTESIAN_POINT('Ctrl Pts',(-6.49810980025971,1.8966301421379,63.2122830821752));
#24927=CARTESIAN_POINT('Ctrl Pts',(-6.54259976850742,1.7282005870635,63.2205083747906));
#24928=CARTESIAN_POINT('Ctrl Pts',(-6.5828356004554,1.57587628700304,63.2279471639027));
#24929=CARTESIAN_POINT('Ctrl Pts',(-6.61770542251439,1.42231133974596,63.2353859530148));
#24930=CARTESIAN_POINT('Ctrl Pts',(-6.64715585439012,1.26791484234833,63.2428247421268));
#24931=CARTESIAN_POINT('Ctrl Pts',(-6.69446442975949,1.01989544607171,63.2547742618096));
#24932=CARTESIAN_POINT('Ctrl Pts',(-6.7279021089193,0.769153761022326,63.2667237814924));
#24933=CARTESIAN_POINT('Ctrl Pts',(-6.74722475137883,0.516959528765004,
63.2786733011752));
#24934=CARTESIAN_POINT('Ctrl Pts',(-6.76024011985427,0.347086238034466,
63.2867222728467));
#24935=CARTESIAN_POINT('Ctrl Pts',(-6.76685219440396,0.176554210769674,
63.2947712445183));
#24936=CARTESIAN_POINT('Ctrl Pts',(-6.76699754938751,0.00575904361896699,
63.3028202161898));
#24937=CARTESIAN_POINT('Ctrl Pts',(-6.76699754938808,0.00575904295474457,
63.3028202162211));
#24938=CARTESIAN_POINT('Ctrl Pts',(-6.76714384492322,-0.166141311942916,
63.3109212714791));
#24939=CARTESIAN_POINT('Ctrl Pts',(-6.76073587822894,-0.338250077316013,
63.3190223267372));
#24940=CARTESIAN_POINT('Ctrl Pts',(-6.74775279763134,-0.510020766301218,
63.3271233819952));
#24941=CARTESIAN_POINT('Ctrl Pts',(-6.73478004839695,-0.681654767744205,
63.3352179907906));
#24942=CARTESIAN_POINT('Ctrl Pts',(-6.71524262925384,-0.852950861782448,
63.343312599586));
#24943=CARTESIAN_POINT('Ctrl Pts',(-6.68917174575775,-1.02336227981893,
63.3514072083814));
#24944=CARTESIAN_POINT('Ctrl Pts',(-6.66311601068548,-1.19367468071303,
63.3594971138239));
#24945=CARTESIAN_POINT('Ctrl Pts',(-6.63053442608599,-1.36310306491456,
63.3675870192664));
#24946=CARTESIAN_POINT('Ctrl Pts',(-6.5915100512617,-1.53110556269516,63.3756769247089));
#24947=CARTESIAN_POINT('Ctrl Pts',(-6.55249553017716,-1.69906563947865,
63.3837647874327));
#24948=CARTESIAN_POINT('Ctrl Pts',(-6.50704153611983,-1.86560018592668,
63.3918526501564));
#24949=CARTESIAN_POINT('Ctrl Pts',(-6.45528230229601,-2.03017718381032,
63.3999405128801));
#24950=CARTESIAN_POINT('Ctrl Pts',(-6.40352824864249,-2.19473771049037,
63.408027566154));
#24951=CARTESIAN_POINT('Ctrl Pts',(-6.34547032152564,-2.3573407257823,63.4161146194278));
#24952=CARTESIAN_POINT('Ctrl Pts',(-6.28129268559602,-2.51746920495126,
63.4242016727017));
#24953=CARTESIAN_POINT('Ctrl Pts',(-6.21710899763722,-2.67761278443071,
63.4322894885945));
#24954=CARTESIAN_POINT('Ctrl Pts',(-6.14680458952733,-2.83528102006325,
63.4403773044873));
#24955=CARTESIAN_POINT('Ctrl Pts',(-6.07061180844132,-2.98997680111615,
63.4484651203801));
#24956=CARTESIAN_POINT('Ctrl Pts',(-5.99439703007437,-3.14471724370401,
63.4565552712705));
#24957=CARTESIAN_POINT('Ctrl Pts',(-5.91229065799742,-3.29648319201542,
63.4646454221609));
#24958=CARTESIAN_POINT('Ctrl Pts',(-5.82457097603429,-3.44480216342521,
63.4727355730513));
#24959=CARTESIAN_POINT('Ctrl Pts',(-5.7367623042207,-3.59327160144396,63.4808339312368));
#24960=CARTESIAN_POINT('Ctrl Pts',(-5.643329138574,-3.73828676081582,63.4889322894223));
#24961=CARTESIAN_POINT('Ctrl Pts',(-5.54459350453892,-3.87940354557564,
63.4970306476078));
#24962=CARTESIAN_POINT('Ctrl Pts',(-5.44580282713146,-4.02059900045095,
63.505133520485));
#24963=CARTESIAN_POINT('Ctrl Pts',(-5.34170401533324,-4.15789145744062,
63.5132363933622));
#24964=CARTESIAN_POINT('Ctrl Pts',(-5.23265910186198,-4.29087027579499,
63.5213392662394));
#24965=CARTESIAN_POINT('Ctrl Pts',(-5.12346411066267,-4.42403211193811,
63.529453291042));
#24966=CARTESIAN_POINT('Ctrl Pts',(-5.00930966717568,-4.55286817695293,
63.5375673158447));
#24967=CARTESIAN_POINT('Ctrl Pts',(-4.89059495869637,-4.67700437780142,
63.5456813406474));
#24968=CARTESIAN_POINT('Ctrl Pts',(-4.81770165410644,-4.75322659167025,
63.5506635209431));
#24969=CARTESIAN_POINT('Ctrl Pts',(-4.74308971382623,-4.82767762154433,
63.5556457012388));
#24970=CARTESIAN_POINT('Ctrl Pts',(-4.66685749085739,-4.90027857983893,
63.5606278815345));
#24971=CARTESIAN_POINT('Ctrl Pts',(-4.54211542089365,-5.01907865500823,
63.5687804377477));
#24972=CARTESIAN_POINT('Ctrl Pts',(-4.41263899382622,-5.13329826570113,
63.576932993961));
#24973=CARTESIAN_POINT('Ctrl Pts',(-4.27880063039264,-5.24253318209352,
63.5850855501743));
#24974=CARTESIAN_POINT('Ctrl Pts',(-4.14511732192962,-5.35164154720187,
63.5932286614546));
#24975=CARTESIAN_POINT('Ctrl Pts',(-4.00708241670659,-5.4557764846935,63.601371772735));
#24976=CARTESIAN_POINT('Ctrl Pts',(-3.86510566326265,-5.5545699394116,63.6095148840153));
#24977=CARTESIAN_POINT('Ctrl Pts',(-3.72326354446627,-5.65326970962408,
63.6176502732927));
#24978=CARTESIAN_POINT('Ctrl Pts',(-3.57748731733342,-5.74663787397875,
63.62578566257));
#24979=CARTESIAN_POINT('Ctrl Pts',(-3.42822034345906,-5.83434608818276,
63.6339210518474));
#24980=CARTESIAN_POINT('Ctrl Pts',(-3.27906355285734,-5.92198955947796,
63.642050435886));
#24981=CARTESIAN_POINT('Ctrl Pts',(-3.12642146010185,-6.0039812152636,63.6501798199246));
#24982=CARTESIAN_POINT('Ctrl Pts',(-2.97076698739765,-6.08003556787198,
63.6583092039632));
#24983=CARTESIAN_POINT('Ctrl Pts',(-2.81519471809391,-6.15604975506593,
63.6664342947553));
#24984=CARTESIAN_POINT('Ctrl Pts',(-2.65661356486749,-6.22613272358849,
63.6745593855475));
#24985=CARTESIAN_POINT('Ctrl Pts',(-2.495521661768,-6.29004456547382,63.6826844763396));
#24986=CARTESIAN_POINT('Ctrl Pts',(-2.33381483595205,-6.35420037271475,
63.6908405823647));
#24987=CARTESIAN_POINT('Ctrl Pts',(-2.16957837914399,-6.41213766546459,
63.6989966883899));
#24988=CARTESIAN_POINT('Ctrl Pts',(-2.00333753862448,-6.46366209716582,
63.707152794415));
#24989=CARTESIAN_POINT('Ctrl Pts',(-1.83776578742289,-6.5149791523478,63.7152760735884));
#24990=CARTESIAN_POINT('Ctrl Pts',(-1.6702061153167,-6.55993478338896,63.7233993527618));
#24991=CARTESIAN_POINT('Ctrl Pts',(-1.50119345572939,-6.59838671255901,
63.7315226319352));
#24992=CARTESIAN_POINT('Ctrl Pts',(-1.33215829067814,-6.63684376192838,
63.7396469927919));
#24993=CARTESIAN_POINT('Ctrl Pts',(-1.16167010952075,-6.6687953033068,63.7477713536486));
#24994=CARTESIAN_POINT('Ctrl Pts',(-0.990274726559195,-6.69415005552894,
63.7558957145053));
#24995=CARTESIAN_POINT('Ctrl Pts',(-0.818823912000534,-6.71951300782267,
63.7640227028907));
#24996=CARTESIAN_POINT('Ctrl Pts',(-0.646465673081908,-6.73827486899703,
63.7721496912762));
#24997=CARTESIAN_POINT('Ctrl Pts',(-0.473751600845935,-6.75039616768497,
63.7802766796616));
#24998=CARTESIAN_POINT('Ctrl Pts',(-0.299920951797434,-6.76259582918885,
63.7884562081016));
#24999=CARTESIAN_POINT('Ctrl Pts',(-0.125730227538434,-6.76806874325794,
63.7966357365417));
#25000=CARTESIAN_POINT('Ctrl Pts',(0.0482584615871252,-6.76682792162511,
63.8048152649818));
#25001=CARTESIAN_POINT('Ctrl Pts',(0.221427781884395,-6.76559294342138,
63.8129562733854));
#25002=CARTESIAN_POINT('Ctrl Pts',(0.394396603800965,-6.75770740860602,
63.8210972817891));
#25003=CARTESIAN_POINT('Ctrl Pts',(0.566616481323942,-6.74323622329013,
63.8292382901928));
#25004=CARTESIAN_POINT('Ctrl Pts',(0.740058673507064,-6.72866233007421,
63.837437078651));
#25005=CARTESIAN_POINT('Ctrl Pts',(0.912740876396846,-6.70740900676458,
63.8456358671093));
#25006=CARTESIAN_POINT('Ctrl Pts',(1.08411431358517,-6.67959468494008,63.8538346555675));
#25007=CARTESIAN_POINT('Ctrl Pts',(1.25548775077344,-6.65178036311559,63.8620334440257));
#25008=CARTESIAN_POINT('Ctrl Pts',(1.42555207109027,-6.61740517985191,63.870232232484));
#25009=CARTESIAN_POINT('Ctrl Pts',(1.59377534453279,-6.57663813442396,63.8784310209422));
#25010=CARTESIAN_POINT('Ctrl Pts',(1.76270160122032,-6.53570072879971,63.8866640710742));
#25011=CARTESIAN_POINT('Ctrl Pts',(1.93029653364513,-6.48819078895483,63.8948971212062));
#25012=CARTESIAN_POINT('Ctrl Pts',(2.09601085815659,-6.4342076033098,63.9031301713382));
#25013=CARTESIAN_POINT('Ctrl Pts',(2.26152784238033,-6.38028870334086,63.9113534171731));
#25014=CARTESIAN_POINT('Ctrl Pts',(2.42516834089234,-6.31991201723672,63.9195766630079));
#25015=CARTESIAN_POINT('Ctrl Pts',(2.58639362657619,-6.25322772721465,63.9277999088428));
#25016=CARTESIAN_POINT('Ctrl Pts',(2.74745918731633,-6.18660950092709,63.9360150079563));
#25017=CARTESIAN_POINT('Ctrl Pts',(2.90611397168133,-6.11369625145372,63.9442301070697));
#25018=CARTESIAN_POINT('Ctrl Pts',(3.06183469079249,-6.03468784000131,63.9524452061832));
#25019=CARTESIAN_POINT('Ctrl Pts',(3.21743229488071,-5.95574189372658,63.9606538103221));
#25020=CARTESIAN_POINT('Ctrl Pts',(3.37010013613797,-5.87071054513674,63.968862414461));
#25021=CARTESIAN_POINT('Ctrl Pts',(3.51933510274833,-5.77984164441928,63.9770710185999));
#25022=CARTESIAN_POINT('Ctrl Pts',(3.6684819332182,-5.68902640963805,63.9852747748489));
#25023=CARTESIAN_POINT('Ctrl Pts',(3.81419962280484,-5.59238067655634,63.9934785310979));
#25024=CARTESIAN_POINT('Ctrl Pts',(3.95600978636036,-5.49019813578901,64.0016822873468));
#25025=CARTESIAN_POINT('Ctrl Pts',(4.09777799186268,-5.38804582826007,64.0098836163111));
#25026=CARTESIAN_POINT('Ctrl Pts',(4.23564068183212,-5.28036018228064,64.0180849452754));
#25027=CARTESIAN_POINT('Ctrl Pts',(4.36914838749145,-5.16747824069738,64.0262862742397));
#25028=CARTESIAN_POINT('Ctrl Pts',(4.50263768116362,-5.05461186661151,64.0344864721624));
#25029=CARTESIAN_POINT('Ctrl Pts',(4.63177291268134,-4.93655085481184,64.0426866700851));
#25030=CARTESIAN_POINT('Ctrl Pts',(4.75613764415157,-4.8136725802535,64.0508868680079));
#25031=CARTESIAN_POINT('Ctrl Pts',(4.88050776195783,-4.69078898373876,64.0590874210877));
#25032=CARTESIAN_POINT('Ctrl Pts',(5.00010671317036,-4.5630879605937,64.0672879741675));
#25033=CARTESIAN_POINT('Ctrl Pts',(5.11455485263038,-4.43098382522832,64.0754885272474));
#25034=CARTESIAN_POINT('Ctrl Pts',(5.22902868917564,-4.29885002847009,64.0836909216006));
#25035=CARTESIAN_POINT('Ctrl Pts',(5.3383491759655,-4.16231142115327,64.0918933159538));
#25036=CARTESIAN_POINT('Ctrl Pts',(5.44217686535818,-4.02181550623102,64.100095710307));
#25037=CARTESIAN_POINT('Ctrl Pts',(5.54610165189218,-3.88118820293071,64.1083057753409));
#25038=CARTESIAN_POINT('Ctrl Pts',(5.64452316505465,-3.73659648669212,64.1165158403747));
#25039=CARTESIAN_POINT('Ctrl Pts',(5.73714470946154,-3.58851774172812,64.1247259054086));
#25040=CARTESIAN_POINT('Ctrl Pts',(5.82981058089664,-3.44036812890343,64.1329398996339));
#25041=CARTESIAN_POINT('Ctrl Pts',(5.91667077117707,-3.28872847070018,64.1411538938592));
#25042=CARTESIAN_POINT('Ctrl Pts',(5.99747456463078,-3.13410080351715,64.1493678880845));
#25043=CARTESIAN_POINT('Ctrl Pts',(6.0783885205673,-2.9792623273238,64.1575930807197));
#25044=CARTESIAN_POINT('Ctrl Pts',(6.15322942463203,-2.82142802472799,64.1658182733549));
#25045=CARTESIAN_POINT('Ctrl Pts',(6.22179424272042,-2.6611210797803,64.1740434659901));
#25046=CARTESIAN_POINT('Ctrl Pts',(6.28345443677379,-2.51695738753749,64.18144036411));
#25047=CARTESIAN_POINT('Ctrl Pts',(6.34003952089641,-2.37079440267211,64.18883726223));
#25048=CARTESIAN_POINT('Ctrl Pts',(6.39143650395114,-2.22302236065245,64.1962341603499));
#25049=CARTESIAN_POINT('Ctrl Pts',(6.45151257719412,-2.05029696916043,64.2048801268408));
#25050=CARTESIAN_POINT('Ctrl Pts',(6.50463635311451,-1.8749810263893,64.2135260933317));
#25051=CARTESIAN_POINT('Ctrl Pts',(6.55059377604674,-1.69764842685927,64.2221720598226));
#25052=CARTESIAN_POINT('Ctrl Pts',(6.59649241318722,-1.52054265983203,64.230806966947));
#25053=CARTESIAN_POINT('Ctrl Pts',(6.63524290022221,-1.34142567366235,64.2394418740713));
#25054=CARTESIAN_POINT('Ctrl Pts',(6.66668044306123,-1.16088796621593,64.2480767811957));
#25055=CARTESIAN_POINT('Ctrl Pts',(6.69916168694868,-0.97435655259756,64.2569983602672));
#25056=CARTESIAN_POINT('Ctrl Pts',(6.72383594159697,-0.786308756225134,
64.2659199393387));
#25057=CARTESIAN_POINT('Ctrl Pts',(6.74057770307013,-0.597412109748195,
64.2748415184102));
#25058=CARTESIAN_POINT('Ctrl Pts',(6.75673675902284,-0.415090107096774,
64.2834525773859));
#25059=CARTESIAN_POINT('Ctrl Pts',(6.76550613345692,-0.231977688015453,
64.2920636363616));
#25060=CARTESIAN_POINT('Ctrl Pts',(6.76682486511335,-0.0486851608162831,
64.3006746953373));
#25061=CARTESIAN_POINT('Ctrl Pts',(6.76814235314494,0.134434513067053,64.3092776336868));
#25062=CARTESIAN_POINT('Ctrl Pts',(6.76202320481354,0.317733652485977,64.3178805720363));
#25063=CARTESIAN_POINT('Ctrl Pts',(6.74845836533785,0.500598333298885,64.3264835103859));
#25064=CARTESIAN_POINT('Ctrl Pts',(6.73490871534439,0.683258247971745,64.3350768154346));
#25065=CARTESIAN_POINT('Ctrl Pts',(6.71393002970185,0.865484371104247,64.3436701204833));
#25066=CARTESIAN_POINT('Ctrl Pts',(6.68556529626049,1.04666406713776,64.352263425532));
#25067=CARTESIAN_POINT('Ctrl Pts',(6.68240500067162,1.06685045088618,64.3532208603725));
#25068=CARTESIAN_POINT('Ctrl Pts',(6.6791530708192,1.08702384669509,64.3541782952131));
#25069=CARTESIAN_POINT('Ctrl Pts',(6.67580960620645,1.10718340923342,64.3551357300536));
#25070=CARTESIAN_POINT('Ctrl Pts',(6.64579230376101,1.28817401507749,64.3637314876012));
#25071=CARTESIAN_POINT('Ctrl Pts',(6.60842798813331,1.46783697545944,64.3723272451488));
#25072=CARTESIAN_POINT('Ctrl Pts',(6.5638683233526,1.64557638342566,64.3809230026964));
#25073=CARTESIAN_POINT('Ctrl Pts',(6.51926708288994,1.82348162830142,64.389526780378));
#25074=CARTESIAN_POINT('Ctrl Pts',(6.46745716711604,1.99945944225569,64.3981305580596));
#25075=CARTESIAN_POINT('Ctrl Pts',(6.40864002585188,2.17292936356644,64.4067343357411));
#25076=CARTESIAN_POINT('Ctrl Pts',(6.34751131950341,2.3532168044754,64.4156762494092));
#25077=CARTESIAN_POINT('Ctrl Pts',(6.2788136026702,2.53079488917563,64.4246181630772));
#25078=CARTESIAN_POINT('Ctrl Pts',(6.20282733183092,2.70503643071425,64.4335600767453));
#25079=CARTESIAN_POINT('Ctrl Pts',(6.12951540362112,2.87314552783606,64.442187279076));
#25080=CARTESIAN_POINT('Ctrl Pts',(6.04941939341233,3.0381486933052,64.4508144814067));
#25081=CARTESIAN_POINT('Ctrl Pts',(5.96283762682577,3.19950878043972,64.4594416837375));
#25082=CARTESIAN_POINT('Ctrl Pts',(5.87617340435945,3.36102253835813,64.4680771021579));
#25083=CARTESIAN_POINT('Ctrl Pts',(5.78301124854136,3.51888602852593,64.4767125205783));
#25084=CARTESIAN_POINT('Ctrl Pts',(5.68369340940687,3.67259012522021,64.4853479389987));
#25085=CARTESIAN_POINT('Ctrl Pts',(5.58422884231159,3.82652129782419,64.4939961150199));
#25086=CARTESIAN_POINT('Ctrl Pts',(5.47859059093992,3.97628054571561,64.502644291041));
#25087=CARTESIAN_POINT('Ctrl Pts',(5.36716272913405,4.12138972180433,64.5112924670621));
#25088=CARTESIAN_POINT('Ctrl Pts',(5.35537408385509,4.13674172242525,64.512207411294));
#25089=CARTESIAN_POINT('Ctrl Pts',(5.34352067183579,4.15204170803573,64.5131223555258));
#25090=CARTESIAN_POINT('Ctrl Pts',(5.33160297273055,4.16728913577769,64.5140372997576));
#25091=CARTESIAN_POINT('Ctrl Pts',(5.22444543830568,4.30438579753439,64.5222639857271));
#25092=CARTESIAN_POINT('Ctrl Pts',(5.11185590415505,4.43752659099536,64.5304906716966));
#25093=CARTESIAN_POINT('Ctrl Pts',(4.99415701639361,4.56625499677871,64.5387173576661));
#25094=CARTESIAN_POINT('Ctrl Pts',(4.87657886026313,4.69485135721585,64.5469356049729));
#25095=CARTESIAN_POINT('Ctrl Pts',(4.753902026276,4.81904407991842,64.5551538522797));
#25096=CARTESIAN_POINT('Ctrl Pts',(4.62649081119084,4.93840781770468,64.5633720995865));
#25097=CARTESIAN_POINT('Ctrl Pts',(4.49920926513555,5.05765007654524,64.571581983013));
#25098=CARTESIAN_POINT('Ctrl Pts',(4.36720320055242,5.172072901194,64.5797918664394));
#25099=CARTESIAN_POINT('Ctrl Pts',(4.23087515662351,5.28128624570435,64.5880017498659));
#25100=CARTESIAN_POINT('Ctrl Pts',(4.09462761950288,5.39043509565046,64.5962067850492));
#25101=CARTESIAN_POINT('Ctrl Pts',(3.95406346356247,5.49438036780918,64.6044118202325));
#25102=CARTESIAN_POINT('Ctrl Pts',(3.80962018394378,5.5927706062459,64.6126168554158));
#25103=CARTESIAN_POINT('Ctrl Pts',(3.66523880839847,5.69111867756653,64.6208183741661));
#25104=CARTESIAN_POINT('Ctrl Pts',(3.5169819162023,5.78391625608548,64.6290198929165));
#25105=CARTESIAN_POINT('Ctrl Pts',(3.36531803745911,5.87085372895224,64.6372214116669));
#25106=CARTESIAN_POINT('Ctrl Pts',(3.27770872470274,5.92107354604876,64.6419590553777));
#25107=CARTESIAN_POINT('Ctrl Pts',(3.18896311695826,5.96933872150464,64.6466966990885));
#25108=CARTESIAN_POINT('Ctrl Pts',(3.09917575053261,6.01559628526638,64.6514343427993));
#25109=CARTESIAN_POINT('Origin',(0.,0.,-3.69717978381041));
#25110=CARTESIAN_POINT('',(3.09917575053263,6.01559628526637,67.0455611218465));
#25111=CARTESIAN_POINT('',(3.09917575053252,6.01559628526643,66.6513920151221));
#25112=CARTESIAN_POINT('',(3.09917575053259,6.01559628526639,-3.69717978381041));
#25113=CARTESIAN_POINT('',(-6.76699996591071,0.000679238137944715,65.6971797933975));
#25114=CARTESIAN_POINT('Ctrl Pts',(-6.76699996593128,0.000679033234083034,
65.6971798029849));
#25115=CARTESIAN_POINT('Ctrl Pts',(-6.76701829841272,-0.182015855690237,
65.7057280919095));
#25116=CARTESIAN_POINT('Ctrl Pts',(-6.75963373113655,-0.364585292346518,
65.7142763808342));
#25117=CARTESIAN_POINT('Ctrl Pts',(-6.74490266290975,-0.546422060199833,
65.7228246697588));
#25118=CARTESIAN_POINT('Ctrl Pts',(-6.73015592228546,-0.72845228436326,
65.7313820532162));
#25119=CARTESIAN_POINT('Ctrl Pts',(-6.70804710543446,-0.909747974781611,
65.7399394366735));
#25120=CARTESIAN_POINT('Ctrl Pts',(-6.67868416120356,-1.08970953693578,
65.7484968201309));
#25121=CARTESIAN_POINT('Ctrl Pts',(-6.64926242066203,-1.27003145382223,
65.7570713388786));
#25122=CARTESIAN_POINT('Ctrl Pts',(-6.6125575580926,-1.44901359345539,65.7656458576263));
#25123=CARTESIAN_POINT('Ctrl Pts',(-6.56872859973054,-1.62606690609029,
65.774220376374));
#25124=CARTESIAN_POINT('Ctrl Pts',(-6.52485489609184,-1.80330097363587,
65.7828036489053));
#25125=CARTESIAN_POINT('Ctrl Pts',(-6.47384266484309,-1.97860198551847,
65.7913869214366));
#25126=CARTESIAN_POINT('Ctrl Pts',(-6.41590032842197,-2.15139767959224,
65.7999701939678));
#25127=CARTESIAN_POINT('Ctrl Pts',(-6.35783972036346,-2.32454608346221,
65.8085709866365));
#25128=CARTESIAN_POINT('Ctrl Pts',(-6.29282082746695,-2.49517865135353,
65.8171717793051));
#25129=CARTESIAN_POINT('Ctrl Pts',(-6.22110047482245,-2.6627425489829,65.8257725719738));
#25130=CARTESIAN_POINT('Ctrl Pts',(-6.15407454921833,-2.8193386186106,65.8338104031931));
#25131=CARTESIAN_POINT('Ctrl Pts',(-6.08119628993791,-2.97325463338034,
65.8418482344124));
#25132=CARTESIAN_POINT('Ctrl Pts',(-6.00271060372069,-3.12406056407029,
65.8498860656317));
#25133=CARTESIAN_POINT('Ctrl Pts',(-5.91828918509872,-3.28627167821175,
65.8585317836841));
#25134=CARTESIAN_POINT('Ctrl Pts',(-5.82721329346294,-3.44520389241049,
65.8671775017364));
#25135=CARTESIAN_POINT('Ctrl Pts',(-5.72975335653186,-3.60030769147747,
65.8758232197888));
#25136=CARTESIAN_POINT('Ctrl Pts',(-5.63241853829777,-3.75521236887612,
65.8844578385011));
#25137=CARTESIAN_POINT('Ctrl Pts',(-5.52871617912909,-3.90629817472001,
65.8930924572134));
#25138=CARTESIAN_POINT('Ctrl Pts',(-5.41896259311802,-4.05304002131581,
65.9017270759257));
#25139=CARTESIAN_POINT('Ctrl Pts',(-5.3053329368074,-4.20496421988718,65.9106666358282));
#25140=CARTESIAN_POINT('Ctrl Pts',(-5.18521696388412,-4.35223173770641,
65.9196061957307));
#25141=CARTESIAN_POINT('Ctrl Pts',(-5.05901649420365,-4.49428983393098,
65.9285457556331));
#25142=CARTESIAN_POINT('Ctrl Pts',(-4.9374592252949,-4.63112129142999,65.9371564089036));
#25143=CARTESIAN_POINT('Ctrl Pts',(-4.81025739461192,-4.76311953171593,
65.945767062174));
#25144=CARTESIAN_POINT('Ctrl Pts',(-4.6778130723278,-4.88982145485488,65.9543777154445));
#25145=CARTESIAN_POINT('Ctrl Pts',(-4.54549411745622,-5.0164034461463,65.9629802181555));
#25146=CARTESIAN_POINT('Ctrl Pts',(-4.40794278427344,-5.13769890536457,
65.9715827208666));
#25147=CARTESIAN_POINT('Ctrl Pts',(-4.26559939339094,-5.2532800053969,65.9801852235776));
#25148=CARTESIAN_POINT('Ctrl Pts',(-4.1234162071291,-5.36873102122812,65.988778044345));
#25149=CARTESIAN_POINT('Ctrl Pts',(-3.97645195903324,-5.47848031647352,
65.9973708651125));
#25150=CARTESIAN_POINT('Ctrl Pts',(-3.82518174281441,-5.58213880465537,
66.0059636858799));
#25151=CARTESIAN_POINT('Ctrl Pts',(-3.80735386072118,-5.59435542833359,
66.0069763888383));
#25152=CARTESIAN_POINT('Ctrl Pts',(-3.78946620925084,-5.60648749735201,
66.0079890917968));
#25153=CARTESIAN_POINT('Ctrl Pts',(-3.77151959710279,-5.61853441109597,
66.0090017947552));
#25154=CARTESIAN_POINT('Ctrl Pts',(-3.61919876497134,-5.72078189440697,
66.0175970525153));
#25155=CARTESIAN_POINT('Ctrl Pts',(-3.4628073215774,-5.81677131581846,66.0261923102754));
#25156=CARTESIAN_POINT('Ctrl Pts',(-3.30288303748162,-5.90620458845748,
66.0347875680355));
#25157=CARTESIAN_POINT('Ctrl Pts',(-3.14280899107559,-5.99572161156379,
66.04339087489));
#25158=CARTESIAN_POINT('Ctrl Pts',(-2.97919576686916,-6.07867008207256,
66.0519941817445));
#25159=CARTESIAN_POINT('Ctrl Pts',(-2.81260401966386,-6.1547987480153,66.060597488599));
#25160=CARTESIAN_POINT('Ctrl Pts',(-2.63910532085218,-6.23408373484635,
66.0695574915389));
#25161=CARTESIAN_POINT('Ctrl Pts',(-2.4623762072421,-6.30597121789813,66.0785174944789));
#25162=CARTESIAN_POINT('Ctrl Pts',(-2.28306956927753,-6.3702340884648,66.0874774974189));
#25163=CARTESIAN_POINT('Ctrl Pts',(-2.11043008894921,-6.43210747310339,
66.0961043406236));
#25164=CARTESIAN_POINT('Ctrl Pts',(-1.93540160429527,-6.48691298856344,
66.1047311838284));
#25165=CARTESIAN_POINT('Ctrl Pts',(-1.7585796753181,-6.53449971501707,66.1133580270332));
#25166=CARTESIAN_POINT('Ctrl Pts',(-1.58158874927383,-6.58213192235222,
66.1219931153193));
#25167=CARTESIAN_POINT('Ctrl Pts',(-1.40280125409471,-6.62253149882609,
66.1306282036055));
#25168=CARTESIAN_POINT('Ctrl Pts',(-1.22282244806186,-6.65559871540615,
66.1392632918917));
#25169=CARTESIAN_POINT('Ctrl Pts',(-1.04257633738337,-6.68871504343887,
66.1479112050169));
#25170=CARTESIAN_POINT('Ctrl Pts',(-0.861135681401127,-6.71447720235611,
66.1565591181421));
#25171=CARTESIAN_POINT('Ctrl Pts',(-0.679111850412633,-6.7328371504611,
66.1652070312673));
#25172=CARTESIAN_POINT('Ctrl Pts',(-0.658691547561236,-6.73489685714129,
66.166177195471));
#25173=CARTESIAN_POINT('Ctrl Pts',(-0.638263905900065,-6.73686345783071,
66.1671473596747));
#25174=CARTESIAN_POINT('Ctrl Pts',(-0.617829788642748,-6.7387369255867,
66.1681175238785));
#25175=CARTESIAN_POINT('Ctrl Pts',(-0.444597190442899,-6.75461946569974,
66.1763422033973));
#25176=CARTESIAN_POINT('Ctrl Pts',(-0.270523469771335,-6.76383871484805,
66.184566882916));
#25177=CARTESIAN_POINT('Ctrl Pts',(-0.0961618693914154,-6.76631671553107,
66.1927915624348));
#25178=CARTESIAN_POINT('Ctrl Pts',(0.0780164572205188,-6.76879211155503,
66.201007596885));
#25179=CARTESIAN_POINT('Ctrl Pts',(0.252481705538154,-6.76454036442842,
66.2092236313352));
#25180=CARTESIAN_POINT('Ctrl Pts',(0.426674816227314,-6.75353519285991,
66.2174396657853));
#25181=CARTESIAN_POINT('Ctrl Pts',(0.600719721436524,-6.74253938461656,
66.2256487099399));
#25182=CARTESIAN_POINT('Ctrl Pts',(0.774492594459042,-6.72480161802293,
66.2338577540945));
#25183=CARTESIAN_POINT('Ctrl Pts',(0.947433578676589,-6.70034764874153,
66.242066798249));
#25184=CARTESIAN_POINT('Ctrl Pts',(1.1202620533378,-6.67590958838562,66.2502705018771));
#25185=CARTESIAN_POINT('Ctrl Pts',(1.29225936359367,-6.64476407866937,66.2584742055051));
#25186=CARTESIAN_POINT('Ctrl Pts',(1.46286988650982,-6.60698877667752,66.2666779091332));
#25187=CARTESIAN_POINT('Ctrl Pts',(1.63340357297601,-6.56923048723597,66.2748779181271));
#25188=CARTESIAN_POINT('Ctrl Pts',(1.80255136717255,-6.52484843138451,66.283077927121));
#25189=CARTESIAN_POINT('Ctrl Pts',(1.96976687326738,-6.47397153723883,66.2912779361149));
#25190=CARTESIAN_POINT('Ctrl Pts',(2.13696900845895,-6.42309871131652,66.2994772894188));
#25191=CARTESIAN_POINT('Ctrl Pts',(2.30223881813281,-6.36573217743598,66.3076766427228));
#25192=CARTESIAN_POINT('Ctrl Pts',(2.46504377013428,-6.30205111144953,66.3158759960267));
#25193=CARTESIAN_POINT('Ctrl Pts',(2.62784766069578,-6.23837046064472,66.3240752958733));
#25194=CARTESIAN_POINT('Ctrl Pts',(2.78818639131588,-6.16837548932268,66.3322745957199));
#25195=CARTESIAN_POINT('Ctrl Pts',(2.94554628395755,-6.09229399233687,66.3404738955665));
#25196=CARTESIAN_POINT('Ctrl Pts',(3.10293369728779,-6.01619918944986,66.3486746293895));
#25197=CARTESIAN_POINT('Ctrl Pts',(3.25734091191964,-5.93401589617232,66.3568753632126));
#25198=CARTESIAN_POINT('Ctrl Pts',(3.4082777346436,-5.84601846417993,66.3650760970356));
#25199=CARTESIAN_POINT('Ctrl Pts',(3.55926833644244,-5.7579896785364,66.3732797527956));
#25200=CARTESIAN_POINT('Ctrl Pts',(3.70678577361999,-5.66414280792534,66.3814834085556));
#25201=CARTESIAN_POINT('Ctrl Pts',(3.8503677394768,-5.56479624701537,66.3896870643155));
#25202=CARTESIAN_POINT('Ctrl Pts',(3.99411418770588,-5.46533587823322,66.3979001178906));
#25203=CARTESIAN_POINT('Ctrl Pts',(4.13391586253542,-5.36036343644528,66.4061131714656));
#25204=CARTESIAN_POINT('Ctrl Pts',(4.2693416978793,-5.2502390866273,66.4143262250406));
#25205=CARTESIAN_POINT('Ctrl Pts',(4.40484766772839,-5.14004957376077,66.4225441384637));
#25206=CARTESIAN_POINT('Ctrl Pts',(4.53597236794302,-5.02470231247019,66.4307620518868));
#25207=CARTESIAN_POINT('Ctrl Pts',(4.66232079823274,-4.90459516926387,66.4389799653099));
#25208=CARTESIAN_POINT('Ctrl Pts',(4.78886628945417,-4.78430069942839,66.4472106959059));
#25209=CARTESIAN_POINT('Ctrl Pts',(4.91062037379979,-4.6592317684667,66.4554414265019));
#25210=CARTESIAN_POINT('Ctrl Pts',(5.02722672795302,-4.52982123551855,66.4636721570979));
#25211=CARTESIAN_POINT('Ctrl Pts',(5.1343157183893,-4.41097313820966,66.4712310987738));
#25212=CARTESIAN_POINT('Ctrl Pts',(5.23706333941518,-4.28846378288316,66.4787900404496));
#25213=CARTESIAN_POINT('Ctrl Pts',(5.3352258976235,-4.16264983169706,66.4863489821254));
#25214=CARTESIAN_POINT('Ctrl Pts',(5.4411146514679,-4.02693329424635,66.4945028742922));
#25215=CARTESIAN_POINT('Ctrl Pts',(5.54199497742943,-3.88695143604734,66.5026567664589));
#25216=CARTESIAN_POINT('Ctrl Pts',(5.63749939601689,-3.74311228256771,66.5108106586256));
#25217=CARTESIAN_POINT('Ctrl Pts',(5.73288727253146,-3.59944865304139,66.5189546007658));
#25218=CARTESIAN_POINT('Ctrl Pts',(5.82291209971961,-3.45193739885122,66.527098542906));
#25219=CARTESIAN_POINT('Ctrl Pts',(5.90724584281413,-3.30102038051194,66.5352424850462));
#25220=CARTESIAN_POINT('Ctrl Pts',(5.99149442575089,-3.15025575807753,66.5433782034391));
#25221=CARTESIAN_POINT('Ctrl Pts',(6.07006318842045,-2.99609253493669,66.5515139218319));
#25222=CARTESIAN_POINT('Ctrl Pts',(6.14266672326913,-2.83900238232413,66.5596496402248));
#25223=CARTESIAN_POINT('Ctrl Pts',(6.2152122152883,-2.68203781529036,66.567778854525));
#25224=CARTESIAN_POINT('Ctrl Pts',(6.28180182217059,-2.52215130819603,66.5759080688252));
#25225=CARTESIAN_POINT('Ctrl Pts',(6.34219552603449,-2.35984001778683,66.5840372831254));
#25226=CARTESIAN_POINT('Ctrl Pts',(6.40255364673221,-2.19762435902875,66.5921617078008));
#25227=CARTESIAN_POINT('Ctrl Pts',(6.45672300712941,-2.03298710389042,66.6002861324763));
#25228=CARTESIAN_POINT('Ctrl Pts',(6.50451129305998,-1.86644631277065,66.6084105571517));
#25229=CARTESIAN_POINT('Ctrl Pts',(6.55258968447877,-1.69889451243442,66.6165843022858));
#25230=CARTESIAN_POINT('Ctrl Pts',(6.5942091160322,-1.52941632984027,66.62475804742));
#25231=CARTESIAN_POINT('Ctrl Pts',(6.62922420344981,-1.35855638837528,66.6329317925542));
#25232=CARTESIAN_POINT('Ctrl Pts',(6.66401506449367,-1.18879058397854,66.6410531954163));
#25233=CARTESIAN_POINT('Ctrl Pts',(6.69228586697066,-1.01766103306341,66.6491745982785));
#25234=CARTESIAN_POINT('Ctrl Pts',(6.7139450268928,-0.845713412369381,66.6572960011407));
#25235=CARTESIAN_POINT('Ctrl Pts',(6.73560586138712,-0.673752497590899,
66.6654180319069));
#25236=CARTESIAN_POINT('Ctrl Pts',(6.75065398932149,-0.500973750163868,
66.6735400626732));
#25237=CARTESIAN_POINT('Ctrl Pts',(6.75904960699328,-0.327928971278944,
66.6816620934394));
#25238=CARTESIAN_POINT('Ctrl Pts',(6.7674474724895,-0.154837861760821,66.6897862987805));
#25239=CARTESIAN_POINT('Ctrl Pts',(6.7691892634495,0.018519055636335,66.6979105041216));
#25240=CARTESIAN_POINT('Ctrl Pts',(6.76428729798188,0.191589014197034,66.7060347094628));
#25241=CARTESIAN_POINT('Ctrl Pts',(6.75933227212995,0.366532335304846,66.7142468537052));
#25242=CARTESIAN_POINT('Ctrl Pts',(6.74758883146797,0.541182065489069,66.7224589979477));
#25243=CARTESIAN_POINT('Ctrl Pts',(6.72912352322345,0.714972453455995,66.7306711421901));
#25244=CARTESIAN_POINT('Ctrl Pts',(6.71082678289187,0.887176326721829,66.7388083186066));
#25245=CARTESIAN_POINT('Ctrl Pts',(6.68593050572258,1.0585361294244,66.746945495023));
#25246=CARTESIAN_POINT('Ctrl Pts',(6.65455087594178,1.22851196148125,66.7550826714394));
#25247=CARTESIAN_POINT('Ctrl Pts',(6.62273759525332,1.40083677516617,66.7633322995949));
#25248=CARTESIAN_POINT('Ctrl Pts',(6.58426054248535,1.57173870365354,66.7715819277504));
#25249=CARTESIAN_POINT('Ctrl Pts',(6.53929285886129,1.74067168243922,66.7798315559058));
#25250=CARTESIAN_POINT('Ctrl Pts',(6.49432517523723,1.9096046612249,66.7880811840613));
#25251=CARTESIAN_POINT('Ctrl Pts',(6.44286703453955,2.07656834123183,66.7963308122168));
#25252=CARTESIAN_POINT('Ctrl Pts',(6.3851417130851,2.24103866629308,66.8045804403722));
#25253=CARTESIAN_POINT('Ctrl Pts',(6.32757961941145,2.40504392462987,66.8128067413558));
#25254=CARTESIAN_POINT('Ctrl Pts',(6.2636138135267,2.56706028210118,66.8210330423394));
#25255=CARTESIAN_POINT('Ctrl Pts',(6.19340007997293,2.7265517507268,66.8292593433229));
#25256=CARTESIAN_POINT('Ctrl Pts',(6.1232678698591,2.885858037729,66.8374760929507));
#25257=CARTESIAN_POINT('Ctrl Pts',(6.04690232226855,3.0426449484445,66.8456928425784));
#25258=CARTESIAN_POINT('Ctrl Pts',(5.9645087528244,3.19639239416582,66.8539095922061));
#25259=CARTESIAN_POINT('Ctrl Pts',(5.88221116536148,3.34996073629267,66.8621167699715));
#25260=CARTESIAN_POINT('Ctrl Pts',(5.7938997203715,3.50049635610298,66.8703239477368));
#25261=CARTESIAN_POINT('Ctrl Pts',(5.69982736677687,3.64750010129424,66.8785311255021));
#25262=CARTESIAN_POINT('Ctrl Pts',(5.60581794891072,3.79440549891113,66.88673281255));
#25263=CARTESIAN_POINT('Ctrl Pts',(5.50605548906791,3.93778342587172,66.894934499598));
#25264=CARTESIAN_POINT('Ctrl Pts',(5.40083858019566,4.07715975044763,66.9031361866459));
#25265=CARTESIAN_POINT('Ctrl Pts',(5.29567291839555,4.21646819022595,66.9113338789704));
#25266=CARTESIAN_POINT('Ctrl Pts',(5.18505831402604,4.35177862356726,66.9195315712949));
#25267=CARTESIAN_POINT('Ctrl Pts',(5.06933638185038,4.48264627732861,66.9277292636194));
#25268=CARTESIAN_POINT('Ctrl Pts',(4.95364975869858,4.61347400081037,66.9359244546677));
#25269=CARTESIAN_POINT('Ctrl Pts',(4.8328591496575,4.73986137687093,66.944119645716));
#25270=CARTESIAN_POINT('Ctrl Pts',(4.70734614836208,4.86139704606615,66.9523148367643));
#25271=CARTESIAN_POINT('Ctrl Pts',(4.58182083059437,4.98294464144183,66.960510831999));
#25272=CARTESIAN_POINT('Ctrl Pts',(4.45157244688807,5.09963932339206,66.9687068272336));
#25273=CARTESIAN_POINT('Ctrl Pts',(4.31701941844626,5.21110663302508,66.9769028224683));
#25274=CARTESIAN_POINT('Ctrl Pts',(4.18246280969302,5.32257690868336,66.9850990357896));
#25275=CARTESIAN_POINT('Ctrl Pts',(4.0436016075609,5.42881930982883,66.9932952491109));
#25276=CARTESIAN_POINT('Ctrl Pts',(3.90088697555653,5.52949995966484,67.0014914624322));
#25277=CARTESIAN_POINT('Ctrl Pts',(3.75808854046217,5.63023972992486,67.0096924886307));
#25278=CARTESIAN_POINT('Ctrl Pts',(3.61143245004889,5.72541101959315,67.0178935148293));
#25279=CARTESIAN_POINT('Ctrl Pts',(3.46139904487163,5.81472317932348,67.0260945410278));
#25280=CARTESIAN_POINT('Ctrl Pts',(3.34268880314117,5.88538922905108,67.0325834013007));
#25281=CARTESIAN_POINT('Ctrl Pts',(3.22186484807763,5.95238807481889,67.0390722615736));
#25282=CARTESIAN_POINT('Ctrl Pts',(3.09917575053264,6.01559628526636,67.0455611218465));
#25283=CARTESIAN_POINT('Ctrl Pts',(3.09917575053256,6.01559628526641,65.0457972463573));
#25284=CARTESIAN_POINT('Ctrl Pts',(2.94385221859564,6.09561743376751,65.0539928534118));
#25285=CARTESIAN_POINT('Ctrl Pts',(2.78541612683539,6.16962484631762,65.0621884604664));
#25286=CARTESIAN_POINT('Ctrl Pts',(2.62437670962481,6.23738213403499,65.0703840675209));
#25287=CARTESIAN_POINT('Ctrl Pts',(2.46331642498624,6.30514820171659,65.0785807365591));
#25288=CARTESIAN_POINT('Ctrl Pts',(2.29965247367174,6.36666239194464,65.0867774055974));
#25289=CARTESIAN_POINT('Ctrl Pts',(2.13391369978768,6.42173662819167,65.0949740746356));
#25290=CARTESIAN_POINT('Ctrl Pts',(1.96812329517018,6.47682802109519,65.1031732970898));
#25291=CARTESIAN_POINT('Ctrl Pts',(1.80025712095075,6.5254753508844,65.1113725195441));
#25292=CARTESIAN_POINT('Ctrl Pts',(1.6308588379582,6.56754051762558,65.1195717419983));
#25293=CARTESIAN_POINT('Ctrl Pts',(1.46128209771362,6.60964999906659,65.1277796021476));
#25294=CARTESIAN_POINT('Ctrl Pts',(1.29017037295865,6.64516337844948,65.1359874622968));
#25295=CARTESIAN_POINT('Ctrl Pts',(1.11807813852233,6.67399357777324,65.1441953224461));
#25296=CARTESIAN_POINT('Ctrl Pts',(0.94589038704666,6.70283977883754,65.1524077382367));
#25297=CARTESIAN_POINT('Ctrl Pts',(0.772721396489648,6.72499535991473,65.1606201540273));
#25298=CARTESIAN_POINT('Ctrl Pts',(0.59913030369686,6.74042520017781,65.1688325698179));
#25299=CARTESIAN_POINT('Ctrl Pts',(0.425289102472883,6.75587727161117,65.1770568179808));
#25300=CARTESIAN_POINT('Ctrl Pts',(0.251024941923443,6.76458422105991,65.1852810661437));
#25301=CARTESIAN_POINT('Ctrl Pts',(0.0768977199021893,6.76656306707281,
65.1935053143066));
#25302=CARTESIAN_POINT('Ctrl Pts',(-0.0636718567609128,6.76816055161938,
65.2001445925837));
#25303=CARTESIAN_POINT('Ctrl Pts',(-0.204152146911855,6.76537432336689,
65.2067838708609));
#25304=CARTESIAN_POINT('Ctrl Pts',(-0.34425177587415,6.75823791493075,65.2134231491381));
#25305=CARTESIAN_POINT('Ctrl Pts',(-0.516250829178352,6.74947661053544,
65.2215741313123));
#25306=CARTESIAN_POINT('Ctrl Pts',(-0.688185389881194,6.73413111849514,
65.2297251134866));
#25307=CARTESIAN_POINT('Ctrl Pts',(-0.859506089281795,6.71219325425658,
65.2378760956609));
#25308=CARTESIAN_POINT('Ctrl Pts',(-1.0306277838118,6.69028087288057,65.2460176097139));
#25309=CARTESIAN_POINT('Ctrl Pts',(-1.20113667741297,6.66179140841808,65.254159123767));
#25310=CARTESIAN_POINT('Ctrl Pts',(-1.37048393519505,6.62676865322551,65.26230063782));
#25311=CARTESIAN_POINT('Ctrl Pts',(-1.53967011731522,6.59177921013702,65.270434408023));
#25312=CARTESIAN_POINT('Ctrl Pts',(-1.70769650764706,6.55026892138597,65.278568178226));
#25313=CARTESIAN_POINT('Ctrl Pts',(-1.87401992936699,6.50233329692775,65.286701948429));
#25314=CARTESIAN_POINT('Ctrl Pts',(-2.04022013280626,6.45443318487764,65.2948296928471));
#25315=CARTESIAN_POINT('Ctrl Pts',(-2.20471952979505,6.40011731610231,65.3029574372651));
#25316=CARTESIAN_POINT('Ctrl Pts',(-2.3669856751762,6.33953214468629,65.3110851816831));
#25317=CARTESIAN_POINT('Ctrl Pts',(-2.52916572328387,6.27897911933535,65.3192086135772));
#25318=CARTESIAN_POINT('Ctrl Pts',(-2.68911453778835,6.21216354366818,65.3273320454713));
#25319=CARTESIAN_POINT('Ctrl Pts',(-2.84631537619127,6.13928153608036,65.3354554773654));
#25320=CARTESIAN_POINT('Ctrl Pts',(-3.00451343488078,6.06593719370327,65.3436304411162));
#25321=CARTESIAN_POINT('Ctrl Pts',(-3.15992817398629,5.9864492971089,65.351805404867));
#25322=CARTESIAN_POINT('Ctrl Pts',(-3.31205345963695,5.9010669273028,65.3599803686178));
#25323=CARTESIAN_POINT('Ctrl Pts',(-3.46318551484137,5.81624202149028,65.3681019577908));
#25324=CARTESIAN_POINT('Ctrl Pts',(-3.61107063285668,5.72559958800872,65.3762235469639));
#25325=CARTESIAN_POINT('Ctrl Pts',(-3.7552376238199,5.62942975696895,65.3843451361369));
#25326=CARTESIAN_POINT('Ctrl Pts',(-3.8994236477821,5.5332472295395,65.3924677975262));
#25327=CARTESIAN_POINT('Ctrl Pts',(-4.03989026247573,5.43153605417728,65.4005904589155));
#25328=CARTESIAN_POINT('Ctrl Pts',(-4.17619579140123,5.32462934971841,65.4087131203049));
#25329=CARTESIAN_POINT('Ctrl Pts',(-4.312545272057,5.2176881731829,65.4168384008471));
#25330=CARTESIAN_POINT('Ctrl Pts',(-4.44473070729526,5.10554835726461,65.4249636813893));
#25331=CARTESIAN_POINT('Ctrl Pts',(-4.5723440382569,4.98858286448332,65.4330889619315));
#25332=CARTESIAN_POINT('Ctrl Pts',(-4.70134768998026,4.87034305692792,65.4413027657193));
#25333=CARTESIAN_POINT('Ctrl Pts',(-4.8256787463408,4.74717206650763,65.4495165695071));
#25334=CARTESIAN_POINT('Ctrl Pts',(-4.94495508350294,4.61949220392658,65.4577303732949));
#25335=CARTESIAN_POINT('Ctrl Pts',(-5.06315011094663,4.49296983393413,65.46586971415));
#25336=CARTESIAN_POINT('Ctrl Pts',(-5.17638150033589,4.36202032483429,65.4740090550052));
#25337=CARTESIAN_POINT('Ctrl Pts',(-5.28431928187561,4.22708631650664,65.4821483958603));
#25338=CARTESIAN_POINT('Ctrl Pts',(-5.39373827004506,4.09030063821819,65.4903994311144));
#25339=CARTESIAN_POINT('Ctrl Pts',(-5.49771707765679,3.94942062669911,65.4986504663685));
#25340=CARTESIAN_POINT('Ctrl Pts',(-5.59595874013158,3.80493558141856,65.5069015016226));
#25341=CARTESIAN_POINT('Ctrl Pts',(-5.69420040260637,3.66045053613801,65.5151525368767));
#25342=CARTESIAN_POINT('Ctrl Pts',(-5.78670477345048,3.51236081820523,65.5234035721308));
#25343=CARTESIAN_POINT('Ctrl Pts',(-5.87322448394943,3.3611788350424,65.531654607385));
#25344=CARTESIAN_POINT('Ctrl Pts',(-5.96439181895416,3.20187573027931,65.540348867812));
#25345=CARTESIAN_POINT('Ctrl Pts',(-6.0491723615721,3.03868961436006,65.549043128239));
#25346=CARTESIAN_POINT('Ctrl Pts',(-6.12724033271902,2.87214465253778,65.557737388666));
#25347=CARTESIAN_POINT('Ctrl Pts',(-6.20517873351879,2.70587610738423,65.5664172191248));
#25348=CARTESIAN_POINT('Ctrl Pts',(-6.27642665120116,2.53626009983261,65.5750970495836));
#25349=CARTESIAN_POINT('Ctrl Pts',(-6.34070319849406,2.36384685388186,65.5837768800424));
#25350=CARTESIAN_POINT('Ctrl Pts',(-6.40487649698476,2.19171055904124,65.5924427679026));
#25351=CARTESIAN_POINT('Ctrl Pts',(-6.46210065051034,2.01678626298182,65.6011086557628));
#25352=CARTESIAN_POINT('Ctrl Pts',(-6.51214175033427,1.83964638546469,65.609774543623));
#25353=CARTESIAN_POINT('Ctrl Pts',(-6.56207425720522,1.66289091481427,65.6184216258543));
#25354=CARTESIAN_POINT('Ctrl Pts',(-6.60485472726086,1.48392974022276,65.6270687080857));
#25355=CARTESIAN_POINT('Ctrl Pts',(-6.64029831080929,1.3033523481635,65.635715790317));
#25356=CARTESIAN_POINT('Ctrl Pts',(-6.67569497199666,1.12301401538497,65.6443514250175));
#25357=CARTESIAN_POINT('Ctrl Pts',(-6.70377405277301,0.941064021336169,
65.652987059718));
#25358=CARTESIAN_POINT('Ctrl Pts',(-6.72440064845059,0.758106139743788,
65.6616226944185));
#25359=CARTESIAN_POINT('Ctrl Pts',(-6.74499123012988,0.57546770227781,65.6702432513166));
#25360=CARTESIAN_POINT('Ctrl Pts',(-6.75815524987472,0.391825182658888,
65.6788638082147));
#25361=CARTESIAN_POINT('Ctrl Pts',(-6.76380896286626,0.207791515346705,
65.6874843651129));
#25362=CARTESIAN_POINT('Ctrl Pts',(-6.76592851327327,0.138798159115133,
65.6907161713452));
#25363=CARTESIAN_POINT('Ctrl Pts',(-6.76699303084327,0.0697499303004344,
65.6939479775776));
#25364=CARTESIAN_POINT('Ctrl Pts',(-6.76699996589014,0.000679443041806397,
65.69717978381));
#25365=CARTESIAN_POINT('',(-6.767,2.89194517400122E-12,65.3028202161898));
#25366=CARTESIAN_POINT('Ctrl Pts',(3.09917575053261,6.01559628526638,64.6514343427993));
#25367=CARTESIAN_POINT('Ctrl Pts',(2.94375971393036,6.09566509125678,64.6596348930289));
#25368=CARTESIAN_POINT('Ctrl Pts',(2.78522125750516,6.16971616999855,64.6678354432586));
#25369=CARTESIAN_POINT('Ctrl Pts',(2.62406952193042,6.23751137426425,64.6760359934882));
#25370=CARTESIAN_POINT('Ctrl Pts',(2.46290172942686,6.30531333354729,64.684237360809));
#25371=CARTESIAN_POINT('Ctrl Pts',(2.29912046921022,6.36685803712996,64.6924387281298));
#25372=CARTESIAN_POINT('Ctrl Pts',(2.13325468635921,6.42195557779143,64.7006400954506));
#25373=CARTESIAN_POINT('Ctrl Pts',(1.96734231772071,6.47706859338858,64.7088437662431));
#25374=CARTESIAN_POINT('Ctrl Pts',(1.79934460013952,6.52573072586477,64.7170474370357));
#25375=CARTESIAN_POINT('Ctrl Pts',(1.62980550425163,6.56780199292816,64.7252511078283));
#25376=CARTESIAN_POINT('Ctrl Pts',(1.46018806547383,6.60989270084456,64.7334585694827));
#25377=CARTESIAN_POINT('Ctrl Pts',(1.28902817689152,6.64538639014321,64.741666031137));
#25378=CARTESIAN_POINT('Ctrl Pts',(1.11687991222064,6.67419420317375,64.7498734927914));
#25379=CARTESIAN_POINT('Ctrl Pts',(0.944529275986097,6.70303588167589,64.7580906028546));
#25380=CARTESIAN_POINT('Ctrl Pts',(0.771188296612574,6.72517592828298,64.7663077129179));
#25381=CARTESIAN_POINT('Ctrl Pts',(0.597417027559221,6.74057726720659,64.7745248229812));
#25382=CARTESIAN_POINT('Ctrl Pts',(0.423526475807104,6.75598917814986,64.7827475735572));
#25383=CARTESIAN_POINT('Ctrl Pts',(0.249205402286185,6.76465314425268,64.7909703241333));
#25384=CARTESIAN_POINT('Ctrl Pts',(0.075013652945595,6.76658421597424,64.7991930747093));
#25385=CARTESIAN_POINT('Ctrl Pts',(-0.0994197767091728,6.76851796693878,
64.8074272338449));
#25386=CARTESIAN_POINT('Ctrl Pts',(-0.273723167262516,6.76370017898385,
64.8156613929804));
#25387=CARTESIAN_POINT('Ctrl Pts',(-0.447341076683874,6.75219778746975,
64.823895552116));
#25388=CARTESIAN_POINT('Ctrl Pts',(-0.503180604735224,6.74849835279881,
64.8265438477991));
#25389=CARTESIAN_POINT('Ctrl Pts',(-0.558949299836695,6.74410784974981,
64.8291921434822));
#25390=CARTESIAN_POINT('Ctrl Pts',(-0.614628923382891,6.73902962499359,
64.8318404391653));
#25391=CARTESIAN_POINT('Ctrl Pts',(-0.786094993744047,6.72339117078174,
64.8399958975721));
#25392=CARTESIAN_POINT('Ctrl Pts',(-0.957243499080527,6.70117883226029,
64.8481513559789));
#25393=CARTESIAN_POINT('Ctrl Pts',(-1.12752523770424,6.67240405238921,64.8563068143857));
#25394=CARTESIAN_POINT('Ctrl Pts',(-1.297599721069,6.6436642952076,64.8644523465276));
#25395=CARTESIAN_POINT('Ctrl Pts',(-1.46680918125153,6.60837805610042,64.8725978786695));
#25396=CARTESIAN_POINT('Ctrl Pts',(-1.63460675862359,6.56660869434612,64.8807434108113));
#25397=CARTESIAN_POINT('Ctrl Pts',(-1.80223538875119,6.52488138813686,64.8888807416119));
#25398=CARTESIAN_POINT('Ctrl Pts',(-1.96845461410872,6.4766840420883,64.8970180724124));
#25399=CARTESIAN_POINT('Ctrl Pts',(-2.13272502719967,6.42213149650147,64.905155403213));
#25400=CARTESIAN_POINT('Ctrl Pts',(-2.29686456631296,6.36762241284122,64.913286251015));
#25401=CARTESIAN_POINT('Ctrl Pts',(-2.45905803934959,6.30676832571617,64.9214170988169));
#25402=CARTESIAN_POINT('Ctrl Pts',(-2.61877853279932,6.23973460943248,64.9295479466189));
#25403=CARTESIAN_POINT('Ctrl Pts',(-2.77840532923954,6.17274021721181,64.9376740246127));
#25404=CARTESIAN_POINT('Ctrl Pts',(-2.93556169900813,6.0995735563644,64.9458001026065));
#25405=CARTESIAN_POINT('Ctrl Pts',(-3.08973814461677,6.02044908604833,64.9539261806002));
#25406=CARTESIAN_POINT('Ctrl Pts',(-3.24446127174295,5.94104405481171,64.9620810721824));
#25407=CARTESIAN_POINT('Ctrl Pts',(-3.39618295244663,5.85563900897581,64.9702359637646));
#25408=CARTESIAN_POINT('Ctrl Pts',(-3.54441014670346,5.76449873900112,64.9783908553468));
#25409=CARTESIAN_POINT('Ctrl Pts',(-3.69205930672856,5.67371388421324,64.9865139457031));
#25410=CARTESIAN_POINT('Ctrl Pts',(-3.83624088114111,5.57723866324328,64.9946370360593));
#25411=CARTESIAN_POINT('Ctrl Pts',(-3.97649411459707,5.47537976368533,65.0027601264156));
#25412=CARTESIAN_POINT('Ctrl Pts',(-4.11675836137747,5.3735128657014,65.0108838546341));
#25413=CARTESIAN_POINT('Ctrl Pts',(-4.25309335673059,5.26626166199667,65.0190075828525));
#25414=CARTESIAN_POINT('Ctrl Pts',(-4.38506931010397,5.15397479093411,65.0271313110709));
#25415=CARTESIAN_POINT('Ctrl Pts',(-4.51708073509931,5.04165774015062,65.0352572227312));
#25416=CARTESIAN_POINT('Ctrl Pts',(-4.64473050674262,4.92430256398938,65.0433831343915));
#25417=CARTESIAN_POINT('Ctrl Pts',(-4.76762379333834,4.8022965719741,65.0515090460517));
#25418=CARTESIAN_POINT('Ctrl Pts',(-4.89130299527776,4.67951033895619,65.0596869237618));
#25419=CARTESIAN_POINT('Ctrl Pts',(-5.01016439802514,4.55201386333625,65.0678648014719));
#25420=CARTESIAN_POINT('Ctrl Pts',(-5.12384551322782,4.42023711542436,65.076042679182));
#25421=CARTESIAN_POINT('Ctrl Pts',(-5.23698405312371,4.28908930934948,65.0841815256555));
#25422=CARTESIAN_POINT('Ctrl Pts',(-5.34499146583222,4.15370232343359,65.0923203721289));
#25423=CARTESIAN_POINT('Ctrl Pts',(-5.44755317658133,4.0145302824015,65.1004592186024));
#25424=CARTESIAN_POINT('Ctrl Pts',(-5.55085266578855,3.87435710621776,65.1086566119308));
#25425=CARTESIAN_POINT('Ctrl Pts',(-5.64862759806098,3.73034452649665,65.1168540052592));
#25426=CARTESIAN_POINT('Ctrl Pts',(-5.74060314250142,3.58298263466387,65.1250513985876));
#25427=CARTESIAN_POINT('Ctrl Pts',(-5.83257868694183,3.43562074283113,65.133248791916));
#25428=CARTESIAN_POINT('Ctrl Pts',(-5.91875471183224,3.2849098923583,65.1414461852444));
#25429=CARTESIAN_POINT('Ctrl Pts',(-5.99890541045201,3.13136118588221,65.1496435785728));
#25430=CARTESIAN_POINT('Ctrl Pts',(-6.08459861006928,2.96719443273324,65.1584078298511));
#25431=CARTESIAN_POINT('Ctrl Pts',(-6.16363353114575,2.79934626405396,65.1671720811293));
#25432=CARTESIAN_POINT('Ctrl Pts',(-6.23570284825551,2.6283643180233,65.1759363324076));
#25433=CARTESIAN_POINT('Ctrl Pts',(-6.30764909610388,2.45767434953112,65.184685617401));
#25434=CARTESIAN_POINT('Ctrl Pts',(-6.37265335096421,2.28386153835232,65.1934349023943));
#25435=CARTESIAN_POINT('Ctrl Pts',(-6.4304543836683,2.10749743049929,65.2021841873877));
#25436=CARTESIAN_POINT('Ctrl Pts',(-6.48811187486979,1.93157130044463,65.2109117446462));
#25437=CARTESIAN_POINT('Ctrl Pts',(-6.53860174470766,1.75310678554235,65.2196393019047));
#25438=CARTESIAN_POINT('Ctrl Pts',(-6.58171120573811,1.57269405933302,65.2283668591632));
#25439=CARTESIAN_POINT('Ctrl Pts',(-6.62475642100836,1.39255020108145,65.2370814097977));
#25440=CARTESIAN_POINT('Ctrl Pts',(-6.66044309148477,1.21046419699874,65.2457959604321));
#25441=CARTESIAN_POINT('Ctrl Pts',(-6.68860767397279,1.02704254228941,65.2545105110666));
#25442=CARTESIAN_POINT('Ctrl Pts',(-6.71670982045616,0.844027501641936,
65.2632057430507));
#25443=CARTESIAN_POINT('Ctrl Pts',(-6.73732310326782,0.659682999136313,
65.2719009750348));
#25444=CARTESIAN_POINT('Ctrl Pts',(-6.75033471810914,0.4746263725189,65.2805962070188));
#25445=CARTESIAN_POINT('Ctrl Pts',(-6.76142011326569,0.316965247638418,
65.2880042100758));
#25446=CARTESIAN_POINT('Ctrl Pts',(-6.76698872150269,0.158787577000224,
65.2954122131328));
#25447=CARTESIAN_POINT('Ctrl Pts',(-6.76699998287805,0.00048138183613871,
65.3028202161898));
#25448=CARTESIAN_POINT('Ctrl Pts',(-6.767,2.89194522689237E-12,65.3028202161898));
#25449=CARTESIAN_POINT('Ctrl Pts',(-6.76700000000008,-0.186007249412905,
65.3115697279958));
#25450=CARTESIAN_POINT('Ctrl Pts',(-6.75932637295453,-0.372014355524879,
65.3203192398017));
#25451=CARTESIAN_POINT('Ctrl Pts',(-6.74400518266949,-0.557389537152518,
65.3290687516077));
#25452=CARTESIAN_POINT('Ctrl Pts',(-6.72868405709673,-0.742763935808937,
65.3378182264582));
#25453=CARTESIAN_POINT('Ctrl Pts',(-6.70571545653024,-0.92750612969265,
65.3465677013087));
#25454=CARTESIAN_POINT('Ctrl Pts',(-6.67517739415689,-1.11098863924745,
65.3553171761593));
#25455=CARTESIAN_POINT('Ctrl Pts',(-6.6446394582311,-1.29447038906452,65.3640666147813));
#25456=CARTESIAN_POINT('Ctrl Pts',(-6.60653217027165,-1.47669218228184,
65.3728160534033));
#25457=CARTESIAN_POINT('Ctrl Pts',(-6.56098496116716,-1.65703510504105,
65.3815654920253));
#25458=CARTESIAN_POINT('Ctrl Pts',(-6.51543793687516,-1.83737729604025,
65.3903148951455));
#25459=CARTESIAN_POINT('Ctrl Pts',(-6.46245112202632,-2.01584035397077,
65.3990642982658));
#25460=CARTESIAN_POINT('Ctrl Pts',(-6.40220448416228,-2.19181813638186,
65.407813701386));
#25461=CARTESIAN_POINT('Ctrl Pts',(-6.34195808575169,-2.36779521935993,
65.4165630697313));
#25462=CARTESIAN_POINT('Ctrl Pts',(-6.27445201489212,-2.54128677544883,
65.4253124380765));
#25463=CARTESIAN_POINT('Ctrl Pts',(-6.19991555136157,-2.71170355237903,
65.4340618064218));
#25464=CARTESIAN_POINT('Ctrl Pts',(-6.1253793778901,-2.88211966613133,65.4428111407189));
#25465=CARTESIAN_POINT('Ctrl Pts',(-6.04381298133587,-3.04946076210504,
65.4515604750159));
#25466=CARTESIAN_POINT('Ctrl Pts',(-5.95549339426275,-3.21315848206912,
65.460309809313));
#25467=CARTESIAN_POINT('Ctrl Pts',(-5.86717414355121,-3.37685557859705,
65.4690591102886));
#25468=CARTESIAN_POINT('Ctrl Pts',(-5.7721018898619,-3.53690907467391,65.4778084112641));
#25469=CARTESIAN_POINT('Ctrl Pts',(-5.6705995346701,-3.69277536784994,65.4865577122397));
#25470=CARTESIAN_POINT('Ctrl Pts',(-5.56909755761702,-3.84864108035885,
65.4953069806205));
#25471=CARTESIAN_POINT('Ctrl Pts',(-5.46116568338001,-4.00031938104373,
65.5040562490012));
#25472=CARTESIAN_POINT('Ctrl Pts',(-5.3471704868604,-4.14729511663314,65.512805517382));
#25473=CARTESIAN_POINT('Ctrl Pts',(-5.23317570555443,-4.29427031688131,
65.5215547538946));
#25474=CARTESIAN_POINT('Ctrl Pts',(-5.1131178217873,-4.43654275987216,65.5303039904072));
#25475=CARTESIAN_POINT('Ctrl Pts',(-4.98740459171939,-4.57362924147732,
65.5390532269198));
#25476=CARTESIAN_POINT('Ctrl Pts',(-4.86169180910754,-4.71071523514514,
65.547802432291));
#25477=CARTESIAN_POINT('Ctrl Pts',(-4.73032391415356,-4.84261509316597,
65.5565516376621));
#25478=CARTESIAN_POINT('Ctrl Pts',(-4.59374707237218,-4.96888084331593,
65.5653008430332));
#25479=CARTESIAN_POINT('Ctrl Pts',(-4.45717070537329,-5.09514615452788,
65.5740500179894));
#25480=CARTESIAN_POINT('Ctrl Pts',(-4.31538563819439,-5.21577720253691,
65.5827991929457));
#25481=CARTESIAN_POINT('Ctrl Pts',(-4.1688734129058,-5.33036429028703,65.5915483679019));
#25482=CARTESIAN_POINT('Ctrl Pts',(-4.02236168477266,-5.4449509892123,65.6002975131698));
#25483=CARTESIAN_POINT('Ctrl Pts',(-3.87112305634363,-5.55349359238812,
65.6090466584377));
#25484=CARTESIAN_POINT('Ctrl Pts',(-3.71567117316652,-5.65562346102526,
65.6177958037056));
#25485=CARTESIAN_POINT('Ctrl Pts',(-3.56021980457219,-5.7577529915882,65.6265449200118));
#25486=CARTESIAN_POINT('Ctrl Pts',(-3.40055544862305,-5.85346967275401,
65.635294036318));
#25487=CARTESIAN_POINT('Ctrl Pts',(-3.23722036323319,-5.94244842803607,
65.6440431526241));
#25488=CARTESIAN_POINT('Ctrl Pts',(-3.07388580495966,-6.03142689616516,
65.6527922406951));
#25489=CARTESIAN_POINT('Ctrl Pts',(-2.90688079257629,-6.11366734484859,
65.661541328766));
#25490=CARTESIAN_POINT('Ctrl Pts',(-2.7367725109454,-6.18889046787335,65.670290416837));
#25491=CARTESIAN_POINT('Ctrl Pts',(-2.5666647641658,-6.26411335438297,65.6790394773992));
#25492=CARTESIAN_POINT('Ctrl Pts',(-2.39345402972038,-6.33231884350311,
65.6877885379614));
#25493=CARTESIAN_POINT('Ctrl Pts',(-2.21772856473993,-6.39327529621059,
65.6965375985236));
#25494=CARTESIAN_POINT('Ctrl Pts',(-2.04200363768215,-6.45423156232099,
65.7052866323036));
#25495=CARTESIAN_POINT('Ctrl Pts',(-1.86376426620028,-6.50793874252075,
65.7140356660836));
#25496=CARTESIAN_POINT('Ctrl Pts',(-1.68361578194613,-6.55421443796142,
65.7227846998636));
#25497=CARTESIAN_POINT('Ctrl Pts',(-1.50346783419786,-6.60048999558698,
65.7315337075879));
#25498=CARTESIAN_POINT('Ctrl Pts',(-1.32141106257158,-6.63933404145513,
65.7402827153121));
#25499=CARTESIAN_POINT('Ctrl Pts',(-1.13806375958949,-6.67061465527046,
65.7490317230363));
#25500=CARTESIAN_POINT('Ctrl Pts',(-0.954716987417697,-6.70189517852503,
65.7577807054312));
#25501=CARTESIAN_POINT('Ctrl Pts',(-0.770079973807906,-6.72561226535852,
65.7665296878262));
#25502=CARTESIAN_POINT('Ctrl Pts',(-0.584779770549973,-6.74168536939804,
65.7752786702211));
#25503=CARTESIAN_POINT('Ctrl Pts',(-0.391490647551475,-6.75845143942408,
65.7844048508971));
#25504=CARTESIAN_POINT('Ctrl Pts',(-0.197480213101951,-6.76689975924033,
65.7935310315732));
#25505=CARTESIAN_POINT('Ctrl Pts',(-0.00346532629546626,-6.76699911271708,
65.8026572122492));
#25506=CARTESIAN_POINT('Ctrl Pts',(0.184486595298346,-6.76709536139767,
65.8114981997791));
#25507=CARTESIAN_POINT('Ctrl Pts',(0.37244237818748,-6.75935659726758,65.8203391873091));
#25508=CARTESIAN_POINT('Ctrl Pts',(0.559750217724292,-6.74380965728998,
65.829180174839));
#25509=CARTESIAN_POINT('Ctrl Pts',(0.745129914459954,-6.72842275717229,
65.8379301534367));
#25510=CARTESIAN_POINT('Ctrl Pts',(0.929874656316376,-6.70538772273442,
65.8466801320345));
#25511=CARTESIAN_POINT('Ctrl Pts',(1.11335688289995,-6.67478280180706,65.8554301106323));
#25512=CARTESIAN_POINT('Ctrl Pts',(1.29683723119073,-6.64417819417981,65.8641799996572));
#25513=CARTESIAN_POINT('Ctrl Pts',(1.4790548073045,-6.60600390230027,65.8729298886822));
#25514=CARTESIAN_POINT('Ctrl Pts',(1.6593906480502,-6.56038959797081,65.8816797777071));
#25515=CARTESIAN_POINT('Ctrl Pts',(1.83972470264481,-6.51477574543195,65.8904295800681));
#25516=CARTESIAN_POINT('Ctrl Pts',(2.01817678126068,-6.46172209820031,65.899179382429));
#25517=CARTESIAN_POINT('Ctrl Pts',(2.19414072347902,-6.40140886723938,65.90792918479));
#25518=CARTESIAN_POINT('Ctrl Pts',(2.37010298132325,-6.34109621361289,65.9166789033955));
#25519=CARTESIAN_POINT('Ctrl Pts',(2.54357687927145,-6.27352420825877,65.925428622001));
#25520=CARTESIAN_POINT('Ctrl Pts',(2.71397317790207,-6.19892237325393,65.9341783406065));
#25521=CARTESIAN_POINT('Ctrl Pts',(2.88436790207433,-6.12432122756854,65.9429279783647));
#25522=CARTESIAN_POINT('Ctrl Pts',(3.05168482126484,-6.04269049717302,65.951677616123));
#25523=CARTESIAN_POINT('Ctrl Pts',(3.21535561997612,-5.95430745234809,65.9604272538812));
#25524=CARTESIAN_POINT('Ctrl Pts',(3.37902496075494,-5.86592519481394,65.9691768137002));
#25525=CARTESIAN_POINT('Ctrl Pts',(3.53904799385078,-5.77079087940107,65.9779263735193));
#25526=CARTESIAN_POINT('Ctrl Pts',(3.69488118815177,-5.66922763746898,65.9866759333383));
#25527=CARTESIAN_POINT('Ctrl Pts',(3.85071304611019,-5.56766526648923,65.9954254181257));
#25528=CARTESIAN_POINT('Ctrl Pts',(4.00235489706147,-5.45967423580582,66.0041749029131));
#25529=CARTESIAN_POINT('Ctrl Pts',(4.14929168607827,-5.34562133936195,66.0129243877006));
#25530=CARTESIAN_POINT('Ctrl Pts',(4.29622726385921,-5.23156938308396,66.0216738003639));
#25531=CARTESIAN_POINT('Ctrl Pts',(4.43845763092223,-5.11145583677067,66.0304232130272));
#25532=CARTESIAN_POINT('Ctrl Pts',(4.5754997066111,-4.98568866204076,66.0391726256905));
#25533=CARTESIAN_POINT('Ctrl Pts',(4.71254069815441,-4.85992248226019,66.0479219691368));
#25534=CARTESIAN_POINT('Ctrl Pts',(4.84439326931459,-4.72850295733854,66.0566713125831));
#25535=CARTESIAN_POINT('Ctrl Pts',(4.97060959434841,-4.59187644221527,66.0654206560294));
#25536=CARTESIAN_POINT('Ctrl Pts',(5.0968249628065,-4.45525096256509,66.0741699331657));
#25537=CARTESIAN_POINT('Ctrl Pts',(5.21740397615966,-4.31341878218172,66.082919210302));
#25538=CARTESIAN_POINT('Ctrl Pts',(5.33193710452053,-4.16686161438525,66.0916684874383));
#25539=CARTESIAN_POINT('Ctrl Pts',(5.44646940289506,-4.02030550864347,66.1004177011713));
#25540=CARTESIAN_POINT('Ctrl Pts',(5.55495572749791,-3.86902470979953,66.1091669149043));
#25541=CARTESIAN_POINT('Ctrl Pts',(5.65702762491584,-3.71353301465586,66.1179161286372));
#25542=CARTESIAN_POINT('Ctrl Pts',(5.75909881655278,-3.55804239466692,66.1266652818733));
#25543=CARTESIAN_POINT('Ctrl Pts',(5.85475551250903,-3.39834117619345,66.1354144351095));
#25544=CARTESIAN_POINT('Ctrl Pts',(5.94367283728211,-3.23497174691756,66.1441635883456));
#25545=CARTESIAN_POINT('Ctrl Pts',(6.0325895767643,-3.07160339300735,66.1529126839911));
#25546=CARTESIAN_POINT('Ctrl Pts',(6.11476689685403,-2.90456712829255,66.1616617796367));
#25547=CARTESIAN_POINT('Ctrl Pts',(6.18992570525379,-2.73443024475636,66.1704108752822));
#25548=CARTESIAN_POINT('Ctrl Pts',(6.26508404388814,-2.56429442462746,66.1791599162432));
#25549=CARTESIAN_POINT('Ctrl Pts',(6.33322384283428,-2.39105828655694,66.1879089572043));
#25550=CARTESIAN_POINT('Ctrl Pts',(6.39411368720141,-2.21531017131767,66.1966579981653));
#25551=CARTESIAN_POINT('Ctrl Pts',(6.45500317120987,-2.03956309619208,66.2054069873477));
#25552=CARTESIAN_POINT('Ctrl Pts',(6.50864269270159,-1.86130434438333,66.2141559765301));
#25553=CARTESIAN_POINT('Ctrl Pts',(6.55485008446409,-1.68113930719652,66.2229049657125));
#25554=CARTESIAN_POINT('Ctrl Pts',(6.60199664749469,-1.49731239211552,66.2318317792419));
#25555=CARTESIAN_POINT('Ctrl Pts',(6.64140563640962,-1.31150116499389,66.2407585927712));
#25556=CARTESIAN_POINT('Ctrl Pts',(6.67293772282219,-1.12436255155384,66.2496854063006));
#25557=CARTESIAN_POINT('Ctrl Pts',(6.7038449494991,-0.940932395048565,66.2584353204561));
#25558=CARTESIAN_POINT('Ctrl Pts',(6.72718449348962,-0.756227260503922,
66.2671852346117));
#25559=CARTESIAN_POINT('Ctrl Pts',(6.74287707373956,-0.570874564538889,
66.2759351487672));
#25560=CARTESIAN_POINT('Ctrl Pts',(6.75856934538687,-0.385525513629619,
66.2846848908512));
#25561=CARTESIAN_POINT('Ctrl Pts',(6.76661493004112,-0.199529212415323,
66.2934346329351));
#25562=CARTESIAN_POINT('Ctrl Pts',(6.76698649908907,-0.0135174385974741,
66.3021843750191));
#25563=CARTESIAN_POINT('Ctrl Pts',(6.76735806132382,0.172490924448746,66.310933956665));
#25564=CARTESIAN_POINT('Ctrl Pts',(6.76005588896273,0.358514472904385,66.3196835383109));
#25565=CARTESIAN_POINT('Ctrl Pts',(6.7451047845456,0.543921359665198,66.3284331199568));
#25566=CARTESIAN_POINT('Ctrl Pts',(6.73015393440655,0.72932509315348,66.3371825527959));
#25567=CARTESIAN_POINT('Ctrl Pts',(6.70755443556855,0.914111900259432,66.3459319856349));
#25568=CARTESIAN_POINT('Ctrl Pts',(6.67738304682267,1.0976541559185,66.3546814184739));
#25569=CARTESIAN_POINT('Ctrl Pts',(6.647212131118,1.28119353391585,66.3634307141353));
#25570=CARTESIAN_POINT('Ctrl Pts',(6.60946960955425,1.46348811672965,66.3721800097966));
#25571=CARTESIAN_POINT('Ctrl Pts',(6.56428366991105,1.64391876348533,66.3809293054579));
#25572=CARTESIAN_POINT('Ctrl Pts',(6.51909837867631,1.82434682110023,66.3896784755687));
#25573=CARTESIAN_POINT('Ctrl Pts',(6.46646995271828,2.00291071820747,66.3984276456796));
#25574=CARTESIAN_POINT('Ctrl Pts',(6.40657713281448,2.17900400213,66.4071768157904));
#25575=CARTESIAN_POINT('Ctrl Pts',(6.34668509278951,2.35509499309951,66.4159258719762));
#25576=CARTESIAN_POINT('Ctrl Pts',(6.27952894037409,2.52871516398412,66.424674928162));
#25577=CARTESIAN_POINT('Ctrl Pts',(6.20533675061323,2.69927486771705,66.4334239843477));
#25578=CARTESIAN_POINT('Ctrl Pts',(6.12832117907792,2.87632521636188,66.44250598563));
#25579=CARTESIAN_POINT('Ctrl Pts',(6.04372366625955,3.05007728920243,66.4515879869122));
#25580=CARTESIAN_POINT('Ctrl Pts',(5.95185378007745,3.21989527478422,66.4606699881945));
#25581=CARTESIAN_POINT('Ctrl Pts',(5.86334450817242,3.38350129286976,66.4694197685016));
#25582=CARTESIAN_POINT('Ctrl Pts',(5.76808562057119,3.54345567125184,66.4781695488088));
#25583=CARTESIAN_POINT('Ctrl Pts',(5.6664006880434,3.69921508465529,66.4869193291159));
#25584=CARTESIAN_POINT('Ctrl Pts',(5.56471941107771,3.85496889852504,66.4956687948694));
#25585=CARTESIAN_POINT('Ctrl Pts',(5.45661270814951,4.00652780919858,66.5044182606229));
#25586=CARTESIAN_POINT('Ctrl Pts',(5.34244776448942,4.15337704569451,66.5131677263764));
#25587=CARTESIAN_POINT('Ctrl Pts',(5.22828631819414,4.3002217835647,66.5219169240959));
#25588=CARTESIAN_POINT('Ctrl Pts',(5.10806717843878,4.44235690972898,66.5306661218155));
#25589=CARTESIAN_POINT('Ctrl Pts',(4.98219864544519,4.57929969070863,66.5394153195351));
#25590=CARTESIAN_POINT('Ctrl Pts',(4.85633329943824,4.71623900430207,66.5481642957254));
#25591=CARTESIAN_POINT('Ctrl Pts',(4.72481904033448,4.84798602483812,66.5569132719156));
#25592=CARTESIAN_POINT('Ctrl Pts',(4.58810250736999,4.97409332259309,66.5656622481058));
#25593=CARTESIAN_POINT('Ctrl Pts',(4.45137708685437,5.10020881822314,66.574411793042));
#25594=CARTESIAN_POINT('Ctrl Pts',(4.30944892635841,5.22068366308107,66.5831613379782));
#25595=CARTESIAN_POINT('Ctrl Pts',(4.16280009466445,5.33510865605019,66.5919108829144));
#25596=CARTESIAN_POINT('Ctrl Pts',(4.0161598834857,5.44952692273053,66.6006599135227));
#25597=CARTESIAN_POINT('Ctrl Pts',(3.86479978232009,5.5578958728878,66.6094089441309));
#25598=CARTESIAN_POINT('Ctrl Pts',(3.70923383580844,5.65984746714024,66.6181579747392));
#25599=CARTESIAN_POINT('Ctrl Pts',(3.55366577799305,5.76180044505528,66.6269071240872));
#25600=CARTESIAN_POINT('Ctrl Pts',(3.39389200026593,5.85733573571203,66.6356562734353));
#25601=CARTESIAN_POINT('Ctrl Pts',(3.23045513625782,5.94612887622069,66.6444054227833));
#25602=CARTESIAN_POINT('Ctrl Pts',(3.18695122151402,5.96976399206781,66.6467342868962));
#25603=CARTESIAN_POINT('Ctrl Pts',(3.14318791262572,5.9929216543538,66.6490631510091));
#25604=CARTESIAN_POINT('Ctrl Pts',(3.09917575053252,6.01559628526643,66.6513920151221));
#25605=CARTESIAN_POINT('Origin',(0.,0.,-3.69717978381041));
#25606=CARTESIAN_POINT('',(3.09917575053257,6.0155962852664,69.0457515827422));
#25607=CARTESIAN_POINT('',(3.09917575053259,6.01559628526639,68.6513920151221));
#25608=CARTESIAN_POINT('',(3.09917575053259,6.01559628526639,-3.69717978381041));
#25609=CARTESIAN_POINT('',(-6.767,3.21349643130162E-12,67.6971797838099));
#25610=CARTESIAN_POINT('Ctrl Pts',(-6.767,3.2134964569793E-12,67.6971797838099));
#25611=CARTESIAN_POINT('Ctrl Pts',(-6.76700000000009,-0.186007249412519,
67.7059292956159));
#25612=CARTESIAN_POINT('Ctrl Pts',(-6.75932637295455,-0.37201435552443,
67.7146788074218));
#25613=CARTESIAN_POINT('Ctrl Pts',(-6.74400518266953,-0.557389537152005,
67.7234283192278));
#25614=CARTESIAN_POINT('Ctrl Pts',(-6.72868405709677,-0.742763935808616,
67.7321777940783));
#25615=CARTESIAN_POINT('Ctrl Pts',(-6.70571545653027,-0.927506129692518,
67.7409272689289));
#25616=CARTESIAN_POINT('Ctrl Pts',(-6.67517739415688,-1.1109886392475,67.7496767437794));
#25617=CARTESIAN_POINT('Ctrl Pts',(-6.64463945823111,-1.29447038906445,
67.7584261824014));
#25618=CARTESIAN_POINT('Ctrl Pts',(-6.60653217027169,-1.47669218228164,
67.7671756210234));
#25619=CARTESIAN_POINT('Ctrl Pts',(-6.56098496116724,-1.65703510504073,
67.7759250596454));
#25620=CARTESIAN_POINT('Ctrl Pts',(-6.51543793687527,-1.83737729603987,
67.7846744627656));
#25621=CARTESIAN_POINT('Ctrl Pts',(-6.46245112202646,-2.01584035397033,
67.7934238658859));
#25622=CARTESIAN_POINT('Ctrl Pts',(-6.40220448416245,-2.19181813638136,
67.8021732690061));
#25623=CARTESIAN_POINT('Ctrl Pts',(-6.34195808575187,-2.36779521935944,
67.8109226373514));
#25624=CARTESIAN_POINT('Ctrl Pts',(-6.27445201489232,-2.54128677544834,
67.8196720056966));
#25625=CARTESIAN_POINT('Ctrl Pts',(-6.19991555136178,-2.71170355237854,
67.8284213740419));
#25626=CARTESIAN_POINT('Ctrl Pts',(-6.12537937789035,-2.88211966613079,
67.837170708339));
#25627=CARTESIAN_POINT('Ctrl Pts',(-6.04381298133617,-3.04946076210445,
67.845920042636));
#25628=CARTESIAN_POINT('Ctrl Pts',(-5.9554933942631,-3.21315848206848,67.8546693769331));
#25629=CARTESIAN_POINT('Ctrl Pts',(-5.86717414355173,-3.37685557859614,
67.8634186779086));
#25630=CARTESIAN_POINT('Ctrl Pts',(-5.77210188986261,-3.53690907467274,
67.8721679788842));
#25631=CARTESIAN_POINT('Ctrl Pts',(-5.67059953467102,-3.69277536784853,
67.8809172798597));
#25632=CARTESIAN_POINT('Ctrl Pts',(-5.56909755761809,-3.84864108035729,
67.8896665482405));
#25633=CARTESIAN_POINT('Ctrl Pts',(-5.46116568338124,-4.00031938104206,
67.8984158166213));
#25634=CARTESIAN_POINT('Ctrl Pts',(-5.34717048686179,-4.14729511663135,
67.907165085002));
#25635=CARTESIAN_POINT('Ctrl Pts',(-5.23317570555586,-4.29427031687956,
67.9159143215146));
#25636=CARTESIAN_POINT('Ctrl Pts',(-5.11311782178878,-4.43654275987045,
67.9246635580272));
#25637=CARTESIAN_POINT('Ctrl Pts',(-4.98740459172092,-4.57362924147565,
67.9334127945399));
#25638=CARTESIAN_POINT('Ctrl Pts',(-4.86169180910908,-4.71071523514356,
67.942161999911));
#25639=CARTESIAN_POINT('Ctrl Pts',(-4.73032391415509,-4.84261509316448,
67.9509112052821));
#25640=CARTESIAN_POINT('Ctrl Pts',(-4.59374707237371,-4.96888084331452,
67.9596604106532));
#25641=CARTESIAN_POINT('Ctrl Pts',(-4.457170705375,-5.09514615452638,67.9684095856094));
#25642=CARTESIAN_POINT('Ctrl Pts',(-4.31538563819628,-5.21577720253533,
67.9771587605656));
#25643=CARTESIAN_POINT('Ctrl Pts',(-4.1688734129079,-5.33036429028539,67.9859079355219));
#25644=CARTESIAN_POINT('Ctrl Pts',(-4.02236168477485,-5.44495098921068,
67.9946570807898));
#25645=CARTESIAN_POINT('Ctrl Pts',(-3.87112305634591,-5.55349359238653,
68.0034062260577));
#25646=CARTESIAN_POINT('Ctrl Pts',(-3.7156711731689,-5.6556234610237,68.0121553713256));
#25647=CARTESIAN_POINT('Ctrl Pts',(-3.56021980457478,-5.75775299158659,
68.0209044876318));
#25648=CARTESIAN_POINT('Ctrl Pts',(-3.40055544862585,-5.85346967275238,
68.0296536039379));
#25649=CARTESIAN_POINT('Ctrl Pts',(-3.2372203632362,-5.94244842803443,68.0384027202441));
#25650=CARTESIAN_POINT('Ctrl Pts',(-3.07388580496283,-6.03142689616354,
68.047151808315));
#25651=CARTESIAN_POINT('Ctrl Pts',(-2.90688079257962,-6.11366734484701,
68.0559008963859));
#25652=CARTESIAN_POINT('Ctrl Pts',(-2.73677251094889,-6.18889046787181,
68.0646499844569));
#25653=CARTESIAN_POINT('Ctrl Pts',(-2.56666476416927,-6.26411335438154,
68.0733990450191));
#25654=CARTESIAN_POINT('Ctrl Pts',(-2.39345402972383,-6.33231884350181,
68.0821481055814));
#25655=CARTESIAN_POINT('Ctrl Pts',(-2.21772856474336,-6.3932752962094,68.0908971661436));
#25656=CARTESIAN_POINT('Ctrl Pts',(-2.04200363768561,-6.4542315623199,68.0996461999236));
#25657=CARTESIAN_POINT('Ctrl Pts',(-1.86376426620378,-6.50793874251975,
68.1083952337036));
#25658=CARTESIAN_POINT('Ctrl Pts',(-1.68361578194965,-6.55421443796052,
68.1171442674836));
#25659=CARTESIAN_POINT('Ctrl Pts',(-1.50346783420135,-6.60048999558619,
68.1258932752078));
#25660=CARTESIAN_POINT('Ctrl Pts',(-1.32141106257502,-6.63933404145445,
68.1346422829321));
#25661=CARTESIAN_POINT('Ctrl Pts',(-1.13806375959289,-6.67061465526988,
68.1433912906563));
#25662=CARTESIAN_POINT('Ctrl Pts',(-0.954716987421232,-6.70189517852452,
68.1521402730512));
#25663=CARTESIAN_POINT('Ctrl Pts',(-0.770079973811584,-6.72561226535809,
68.1608892554461));
#25664=CARTESIAN_POINT('Ctrl Pts',(-0.584779770553788,-6.74168536939771,
68.169638237841));
#25665=CARTESIAN_POINT('Ctrl Pts',(-0.391490647555237,-6.75845143942386,
68.178764418517));
#25666=CARTESIAN_POINT('Ctrl Pts',(-0.197480213105655,-6.76689975924023,
68.1878905991931));
#25667=CARTESIAN_POINT('Ctrl Pts',(-0.003465326299107,-6.76699911271707,
68.1970167798692));
#25668=CARTESIAN_POINT('Ctrl Pts',(0.184486595294705,-6.76709536139777,
68.2058577673991));
#25669=CARTESIAN_POINT('Ctrl Pts',(0.372442378183841,-6.75935659726778,
68.214698754929));
#25670=CARTESIAN_POINT('Ctrl Pts',(0.559750217720661,-6.74380965729028,
68.2235397424589));
#25671=CARTESIAN_POINT('Ctrl Pts',(0.745129914456266,-6.7284227571727,68.2322897210567));
#25672=CARTESIAN_POINT('Ctrl Pts',(0.929874656312636,-6.70538772273494,
68.2410396996545));
#25673=CARTESIAN_POINT('Ctrl Pts',(1.11335688289617,-6.67478280180769,68.2497896782522));
#25674=CARTESIAN_POINT('Ctrl Pts',(1.29683723118696,-6.64417819418055,68.2585395672772));
#25675=CARTESIAN_POINT('Ctrl Pts',(1.47905480730075,-6.60600390230111,68.2672894563021));
#25676=CARTESIAN_POINT('Ctrl Pts',(1.65939064804648,-6.56038959797175,68.2760393453271));
#25677=CARTESIAN_POINT('Ctrl Pts',(1.83972470264112,-6.51477574543299,68.284789147688));
#25678=CARTESIAN_POINT('Ctrl Pts',(2.01817678125701,-6.46172209820146,68.293538950049));
#25679=CARTESIAN_POINT('Ctrl Pts',(2.19414072347539,-6.40140886724063,68.3022887524099));
#25680=CARTESIAN_POINT('Ctrl Pts',(2.37010298131958,-6.34109621361426,68.3110384710154));
#25681=CARTESIAN_POINT('Ctrl Pts',(2.54357687926777,-6.27352420826026,68.3197881896209));
#25682=CARTESIAN_POINT('Ctrl Pts',(2.71397317789837,-6.19892237325555,68.3285379082264));
#25683=CARTESIAN_POINT('Ctrl Pts',(2.88436790207068,-6.12432122757026,68.3372875459847));
#25684=CARTESIAN_POINT('Ctrl Pts',(3.05168482126123,-6.04269049717484,68.3460371837429));
#25685=CARTESIAN_POINT('Ctrl Pts',(3.21535561997257,-5.95430745235001,68.3547868215012));
#25686=CARTESIAN_POINT('Ctrl Pts',(3.37902496075149,-5.86592519481592,68.3635363813202));
#25687=CARTESIAN_POINT('Ctrl Pts',(3.53904799384745,-5.77079087940312,68.3722859411392));
#25688=CARTESIAN_POINT('Ctrl Pts',(3.69488118814855,-5.66922763747109,68.3810355009582));
#25689=CARTESIAN_POINT('Ctrl Pts',(3.85071304610708,-5.56766526649138,68.3897849857456));
#25690=CARTESIAN_POINT('Ctrl Pts',(4.00235489705847,-5.45967423580802,68.3985344705331));
#25691=CARTESIAN_POINT('Ctrl Pts',(4.14929168607538,-5.34562133936419,68.4072839553205));
#25692=CARTESIAN_POINT('Ctrl Pts',(4.29622726385643,-5.23156938308624,68.4160333679838));
#25693=CARTESIAN_POINT('Ctrl Pts',(4.43845763091956,-5.11145583677299,68.4247827806471));
#25694=CARTESIAN_POINT('Ctrl Pts',(4.57549970660854,-4.98568866204311,68.4335321933104));
#25695=CARTESIAN_POINT('Ctrl Pts',(4.71254069815183,-4.8599224822627,68.4422815367568));
#25696=CARTESIAN_POINT('Ctrl Pts',(4.84439326931198,-4.72850295734121,68.4510308802031));
#25697=CARTESIAN_POINT('Ctrl Pts',(4.97060959434579,-4.5918764422181,68.4597802236494));
#25698=CARTESIAN_POINT('Ctrl Pts',(5.096824962804,-4.45525096256795,68.4685295007857));
#25699=CARTESIAN_POINT('Ctrl Pts',(5.21740397615728,-4.3134187821846,68.477278777922));
#25700=CARTESIAN_POINT('Ctrl Pts',(5.33193710451827,-4.16686161438814,68.4860280550583));
#25701=CARTESIAN_POINT('Ctrl Pts',(5.4464694028928,-4.02030550864653,68.4947772687912));
#25702=CARTESIAN_POINT('Ctrl Pts',(5.55495572749567,-3.86902470980275,68.5035264825242));
#25703=CARTESIAN_POINT('Ctrl Pts',(5.65702762491362,-3.71353301465925,68.5122756962572));
#25704=CARTESIAN_POINT('Ctrl Pts',(5.75909881655069,-3.55804239467031,68.5210248494933));
#25705=CARTESIAN_POINT('Ctrl Pts',(5.85475551250706,-3.39834117619685,68.5297740027294));
#25706=CARTESIAN_POINT('Ctrl Pts',(5.94367283728026,-3.23497174692096,68.5385231559655));
#25707=CARTESIAN_POINT('Ctrl Pts',(6.03258957676254,-3.07160339301079,68.5472722516111));
#25708=CARTESIAN_POINT('Ctrl Pts',(6.11476689685237,-2.90456712829604,68.5560213472566));
#25709=CARTESIAN_POINT('Ctrl Pts',(6.18992570525223,-2.7344302447599,68.5647704429021));
#25710=CARTESIAN_POINT('Ctrl Pts',(6.26508404388672,-2.56429442463093,68.5735194838632));
#25711=CARTESIAN_POINT('Ctrl Pts',(6.33322384283301,-2.39105828656032,68.5822685248242));
#25712=CARTESIAN_POINT('Ctrl Pts',(6.39411368720027,-2.21531017132097,68.5910175657853));
#25713=CARTESIAN_POINT('Ctrl Pts',(6.45500317120888,-2.03956309619522,68.5997665549677));
#25714=CARTESIAN_POINT('Ctrl Pts',(6.50864269270074,-1.86130434438631,68.6085155441501));
#25715=CARTESIAN_POINT('Ctrl Pts',(6.55485008446336,-1.68113930719934,68.6172645333325));
#25716=CARTESIAN_POINT('Ctrl Pts',(6.60199664749406,-1.4973123921183,68.6261913468619));
#25717=CARTESIAN_POINT('Ctrl Pts',(6.64140563640908,-1.31150116499662,68.6351181603912));
#25718=CARTESIAN_POINT('Ctrl Pts',(6.67293772282174,-1.12436255155652,68.6440449739206));
#25719=CARTESIAN_POINT('Ctrl Pts',(6.70384494949872,-0.940932395051262,
68.6527948880761));
#25720=CARTESIAN_POINT('Ctrl Pts',(6.72718449348931,-0.756227260506631,
68.6615448022316));
#25721=CARTESIAN_POINT('Ctrl Pts',(6.74287707373933,-0.570874564541605,
68.6702947163872));
#25722=CARTESIAN_POINT('Ctrl Pts',(6.7585693453867,-0.38552551363247,68.6790444584712));
#25723=CARTESIAN_POINT('Ctrl Pts',(6.76661493004103,-0.199529212418304,
68.6877942005551));
#25724=CARTESIAN_POINT('Ctrl Pts',(6.76698649908907,-0.0135174386005844,
68.6965439426391));
#25725=CARTESIAN_POINT('Ctrl Pts',(6.7673580613239,0.172490924445634,68.705293524285));
#25726=CARTESIAN_POINT('Ctrl Pts',(6.7600558889629,0.358514472901276,68.7140431059309));
#25727=CARTESIAN_POINT('Ctrl Pts',(6.74510478454585,0.543921359662094,68.7227926875768));
#25728=CARTESIAN_POINT('Ctrl Pts',(6.73015393440688,0.729325093150383,68.7315421204158));
#25729=CARTESIAN_POINT('Ctrl Pts',(6.70755443556897,0.914111900256345,68.7402915532549));
#25730=CARTESIAN_POINT('Ctrl Pts',(6.67738304682318,1.09765415591543,68.7490409860939));
#25731=CARTESIAN_POINT('Ctrl Pts',(6.64721213111858,1.28119353391286,68.7577902817552));
#25732=CARTESIAN_POINT('Ctrl Pts',(6.6094696095549,1.46348811672673,68.7665395774166));
#25733=CARTESIAN_POINT('Ctrl Pts',(6.56428366991176,1.6439187634825,68.7752888730779));
#25734=CARTESIAN_POINT('Ctrl Pts',(6.51909837867709,1.82434682109747,68.7840380431887));
#25735=CARTESIAN_POINT('Ctrl Pts',(6.46646995271911,2.00291071820479,68.7927872132996));
#25736=CARTESIAN_POINT('Ctrl Pts',(6.40657713281536,2.17900400212741,68.8015363834104));
#25737=CARTESIAN_POINT('Ctrl Pts',(6.34668509279046,2.35509499309694,68.8102854395962));
#25738=CARTESIAN_POINT('Ctrl Pts',(6.27952894037512,2.52871516398158,68.8190344957819));
#25739=CARTESIAN_POINT('Ctrl Pts',(6.20533675061432,2.69927486771453,68.8277835519677));
#25740=CARTESIAN_POINT('Ctrl Pts',(6.12832117907903,2.87632521635952,68.83686555325));
#25741=CARTESIAN_POINT('Ctrl Pts',(6.04372366626067,3.05007728920021,68.8459475545323));
#25742=CARTESIAN_POINT('Ctrl Pts',(5.95185378007858,3.21989527478214,68.8550295558145));
#25743=CARTESIAN_POINT('Ctrl Pts',(5.86334450817363,3.38350129286766,68.8637793361217));
#25744=CARTESIAN_POINT('Ctrl Pts',(5.76808562057249,3.54345567124972,68.8725291164288));
#25745=CARTESIAN_POINT('Ctrl Pts',(5.6664006880448,3.69921508465315,68.8812788967359));
#25746=CARTESIAN_POINT('Ctrl Pts',(5.5647194110792,3.85496889852289,68.8900283624894));
#25747=CARTESIAN_POINT('Ctrl Pts',(5.4566127081511,4.00652780919642,68.8987778282429));
#25748=CARTESIAN_POINT('Ctrl Pts',(5.34244776449111,4.15337704569234,68.9075272939964));
#25749=CARTESIAN_POINT('Ctrl Pts',(5.22828631819588,4.30022178356258,68.9162764917159));
#25750=CARTESIAN_POINT('Ctrl Pts',(5.10806717844059,4.44235690972691,68.9250256894355));
#25751=CARTESIAN_POINT('Ctrl Pts',(4.98219864544705,4.5792996907066,68.9337748871551));
#25752=CARTESIAN_POINT('Ctrl Pts',(4.85633329944003,4.71623900430024,68.9425238633454));
#25753=CARTESIAN_POINT('Ctrl Pts',(4.72481904033618,4.84798602483647,68.9512728395356));
#25754=CARTESIAN_POINT('Ctrl Pts',(4.58810250737159,4.97409332259162,68.9600218157259));
#25755=CARTESIAN_POINT('Ctrl Pts',(4.45137708685601,5.10020881822171,68.968771360662));
#25756=CARTESIAN_POINT('Ctrl Pts',(4.30944892636009,5.22068366307968,68.9775209055982));
#25757=CARTESIAN_POINT('Ctrl Pts',(4.16280009466617,5.33510865604885,68.9862704505344));
#25758=CARTESIAN_POINT('Ctrl Pts',(4.0161598834874,5.44952692272927,68.9950194811427));
#25759=CARTESIAN_POINT('Ctrl Pts',(3.86479978232178,5.55789587288663,69.003768511751));
#25760=CARTESIAN_POINT('Ctrl Pts',(3.7092338358101,5.65984746713915,69.0125175423592));
#25761=CARTESIAN_POINT('Ctrl Pts',(3.55366577799474,5.76180044505424,69.0212666917073));
#25762=CARTESIAN_POINT('Ctrl Pts',(3.39389200026765,5.85733573571103,69.0300158410553));
#25763=CARTESIAN_POINT('Ctrl Pts',(3.23045513625957,5.94612887621974,69.0387649904033));
#25764=CARTESIAN_POINT('Ctrl Pts',(3.18695122151521,5.96976399206718,69.0410938545163));
#25765=CARTESIAN_POINT('Ctrl Pts',(3.14318791262635,5.99292165435348,69.0434227186292));
#25766=CARTESIAN_POINT('Ctrl Pts',(3.09917575053258,6.0155962852664,69.0457515827422));
#25767=CARTESIAN_POINT('Ctrl Pts',(3.09917575053264,6.01559628526636,67.0455611218465));
#25768=CARTESIAN_POINT('Ctrl Pts',(2.94392938397932,6.09557767892451,67.0537718920013));
#25769=CARTESIAN_POINT('Ctrl Pts',(2.78569628280582,6.16948810613674,67.0619826621561));
#25770=CARTESIAN_POINT('Ctrl Pts',(2.62499755773111,6.23712087600567,67.0701934323109));
#25771=CARTESIAN_POINT('Ctrl Pts',(2.46419199460855,6.30479861046969,67.0784096612686));
#25772=CARTESIAN_POINT('Ctrl Pts',(2.30091787514996,6.36619024349981,67.0866258902262));
#25773=CARTESIAN_POINT('Ctrl Pts',(2.13571210467178,6.42113874682353,67.0948421191838));
#25774=CARTESIAN_POINT('Ctrl Pts',(1.97029709898946,6.47615684312379,67.1030687540997));
#25775=CARTESIAN_POINT('Ctrl Pts',(1.8029459010291,6.52471541889638,67.1112953890155));
#25776=CARTESIAN_POINT('Ctrl Pts',(1.63420697239288,6.5667081990433,67.1195220239313));
#25777=CARTESIAN_POINT('Ctrl Pts',(1.61171377658031,6.5723059104558,67.1206186488272));
#25778=CARTESIAN_POINT('Ctrl Pts',(1.58919593090922,6.57778702714842,67.121715273723));
#25779=CARTESIAN_POINT('Ctrl Pts',(1.5666547419559,6.58315136689922,67.1228118986189));
#25780=CARTESIAN_POINT('Ctrl Pts',(1.3975925030413,6.62338470554202,67.131036746941));
#25781=CARTESIAN_POINT('Ctrl Pts',(1.22674213922248,6.65715778207088,67.1392615952631));
#25782=CARTESIAN_POINT('Ctrl Pts',(1.05463850430982,6.68431197844828,67.1474864435852));
#25783=CARTESIAN_POINT('Ctrl Pts',(0.882728696248987,6.71143559317991,67.1557020289045));
#25784=CARTESIAN_POINT('Ctrl Pts',(0.709568778831039,6.73195511582117,67.1639176142237));
#25785=CARTESIAN_POINT('Ctrl Pts',(0.535707054474028,6.74576214758472,67.172133199543));
#25786=CARTESIAN_POINT('Ctrl Pts',(0.362006204685331,6.75955640367678,67.1803411829663));
#25787=CARTESIAN_POINT('Ctrl Pts',(0.187605196610105,6.76665051016176,67.1885491663896));
#25788=CARTESIAN_POINT('Ctrl Pts',(0.0130608670671646,6.76698739571395,
67.1967571498129));
#25789=CARTESIAN_POINT('Ctrl Pts',(-0.161357014407913,6.76732403721051,
67.2049591869895));
#25790=CARTESIAN_POINT('Ctrl Pts',(-0.335917653226478,6.76091320749244,
67.2131612241661));
#25791=CARTESIAN_POINT('Ctrl Pts',(-0.510060678331711,6.74774978080988,
67.2213632613427));
#25792=CARTESIAN_POINT('Ctrl Pts',(-0.684112515557719,6.73459324699577,
67.2295610036222));
#25793=CARTESIAN_POINT('Ctrl Pts',(-0.857746817808679,6.71469118730537,
67.2377587459017));
#25794=CARTESIAN_POINT('Ctrl Pts',(-1.03040471682381,6.68809054361163,67.2459564881812));
#25795=CARTESIAN_POINT('Ctrl Pts',(-1.20302978779612,6.66149495759017,67.2541526717956));
#25796=CARTESIAN_POINT('Ctrl Pts',(-1.37467847013956,6.62820337287994,67.2623488554101));
#25797=CARTESIAN_POINT('Ctrl Pts',(-1.54479820349252,6.58831446657537,67.2705450390245));
#25798=CARTESIAN_POINT('Ctrl Pts',(-1.71490541365946,6.54842849665086,67.2787406192854));
#25799=CARTESIAN_POINT('Ctrl Pts',(-1.88348354943207,6.50194625336897,67.2869361995464));
#25800=CARTESIAN_POINT('Ctrl Pts',(-2.04999146898421,6.44901728770299,67.2951317798074));
#25801=CARTESIAN_POINT('Ctrl Pts',(-2.21651742537692,6.39608258854806,67.3033282478482));
#25802=CARTESIAN_POINT('Ctrl Pts',(-2.38097237672716,6.33669988443642,67.3115247158889));
#25803=CARTESIAN_POINT('Ctrl Pts',(-2.5428314909209,6.27106825100644,67.3197211839297));
#25804=CARTESIAN_POINT('Ctrl Pts',(-2.70473758685117,6.20541756713173,67.3279200311032));
#25805=CARTESIAN_POINT('Ctrl Pts',(-2.86404601234771,6.13351447581643,67.3361188782766));
#25806=CARTESIAN_POINT('Ctrl Pts',(-3.02025297689143,6.05560574637901,67.3443177254501));
#25807=CARTESIAN_POINT('Ctrl Pts',(-3.17662319290361,5.97761559474301,67.3525251412161));
#25808=CARTESIAN_POINT('Ctrl Pts',(-3.32988515067514,5.89360742577439,67.3607325569822));
#25809=CARTESIAN_POINT('Ctrl Pts',(-3.47955981218855,5.80387392294168,67.3689399727482));
#25810=CARTESIAN_POINT('Ctrl Pts',(-3.62931469405645,5.71409232610739,67.3771517874004));
#25811=CARTESIAN_POINT('Ctrl Pts',(-3.77547814668973,5.61857947422762,67.3853636020527));
#25812=CARTESIAN_POINT('Ctrl Pts',(-3.91760119818977,5.51767069078448,67.3935754167049));
#25813=CARTESIAN_POINT('Ctrl Pts',(-4.059933547489,5.41661330381735,67.4017993245026));
#25814=CARTESIAN_POINT('Ctrl Pts',(-4.19821332021664,5.31014432368578,67.4100232323003));
#25815=CARTESIAN_POINT('Ctrl Pts',(-4.33202464246535,5.19863938902026,67.418247140098));
#25816=CARTESIAN_POINT('Ctrl Pts',(-4.4556638329424,5.09561088870684,67.4258458790206));
#25817=CARTESIAN_POINT('Ctrl Pts',(-4.57548834913575,4.98828355846426,67.4334446179433));
#25818=CARTESIAN_POINT('Ctrl Pts',(-4.69119948508499,4.87698025330617,67.441043356866));
#25819=CARTESIAN_POINT('Ctrl Pts',(-4.81349361404285,4.75934472373701,67.4490744002923));
#25820=CARTESIAN_POINT('Ctrl Pts',(-4.93157806935784,4.63689647249755,67.4571054437187));
#25821=CARTESIAN_POINT('Ctrl Pts',(-5.04503820716544,4.50997544208845,67.4651364871451));
#25822=CARTESIAN_POINT('Ctrl Pts',(-5.15836481398825,4.38320378475882,67.4731580788543));
#25823=CARTESIAN_POINT('Ctrl Pts',(-5.26707768355398,4.25197009973112,67.4811796705635));
#25824=CARTESIAN_POINT('Ctrl Pts',(-5.37079616114844,4.11665368902865,67.4892012622726));
#25825=CARTESIAN_POINT('Ctrl Pts',(-5.47441571004999,3.98146634573971,67.4972152028323));
#25826=CARTESIAN_POINT('Ctrl Pts',(-5.57305011945073,3.84220432322443,67.5052291433919));
#25827=CARTESIAN_POINT('Ctrl Pts',(-5.66635657107553,3.69928266146684,67.5132430839515));
#25828=CARTESIAN_POINT('Ctrl Pts',(-5.75958926685771,3.55647397482947,67.5212506897408));
#25829=CARTESIAN_POINT('Ctrl Pts',(-5.84750218570977,3.41001172319943,67.5292582955302));
#25830=CARTESIAN_POINT('Ctrl Pts',(-5.92979385145621,3.26034260151171,67.5372659013195));
#25831=CARTESIAN_POINT('Ctrl Pts',(-6.01204998303797,3.11073810808457,67.545270049364));
#25832=CARTESIAN_POINT('Ctrl Pts',(-6.08868950917054,2.95792982886514,67.5532741974085));
#25833=CARTESIAN_POINT('Ctrl Pts',(-6.15945519598822,2.8023919584194,67.561278345453));
#25834=CARTESIAN_POINT('Ctrl Pts',(-6.23020456345916,2.64688995671955,67.5692806476528));
#25835=CARTESIAN_POINT('Ctrl Pts',(-6.29508263136301,2.48865995930421,67.5772829498525));
#25836=CARTESIAN_POINT('Ctrl Pts',(-6.35387900112164,2.32819901192006,67.5852852520523));
#25837=CARTESIAN_POINT('Ctrl Pts',(-6.41267363960505,2.16774278935247,67.5932873186222));
#25838=CARTESIAN_POINT('Ctrl Pts',(-6.46538680803414,2.00505610189901,67.601289385192));
#25839=CARTESIAN_POINT('Ctrl Pts',(-6.51185703421414,1.8406539506262,67.6092914517618));
#25840=CARTESIAN_POINT('Ctrl Pts',(-6.55835314632055,1.67616022024263,67.6172979758289));
#25841=CARTESIAN_POINT('Ctrl Pts',(-6.59859926635847,1.50994948013485,67.625304499896));
#25842=CARTESIAN_POINT('Ctrl Pts',(-6.6324842955872,1.34255021090059,67.6333110239631));
#25843=CARTESIAN_POINT('Ctrl Pts',(-6.66637931588397,1.17510158365994,67.6413199087697));
#25844=CARTESIAN_POINT('Ctrl Pts',(-6.6939094467974,1.00646410080563,67.6493287935762));
#25845=CARTESIAN_POINT('Ctrl Pts',(-6.71501519550499,0.837173771768535,
67.6573376783828));
#25846=CARTESIAN_POINT('Ctrl Pts',(-6.73614212232804,0.667713571944716,
67.6653545995348));
#25847=CARTESIAN_POINT('Ctrl Pts',(-6.75083175893498,0.497599592758307,
67.6733715206868));
#25848=CARTESIAN_POINT('Ctrl Pts',(-6.75907666069919,0.327370882626328,
67.6813884418388));
#25849=CARTESIAN_POINT('Ctrl Pts',(-6.76436225982512,0.218241538552459,
67.686527888329));
#25850=CARTESIAN_POINT('Ctrl Pts',(-6.7670002793358,0.109065054824402,67.6916673348192));
#25851=CARTESIAN_POINT('Ctrl Pts',(-6.76699999997781,-1.73301632199464E-5,
67.6968067813093));
#25852=CARTESIAN_POINT('',(-6.767,7.47259830383148E-10,67.3028202161548));
#25853=CARTESIAN_POINT('Ctrl Pts',(3.09917575053252,6.01559628526643,66.6513920151221));
#25854=CARTESIAN_POINT('Ctrl Pts',(2.93382384459251,6.10078395293766,66.6601414630345));
#25855=CARTESIAN_POINT('Ctrl Pts',(2.76495772122964,6.17915010267058,66.6688909109469));
#25856=CARTESIAN_POINT('Ctrl Pts',(2.59315093316685,6.25042856433188,66.6776403588593));
#25857=CARTESIAN_POINT('Ctrl Pts',(2.42134553245595,6.3217064504146,66.6863897361193));
#25858=CARTESIAN_POINT('Ctrl Pts',(2.24659977927572,6.38589665313464,66.6951391133793));
#25859=CARTESIAN_POINT('Ctrl Pts',(2.06950718689904,6.4427811543908,66.7038884906393));
#25860=CARTESIAN_POINT('Ctrl Pts',(1.89241596572839,6.49966521519731,66.712637800154));
#25861=CARTESIAN_POINT('Ctrl Pts',(1.71297821457167,6.54924360009554,66.7213871096686));
#25862=CARTESIAN_POINT('Ctrl Pts',(1.53180337335805,6.59134792173565,66.7301364191833));
#25863=CARTESIAN_POINT('Ctrl Pts',(1.35062987477742,6.63345193135313,66.7388856638594));
#25864=CARTESIAN_POINT('Ctrl Pts',(1.1677195910291,6.66808192368245,66.7476349085355));
#25865=CARTESIAN_POINT('Ctrl Pts',(0.983693746906412,6.69512028363175,66.7563841532116));
#25866=CARTESIAN_POINT('Ctrl Pts',(0.799669205419417,6.72215845218872,66.7651333359558));
#25867=CARTESIAN_POINT('Ctrl Pts',(0.614529402873001,6.74160505424583,66.7738825187));
#25868=CARTESIAN_POINT('Ctrl Pts',(0.428903127362753,6.75339404354125,66.7826317014442));
#25869=CARTESIAN_POINT('Ctrl Pts',(0.243278104163323,6.76518295330332,66.7913808251628));
#25870=CARTESIAN_POINT('Ctrl Pts',(0.0571669005385001,6.76931433552276,
66.8001299488814));
#25871=CARTESIAN_POINT('Ctrl Pts',(-0.12879840477819,6.76577415902472,66.8088790726));
#25872=CARTESIAN_POINT('Ctrl Pts',(-0.314762517259757,6.76223400523438,
66.8176281401992));
#25873=CARTESIAN_POINT('Ctrl Pts',(-0.50058044682015,6.75102239665084,66.8263772077984));
#25874=CARTESIAN_POINT('Ctrl Pts',(-0.685621118843231,6.73217741012491,
66.8351262753976));
#25875=CARTESIAN_POINT('Ctrl Pts',(-0.870660665415269,6.71333253821762,
66.8438752897834));
#25876=CARTESIAN_POINT('Ctrl Pts',(-1.0549226788558,6.68685441030598,66.8526243041692));
#25877=CARTESIAN_POINT('Ctrl Pts',(-1.23778137635361,6.65283295028157,66.861373318555));
#25878=CARTESIAN_POINT('Ctrl Pts',(-1.42999922977429,6.61707018862126,66.8705701289217));
#25879=CARTESIAN_POINT('Ctrl Pts',(-1.62066601230776,6.57297172935087,66.8797669392883));
#25880=CARTESIAN_POINT('Ctrl Pts',(-1.80906628496005,6.52070304312509,66.888963749655));
#25881=CARTESIAN_POINT('Ctrl Pts',(-1.98831342541176,6.47097374916367,66.8977137473928));
#25882=CARTESIAN_POINT('Ctrl Pts',(-2.16550875892385,6.41384933990986,66.9064637451305));
#25883=CARTESIAN_POINT('Ctrl Pts',(-2.34005036709733,6.34952386242052,66.9152137428683));
#25884=CARTESIAN_POINT('Ctrl Pts',(-2.51458843542848,6.28519968950292,66.9239635631491));
#25885=CARTESIAN_POINT('Ctrl Pts',(-2.68647261713858,6.21367483972914,66.93271338343));
#25886=CARTESIAN_POINT('Ctrl Pts',(-2.85511905904581,6.13519226745775,66.9414632037109));
#25887=CARTESIAN_POINT('Ctrl Pts',(-3.02376230484788,6.05671118254982,66.9502128581694));
#25888=CARTESIAN_POINT('Ctrl Pts',(-3.18916767375867,5.97127275994789,66.9589625126279));
#25889=CARTESIAN_POINT('Ctrl Pts',(-3.35077334098813,5.87916720440262,66.9677121670865));
#25890=CARTESIAN_POINT('Ctrl Pts',(-3.51237616033454,5.78706327198018,66.9764616673549));
#25891=CARTESIAN_POINT('Ctrl Pts',(-3.67017916298451,5.68829258364782,66.9852111676233));
#25892=CARTESIAN_POINT('Ctrl Pts',(-3.82364636562683,5.5831906174363,66.9939606678918));
#25893=CARTESIAN_POINT('Ctrl Pts',(-3.97711106775081,5.478090363704,67.0027100256002));
#25894=CARTESIAN_POINT('Ctrl Pts',(-4.12623987478277,5.36665920046031,67.0114593833086));
#25895=CARTESIAN_POINT('Ctrl Pts',(-4.27052628210351,5.24927559515246,67.0202087410171));
#25896=CARTESIAN_POINT('Ctrl Pts',(-4.41481053021487,5.1318937464604,67.0289579677936));
#25897=CARTESIAN_POINT('Ctrl Pts',(-4.5542523013313,5.00855981480445,67.0377071945701));
#25898=CARTESIAN_POINT('Ctrl Pts',(-4.68837800627241,4.87969268195253,67.0464564213466));
#25899=CARTESIAN_POINT('Ctrl Pts',(-4.82250188225663,4.75082730635089,67.0552055288175));
#25900=CARTESIAN_POINT('Ctrl Pts',(-4.95130963049816,4.61642907906904,67.0639546362883));
#25901=CARTESIAN_POINT('Ctrl Pts',(-5.07436379030302,4.47695444735164,67.0727037437591));
#25902=CARTESIAN_POINT('Ctrl Pts',(-5.19741643559869,4.33748153224107,67.0814527435489));
#25903=CARTESIAN_POINT('Ctrl Pts',(-5.31471544459966,4.1929325525815,67.0902017433387));
#25904=CARTESIAN_POINT('Ctrl Pts',(-5.42586245272949,4.04379841783197,67.0989507431285));
#25905=CARTESIAN_POINT('Ctrl Pts',(-5.53702160016571,3.89464799488013,67.1077006984706));
#25906=CARTESIAN_POINT('Ctrl Pts',(-5.6420272307877,3.74091164447592,67.1164506538128));
#25907=CARTESIAN_POINT('Ctrl Pts',(-5.74052265230589,3.58311159167043,67.1252006091549));
#25908=CARTESIAN_POINT('Ctrl Pts',(-5.83901427064644,3.42531763195659,67.1339502266374));
#25909=CARTESIAN_POINT('Ctrl Pts',(-5.93099603113573,3.26346052699549,67.1426998441198));
#25910=CARTESIAN_POINT('Ctrl Pts',(-6.01615550620697,3.0980900447107,67.1514494616023));
#25911=CARTESIAN_POINT('Ctrl Pts',(-6.10131214576855,2.93272506867873,67.1601987877534));
#25912=CARTESIAN_POINT('Ctrl Pts',(-6.17964682326917,2.76384720420987,67.1689481139045));
#25913=CARTESIAN_POINT('Ctrl Pts',(-6.25089348286849,2.59203002795728,67.1776974400556));
#25914=CARTESIAN_POINT('Ctrl Pts',(-6.32213814887732,2.42021765941204,67.1864465213871));
#25915=CARTESIAN_POINT('Ctrl Pts',(-6.38629508411105,2.24546640836128,67.1951956027187));
#25916=CARTESIAN_POINT('Ctrl Pts',(-6.4431463981845,2.06836976664282,67.2039446840503));
#25917=CARTESIAN_POINT('Ctrl Pts',(-6.50000285282457,1.8912571116255,67.2126945564847));
#25918=CARTESIAN_POINT('Ctrl Pts',(-6.54955227672125,1.71179891444558,67.2214444289191));
#25919=CARTESIAN_POINT('Ctrl Pts',(-6.5916263592538,1.53060476282758,67.2301943013535));
#25920=CARTESIAN_POINT('Ctrl Pts',(-6.63369752054311,1.34942319169048,67.238943566276));
#25921=CARTESIAN_POINT('Ctrl Pts',(-6.66829431423489,1.16650618647076,67.2476928311985));
#25922=CARTESIAN_POINT('Ctrl Pts',(-6.69529923744774,0.982474997662425,
67.256442096121));
#25923=CARTESIAN_POINT('Ctrl Pts',(-6.72230554730919,0.798434359221862,
67.2651918103007));
#25924=CARTESIAN_POINT('Ctrl Pts',(-6.741719164963,0.613279706284663,67.2739415244804));
#25925=CARTESIAN_POINT('Ctrl Pts',(-6.75347414816993,0.427639953699858,
67.2826912386601));
#25926=CARTESIAN_POINT('Ctrl Pts',(-6.7624883775708,0.285283364476322,67.289400897825));
#25927=CARTESIAN_POINT('Ctrl Pts',(-6.76699999998425,0.142641701617036,
67.2961105569899));
#25928=CARTESIAN_POINT('Ctrl Pts',(-6.767,7.4716449424778E-10,67.3028202161548));
#25929=CARTESIAN_POINT('Ctrl Pts',(-6.767,3.03919765936208E-12,67.3028202161898));
#25930=CARTESIAN_POINT('Ctrl Pts',(-6.76700000000008,-0.186007249412693,
67.3115697279958));
#25931=CARTESIAN_POINT('Ctrl Pts',(-6.75932637295454,-0.372014355524604,
67.3203192398017));
#25932=CARTESIAN_POINT('Ctrl Pts',(-6.74400518266952,-0.557389537152179,
67.3290687516077));
#25933=CARTESIAN_POINT('Ctrl Pts',(-6.72868405709675,-0.74276393580879,
67.3378182264582));
#25934=CARTESIAN_POINT('Ctrl Pts',(-6.70571545653024,-0.927506129692694,
67.3465677013088));
#25935=CARTESIAN_POINT('Ctrl Pts',(-6.67517739415685,-1.11098863924768,
67.3553171761593));
#25936=CARTESIAN_POINT('Ctrl Pts',(-6.64463945823104,-1.29447038906488,
67.3640666147813));
#25937=CARTESIAN_POINT('Ctrl Pts',(-6.60653217027155,-1.47669218228232,
67.3728160534033));
#25938=CARTESIAN_POINT('Ctrl Pts',(-6.56098496116701,-1.65703510504165,
67.3815654920253));
#25939=CARTESIAN_POINT('Ctrl Pts',(-6.51543793687498,-1.8373772960409,67.3903148951456));
#25940=CARTESIAN_POINT('Ctrl Pts',(-6.4624511220261,-2.01584035397147,67.3990642982658));
#25941=CARTESIAN_POINT('Ctrl Pts',(-6.40220448416202,-2.19181813638262,
67.407813701386));
#25942=CARTESIAN_POINT('Ctrl Pts',(-6.34195808575139,-2.36779521936074,
67.4165630697313));
#25943=CARTESIAN_POINT('Ctrl Pts',(-6.27445201489178,-2.54128677544969,
67.4253124380766));
#25944=CARTESIAN_POINT('Ctrl Pts',(-6.19991555136117,-2.71170355237994,
67.4340618064219));
#25945=CARTESIAN_POINT('Ctrl Pts',(-6.1253793778897,-2.88211966613217,67.4428111407189));
#25946=CARTESIAN_POINT('Ctrl Pts',(-6.04381298133548,-3.04946076210581,
67.451560475016));
#25947=CARTESIAN_POINT('Ctrl Pts',(-5.95549339426237,-3.21315848206982,
67.460309809313));
#25948=CARTESIAN_POINT('Ctrl Pts',(-5.86717414355091,-3.37685557859757,
67.4690591102886));
#25949=CARTESIAN_POINT('Ctrl Pts',(-5.77210188986168,-3.53690907467426,
67.4778084112641));
#25950=CARTESIAN_POINT('Ctrl Pts',(-5.67059953466998,-3.69277536785013,
67.4865577122397));
#25951=CARTESIAN_POINT('Ctrl Pts',(-5.569097557617,-3.84864108035887,67.4953069806205));
#25952=CARTESIAN_POINT('Ctrl Pts',(-5.46116568338011,-4.00031938104359,
67.5040562490012));
#25953=CARTESIAN_POINT('Ctrl Pts',(-5.34717048686063,-4.14729511663285,
67.512805517382));
#25954=CARTESIAN_POINT('Ctrl Pts',(-5.23317570555466,-4.29427031688103,
67.5215547538946));
#25955=CARTESIAN_POINT('Ctrl Pts',(-5.11311782178753,-4.43654275987189,
67.5303039904072));
#25956=CARTESIAN_POINT('Ctrl Pts',(-4.98740459171963,-4.57362924147705,
67.5390532269198));
#25957=CARTESIAN_POINT('Ctrl Pts',(-4.86169180910784,-4.71071523514483,
67.547802432291));
#25958=CARTESIAN_POINT('Ctrl Pts',(-4.73032391415391,-4.84261509316563,
67.5565516376621));
#25959=CARTESIAN_POINT('Ctrl Pts',(-4.59374707237259,-4.96888084331555,
67.5653008430332));
#25960=CARTESIAN_POINT('Ctrl Pts',(-4.45717070537371,-5.09514615452751,
67.5740500179894));
#25961=CARTESIAN_POINT('Ctrl Pts',(-4.31538563819482,-5.21577720253655,
67.5827991929456));
#25962=CARTESIAN_POINT('Ctrl Pts',(-4.16887341290624,-5.33036429028668,
67.5915483679019));
#25963=CARTESIAN_POINT('Ctrl Pts',(-4.02236168477337,-5.44495098921177,
67.6002975131697));
#25964=CARTESIAN_POINT('Ctrl Pts',(-3.87112305634461,-5.55349359238743,
67.6090466584377));
#25965=CARTESIAN_POINT('Ctrl Pts',(-3.71567117316779,-5.65562346102443,
67.6177958037056));
#25966=CARTESIAN_POINT('Ctrl Pts',(-3.56021980457348,-5.7577529915874,67.6265449200117));
#25967=CARTESIAN_POINT('Ctrl Pts',(-3.40055544862437,-5.85346967275325,
67.6352940363179));
#25968=CARTESIAN_POINT('Ctrl Pts',(-3.23722036323453,-5.94244842803534,
67.6440431526241));
#25969=CARTESIAN_POINT('Ctrl Pts',(-3.07388580496107,-6.03142689616444,
67.652792240695));
#25970=CARTESIAN_POINT('Ctrl Pts',(-2.90688079257778,-6.11366734484788,
67.6615413287659));
#25971=CARTESIAN_POINT('Ctrl Pts',(-2.73677251094698,-6.18889046787265,
67.6702904168369));
#25972=CARTESIAN_POINT('Ctrl Pts',(-2.56666476416739,-6.26411335438231,
67.6790394773991));
#25973=CARTESIAN_POINT('Ctrl Pts',(-2.39345402972199,-6.3323188435025,67.6877885379613));
#25974=CARTESIAN_POINT('Ctrl Pts',(-2.21772856474156,-6.39327529621002,
67.6965375985235));
#25975=CARTESIAN_POINT('Ctrl Pts',(-2.04200363768404,-6.45423156232039,
67.7052866323035));
#25976=CARTESIAN_POINT('Ctrl Pts',(-1.86376426620244,-6.50793874252012,
67.7140356660835));
#25977=CARTESIAN_POINT('Ctrl Pts',(-1.68361578194855,-6.5542144379608,67.7227846998635));
#25978=CARTESIAN_POINT('Ctrl Pts',(-1.50346783420042,-6.6004899955864,67.7315337075878));
#25979=CARTESIAN_POINT('Ctrl Pts',(-1.32141106257428,-6.63933404145459,
67.740282715312));
#25980=CARTESIAN_POINT('Ctrl Pts',(-1.13806375959234,-6.67061465526997,
67.7490317230362));
#25981=CARTESIAN_POINT('Ctrl Pts',(-0.954716987421247,-6.7018951785245,
67.7577807054311));
#25982=CARTESIAN_POINT('Ctrl Pts',(-0.770079973812172,-6.72561226535801,
67.766529687826));
#25983=CARTESIAN_POINT('Ctrl Pts',(-0.584779770554954,-6.7416853693976,
67.7752786702208));
#25984=CARTESIAN_POINT('Ctrl Pts',(-0.391490647556406,-6.75845143942379,
67.7844048508969));
#25985=CARTESIAN_POINT('Ctrl Pts',(-0.197480213106823,-6.76689975924019,
67.793531031573));
#25986=CARTESIAN_POINT('Ctrl Pts',(-0.0034653263002745,-6.76699911271707,
67.802657212249));
#25987=CARTESIAN_POINT('Ctrl Pts',(0.184486595293601,-6.7670953613978,67.8114981997789));
#25988=CARTESIAN_POINT('Ctrl Pts',(0.3724423781828,-6.75935659726783,67.8203391873089));
#25989=CARTESIAN_POINT('Ctrl Pts',(0.559750217719686,-6.74380965729036,
67.8291801748388));
#25990=CARTESIAN_POINT('Ctrl Pts',(0.745129914455358,-6.7284227571728,67.8379301534365));
#25991=CARTESIAN_POINT('Ctrl Pts',(0.929874656311797,-6.70538772273506,
67.8466801320343));
#25992=CARTESIAN_POINT('Ctrl Pts',(1.1133568828954,-6.67478280180782,67.8554301106321));
#25993=CARTESIAN_POINT('Ctrl Pts',(1.29683723118625,-6.64417819418069,67.864179999657));
#25994=CARTESIAN_POINT('Ctrl Pts',(1.47905480730011,-6.60600390230125,67.872929888682));
#25995=CARTESIAN_POINT('Ctrl Pts',(1.65939064804591,-6.56038959797189,67.8816797777069));
#25996=CARTESIAN_POINT('Ctrl Pts',(1.83972470264048,-6.51477574543317,67.8904295800679));
#25997=CARTESIAN_POINT('Ctrl Pts',(2.01817678125632,-6.46172209820167,67.8991793824288));
#25998=CARTESIAN_POINT('Ctrl Pts',(2.19414072347464,-6.40140886724088,67.9079291847898));
#25999=CARTESIAN_POINT('Ctrl Pts',(2.37010298131884,-6.34109621361454,67.9166789033953));
#26000=CARTESIAN_POINT('Ctrl Pts',(2.54357687926704,-6.27352420826056,67.9254286220007));
#26001=CARTESIAN_POINT('Ctrl Pts',(2.71397317789765,-6.19892237325586,67.9341783406062));
#26002=CARTESIAN_POINT('Ctrl Pts',(2.88436790207003,-6.12432122757057,67.9429279783645));
#26003=CARTESIAN_POINT('Ctrl Pts',(3.05168482126065,-6.04269049717514,67.9516776161228));
#26004=CARTESIAN_POINT('Ctrl Pts',(3.21535561997204,-5.95430745235029,67.960427253881));
#26005=CARTESIAN_POINT('Ctrl Pts',(3.37902496075098,-5.86592519481622,67.9691768137));
#26006=CARTESIAN_POINT('Ctrl Pts',(3.53904799384694,-5.77079087940343,67.9779263735191));
#26007=CARTESIAN_POINT('Ctrl Pts',(3.69488118814805,-5.66922763747141,67.9866759333381));
#26008=CARTESIAN_POINT('Ctrl Pts',(3.85071304610654,-5.56766526649176,67.9954254181255));
#26009=CARTESIAN_POINT('Ctrl Pts',(4.00235489705789,-5.45967423580845,68.0041749029129));
#26010=CARTESIAN_POINT('Ctrl Pts',(4.14929168607475,-5.34562133936467,68.0129243877004));
#26011=CARTESIAN_POINT('Ctrl Pts',(4.29622726385583,-5.23156938308674,68.0216738003637));
#26012=CARTESIAN_POINT('Ctrl Pts',(4.43845763091897,-5.1114558367735,68.030423213027));
#26013=CARTESIAN_POINT('Ctrl Pts',(4.57549970660796,-4.98568866204364,68.0391726256903));
#26014=CARTESIAN_POINT('Ctrl Pts',(4.71254069815131,-4.8599224822632,68.0479219691366));
#26015=CARTESIAN_POINT('Ctrl Pts',(4.84439326931152,-4.72850295734168,68.0566713125829));
#26016=CARTESIAN_POINT('Ctrl Pts',(4.97060959434539,-4.59187644221853,68.0654206560292));
#26017=CARTESIAN_POINT('Ctrl Pts',(5.0968249628037,-4.4552509625683,68.0741699331655));
#26018=CARTESIAN_POINT('Ctrl Pts',(5.21740397615707,-4.31341878218486,68.0829192103018));
#26019=CARTESIAN_POINT('Ctrl Pts',(5.33193710451814,-4.1668616143883,68.0916684874381));
#26020=CARTESIAN_POINT('Ctrl Pts',(5.44646940289264,-4.02030550864675,68.1004177011711));
#26021=CARTESIAN_POINT('Ctrl Pts',(5.55495572749547,-3.86902470980302,68.1091669149041));
#26022=CARTESIAN_POINT('Ctrl Pts',(5.6570276249134,-3.71353301465958,68.117916128637));
#26023=CARTESIAN_POINT('Ctrl Pts',(5.75909881655048,-3.55804239467065,68.1266652818732));
#26024=CARTESIAN_POINT('Ctrl Pts',(5.85475551250685,-3.3983411761972,68.1354144351093));
#26025=CARTESIAN_POINT('Ctrl Pts',(5.94367283728007,-3.23497174692131,68.1441635883454));
#26026=CARTESIAN_POINT('Ctrl Pts',(6.0325895767623,-3.07160339301126,68.1529126839909));
#26027=CARTESIAN_POINT('Ctrl Pts',(6.11476689685209,-2.90456712829663,68.1616617796365));
#26028=CARTESIAN_POINT('Ctrl Pts',(6.18992570525191,-2.73443024476062,68.170410875282));
#26029=CARTESIAN_POINT('Ctrl Pts',(6.26508404388637,-2.56429442463177,68.179159916243));
#26030=CARTESIAN_POINT('Ctrl Pts',(6.33322384283264,-2.3910582865613,68.1879089572041));
#26031=CARTESIAN_POINT('Ctrl Pts',(6.39411368719989,-2.21531017132207,68.1966579981651));
#26032=CARTESIAN_POINT('Ctrl Pts',(6.45500317120842,-2.03956309619664,68.2054069873475));
#26033=CARTESIAN_POINT('Ctrl Pts',(6.50864269270023,-1.86130434438805,68.2141559765299));
#26034=CARTESIAN_POINT('Ctrl Pts',(6.55485008446283,-1.6811393072014,68.2229049657123));
#26035=CARTESIAN_POINT('Ctrl Pts',(6.60199664749361,-1.49731239212032,68.2318317792416));
#26036=CARTESIAN_POINT('Ctrl Pts',(6.6414056364087,-1.31150116499859,68.240758592771));
#26037=CARTESIAN_POINT('Ctrl Pts',(6.67293772282141,-1.12436255155843,68.2496854063004));
#26038=CARTESIAN_POINT('Ctrl Pts',(6.70384494949845,-0.940932395053181,
68.2584353204559));
#26039=CARTESIAN_POINT('Ctrl Pts',(6.7271844934891,-0.756227260508557,68.2671852346114));
#26040=CARTESIAN_POINT('Ctrl Pts',(6.74287707373917,-0.570874564543536,
68.275935148767));
#26041=CARTESIAN_POINT('Ctrl Pts',(6.7585693453866,-0.385525513634341,68.284684890851));
#26042=CARTESIAN_POINT('Ctrl Pts',(6.76661493004097,-0.199529212420114,
68.2934346329349));
#26043=CARTESIAN_POINT('Ctrl Pts',(6.76698649908906,-0.0135174386023304,
68.3021843750189));
#26044=CARTESIAN_POINT('Ctrl Pts',(6.76735806132394,0.172490924443888,68.3109339566648));
#26045=CARTESIAN_POINT('Ctrl Pts',(6.76005588896299,0.358514472899531,68.3196835383107));
#26046=CARTESIAN_POINT('Ctrl Pts',(6.74510478454599,0.543921359660353,68.3284331199566));
#26047=CARTESIAN_POINT('Ctrl Pts',(6.73015393440708,0.729325093148581,68.3371825527956));
#26048=CARTESIAN_POINT('Ctrl Pts',(6.70755443556923,0.914111900254487,68.3459319856347));
#26049=CARTESIAN_POINT('Ctrl Pts',(6.67738304682349,1.09765415591352,68.3546814184737));
#26050=CARTESIAN_POINT('Ctrl Pts',(6.64721213111896,1.28119353391089,68.3634307141351));
#26051=CARTESIAN_POINT('Ctrl Pts',(6.60946960955534,1.46348811672471,68.3721800097964));
#26052=CARTESIAN_POINT('Ctrl Pts',(6.56428366991228,1.64391876348043,68.3809293054577));
#26053=CARTESIAN_POINT('Ctrl Pts',(6.51909837867768,1.82434682109535,68.3896784755685));
#26054=CARTESIAN_POINT('Ctrl Pts',(6.46646995271977,2.00291071820264,68.3984276456794));
#26055=CARTESIAN_POINT('Ctrl Pts',(6.40657713281611,2.17900400212521,68.4071768157902));
#26056=CARTESIAN_POINT('Ctrl Pts',(6.34668509279127,2.35509499309477,68.415925871976));
#26057=CARTESIAN_POINT('Ctrl Pts',(6.27952894037599,2.52871516397942,68.4246749281617));
#26058=CARTESIAN_POINT('Ctrl Pts',(6.20533675061525,2.69927486771241,68.4334239843475));
#26059=CARTESIAN_POINT('Ctrl Pts',(6.12832117907997,2.87632521635753,68.4425059856298));
#26060=CARTESIAN_POINT('Ctrl Pts',(6.04372366626161,3.05007728919837,68.451587986912));
#26061=CARTESIAN_POINT('Ctrl Pts',(5.9518537800795,3.21989527478044,68.4606699881943));
#26062=CARTESIAN_POINT('Ctrl Pts',(5.86334450817457,3.38350129286604,68.4694197685015));
#26063=CARTESIAN_POINT('Ctrl Pts',(5.76808562057344,3.54345567124818,68.4781695488086));
#26064=CARTESIAN_POINT('Ctrl Pts',(5.66640068804575,3.69921508465169,68.4869193291157));
#26065=CARTESIAN_POINT('Ctrl Pts',(5.56471941108019,3.85496889852145,68.4956687948692));
#26066=CARTESIAN_POINT('Ctrl Pts',(5.45661270815213,4.00652780919501,68.5044182606227));
#26067=CARTESIAN_POINT('Ctrl Pts',(5.34244776449218,4.15337704569096,68.5131677263761));
#26068=CARTESIAN_POINT('Ctrl Pts',(5.22828631819699,4.30022178356123,68.5219169240957));
#26069=CARTESIAN_POINT('Ctrl Pts',(5.10806717844173,4.44235690972559,68.5306661218153));
#26070=CARTESIAN_POINT('Ctrl Pts',(4.98219864544823,4.57929969070532,68.5394153195349));
#26071=CARTESIAN_POINT('Ctrl Pts',(4.85633329944151,4.7162390042987,68.5481642957252));
#26072=CARTESIAN_POINT('Ctrl Pts',(4.72481904033797,4.8479860248347,68.5569132719154));
#26073=CARTESIAN_POINT('Ctrl Pts',(4.58810250737372,4.97409332258965,68.5656622481056));
#26074=CARTESIAN_POINT('Ctrl Pts',(4.4513770868582,5.1002088182198,68.5744117930418));
#26075=CARTESIAN_POINT('Ctrl Pts',(4.30944892636232,5.22068366307784,68.583161337978));
#26076=CARTESIAN_POINT('Ctrl Pts',(4.16280009466845,5.33510865604707,68.5919108829141));
#26077=CARTESIAN_POINT('Ctrl Pts',(4.01615988348994,5.44952692272739,68.6006599135224));
#26078=CARTESIAN_POINT('Ctrl Pts',(3.86479978232458,5.55789587288468,68.6094089441307));
#26079=CARTESIAN_POINT('Ctrl Pts',(3.70923383581317,5.65984746713714,68.6181579747389));
#26080=CARTESIAN_POINT('Ctrl Pts',(3.55366577799792,5.76180044505228,68.626907124087));
#26081=CARTESIAN_POINT('Ctrl Pts',(3.39389200027093,5.85733573570912,68.635656273435));
#26082=CARTESIAN_POINT('Ctrl Pts',(3.23045513626296,5.9461288762179,68.644405422783));
#26083=CARTESIAN_POINT('Ctrl Pts',(3.18695122151749,5.96976399206598,68.646734286896));
#26084=CARTESIAN_POINT('Ctrl Pts',(3.1431879126275,5.99292165435288,68.6490631510091));
#26085=CARTESIAN_POINT('Ctrl Pts',(3.09917575053259,6.01559628526639,68.6513920151221));
#26086=CARTESIAN_POINT('Origin',(0.,0.,-3.69717978381041));
#26087=CARTESIAN_POINT('',(3.09917575053257,6.0155962852664,71.0459800471047));
#26088=CARTESIAN_POINT('',(3.09917575053263,6.01559628526637,70.6515467266273));
#26089=CARTESIAN_POINT('',(3.09917575053259,6.01559628526639,-3.69717978381041));
#26090=CARTESIAN_POINT('',(-6.767,3.55173084953114E-12,69.6971797838099));
#26091=CARTESIAN_POINT('Ctrl Pts',(-6.76699999999339,9.45791233018501E-6,
69.6973826905095));
#26092=CARTESIAN_POINT('Ctrl Pts',(-6.76700023814962,-0.170387891941315,
69.7054353713839));
#26093=CARTESIAN_POINT('Ctrl Pts',(-6.76056010934896,-0.341058540649849,
69.7134880522583));
#26094=CARTESIAN_POINT('Ctrl Pts',(-6.7476435435305,-0.511464181982631,
69.7215407331328));
#26095=CARTESIAN_POINT('Ctrl Pts',(-6.7347406520964,-0.681689419927384,
69.7295848888733));
#26096=CARTESIAN_POINT('Ctrl Pts',(-6.71537499519369,-0.851649838935862,
69.7376290446138));
#26097=CARTESIAN_POINT('Ctrl Pts',(-6.68956246968668,-1.02080505688376,
69.7456732003543));
#26098=CARTESIAN_POINT('Ctrl Pts',(-6.66377158270051,-1.18981847279425,
69.7537106127162));
#26099=CARTESIAN_POINT('Ctrl Pts',(-6.63154463910887,-1.3580276630686,69.7617480250781));
#26100=CARTESIAN_POINT('Ctrl Pts',(-6.59294948837972,-1.52489542056944,
69.76978543744));
#26101=CARTESIAN_POINT('Ctrl Pts',(-6.55437819706301,-1.69166002089703,
69.7778178810965));
#26102=CARTESIAN_POINT('Ctrl Pts',(-6.50944661927347,-1.8570844755594,69.785850324753));
#26103=CARTESIAN_POINT('Ctrl Pts',(-6.45827400213015,-2.02063997619809,
69.7938827684094));
#26104=CARTESIAN_POINT('Ctrl Pts',(-6.40703937467019,-2.18439367128042,
69.8019249456774));
#26105=CARTESIAN_POINT('Ctrl Pts',(-6.34954865059723,-2.34627351135502,
69.8099671229453));
#26106=CARTESIAN_POINT('Ctrl Pts',(-6.28597224545374,-2.50576174633288,
69.8180093002133));
#26107=CARTESIAN_POINT('Ctrl Pts',(-6.22249789812155,-2.66499395833884,
69.8260385675501));
#26108=CARTESIAN_POINT('Ctrl Pts',(-6.15295753512077,-2.82184188993491,
69.834067834887));
#26109=CARTESIAN_POINT('Ctrl Pts',(-6.07756960555274,-2.97580857745615,
69.8420971022238));
#26110=CARTESIAN_POINT('Ctrl Pts',(-6.00217581822731,-3.12978722842443,
69.850126993447));
#26111=CARTESIAN_POINT('Ctrl Pts',(-5.92093372446528,-3.28088385300036,
69.8581568846703));
#26112=CARTESIAN_POINT('Ctrl Pts',(-5.83410840710039,-3.42862481094105,
69.8661867758935));
#26113=CARTESIAN_POINT('Ctrl Pts',(-5.74725905045123,-3.57640667385042,
69.8742188903488));
#26114=CARTESIAN_POINT('Ctrl Pts',(-5.65482358347639,-3.72083069817106,
69.8822510048042));
#26115=CARTESIAN_POINT('Ctrl Pts',(-5.55711110814656,-3.86145116914796,
69.8902831192596));
#26116=CARTESIAN_POINT('Ctrl Pts',(-5.45916898367373,-4.00240213395934,
69.8983341112246));
#26117=CARTESIAN_POINT('Ctrl Pts',(-5.35592524515943,-4.13953134509173,
69.9063851031897));
#26118=CARTESIAN_POINT('Ctrl Pts',(-5.24773194102639,-4.27242302155713,
69.9144360951548));
#26119=CARTESIAN_POINT('Ctrl Pts',(-5.13961422382154,-4.40522185610699,
69.9224814624672));
#26120=CARTESIAN_POINT('Ctrl Pts',(-5.02655413405461,-4.53378882241542,
69.9305268297797));
#26121=CARTESIAN_POINT('Ctrl Pts',(-4.90893979515681,-4.657746138158,69.9385721970921));
#26122=CARTESIAN_POINT('Ctrl Pts',(-4.79113743472779,-4.78190161548982,
69.946630425951));
#26123=CARTESIAN_POINT('Ctrl Pts',(-4.66876654729672,-4.90143245847534,
69.9546886548099));
#26124=CARTESIAN_POINT('Ctrl Pts',(-4.54224976776608,-5.01600000470784,
69.9627468836688));
#26125=CARTESIAN_POINT('Ctrl Pts',(-4.41587192249547,-5.13044173871749,
69.9707962633926));
#26126=CARTESIAN_POINT('Ctrl Pts',(-4.28535761607779,-5.23993089425125,
69.9788456431165));
#26127=CARTESIAN_POINT('Ctrl Pts',(-4.15115592680216,-5.34417378753492,
69.9868950228404));
#26128=CARTESIAN_POINT('Ctrl Pts',(-4.01391333858133,-5.45077873830045,
69.995126794831));
#26129=CARTESIAN_POINT('Ctrl Pts',(-3.87236008956517,-5.55225004774207,
70.0033585668217));
#26130=CARTESIAN_POINT('Ctrl Pts',(-3.72691577815881,-5.64821987731629,
70.0115903388123));
#26131=CARTESIAN_POINT('Ctrl Pts',(-3.58164514179658,-5.74407510932239,
70.0198122812445));
#26132=CARTESIAN_POINT('Ctrl Pts',(-3.43249299106102,-5.83444174709155,
70.0280342236766));
#26133=CARTESIAN_POINT('Ctrl Pts',(-3.27991217517725,-5.91899190091726,
70.0362561661088));
#26134=CARTESIAN_POINT('Ctrl Pts',(-3.12748298512894,-6.00345803377585,
70.0444699380585));
#26135=CARTESIAN_POINT('Ctrl Pts',(-2.97163222661652,-6.08211902122219,
70.0526837100081));
#26136=CARTESIAN_POINT('Ctrl Pts',(-2.81284200812162,-6.15468998710303,
70.0608974819577));
#26137=CARTESIAN_POINT('Ctrl Pts',(-2.65417778254027,-6.22720337117867,
70.0691047366479));
#26138=CARTESIAN_POINT('Ctrl Pts',(-2.49257906689244,-6.29363621003319,
70.077311991338));
#26139=CARTESIAN_POINT('Ctrl Pts',(-2.32855295424396,-6.35374929779904,
70.0855192460282));
#26140=CARTESIAN_POINT('Ctrl Pts',(-2.1646241453794,-6.41382672520076,70.093721632));
#26141=CARTESIAN_POINT('Ctrl Pts',(-1.99827114366252,-6.46759174702125,
70.1019240179719));
#26142=CARTESIAN_POINT('Ctrl Pts',(-1.83002151089933,-6.51485305050281,
70.1101264039437));
#26143=CARTESIAN_POINT('Ctrl Pts',(-1.66182209656591,-6.56210024763292,
70.1183263417025));
#26144=CARTESIAN_POINT('Ctrl Pts',(-1.49172752230965,-6.60284749270681,
70.1265262794613));
#26145=CARTESIAN_POINT('Ctrl Pts',(-1.32028126071456,-6.63695309555567,
70.1347262172201));
#26146=CARTESIAN_POINT('Ctrl Pts',(-1.14885897172868,-6.67105392956162,
70.1429250084162));
#26147=CARTESIAN_POINT('Ctrl Pts',(-0.97608572307747,-6.69851490021167,
70.1511237996122));
#26148=CARTESIAN_POINT('Ctrl Pts',(-0.802515971789543,-6.71924527867697,
70.1593225908082));
#26149=CARTESIAN_POINT('Ctrl Pts',(-0.628939003574673,-6.73997651909905,
70.1675217229051));
#26150=CARTESIAN_POINT('Ctrl Pts',(-0.45456582265216,-6.75397656721264,
70.175720855002));
#26151=CARTESIAN_POINT('Ctrl Pts',(-0.279956871417882,-6.76120648628231,
70.1839199870989));
#26152=CARTESIAN_POINT('Ctrl Pts',(-0.105308985192508,-6.76843801750778,
70.1921209474705));
#26153=CARTESIAN_POINT('Ctrl Pts',(0.0695744180061118,-6.76889639811614,
70.2003219078421));
#26154=CARTESIAN_POINT('Ctrl Pts',(0.244131967469593,-6.76259481134715,
70.2085228682137));
#26155=CARTESIAN_POINT('Ctrl Pts',(0.418853119391245,-6.75628731847391,
70.21673151486));
#26156=CARTESIAN_POINT('Ctrl Pts',(0.593247448734452,-6.74320721279566,
70.2249401615063));
#26157=CARTESIAN_POINT('Ctrl Pts',(0.766756831578491,-6.72341973710014,
70.2331488081527));
#26158=CARTESIAN_POINT('Ctrl Pts',(0.940349052680784,-6.70362281430732,
70.2413613738377));
#26159=CARTESIAN_POINT('Ctrl Pts',(1.11305513080198,-6.67711219103453,70.2495739395228));
#26160=CARTESIAN_POINT('Ctrl Pts',(1.28432629738894,-6.64400443722272,70.2577865052078));
#26161=CARTESIAN_POINT('Ctrl Pts',(1.45583247274901,-6.61085125479174,70.2660103397189));
#26162=CARTESIAN_POINT('Ctrl Pts',(1.62589945247983,-6.57108293215374,70.27423417423));
#26163=CARTESIAN_POINT('Ctrl Pts',(1.79399161177041,-6.52486651946976,70.2824580087412));
#26164=CARTESIAN_POINT('Ctrl Pts',(1.94843669693945,-6.48240232706894,70.2900141661898));
#26165=CARTESIAN_POINT('Ctrl Pts',(2.10121458872838,-6.43449519935904,70.2975703236385));
#26166=CARTESIAN_POINT('Ctrl Pts',(2.25192491332738,-6.38131045982998,70.3051264810871));
#26167=CARTESIAN_POINT('Ctrl Pts',(2.42436692962267,-6.32045674098269,70.3137721994834));
#26168=CARTESIAN_POINT('Ctrl Pts',(2.59449505643908,-6.2525546804886,70.3224179178797));
#26169=CARTESIAN_POINT('Ctrl Pts',(2.7617273009984,-6.17779502046807,70.3310636362759));
#26170=CARTESIAN_POINT('Ctrl Pts',(2.92874485337425,-6.10313133664333,70.3396982553285));
#26171=CARTESIAN_POINT('Ctrl Pts',(3.09287365973293,-6.02162773232303,70.348332874381));
#26172=CARTESIAN_POINT('Ctrl Pts',(3.25354948255545,-5.93352380669052,70.3569674934336));
#26173=CARTESIAN_POINT('Ctrl Pts',(3.41989974152747,-5.84230839800014,70.365907053165));
#26174=CARTESIAN_POINT('Ctrl Pts',(3.58254836182367,-5.74401804445167,70.3748466128964));
#26175=CARTESIAN_POINT('Ctrl Pts',(3.74089174189155,-5.63897313129329,70.3837861726279));
#26176=CARTESIAN_POINT('Ctrl Pts',(3.89340931949669,-5.53779305235478,70.3923968262245));
#26177=CARTESIAN_POINT('Ctrl Pts',(4.04193248917253,-5.43034673214416,70.4010074798212));
#26178=CARTESIAN_POINT('Ctrl Pts',(4.18594637031747,-5.31696736728993,70.4096181334179));
#26179=CARTESIAN_POINT('Ctrl Pts',(4.3298239325841,-5.2036953236725,70.4182206364486));
#26180=CARTESIAN_POINT('Ctrl Pts',(4.46920047740784,-5.08450162030227,70.4268231394793));
#26181=CARTESIAN_POINT('Ctrl Pts',(4.60359068792702,-4.95976227031414,70.43542564251));
#26182=CARTESIAN_POINT('Ctrl Pts',(4.7378296448132,-4.83516331209852,70.4440184635867));
#26183=CARTESIAN_POINT('Ctrl Pts',(4.86709324015349,-4.70503136595633,70.4526112846635));
#26184=CARTESIAN_POINT('Ctrl Pts',(4.99092964177323,-4.56978230453808,70.4612041057402));
#26185=CARTESIAN_POINT('Ctrl Pts',(5.00552430251826,-4.55384261199481,70.4622168072304));
#26186=CARTESIAN_POINT('Ctrl Pts',(5.02004362027724,-4.53783188958982,70.4632295087205));
#26187=CARTESIAN_POINT('Ctrl Pts',(5.03448688702477,-4.52175085385912,70.4642422102107));
#26188=CARTESIAN_POINT('Ctrl Pts',(5.15707344790452,-4.38526380421377,70.4728374674366));
#26189=CARTESIAN_POINT('Ctrl Pts',(5.27403422616259,-4.24386923268498,70.4814327246625));
#26190=CARTESIAN_POINT('Ctrl Pts',(5.38499870673418,-4.09805782395408,70.4900279818884));
#26191=CARTESIAN_POINT('Ctrl Pts',(5.49606710069976,-3.95210986920155,70.4986312881977));
#26192=CARTESIAN_POINT('Ctrl Pts',(5.60112780376439,-3.80173706426982,70.5072345945069));
#26193=CARTESIAN_POINT('Ctrl Pts',(5.69985346619164,-3.64745931628348,70.5158379008161));
#26194=CARTESIAN_POINT('Ctrl Pts',(5.80267233843029,-3.48678514434604,70.5247979040259));
#26195=CARTESIAN_POINT('Ctrl Pts',(5.89861947511329,-3.32187565648612,70.5337579072358));
#26196=CARTESIAN_POINT('Ctrl Pts',(5.98737850424075,-3.15334546901474,70.5427179104456));
#26197=CARTESIAN_POINT('Ctrl Pts',(6.07283719878345,-2.99108175394348,70.5513447530883));
#26198=CARTESIAN_POINT('Ctrl Pts',(6.15163261348022,-2.82546202870845,70.5599715957312));
#26199=CARTESIAN_POINT('Ctrl Pts',(6.22353184835703,-2.65705482301094,70.5685984383739));
#26200=CARTESIAN_POINT('Ctrl Pts',(6.29549980069985,-2.48848666265999,70.5772335260943));
#26201=CARTESIAN_POINT('Ctrl Pts',(6.36055830594989,-2.31712598789673,70.5858686138146));
#26202=CARTESIAN_POINT('Ctrl Pts',(6.4185237904181,-2.14355810554249,70.5945037015349));
#26203=CARTESIAN_POINT('Ctrl Pts',(6.47657536526006,-1.9697324400609,70.6031516140929));
#26204=CARTESIAN_POINT('Ctrl Pts',(6.5275127786828,-1.79369330782663,70.6117995266509));
#26205=CARTESIAN_POINT('Ctrl Pts',(6.57120277754873,-1.61603931150697,70.6204474392089));
#26206=CARTESIAN_POINT('Ctrl Pts',(6.57610414329484,-1.59610918482298,70.6214176059172));
#26207=CARTESIAN_POINT('Ctrl Pts',(6.58091435011396,-1.5761587425345,70.6223877726256));
#26208=CARTESIAN_POINT('Ctrl Pts',(6.58563325034586,-1.55618883556562,70.6233579393339));
#26209=CARTESIAN_POINT('Ctrl Pts',(6.62563817172745,-1.38689206745695,70.6315826190234));
#26210=CARTESIAN_POINT('Ctrl Pts',(6.65916345610177,-1.21582859578257,70.6398072987129));
#26211=CARTESIAN_POINT('Ctrl Pts',(6.68605437655763,-1.04353527669869,70.6480319784024));
#26212=CARTESIAN_POINT('Ctrl Pts',(6.71291703161691,-0.871423057365544,
70.6562480130241));
#26213=CARTESIAN_POINT('Ctrl Pts',(6.73315915458184,-0.698083916077889,
70.6644640476457));
#26214=CARTESIAN_POINT('Ctrl Pts',(6.74667636948375,-0.524067710748956,
70.6726800822673));
#26215=CARTESIAN_POINT('Ctrl Pts',(6.76018208378677,-0.350199560370123,
70.680889126594));
#26216=CARTESIAN_POINT('Ctrl Pts',(6.76697425772295,-0.175655848560904,
70.6890981709207));
#26217=CARTESIAN_POINT('Ctrl Pts',(6.76699992692022,-0.00099451580590046,
70.6973072152474));
#26218=CARTESIAN_POINT('Ctrl Pts',(6.76702557941799,0.173553188203546,70.705510919048));
#26219=CARTESIAN_POINT('Ctrl Pts',(6.76029349563374,0.348218003599608,70.7137146228486));
#26220=CARTESIAN_POINT('Ctrl Pts',(6.7468026937055,0.522438907632548,70.7219183266492));
#26221=CARTESIAN_POINT('Ctrl Pts',(6.73331796751756,0.696581349245336,70.7301183358159));
#26222=CARTESIAN_POINT('Ctrl Pts',(6.71308061502162,0.870279921184807,70.7383183449826));
#26223=CARTESIAN_POINT('Ctrl Pts',(6.68614171254121,1.04297555091983,70.7465183541493));
#26224=CARTESIAN_POINT('Ctrl Pts',(6.65920496415265,1.21565737154555,70.7547177076259));
#26225=CARTESIAN_POINT('Ctrl Pts',(6.62556777971534,1.3873360544997,70.7629170611024));
#26226=CARTESIAN_POINT('Ctrl Pts',(6.58533293037598,1.5574592116989,70.771116414579));
#26227=CARTESIAN_POINT('Ctrl Pts',(6.54509834335656,1.7275812597428,70.779315714598));
#26228=CARTESIAN_POINT('Ctrl Pts',(6.49826625857153,1.89614745309137,70.7875150146171));
#26229=CARTESIAN_POINT('Ctrl Pts',(6.44499022875867,2.06261725756509,70.7957143146362));
#26230=CARTESIAN_POINT('Ctrl Pts',(6.39170488149717,2.22911617595471,70.8039150486314));
#26231=CARTESIAN_POINT('Ctrl Pts',(6.33197345316412,2.39351763354346,70.8121157826267));
#26232=CARTESIAN_POINT('Ctrl Pts',(6.26599888527343,2.55529782408082,70.8203165166219));
#26233=CARTESIAN_POINT('Ctrl Pts',(6.20000081052336,2.71713565719636,70.8285201725537));
#26234=CARTESIAN_POINT('Ctrl Pts',(6.12775530030852,2.87635003099543,70.8367238284854));
#26235=CARTESIAN_POINT('Ctrl Pts',(6.04951281281268,3.03243857771517,70.8449274844172));
#26236=CARTESIAN_POINT('Ctrl Pts',(5.97118069353488,3.18870593386484,70.8531405381624));
#26237=CARTESIAN_POINT('Ctrl Pts',(5.8868380327729,3.34183998814974,70.8613535919076));
#26238=CARTESIAN_POINT('Ctrl Pts',(5.79678102521562,3.49136345081691,70.8695666456529));
#26239=CARTESIAN_POINT('Ctrl Pts',(5.70667072891441,3.64097538985842,70.8777845592455));
#26240=CARTESIAN_POINT('Ctrl Pts',(5.61083954201652,3.7869721792818,70.8860024728382));
#26241=CARTESIAN_POINT('Ctrl Pts',(5.5096260433671,3.92890695515317,70.8942203864308));
#26242=CARTESIAN_POINT('Ctrl Pts',(5.40825468583711,4.071063101347,70.9024511171937));
#26243=CARTESIAN_POINT('Ctrl Pts',(5.30148445975244,4.2091442897715,70.9106818479565));
#26244=CARTESIAN_POINT('Ctrl Pts',(5.18969401191639,4.34273704737913,70.9189125787194));
#26245=CARTESIAN_POINT('Ctrl Pts',(5.08702788545851,4.46542598200542,70.9264715183399));
#26246=CARTESIAN_POINT('Ctrl Pts',(4.98012818282313,4.58432953735254,70.9340304579604));
#26247=CARTESIAN_POINT('Ctrl Pts',(4.86931389109609,4.69915643812574,70.9415893975809));
#26248=CARTESIAN_POINT('Ctrl Pts',(4.74974381084406,4.82305617638663,70.9497455929863));
#26249=CARTESIAN_POINT('Ctrl Pts',(4.62524577628951,4.94259225461675,70.9579017883918));
#26250=CARTESIAN_POINT('Ctrl Pts',(4.49617258679411,5.05734328177959,70.9660579837973));
#26251=CARTESIAN_POINT('Ctrl Pts',(4.36729915372743,5.17191671779847,70.9742015565003));
#26252=CARTESIAN_POINT('Ctrl Pts',(4.23386494243849,5.28171961546955,70.9823451292033));
#26253=CARTESIAN_POINT('Ctrl Pts',(4.09626143376372,5.38636531125211,70.9904887019063));
#26254=CARTESIAN_POINT('Ctrl Pts',(3.9587811050275,5.49091733027817,70.9986249846441));
#26255=CARTESIAN_POINT('Ctrl Pts',(3.81713919384544,5.59032111347143,71.0067612673819));
#26256=CARTESIAN_POINT('Ctrl Pts',(3.67176281342898,5.68422790200394,71.0148975501198));
#26257=CARTESIAN_POINT('Ctrl Pts',(3.52651322166004,5.77805279061105,71.0230267368749));
#26258=CARTESIAN_POINT('Ctrl Pts',(3.37753595374531,5.86639003610613,71.03115592363));
#26259=CARTESIAN_POINT('Ctrl Pts',(3.2252896247094,5.94893232746364,71.0392851103851));
#26260=CARTESIAN_POINT('Ctrl Pts',(3.18349456494932,5.97159205280392,71.0415167559583));
#26261=CARTESIAN_POINT('Ctrl Pts',(3.14145331564828,5.99381530157255,71.0437484015315));
#26262=CARTESIAN_POINT('Ctrl Pts',(3.09917575053257,6.0155962852664,71.0459800471047));
#26263=CARTESIAN_POINT('Ctrl Pts',(3.09917575053258,6.0155962852664,69.0457515827422));
#26264=CARTESIAN_POINT('Ctrl Pts',(2.93382384459269,6.10078395293757,69.0545010306546));
#26265=CARTESIAN_POINT('Ctrl Pts',(2.76495772122994,6.17915010267045,69.063250478567));
#26266=CARTESIAN_POINT('Ctrl Pts',(2.59315093316727,6.25042856433171,69.0719999264794));
#26267=CARTESIAN_POINT('Ctrl Pts',(2.42134553245631,6.32170645041446,69.0807493037394));
#26268=CARTESIAN_POINT('Ctrl Pts',(2.24659977927603,6.38589665313453,69.0894986809994));
#26269=CARTESIAN_POINT('Ctrl Pts',(2.0695071868993,6.44278115439072,69.0982480582594));
#26270=CARTESIAN_POINT('Ctrl Pts',(1.89241596572864,6.49966521519723,69.1069973677741));
#26271=CARTESIAN_POINT('Ctrl Pts',(1.71297821457193,6.54924360009547,69.1157466772887));
#26272=CARTESIAN_POINT('Ctrl Pts',(1.53180337335832,6.59134792173559,69.1244959868034));
#26273=CARTESIAN_POINT('Ctrl Pts',(1.35062987477775,6.63345193135306,69.1332452314795));
#26274=CARTESIAN_POINT('Ctrl Pts',(1.16771959102949,6.66808192368238,69.1419944761556));
#26275=CARTESIAN_POINT('Ctrl Pts',(0.98369374690687,6.69512028363168,69.1507437208317));
#26276=CARTESIAN_POINT('Ctrl Pts',(0.799669205420005,6.72215845218865,69.1594929035759));
#26277=CARTESIAN_POINT('Ctrl Pts',(0.614529402873718,6.74160505424577,69.1682420863201));
#26278=CARTESIAN_POINT('Ctrl Pts',(0.4289031273636,6.7533940435412,69.1769912690643));
#26279=CARTESIAN_POINT('Ctrl Pts',(0.243278104164236,6.76518295330329,69.1857403927829));
#26280=CARTESIAN_POINT('Ctrl Pts',(0.0571669005394799,6.76931433552275,
69.1944895165015));
#26281=CARTESIAN_POINT('Ctrl Pts',(-0.128798404777146,6.76577415902474,
69.2032386402201));
#26282=CARTESIAN_POINT('Ctrl Pts',(-0.314762517258584,6.76223400523443,
69.2119877078193));
#26283=CARTESIAN_POINT('Ctrl Pts',(-0.500580446818851,6.75102239665093,
69.2207367754185));
#26284=CARTESIAN_POINT('Ctrl Pts',(-0.685621118841808,6.73217741012506,
69.2294858430177));
#26285=CARTESIAN_POINT('Ctrl Pts',(-0.870660665413722,6.71333253821782,
69.2382348574035));
#26286=CARTESIAN_POINT('Ctrl Pts',(-1.05492267885413,6.68685441030624,69.2469838717893));
#26287=CARTESIAN_POINT('Ctrl Pts',(-1.23778137635183,6.6528329502819,69.255732886175));
#26288=CARTESIAN_POINT('Ctrl Pts',(-1.42999922978777,6.6170701886188,69.2649296965424));
#26289=CARTESIAN_POINT('Ctrl Pts',(-1.62066601233625,6.5729717293443,69.2741265069098));
#26290=CARTESIAN_POINT('Ctrl Pts',(-1.80906628500315,6.52070304311314,69.2833233172772));
#26291=CARTESIAN_POINT('Ctrl Pts',(-1.98831342545459,6.47097374915052,69.292073315015));
#26292=CARTESIAN_POINT('Ctrl Pts',(-2.16550875896636,6.41384933989551,69.3008233127528));
#26293=CARTESIAN_POINT('Ctrl Pts',(-2.34005036713947,6.34952386240499,69.3095733104905));
#26294=CARTESIAN_POINT('Ctrl Pts',(-2.51458843547026,6.28519968948621,69.3183231307714));
#26295=CARTESIAN_POINT('Ctrl Pts',(-2.68647261717993,6.21367483971126,69.3270729510522));
#26296=CARTESIAN_POINT('Ctrl Pts',(-2.8551190590867,6.13519226743872,69.3358227713331));
#26297=CARTESIAN_POINT('Ctrl Pts',(-3.02376230488813,6.05671118252972,69.3445724257916));
#26298=CARTESIAN_POINT('Ctrl Pts',(-3.18916767379823,5.97127275992676,69.3533220802502));
#26299=CARTESIAN_POINT('Ctrl Pts',(-3.35077334102697,5.87916720438048,69.3620717347087));
#26300=CARTESIAN_POINT('Ctrl Pts',(-3.51237616037272,5.78706327195701,69.3708212349771));
#26301=CARTESIAN_POINT('Ctrl Pts',(-3.67017916302199,5.68829258362363,69.3795707352456));
#26302=CARTESIAN_POINT('Ctrl Pts',(-3.82364636566356,5.58319061741115,69.388320235514));
#26303=CARTESIAN_POINT('Ctrl Pts',(-3.97711106778701,5.47809036367773,69.3970695932224));
#26304=CARTESIAN_POINT('Ctrl Pts',(-4.12623987481839,5.36665920043293,69.4058189509309));
#26305=CARTESIAN_POINT('Ctrl Pts',(-4.27052628213849,5.249275595124,69.4145683086393));
#26306=CARTESIAN_POINT('Ctrl Pts',(-4.41481053024907,5.13189374643098,69.4233175354158));
#26307=CARTESIAN_POINT('Ctrl Pts',(-4.55425230136467,5.0085598147741,69.4320667621924));
#26308=CARTESIAN_POINT('Ctrl Pts',(-4.68837800630493,4.87969268192129,69.4408159889689));
#26309=CARTESIAN_POINT('Ctrl Pts',(-4.82250188228843,4.75082730631862,69.4495650964397));
#26310=CARTESIAN_POINT('Ctrl Pts',(-4.95130963052918,4.61642907903577,69.4583142039106));
#26311=CARTESIAN_POINT('Ctrl Pts',(-5.07436379033323,4.4769544473174,69.4670633113814));
#26312=CARTESIAN_POINT('Ctrl Pts',(-5.19741643562771,4.33748153220628,69.4758123111712));
#26313=CARTESIAN_POINT('Ctrl Pts',(-5.31471544462747,4.19293255254623,69.4845613109609));
#26314=CARTESIAN_POINT('Ctrl Pts',(-5.42586245275609,4.04379841779628,69.4933103107507));
#26315=CARTESIAN_POINT('Ctrl Pts',(-5.53702160019133,3.89464799484371,69.5020602660928));
#26316=CARTESIAN_POINT('Ctrl Pts',(-5.64202723081231,3.74091164443881,69.510810221435));
#26317=CARTESIAN_POINT('Ctrl Pts',(-5.74052265232945,3.58311159163267,69.5195601767771));
#26318=CARTESIAN_POINT('Ctrl Pts',(-5.83901427066901,3.42531763191813,69.5283097942596));
#26319=CARTESIAN_POINT('Ctrl Pts',(-5.93099603115726,3.26346052695637,69.537059411742));
#26320=CARTESIAN_POINT('Ctrl Pts',(-6.01615550622744,3.09809004467095,69.5458090292245));
#26321=CARTESIAN_POINT('Ctrl Pts',(-6.10131214578792,2.93272506863843,69.5545583553756));
#26322=CARTESIAN_POINT('Ctrl Pts',(-6.17964682328743,2.76384720416905,69.5633076815267));
#26323=CARTESIAN_POINT('Ctrl Pts',(-6.25089348288561,2.59203002791599,69.5720570076778));
#26324=CARTESIAN_POINT('Ctrl Pts',(-6.32213814889331,2.42021765937028,69.5808060890094));
#26325=CARTESIAN_POINT('Ctrl Pts',(-6.38629508412588,2.2454664083191,69.5895551703409));
#26326=CARTESIAN_POINT('Ctrl Pts',(-6.44314639819816,2.06836976660027,69.5983042516725));
#26327=CARTESIAN_POINT('Ctrl Pts',(-6.50000285283706,1.89125711158257,69.6070541241069));
#26328=CARTESIAN_POINT('Ctrl Pts',(-6.54955227673255,1.71179891440232,69.6158039965413));
#26329=CARTESIAN_POINT('Ctrl Pts',(-6.59162635926391,1.53060476278405,69.6245538689757));
#26330=CARTESIAN_POINT('Ctrl Pts',(-6.633697520552,1.34942319164679,69.6333031338982));
#26331=CARTESIAN_POINT('Ctrl Pts',(-6.66829431424255,1.16650618642697,69.6420523988207));
#26332=CARTESIAN_POINT('Ctrl Pts',(-6.69529923745417,0.98247499761859,69.6508016637432));
#26333=CARTESIAN_POINT('Ctrl Pts',(-6.72230554731443,0.798434359177787,
69.6595513779229));
#26334=CARTESIAN_POINT('Ctrl Pts',(-6.74171916496702,0.613279706240395,
69.6683010921026));
#26335=CARTESIAN_POINT('Ctrl Pts',(-6.75347414817274,0.427639953655449,
69.6770508062823));
#26336=CARTESIAN_POINT('Ctrl Pts',(-6.7624883775874,0.285283364199281,69.6837604654581));
#26337=CARTESIAN_POINT('Ctrl Pts',(-6.76699999999993,0.142641701106463,
69.690470124634));
#26338=CARTESIAN_POINT('Ctrl Pts',(-6.767,3.55173088245946E-12,69.6971797838099));
#26339=CARTESIAN_POINT('',(-6.767,3.37743206882749E-12,69.3028202161898));
#26340=CARTESIAN_POINT('Ctrl Pts',(3.09917575053259,6.01559628526639,68.6513920151221));
#26341=CARTESIAN_POINT('Ctrl Pts',(2.93382384459265,6.1007839529376,68.6601414630345));
#26342=CARTESIAN_POINT('Ctrl Pts',(2.76495772122983,6.1791501026705,68.6688909109469));
#26343=CARTESIAN_POINT('Ctrl Pts',(2.5931509331671,6.25042856433178,68.6776403588593));
#26344=CARTESIAN_POINT('Ctrl Pts',(2.42134553245614,6.32170645041452,68.6863897361193));
#26345=CARTESIAN_POINT('Ctrl Pts',(2.24659977927586,6.38589665313459,68.6951391133793));
#26346=CARTESIAN_POINT('Ctrl Pts',(2.06950718689913,6.44278115439077,68.7038884906393));
#26347=CARTESIAN_POINT('Ctrl Pts',(1.89241596572853,6.49966521519726,68.712637800154));
#26348=CARTESIAN_POINT('Ctrl Pts',(1.71297821457188,6.54924360009549,68.7213871096686));
#26349=CARTESIAN_POINT('Ctrl Pts',(1.53180337335833,6.59134792173559,68.7301364191833));
#26350=CARTESIAN_POINT('Ctrl Pts',(1.3506298747777,6.63345193135307,68.7388856638594));
#26351=CARTESIAN_POINT('Ctrl Pts',(1.16771959102938,6.6680819236824,68.7476349085355));
#26352=CARTESIAN_POINT('Ctrl Pts',(0.983693746906693,6.69512028363171,68.7563841532117));
#26353=CARTESIAN_POINT('Ctrl Pts',(0.7996692054197,6.72215845218869,68.7651333359558));
#26354=CARTESIAN_POINT('Ctrl Pts',(0.614529402873285,6.74160505424581,68.7738825187));
#26355=CARTESIAN_POINT('Ctrl Pts',(0.428903127363038,6.75339404354123,68.7826317014442));
#26356=CARTESIAN_POINT('Ctrl Pts',(0.243278104163609,6.76518295330331,68.7913808251628));
#26357=CARTESIAN_POINT('Ctrl Pts',(0.0571669005387894,6.76931433552276,
68.8001299488814));
#26358=CARTESIAN_POINT('Ctrl Pts',(-0.1287984047779,6.76577415902472,68.8088790726));
#26359=CARTESIAN_POINT('Ctrl Pts',(-0.31476251725921,6.7622340052344,68.8176281401992));
#26360=CARTESIAN_POINT('Ctrl Pts',(-0.500580446819348,6.75102239665089,
68.8263772077984));
#26361=CARTESIAN_POINT('Ctrl Pts',(-0.685621118842176,6.73217741012502,
68.8351262753976));
#26362=CARTESIAN_POINT('Ctrl Pts',(-0.870660665414088,6.71333253821777,
68.8438752897834));
#26363=CARTESIAN_POINT('Ctrl Pts',(-1.0549226788545,6.68685441030618,68.8526243041692));
#26364=CARTESIAN_POINT('Ctrl Pts',(-1.23778137635219,6.65283295028183,68.861373318555));
#26365=CARTESIAN_POINT('Ctrl Pts',(-1.42999922978813,6.61707018861873,68.8705701289224));
#26366=CARTESIAN_POINT('Ctrl Pts',(-1.62066601233661,6.57297172934421,68.8797669392897));
#26367=CARTESIAN_POINT('Ctrl Pts',(-1.8090662850035,6.52070304311304,68.8889637496571));
#26368=CARTESIAN_POINT('Ctrl Pts',(-1.98831342545488,6.47097374915043,68.8977137473949));
#26369=CARTESIAN_POINT('Ctrl Pts',(-2.16550875896658,6.41384933989543,68.9064637451326));
#26370=CARTESIAN_POINT('Ctrl Pts',(-2.34005036713964,6.34952386240493,68.9152137428704));
#26371=CARTESIAN_POINT('Ctrl Pts',(-2.51458843547036,6.28519968948617,68.9239635631513));
#26372=CARTESIAN_POINT('Ctrl Pts',(-2.68647261717998,6.21367483971124,68.9327133834321));
#26373=CARTESIAN_POINT('Ctrl Pts',(-2.85511905908669,6.13519226743873,68.941463203713));
#26374=CARTESIAN_POINT('Ctrl Pts',(-3.02376230488824,6.05671118252967,68.9502128581715));
#26375=CARTESIAN_POINT('Ctrl Pts',(-3.18916767379845,5.97127275992665,68.9589625126301));
#26376=CARTESIAN_POINT('Ctrl Pts',(-3.3507733410273,5.87916720438029,68.9677121670886));
#26377=CARTESIAN_POINT('Ctrl Pts',(-3.51237616037321,5.78706327195672,68.9764616673571));
#26378=CARTESIAN_POINT('Ctrl Pts',(-3.67017916302262,5.68829258362323,68.9852111676255));
#26379=CARTESIAN_POINT('Ctrl Pts',(-3.82364636566434,5.58319061741061,68.9939606678939));
#26380=CARTESIAN_POINT('Ctrl Pts',(-3.97711106778762,5.47809036367728,69.0027100256024));
#26381=CARTESIAN_POINT('Ctrl Pts',(-4.12623987481883,5.36665920043258,69.0114593833108));
#26382=CARTESIAN_POINT('Ctrl Pts',(-4.27052628213878,5.24927559512376,69.0202087410192));
#26383=CARTESIAN_POINT('Ctrl Pts',(-4.41481053024945,5.13189374643065,69.0289579677958));
#26384=CARTESIAN_POINT('Ctrl Pts',(-4.55425230136514,5.00855981477369,69.0377071945723));
#26385=CARTESIAN_POINT('Ctrl Pts',(-4.68837800630548,4.87969268192077,69.0464564213488));
#26386=CARTESIAN_POINT('Ctrl Pts',(-4.82250188228901,4.75082730631804,69.0552055288197));
#26387=CARTESIAN_POINT('Ctrl Pts',(-4.95130963052979,4.61642907903513,69.0639546362905));
#26388=CARTESIAN_POINT('Ctrl Pts',(-5.07436379033386,4.47695444731669,69.0727037437614));
#26389=CARTESIAN_POINT('Ctrl Pts',(-5.19741643562836,4.33748153220551,69.0814527435511));
#26390=CARTESIAN_POINT('Ctrl Pts',(-5.31471544462814,4.19293255254539,69.0902017433409));
#26391=CARTESIAN_POINT('Ctrl Pts',(-5.42586245275677,4.04379841779537,69.0989507431306));
#26392=CARTESIAN_POINT('Ctrl Pts',(-5.53702160019199,3.89464799484278,69.1077006984728));
#26393=CARTESIAN_POINT('Ctrl Pts',(-5.64202723081294,3.74091164443786,69.1164506538149));
#26394=CARTESIAN_POINT('Ctrl Pts',(-5.74052265233006,3.58311159163171,69.1252006091571));
#26395=CARTESIAN_POINT('Ctrl Pts',(-5.83901427066959,3.42531763191715,69.1339502266395));
#26396=CARTESIAN_POINT('Ctrl Pts',(-5.93099603115781,3.26346052695537,69.142699844122));
#26397=CARTESIAN_POINT('Ctrl Pts',(-6.01615550622796,3.09809004466994,69.1514494616044));
#26398=CARTESIAN_POINT('Ctrl Pts',(-6.10131214578848,2.93272506863729,69.1601987877555));
#26399=CARTESIAN_POINT('Ctrl Pts',(-6.179646823288,2.76384720416778,69.1689481139067));
#26400=CARTESIAN_POINT('Ctrl Pts',(-6.2508934828862,2.59203002791459,69.1776974400578));
#26401=CARTESIAN_POINT('Ctrl Pts',(-6.32213814889385,2.42021765936886,69.1864465213893));
#26402=CARTESIAN_POINT('Ctrl Pts',(-6.38629508412638,2.24546640831767,69.1951956027209));
#26403=CARTESIAN_POINT('Ctrl Pts',(-6.44314639819863,2.06836976659882,69.2039446840525));
#26404=CARTESIAN_POINT('Ctrl Pts',(-6.50000285283748,1.89125711158111,69.2126945564869));
#26405=CARTESIAN_POINT('Ctrl Pts',(-6.54955227673294,1.71179891440085,69.2214444289213));
#26406=CARTESIAN_POINT('Ctrl Pts',(-6.59162635926426,1.53060476278256,69.2301943013557));
#26407=CARTESIAN_POINT('Ctrl Pts',(-6.63369752055237,1.34942319164499,69.2389435662782));
#26408=CARTESIAN_POINT('Ctrl Pts',(-6.66829431424293,1.16650618642484,69.2476928312007));
#26409=CARTESIAN_POINT('Ctrl Pts',(-6.69529923745453,0.982474997616134,
69.2564420961232));
#26410=CARTESIAN_POINT('Ctrl Pts',(-6.72230554731471,0.798434359175384,
69.2651918103029));
#26411=CARTESIAN_POINT('Ctrl Pts',(-6.74171916496724,0.61327970623805,69.2739415244826));
#26412=CARTESIAN_POINT('Ctrl Pts',(-6.75347414817289,0.427639953653164,
69.2826912386623));
#26413=CARTESIAN_POINT('Ctrl Pts',(-6.76248837758745,0.285283364197696,
69.2894008978381));
#26414=CARTESIAN_POINT('Ctrl Pts',(-6.76699999999993,0.142641701105583,
69.296110557014));
#26415=CARTESIAN_POINT('Ctrl Pts',(-6.767,3.37743208484225E-12,69.3028202161898));
#26416=CARTESIAN_POINT('Ctrl Pts',(-6.76699999999291,9.79885374254829E-6,
69.3030322358393));
#26417=CARTESIAN_POINT('Ctrl Pts',(-6.76700024703085,-0.170592373230755,
69.3111047379646));
#26418=CARTESIAN_POINT('Ctrl Pts',(-6.76054465261952,-0.34148283825778,
69.3191772400899));
#26419=CARTESIAN_POINT('Ctrl Pts',(-6.74759363237739,-0.512122223985705,
69.3272497422151));
#26420=CARTESIAN_POINT('Ctrl Pts',(-6.73465748998322,-0.682565582930617,
69.3353129708271));
#26421=CARTESIAN_POINT('Ctrl Pts',(-6.71524079823711,-0.852758068662661,
69.343376199439));
#26422=CARTESIAN_POINT('Ctrl Pts',(-6.68935590325772,-1.02215781538423,
69.3514394280509));
#26423=CARTESIAN_POINT('Ctrl Pts',(-6.66349507694572,-1.19140004838353,
69.359495159195));
#26424=CARTESIAN_POINT('Ctrl Pts',(-6.63117807340899,-1.35985064332614,
69.3675508903391));
#26425=CARTESIAN_POINT('Ctrl Pts',(-6.59246920217326,-1.5269704707024,69.3756066214832));
#26426=CARTESIAN_POINT('Ctrl Pts',(-6.55378785924245,-1.69397144869297,
69.3836566236918));
#26427=CARTESIAN_POINT('Ctrl Pts',(-6.50872378100871,-1.85964318114955,
69.3917066259005));
#26428=CARTESIAN_POINT('Ctrl Pts',(-6.45739273669824,-2.02345448281813,
69.3997566281092));
#26429=CARTESIAN_POINT('Ctrl Pts',(-6.40448593360075,-2.19229445868348,
69.408053749033));
#26430=CARTESIAN_POINT('Ctrl Pts',(-6.34492130354424,-2.35915755413341,
69.4163508699567));
#26431=CARTESIAN_POINT('Ctrl Pts',(-6.27888194073216,-2.52347589137435,
69.4246479908805));
#26432=CARTESIAN_POINT('Ctrl Pts',(-6.21484943481896,-2.68280079175183,
69.4326929722673));
#26433=CARTESIAN_POINT('Ctrl Pts',(-6.14473012506522,-2.83973297375626,
69.440737953654));
#26434=CARTESIAN_POINT('Ctrl Pts',(-6.06874066805516,-2.99377282102256,
69.4487829350408));
#26435=CARTESIAN_POINT('Ctrl Pts',(-5.99275166831572,-3.14781174134588,
69.4568278680164));
#26436=CARTESIAN_POINT('Ctrl Pts',(-5.91089275629488,-3.29895802662626,
69.464872800992));
#26437=CARTESIAN_POINT('Ctrl Pts',(-5.82342738705123,-3.44673504460986,
69.4729177339677));
#26438=CARTESIAN_POINT('Ctrl Pts',(-5.73594524274834,-3.59454040487626,
69.480964209888));
#26439=CARTESIAN_POINT('Ctrl Pts',(-5.64285469123482,-3.73897489061653,
69.4890106858083));
#26440=CARTESIAN_POINT('Ctrl Pts',(-5.54446342091688,-3.87958945948083,
69.4970571617286));
#26441=CARTESIAN_POINT('Ctrl Pts',(-5.44603381235406,-4.02025881893535,
69.5051067729654));
#26442=CARTESIAN_POINT('Ctrl Pts',(-5.34229958796078,-4.15710499374216,
69.5131563842021));
#26443=CARTESIAN_POINT('Ctrl Pts',(-5.23360964023565,-4.28971084499089,
69.5212059954388));
#26444=CARTESIAN_POINT('Ctrl Pts',(-5.12480134792087,-4.42246108111955,
69.5292643713126));
#26445=CARTESIAN_POINT('Ctrl Pts',(-5.01102679745427,-4.55096148893403,
69.5373227471863));
#26446=CARTESIAN_POINT('Ctrl Pts',(-4.89267321585187,-4.67483024321587,
69.5453811230601));
#26447=CARTESIAN_POINT('Ctrl Pts',(-4.77424238184176,-4.79877984979959,
69.5534447588417));
#26448=CARTESIAN_POINT('Ctrl Pts',(-4.65122683144362,-4.91809152404778,
69.5615083946234));
#26449=CARTESIAN_POINT('Ctrl Pts',(-4.52404758038812,-5.03242312314698,
69.569572030405));
#26450=CARTESIAN_POINT('Ctrl Pts',(-4.39670069411057,-5.14690542295281,
69.5776462948809));
#26451=CARTESIAN_POINT('Ctrl Pts',(-4.26517943979858,-5.25639431088611,
69.5857205593568));
#26452=CARTESIAN_POINT('Ctrl Pts',(-4.12993502195336,-5.3605900528247,69.5937948238327));
#26453=CARTESIAN_POINT('Ctrl Pts',(-4.10150064171555,-5.38249662311164,
69.5954923926485));
#26454=CARTESIAN_POINT('Ctrl Pts',(-4.0729017780956,-5.40416938177994,69.5971899614643));
#26455=CARTESIAN_POINT('Ctrl Pts',(-4.04414276360816,-5.42560580097336,
69.5988875302802));
#26456=CARTESIAN_POINT('Ctrl Pts',(-3.9047801226389,-5.52948404732367,69.6071137396137));
#26457=CARTESIAN_POINT('Ctrl Pts',(-3.76121775700442,-5.62813453010611,
69.6153399489473));
#26458=CARTESIAN_POINT('Ctrl Pts',(-3.61388435296551,-5.72119995135558,
69.6235661582808));
#26459=CARTESIAN_POINT('Ctrl Pts',(-3.4667164716947,-5.81416081759093,69.6317831258206));
#26460=CARTESIAN_POINT('Ctrl Pts',(-3.31578628869878,-5.90154892689321,
69.6400000933603));
#26461=CARTESIAN_POINT('Ctrl Pts',(-3.16155469770833,-5.98304779300637,
69.6482170609001));
#26462=CARTESIAN_POINT('Ctrl Pts',(-3.00746542378782,-6.06447145610986,
69.65642644624));
#26463=CARTESIAN_POINT('Ctrl Pts',(-2.85008112393073,-6.14001653212085,
69.6646358315799));
#26464=CARTESIAN_POINT('Ctrl Pts',(-2.68989082509428,-6.2094103060656,69.6728452169198));
#26465=CARTESIAN_POINT('Ctrl Pts',(-2.52981620056308,-6.27875397038043,
69.6810486742169));
#26466=CARTESIAN_POINT('Ctrl Pts',(-2.36693994070157,-6.34195503812928,
69.689252131514));
#26467=CARTESIAN_POINT('Ctrl Pts',(-2.20177485896343,-6.39878710932287,
69.6974555888112));
#26468=CARTESIAN_POINT('Ctrl Pts',(-2.03669591213926,-6.45558954213581,
69.7056547679396));
#26469=CARTESIAN_POINT('Ctrl Pts',(-1.86933085969487,-6.50602947896676,
69.7138539470679));
#26470=CARTESIAN_POINT('Ctrl Pts',(-1.70021172503698,-6.54992893778603,
69.7220531261963));
#26471=CARTESIAN_POINT('Ctrl Pts',(-1.53112445606874,-6.59382012500118,
69.7302507604227));
#26472=CARTESIAN_POINT('Ctrl Pts',(-1.36028410843392,-6.6311731929181,69.738448394649));
#26473=CARTESIAN_POINT('Ctrl Pts',(-1.18823737214972,-6.66186017171081,
69.7466460288754));
#26474=CARTESIAN_POINT('Ctrl Pts',(-1.01620305438703,-6.69254493548384,
69.7548430713875));
#26475=CARTESIAN_POINT('Ctrl Pts',(-0.842962874346927,-6.71656450454903,
69.7630401138996));
#26476=CARTESIAN_POINT('Ctrl Pts',(-0.669073155748615,-6.73384215082716,
69.7712371564118));
#26477=CARTESIAN_POINT('Ctrl Pts',(-0.495164384536056,-6.75112169016909,
69.7794350970511));
#26478=CARTESIAN_POINT('Ctrl Pts',(-0.320606289974542,-6.76165779956088,
69.7876330376905));
#26479=CARTESIAN_POINT('Ctrl Pts',(-0.145959805460637,-6.76542568765557,
69.7958309783299));
#26480=CARTESIAN_POINT('Ctrl Pts',(0.0287375564089473,-6.76919467339723,
69.8040313071624));
#26481=CARTESIAN_POINT('Ctrl Pts',(0.203523001014131,-6.76619150273411,
69.8122316359949));
#26482=CARTESIAN_POINT('Ctrl Pts',(0.377836053506462,-6.75644351095091,
69.8204319648274));
#26483=CARTESIAN_POINT('Ctrl Pts',(0.552330744723304,-6.7466853615073,69.8286408386154));
#26484=CARTESIAN_POINT('Ctrl Pts',(0.726351701803452,-6.73016836955846,
69.8368497124034));
#26485=CARTESIAN_POINT('Ctrl Pts',(0.89934302486302,-6.70697182964341,69.8450585861914));
#26486=CARTESIAN_POINT('Ctrl Pts',(1.07242719045789,-6.6837628404012,69.8532718655915));
#26487=CARTESIAN_POINT('Ctrl Pts',(1.24448026737596,-6.65386721803353,69.8614851449915));
#26488=CARTESIAN_POINT('Ctrl Pts',(1.41495709764256,-6.61741531202561,69.8696984243915));
#26489=CARTESIAN_POINT('Ctrl Pts',(1.58568327706861,-6.58091008937572,69.8779237170036));
#26490=CARTESIAN_POINT('Ctrl Pts',(1.75482825487382,-6.53782950742589,69.8861490096157));
#26491=CARTESIAN_POINT('Ctrl Pts',(1.92186133355828,-6.48835402968839,69.8943743022278));
#26492=CARTESIAN_POINT('Ctrl Pts',(2.07292268937523,-6.44360940302174,69.9018130913812));
#26493=CARTESIAN_POINT('Ctrl Pts',(2.22225675967473,-6.3936350772232,69.9092518805345));
#26494=CARTESIAN_POINT('Ctrl Pts',(2.36948624373537,-6.33859794755503,69.9166906696879));
#26495=CARTESIAN_POINT('Ctrl Pts',(2.53230028618154,-6.27773501902492,69.9249168707148));
#26496=CARTESIAN_POINT('Ctrl Pts',(2.69299538908088,-6.21050989780627,69.9331430717417));
#26497=CARTESIAN_POINT('Ctrl Pts',(2.85103898890883,-6.137089349498,69.9413692727686));
#26498=CARTESIAN_POINT('Ctrl Pts',(3.00890506006193,-6.0637512737015,69.9495862333924));
#26499=CARTESIAN_POINT('Ctrl Pts',(3.16412523665829,-5.98423177831405,69.9578031940162));
#26500=CARTESIAN_POINT('Ctrl Pts',(3.3161838111228,-5.89874681020021,69.9660201546399));
#26501=CARTESIAN_POINT('Ctrl Pts',(3.46810209919027,-5.81334070891922,69.9742295344495));
#26502=CARTESIAN_POINT('Ctrl Pts',(3.61686428345511,-5.72198027025017,69.9824389142591));
#26503=CARTESIAN_POINT('Ctrl Pts',(3.76197620713176,-5.62492880105824,69.9906482940687));
#26504=CARTESIAN_POINT('Ctrl Pts',(3.90698336903285,-5.52794739698555,69.9988517472172));
#26505=CARTESIAN_POINT('Ctrl Pts',(4.04834522243183,-5.42528334452511,70.0070552003656));
#26506=CARTESIAN_POINT('Ctrl Pts',(4.18559365423153,-5.31724503494589,70.015258653514));
#26507=CARTESIAN_POINT('Ctrl Pts',(4.32277053290059,-5.20926305008512,70.0234578298722));
#26508=CARTESIAN_POINT('Ctrl Pts',(4.45583798104866,-5.0959126111233,70.0316570062303));
#26509=CARTESIAN_POINT('Ctrl Pts',(4.58435817621401,-4.97754448620801,70.0398561825885));
#26510=CARTESIAN_POINT('Ctrl Pts',(4.71285418836387,-4.85919863404289,70.0480538161478));
#26511=CARTESIAN_POINT('Ctrl Pts',(4.83680438412177,-4.73583721471198,70.0562514497071));
#26512=CARTESIAN_POINT('Ctrl Pts',(4.95580503290423,-4.60785041812786,70.0644490832665));
#26513=CARTESIAN_POINT('Ctrl Pts',(5.07479711071924,-4.47987283973439,70.072646126395));
#26514=CARTESIAN_POINT('Ctrl Pts',(5.18884010664361,-4.34727080963164,70.0808431695235));
#26515=CARTESIAN_POINT('Ctrl Pts',(5.29756814212362,-4.21047037509551,70.089040212652));
#26516=CARTESIAN_POINT('Ctrl Pts',(5.40630810765516,-4.07365493029798,70.0972381551911));
#26517=CARTESIAN_POINT('Ctrl Pts',(5.50973172766425,-3.93264044414168,70.1054360977301));
#26518=CARTESIAN_POINT('Ctrl Pts',(5.60751428151198,-3.78788497484271,70.1136340402692));
#26519=CARTESIAN_POINT('Ctrl Pts',(5.70532533631333,-3.64308731326349,70.1218343722855));
#26520=CARTESIAN_POINT('Ctrl Pts',(5.79749184914728,-3.49454679375442,70.1300347043018));
#26521=CARTESIAN_POINT('Ctrl Pts',(5.88373316257174,-3.3427493282706,70.138235036318));
#26522=CARTESIAN_POINT('Ctrl Pts',(5.9700643627525,-3.19079364880273,70.1464439152965));
#26523=CARTESIAN_POINT('Ctrl Pts',(6.05045784807698,-3.0355745537015,70.1546527942749));
#26524=CARTESIAN_POINT('Ctrl Pts',(6.12467911357747,-2.87760225808013,70.1628616732534));
#26525=CARTESIAN_POINT('Ctrl Pts',(6.19894022277438,-2.71954515926731,70.1710749589484));
#26526=CARTESIAN_POINT('Ctrl Pts',(6.26702236708854,-2.55873224350469,70.1792882446435));
#26527=CARTESIAN_POINT('Ctrl Pts',(6.3287397748899,-2.39569235540095,70.1875015303385));
#26528=CARTESIAN_POINT('Ctrl Pts',(6.39054746765106,-2.2324139600386,70.1957268310581));
#26529=CARTESIAN_POINT('Ctrl Pts',(6.44597170293687,-2.06690242195696,70.2039521317777));
#26530=CARTESIAN_POINT('Ctrl Pts',(6.49487666602076,-1.89970158003278,70.2121774324973));
#26531=CARTESIAN_POINT('Ctrl Pts',(6.53910530522891,-1.74848858964412,70.2196162246968));
#26532=CARTESIAN_POINT('Ctrl Pts',(6.57800243450117,-1.59589426002877,70.2270550168962));
#26533=CARTESIAN_POINT('Ctrl Pts',(6.61150393632732,-1.44232614201103,70.2344938090957));
#26534=CARTESIAN_POINT('Ctrl Pts',(6.64821996084301,-1.27402291742043,70.2426463653059));
#26535=CARTESIAN_POINT('Ctrl Pts',(6.67856269821642,-1.10405355869292,70.2507989215161));
#26536=CARTESIAN_POINT('Ctrl Pts',(6.70238019229282,-0.932946278175195,
70.2589514777263));
#26537=CARTESIAN_POINT('Ctrl Pts',(6.72617009322831,-0.762037229565748,
70.2670945890036));
#26538=CARTESIAN_POINT('Ctrl Pts',(6.74344974919201,-0.589993241758193,
70.275237700281));
#26539=CARTESIAN_POINT('Ctrl Pts',(6.7541175053542,-0.417355632366388,70.2833808115583));
#26540=CARTESIAN_POINT('Ctrl Pts',(6.76477514542661,-0.24488173289927,70.2915162008326));
#26541=CARTESIAN_POINT('Ctrl Pts',(6.76883334602624,-0.0718156949128621,
70.299651590107));
#26542=CARTESIAN_POINT('Ctrl Pts',(6.76624184566292,0.101293069852138,70.3077869793814));
#26543=CARTESIAN_POINT('Ctrl Pts',(6.76365225824779,0.274274052231617,70.315916363417));
#26544=CARTESIAN_POINT('Ctrl Pts',(6.75442274912214,0.447297334609687,70.3240457474528));
#26545=CARTESIAN_POINT('Ctrl Pts',(6.7385550331034,0.619810508007817,70.3321751314884));
#26546=CARTESIAN_POINT('Ctrl Pts',(6.72269569705731,0.792232574678687,70.3403002222776));
#26547=CARTESIAN_POINT('Ctrl Pts',(6.70020516934282,0.964144705670353,70.3484253130669));
#26548=CARTESIAN_POINT('Ctrl Pts',(6.6711372089452,1.13499662529313,70.3565504038561));
#26549=CARTESIAN_POINT('Ctrl Pts',(6.64195828982401,1.30650072383258,70.364706509883));
#26550=CARTESIAN_POINT('Ctrl Pts',(6.60615163732752,1.47693612887344,70.37286261591));
#26551=CARTESIAN_POINT('Ctrl Pts',(6.56382402666672,1.64575306378349,70.3810187219369));
#26552=CARTESIAN_POINT('Ctrl Pts',(6.52166677700755,1.81389054096667,70.3891420011076));
#26553=CARTESIAN_POINT('Ctrl Pts',(6.47304107356705,1.98042219989944,70.3972652802783));
#26554=CARTESIAN_POINT('Ctrl Pts',(6.41810321571569,2.14481703471879,70.405388559449));
#26555=CARTESIAN_POINT('Ctrl Pts',(6.36315804242397,2.30923376010065,70.413512920303));
#26556=CARTESIAN_POINT('Ctrl Pts',(6.30189915652911,2.47151274762659,70.421637281157));
#26557=CARTESIAN_POINT('Ctrl Pts',(6.23453208593151,2.63114018430994,70.429761642011));
#26558=CARTESIAN_POINT('Ctrl Pts',(6.16714322790689,2.79081924667771,70.4378886303938));
#26559=CARTESIAN_POINT('Ctrl Pts',(6.09364239355962,2.94784471368909,70.4460156187766));
#26560=CARTESIAN_POINT('Ctrl Pts',(6.01428238284227,3.10172474914089,70.4541426071594));
#26561=CARTESIAN_POINT('Ctrl Pts',(5.93440931861393,3.25659960165164,70.4623221356048));
#26562=CARTESIAN_POINT('Ctrl Pts',(5.84860122980117,3.40828787786311,70.4705016640501));
#26563=CARTESIAN_POINT('Ctrl Pts',(5.75716122730205,3.55631601560519,70.4786811924954));
#26564=CARTESIAN_POINT('Ctrl Pts',(5.66615184533946,3.70364704098556,70.4868222008966));
#26565=CARTESIAN_POINT('Ctrl Pts',(5.56956373772252,3.84735205990366,70.4949632092979));
#26566=CARTESIAN_POINT('Ctrl Pts',(5.46773726086385,3.98699614323379,70.5031042176991));
#26567=CARTESIAN_POINT('Ctrl Pts',(5.36518807985398,4.12763133773487,70.5113030061665));
#26568=CARTESIAN_POINT('Ctrl Pts',(5.25732613262743,4.26414744429977,70.5195017946338));
#26569=CARTESIAN_POINT('Ctrl Pts',(5.14453768453907,4.39613705568394,70.5277005831012));
#26570=CARTESIAN_POINT('Ctrl Pts',(5.03174923645066,4.52812666706816,70.5358993715686));
#26571=CARTESIAN_POINT('Ctrl Pts',(4.91403458704895,4.6555895544032,70.5440981600359));
#26572=CARTESIAN_POINT('Ctrl Pts',(4.79181446060722,4.77815897340342,70.5522969485033));
#26573=CARTESIAN_POINT('Ctrl Pts',(4.66852063006232,4.90180516504276,70.560567763347));
#26574=CARTESIAN_POINT('Ctrl Pts',(4.54025684618928,5.02085771462031,70.5688385781906));
#26575=CARTESIAN_POINT('Ctrl Pts',(4.40739849221652,5.13489313723349,70.5771093930343));
#26576=CARTESIAN_POINT('Ctrl Pts',(4.27530604256738,5.24827116630976,70.5853325281299));
#26577=CARTESIAN_POINT('Ctrl Pts',(4.13867210375974,5.35668949579421,70.5935556632255));
#26578=CARTESIAN_POINT('Ctrl Pts',(3.99790500771599,5.45976597935108,70.601778798321));
#26579=CARTESIAN_POINT('Ctrl Pts',(3.85591360860525,5.5637389568934,70.6100734530388));
#26580=CARTESIAN_POINT('Ctrl Pts',(3.70971705065656,5.66227644336873,70.6183681077565));
#26581=CARTESIAN_POINT('Ctrl Pts',(3.55977124940387,5.75502542582721,70.6266627624742));
#26582=CARTESIAN_POINT('Ctrl Pts',(3.40982544815124,5.84777440828565,70.6349574171919));
#26583=CARTESIAN_POINT('Ctrl Pts',(3.25613069578252,5.93473464875063,70.6432520719096));
#26584=CARTESIAN_POINT('Ctrl Pts',(3.09917575053263,6.01559628526637,70.6515467266273));
#26585=CARTESIAN_POINT('Origin',(0.,0.,-3.69717978381041));
#26586=CARTESIAN_POINT('',(3.09917575053265,6.01559628526636,73.0456387728543));
#26587=CARTESIAN_POINT('',(3.09917575053262,6.01559628526637,72.6513920151221));
#26588=CARTESIAN_POINT('',(3.09917575053259,6.01559628526639,-3.69717978381041));
#26589=CARTESIAN_POINT('',(-6.76699866280443,0.00425412777605735,71.6971797837803));
#26590=CARTESIAN_POINT('Ctrl Pts',(-6.76699866280482,0.00425412714360294,
71.6971797838099));
#26591=CARTESIAN_POINT('Ctrl Pts',(-6.76710997009626,-0.172801298538676,
71.7054757833312));
#26592=CARTESIAN_POINT('Ctrl Pts',(-6.760268040189,-0.349875666979543,71.7137717828525));
#26593=CARTESIAN_POINT('Ctrl Pts',(-6.7464953643748,-0.526392722659913,
71.7220677823738));
#26594=CARTESIAN_POINT('Ctrl Pts',(-6.73275154850618,-0.702539895777978,
71.7303463980477));
#26595=CARTESIAN_POINT('Ctrl Pts',(-6.71210605334925,-0.878131742588406,
71.7386250137217));
#26596=CARTESIAN_POINT('Ctrl Pts',(-6.684633245895,-1.05260028874936,71.7469036293956));
#26597=CARTESIAN_POINT('Ctrl Pts',(-6.65715276890628,-1.22711754098203,
71.7551845561958));
#26598=CARTESIAN_POINT('Ctrl Pts',(-6.62284123491531,-1.4005105231155,71.763465482996));
#26599=CARTESIAN_POINT('Ctrl Pts',(-6.58182431353282,-1.57222062885213,
71.7717464097962));
#26600=CARTESIAN_POINT('Ctrl Pts',(-6.54078908784747,-1.74400736232374,
71.7800310320613));
#26601=CARTESIAN_POINT('Ctrl Pts',(-6.49304259177669,-1.91410938374628,
71.7883156543264));
#26602=CARTESIAN_POINT('Ctrl Pts',(-6.43876066150863,-2.08198226308701,
71.7966002765915));
#26603=CARTESIAN_POINT('Ctrl Pts',(-6.38433238472729,-2.25030773522326,
71.804907234569));
#26604=CARTESIAN_POINT('Ctrl Pts',(-6.32333350806107,-2.41639169931005,
71.8132141925465));
#26605=CARTESIAN_POINT('Ctrl Pts',(-6.25598989030927,-2.5797053111447,71.821521150524));
#26606=CARTESIAN_POINT('Ctrl Pts',(-6.18869916031527,-2.74289066597393,
71.8298215847002));
#26607=CARTESIAN_POINT('Ctrl Pts',(-6.1150738337816,-2.90330971843124,71.8381220188764));
#26608=CARTESIAN_POINT('Ctrl Pts',(-6.03538536448875,-3.06045952466537,
71.8464224530525));
#26609=CARTESIAN_POINT('Ctrl Pts',(-5.95556533654408,-3.21786877140359,
71.8547365905153));
#26610=CARTESIAN_POINT('Ctrl Pts',(-5.86966232667769,-3.37199767841978,
71.863050727978));
#26611=CARTESIAN_POINT('Ctrl Pts',(-5.77799260821506,-3.52237000035659,
71.8713648654408));
#26612=CARTESIAN_POINT('Ctrl Pts',(-5.68640927847976,-3.67260061275471,
71.8796711677343));
#26613=CARTESIAN_POINT('Ctrl Pts',(-5.5890703469852,-3.81908146603657,71.8879774700278));
#26614=CARTESIAN_POINT('Ctrl Pts',(-5.48633121941073,-3.96137081714388,
71.8962837723214));
#26615=CARTESIAN_POINT('Ctrl Pts',(-5.38551320208138,-4.1009995117259,71.9044347557718));
#26616=CARTESIAN_POINT('Ctrl Pts',(-5.27920294434396,-4.23699626317783,
71.9125857392222));
#26617=CARTESIAN_POINT('Ctrl Pts',(-5.1676920987235,-4.36889544081691,71.9207367226727));
#26618=CARTESIAN_POINT('Ctrl Pts',(-5.0563107831579,-4.50064140548713,71.9288782380097));
#26619=CARTESIAN_POINT('Ctrl Pts',(-4.93974113838109,-4.62829899449591,
71.9370197533468));
#26620=CARTESIAN_POINT('Ctrl Pts',(-4.81831816033767,-4.75143126918197,
71.9451612686838));
#26621=CARTESIAN_POINT('Ctrl Pts',(-4.69701067436911,-4.87444642598711,
71.9532950401777));
#26622=CARTESIAN_POINT('Ctrl Pts',(-4.57085930045932,-4.99294457905048,
71.9614288116715));
#26623=CARTESIAN_POINT('Ctrl Pts',(-4.44023937580192,-5.1065216425252,71.9695625831654));
#26624=CARTESIAN_POINT('Ctrl Pts',(-4.30971621890314,-5.2200145641824,71.97769032888));
#26625=CARTESIAN_POINT('Ctrl Pts',(-4.17473137769658,-5.32859341648519,
71.9858180745945));
#26626=CARTESIAN_POINT('Ctrl Pts',(-4.03569712435546,-5.43189080527849,
71.9939458203091));
#26627=CARTESIAN_POINT('Ctrl Pts',(-3.89673664151605,-5.5351333852746,72.0020692535046));
#26628=CARTESIAN_POINT('Ctrl Pts',(-3.75373131839898,-5.63309986499319,
72.0101926867));
#26629=CARTESIAN_POINT('Ctrl Pts',(-3.60712658657559,-5.72546301956615,
72.0183161198954));
#26630=CARTESIAN_POINT('Ctrl Pts',(-3.45959189018067,-5.81841206560659,
72.0264910828401));
#26631=CARTESIAN_POINT('Ctrl Pts',(-3.30841224985171,-5.90568621161012,
72.0346660457848));
#26632=CARTESIAN_POINT('Ctrl Pts',(-3.15407179309374,-5.98699591815549,
72.0428410087295));
#26633=CARTESIAN_POINT('Ctrl Pts',(-3.00073898990254,-6.06777477221062,
72.0509625992095));
#26634=CARTESIAN_POINT('Ctrl Pts',(-2.84428685973461,-6.14266668689104,
72.0590841896896));
#26635=CARTESIAN_POINT('Ctrl Pts',(-2.68521500197278,-6.21143376308404,
72.0672057801696));
#26636=CARTESIAN_POINT('Ctrl Pts',(-2.52612214344734,-6.28020991794834,
72.075328442867));
#26637=CARTESIAN_POINT('Ctrl Pts',(-2.36440920441213,-6.34285947848565,
72.0834511055644));
#26638=CARTESIAN_POINT('Ctrl Pts',(-2.20059583500245,-6.39919268118799,
72.0915737682618));
#26639=CARTESIAN_POINT('Ctrl Pts',(-2.03672964396345,-6.45554404853441,
72.0996990501122));
#26640=CARTESIAN_POINT('Ctrl Pts',(-1.87076201978423,-6.50557488337561,
72.1078243319625));
#26641=CARTESIAN_POINT('Ctrl Pts',(-1.70322779292431,-6.54914529426628,
72.1159496138129));
#26642=CARTESIAN_POINT('Ctrl Pts',(-1.53386839200249,-6.59319037582763,
72.1241634152092));
#26643=CARTESIAN_POINT('Ctrl Pts',(-1.36290842597664,-6.63063334804685,
72.1323772166055));
#26644=CARTESIAN_POINT('Ctrl Pts',(-1.19091005837655,-6.66138290693889,
72.1405910180017));
#26645=CARTESIAN_POINT('Ctrl Pts',(-1.02047087970615,-6.69185371683762,
72.1487303601552));
#26646=CARTESIAN_POINT('Ctrl Pts',(-0.849012418815287,-6.71575198123387,
72.1568697023087));
#26647=CARTESIAN_POINT('Ctrl Pts',(-0.677085565759804,-6.73304122493244,
72.1650090444622));
#26648=CARTESIAN_POINT('Ctrl Pts',(-0.502799515293674,-6.75056771335597,
72.1732600754798));
#26649=CARTESIAN_POINT('Ctrl Pts',(-0.328032516604215,-6.76130246251573,
72.1815111064974));
#26650=CARTESIAN_POINT('Ctrl Pts',(-0.153356693526112,-6.76526205882305,
72.1897621375151));
#26651=CARTESIAN_POINT('Ctrl Pts',(0.0213191295519908,-6.76922165513038,
72.1980131685327));
#26652=CARTESIAN_POINT('Ctrl Pts',(0.195903394273016,-6.76640617183079,
72.2062641995503));
#26653=CARTESIAN_POINT('Ctrl Pts',(0.369831528183824,-6.75688638655122,
72.214515230568));
#26654=CARTESIAN_POINT('Ctrl Pts',(0.543353537741656,-6.74738883008853,
72.2227469953257));
#26655=CARTESIAN_POINT('Ctrl Pts',(0.716764193046762,-6.73118877289631,
72.2309787600834));
#26656=CARTESIAN_POINT('Ctrl Pts',(0.889505497419388,-6.70828360835025,
72.2392105248411));
#26657=CARTESIAN_POINT('Ctrl Pts',(1.06204053146055,-6.68540579485322,72.2474324600514));
#26658=CARTESIAN_POINT('Ctrl Pts',(1.23390745439928,-6.65583886355904,72.2556543952617));
#26659=CARTESIAN_POINT('Ctrl Pts',(1.40454935786716,-6.61963217265997,72.263876330472));
#26660=CARTESIAN_POINT('Ctrl Pts',(1.57502168768379,-6.58346146179072,72.2720900952181));
#26661=CARTESIAN_POINT('Ctrl Pts',(1.74427107428641,-6.54066420544886,72.2803038599641));
#26662=CARTESIAN_POINT('Ctrl Pts',(1.91174672088437,-6.49134142340301,72.2885176247101));
#26663=CARTESIAN_POINT('Ctrl Pts',(2.07908948347132,-6.44205777665383,72.296724872222));
#26664=CARTESIAN_POINT('Ctrl Pts',(2.24466096707993,-6.3862590178193,72.3049321197339));
#26665=CARTESIAN_POINT('Ctrl Pts',(2.40792145601167,-6.32409703133014,72.3131393672457));
#26666=CARTESIAN_POINT('Ctrl Pts',(2.57108509590641,-6.26197192044125,72.3213417460719));
#26667=CARTESIAN_POINT('Ctrl Pts',(2.73194013820082,-6.19349122886557,72.3295441248979));
#26668=CARTESIAN_POINT('Ctrl Pts',(2.88996281538841,-6.11885642303137,72.337746503724));
#26669=CARTESIAN_POINT('Ctrl Pts',(3.04793832801866,-6.04424389322516,72.3459464344106));
#26670=CARTESIAN_POINT('Ctrl Pts',(3.20308283423616,-5.96348105731483,72.3541463650972));
#26671=CARTESIAN_POINT('Ctrl Pts',(3.35489309014139,-5.87681728095417,72.3623462957837));
#26672=CARTESIAN_POINT('Ctrl Pts',(3.50668211989362,-5.79016562194728,72.3705450799537));
#26673=CARTESIAN_POINT('Ctrl Pts',(3.65513751625434,-5.69761484265509,72.3787438641236));
#26674=CARTESIAN_POINT('Ctrl Pts',(3.79978115629632,-5.59945998862885,72.3869426482935));
#26675=CARTESIAN_POINT('Ctrl Pts',(3.94443081146807,-5.50130105274887,72.3951417734169));
#26676=CARTESIAN_POINT('Ctrl Pts',(4.08526809787329,-5.397537779052,72.4033408985403));
#26677=CARTESIAN_POINT('Ctrl Pts',(4.22184433275263,-5.28850824240679,72.4115400236636));
#26678=CARTESIAN_POINT('Ctrl Pts',(4.35845102294825,-5.17945439312017,72.4197409771209));
#26679=CARTESIAN_POINT('Ctrl Pts',(4.49079448907771,-5.06513216553043,72.4279419305781));
#26680=CARTESIAN_POINT('Ctrl Pts',(4.618459521793,-4.94591959554132,72.4361428840353));
#26681=CARTESIAN_POINT('Ctrl Pts',(4.74624420950643,-4.82659529268741,72.4443515238969));
#26682=CARTESIAN_POINT('Ctrl Pts',(4.869341440735,-4.70237173481074,72.4525601637585));
#26683=CARTESIAN_POINT('Ctrl Pts',(4.98737259226172,-4.57366413567466,72.4607688036201));
#26684=CARTESIAN_POINT('Ctrl Pts',(5.10546009610742,-4.44489508689934,72.4689813625818));
#26685=CARTESIAN_POINT('Ctrl Pts',(5.218476466004,-4.31163800160049,72.4771939215434));
#26686=CARTESIAN_POINT('Ctrl Pts',(5.3260837968463,-4.17434071309127,72.4854064805051));
#26687=CARTESIAN_POINT('Ctrl Pts',(5.43383878278655,-4.03685502993994,72.4936303084592));
#26688=CARTESIAN_POINT('Ctrl Pts',(5.53616968615477,-3.89531835452426,72.5018541364133));
#26689=CARTESIAN_POINT('Ctrl Pts',(5.63278162498075,-3.7502080162678,72.5100779643675));
#26690=CARTESIAN_POINT('Ctrl Pts',(5.7215508871709,-3.61687731387508,72.51763420585));
#26691=CARTESIAN_POINT('Ctrl Pts',(5.80549240220805,-3.48053009560183,72.5251904473325));
#26692=CARTESIAN_POINT('Ctrl Pts',(5.88441226823254,-3.34155371907656,72.5327466888151));
#26693=CARTESIAN_POINT('Ctrl Pts',(5.97471142243015,-3.18253863344799,72.5413924487378));
#26694=CARTESIAN_POINT('Ctrl Pts',(6.05864195515587,-3.01971896039609,72.5500382086606));
#26695=CARTESIAN_POINT('Ctrl Pts',(6.13588950645292,-2.85362032593703,72.5586839685834));
#26696=CARTESIAN_POINT('Ctrl Pts',(6.21303788316409,-2.68773493789175,72.5673186286118));
#26697=CARTESIAN_POINT('Ctrl Pts',(6.28352025936741,-2.51857925802448,72.5759532886402));
#26698=CARTESIAN_POINT('Ctrl Pts',(6.3470677158327,-2.34670415916328,72.5845879486686));
#26699=CARTESIAN_POINT('Ctrl Pts',(6.41285895373634,-2.16876036490517,72.5935274877744));
#26700=CARTESIAN_POINT('Ctrl Pts',(6.47121642530732,-1.98790187377263,72.6024670268802));
#26701=CARTESIAN_POINT('Ctrl Pts',(6.52189446506045,-1.80476635236085,72.611406565986));
#26702=CARTESIAN_POINT('Ctrl Pts',(6.57070828173273,-1.62836758453311,72.6200172586089));
#26703=CARTESIAN_POINT('Ctrl Pts',(6.61239743854976,-1.44985664561382,72.6286279512318));
#26704=CARTESIAN_POINT('Ctrl Pts',(6.64679165257546,-1.26982271489104,72.6372386438547));
#26705=CARTESIAN_POINT('Ctrl Pts',(6.68115330679366,-1.08995921603576,72.645841185034));
#26706=CARTESIAN_POINT('Ctrl Pts',(6.70823372962631,-0.908575898445952,
72.6544437262134));
#26707=CARTESIAN_POINT('Ctrl Pts',(6.72791303388148,-0.726274884962787,
72.6630462673927));
#26708=CARTESIAN_POINT('Ctrl Pts',(6.74757018639307,-0.544179076158229,
72.6716391252375));
#26709=CARTESIAN_POINT('Ctrl Pts',(6.75984280769998,-0.361167934827881,
72.6802319830824));
#26710=CARTESIAN_POINT('Ctrl Pts',(6.76466242796618,-0.17785172381141,72.6888248409272));
#26711=CARTESIAN_POINT('Ctrl Pts',(6.76523034021714,-0.156250951077203,
72.6898373665975));
#26712=CARTESIAN_POINT('Ctrl Pts',(6.76569482857818,-0.134645951108895,
72.6908498922679));
#26713=CARTESIAN_POINT('Ctrl Pts',(6.76605582831728,-0.113037728629765,
72.6918624179382));
#26714=CARTESIAN_POINT('Ctrl Pts',(6.76912031005088,0.0703917753572885,
72.7004576219937));
#26715=CARTESIAN_POINT('Ctrl Pts',(6.76471943308091,0.253837892281212,72.7090528260492));
#26716=CARTESIAN_POINT('Ctrl Pts',(6.75289517804965,0.436687204156235,72.7176480301047));
#26717=CARTESIAN_POINT('Ctrl Pts',(6.74105985136034,0.619707727245074,72.7262512822917));
#26718=CARTESIAN_POINT('Ctrl Pts',(6.72178729207275,0.802130025140826,72.7348545344788));
#26719=CARTESIAN_POINT('Ctrl Pts',(6.6951712328786,0.983346918658345,72.7434577866658));
#26720=CARTESIAN_POINT('Ctrl Pts',(6.66745140268478,1.17207889734512,72.7524178166988));
#26721=CARTESIAN_POINT('Ctrl Pts',(6.63176608822662,1.35950298913168,72.7613778467318));
#26722=CARTESIAN_POINT('Ctrl Pts',(6.58827941477441,1.54494768612398,72.7703378767648));
#26723=CARTESIAN_POINT('Ctrl Pts',(6.54641010443929,1.72349529512664,72.7789646639684));
#26724=CARTESIAN_POINT('Ctrl Pts',(6.49730939112459,1.90020781690629,72.787591451172));
#26725=CARTESIAN_POINT('Ctrl Pts',(6.44117420192469,2.07450329005763,72.7962182383755));
#26726=CARTESIAN_POINT('Ctrl Pts',(6.38498536309693,2.24896534120404,72.8048532703883));
#26727=CARTESIAN_POINT('Ctrl Pts',(6.32174873097116,2.42100544554549,72.813488302401));
#26728=CARTESIAN_POINT('Ctrl Pts',(6.25170947614221,2.59006131701813,72.8221233344138));
#26729=CARTESIAN_POINT('Ctrl Pts',(6.1815661980465,2.75936827260152,72.8307711912951));
#26730=CARTESIAN_POINT('Ctrl Pts',(6.10460023137856,2.92568185962392,72.8394190481764));
#26731=CARTESIAN_POINT('Ctrl Pts',(6.02110345828126,3.08846274782027,72.8480669050578));
#26732=CARTESIAN_POINT('Ctrl Pts',(6.01173391866099,3.10672910620517,72.8490373190591));
#26733=CARTESIAN_POINT('Ctrl Pts',(6.00228218838025,3.12495100935973,72.8500077330604));
#26734=CARTESIAN_POINT('Ctrl Pts',(5.99274871423678,3.14312771741994,72.8509781470618));
#26735=CARTESIAN_POINT('Ctrl Pts',(5.91195798973253,3.2971648911917,72.8592018490467));
#26736=CARTESIAN_POINT('Ctrl Pts',(5.82511795541957,3.44828807780692,72.8674255510317));
#26737=CARTESIAN_POINT('Ctrl Pts',(5.73246370899244,3.59599065976049,72.8756492530166));
#26738=CARTESIAN_POINT('Ctrl Pts',(5.63990139356365,3.74354669208099,72.8838647954928));
#26739=CARTESIAN_POINT('Ctrl Pts',(5.54153653989995,3.88768857565882,72.892080337969));
#26740=CARTESIAN_POINT('Ctrl Pts',(5.43765081670197,4.02793279432769,72.9002958804452));
#26741=CARTESIAN_POINT('Ctrl Pts',(5.33384931557788,4.16806331441907,72.9085047624294));
#26742=CARTESIAN_POINT('Ctrl Pts',(5.22453606946594,4.30430217536412,72.9167136444136));
#26743=CARTESIAN_POINT('Ctrl Pts',(5.11003689418772,4.43619340651874,72.9249225263979));
#26744=CARTESIAN_POINT('Ctrl Pts',(4.99560976981379,4.56800164246882,72.9331262427783));
#26745=CARTESIAN_POINT('Ctrl Pts',(4.87600344979385,4.69546742774049,72.9413299591588));
#26746=CARTESIAN_POINT('Ctrl Pts',(4.75158504079528,4.81816651850997,72.9495336755393));
#26747=CARTESIAN_POINT('Ctrl Pts',(4.62721570596386,4.94081721326043,72.9577341561401));
#26748=CARTESIAN_POINT('Ctrl Pts',(4.49803831604578,5.05870470586012,72.965934636741));
#26749=CARTESIAN_POINT('Ctrl Pts',(4.36445807469834,5.17144029398005,72.9741351173419));
#26750=CARTESIAN_POINT('Ctrl Pts',(4.23091161640792,5.28414737075158,72.9823335240035));
#26751=CARTESIAN_POINT('Ctrl Pts',(4.09296479954159,5.39170490879654,72.9905319306652));
#26752=CARTESIAN_POINT('Ctrl Pts',(3.95105725379949,5.49376333465489,72.9987303373268));
#26753=CARTESIAN_POINT('Ctrl Pts',(3.80912557661074,5.59583911559782,73.0069301381315));
#26754=CARTESIAN_POINT('Ctrl Pts',(3.66323211271051,5.6924137021884,73.0151299389361));
#26755=CARTESIAN_POINT('Ctrl Pts',(3.5138472998094,5.78317958856737,73.0233297397407));
#26756=CARTESIAN_POINT('Ctrl Pts',(3.37837121459391,5.86549456235173,73.0307660841119));
#26757=CARTESIAN_POINT('Ctrl Pts',(3.24002419105521,5.94303256079619,73.0382024284831));
#26758=CARTESIAN_POINT('Ctrl Pts',(3.09917575053266,6.01559628526635,73.0456387728543));
#26759=CARTESIAN_POINT('Ctrl Pts',(3.09917575053257,6.0155962852664,71.0459800471047));
#26760=CARTESIAN_POINT('Ctrl Pts',(2.94528128221868,6.09488119431318,71.0541034550639));
#26761=CARTESIAN_POINT('Ctrl Pts',(2.78825364105546,6.16830242277946,71.062226863023));
#26762=CARTESIAN_POINT('Ctrl Pts',(2.62858557352308,6.23560958388724,71.0703502709822));
#26763=CARTESIAN_POINT('Ctrl Pts',(2.46894669294983,6.30290444139925,71.0784721940009));
#26764=CARTESIAN_POINT('Ctrl Pts',(2.30666868121677,6.36408730878024,71.0865941170196));
#26765=CARTESIAN_POINT('Ctrl Pts',(2.14226612133535,6.41895512255529,71.0947160400382));
#26766=CARTESIAN_POINT('Ctrl Pts',(1.97787374744511,6.47381953685124,71.1028374598419));
#26767=CARTESIAN_POINT('Ctrl Pts',(1.81135743428406,6.52236955980444,71.1109588796455));
#26768=CARTESIAN_POINT('Ctrl Pts',(1.64324870502509,6.5644514388815,71.1190802994492));
#26769=CARTESIAN_POINT('Ctrl Pts',(1.47511838094152,6.60653872369091,71.12720276251));
#26770=CARTESIAN_POINT('Ctrl Pts',(1.30539558840919,6.64215612106347,71.1353252255708));
#26771=CARTESIAN_POINT('Ctrl Pts',(1.13462382372935,6.67120062497193,71.1434476886317));
#26772=CARTESIAN_POINT('Ctrl Pts',(0.963797602644333,6.70025439071166,71.151572741817));
#26773=CARTESIAN_POINT('Ctrl Pts',(0.791922103931048,6.72273102820475,71.1596977950024));
#26774=CARTESIAN_POINT('Ctrl Pts',(0.619547709861253,6.73857920003955,71.1678228481878));
#26775=CARTESIAN_POINT('Ctrl Pts',(0.446986941157791,6.75444450723391,71.1759566863427));
#26776=CARTESIAN_POINT('Ctrl Pts',(0.27392656437441,6.76366700033922,71.1840905244977));
#26777=CARTESIAN_POINT('Ctrl Pts',(0.100919640950755,6.76624742572058,71.1922243626527));
#26778=CARTESIAN_POINT('Ctrl Pts',(-0.0721868955381545,6.76882933684643,
71.2003628840685));
#26779=CARTESIAN_POINT('Ctrl Pts',(-0.24523955230309,6.76476156860712,71.2085014054843));
#26780=CARTESIAN_POINT('Ctrl Pts',(-0.417688915932793,6.7540969025849,71.2166399269001));
#26781=CARTESIAN_POINT('Ctrl Pts',(-0.59039269941501,6.74341650265274,71.224790455327));
#26782=CARTESIAN_POINT('Ctrl Pts',(-0.762491048290902,6.72611979841986,
71.2329409837539));
#26783=CARTESIAN_POINT('Ctrl Pts',(-0.933442180150514,6.70231114588959,
71.2410915121808));
#26784=CARTESIAN_POINT('Ctrl Pts',(-1.06438675730829,6.68407427372409,71.2473346267297));
#26785=CARTESIAN_POINT('Ctrl Pts',(-1.19465840221116,6.66201776807838,71.2535777412787));
#26786=CARTESIAN_POINT('Ctrl Pts',(-1.32401957757086,6.63620834198333,71.2598208558276));
#26787=CARTESIAN_POINT('Ctrl Pts',(-1.49444388145069,6.60220622764293,71.2680457227406));
#26788=CARTESIAN_POINT('Ctrl Pts',(-1.66379679169306,6.5615871648036,71.2762705896536));
#26789=CARTESIAN_POINT('Ctrl Pts',(-1.83152606531344,6.51443023387905,71.2844954565667));
#26790=CARTESIAN_POINT('Ctrl Pts',(-1.99906637308398,6.46732643052929,71.2927110572441));
#26791=CARTESIAN_POINT('Ctrl Pts',(-2.16498634442235,6.41369952218237,71.3009266579215));
#26792=CARTESIAN_POINT('Ctrl Pts',(-2.32874247392045,6.3536798384998,71.3091422585989));
#26793=CARTESIAN_POINT('Ctrl Pts',(-2.49234701567201,6.29371571456102,71.3173502541602));
#26794=CARTESIAN_POINT('Ctrl Pts',(-2.65379136996565,6.22737072327476,71.3255582497214));
#26795=CARTESIAN_POINT('Ctrl Pts',(-2.81254569725204,6.15482539970624,71.3337662452826));
#26796=CARTESIAN_POINT('Ctrl Pts',(-2.97118495356932,6.08233265965358,71.3419682913871));
#26797=CARTESIAN_POINT('Ctrl Pts',(-3.12713774158111,6.00364868748302,71.3501703374915));
#26798=CARTESIAN_POINT('Ctrl Pts',(-3.27989268945061,5.9190026985708,71.358372383596));
#26799=CARTESIAN_POINT('Ctrl Pts',(-3.43256758949943,5.83440106649964,71.3665701316013));
#26800=CARTESIAN_POINT('Ctrl Pts',(-3.58204767471219,5.74384381519619,71.3747678796066));
#26801=CARTESIAN_POINT('Ctrl Pts',(-3.72784466929285,5.64760684906668,71.3829656276119));
#26802=CARTESIAN_POINT('Ctrl Pts',(-3.8736138560854,5.55138823816575,71.3911618120648));
#26803=CARTESIAN_POINT('Ctrl Pts',(-4.01570104893917,5.4494922624656,71.3993579965177));
#26804=CARTESIAN_POINT('Ctrl Pts',(-4.15364529628144,5.34223920773669,71.4075541809706));
#26805=CARTESIAN_POINT('Ctrl Pts',(-4.29157933885618,5.23499408731828,71.4157497590905));
#26806=CARTESIAN_POINT('Ctrl Pts',(-4.42537076246738,5.12239289666284,71.4239453372103));
#26807=CARTESIAN_POINT('Ctrl Pts',(-4.55459022422153,5.00479738744994,71.4321409153302));
#26808=CARTESIAN_POINT('Ctrl Pts',(-4.68382363661001,4.88718918253372,71.440337378251));
#26809=CARTESIAN_POINT('Ctrl Pts',(-4.80848383831349,4.76458582639101,71.448533841172));
#26810=CARTESIAN_POINT('Ctrl Pts',(-4.92817697687412,4.63738726920751,71.4567303040928));
#26811=CARTESIAN_POINT('Ctrl Pts',(-5.04790481445122,4.51015183718821,71.4649291431666));
#26812=CARTESIAN_POINT('Ctrl Pts',(-5.1626624748459,4.37831881191929,71.4731279822405));
#26813=CARTESIAN_POINT('Ctrl Pts',(-5.2720951319704,4.24232270336121,71.4813268213143));
#26814=CARTESIAN_POINT('Ctrl Pts',(-5.3816420947562,4.1061845428277,71.4895342243191));
#26815=CARTESIAN_POINT('Ctrl Pts',(-5.48585271661665,3.96587489127608,71.4977416273239));
#26816=CARTESIAN_POINT('Ctrl Pts',(-5.58441382762827,3.82185965228895,71.5059490303287));
#26817=CARTESIAN_POINT('Ctrl Pts',(-5.68302773324149,3.6777672710386,71.5141608296574));
#26818=CARTESIAN_POINT('Ctrl Pts',(-5.77598590437935,3.52996564884307,71.5223726289861));
#26819=CARTESIAN_POINT('Ctrl Pts',(-5.86302028930166,3.37894689026583,71.5305844283148));
#26820=CARTESIAN_POINT('Ctrl Pts',(-5.95018280115931,3.22770581069748,71.5388083165747));
#26821=CARTESIAN_POINT('Ctrl Pts',(-6.03140393182022,3.0732384474288,71.5470322048345));
#26822=CARTESIAN_POINT('Ctrl Pts',(-6.10646253281745,2.91605972766277,71.5552560930943));
#26823=CARTESIAN_POINT('Ctrl Pts',(-6.17581547150636,2.77082912157225,71.5628548334211));
#26824=CARTESIAN_POINT('Ctrl Pts',(-6.23990762182496,2.62328413230967,71.5704535737478));
#26825=CARTESIAN_POINT('Ctrl Pts',(-6.29860228027418,2.47384282340752,71.5780523140746));
#26826=CARTESIAN_POINT('Ctrl Pts',(-6.37026715086443,2.29137831392281,71.5873302067577));
#26827=CARTESIAN_POINT('Ctrl Pts',(-6.43405481597993,2.10565672200331,71.5966080994409));
#26828=CARTESIAN_POINT('Ctrl Pts',(-6.48969440919368,1.91733029895224,71.605885992124));
#26829=CARTESIAN_POINT('Ctrl Pts',(-6.54508447752907,1.72984845662311,71.6151222765763));
#26830=CARTESIAN_POINT('Ctrl Pts',(-6.59239930158858,1.53978526431313,71.6243585610285));
#26831=CARTESIAN_POINT('Ctrl Pts',(-6.63141809376621,1.34780676124961,71.6335948454807));
#26832=CARTESIAN_POINT('Ctrl Pts',(-6.67031674077142,1.15641939104959,71.6428026899191));
#26833=CARTESIAN_POINT('Ctrl Pts',(-6.70097026540113,0.963128656625589,
71.6520105343576));
#26834=CARTESIAN_POINT('Ctrl Pts',(-6.72320763806499,0.768614373704144,
71.661218378796));
#26835=CARTESIAN_POINT('Ctrl Pts',(-6.74533483520506,0.575063815829266,
71.6703806027783));
#26836=CARTESIAN_POINT('Ctrl Pts',(-6.75912898518562,0.38030198423871,71.6795428267606));
#26837=CARTESIAN_POINT('Ctrl Pts',(-6.76447027988159,0.185015763108659,
71.6887050507429));
#26838=CARTESIAN_POINT('Ctrl Pts',(-6.76611711609041,0.124804814575345,
71.6915299617554));
#26839=CARTESIAN_POINT('Ctrl Pts',(-6.76696076101341,0.0645441290638371,
71.6943548727678));
#26840=CARTESIAN_POINT('Ctrl Pts',(-6.76699866280442,0.00425412777616787,
71.6971797837803));
#26841=CARTESIAN_POINT('',(-6.767,3.33069726313195E-12,71.3028202161898));
#26842=CARTESIAN_POINT('Ctrl Pts',(3.09917575053263,6.01559628526637,70.6515467266273));
#26843=CARTESIAN_POINT('Ctrl Pts',(2.9439427023012,6.09557081745671,70.659750383631));
#26844=CARTESIAN_POINT('Ctrl Pts',(2.78552095797009,6.16957970902551,70.6679540406346));
#26845=CARTESIAN_POINT('Ctrl Pts',(2.6244105723732,6.23736788618531,70.6761576976383));
#26846=CARTESIAN_POINT('Ctrl Pts',(2.46334681024357,6.30513644623696,70.6843589805992));
#26847=CARTESIAN_POINT('Ctrl Pts',(2.29959628492877,6.36668773544609,70.6925602635602));
#26848=CARTESIAN_POINT('Ctrl Pts',(2.13368096420307,6.42181396047857,70.7007615465212));
#26849=CARTESIAN_POINT('Ctrl Pts',(1.96778778005423,6.47693283051869,70.7089617352593));
#26850=CARTESIAN_POINT('Ctrl Pts',(1.79973071539011,6.5256282300274,70.7171619239975));
#26851=CARTESIAN_POINT('Ctrl Pts',(1.63004892512788,6.56774158304736,70.7253621127356));
#26852=CARTESIAN_POINT('Ctrl Pts',(1.46035902418122,6.60985694905949,70.7335626934377));
#26853=CARTESIAN_POINT('Ctrl Pts',(1.28904459066358,6.64538955544581,70.7417632741398));
#26854=CARTESIAN_POINT('Ctrl Pts',(1.11665710991708,6.67423148376438,70.7499638548418));
#26855=CARTESIAN_POINT('Ctrl Pts',(0.944230149166233,6.70308001743184,70.7581663136325));
#26856=CARTESIAN_POINT('Ctrl Pts',(0.770730005020289,6.72523476202848,70.7663687724232));
#26857=CARTESIAN_POINT('Ctrl Pts',(0.596715517112192,6.74063940525211,70.7745712312139));
#26858=CARTESIAN_POINT('Ctrl Pts',(0.422537942991574,6.75605848569272,70.7827813773411));
#26859=CARTESIAN_POINT('Ctrl Pts',(0.247845419383574,6.76471479416275,70.7909915234684));
#26860=CARTESIAN_POINT('Ctrl Pts',(0.0731999817781087,6.76660407905381,
70.7992016695956));
#26861=CARTESIAN_POINT('Ctrl Pts',(-0.101529741369486,6.76849427573165,
70.8074157780171));
#26862=CARTESIAN_POINT('Ctrl Pts',(-0.276211975285269,6.76361094738318,
70.8156298864387));
#26863=CARTESIAN_POINT('Ctrl Pts',(-0.450287629949019,6.7520019290811,70.8238439948602));
#26864=CARTESIAN_POINT('Ctrl Pts',(-0.624599517681842,6.74037715651386,
70.8320692504122));
#26865=CARTESIAN_POINT('Ctrl Pts',(-0.798302824744355,6.72200849130114,
70.8402945059643));
#26866=CARTESIAN_POINT('Ctrl Pts',(-0.970845301162993,6.69699547567488,
70.8485197615163));
#26867=CARTESIAN_POINT('Ctrl Pts',(-1.12174326554916,6.67512020635276,70.8557132036479));
#26868=CARTESIAN_POINT('Ctrl Pts',(-1.27175336889713,6.6481638471377,70.8629066457795));
#26869=CARTESIAN_POINT('Ctrl Pts',(-1.4205150722726,6.61622444672537,70.8701000879111));
#26870=CARTESIAN_POINT('Ctrl Pts',(-1.59931525177151,6.57783573244453,70.8787460546831));
#26871=CARTESIAN_POINT('Ctrl Pts',(-1.77671762482904,6.53216062412131,70.8873920214552));
#26872=CARTESIAN_POINT('Ctrl Pts',(-1.95212060784793,6.47931432579215,70.8960379882273));
#26873=CARTESIAN_POINT('Ctrl Pts',(-2.12729922655089,6.42653562507947,70.9046728956298));
#26874=CARTESIAN_POINT('Ctrl Pts',(-2.30048326441725,6.3666041132729,70.9133078030323));
#26875=CARTESIAN_POINT('Ctrl Pts',(-2.47108253964659,6.2996857129744,70.9219427104347));
#26876=CARTESIAN_POINT('Ctrl Pts',(-2.64734556468008,6.23054567910755,70.9308642893664));
#26877=CARTESIAN_POINT('Ctrl Pts',(-2.82084893431632,6.15394690570235,70.9397858682981));
#26878=CARTESIAN_POINT('Ctrl Pts',(-2.99095705046808,6.07012890491259,70.9487074472297));
#26879=CARTESIAN_POINT('Ctrl Pts',(-3.15514447480237,5.98922822848487,70.9573185064721));
#26880=CARTESIAN_POINT('Ctrl Pts',(-3.31616868156277,5.90160250839127,70.9659295657144));
#26881=CARTESIAN_POINT('Ctrl Pts',(-3.47347649773597,5.80751668268597,70.9745406249567));
#26882=CARTESIAN_POINT('Ctrl Pts',(-3.63063596528066,5.71351958431505,70.9831435635674));
#26883=CARTESIAN_POINT('Ctrl Pts',(-3.78408576889572,5.61307468256466,70.9917465021781));
#26884=CARTESIAN_POINT('Ctrl Pts',(-3.93329660906198,5.50649314765228,71.0003494407888));
#26885=CARTESIAN_POINT('Ctrl Pts',(-4.08234036746297,5.40003095950438,71.0089427460903));
#26886=CARTESIAN_POINT('Ctrl Pts',(-4.22715438425042,5.28744602375377,71.0175360513917));
#26887=CARTESIAN_POINT('Ctrl Pts',(-4.36723749492794,5.16909331149048,71.0261293566931));
#26888=CARTESIAN_POINT('Ctrl Pts',(-4.38284502636412,5.15590689902238,71.0270867903337));
#26889=CARTESIAN_POINT('Ctrl Pts',(-4.39839385969793,5.14264893227633,71.0280442239742));
#26890=CARTESIAN_POINT('Ctrl Pts',(-4.4138833242873,5.12931993538895,71.0290016576147));
#26891=CARTESIAN_POINT('Ctrl Pts',(-4.55294640901641,5.00965334440973,71.0375974147313));
#26892=CARTESIAN_POINT('Ctrl Pts',(-4.6870585652526,4.88439841367468,71.0461931718478));
#26893=CARTESIAN_POINT('Ctrl Pts',(-4.81578937574708,4.75399428780069,71.0547889289644));
#26894=CARTESIAN_POINT('Ctrl Pts',(-4.94464029633862,4.62346849057112,71.0633927062061));
#26895=CARTESIAN_POINT('Ctrl Pts',(-5.06809963465862,4.48778412577931,71.0719964834479));
#26896=CARTESIAN_POINT('Ctrl Pts',(-5.18577603295225,4.34741485667725,71.0806002606897));
#26897=CARTESIAN_POINT('Ctrl Pts',(-5.30807722583018,4.20152894154455,71.0895421745755));
#26898=CARTESIAN_POINT('Ctrl Pts',(-5.42413150450199,4.05058272992237,71.0984840884612));
#26899=CARTESIAN_POINT('Ctrl Pts',(-5.53354862518995,3.89514166785477,71.107426002347));
#26900=CARTESIAN_POINT('Ctrl Pts',(-5.63911479380902,3.74517137741593,71.1160532042246));
#26901=CARTESIAN_POINT('Ctrl Pts',(-5.73850291385411,3.59101751378756,71.1246804061022));
#26902=CARTESIAN_POINT('Ctrl Pts',(-5.83140896297384,3.43321401991608,71.1333076079797));
#26903=CARTESIAN_POINT('Ctrl Pts',(-5.92440349085702,3.27526024241789,71.141943025944));
#26904=CARTESIAN_POINT('Ctrl Pts',(-6.01090347907038,3.11365016409605,71.1505784439083));
#26905=CARTESIAN_POINT('Ctrl Pts',(-6.09065166593395,2.94894070544934,71.1592138618726));
#26906=CARTESIAN_POINT('Ctrl Pts',(-6.1705176693811,2.78398791204526,71.1678620374365));
#26907=CARTESIAN_POINT('Ctrl Pts',(-6.24361181285047,2.61592686600952,71.1765102130005));
#26908=CARTESIAN_POINT('Ctrl Pts',(-6.30972503147885,2.44533413404574,71.1851583885645));
#26909=CARTESIAN_POINT('Ctrl Pts',(-6.31671957513785,2.42728602904672,71.1860733348159));
#26910=CARTESIAN_POINT('Ctrl Pts',(-6.32363602825061,2.40920960056799,71.1869882810673));
#26911=CARTESIAN_POINT('Ctrl Pts',(-6.33047417610556,2.39110554046881,71.1879032273187));
#26912=CARTESIAN_POINT('Ctrl Pts',(-6.4020466281971,2.20161680732105,71.197479643058));
#26913=CARTESIAN_POINT('Ctrl Pts',(-6.46516290430702,2.00876335141052,71.2070560587972));
#26914=CARTESIAN_POINT('Ctrl Pts',(-6.51953438499267,1.81327339441637,71.2166324745365));
#26915=CARTESIAN_POINT('Ctrl Pts',(-6.57162171866669,1.62599597449942,71.2258065848553));
#26916=CARTESIAN_POINT('Ctrl Pts',(-6.61568378131449,1.436299258653,71.2349806951742));
#26917=CARTESIAN_POINT('Ctrl Pts',(-6.6515147912199,1.24484536476742,71.2441548054931));
#26918=CARTESIAN_POINT('Ctrl Pts',(-6.68724741901072,1.05391715070428,71.2533037262242));
#26919=CARTESIAN_POINT('Ctrl Pts',(-6.71479403405442,0.861241579233054,
71.2624526469552));
#26920=CARTESIAN_POINT('Ctrl Pts',(-6.7339988753798,0.667493929847773,71.2716015676862));
#26921=CARTESIAN_POINT('Ctrl Pts',(-6.753122924958,0.474561346353395,71.2807120003465));
#26922=CARTESIAN_POINT('Ctrl Pts',(-6.76397515626355,0.280565880181399,
71.2898224330069));
#26923=CARTESIAN_POINT('Ctrl Pts',(-6.76645108534723,0.086189962311772,
71.2989328656672));
#26924=CARTESIAN_POINT('Ctrl Pts',(-6.76680323855356,0.0585437331999436,
71.3002286491748));
#26925=CARTESIAN_POINT('Ctrl Pts',(-6.76698602565755,0.0308898307818761,
71.3015244326823));
#26926=CARTESIAN_POINT('Ctrl Pts',(-6.76699922901903,0.00323024083590044,
71.3028202161898));
#26927=CARTESIAN_POINT('Ctrl Pts',(-6.767,3.33069737261845E-12,71.3028202161898));
#26928=CARTESIAN_POINT('Ctrl Pts',(-6.76700000000009,-0.186007249412401,
71.3115697279958));
#26929=CARTESIAN_POINT('Ctrl Pts',(-6.75932637295456,-0.372014355524311,
71.3203192398017));
#26930=CARTESIAN_POINT('Ctrl Pts',(-6.74400518266954,-0.557389537151886,
71.3290687516077));
#26931=CARTESIAN_POINT('Ctrl Pts',(-6.72868405709679,-0.742763935808368,
71.3378182264582));
#26932=CARTESIAN_POINT('Ctrl Pts',(-6.70571545653032,-0.927506129692142,
71.3465677013088));
#26933=CARTESIAN_POINT('Ctrl Pts',(-6.67517739415696,-1.110988639247,71.3553171761593));
#26934=CARTESIAN_POINT('Ctrl Pts',(-6.6446394582312,-1.29447038906401,71.3640666147813));
#26935=CARTESIAN_POINT('Ctrl Pts',(-6.60653217027178,-1.47669218228127,
71.3728160534033));
#26936=CARTESIAN_POINT('Ctrl Pts',(-6.56098496116732,-1.65703510504042,
71.3815654920253));
#26937=CARTESIAN_POINT('Ctrl Pts',(-6.51543793687533,-1.83737729603968,
71.3903148951455));
#26938=CARTESIAN_POINT('Ctrl Pts',(-6.46245112202648,-2.01584035397027,
71.3990642982658));
#26939=CARTESIAN_POINT('Ctrl Pts',(-6.40220448416243,-2.19181813638142,
71.407813701386));
#26940=CARTESIAN_POINT('Ctrl Pts',(-6.34195808575187,-2.36779521935944,
71.4165630697313));
#26941=CARTESIAN_POINT('Ctrl Pts',(-6.27445201489234,-2.54128677544828,
71.4253124380765));
#26942=CARTESIAN_POINT('Ctrl Pts',(-6.19991555136183,-2.71170355237842,
71.4340618064218));
#26943=CARTESIAN_POINT('Ctrl Pts',(-6.12537937789038,-2.88211966613073,
71.4428111407189));
#26944=CARTESIAN_POINT('Ctrl Pts',(-6.04381298133617,-3.04946076210445,
71.4515604750159));
#26945=CARTESIAN_POINT('Ctrl Pts',(-5.95549339426307,-3.21315848206854,
71.460309809313));
#26946=CARTESIAN_POINT('Ctrl Pts',(-5.8671741435517,-3.37685557859619,71.4690591102885));
#26947=CARTESIAN_POINT('Ctrl Pts',(-5.77210188986257,-3.53690907467279,
71.4778084112641));
#26948=CARTESIAN_POINT('Ctrl Pts',(-5.67059953467099,-3.69277536784858,
71.4865577122396));
#26949=CARTESIAN_POINT('Ctrl Pts',(-5.56909755761795,-3.8486410803575,71.4953069806204));
#26950=CARTESIAN_POINT('Ctrl Pts',(-5.46116568338098,-4.00031938104242,
71.5040562490012));
#26951=CARTESIAN_POINT('Ctrl Pts',(-5.3471704868614,-4.14729511663185,71.5128055173819));
#26952=CARTESIAN_POINT('Ctrl Pts',(-5.23317570555527,-4.29427031688031,
71.5215547538946));
#26953=CARTESIAN_POINT('Ctrl Pts',(-5.11311782178796,-4.43654275987142,
71.5303039904072));
#26954=CARTESIAN_POINT('Ctrl Pts',(-4.98740459171984,-4.57362924147682,
71.5390532269198));
#26955=CARTESIAN_POINT('Ctrl Pts',(-4.86169180910801,-4.71071523514466,
71.547802432291));
#26956=CARTESIAN_POINT('Ctrl Pts',(-4.73032391415404,-4.8426150931655,71.5565516376621));
#26957=CARTESIAN_POINT('Ctrl Pts',(-4.59374707237268,-4.96888084331547,
71.5653008430332));
#26958=CARTESIAN_POINT('Ctrl Pts',(-4.4571707053739,-5.09514615452734,71.5740500179894));
#26959=CARTESIAN_POINT('Ctrl Pts',(-4.31538563819511,-5.2157772025363,71.5827991929456));
#26960=CARTESIAN_POINT('Ctrl Pts',(-4.16887341290665,-5.33036429028637,
71.5915483679019));
#26961=CARTESIAN_POINT('Ctrl Pts',(-4.02236168477358,-5.44495098921162,
71.6002975131698));
#26962=CARTESIAN_POINT('Ctrl Pts',(-3.87112305634461,-5.55349359238743,
71.6090466584377));
#26963=CARTESIAN_POINT('Ctrl Pts',(-3.71567117316758,-5.65562346102457,
71.6177958037056));
#26964=CARTESIAN_POINT('Ctrl Pts',(-3.56021980457321,-5.75775299158756,
71.6265449200118));
#26965=CARTESIAN_POINT('Ctrl Pts',(-3.40055544862404,-5.85346967275344,
71.6352940363179));
#26966=CARTESIAN_POINT('Ctrl Pts',(-3.23722036323414,-5.94244842803556,
71.6440431526241));
#26967=CARTESIAN_POINT('Ctrl Pts',(-3.07388580496062,-6.03142689616467,
71.652792240695));
#26968=CARTESIAN_POINT('Ctrl Pts',(-2.90688079257727,-6.11366734484813,
71.661541328766));
#26969=CARTESIAN_POINT('Ctrl Pts',(-2.7367725109464,-6.18889046787291,71.6702904168369));
#26970=CARTESIAN_POINT('Ctrl Pts',(-2.56666476416692,-6.2641133543825,71.6790394773992));
#26971=CARTESIAN_POINT('Ctrl Pts',(-2.39345402972164,-6.33231884350263,
71.6877885379614));
#26972=CARTESIAN_POINT('Ctrl Pts',(-2.21772856474133,-6.3932752962101,71.6965375985236));
#26973=CARTESIAN_POINT('Ctrl Pts',(-2.04200363768374,-6.45423156232048,
71.7052866323036));
#26974=CARTESIAN_POINT('Ctrl Pts',(-1.86376426620208,-6.50793874252023,
71.7140356660836));
#26975=CARTESIAN_POINT('Ctrl Pts',(-1.68361578194813,-6.55421443796091,
71.7227846998636));
#26976=CARTESIAN_POINT('Ctrl Pts',(-1.50346783420031,-6.60048999558641,
71.7315337075878));
#26977=CARTESIAN_POINT('Ctrl Pts',(-1.32141106257449,-6.63933404145454,
71.740282715312));
#26978=CARTESIAN_POINT('Ctrl Pts',(-1.13806375959286,-6.67061465526989,
71.7490317230362));
#26979=CARTESIAN_POINT('Ctrl Pts',(-0.954716987421707,-6.70189517852444,
71.7577807054311));
#26980=CARTESIAN_POINT('Ctrl Pts',(-0.770079973812568,-6.72561226535797,
71.766529687826));
#26981=CARTESIAN_POINT('Ctrl Pts',(-0.584779770555288,-6.74168536939758,
71.7752786702208));
#26982=CARTESIAN_POINT('Ctrl Pts',(-0.391490647556741,-6.75845143942377,
71.7844048508969));
#26983=CARTESIAN_POINT('Ctrl Pts',(-0.197480213107163,-6.76689975924018,
71.793531031573));
#26984=CARTESIAN_POINT('Ctrl Pts',(-0.00346532630061558,-6.76699911271707,
71.802657212249));
#26985=CARTESIAN_POINT('Ctrl Pts',(0.184486595293259,-6.76709536139781,
71.8114981997789));
#26986=CARTESIAN_POINT('Ctrl Pts',(0.37244237818246,-6.75935659726785,71.8203391873089));
#26987=CARTESIAN_POINT('Ctrl Pts',(0.559750217719346,-6.74380965729039,
71.8291801748388));
#26988=CARTESIAN_POINT('Ctrl Pts',(0.745129914455018,-6.72842275717284,
71.8379301534366));
#26989=CARTESIAN_POINT('Ctrl Pts',(0.929874656311454,-6.70538772273511,
71.8466801320343));
#26990=CARTESIAN_POINT('Ctrl Pts',(1.11335688289505,-6.67478280180788,71.8554301106321));
#26991=CARTESIAN_POINT('Ctrl Pts',(1.29683723118585,-6.64417819418076,71.864179999657));
#26992=CARTESIAN_POINT('Ctrl Pts',(1.47905480729965,-6.60600390230136,71.872929888682));
#26993=CARTESIAN_POINT('Ctrl Pts',(1.65939064804539,-6.56038959797202,71.8816797777069));
#26994=CARTESIAN_POINT('Ctrl Pts',(1.83972470263996,-6.51477574543332,71.8904295800679));
#26995=CARTESIAN_POINT('Ctrl Pts',(2.0181767812558,-6.46172209820184,71.8991793824288));
#26996=CARTESIAN_POINT('Ctrl Pts',(2.19414072347413,-6.40140886724106,71.9079291847898));
#26997=CARTESIAN_POINT('Ctrl Pts',(2.37010298131828,-6.34109621361475,71.9166789033952));
#26998=CARTESIAN_POINT('Ctrl Pts',(2.54357687926641,-6.27352420826081,71.9254286220007));
#26999=CARTESIAN_POINT('Ctrl Pts',(2.71397317789698,-6.19892237325616,71.9341783406062));
#27000=CARTESIAN_POINT('Ctrl Pts',(2.88436790206936,-6.12432122757089,71.9429279783645));
#27001=CARTESIAN_POINT('Ctrl Pts',(3.05168482125999,-6.04269049717547,71.9516776161228));
#27002=CARTESIAN_POINT('Ctrl Pts',(3.21535561997139,-5.95430745235064,71.960427253881));
#27003=CARTESIAN_POINT('Ctrl Pts',(3.37902496075022,-5.86592519481665,71.9691768137));
#27004=CARTESIAN_POINT('Ctrl Pts',(3.53904799384609,-5.77079087940395,71.977926373519));
#27005=CARTESIAN_POINT('Ctrl Pts',(3.69488118814711,-5.66922763747202,71.986675933338));
#27006=CARTESIAN_POINT('Ctrl Pts',(3.85071304610566,-5.56766526649236,71.9954254181255));
#27007=CARTESIAN_POINT('Ctrl Pts',(4.00235489705708,-5.45967423580904,72.0041749029129));
#27008=CARTESIAN_POINT('Ctrl Pts',(4.14929168607401,-5.34562133936525,72.0129243877004));
#27009=CARTESIAN_POINT('Ctrl Pts',(4.296227263855,-5.23156938308742,72.0216738003636));
#27010=CARTESIAN_POINT('Ctrl Pts',(4.43845763091806,-5.11145583677428,72.0304232130269));
#27011=CARTESIAN_POINT('Ctrl Pts',(4.57549970660699,-4.98568866204453,72.0391726256902));
#27012=CARTESIAN_POINT('Ctrl Pts',(4.71254069815041,-4.85992248226408,72.0479219691366));
#27013=CARTESIAN_POINT('Ctrl Pts',(4.84439326931069,-4.72850295734253,72.0566713125829));
#27014=CARTESIAN_POINT('Ctrl Pts',(4.97060959434462,-4.59187644221937,72.0654206560292));
#27015=CARTESIAN_POINT('Ctrl Pts',(5.09682496280291,-4.45525096256921,72.0741699331655));
#27016=CARTESIAN_POINT('Ctrl Pts',(5.21740397615626,-4.31341878218583,72.0829192103018));
#27017=CARTESIAN_POINT('Ctrl Pts',(5.33193710451733,-4.16686161438935,72.0916684874381));
#27018=CARTESIAN_POINT('Ctrl Pts',(5.44646940289189,-4.02030550864777,72.1004177011711));
#27019=CARTESIAN_POINT('Ctrl Pts',(5.55495572749479,-3.86902470980401,72.1091669149041));
#27020=CARTESIAN_POINT('Ctrl Pts',(5.65702762491277,-3.71353301466054,72.117916128637));
#27021=CARTESIAN_POINT('Ctrl Pts',(5.75909881654984,-3.55804239467168,72.1266652818731));
#27022=CARTESIAN_POINT('Ctrl Pts',(5.85475551250622,-3.3983411761983,72.1354144351092));
#27023=CARTESIAN_POINT('Ctrl Pts',(5.94367283727943,-3.23497174692248,72.1441635883454));
#27024=CARTESIAN_POINT('Ctrl Pts',(6.03258957676172,-3.0716033930124,72.1529126839909));
#27025=CARTESIAN_POINT('Ctrl Pts',(6.11476689685157,-2.90456712829772,72.1616617796364));
#27026=CARTESIAN_POINT('Ctrl Pts',(6.18992570525145,-2.73443024476167,72.170410875282));
#27027=CARTESIAN_POINT('Ctrl Pts',(6.26508404388594,-2.56429442463283,72.179159916243));
#27028=CARTESIAN_POINT('Ctrl Pts',(6.33322384283223,-2.39105828656237,72.187908957204));
#27029=CARTESIAN_POINT('Ctrl Pts',(6.39411368719952,-2.21531017132315,72.1966579981651));
#27030=CARTESIAN_POINT('Ctrl Pts',(6.4550031712082,-2.03956309619737,72.2054069873475));
#27031=CARTESIAN_POINT('Ctrl Pts',(6.50864269270014,-1.86130434438842,72.2141559765299));
#27032=CARTESIAN_POINT('Ctrl Pts',(6.55485008446284,-1.6811393072014,72.2229049657123));
#27033=CARTESIAN_POINT('Ctrl Pts',(6.60199664749361,-1.49731239212031,72.2318317792417));
#27034=CARTESIAN_POINT('Ctrl Pts',(6.6414056364087,-1.31150116499858,72.2407585927711));
#27035=CARTESIAN_POINT('Ctrl Pts',(6.67293772282141,-1.12436255155843,72.2496854063004));
#27036=CARTESIAN_POINT('Ctrl Pts',(6.70384494949845,-0.94093239505318,72.258435320456));
#27037=CARTESIAN_POINT('Ctrl Pts',(6.7271844934891,-0.756227260508556,72.2671852346115));
#27038=CARTESIAN_POINT('Ctrl Pts',(6.74287707373917,-0.570874564543536,
72.275935148767));
#27039=CARTESIAN_POINT('Ctrl Pts',(6.7585693453866,-0.385525513634342,72.284684890851));
#27040=CARTESIAN_POINT('Ctrl Pts',(6.76661493004097,-0.199529212420115,
72.293434632935));
#27041=CARTESIAN_POINT('Ctrl Pts',(6.76698649908906,-0.0135174386023319,
72.3021843750189));
#27042=CARTESIAN_POINT('Ctrl Pts',(6.76735806132394,0.17249092444395,72.3109339566648));
#27043=CARTESIAN_POINT('Ctrl Pts',(6.76005588896299,0.358514472899656,72.3196835383107));
#27044=CARTESIAN_POINT('Ctrl Pts',(6.74510478454598,0.543921359660541,72.3284331199566));
#27045=CARTESIAN_POINT('Ctrl Pts',(6.73015393440705,0.729325093148832,72.3371825527957));
#27046=CARTESIAN_POINT('Ctrl Pts',(6.70755443556919,0.914111900254797,72.3459319856347));
#27047=CARTESIAN_POINT('Ctrl Pts',(6.67738304682343,1.09765415591389,72.3546814184738));
#27048=CARTESIAN_POINT('Ctrl Pts',(6.6472121311189,1.28119353391119,72.3634307141351));
#27049=CARTESIAN_POINT('Ctrl Pts',(6.60946960955529,1.46348811672496,72.3721800097964));
#27050=CARTESIAN_POINT('Ctrl Pts',(6.56428366991223,1.64391876348061,72.3809293054577));
#27051=CARTESIAN_POINT('Ctrl Pts',(6.51909837867761,1.82434682109559,72.3896784755686));
#27052=CARTESIAN_POINT('Ctrl Pts',(6.46646995271968,2.00291071820293,72.3984276456794));
#27053=CARTESIAN_POINT('Ctrl Pts',(6.40657713281599,2.17900400212557,72.4071768157902));
#27054=CARTESIAN_POINT('Ctrl Pts',(6.34668509279116,2.35509499309505,72.415925871976));
#27055=CARTESIAN_POINT('Ctrl Pts',(6.27952894037589,2.52871516397964,72.4246749281618));
#27056=CARTESIAN_POINT('Ctrl Pts',(6.20533675061518,2.69927486771257,72.4334239843475));
#27057=CARTESIAN_POINT('Ctrl Pts',(6.12832117907992,2.87632521635763,72.4425059856298));
#27058=CARTESIAN_POINT('Ctrl Pts',(6.04372366626158,3.05007728919841,72.4515879869121));
#27059=CARTESIAN_POINT('Ctrl Pts',(5.95185378007951,3.21989527478043,72.4606699881944));
#27060=CARTESIAN_POINT('Ctrl Pts',(5.86334450817457,3.38350129286602,72.4694197685015));
#27061=CARTESIAN_POINT('Ctrl Pts',(5.76808562057345,3.54345567124816,72.4781695488086));
#27062=CARTESIAN_POINT('Ctrl Pts',(5.66640068804577,3.69921508465167,72.4869193291157));
#27063=CARTESIAN_POINT('Ctrl Pts',(5.5647194110802,3.85496889852143,72.4956687948692));
#27064=CARTESIAN_POINT('Ctrl Pts',(5.45661270815215,4.00652780919499,72.5044182606227));
#27065=CARTESIAN_POINT('Ctrl Pts',(5.34244776449219,4.15337704569094,72.5131677263762));
#27066=CARTESIAN_POINT('Ctrl Pts',(5.22828631819701,4.30022178356121,72.5219169240958));
#27067=CARTESIAN_POINT('Ctrl Pts',(5.10806717844175,4.44235690972558,72.5306661218154));
#27068=CARTESIAN_POINT('Ctrl Pts',(4.98219864544825,4.5792996907053,72.539415319535));
#27069=CARTESIAN_POINT('Ctrl Pts',(4.85633329944131,4.71623900429892,72.5481642957252));
#27070=CARTESIAN_POINT('Ctrl Pts',(4.72481904033754,4.84798602483514,72.5569132719154));
#27071=CARTESIAN_POINT('Ctrl Pts',(4.58810250737304,4.97409332259029,72.5656622481057));
#27072=CARTESIAN_POINT('Ctrl Pts',(4.45137708685749,5.10020881822042,72.5744117930419));
#27073=CARTESIAN_POINT('Ctrl Pts',(4.3094489263616,5.22068366307843,72.583161337978));
#27074=CARTESIAN_POINT('Ctrl Pts',(4.16280009466772,5.33510865604764,72.5919108829142));
#27075=CARTESIAN_POINT('Ctrl Pts',(4.01615988348899,5.44952692272811,72.6006599135225));
#27076=CARTESIAN_POINT('Ctrl Pts',(3.8647997823234,5.55789587288551,72.6094089441308));
#27077=CARTESIAN_POINT('Ctrl Pts',(3.70923383581175,5.65984746713807,72.6181579747391));
#27078=CARTESIAN_POINT('Ctrl Pts',(3.55366577799648,5.76180044505317,72.6269071240871));
#27079=CARTESIAN_POINT('Ctrl Pts',(3.39389200026947,5.85733573570998,72.6356562734351));
#27080=CARTESIAN_POINT('Ctrl Pts',(3.23045513626147,5.94612887621871,72.6444054227831));
#27081=CARTESIAN_POINT('Ctrl Pts',(3.1869512215165,5.9697639920665,72.6467342868961));
#27082=CARTESIAN_POINT('Ctrl Pts',(3.14318791262702,5.99292165435313,72.6490631510091));
#27083=CARTESIAN_POINT('Ctrl Pts',(3.09917575053262,6.01559628526637,72.6513920151221));
#27084=CARTESIAN_POINT('Origin',(0.,0.,-3.69717978381041));
#27085=CARTESIAN_POINT('',(3.09917575053257,6.0155962852664,75.0456602561759));
#27086=CARTESIAN_POINT('',(3.09917575053252,6.01559628526642,74.65129258962));
#27087=CARTESIAN_POINT('',(3.09917575053259,6.01559628526639,-3.69717978381041));
#27088=CARTESIAN_POINT('',(-6.76699811314402,-0.00505338552136531,73.6971797838396));
#27089=CARTESIAN_POINT('Ctrl Pts',(-6.76699811314402,-0.00505338552137147,
73.6971797838396));
#27090=CARTESIAN_POINT('Ctrl Pts',(-6.76684798857142,-0.206085484741003,
73.7066067669995));
#27091=CARTESIAN_POINT('Ctrl Pts',(-6.75773564685474,-0.40676139421809,
73.7160337501595));
#27092=CARTESIAN_POINT('Ctrl Pts',(-6.7397798239725,-0.606347197876985,
73.7254607333194));
#27093=CARTESIAN_POINT('Ctrl Pts',(-6.72173924480955,-0.806875099846274,
73.7349322143582));
#27094=CARTESIAN_POINT('Ctrl Pts',(-6.69477160047039,-1.00630246036111,
73.7444036953969));
#27095=CARTESIAN_POINT('Ctrl Pts',(-6.65904688194988,-1.20390349446855,
73.7538751764357));
#27096=CARTESIAN_POINT('Ctrl Pts',(-6.62310148542693,-1.40272514565269,
73.7634051645139));
#27097=CARTESIAN_POINT('Ctrl Pts',(-6.57829056854179,-1.59969771800889,
73.7729351525921));
#27098=CARTESIAN_POINT('Ctrl Pts',(-6.52483603914106,-1.79410246706424,
73.7824651406703));
#27099=CARTESIAN_POINT('Ctrl Pts',(-6.48144530150877,-1.95190697035518,
73.7902009343809));
#27100=CARTESIAN_POINT('Ctrl Pts',(-6.43236015357818,-2.1080198794279,73.7979367280915));
#27101=CARTESIAN_POINT('Ctrl Pts',(-6.37772216023483,-2.2620674275648,73.8056725218021));
#27102=CARTESIAN_POINT('Ctrl Pts',(-6.31963014829381,-2.4258533109448,73.813897344734));
#27103=CARTESIAN_POINT('Ctrl Pts',(-6.25514327880184,-2.58762986612481,
73.822122167666));
#27104=CARTESIAN_POINT('Ctrl Pts',(-6.18441902472954,-2.74686190525904,
73.830346990598));
#27105=CARTESIAN_POINT('Ctrl Pts',(-6.11377442809694,-2.9059145997438,73.8385625498291));
#27106=CARTESIAN_POINT('Ctrl Pts',(-6.03690658021127,-3.06242816004967,
73.8467781090602));
#27107=CARTESIAN_POINT('Ctrl Pts',(-5.95402242007101,-3.21588339671882,
73.8549936682913));
#27108=CARTESIAN_POINT('Ctrl Pts',(-5.87121495973981,-3.36919662812023,
73.8632016249621));
#27109=CARTESIAN_POINT('Ctrl Pts',(-5.78240244418765,-3.51945685846059,
73.8714095816328));
#27110=CARTESIAN_POINT('Ctrl Pts',(-5.68783953845758,-3.6661656242945,73.8796175383036));
#27111=CARTESIAN_POINT('Ctrl Pts',(-5.59334514600925,-3.81276809581638,
73.8878195480966));
#27112=CARTESIAN_POINT('Ctrl Pts',(-5.49310885546529,-3.95582392768004,
73.8960215578896));
#27113=CARTESIAN_POINT('Ctrl Pts',(-5.38743085978608,-4.09485991592199,
73.9042235676825));
#27114=CARTESIAN_POINT('Ctrl Pts',(-5.28180820900181,-4.2338230892689,73.9124212819799));
#27115=CARTESIAN_POINT('Ctrl Pts',(-5.17074974710591,-4.36877032801805,
73.9206189962772));
#27116=CARTESIAN_POINT('Ctrl Pts',(-5.05459856036554,-4.4992579825512,73.9288167105745));
#27117=CARTESIAN_POINT('Ctrl Pts',(-4.93846946939272,-4.62972081405012,
73.9370128653975));
#27118=CARTESIAN_POINT('Ctrl Pts',(-4.81724981695655,-4.75572547929968,
73.9452090202206));
#27119=CARTESIAN_POINT('Ctrl Pts',(-4.69132269250438,-4.87686173628015,
73.9534051750436));
#27120=CARTESIAN_POINT('Ctrl Pts',(-4.56540484558621,-4.9979890686882,73.9616007260245));
#27121=CARTESIAN_POINT('Ctrl Pts',(-4.4347804753286,-5.11424845772864,73.9697962770053));
#27122=CARTESIAN_POINT('Ctrl Pts',(-4.29986917423884,-5.22526689121529,
73.9779918279862));
#27123=CARTESIAN_POINT('Ctrl Pts',(-4.16494326651792,-5.33629734449046,
73.9861882662863));
#27124=CARTESIAN_POINT('Ctrl Pts',(-4.02572978039465,-5.44208548366305,
73.9943847045864));
#27125=CARTESIAN_POINT('Ctrl Pts',(-3.88268102096551,-5.54229889932276,
74.0025811428865));
#27126=CARTESIAN_POINT('Ctrl Pts',(-3.73959074715509,-5.6425413980585,74.0107799598865));
#27127=CARTESIAN_POINT('Ctrl Pts',(-3.59266327682294,-5.73720574489927,
74.0189787768865));
#27128=CARTESIAN_POINT('Ctrl Pts',(-3.44237951929786,-5.82600311063414,
74.0271775938864));
#27129=CARTESIAN_POINT('Ctrl Pts',(-3.29193870951321,-5.9148932730036,74.0353849789629));
#27130=CARTESIAN_POINT('Ctrl Pts',(-3.13813491446167,-5.99790402210956,
74.0435923640394));
#27131=CARTESIAN_POINT('Ctrl Pts',(-2.98147413730228,-6.07479225723791,
74.0517997491159));
#27132=CARTESIAN_POINT('Ctrl Pts',(-2.82472940140128,-6.15172169884808,
74.0600115327517));
#27133=CARTESIAN_POINT('Ctrl Pts',(-2.66512495873763,-6.22252193992118,
74.0682233163875));
#27134=CARTESIAN_POINT('Ctrl Pts',(-2.50318627035949,-6.28699828979488,
74.0764351000234));
#27135=CARTESIAN_POINT('Ctrl Pts',(-2.34100910679523,-6.35156958924296,
74.0846589765485));
#27136=CARTESIAN_POINT('Ctrl Pts',(-2.17649116610084,-6.40979826653793,
74.0928828530736));
#27137=CARTESIAN_POINT('Ctrl Pts',(-2.01017376801462,-6.46153932297761,
74.1011067295988));
#27138=CARTESIAN_POINT('Ctrl Pts',(-1.85649201112722,-6.5093494531766,74.1087058130822));
#27139=CARTESIAN_POINT('Ctrl Pts',(-1.7012741896522,-6.55162078995792,74.1163048965656));
#27140=CARTESIAN_POINT('Ctrl Pts',(-1.54495370933529,-6.58827800233196,
74.1239039800491));
#27141=CARTESIAN_POINT('Ctrl Pts',(-1.37727264099333,-6.62759927693945,
74.1320553267846));
#27142=CARTESIAN_POINT('Ctrl Pts',(-1.20782614281645,-6.66057652599887,
74.1402066735201));
#27143=CARTESIAN_POINT('Ctrl Pts',(-1.03713977751074,-6.68704943019752,
74.1483580202556));
#27144=CARTESIAN_POINT('Ctrl Pts',(-0.866651660399433,-6.71349158674127,
74.1564998993938));
#27145=CARTESIAN_POINT('Ctrl Pts',(-0.694926900390888,-6.73344438107405,
74.164641778532));
#27146=CARTESIAN_POINT('Ctrl Pts',(-0.522504970112164,-6.74679757782966,
74.1727836576702));
#27147=CARTESIAN_POINT('Ctrl Pts',(-0.350247027367419,-6.76013807458936,
74.1809177932071));
#27148=CARTESIAN_POINT('Ctrl Pts',(-0.177293596488486,-6.76689144186465,
74.1890519287439));
#27149=CARTESIAN_POINT('Ctrl Pts',(-0.00419306548881221,-6.76699870091622,
74.1971860642808));
#27150=CARTESIAN_POINT('Ctrl Pts',(0.168779231809186,-6.76710588050977,
74.2053141740112));
#27151=CARTESIAN_POINT('Ctrl Pts',(0.341898048117475,-6.76057675506325,
74.2134422837416));
#27152=CARTESIAN_POINT('Ctrl Pts',(0.514611168556591,-6.74740426721245,
74.221570393472));
#27153=CARTESIAN_POINT('Ctrl Pts',(0.687232646626987,-6.73423876874374,
74.2296941903903));
#27154=CARTESIAN_POINT('Ctrl Pts',(0.85944849372861,-6.71443695573693,74.2378179873086));
#27155=CARTESIAN_POINT('Ctrl Pts',(1.03070779855958,-6.68804384211022,74.2459417842269));
#27156=CARTESIAN_POINT('Ctrl Pts',(1.20304095111717,-6.66148523566493,74.2541165198131));
#27157=CARTESIAN_POINT('Ctrl Pts',(1.37440514971835,-6.62825239333862,74.2622912553993));
#27158=CARTESIAN_POINT('Ctrl Pts',(1.54424509702084,-6.588444131988,74.2704659909855));
#27159=CARTESIAN_POINT('Ctrl Pts',(1.71298839852233,-6.5488929100639,74.2785879428209));
#27160=CARTESIAN_POINT('Ctrl Pts',(1.88022672055067,-6.50285104346772,74.2867098946563));
#27161=CARTESIAN_POINT('Ctrl Pts',(2.04542682387103,-6.45046650314447,74.2948318464917));
#27162=CARTESIAN_POINT('Ctrl Pts',(2.21064871158063,-6.39807505504579,74.3029548693419));
#27163=CARTESIAN_POINT('Ctrl Pts',(2.37383149636435,-6.33933937790731,74.3110778921922));
#27164=CARTESIAN_POINT('Ctrl Pts',(2.53445836165528,-6.27445693371432,74.3192009150424));
#27165=CARTESIAN_POINT('Ctrl Pts',(2.69513699027794,-6.20955358061871,74.3273265556037));
#27166=CARTESIAN_POINT('Ctrl Pts',(2.85325772009297,-6.13849965297926,74.335452196165));
#27167=CARTESIAN_POINT('Ctrl Pts',(3.00832497268535,-6.06154022165305,74.3435778367264));
#27168=CARTESIAN_POINT('Ctrl Pts',(3.16506191321886,-5.98375212900542,74.3517909701905));
#27169=CARTESIAN_POINT('Ctrl Pts',(3.31867889515768,-5.89993079157754,74.3600041036546));
#27170=CARTESIAN_POINT('Ctrl Pts',(3.46869173861445,-5.81037577291416,74.3682172371187));
#27171=CARTESIAN_POINT('Ctrl Pts',(3.61736322108309,-5.72162152307537,74.3763569316921));
#27172=CARTESIAN_POINT('Ctrl Pts',(3.76249448685049,-5.62723596626766,74.3844966262655));
#27173=CARTESIAN_POINT('Ctrl Pts',(3.90364563443486,-5.52755278226791,74.3926363208389));
#27174=CARTESIAN_POINT('Ctrl Pts',(4.0467070472529,-5.42652053859676,74.4008861737484));
#27175=CARTESIAN_POINT('Ctrl Pts',(4.18567953042559,-5.32004648992106,74.4091360266578));
#27176=CARTESIAN_POINT('Ctrl Pts',(4.32014216904989,-5.20851808475279,74.4173858795673));
#27177=CARTESIAN_POINT('Ctrl Pts',(4.45460480767419,-5.09698967958453,74.4256357324768));
#27178=CARTESIAN_POINT('Ctrl Pts',(4.58455736100398,-4.98040722385045,74.4338855853863));
#27179=CARTESIAN_POINT('Ctrl Pts',(4.70962011429032,-4.85919410798458,74.4421354382958));
#27180=CARTESIAN_POINT('Ctrl Pts',(4.83439740687436,-4.73825766587068,74.4503664605883));
#27181=CARTESIAN_POINT('Ctrl Pts',(4.95469679166588,-4.61233432069282,74.4585974828808));
#27182=CARTESIAN_POINT('Ctrl Pts',(5.07009529176753,-4.48178789462383,74.4668285051733));
#27183=CARTESIAN_POINT('Ctrl Pts',(5.18535602745416,-4.35139731678514,74.4750497011512));
#27184=CARTESIAN_POINT('Ctrl Pts',(5.29572729358617,-4.21639491369581,74.4832708971291));
#27185=CARTESIAN_POINT('Ctrl Pts',(5.40082100489027,-4.07718303159622,74.4914920931069));
#27186=CARTESIAN_POINT('Ctrl Pts',(5.50581032135212,-3.93810943562516,74.4997051225594));
#27187=CARTESIAN_POINT('Ctrl Pts',(5.60553230885063,-3.79483497208888,74.507918152012));
#27188=CARTESIAN_POINT('Ctrl Pts',(5.69963736852876,-3.64779698822051,74.5161311814645));
#27189=CARTESIAN_POINT('Ctrl Pts',(5.79366780682141,-3.50087559933768,74.5243376983274));
#27190=CARTESIAN_POINT('Ctrl Pts',(5.88208999633018,-3.3501969347092,74.5325442151903));
#27191=CARTESIAN_POINT('Ctrl Pts',(5.96459605500922,-3.1962294818377,74.5407507320531));
#27192=CARTESIAN_POINT('Ctrl Pts',(6.04705321906005,-3.04235327294858,74.5489523855812));
#27193=CARTESIAN_POINT('Ctrl Pts',(6.12360106782642,-2.88519247348388,74.5571540391092));
#27194=CARTESIAN_POINT('Ctrl Pts',(6.19397627050322,-2.72524255075453,74.5653556926372));
#27195=CARTESIAN_POINT('Ctrl Pts',(6.26433055714531,-2.56534016633423,74.5735549085727));
#27196=CARTESIAN_POINT('Ctrl Pts',(6.328515704314,-2.40265063592481,74.5817541245082));
#27197=CARTESIAN_POINT('Ctrl Pts',(6.38631528380104,-2.23769213608334,74.5899533404436));
#27198=CARTESIAN_POINT('Ctrl Pts',(6.44410682728185,-2.07275657079511,74.5981514164236));
#27199=CARTESIAN_POINT('Ctrl Pts',(6.49551445196764,-1.90555300229453,74.6063494924035));
#27200=CARTESIAN_POINT('Ctrl Pts',(6.54037064899189,-1.73661762452344,74.6145475683835));
#27201=CARTESIAN_POINT('Ctrl Pts',(6.58522875098158,-1.56767507235778,74.6227459925216));
#27202=CARTESIAN_POINT('Ctrl Pts',(6.62353477893024,-1.39700091089266,74.6309444166597));
#27203=CARTESIAN_POINT('Ctrl Pts',(6.65517166661411,-1.22514451714757,74.6391428407978));
#27204=CARTESIAN_POINT('Ctrl Pts',(6.68681563995494,-1.05324963303441,74.6473431011223));
#27205=CARTESIAN_POINT('Ctrl Pts',(6.71178743317195,-0.880172341777026,
74.6555433614467));
#27206=CARTESIAN_POINT('Ctrl Pts',(6.73002145600003,-0.706470241255208,
74.6637436217712));
#27207=CARTESIAN_POINT('Ctrl Pts',(6.74827260585864,-0.532604984132883,
74.671951584516));
#27208=CARTESIAN_POINT('Ctrl Pts',(6.75977330347216,-0.358114102214749,
74.6801595472608));
#27209=CARTESIAN_POINT('Ctrl Pts',(6.76450995960047,-0.183559272351012,
74.6883675100057));
#27210=CARTESIAN_POINT('Ctrl Pts',(6.76924888186432,-0.00892093106215111,
74.6965793996465));
#27211=CARTESIAN_POINT('Ctrl Pts',(6.76721731464129,0.165781060886628,74.7047912892873));
#27212=CARTESIAN_POINT('Ctrl Pts',(6.75845380030758,0.339987101384871,74.7130031789282));
#27213=CARTESIAN_POINT('Ctrl Pts',(6.74967823927898,0.514432612823238,74.7212263569774));
#27214=CARTESIAN_POINT('Ctrl Pts',(6.73415226842231,0.688380453082736,74.7294495350267));
#27215=CARTESIAN_POINT('Ctrl Pts',(6.71196625382715,0.861276963285036,74.737672713076));
#27216=CARTESIAN_POINT('Ctrl Pts',(6.69155672835339,1.02032922182219,74.7452374408982));
#27217=CARTESIAN_POINT('Ctrl Pts',(6.66551165699124,1.17849166295503,74.7528021687204));
#27218=CARTESIAN_POINT('Ctrl Pts',(6.63393905664814,1.33534324901066,74.7603668965425));
#27219=CARTESIAN_POINT('Ctrl Pts',(6.59784581407433,1.514653229249,74.7690147606185));
#27220=CARTESIAN_POINT('Ctrl Pts',(6.55444614030209,1.69265943061418,74.7776626246944));
#27221=CARTESIAN_POINT('Ctrl Pts',(6.50384734659557,1.86875859655059,74.7863104887704));
#27222=CARTESIAN_POINT('Ctrl Pts',(6.45331376152844,2.04463081662196,74.7949472080065));
#27223=CARTESIAN_POINT('Ctrl Pts',(6.39559964071816,2.21860061058749,74.8035839272427));
#27224=CARTESIAN_POINT('Ctrl Pts',(6.33086315836925,2.39007545278449,74.8122206464788));
#27225=CARTESIAN_POINT('Ctrl Pts',(6.26386469293625,2.56754186539624,74.8211591447444));
#27226=CARTESIAN_POINT('Ctrl Pts',(6.1893442944921,2.74233550284023,74.83009764301));
#27227=CARTESIAN_POINT('Ctrl Pts',(6.10753435341912,2.91381418793396,74.8390361412756));
#27228=CARTESIAN_POINT('Ctrl Pts',(6.02870710322883,3.07904096887162,74.8476487527733));
#27229=CARTESIAN_POINT('Ctrl Pts',(5.9431125609327,3.24118991098983,74.856261364271));
#27230=CARTESIAN_POINT('Ctrl Pts',(5.85100847465207,3.39970422677469,74.8648739757687));
#27231=CARTESIAN_POINT('Ctrl Pts',(5.75899218745423,3.55806743730355,74.8734783772138));
#27232=CARTESIAN_POINT('Ctrl Pts',(5.66047888052456,3.71280266671292,74.8820827786589));
#27233=CARTESIAN_POINT('Ctrl Pts',(5.55577284468835,3.86337638578272,74.890687180104));
#27234=CARTESIAN_POINT('Ctrl Pts',(5.45118572917823,4.01377909010987,74.8992818090635));
#27235=CARTESIAN_POINT('Ctrl Pts',(5.34042008979548,4.16002946362168,74.907876438023));
#27236=CARTESIAN_POINT('Ctrl Pts',(5.22382438185899,4.30162153466521,74.9164710669825));
#27237=CARTESIAN_POINT('Ctrl Pts',(5.21020600002388,4.31815949238614,74.917474919877));
#27238=CARTESIAN_POINT('Ctrl Pts',(5.19650813218543,4.33463393194399,74.9184787727716));
#27239=CARTESIAN_POINT('Ctrl Pts',(5.18273137234608,4.35104407264507,74.9194826256661));
#27240=CARTESIAN_POINT('Ctrl Pts',(5.0648095340086,4.49150626995506,74.9280750799241));
#27241=CARTESIAN_POINT('Ctrl Pts',(4.9412437964944,4.62708890396287,74.9366675341821));
#27242=CARTESIAN_POINT('Ctrl Pts',(4.81246774574751,4.7573567446787,74.9452599884402));
#27243=CARTESIAN_POINT('Ctrl Pts',(4.68348043585812,4.887838291842,74.9538665387549));
#27244=CARTESIAN_POINT('Ctrl Pts',(4.5492659386127,5.01298739568452,74.9624730890697));
#27245=CARTESIAN_POINT('Ctrl Pts',(4.41029378809865,5.1324066189906,74.9710796393844));
#27246=CARTESIAN_POINT('Ctrl Pts',(4.27120756351748,5.25192386651551,74.9796932543103));
#27247=CARTESIAN_POINT('Ctrl Pts',(4.1273561282961,5.36570165351677,74.9883068692362));
#27248=CARTESIAN_POINT('Ctrl Pts',(3.97924031196239,5.47338428576447,74.996920484162));
#27249=CARTESIAN_POINT('Ctrl Pts',(3.83087972288424,5.58124487181938,75.0055483337471));
#27250=CARTESIAN_POINT('Ctrl Pts',(3.67824091424832,5.68298998936973,75.0141761833322));
#27251=CARTESIAN_POINT('Ctrl Pts',(3.52185349553243,5.77830744734182,75.0228040329172));
#27252=CARTESIAN_POINT('Ctrl Pts',(3.38375706251097,5.86247662833286,75.0304227740035));
#27253=CARTESIAN_POINT('Ctrl Pts',(3.24273811510174,5.94163437395071,75.0380415150897));
#27254=CARTESIAN_POINT('Ctrl Pts',(3.09917575053257,6.0155962852664,75.0456602561759));
#27255=CARTESIAN_POINT('Ctrl Pts',(3.09917575053266,6.01559628526635,73.0456387728543));
#27256=CARTESIAN_POINT('Ctrl Pts',(2.9438003872764,6.0956441367509,73.0538420919943));
#27257=CARTESIAN_POINT('Ctrl Pts',(2.78538097620002,6.16963789028042,73.0620454111343));
#27258=CARTESIAN_POINT('Ctrl Pts',(2.62443417564996,6.23735795491012,73.0702487302742));
#27259=CARTESIAN_POINT('Ctrl Pts',(2.46263547823033,6.30543646413684,73.0784954698604));
#27260=CARTESIAN_POINT('Ctrl Pts',(2.29828289869186,6.36717454230061,73.0867422094466));
#27261=CARTESIAN_POINT('Ctrl Pts',(2.13191836530622,6.42239932452585,73.0949889490328));
#27262=CARTESIAN_POINT('Ctrl Pts',(1.96614521010812,6.47742779849382,73.1032063738257));
#27263=CARTESIAN_POINT('Ctrl Pts',(1.79837474182039,6.52598916190316,73.1114237986185));
#27264=CARTESIAN_POINT('Ctrl Pts',(1.62915472964356,6.56796344896042,73.1196412234114));
#27265=CARTESIAN_POINT('Ctrl Pts',(1.45902920573916,6.61016234425814,73.1279026203942));
#27266=CARTESIAN_POINT('Ctrl Pts',(1.28743894176949,6.64570340328322,73.1361640173771));
#27267=CARTESIAN_POINT('Ctrl Pts',(1.11494689210193,6.6745173928751,73.1444254143599));
#27268=CARTESIAN_POINT('Ctrl Pts',(0.942454842434423,6.70333138246697,73.1526868113428));
#27269=CARTESIAN_POINT('Ctrl Pts',(0.769061373292736,6.72541831514887,73.1609482083256));
#27270=CARTESIAN_POINT('Ctrl Pts',(0.595330304088778,6.7407618878754,73.1692096053084));
#27271=CARTESIAN_POINT('Ctrl Pts',(0.423858878567678,6.75590589349317,73.1773635499306));
#27272=CARTESIAN_POINT('Ctrl Pts',(0.251528364636971,6.76452759997373,73.1855174945528));
#27273=CARTESIAN_POINT('Ctrl Pts',(0.0788809832144273,6.76654023785325,
73.193671439175));
#27274=CARTESIAN_POINT('Ctrl Pts',(-0.0935557238406468,6.76855041979508,
73.2018154338801));
#27275=CARTESIAN_POINT('Ctrl Pts',(-0.266308167148405,6.76396758206107,
73.2099594285852));
#27276=CARTESIAN_POINT('Ctrl Pts',(-0.438827156451265,6.75275645397944,
73.2181034232904));
#27277=CARTESIAN_POINT('Ctrl Pts',(-0.611171938803255,6.74155664671789,
73.2262391943183));
#27278=CARTESIAN_POINT('Ctrl Pts',(-0.783283374325619,6.72374189737634,
73.2343749653461));
#27279=CARTESIAN_POINT('Ctrl Pts',(-0.954610411039097,6.69932891886462,
73.242510736374));
#27280=CARTESIAN_POINT('Ctrl Pts',(-1.12580048206165,6.67493545706511,73.2506400033409));
#27281=CARTESIAN_POINT('Ctrl Pts',(-1.29620704255985,6.64395432029271,73.2587692703078));
#27282=CARTESIAN_POINT('Ctrl Pts',(-1.46528231078734,6.60645417373751,73.2668985372747));
#27283=CARTESIAN_POINT('Ctrl Pts',(-1.63425796263297,6.56897612165513,73.2750230146105));
#27284=CARTESIAN_POINT('Ctrl Pts',(-1.80190352818636,6.52498678775252,73.2831474919462));
#27285=CARTESIAN_POINT('Ctrl Pts',(-1.967679599671,6.4746062423161,73.291271969282));
#27286=CARTESIAN_POINT('Ctrl Pts',(-2.13446028624788,6.42392038709735,73.2994456815434));
#27287=CARTESIAN_POINT('Ctrl Pts',(-2.29934837463323,6.36676565786725,73.3076193938048));
#27288=CARTESIAN_POINT('Ctrl Pts',(-2.46180767628279,6.30331594995802,73.3157931060662));
#27289=CARTESIAN_POINT('Ctrl Pts',(-2.62322832714176,6.24027189496378,73.3239145613462));
#27290=CARTESIAN_POINT('Ctrl Pts',(-2.78225082007247,6.1710132738783,73.3320360166262));
#27291=CARTESIAN_POINT('Ctrl Pts',(-2.93836730018601,6.09575972370939,73.3401574719062));
#27292=CARTESIAN_POINT('Ctrl Pts',(-3.09449584766683,6.02050035665153,73.348279554952));
#27293=CARTESIAN_POINT('Ctrl Pts',(-3.24771760519109,5.93924529635381,73.3564016379978));
#27294=CARTESIAN_POINT('Ctrl Pts',(-3.39754771358598,5.85226097623019,73.3645237210436));
#27295=CARTESIAN_POINT('Ctrl Pts',(-3.54741793373219,5.76525336910867,73.3726479784919));
#27296=CARTESIAN_POINT('Ctrl Pts',(-3.69389438039104,5.67251363174842,73.3807722359403));
#27297=CARTESIAN_POINT('Ctrl Pts',(-3.83651970643785,5.57435247738372,73.3888964933887));
#27298=CARTESIAN_POINT('Ctrl Pts',(-3.9806862301632,5.47513060156496,73.3971085409026));
#27299=CARTESIAN_POINT('Ctrl Pts',(-4.12091760154934,5.37036967537356,73.4053205884165));
#27300=CARTESIAN_POINT('Ctrl Pts',(-4.25677506424986,5.26043297195018,73.4135326359304));
#27301=CARTESIAN_POINT('Ctrl Pts',(-4.39139473239348,5.15149789957744,73.4216698636478));
#27302=CARTESIAN_POINT('Ctrl Pts',(-4.52171962839195,5.03748125929308,73.4298070913652));
#27303=CARTESIAN_POINT('Ctrl Pts',(-4.64735964561845,4.91877396556064,73.4379443190825));
#27304=CARTESIAN_POINT('Ctrl Pts',(-4.77473250617606,4.79842944551418,73.4461937764947));
#27305=CARTESIAN_POINT('Ctrl Pts',(-4.89729004003016,4.67326421850854,73.4544432339068));
#27306=CARTESIAN_POINT('Ctrl Pts',(-5.01466794408449,4.54372032706365,73.462692691319));
#27307=CARTESIAN_POINT('Ctrl Pts',(-5.13204584813878,4.41417643561881,73.4709421487311));
#27308=CARTESIAN_POINT('Ctrl Pts',(-5.24424392380754,4.28025421525507,73.4791916061433));
#27309=CARTESIAN_POINT('Ctrl Pts',(-5.35094358129603,4.14242583395126,73.4874410635555));
#27310=CARTESIAN_POINT('Ctrl Pts',(-5.45771720077136,4.00450191287571,73.4956962393202));
#27311=CARTESIAN_POINT('Ctrl Pts',(-5.55930636755762,3.86225133982876,73.5039514150849));
#27312=CARTESIAN_POINT('Ctrl Pts',(-5.65534280373195,3.71609832650822,73.5122065908496));
#27313=CARTESIAN_POINT('Ctrl Pts',(-5.75122614844573,3.57017829536785,73.5204486070577));
#27314=CARTESIAN_POINT('Ctrl Pts',(-5.84157421225403,3.4203685181075,73.5286906232659));
#27315=CARTESIAN_POINT('Ctrl Pts',(-5.92605926931867,3.26712573013685,73.536932639474));
#27316=CARTESIAN_POINT('Ctrl Pts',(-6.01046493164367,3.11402695190798,73.5451669102565));
#27317=CARTESIAN_POINT('Ctrl Pts',(-6.08901838818733,2.95750189607801,73.553401181039));
#27318=CARTESIAN_POINT('Ctrl Pts',(-6.16143498754642,2.79803643547378,73.5616354518214));
#27319=CARTESIAN_POINT('Ctrl Pts',(-6.23379639318408,2.63869251457578,73.569863446694));
#27320=CARTESIAN_POINT('Ctrl Pts',(-6.30003011072029,2.47641297433791,73.5780914415667));
#27321=CARTESIAN_POINT('Ctrl Pts',(-6.35989721255139,2.31170855554526,73.5863194364393));
#27322=CARTESIAN_POINT('Ctrl Pts',(-6.41972931476821,2.14710042655032,73.5945426210466));
#27323=CARTESIAN_POINT('Ctrl Pts',(-6.47320209467886,1.98007057609258,73.6027658056538));
#27324=CARTESIAN_POINT('Ctrl Pts',(-6.52012456255799,1.81115010110371,73.6109889902611));
#27325=CARTESIAN_POINT('Ctrl Pts',(-6.56702979874941,1.64229166004028,73.6192091550069));
#27326=CARTESIAN_POINT('Ctrl Pts',(-6.60738941932224,1.47154431938259,73.6274293197528));
#27327=CARTESIAN_POINT('Ctrl Pts',(-6.64106211326897,1.29945488867581,73.6356494844986));
#27328=CARTESIAN_POINT('Ctrl Pts',(-6.67472745511617,1.12740303199343,73.6438678544529));
#27329=CARTESIAN_POINT('Ctrl Pts',(-6.70170871299765,0.954010018103379,
73.6520862244071));
#27330=CARTESIAN_POINT('Ctrl Pts',(-6.72191555794214,0.779833464205928,
73.6603045943613));
#27331=CARTESIAN_POINT('Ctrl Pts',(-6.74212466589795,0.605637403873252,
73.6685238847098));
#27332=CARTESIAN_POINT('Ctrl Pts',(-6.75555780237903,0.43065798111306,73.6767431750583));
#27333=CARTESIAN_POINT('Ctrl Pts',(-6.76217640569453,0.255458916987017,
73.6849624654068));
#27334=CARTESIAN_POINT('Ctrl Pts',(-6.76545574736762,0.168652446696076,
73.6890349048745));
#27335=CARTESIAN_POINT('Ctrl Pts',(-6.76706296667692,0.0817921139574352,
73.6931073443422));
#27336=CARTESIAN_POINT('Ctrl Pts',(-6.7669981131445,-0.00505338488856453,
73.6971797838099));
#27337=CARTESIAN_POINT('',(-6.76699967339098,-0.00123438120911981,73.3028202161898));
#27338=CARTESIAN_POINT('Ctrl Pts',(3.09917575053262,6.01559628526637,72.6513920151221));
#27339=CARTESIAN_POINT('Ctrl Pts',(2.93382384459274,6.10078395293755,72.6601414630345));
#27340=CARTESIAN_POINT('Ctrl Pts',(2.76495772122998,6.17915010267043,72.6688909109469));
#27341=CARTESIAN_POINT('Ctrl Pts',(2.59315093316731,6.25042856433169,72.6776403588593));
#27342=CARTESIAN_POINT('Ctrl Pts',(2.42134553245636,6.32170645041444,72.6863897361193));
#27343=CARTESIAN_POINT('Ctrl Pts',(2.24659977927608,6.38589665313451,72.6951391133793));
#27344=CARTESIAN_POINT('Ctrl Pts',(2.06950718689935,6.4427811543907,72.7038884906393));
#27345=CARTESIAN_POINT('Ctrl Pts',(1.89241596572876,6.4996652151972,72.712637800154));
#27346=CARTESIAN_POINT('Ctrl Pts',(1.71297821457211,6.54924360009543,72.7213871096686));
#27347=CARTESIAN_POINT('Ctrl Pts',(1.53180337335856,6.59134792173553,72.7301364191833));
#27348=CARTESIAN_POINT('Ctrl Pts',(1.35062987477787,6.63345193135304,72.7388856638594));
#27349=CARTESIAN_POINT('Ctrl Pts',(1.16771959102949,6.66808192368239,72.7476349085355));
#27350=CARTESIAN_POINT('Ctrl Pts',(0.983693746906737,6.6951202836317,72.7563841532117));
#27351=CARTESIAN_POINT('Ctrl Pts',(0.799669205419682,6.72215845218869,72.7651333359559));
#27352=CARTESIAN_POINT('Ctrl Pts',(0.614529402873204,6.74160505424582,72.7738825187));
#27353=CARTESIAN_POINT('Ctrl Pts',(0.428903127362894,6.75339404354124,72.7826317014442));
#27354=CARTESIAN_POINT('Ctrl Pts',(0.243278104163466,6.76518295330332,72.7913808251628));
#27355=CARTESIAN_POINT('Ctrl Pts',(0.0571669005386472,6.76931433552276,
72.8001299488814));
#27356=CARTESIAN_POINT('Ctrl Pts',(-0.128798404778041,6.76577415902472,
72.8088790726));
#27357=CARTESIAN_POINT('Ctrl Pts',(-0.314762517259671,6.76223400523439,
72.8176281401992));
#27358=CARTESIAN_POINT('Ctrl Pts',(-0.500580446820127,6.75102239665084,
72.8263772077985));
#27359=CARTESIAN_POINT('Ctrl Pts',(-0.68562111884327,6.73217741012491,72.8351262753977));
#27360=CARTESIAN_POINT('Ctrl Pts',(-0.870660665415115,6.71333253821764,
72.8438752897835));
#27361=CARTESIAN_POINT('Ctrl Pts',(-1.05492267885546,6.68685441030603,72.8526243041693));
#27362=CARTESIAN_POINT('Ctrl Pts',(-1.23778137635308,6.65283295028167,72.861373318555));
#27363=CARTESIAN_POINT('Ctrl Pts',(-1.42999922978902,6.61707018861854,72.8705701289224));
#27364=CARTESIAN_POINT('Ctrl Pts',(-1.62066601233749,6.572971729344,72.8797669392898));
#27365=CARTESIAN_POINT('Ctrl Pts',(-1.80906628500437,6.5207030431128,72.8889637496572));
#27366=CARTESIAN_POINT('Ctrl Pts',(-1.98831342545581,6.47097374915014,72.897713747395));
#27367=CARTESIAN_POINT('Ctrl Pts',(-2.16550875896756,6.4138493398951,72.9064637451327));
#27368=CARTESIAN_POINT('Ctrl Pts',(-2.34005036714066,6.34952386240456,72.9152137428705));
#27369=CARTESIAN_POINT('Ctrl Pts',(-2.51458843547144,6.28519968948574,72.9239635631513));
#27370=CARTESIAN_POINT('Ctrl Pts',(-2.6864726171811,6.21367483971075,72.9327133834322));
#27371=CARTESIAN_POINT('Ctrl Pts',(-2.85511905908785,6.13519226743819,72.9414632037131));
#27372=CARTESIAN_POINT('Ctrl Pts',(-3.02376230488932,6.05671118252913,72.9502128581716));
#27373=CARTESIAN_POINT('Ctrl Pts',(-3.18916767379947,5.9712727599261,72.9589625126302));
#27374=CARTESIAN_POINT('Ctrl Pts',(-3.35077334102824,5.87916720437975,72.9677121670887));
#27375=CARTESIAN_POINT('Ctrl Pts',(-3.51237616037403,5.78706327195622,72.9764616673571));
#27376=CARTESIAN_POINT('Ctrl Pts',(-3.67017916302332,5.68829258362278,72.9852111676256));
#27377=CARTESIAN_POINT('Ctrl Pts',(-3.82364636566492,5.58319061741022,72.993960667894));
#27378=CARTESIAN_POINT('Ctrl Pts',(-3.97711106778829,5.4780903636768,73.0027100256024));
#27379=CARTESIAN_POINT('Ctrl Pts',(-4.12623987481959,5.36665920043201,73.0114593833109));
#27380=CARTESIAN_POINT('Ctrl Pts',(-4.27052628213962,5.24927559512308,73.0202087410193));
#27381=CARTESIAN_POINT('Ctrl Pts',(-4.41481053025007,5.13189374643011,73.0289579677958));
#27382=CARTESIAN_POINT('Ctrl Pts',(-4.55425230136555,5.0085598147733,73.0377071945723));
#27383=CARTESIAN_POINT('Ctrl Pts',(-4.6883780063057,4.87969268192056,73.0464564213489));
#27384=CARTESIAN_POINT('Ctrl Pts',(-4.82250188228922,4.75082730631782,73.0552055288197));
#27385=CARTESIAN_POINT('Ctrl Pts',(-4.95130963053,4.6164290790349,73.0639546362906));
#27386=CARTESIAN_POINT('Ctrl Pts',(-5.07436379033406,4.47695444731646,73.0727037437614));
#27387=CARTESIAN_POINT('Ctrl Pts',(-5.19741643562834,4.33748153220551,73.0814527435511));
#27388=CARTESIAN_POINT('Ctrl Pts',(-5.31471544462792,4.19293255254564,73.0902017433409));
#27389=CARTESIAN_POINT('Ctrl Pts',(-5.42586245275638,4.04379841779589,73.0989507431306));
#27390=CARTESIAN_POINT('Ctrl Pts',(-5.53702160019161,3.89464799484331,73.1077006984728));
#27391=CARTESIAN_POINT('Ctrl Pts',(-5.64202723081257,3.74091164443841,73.1164506538149));
#27392=CARTESIAN_POINT('Ctrl Pts',(-5.74052265232971,3.58311159163227,73.1252006091571));
#27393=CARTESIAN_POINT('Ctrl Pts',(-5.83901427066928,3.42531763191766,73.1339502266395));
#27394=CARTESIAN_POINT('Ctrl Pts',(-5.93099603115756,3.26346052695584,73.142699844122));
#27395=CARTESIAN_POINT('Ctrl Pts',(-6.01615550622775,3.09809004467036,73.1514494616045));
#27396=CARTESIAN_POINT('Ctrl Pts',(-6.10131214578824,2.93272506863777,73.1601987877556));
#27397=CARTESIAN_POINT('Ctrl Pts',(-6.17964682328776,2.76384720416832,73.1689481139067));
#27398=CARTESIAN_POINT('Ctrl Pts',(-6.25089348288594,2.5920300279152,73.1776974400578));
#27399=CARTESIAN_POINT('Ctrl Pts',(-6.32213814889374,2.42021765936918,73.1864465213893));
#27400=CARTESIAN_POINT('Ctrl Pts',(-6.38629508412638,2.24546640831769,73.1951956027209));
#27401=CARTESIAN_POINT('Ctrl Pts',(-6.44314639819872,2.06836976659854,73.2039446840525));
#27402=CARTESIAN_POINT('Ctrl Pts',(-6.50000285283759,1.89125711158076,73.2126945564869));
#27403=CARTESIAN_POINT('Ctrl Pts',(-6.54955227673305,1.71179891440045,73.2214444289213));
#27404=CARTESIAN_POINT('Ctrl Pts',(-6.59162635926436,1.53060476278209,73.2301943013557));
#27405=CARTESIAN_POINT('Ctrl Pts',(-6.6336975205524,1.34942319164483,73.2389435662782));
#27406=CARTESIAN_POINT('Ctrl Pts',(-6.66829431424289,1.166506186425,73.2476928312007));
#27407=CARTESIAN_POINT('Ctrl Pts',(-6.69529923745446,0.982474997616606,
73.2564420961232));
#27408=CARTESIAN_POINT('Ctrl Pts',(-6.72230554731467,0.798434359175797,
73.2651918103029));
#27409=CARTESIAN_POINT('Ctrl Pts',(-6.74171916496721,0.6132797062384,73.2739415244826));
#27410=CARTESIAN_POINT('Ctrl Pts',(-6.75347414817287,0.427639953653452,
73.2826912386623));
#27411=CARTESIAN_POINT('Ctrl Pts',(-6.76248837758744,0.285283364197985,
73.2894008978381));
#27412=CARTESIAN_POINT('Ctrl Pts',(-6.76699999999992,0.142641701105874,
73.296110557014));
#27413=CARTESIAN_POINT('Ctrl Pts',(-6.767,3.66893179809862E-12,73.3028202161898));
#27414=CARTESIAN_POINT('Ctrl Pts',(-6.76699905248981,-0.00358100572350501,
73.3028202161898));
#27415=CARTESIAN_POINT('Ctrl Pts',(-6.7668945298339,-0.201096667011066,
73.3120892241327));
#27416=CARTESIAN_POINT('Ctrl Pts',(-6.7581382485434,-0.398339799715601,
73.3213582320757));
#27417=CARTESIAN_POINT('Ctrl Pts',(-6.74082625458302,-0.594601047362251,
73.3306272400186));
#27418=CARTESIAN_POINT('Ctrl Pts',(-6.72346196364603,-0.791455171248329,
73.3399242482654));
#27419=CARTESIAN_POINT('Ctrl Pts',(-6.69749027576094,-0.987321300288637,
73.3492212565122));
#27420=CARTESIAN_POINT('Ctrl Pts',(-6.66305861989671,-1.18149855176388,
73.358518264759));
#27421=CARTESIAN_POINT('Ctrl Pts',(-6.62848720793987,-1.37646395743209,
73.3678530090227));
#27422=CARTESIAN_POINT('Ctrl Pts',(-6.58538708590094,-1.56972658068534,
73.3771877532863));
#27423=CARTESIAN_POINT('Ctrl Pts',(-6.53395714227279,-1.76059451974109,
73.3865224975499));
#27424=CARTESIAN_POINT('Ctrl Pts',(-6.48620301544764,-1.93782068655211,
73.3951900660907));
#27425=CARTESIAN_POINT('Ctrl Pts',(-6.4312677765939,-2.11298232444131,73.4038576346315));
#27426=CARTESIAN_POINT('Ctrl Pts',(-6.3693478532621,-2.28554083843309,73.4125252031723));
#27427=CARTESIAN_POINT('Ctrl Pts',(-6.31058250118312,-2.44930818960721,
73.4207511939287));
#27428=CARTESIAN_POINT('Ctrl Pts',(-6.24541983593963,-2.61102258676869,
73.4289771846852));
#27429=CARTESIAN_POINT('Ctrl Pts',(-6.17402305823175,-2.77014950434496,
73.4372031754416));
#27430=CARTESIAN_POINT('Ctrl Pts',(-6.10270113114897,-2.92910959717604,
73.4454205422718));
#27431=CARTESIAN_POINT('Ctrl Pts',(-6.02515825204532,-3.08548728810339,
73.4536379091019));
#27432=CARTESIAN_POINT('Ctrl Pts',(-5.94160691409611,-3.23876462225418,
73.4618552759321));
#27433=CARTESIAN_POINT('Ctrl Pts',(-5.85812645102926,-3.39191193439344,
73.4700656721389));
#27434=CARTESIAN_POINT('Ctrl Pts',(-5.76864785070083,-3.54196381487223,
73.4782760683457));
#27435=CARTESIAN_POINT('Ctrl Pts',(-5.67343110477985,-3.68842357916176,
73.4864864645525));
#27436=CARTESIAN_POINT('Ctrl Pts',(-5.57827608214668,-3.83478840239765,
73.4946915384534));
#27437=CARTESIAN_POINT('Ctrl Pts',(-5.4773905178737,-3.97756544843949,73.5028966123542));
#27438=CARTESIAN_POINT('Ctrl Pts',(-5.37107965378552,-4.11628380371073,
73.5111016862551));
#27439=CARTESIAN_POINT('Ctrl Pts',(-5.264816442573,-4.25493997974382,73.5193030823065));
#27440=CARTESIAN_POINT('Ctrl Pts',(-5.15313299397265,-4.38954080574244,
73.5275044783578));
#27441=CARTESIAN_POINT('Ctrl Pts',(-5.03637711933686,-4.51964539668989,
73.5357058744091));
#27442=CARTESIAN_POINT('Ctrl Pts',(-4.91963039055831,-4.6497397961329,73.5439066280191));
#27443=CARTESIAN_POINT('Ctrl Pts',(-4.79781225981491,-4.77533838980424,
73.5521073816291));
#27444=CARTESIAN_POINT('Ctrl Pts',(-4.67131022207002,-4.89603408987153,
73.5603081352391));
#27445=CARTESIAN_POINT('Ctrl Pts',(-4.54480882726469,-5.01672917650965,
73.5685088471693));
#27446=CARTESIAN_POINT('Ctrl Pts',(-4.41362383142904,-5.13252117101907,
73.5767095590994));
#27447=CARTESIAN_POINT('Ctrl Pts',(-4.27817882947111,-5.2430406161945,73.5849102710296));
#27448=CARTESIAN_POINT('Ctrl Pts',(-4.14270996986308,-5.35357952856485,
73.5931124274554));
#27449=CARTESIAN_POINT('Ctrl Pts',(-4.00297988682076,-5.4588438147124,73.6013145838811));
#27450=CARTESIAN_POINT('Ctrl Pts',(-3.8594444509964,-5.55850497253291,73.6095167403069));
#27451=CARTESIAN_POINT('Ctrl Pts',(-3.71585771994449,-5.65820174623976,
73.6177218279356));
#27452=CARTESIAN_POINT('Ctrl Pts',(-3.56846322126033,-5.75229119848255,
73.6259269155642));
#27453=CARTESIAN_POINT('Ctrl Pts',(-3.4177449647962,-5.84048870862792,73.6341320031929));
#27454=CARTESIAN_POINT('Ctrl Pts',(-3.26685453089381,-5.92878697379604,
73.642346464145));
#27455=CARTESIAN_POINT('Ctrl Pts',(-3.11263306310723,-6.01117966866163,
73.6505609250971));
#27456=CARTESIAN_POINT('Ctrl Pts',(-2.95558922926776,-6.08742813574308,
73.6587753860492));
#27457=CARTESIAN_POINT('Ctrl Pts',(-2.79845235217987,-6.16372177750531,
73.6669947137962));
#27458=CARTESIAN_POINT('Ctrl Pts',(-2.63849010344047,-6.23386379139131,
73.6752140415432));
#27459=CARTESIAN_POINT('Ctrl Pts',(-2.47623009019335,-6.29766413366266,
73.6834333692902));
#27460=CARTESIAN_POINT('Ctrl Pts',(-2.31371866493584,-6.36156333067951,
73.6916654323851));
#27461=CARTESIAN_POINT('Ctrl Pts',(-2.14890269852081,-6.41910110179752,
73.69989749548));
#27462=CARTESIAN_POINT('Ctrl Pts',(-1.98232516376679,-6.47013724314229,
73.7081295585748));
#27463=CARTESIAN_POINT('Ctrl Pts',(-1.83259280338129,-6.51601234820857,
73.7155291532432));
#27464=CARTESIAN_POINT('Ctrl Pts',(-1.68143748548776,-6.55663493444886,
73.7229287479116));
#27465=CARTESIAN_POINT('Ctrl Pts',(-1.52925889565088,-6.5919387307584,73.73032834258));
#27466=CARTESIAN_POINT('Ctrl Pts',(-1.3615344729331,-6.63084899311601,73.7384838442536));
#27467=CARTESIAN_POINT('Ctrl Pts',(-1.19205048369878,-6.66341720214219,
73.7466393459272));
#27468=CARTESIAN_POINT('Ctrl Pts',(-1.02133203116545,-6.68948203391828,
73.7547948476007));
#27469=CARTESIAN_POINT('Ctrl Pts',(-0.85082136254669,-6.71551514180807,
73.7629404230945));
#27470=CARTESIAN_POINT('Ctrl Pts',(-0.679079578733357,-6.73506057376915,
73.7710859985883));
#27471=CARTESIAN_POINT('Ctrl Pts',(-0.50664583599944,-6.7480070388867,73.779231574082));
#27472=CARTESIAN_POINT('Ctrl Pts',(-0.334385706404295,-6.76094046898912,
73.7873689482869));
#27473=CARTESIAN_POINT('Ctrl Pts',(-0.161435366625639,-6.76728813231959,
73.7955063224918));
#27474=CARTESIAN_POINT('Ctrl Pts',(0.0116569628525796,-6.76698995973964,
73.8036436966968));
#27475=CARTESIAN_POINT('Ctrl Pts',(0.184611391120607,-6.76669202471129,
73.8117745879238));
#27476=CARTESIAN_POINT('Ctrl Pts',(0.357707220051187,-6.75975879677122,
73.8199054791507));
#27477=CARTESIAN_POINT('Ctrl Pts',(0.53039224945409,-6.74618211003224,73.8280363703777));
#27478=CARTESIAN_POINT('Ctrl Pts',(0.702975976759167,-6.73261338777549,
73.8361624917857));
#27479=CARTESIAN_POINT('Ctrl Pts',(0.875149020997245,-6.71240899658853,
73.8442886131937));
#27480=CARTESIAN_POINT('Ctrl Pts',(1.04636033042912,-6.68561284093719,73.8524147346016));
#27481=CARTESIAN_POINT('Ctrl Pts',(1.21817723480565,-6.65872190406812,73.8605695990761));
#27482=CARTESIAN_POINT('Ctrl Pts',(1.38902521657901,-6.62519249248478,73.8687244635505));
#27483=CARTESIAN_POINT('Ctrl Pts',(1.55835308561361,-6.5851214613368,73.8768793280249));
#27484=CARTESIAN_POINT('Ctrl Pts',(1.72702209283733,-6.5452063482447,73.8850024615811));
#27485=CARTESIAN_POINT('Ctrl Pts',(1.89418244129293,-6.49880053328504,73.8931255951372));
#27486=CARTESIAN_POINT('Ctrl Pts',(2.05930044737118,-6.44605078070728,73.9012487286933));
#27487=CARTESIAN_POINT('Ctrl Pts',(2.22443141676527,-6.39329688677801,73.9093724999918));
#27488=CARTESIAN_POINT('Ctrl Pts',(2.38751937590625,-6.33419817444008,73.9174962712903));
#27489=CARTESIAN_POINT('Ctrl Pts',(2.54804689179495,-6.26895095189092,73.9256200425888));
#27490=CARTESIAN_POINT('Ctrl Pts',(2.70861755005445,-6.20368619390647,73.9337459971813));
#27491=CARTESIAN_POINT('Ctrl Pts',(2.86662605611284,-6.13226977309168,73.9418719517737));
#27492=CARTESIAN_POINT('Ctrl Pts',(3.02157604846565,-6.05494567963568,73.9499979063661));
#27493=CARTESIAN_POINT('Ctrl Pts',(3.17751461768377,-5.97712826050239,73.9581757043346));
#27494=CARTESIAN_POINT('Ctrl Pts',(3.33035517554299,-5.89332769382333,73.9663535023031));
#27495=CARTESIAN_POINT('Ctrl Pts',(3.47961871874631,-5.80383860665942,73.9745313002715));
#27496=CARTESIAN_POINT('Ctrl Pts',(3.62817207918886,-5.71477530067164,73.9826701889992));
#27497=CARTESIAN_POINT('Ctrl Pts',(3.77318211615054,-5.62007773840826,73.9908090777269));
#27498=CARTESIAN_POINT('Ctrl Pts',(3.91420772899504,-5.52007851885057,73.9989479664547));
#27499=CARTESIAN_POINT('Ctrl Pts',(4.0562446346044,-5.41936220624013,74.0071452190435));
#27500=CARTESIAN_POINT('Ctrl Pts',(4.19423945743656,-5.31326814462259,74.0153424716324));
#27501=CARTESIAN_POINT('Ctrl Pts',(4.32777758708844,-5.20217552151934,74.0235397242212));
#27502=CARTESIAN_POINT('Ctrl Pts',(4.46131571674026,-5.09108289841613,74.03173697681));
#27503=CARTESIAN_POINT('Ctrl Pts',(4.59039691733635,-4.97499200813957,74.0399342293989));
#27504=CARTESIAN_POINT('Ctrl Pts',(4.71464653915873,-4.85431735785771,74.0481314819877));
#27505=CARTESIAN_POINT('Ctrl Pts',(4.83933408596642,-4.73321738278469,74.0563576262679));
#27506=CARTESIAN_POINT('Ctrl Pts',(4.95952710313247,-4.6071409550378,74.064583770548));
#27507=CARTESIAN_POINT('Ctrl Pts',(5.07480476132472,-4.47645458308648,74.0728099148282));
#27508=CARTESIAN_POINT('Ctrl Pts',(5.18995290982151,-4.34591503188515,74.0810268173744));
#27509=CARTESIAN_POINT('Ctrl Pts',(5.30019646045681,-4.21077611595185,74.0892437199207));
#27510=CARTESIAN_POINT('Ctrl Pts',(5.40514976365807,-4.07144262300565,74.097460622467));
#27511=CARTESIAN_POINT('Ctrl Pts',(5.51000622205972,-3.93223769889713,74.1056699429338));
#27512=CARTESIAN_POINT('Ctrl Pts',(5.60958194035312,-3.78884619070722,74.1138792634006));
#27513=CARTESIAN_POINT('Ctrl Pts',(5.7035300177456,-3.64170761273813,74.1220885838675));
#27514=CARTESIAN_POINT('Ctrl Pts',(5.79741025624129,-3.49467528195454,74.1302919764723));
#27515=CARTESIAN_POINT('Ctrl Pts',(5.88567075572104,-3.34390157177274,74.138495369077));
#27516=CARTESIAN_POINT('Ctrl Pts',(5.96800656585284,-3.18985683533563,74.1466987616818));
#27517=CARTESIAN_POINT('Ctrl Pts',(6.05029943927973,-3.03589243057171,74.1548978763588));
#27518=CARTESIAN_POINT('Ctrl Pts',(6.12667360978057,-2.87866071332104,74.1630969910359));
#27519=CARTESIAN_POINT('Ctrl Pts',(6.19686888050713,-2.71865869093608,74.1712961057129));
#27520=CARTESIAN_POINT('Ctrl Pts',(6.26705092974843,-2.55868680540164,74.1794936760626));
#27521=CARTESIAN_POINT('Ctrl Pts',(6.33105624777745,-2.3959459796825,74.1876912464123));
#27522=CARTESIAN_POINT('Ctrl Pts',(6.38867168667037,-2.2309556427541,74.195888816762));
#27523=CARTESIAN_POINT('Ctrl Pts',(6.44628296930304,-2.0659772078921,74.2040857957557));
#27524=CARTESIAN_POINT('Ctrl Pts',(6.49750517172593,-1.89874992334064,74.2122827747494));
#27525=CARTESIAN_POINT('Ctrl Pts',(6.54217420807248,-1.72981086573973,74.2204797537431));
#27526=CARTESIAN_POINT('Ctrl Pts',(6.58684814096861,-1.56085328930478,74.2286776312768));
#27527=CARTESIAN_POINT('Ctrl Pts',(6.6249673849238,-1.39018391282502,74.2368755088104));
#27528=CARTESIAN_POINT('Ctrl Pts',(6.65641840003207,-1.21835261058305,74.2450733863441));
#27529=CARTESIAN_POINT('Ctrl Pts',(6.6878785791955,-1.04647124091,74.2532736525384));
#27530=CARTESIAN_POINT('Ctrl Pts',(6.71266659481192,-0.873427623847161,
74.2614739187327));
#27531=CARTESIAN_POINT('Ctrl Pts',(6.73072044516196,-0.699779457457002,
74.269674184927));
#27532=CARTESIAN_POINT('Ctrl Pts',(6.74879311057494,-0.525950321294897,
74.277882997139));
#27533=CARTESIAN_POINT('Ctrl Pts',(6.76011755247661,-0.35151573431645,74.286091809351));
#27534=CARTESIAN_POINT('Ctrl Pts',(6.76468379567344,-0.177037127612258,
74.294300621563));
#27535=CARTESIAN_POINT('Ctrl Pts',(6.76925248981363,-0.00246486904519361,
74.3025138398771));
#27536=CARTESIAN_POINT('Ctrl Pts',(6.76705575824902,0.172151098040432,74.3107270581912));
#27537=CARTESIAN_POINT('Ctrl Pts',(6.75813573864054,0.346251842030471,74.3189402765053));
#27538=CARTESIAN_POINT('Ctrl Pts',(6.74920267048595,0.520607267252796,74.3271655094295));
#27539=CARTESIAN_POINT('Ctrl Pts',(6.73352669172724,0.694445605969707,74.3353907423537));
#27540=CARTESIAN_POINT('Ctrl Pts',(6.71120171431555,0.867214246751078,74.343615975278));
#27541=CARTESIAN_POINT('Ctrl Pts',(6.69100924580547,1.02347981755876,74.3510555239838));
#27542=CARTESIAN_POINT('Ctrl Pts',(6.6653780545573,1.17887021819433,74.3584950726896));
#27543=CARTESIAN_POINT('Ctrl Pts',(6.63441304834135,1.33298631050661,74.3659346213954));
#27544=CARTESIAN_POINT('Ctrl Pts',(6.60017157051125,1.50340974660639,74.3741613641998));
#27545=CARTESIAN_POINT('Ctrl Pts',(6.55931130238019,1.67275119429102,74.3823881070042));
#27546=CARTESIAN_POINT('Ctrl Pts',(6.51191234648319,1.84045825590252,74.3906148498087));
#27547=CARTESIAN_POINT('Ctrl Pts',(6.46456732214236,2.00797449679571,74.3988322320474));
#27548=CARTESIAN_POINT('Ctrl Pts',(6.41069852222834,2.17385971274366,74.4070496142861));
#27549=CARTESIAN_POINT('Ctrl Pts',(6.35043729118156,2.33757036488117,74.4152669965248));
#27550=CARTESIAN_POINT('Ctrl Pts',(6.29023253077494,2.50112760419973,74.4234766782763));
#27551=CARTESIAN_POINT('Ctrl Pts',(6.22364739306416,2.66251400373133,74.4316863600279));
#27552=CARTESIAN_POINT('Ctrl Pts',(6.15086340626104,2.82119980815234,74.4398960417794));
#27553=CARTESIAN_POINT('Ctrl Pts',(6.07813302054994,2.97976874988449,74.448099677587));
#27554=CARTESIAN_POINT('Ctrl Pts',(5.99921302826485,3.13564073349938,74.4563033133946));
#27555=CARTESIAN_POINT('Ctrl Pts',(5.91433360269426,3.28830458383064,74.4645069492022));
#27556=CARTESIAN_POINT('Ctrl Pts',(5.82949891879122,3.4408879619486,74.4727062607068));
#27557=CARTESIAN_POINT('Ctrl Pts',(5.73871123386279,3.5902662631069,74.4809055722115));
#27558=CARTESIAN_POINT('Ctrl Pts',(5.64224736972041,3.73595150114173,74.4891048837162));
#27559=CARTESIAN_POINT('Ctrl Pts',(5.54580997815359,3.88159675878073,74.497301945084));
#27560=CARTESIAN_POINT('Ctrl Pts',(5.44369970712473,4.02355067278505,74.5054990064518));
#27561=CARTESIAN_POINT('Ctrl Pts',(5.33623763147803,4.16135277769114,74.5136960678197));
#27562=CARTESIAN_POINT('Ctrl Pts',(5.22878551558251,4.29914211088527,74.5218923694712));
#27563=CARTESIAN_POINT('Ctrl Pts',(5.11598280375026,4.43278011886775,74.5300886711228));
#27564=CARTESIAN_POINT('Ctrl Pts',(4.99819194940795,4.56183803273128,74.5382849727743));
#27565=CARTESIAN_POINT('Ctrl Pts',(4.88039060421225,4.69090744093078,74.5464820044163));
#27566=CARTESIAN_POINT('Ctrl Pts',(4.75760047408038,4.81539567833841,74.5546790360583));
#27567=CARTESIAN_POINT('Ctrl Pts',(4.63022211397191,4.93490954073988,74.5628760677003));
#27568=CARTESIAN_POINT('Ctrl Pts',(4.50275829987343,5.05450358109619,74.5710785984637));
#27569=CARTESIAN_POINT('Ctrl Pts',(4.37070036836415,5.16911633407734,74.579281129227));
#27570=CARTESIAN_POINT('Ctrl Pts',(4.23448385801849,5.27839326463848,74.5874836599903));
#27571=CARTESIAN_POINT('Ctrl Pts',(4.09821754742812,5.38771014643512,74.5956891895681));
#27572=CARTESIAN_POINT('Ctrl Pts',(3.95778991377851,5.49168710161214,74.6038947191459));
#27573=CARTESIAN_POINT('Ctrl Pts',(3.81366689612691,5.59001196826856,74.6121002487237));
#27574=CARTESIAN_POINT('Ctrl Pts',(3.66939428475425,5.68843889206281,74.6203142953012));
#27575=CARTESIAN_POINT('Ctrl Pts',(3.5214189293987,5.78120181515348,74.6285283418787));
#27576=CARTESIAN_POINT('Ctrl Pts',(3.37023360463566,5.86803326934881,74.6367423884562));
#27577=CARTESIAN_POINT('Ctrl Pts',(3.28096469730114,5.91930378155252,74.6415924555108));
#27578=CARTESIAN_POINT('Ctrl Pts',(3.19057711381039,5.9685072062785,74.6464425225654));
#27579=CARTESIAN_POINT('Ctrl Pts',(3.09917575053252,6.01559628526642,74.65129258962));
#27580=CARTESIAN_POINT('Origin',(0.,0.,-3.69717978381041));
#27581=CARTESIAN_POINT('',(3.09917575053268,6.01559628526634,77.0459357433347));
#27582=CARTESIAN_POINT('',(3.09917575053257,6.0155962852664,76.6515786160344));
#27583=CARTESIAN_POINT('',(3.09917575053259,6.01559628526639,-3.69717978381041));
#27584=CARTESIAN_POINT('',(-6.7669993834644,-0.0028886315797119,75.6971797837722));
#27585=CARTESIAN_POINT('Ctrl Pts',(-6.76699938346406,-0.00288863237634982,
75.6971797838099));
#27586=CARTESIAN_POINT('Ctrl Pts',(-6.76694558422489,-0.12892039096998,
75.7031402796343));
#27587=CARTESIAN_POINT('Ctrl Pts',(-6.76337111739666,-0.254880375023853,
75.7091007754587));
#27588=CARTESIAN_POINT('Ctrl Pts',(-6.75628652671121,-0.380632853259699,
75.7150612712831));
#27589=CARTESIAN_POINT('Ctrl Pts',(-6.74651377909609,-0.554100493994067,
75.7232834006818));
#27590=CARTESIAN_POINT('Ctrl Pts',(-6.73004235460007,-0.727434860285483,
75.7315055300805));
#27591=CARTESIAN_POINT('Ctrl Pts',(-6.70687319369236,-0.900078309776879,
75.7397276594792));
#27592=CARTESIAN_POINT('Ctrl Pts',(-6.68373002776888,-1.07252805938576,
75.7479405639377));
#27593=CARTESIAN_POINT('Ctrl Pts',(-6.65390413616611,-1.2442880832005,75.7561534683962));
#27594=CARTESIAN_POINT('Ctrl Pts',(-6.61744842796308,-1.41480221347329,
75.7643663728547));
#27595=CARTESIAN_POINT('Ctrl Pts',(-6.58102628549849,-1.5851593468592,75.772571715474));
#27596=CARTESIAN_POINT('Ctrl Pts',(-6.53798655766103,-1.75427252235299,
75.7807770580933));
#27597=CARTESIAN_POINT('Ctrl Pts',(-6.48843377827388,-1.92159207558593,
75.7889824007127));
#27598=CARTESIAN_POINT('Ctrl Pts',(-6.43891665472678,-2.08879123356953,
75.7971818391549));
#27599=CARTESIAN_POINT('Ctrl Pts',(-6.38289591568522,-2.25419899708455,
75.8053812775971));
#27600=CARTESIAN_POINT('Ctrl Pts',(-6.32052688106321,-2.41727717603038,
75.8135807160394));
#27601=CARTESIAN_POINT('Ctrl Pts',(-6.25819018009885,-2.58027081119515,
75.821775903689));
#27602=CARTESIAN_POINT('Ctrl Pts',(-6.18951186787573,-2.74093693321145,
75.8299710913385));
#27603=CARTESIAN_POINT('Ctrl Pts',(-6.1146967252889,-2.89875369042305,75.8381662789881));
#27604=CARTESIAN_POINT('Ctrl Pts',(-6.03989512918573,-3.05654187237502,
75.8463599827673));
#27605=CARTESIAN_POINT('Ctrl Pts',(-5.95895906378854,-3.21148139032135,
75.8545536865464));
#27606=CARTESIAN_POINT('Ctrl Pts',(-5.87214107893503,-3.36307123758683,
75.8627473903256));
#27607=CARTESIAN_POINT('Ctrl Pts',(-5.78532900198887,-3.51465076926186,
75.8709405365286));
#27608=CARTESIAN_POINT('Ctrl Pts',(-5.69263598035683,-3.6628807721734,75.8791336827315));
#27609=CARTESIAN_POINT('Ctrl Pts',(-5.59436004092235,-3.80728574348331,
75.8873268289345));
#27610=CARTESIAN_POINT('Ctrl Pts',(-5.49607288063054,-3.95170720252756,
75.8955209106067));
#27611=CARTESIAN_POINT('Ctrl Pts',(-5.39220173462517,-4.09230246297833,
75.903714992279));
#27612=CARTESIAN_POINT('Ctrl Pts',(-5.28308741197602,-4.22862582849565,
75.9119090739513));
#27613=CARTESIAN_POINT('Ctrl Pts',(-5.17394074735488,-4.36498960086665,
75.9201055843859));
#27614=CARTESIAN_POINT('Ctrl Pts',(-5.05954803483568,-4.4970786759378,75.9283020948205));
#27615=CARTESIAN_POINT('Ctrl Pts',(-4.9402897543287,-4.62448117557796,75.9364986052552));
#27616=CARTESIAN_POINT('Ctrl Pts',(-4.8209054916518,-4.75201826078559,75.9447037743269));
#27617=CARTESIAN_POINT('Ctrl Pts',(-4.69664563788882,-4.87485861704672,
75.9529089433986));
#27618=CARTESIAN_POINT('Ctrl Pts',(-4.56792757942939,-4.99262722713086,
75.9611141124703));
#27619=CARTESIAN_POINT('Ctrl Pts',(-4.43913979586148,-5.11045963113181,
75.9693237261888));
#27620=CARTESIAN_POINT('Ctrl Pts',(-4.30588926724456,-5.22321458055498,
75.9775333399073));
#27621=CARTESIAN_POINT('Ctrl Pts',(-4.16862561853974,-5.33055808076923,
75.9857429536257));
#27622=CARTESIAN_POINT('Ctrl Pts',(-4.03115813489194,-5.43806098484935,
75.9939647585264));
#27623=CARTESIAN_POINT('Ctrl Pts',(-3.88966591261312,-5.54013617011796,
76.002186563427));
#27624=CARTESIAN_POINT('Ctrl Pts',(-3.74462772472484,-5.63649289924348,
76.0104083683277));
#27625=CARTESIAN_POINT('Ctrl Pts',(-3.61006253213103,-5.72589184996997,
76.0180364887284));
#27626=CARTESIAN_POINT('Ctrl Pts',(-3.47244546280035,-5.81036873395858,
76.0256646091292));
#27627=CARTESIAN_POINT('Ctrl Pts',(-3.33217612770128,-5.88972760439545,
76.03329272953));
#27628=CARTESIAN_POINT('Ctrl Pts',(-3.18130721697897,-5.97508329764449,
76.0414972755551));
#27629=CARTESIAN_POINT('Ctrl Pts',(-3.0269371937853,-6.05476244532253,76.0497018215801));
#27630=CARTESIAN_POINT('Ctrl Pts',(-2.86953283138995,-6.12846394535982,
76.0579063676052));
#27631=CARTESIAN_POINT('Ctrl Pts',(-2.71230795975889,-6.20208140237333,
76.0661015578525));
#27632=CARTESIAN_POINT('Ctrl Pts',(-2.55205596184382,-6.26973463211893,
76.0742967480997));
#27633=CARTESIAN_POINT('Ctrl Pts',(-2.38927063934438,-6.33116693919588,
76.082491938347));
#27634=CARTESIAN_POINT('Ctrl Pts',(-2.22663776963892,-6.39254171327962,
76.0906794535802));
#27635=CARTESIAN_POINT('Ctrl Pts',(-2.06147663517094,-6.44770703976832,
76.0988669688133));
#27636=CARTESIAN_POINT('Ctrl Pts',(-1.89430363851353,-6.49645308804077,
76.1070544840465));
#27637=CARTESIAN_POINT('Ctrl Pts',(-1.72725314759053,-6.54516341481176,
76.1152359994017));
#27638=CARTESIAN_POINT('Ctrl Pts',(-1.55819407566226,-6.58746373160529,
76.123417514757));
#27639=CARTESIAN_POINT('Ctrl Pts',(-1.38766077589796,-6.62319307970365,
76.1315990301122));
#27640=CARTESIAN_POINT('Ctrl Pts',(-1.21721771192587,-6.65890352201624,
76.13977621631));
#27641=CARTESIAN_POINT('Ctrl Pts',(-1.04530232627216,-6.68804984785324,
76.1479534025077));
#27642=CARTESIAN_POINT('Ctrl Pts',(-0.872462095912834,-6.71052150664875,
76.1561305887054));
#27643=CARTESIAN_POINT('Ctrl Pts',(-0.699654505435783,-6.73298892180089,
76.1643062306886));
#27644=CARTESIAN_POINT('Ctrl Pts',(-0.525922774676362,-6.74878412739203,
76.1724818726718));
#27645=CARTESIAN_POINT('Ctrl Pts',(-0.351822777305957,-6.75784801052589,
76.180657514655));
#27646=CARTESIAN_POINT('Ctrl Pts',(-0.177735405281618,-6.76691123636703,
76.1888325637587));
#27647=CARTESIAN_POINT('Ctrl Pts',(-0.00328018015343351,-6.76924409207052,
76.1970076128625));
#27648=CARTESIAN_POINT('Ctrl Pts',(0.170983807039123,-6.76483950568899,
76.2051826619662));
#27649=CARTESIAN_POINT('Ctrl Pts',(0.345267310525105,-6.76043442602596,
76.2133586266158));
#27650=CARTESIAN_POINT('Ctrl Pts',(0.519359172578241,-6.74929041020694,
76.2215345912652));
#27651=CARTESIAN_POINT('Ctrl Pts',(0.692702185721435,-6.73145249421674,
76.2297105559148));
#27652=CARTESIAN_POINT('Ctrl Pts',(0.866096596041697,-6.71360928918426,
76.2378889447837));
#27653=CARTESIAN_POINT('Ctrl Pts',(1.0387413563423,-6.68906826780223,76.2460673336527));
#27654=CARTESIAN_POINT('Ctrl Pts',(1.21008622448555,-6.65792612825573,76.2542457225217));
#27655=CARTESIAN_POINT('Ctrl Pts',(1.38161435648938,-6.62675068027821,76.2624328586799));
#27656=CARTESIAN_POINT('Ctrl Pts',(1.55183946318712,-6.58896007342355,76.2706199948381));
#27657=CARTESIAN_POINT('Ctrl Pts',(1.72022233242441,-6.54470198916867,76.2788071309962));
#27658=CARTESIAN_POINT('Ctrl Pts',(1.88869703941729,-6.50041976609764,76.286998732503));
#27659=CARTESIAN_POINT('Ctrl Pts',(2.05532716133459,-6.44966313953455,76.2951903340098));
#27660=CARTESIAN_POINT('Ctrl Pts',(2.21959057958728,-6.39262908817706,76.3033819355166));
#27661=CARTESIAN_POINT('Ctrl Pts',(2.38410261633552,-6.33550871376484,76.3115859353021));
#27662=CARTESIAN_POINT('Ctrl Pts',(2.54624045477815,-6.27209205858042,76.3197899350876));
#27663=CARTESIAN_POINT('Ctrl Pts',(2.70550261315695,-6.20262401006227,76.3279939348731));
#27664=CARTESIAN_POINT('Ctrl Pts',(2.85776488207488,-6.13620922080946,76.3358373525076));
#27665=CARTESIAN_POINT('Ctrl Pts',(3.00739862593188,-6.06426375596948,76.3436807701422));
#27666=CARTESIAN_POINT('Ctrl Pts',(3.15398921111939,-5.98703942329951,76.3515241877767));
#27667=CARTESIAN_POINT('Ctrl Pts',(3.30726280273132,-5.90629446404432,76.3597251836989));
#27668=CARTESIAN_POINT('Ctrl Pts',(3.45765999779837,-5.81954056214517,76.3679261796212));
#27669=CARTESIAN_POINT('Ctrl Pts',(3.60467527032724,-5.72700665230025,76.3761271755434));
#27670=CARTESIAN_POINT('Ctrl Pts',(3.75152072858995,-5.63457962643904,76.3843186986668));
#27671=CARTESIAN_POINT('Ctrl Pts',(3.89499173933582,-5.53638607589065,76.3925102217901));
#27672=CARTESIAN_POINT('Ctrl Pts',(4.03460543786044,-5.43270171837061,76.4007017449135));
#27673=CARTESIAN_POINT('Ctrl Pts',(4.17408639711627,-5.32911593990082,76.4088854798556));
#27674=CARTESIAN_POINT('Ctrl Pts',(4.30971705897001,-5.22004996373768,76.4170692147977));
#27675=CARTESIAN_POINT('Ctrl Pts',(4.44104169035459,-5.10582390065819,76.4252529497398));
#27676=CARTESIAN_POINT('Ctrl Pts',(4.57226828555852,-4.991683109373,76.4334305753778));
#27677=CARTESIAN_POINT('Ctrl Pts',(4.69919498096423,-4.87239013893223,76.4416082010157));
#27678=CARTESIAN_POINT('Ctrl Pts',(4.82139738678169,-4.74830667067058,76.4497858266537));
#27679=CARTESIAN_POINT('Ctrl Pts',(4.94353351904604,-4.62429049611128,76.4579590173519));
#27680=CARTESIAN_POINT('Ctrl Pts',(5.06095021247574,-4.49548925547615,76.4661322080501));
#27681=CARTESIAN_POINT('Ctrl Pts',(5.17325833158268,-4.3623029737411,76.4743053987483));
#27682=CARTESIAN_POINT('Ctrl Pts',(5.28554317670111,-4.22914429264627,76.4824768956888));
#27683=CARTESIAN_POINT('Ctrl Pts',(5.39272131867777,-4.09160265213043,76.4906483926292));
#27684=CARTESIAN_POINT('Ctrl Pts',(5.49444231288773,-3.95011299463052,76.4988198895697));
#27685=CARTESIAN_POINT('Ctrl Pts',(5.5961547940308,-3.80863517845135,76.5069907026346));
#27686=CARTESIAN_POINT('Ctrl Pts',(5.69241082521676,-3.6632102959724,76.5151615156995));
#27687=CARTESIAN_POINT('Ctrl Pts',(5.7829019613343,-3.51430418512626,76.5233323287644));
#27688=CARTESIAN_POINT('Ctrl Pts',(5.87340226301671,-3.3653829920447,76.5315039694255));
#27689=CARTESIAN_POINT('Ctrl Pts',(5.95813631873793,-3.21298017692343,76.5396756100866));
#27690=CARTESIAN_POINT('Ctrl Pts',(6.03684050559114,-3.05758821786946,76.5478472507477));
#27691=CARTESIAN_POINT('Ctrl Pts',(6.11556722283918,-2.90215177525838,76.5560212306781));
#27692=CARTESIAN_POINT('Ctrl Pts',(6.18826047013951,-2.74372480665621,76.5641952106085));
#27693=CARTESIAN_POINT('Ctrl Pts',(6.25470382725598,-2.58282191281346,76.5723691905389));
#27694=CARTESIAN_POINT('Ctrl Pts',(6.3212173727178,-2.42174904700708,76.5805518051644));
#27695=CARTESIAN_POINT('Ctrl Pts',(6.38146769987743,-2.2581953650045,76.5887344197898));
#27696=CARTESIAN_POINT('Ctrl Pts',(6.43528722598349,-2.09269379487151,76.5969170344152));
#27697=CARTESIAN_POINT('Ctrl Pts',(6.48913567283891,-1.92710328992665,76.6051040460944));
#27698=CARTESIAN_POINT('Ctrl Pts',(6.53654633228566,-1.7595631576783,76.6132910577736));
#27699=CARTESIAN_POINT('Ctrl Pts',(6.57740232329675,-1.59061864615329,76.6214780694527));
#27700=CARTESIAN_POINT('Ctrl Pts',(6.61831981538679,-1.42141982015728,76.6296774051519));
#27701=CARTESIAN_POINT('Ctrl Pts',(6.65266284940058,-1.25081274422523,76.6378767408511));
#27702=CARTESIAN_POINT('Ctrl Pts',(6.68036599908149,-1.07935124881386,76.6460760765503));
#27703=CARTESIAN_POINT('Ctrl Pts',(6.7070347716732,-0.914291763447366,76.6539692663747));
#27704=CARTESIAN_POINT('Ctrl Pts',(6.72755054752573,-0.748440793180089,
76.6618624561991));
#27705=CARTESIAN_POINT('Ctrl Pts',(6.7419006060402,-0.582293069059596,76.6697556460235));
#27706=CARTESIAN_POINT('Ctrl Pts',(6.75680918446336,-0.409678694533961,
76.6779560473938));
#27707=CARTESIAN_POINT('Ctrl Pts',(6.76510607348375,-0.236238752306226,
76.6861564487641));
#27708=CARTESIAN_POINT('Ctrl Pts',(6.76671116160101,-0.0625224396867994,
76.6943568501344));
#27709=CARTESIAN_POINT('Ctrl Pts',(6.76831441495384,0.110995299093639,76.7025478776862));
#27710=CARTESIAN_POINT('Ctrl Pts',(6.76324109415873,0.284788421595302,76.710738905238));
#27711=CARTESIAN_POINT('Ctrl Pts',(6.7514627060908,0.458301569127896,76.7189299327898));
#27712=CARTESIAN_POINT('Ctrl Pts',(6.73969537533962,0.631651825964342,76.7271132707676));
#27713=CARTESIAN_POINT('Ctrl Pts',(6.72123553599781,0.804722273265913,76.7352966087455));
#27714=CARTESIAN_POINT('Ctrl Pts',(6.69610671255181,0.976956444330344,76.7434799467234));
#27715=CARTESIAN_POINT('Ctrl Pts',(6.67099634724974,1.14906410238369,76.7516572737063));
#27716=CARTESIAN_POINT('Ctrl Pts',(6.63922680585662,1.32033635172206,76.7598346006892));
#27717=CARTESIAN_POINT('Ctrl Pts',(6.6008735259449,1.49022068650244,76.7680119276722));
#27718=CARTESIAN_POINT('Ctrl Pts',(6.56254058675614,1.66001492285582,76.7761849177967));
#27719=CARTESIAN_POINT('Ctrl Pts',(6.51763094366037,1.82842235944485,76.7843579079213));
#27720=CARTESIAN_POINT('Ctrl Pts',(6.46627134011109,1.99489948520167,76.7925308980459));
#27721=CARTESIAN_POINT('Ctrl Pts',(6.41492143745227,2.16134516647203,76.800702344442));
#27722=CARTESIAN_POINT('Ctrl Pts',(6.35712410075653,2.32586091634325,76.8088737908381));
#27723=CARTESIAN_POINT('Ctrl Pts',(6.29305635190756,2.4879169503253,76.8170452372342));
#27724=CARTESIAN_POINT('Ctrl Pts',(6.22899324904884,2.64996123251699,76.8252160910629));
#27725=CARTESIAN_POINT('Ctrl Pts',(6.15866077139806,2.80954581770161,76.8333869448916));
#27726=CARTESIAN_POINT('Ctrl Pts',(6.08228461484099,2.96615961540652,76.8415577987203));
#27727=CARTESIAN_POINT('Ctrl Pts',(6.005899868952,3.12279102604134,76.8497295714506));
#27728=CARTESIAN_POINT('Ctrl Pts',(5.92347024850822,3.27645065885469,76.8579013441809));
#27729=CARTESIAN_POINT('Ctrl Pts',(5.83526806284311,3.42665078973088,76.8660731169113));
#27730=CARTESIAN_POINT('Ctrl Pts',(5.74703964218504,3.57689559636364,76.8742473202662));
#27731=CARTESIAN_POINT('Ctrl Pts',(5.65303541946452,3.72367854019776,76.8824215236211));
#27732=CARTESIAN_POINT('Ctrl Pts',(5.55357179756744,3.86653970486062,76.890595726976));
#27733=CARTESIAN_POINT('Ctrl Pts',(5.45400136205057,4.0095542876057,76.898778708578));
#27734=CARTESIAN_POINT('Ctrl Pts',(5.34896002110029,4.14863838027531,76.90696169018));
#27735=CARTESIAN_POINT('Ctrl Pts',(5.23880596380514,4.28336328993931,76.915144671782));
#27736=CARTESIAN_POINT('Ctrl Pts',(5.12859165816888,4.41816188687832,76.9233321290345));
#27737=CARTESIAN_POINT('Ctrl Pts',(5.01325930138959,4.54859627816795,76.9315195862871));
#27738=CARTESIAN_POINT('Ctrl Pts',(4.89320480833117,4.67427381565572,76.9397070435396));
#27739=CARTESIAN_POINT('Ctrl Pts',(4.77296769160171,4.80014253043873,76.9479069553323));
#27740=CARTESIAN_POINT('Ctrl Pts',(4.64799434283454,4.92123967936631,76.9561068671249));
#27741=CARTESIAN_POINT('Ctrl Pts',(4.51871566902883,5.03721130214659,76.9643067789176));
#27742=CARTESIAN_POINT('Ctrl Pts',(4.39426875893537,5.1488485094962,76.9722002207019));
#27743=CARTESIAN_POINT('Ctrl Pts',(4.26583276678869,5.255736246645,76.9800936624861));
#27744=CARTESIAN_POINT('Ctrl Pts',(4.13381722501289,5.35759686335084,76.9879871042704));
#27745=CARTESIAN_POINT('Ctrl Pts',(3.99656214708984,5.46350020393626,76.9961938271503));
#27746=CARTESIAN_POINT('Ctrl Pts',(3.85503363666689,5.56428086779919,77.0044005500301));
#27747=CARTESIAN_POINT('Ctrl Pts',(3.70965096763684,5.65957407393092,77.0126072729099));
#27748=CARTESIAN_POINT('Ctrl Pts',(3.56445821167055,5.75474279875514,77.0208032753655));
#27749=CARTESIAN_POINT('Ctrl Pts',(3.41542162516261,5.84443814881979,77.0289992778211));
#27750=CARTESIAN_POINT('Ctrl Pts',(3.26299338575027,5.92833561503986,77.0371952802767));
#27751=CARTESIAN_POINT('Ctrl Pts',(3.20880870231055,5.9581592072171,77.0401087679627));
#27752=CARTESIAN_POINT('Ctrl Pts',(3.15419573595972,5.98725053256884,77.0430222556487));
#27753=CARTESIAN_POINT('Ctrl Pts',(3.09917575053268,6.01559628526634,77.0459357433347));
#27754=CARTESIAN_POINT('Ctrl Pts',(3.09917575053257,6.0155962852664,75.0456602561759));
#27755=CARTESIAN_POINT('Ctrl Pts',(2.936252244306,6.09953286540656,75.0543064777294));
#27756=CARTESIAN_POINT('Ctrl Pts',(2.77005294528275,6.17677667981186,75.0629526992828));
#27757=CARTESIAN_POINT('Ctrl Pts',(2.60114913456995,6.24710430357346,75.0715989208363));
#27758=CARTESIAN_POINT('Ctrl Pts',(2.55557118817139,6.26608190184443,75.0739320654874));
#27759=CARTESIAN_POINT('Ctrl Pts',(2.50979639803627,6.28455616581868,75.0762652101384));
#27760=CARTESIAN_POINT('Ctrl Pts',(2.46383617595217,6.30252332784809,75.0785983547895));
#27761=CARTESIAN_POINT('Ctrl Pts',(2.30188633020025,6.36583414288156,75.086819647012));
#27762=CARTESIAN_POINT('Ctrl Pts',(2.13727981104482,6.42298273401547,75.0950409392344));
#27763=CARTESIAN_POINT('Ctrl Pts',(1.97052598322084,6.47374052225231,75.1032622314568));
#27764=CARTESIAN_POINT('Ctrl Pts',(1.80394795520669,6.52444479921665,75.1114748564023));
#27765=CARTESIAN_POINT('Ctrl Pts',(1.63522746682688,6.56877158618861,75.1196874813477));
#27766=CARTESIAN_POINT('Ctrl Pts',(1.46489384591365,6.60654032154534,75.1279001062932));
#27767=CARTESIAN_POINT('Ctrl Pts',(1.29470559624531,6.64427682317129,75.1361057221731));
#27768=CARTESIAN_POINT('Ctrl Pts',(1.12290730418151,6.67546634280842,75.1443113380531));
#27769=CARTESIAN_POINT('Ctrl Pts',(0.950043535671968,6.69997808058563,75.152516953933));
#27770=CARTESIAN_POINT('Ctrl Pts',(0.777292597003479,6.7244738193163,75.1607172139287));
#27771=CARTESIAN_POINT('Ctrl Pts',(0.603477921062569,6.74230040791232,75.1689174739244));
#27772=CARTESIAN_POINT('Ctrl Pts',(0.429154437381481,6.75337807833056,75.1771177339201));
#27773=CARTESIAN_POINT('Ctrl Pts',(0.254909749631426,6.7644507415327,75.1853142873175));
#27774=CARTESIAN_POINT('Ctrl Pts',(0.0801570696198197,6.7687805413485,75.1935108407149));
#27775=CARTESIAN_POINT('Ctrl Pts',(-0.0945432858093703,6.76633952496536,
75.2017073941123));
#27776=CARTESIAN_POINT('Ctrl Pts',(-0.269229525155645,6.76389870582045,
75.2099032852145));
#27777=CARTESIAN_POINT('Ctrl Pts',(-0.443863089772879,6.75468815641717,
75.2180991763166));
#27778=CARTESIAN_POINT('Ctrl Pts',(-0.61788301799291,6.73873204513104,75.2262950674187));
#27779=CARTESIAN_POINT('Ctrl Pts',(-0.791901732066226,6.72277604517159,
75.2344909013376));
#27780=CARTESIAN_POINT('Ctrl Pts',(-0.96530646080996,6.70007460874533,75.2426867352565));
#27781=CARTESIAN_POINT('Ctrl Pts',(-1.13754084878975,6.67070384722142,75.2508825691754));
#27782=CARTESIAN_POINT('Ctrl Pts',(-1.30980535679711,6.64132794939369,75.2590798363665));
#27783=CARTESIAN_POINT('Ctrl Pts',(-1.48089876252137,6.60528046312545,75.2672771035575));
#27784=CARTESIAN_POINT('Ctrl Pts',(-1.65027434260422,6.56268874731556,75.2754743707485));
#27785=CARTESIAN_POINT('Ctrl Pts',(-1.81971034495408,6.52008183753246,75.283674562195));
#27786=CARTESIAN_POINT('Ctrl Pts',(-1.98742695312793,6.47092613517448,75.2918747536415));
#27787=CARTESIAN_POINT('Ctrl Pts',(-2.15289200691712,6.41539905279105,75.300074945088));
#27788=CARTESIAN_POINT('Ctrl Pts',(-2.31854714189323,6.35980818259574,75.3082845566633));
#27789=CARTESIAN_POINT('Ctrl Pts',(-2.48194521447529,6.29783142399216,75.3164941682387));
#27790=CARTESIAN_POINT('Ctrl Pts',(-2.64257248217977,6.2296949906417,75.324703779814));
#27791=CARTESIAN_POINT('Ctrl Pts',(-2.8032949711322,6.16151816541813,75.3329182581188));
#27792=CARTESIAN_POINT('Ctrl Pts',(-2.96124305689478,6.0871745393371,75.3411327364236));
#27793=CARTESIAN_POINT('Ctrl Pts',(-3.11592718696044,6.00693655414811,75.3493472147284));
#27794=CARTESIAN_POINT('Ctrl Pts',(-3.27085351692534,5.92657293466219,75.3575745550238));
#27795=CARTESIAN_POINT('Ctrl Pts',(-3.4225053663222,5.84029668953091,75.3658018953191));
#27796=CARTESIAN_POINT('Ctrl Pts',(-3.57042063114997,5.74842461172265,75.3740292356145));
#27797=CARTESIAN_POINT('Ctrl Pts',(-3.70706071678748,5.66355569306146,75.3816294280884));
#27798=CARTESIAN_POINT('Ctrl Pts',(-3.8405123192312,5.57391213840449,75.3892296205624));
#27799=CARTESIAN_POINT('Ctrl Pts',(-3.97043679625273,5.47977377698773,75.3968298130363));
#27800=CARTESIAN_POINT('Ctrl Pts',(-4.10880138720218,5.37952002828168,75.4049237268769));
#27801=CARTESIAN_POINT('Ctrl Pts',(-4.24360748295849,5.27384752031896,75.4130176407175));
#27802=CARTESIAN_POINT('Ctrl Pts',(-4.37439261120662,5.16303963601104,75.421111554558));
#27803=CARTESIAN_POINT('Ctrl Pts',(-4.50501851826732,5.05236665207865,75.4291956146592));
#27804=CARTESIAN_POINT('Ctrl Pts',(-4.6316329194727,4.93657097059121,75.4372796747604));
#27805=CARTESIAN_POINT('Ctrl Pts',(-4.75380155701409,4.81597962584254,75.4453637348615));
#27806=CARTESIAN_POINT('Ctrl Pts',(-4.87584800581626,4.69550889228077,75.4534397095724));
#27807=CARTESIAN_POINT('Ctrl Pts',(-4.99345727873904,4.5702523008029,75.4615156842834));
#27808=CARTESIAN_POINT('Ctrl Pts',(-5.10622758671122,4.44057753368966,75.4695916589943));
#27809=CARTESIAN_POINT('Ctrl Pts',(-5.21890957791099,4.31100432218179,75.477661308955));
#27810=CARTESIAN_POINT('Ctrl Pts',(-5.32675990559054,4.17702010185328,75.4857309589158));
#27811=CARTESIAN_POINT('Ctrl Pts',(-5.42941317645325,4.0390297794589,75.4938006088766));
#27812=CARTESIAN_POINT('Ctrl Pts',(-5.53721182958505,3.89412284396309,75.5022747411639));
#27813=CARTESIAN_POINT('Ctrl Pts',(-5.63927870639082,3.74479814434747,75.5107488734512));
#27814=CARTESIAN_POINT('Ctrl Pts',(-5.73523751793923,3.59156506453974,75.5192230057385));
#27815=CARTESIAN_POINT('Ctrl Pts',(-5.82654210433266,3.44576414487559,75.5272861229349));
#27816=CARTESIAN_POINT('Ctrl Pts',(-5.91231690917891,3.29642536596832,75.5353492401312));
#27817=CARTESIAN_POINT('Ctrl Pts',(-5.9922817639834,3.14401785316687,75.5434123573276));
#27818=CARTESIAN_POINT('Ctrl Pts',(-6.07224075178296,2.99162152247324,75.5514748829347));
#27819=CARTESIAN_POINT('Ctrl Pts',(-6.14639046491053,2.83615723480353,75.5595374085418));
#27820=CARTESIAN_POINT('Ctrl Pts',(-6.21449666504386,2.67811878006908,75.5675999341489));
#27821=CARTESIAN_POINT('Ctrl Pts',(-6.28261123627576,2.52006090044411,75.5756634507406));
#27822=CARTESIAN_POINT('Ctrl Pts',(-6.34468066901941,2.35942856529058,75.5837269673323));
#27823=CARTESIAN_POINT('Ctrl Pts',(-6.40051890149288,2.19673548513068,75.591790483924));
#27824=CARTESIAN_POINT('Ctrl Pts',(-6.45637495898567,2.03399046909878,75.5998565746004));
#27825=CARTESIAN_POINT('Ctrl Pts',(-6.50599573664958,1.86918374994993,75.6079226652768));
#27826=CARTESIAN_POINT('Ctrl Pts',(-6.54924509258621,1.70284400848564,75.6159887559532));
#27827=CARTESIAN_POINT('Ctrl Pts',(-6.59253813844064,1.53633623285129,75.6240629948859));
#27828=CARTESIAN_POINT('Ctrl Pts',(-6.62944681890226,1.36829270265695,75.6321372338187));
#27829=CARTESIAN_POINT('Ctrl Pts',(-6.65988602009892,1.19925276705582,75.6402114727514));
#27830=CARTESIAN_POINT('Ctrl Pts',(-6.69034314218094,1.03011331027184,75.6482904653407));
#27831=CARTESIAN_POINT('Ctrl Pts',(-6.71432314705273,0.859976646327041,
75.6563694579301));
#27832=CARTESIAN_POINT('Ctrl Pts',(-6.73179286057427,0.689386598594249,
75.6644484505195));
#27833=CARTESIAN_POINT('Ctrl Pts',(-6.74928514849801,0.51857611402685,75.6725378828008));
#27834=CARTESIAN_POINT('Ctrl Pts',(-6.76025032810092,0.347311445157489,
75.6806273150821));
#27835=CARTESIAN_POINT('Ctrl Pts',(-6.76470730673057,0.176136464896053,
75.6887167473634));
#27836=CARTESIAN_POINT('Ctrl Pts',(-6.76626158030231,0.116442943775122,
75.6915377594997));
#27837=CARTESIAN_POINT('Ctrl Pts',(-6.7670248458201,0.0567602853936582,
75.694358771636));
#27838=CARTESIAN_POINT('Ctrl Pts',(-6.7669993834644,-0.00288863157981475,
75.6971797837723));
#27839=CARTESIAN_POINT('',(-6.76699950924454,-0.00257718532368157,75.3028202161604));
#27840=CARTESIAN_POINT('Ctrl Pts',(3.09917575053252,6.01559628526642,74.65129258962));
#27841=CARTESIAN_POINT('Ctrl Pts',(2.94413043308495,6.09547410041237,74.6595198212406));
#27842=CARTESIAN_POINT('Ctrl Pts',(2.78616723896163,6.16926519409222,74.6677470528611));
#27843=CARTESIAN_POINT('Ctrl Pts',(2.62581165236062,6.23677818800117,74.6759742844817));
#27844=CARTESIAN_POINT('Ctrl Pts',(2.57537278231676,6.25801398775238,74.6785621099221));
#27845=CARTESIAN_POINT('Ctrl Pts',(2.52469732381167,6.27862901756869,74.6811499353626));
#27846=CARTESIAN_POINT('Ctrl Pts',(2.47380190500018,6.29861835125907,74.6837377608031));
#27847=CARTESIAN_POINT('Ctrl Pts',(2.3134576069224,6.36159407195207,74.6918906174548));
#27848=CARTESIAN_POINT('Ctrl Pts',(2.15045627898565,6.41854141552854,74.7000434741066));
#27849=CARTESIAN_POINT('Ctrl Pts',(1.98529534587594,6.46922649082897,74.7081963307584));
#27850=CARTESIAN_POINT('Ctrl Pts',(1.82032574068788,6.51985285085133,74.7163397428697));
#27851=CARTESIAN_POINT('Ctrl Pts',(1.65320185620246,6.5642312770898,74.724483154981));
#27852=CARTESIAN_POINT('Ctrl Pts',(1.48444204070888,6.6021754617532,74.7326265670922));
#27853=CARTESIAN_POINT('Ctrl Pts',(1.31584224855384,6.64008366655321,74.7407622573653));
#27854=CARTESIAN_POINT('Ctrl Pts',(1.14560996789608,6.67156969676873,74.7488979476384));
#27855=CARTESIAN_POINT('Ctrl Pts',(0.974279696714471,6.69649670145293,74.7570336379114));
#27856=CARTESIAN_POINT('Ctrl Pts',(0.803075891661222,6.7214053064594,74.765163322887));
#27857=CARTESIAN_POINT('Ctrl Pts',(0.63077607008167,6.73976447380729,74.7732930078626));
#27858=CARTESIAN_POINT('Ctrl Pts',(0.457925940292265,6.75148819396194,74.7814226928381));
#27859=CARTESIAN_POINT('Ctrl Pts',(0.285167097745749,6.76320572247479,74.7895480842877));
#27860=CARTESIAN_POINT('Ctrl Pts',(0.111858889681834,6.768294758233,74.7976734757372));
#27861=CARTESIAN_POINT('Ctrl Pts',(-0.0614468195600911,6.76672101452143,
74.8057988671868));
#27862=CARTESIAN_POINT('Ctrl Pts',(-0.23540362763242,6.76514135835208,74.8139547852294));
#27863=CARTESIAN_POINT('Ctrl Pts',(-0.409357548712867,6.75684871675658,
74.8221107032721));
#27864=CARTESIAN_POINT('Ctrl Pts',(-0.582748894518102,6.7418612212013,74.8302666213148));
#27865=CARTESIAN_POINT('Ctrl Pts',(-0.75545270009904,6.72693315482924,74.8383901990945));
#27866=CARTESIAN_POINT('Ctrl Pts',(-0.927598018683367,6.70536328383634,
74.8465137768742));
#27867=CARTESIAN_POINT('Ctrl Pts',(-1.09863573120725,6.6772216175678,74.8546373546539));
#27868=CARTESIAN_POINT('Ctrl Pts',(-1.26969619627758,6.64907620771219,74.8627620130846));
#27869=CARTESIAN_POINT('Ctrl Pts',(-1.43964840083078,6.61435732068323,74.8708866715153));
#27870=CARTESIAN_POINT('Ctrl Pts',(-1.6079523839229,6.57318629973597,74.879011329946));
#27871=CARTESIAN_POINT('Ctrl Pts',(-1.77631077131051,6.53200197024813,74.8871386146742));
#27872=CARTESIAN_POINT('Ctrl Pts',(-1.94301952115045,6.48436144051514,74.8952658994024));
#27873=CARTESIAN_POINT('Ctrl Pts',(-2.1075528641131,6.43043621576085,74.9033931841305));
#27874=CARTESIAN_POINT('Ctrl Pts',(-2.27313268126583,6.37616801276954,74.9115721604705));
#27875=CARTESIAN_POINT('Ctrl Pts',(-2.4365089680254,6.31553501475819,74.9197511368105));
#27876=CARTESIAN_POINT('Ctrl Pts',(-2.59716616673497,6.24876122942517,74.9279301131506));
#27877=CARTESIAN_POINT('Ctrl Pts',(-2.75708328973481,6.18229504099394,74.9360714126123));
#27878=CARTESIAN_POINT('Ctrl Pts',(-2.91430601824737,6.10974473297503,74.944212712074));
#27879=CARTESIAN_POINT('Ctrl Pts',(-3.0683508613743,6.03137728810789,74.9523540115358));
#27880=CARTESIAN_POINT('Ctrl Pts',(-3.22346505384107,5.95246583168064,74.960551826315));
#27881=CARTESIAN_POINT('Ctrl Pts',(-3.37535675287037,5.86765636976144,74.9687496410941));
#27882=CARTESIAN_POINT('Ctrl Pts',(-3.52356256017727,5.77726543310215,74.9769474558732));
#27883=CARTESIAN_POINT('Ctrl Pts',(-3.67176836748422,5.68687449644283,74.9851452706524));
#27884=CARTESIAN_POINT('Ctrl Pts',(-3.81628800975053,5.59090234420921,74.9933430854316));
#27885=CARTESIAN_POINT('Ctrl Pts',(-3.95669274005271,5.48970596305614,75.0015409002108));
#27886=CARTESIAN_POINT('Ctrl Pts',(-4.09673947537978,5.38876760594453,75.0097178127276));
#27887=CARTESIAN_POINT('Ctrl Pts',(-4.23313948046358,5.28230936702573,75.0178947252445));
#27888=CARTESIAN_POINT('Ctrl Pts',(-4.36542511513103,5.17062400143186,75.0260716377614));
#27889=CARTESIAN_POINT('Ctrl Pts',(-4.49755300339918,5.0590718170736,75.034238799571));
#27890=CARTESIAN_POINT('Ctrl Pts',(-4.62557601351266,4.94230514731659,75.0424059613805));
#27891=CARTESIAN_POINT('Ctrl Pts',(-4.74905519303882,4.8206600972762,75.0505731231901));
#27892=CARTESIAN_POINT('Ctrl Pts',(-4.8724128025047,4.69913481152419,75.0587322441108));
#27893=CARTESIAN_POINT('Ctrl Pts',(-4.99123523133266,4.57274096208986,75.0668913650316));
#27894=CARTESIAN_POINT('Ctrl Pts',(-5.10511635540047,4.44185501765002,75.0750504859523));
#27895=CARTESIAN_POINT('Ctrl Pts',(-5.21890902677056,4.31107073373535,75.0832032695958));
#27896=CARTESIAN_POINT('Ctrl Pts',(-5.32776779859115,4.17580157616478,75.0913560532393));
#27897=CARTESIAN_POINT('Ctrl Pts',(-5.43132319685854,4.03646099092589,75.0995088368828));
#27898=CARTESIAN_POINT('Ctrl Pts',(-5.53892443555819,3.89167646183618,75.1079801443527));
#27899=CARTESIAN_POINT('Ctrl Pts',(-5.64079924473297,3.74249622148247,75.1164514518226));
#27900=CARTESIAN_POINT('Ctrl Pts',(-5.73657842999148,3.58942292249834,75.1249227592925));
#27901=CARTESIAN_POINT('Ctrl Pts',(-5.82867849433613,3.44222955634225,75.1330686624024));
#27902=CARTESIAN_POINT('Ctrl Pts',(-5.91514230575042,3.29143698702313,75.1412145655123));
#27903=CARTESIAN_POINT('Ctrl Pts',(-5.99568538203235,3.13752223891458,75.1493604686222));
#27904=CARTESIAN_POINT('Ctrl Pts',(-6.07622062204455,2.98362246561874,75.1575055791936));
#27905=CARTESIAN_POINT('Ctrl Pts',(-6.15083610494592,2.82660144059169,75.1656506897649));
#27906=CARTESIAN_POINT('Ctrl Pts',(-6.21929326435158,2.66696087185227,75.1737958003362));
#27907=CARTESIAN_POINT('Ctrl Pts',(-6.28775664497366,2.50730579537495,75.181941651115));
#27908=CARTESIAN_POINT('Ctrl Pts',(-6.3500604445398,2.34503103571817,75.1900875018937));
#27909=CARTESIAN_POINT('Ctrl Pts',(-6.40601422093905,2.18065834121871,75.1982333526724));
#27910=CARTESIAN_POINT('Ctrl Pts',(-6.46198361135054,2.01623977819294,75.206381476567));
#27911=CARTESIAN_POINT('Ctrl Pts',(-6.51159933340503,1.84972245903932,75.2145296004615));
#27912=CARTESIAN_POINT('Ctrl Pts',(-6.55472079588228,1.68164332961196,75.2226777243561));
#27913=CARTESIAN_POINT('Ctrl Pts',(-6.59788165812257,1.51341062752053,75.2308332931315));
#27914=CARTESIAN_POINT('Ctrl Pts',(-6.63453632191359,1.3436136182976,75.2389888619069));
#27915=CARTESIAN_POINT('Ctrl Pts',(-6.66459516543763,1.17280018793716,75.2471444306823));
#27916=CARTESIAN_POINT('Ctrl Pts',(-6.69467028720986,1.00189425423693,75.2553044160738));
#27917=CARTESIAN_POINT('Ctrl Pts',(-6.71814242126883,0.829971162146733,
75.2634644014653));
#27918=CARTESIAN_POINT('Ctrl Pts',(-6.73497384065071,0.657583732881759,
75.2716243868568));
#27919=CARTESIAN_POINT('Ctrl Pts',(-6.75182495625526,0.484994574866744,
75.2797939211097));
#27920=CARTESIAN_POINT('Ctrl Pts',(-6.7620198204316,0.311940356769789,75.2879634553625));
#27921=CARTESIAN_POINT('Ctrl Pts',(-6.76557278506292,0.13897442216476,75.2961329896153));
#27922=CARTESIAN_POINT('Ctrl Pts',(-6.76654221933179,0.0917802838171845,
75.2983620651304));
#27923=CARTESIAN_POINT('Ctrl Pts',(-6.76701747370815,0.0445926923504295,
75.3005911406454));
#27924=CARTESIAN_POINT('Ctrl Pts',(-6.76699950924454,-0.00257718532368525,
75.3028202161604));
#27925=CARTESIAN_POINT('Ctrl Pts',(-6.7669995092443,-0.00257718594549182,
75.3028202161898));
#27926=CARTESIAN_POINT('Ctrl Pts',(-6.76695511988582,-0.119131743290941,
75.3083281573327));
#27927=CARTESIAN_POINT('Ctrl Pts',(-6.7638995537784,-0.235635131100597,
75.3138360984756));
#27928=CARTESIAN_POINT('Ctrl Pts',(-6.75783999317536,-0.351976741617549,
75.3193440396185));
#27929=CARTESIAN_POINT('Ctrl Pts',(-6.74832645104384,-0.534633684225855,
75.327991536286));
#27930=CARTESIAN_POINT('Ctrl Pts',(-6.73139459518651,-0.717067462451649,
75.3366390329534));
#27931=CARTESIAN_POINT('Ctrl Pts',(-6.70706262624517,-0.898665637278532,
75.3452865296209));
#27932=CARTESIAN_POINT('Ctrl Pts',(-6.68276187306911,-1.08003083769983,
75.3539229323145));
#27933=CARTESIAN_POINT('Ctrl Pts',(-6.65107997811199,-1.26056227178707,
75.3625593350081));
#27934=CARTESIAN_POINT('Ctrl Pts',(-6.61208702713136,-1.43965070265018,
75.3711957377018));
#27935=CARTESIAN_POINT('Ctrl Pts',(-6.57180993352493,-1.62463699664177,
75.3801165603368));
#27936=CARTESIAN_POINT('Ctrl Pts',(-6.52373201512505,-1.80808330155989,
75.3890373829718));
#27937=CARTESIAN_POINT('Ctrl Pts',(-6.4679886896944,-1.98932433504074,75.3979582056069));
#27938=CARTESIAN_POINT('Ctrl Pts',(-6.41417229764686,-2.16430023462252,
75.4065706535476));
#27939=CARTESIAN_POINT('Ctrl Pts',(-6.35321164717404,-2.33722043335061,
75.4151831014883));
#27940=CARTESIAN_POINT('Ctrl Pts',(-6.28528044630663,-2.50749650274444,
75.423795549429));
#27941=CARTESIAN_POINT('Ctrl Pts',(-6.21741364601772,-2.67761114591238,
75.4323998325408));
#27942=CARTESIAN_POINT('Ctrl Pts',(-6.14258958304672,-2.84508637535941,
75.4410041156527));
#27943=CARTESIAN_POINT('Ctrl Pts',(-6.06103140439988,-3.0093499821188,75.4496083987645));
#27944=CARTESIAN_POINT('Ctrl Pts',(-5.97956517166778,-3.17342840367871,
75.4582029817004));
#27945=CARTESIAN_POINT('Ctrl Pts',(-5.89138010394163,-3.33430215333452,
75.4667975646363));
#27946=CARTESIAN_POINT('Ctrl Pts',(-5.79674706374688,-3.49141983710666,
75.4753921475722));
#27947=CARTESIAN_POINT('Ctrl Pts',(-5.78627411962668,-3.50880789437562,
75.4763433014889));
#27948=CARTESIAN_POINT('Ctrl Pts',(-5.7757222510552,-3.52614997036092,75.4772944554055));
#27949=CARTESIAN_POINT('Ctrl Pts',(-5.76509186076488,-3.54344533426756,
75.4782456093221));
#27950=CARTESIAN_POINT('Ctrl Pts',(-5.66902795920877,-3.69973876191513,
75.4868409246132));
#27951=CARTESIAN_POINT('Ctrl Pts',(-5.56666113924929,-3.85203150406105,
75.4954362399043));
#27952=CARTESIAN_POINT('Ctrl Pts',(-5.45835665296343,-3.99982895247407,
75.5040315551953));
#27953=CARTESIAN_POINT('Ctrl Pts',(-5.34995091271714,-4.14776457685291,
75.5126349062543));
#27954=CARTESIAN_POINT('Ctrl Pts',(-5.23559660637491,-4.29119627254647,
75.5212382573133));
#27955=CARTESIAN_POINT('Ctrl Pts',(-5.11569926429793,-4.42966251956756,
75.5298416083722));
#27956=CARTESIAN_POINT('Ctrl Pts',(-4.99108064550539,-4.57358124332105,
75.53878373926));
#27957=CARTESIAN_POINT('Ctrl Pts',(-4.86047385924745,-4.71213526341169,
75.5477258701478));
#27958=CARTESIAN_POINT('Ctrl Pts',(-4.724375335431,-4.84484950127156,75.5566680010357));
#27959=CARTESIAN_POINT('Ctrl Pts',(-4.5930757902966,-4.97288409397118,75.565294822879));
#27960=CARTESIAN_POINT('Ctrl Pts',(-4.4566654365246,-5.09548354393135,75.5739216447223));
#27961=CARTESIAN_POINT('Ctrl Pts',(-4.31562317917473,-5.2122629994437,75.5825484665656));
#27962=CARTESIAN_POINT('Ctrl Pts',(-4.17444631306465,-5.32915390763711,
75.5911835217272));
#27963=CARTESIAN_POINT('Ctrl Pts',(-4.02862896005788,-5.44021354694062,
75.5998185768888));
#27964=CARTESIAN_POINT('Ctrl Pts',(-3.87868012836255,-5.54509958989426,
75.6084536320504));
#27965=CARTESIAN_POINT('Ctrl Pts',(-3.72850930140897,-5.65014091384562,
75.6171014711816));
#27966=CARTESIAN_POINT('Ctrl Pts',(-3.57419502728713,-5.7489902088327,75.6257493103127));
#27967=CARTESIAN_POINT('Ctrl Pts',(-3.41627335681156,-5.84134961730074,
75.6343971494439));
#27968=CARTESIAN_POINT('Ctrl Pts',(-3.39953355785119,-5.851139774188,75.6353138259713));
#27969=CARTESIAN_POINT('Ctrl Pts',(-3.38275324631712,-5.86085705344682,
75.6362305024987));
#27970=CARTESIAN_POINT('Ctrl Pts',(-3.36593307495136,-5.87050113150049,
75.6371471790261));
#27971=CARTESIAN_POINT('Ctrl Pts',(-3.21504622272769,-5.95701419658615,
75.6453703078352));
#27972=CARTESIAN_POINT('Ctrl Pts',(-3.06062266175904,-6.03782044790086,
75.6535934366442));
#27973=CARTESIAN_POINT('Ctrl Pts',(-2.90313284033744,-6.11261880959006,
75.6618165654533));
#27974=CARTESIAN_POINT('Ctrl Pts',(-2.74580854084296,-6.18733855814185,
75.6700310517474));
#27975=CARTESIAN_POINT('Ctrl Pts',(-2.58542471950291,-6.25606283843597,
75.6782455380416));
#27976=CARTESIAN_POINT('Ctrl Pts',(-2.42247862355748,-6.31853514023678,
75.6864600243357));
#27977=CARTESIAN_POINT('Ctrl Pts',(-2.2596711106832,-6.3809543103354,75.6946675243395));
#27978=CARTESIAN_POINT('Ctrl Pts',(-2.09430599618221,-6.43713196409455,
75.7028750243433));
#27979=CARTESIAN_POINT('Ctrl Pts',(-1.92690291084765,-6.48685857500893,
75.7110825243471));
#27980=CARTESIAN_POINT('Ctrl Pts',(-1.75960864155004,-6.53655286242867,
75.7192846892783));
#27981=CARTESIAN_POINT('Ctrl Pts',(-1.59027938264561,-6.57980435797223,
75.7274868542094));
#27982=CARTESIAN_POINT('Ctrl Pts',(-1.41945251573209,-6.6164524902384,75.7356890191405));
#27983=CARTESIAN_POINT('Ctrl Pts',(-1.24870245337201,-6.65308414533393,
75.7438874963402));
#27984=CARTESIAN_POINT('Ctrl Pts',(-1.07645647432253,-6.68311827694216,
75.7520859735398));
#27985=CARTESIAN_POINT('Ctrl Pts',(-0.90326490629413,-6.70644477417487,
75.7602844507395));
#27986=CARTESIAN_POINT('Ctrl Pts',(-0.730087019760185,-6.72976942870042,
75.7684822802897));
#27987=CARTESIAN_POINT('Ctrl Pts',(-0.555964046950391,-6.74638744779066,
75.77668010984));
#27988=CARTESIAN_POINT('Ctrl Pts',(-0.381454617778284,-6.75624018034999,
75.7848779393902));
#27989=CARTESIAN_POINT('Ctrl Pts',(-0.206946137542495,-6.76609285933275,
75.7930757243628));
#27990=CARTESIAN_POINT('Ctrl Pts',(-0.0320515631633243,-6.76918030376751,
75.8012735093354));
#27991=CARTESIAN_POINT('Ctrl Pts',(0.142667390920719,-6.76549591793299,
75.8094712943079));
#27992=CARTESIAN_POINT('Ctrl Pts',(0.317417124460915,-6.7618108830367,75.8176705234476));
#27993=CARTESIAN_POINT('Ctrl Pts',(0.491990817478394,-6.75135164868189,
75.8258697525873));
#27994=CARTESIAN_POINT('Ctrl Pts',(0.665828741854239,-6.73416372584754,
75.8340689817269));
#27995=CARTESIAN_POINT('Ctrl Pts',(0.839728860361798,-6.71696965367645,
75.8422711443113));
#27996=CARTESIAN_POINT('Ctrl Pts',(1.01289232915633,-6.69304213281326,75.8504733068957));
#27997=CARTESIAN_POINT('Ctrl Pts',(1.18476645688375,-6.66247832586667,75.8586754694801));
#27998=CARTESIAN_POINT('Ctrl Pts',(1.35683740336337,-6.63187951929318,75.8668870246323));
#27999=CARTESIAN_POINT('Ctrl Pts',(1.5276157055801,-6.59462930720231,75.8750985797845));
#28000=CARTESIAN_POINT('Ctrl Pts',(1.69655971005235,-6.55087583077462,75.8833101349367));
#28001=CARTESIAN_POINT('Ctrl Pts',(1.86560396893598,-6.50709639024694,75.8915265629735));
#28002=CARTESIAN_POINT('Ctrl Pts',(2.03281141742198,-6.45680609585874,75.8997429910102));
#28003=CARTESIAN_POINT('Ctrl Pts',(2.19765751844408,-6.40020237427116,75.907959419047));
#28004=CARTESIAN_POINT('Ctrl Pts',(2.36275989240819,-6.34351065544149,75.9161886205019));
#28005=CARTESIAN_POINT('Ctrl Pts',(2.52549324862212,-6.28048602473466,75.9244178219569));
#28006=CARTESIAN_POINT('Ctrl Pts',(2.6853536801091,-6.21137381041622,75.9326470234118));
#28007=CARTESIAN_POINT('Ctrl Pts',(2.82977491730534,-6.14893639920448,75.9400814550858));
#28008=CARTESIAN_POINT('Ctrl Pts',(2.9718514988971,-6.08153118812264,75.9475158867598));
#28009=CARTESIAN_POINT('Ctrl Pts',(3.11123121399388,-6.00937012781457,75.9549503184337));
#28010=CARTESIAN_POINT('Ctrl Pts',(3.26423963955559,-5.93015307519732,75.9631116974737));
#28011=CARTESIAN_POINT('Ctrl Pts',(3.41446835462247,-5.84496017405954,75.9712730765136));
#28012=CARTESIAN_POINT('Ctrl Pts',(3.56141261819242,-5.75400983341007,75.9794344555535));
#28013=CARTESIAN_POINT('Ctrl Pts',(3.70817816975507,-5.66317010557085,75.9875859088134));
#28014=CARTESIAN_POINT('Ctrl Pts',(3.85166691434113,-5.56658706664381,75.9957373620734));
#28015=CARTESIAN_POINT('Ctrl Pts',(3.99139590383308,-5.46452630507572,76.0038888153333));
#28016=CARTESIAN_POINT('Ctrl Pts',(4.13098424279492,-5.36256827738032,76.0120320633795));
#28017=CARTESIAN_POINT('Ctrl Pts',(4.26682006869858,-5.25514371809648,76.0201753114257));
#28018=CARTESIAN_POINT('Ctrl Pts',(4.39844678641759,-5.14256306398403,76.0283185594719));
#28019=CARTESIAN_POINT('Ctrl Pts',(4.52996858175746,-5.03007215023948,76.0364553163667));
#28020=CARTESIAN_POINT('Ctrl Pts',(4.65728767356832,-4.91243356157915,76.0445920732614));
#28021=CARTESIAN_POINT('Ctrl Pts',(4.77997812395736,-4.78999980527026,76.0527288301562));
#28022=CARTESIAN_POINT('Ctrl Pts',(4.90259646587445,-4.66763800656731,76.0608608048604));
#28023=CARTESIAN_POINT('Ctrl Pts',(5.020591326389,-4.54048690999453,76.0689927795647));
#28024=CARTESIAN_POINT('Ctrl Pts',(5.1335714292822,-4.40893789709694,76.077124754269));
#28025=CARTESIAN_POINT('Ctrl Pts',(5.24681857948396,-4.27707794617628,76.0852759502511));
#28026=CARTESIAN_POINT('Ctrl Pts',(5.35502696583186,-4.14079951400846,76.0934271462333));
#28027=CARTESIAN_POINT('Ctrl Pts',(5.45784078059092,-4.00053284122487,76.1015783422155));
#28028=CARTESIAN_POINT('Ctrl Pts',(5.56037376191622,-3.86064930344557,76.1097072734042));
#28029=CARTESIAN_POINT('Ctrl Pts',(5.65754139674202,-3.71679958764573,76.1178362045929));
#28030=CARTESIAN_POINT('Ctrl Pts',(5.74903230606199,-3.56944204937628,76.1259651357815));
#28031=CARTESIAN_POINT('Ctrl Pts',(5.84053009743602,-3.4220734266991,76.134094678438));
#28032=CARTESIAN_POINT('Ctrl Pts',(5.92635012001298,-3.27119676626935,76.1422242210945));
#28033=CARTESIAN_POINT('Ctrl Pts',(6.00622549307182,-3.11729759990511,76.1503537637509));
#28034=CARTESIAN_POINT('Ctrl Pts',(6.08612202231604,-2.96335767104841,76.1584854596381));
#28035=CARTESIAN_POINT('Ctrl Pts',(6.16007059859276,-2.80639396625127,76.1666171555253));
#28036=CARTESIAN_POINT('Ctrl Pts',(6.22785129877049,-2.64691465680378,76.1747488514126));
#28037=CARTESIAN_POINT('Ctrl Pts',(6.29592669305193,-2.48674196986045,76.1829159019483));
#28038=CARTESIAN_POINT('Ctrl Pts',(6.35778031115257,-2.32403209590914,76.1910829524841));
#28039=CARTESIAN_POINT('Ctrl Pts',(6.41323926741714,-2.15931727609884,76.1992500030198));
#28040=CARTESIAN_POINT('Ctrl Pts',(6.46854518928777,-1.9950569731839,76.2073945172564));
#28041=CARTESIAN_POINT('Ctrl Pts',(6.51749164193093,-1.82880314043243,76.215539031493));
#28042=CARTESIAN_POINT('Ctrl Pts',(6.55995811662626,-1.66109557464622,76.2236835457296));
#28043=CARTESIAN_POINT('Ctrl Pts',(6.60260085177428,-1.49269192538062,76.231861864415));
#28044=CARTESIAN_POINT('Ctrl Pts',(6.63870963807863,-1.32282281502014,76.2400401831002));
#28045=CARTESIAN_POINT('Ctrl Pts',(6.66821487842452,-1.15204137736361,76.2482185017856));
#28046=CARTESIAN_POINT('Ctrl Pts',(6.69772011877043,-0.981259939707015,
76.2563968204709));
#28047=CARTESIAN_POINT('Ctrl Pts',(6.72062182365632,-0.809566545632992,
76.2645751391562));
#28048=CARTESIAN_POINT('Ctrl Pts',(6.73690308377848,-0.637515364345049,
76.2727534578415));
#28049=CARTESIAN_POINT('Ctrl Pts',(6.75327610140381,-0.464494541475684,
76.280977867683));
#28050=CARTESIAN_POINT('Ctrl Pts',(6.76300227069972,-0.290601008063937,
76.2892022775245));
#28051=CARTESIAN_POINT('Ctrl Pts',(6.76599905201254,-0.11638654632469,76.2974266873659));
#28052=CARTESIAN_POINT('Ctrl Pts',(6.76899247840497,0.0576328809457218,
76.3056418899155));
#28053=CARTESIAN_POINT('Ctrl Pts',(6.76527151208416,0.231972165641657,76.3138570924651));
#28054=CARTESIAN_POINT('Ctrl Pts',(6.75480521895299,0.406073212617499,76.3220722950146));
#28055=CARTESIAN_POINT('Ctrl Pts',(6.74434854016002,0.580014330349336,76.3302799510781));
#28056=CARTESIAN_POINT('Ctrl Pts',(6.7271588959771,0.753717290306709,76.3384876071415));
#28057=CARTESIAN_POINT('Ctrl Pts',(6.70325736954728,0.926622705101763,76.346695263205));
#28058=CARTESIAN_POINT('Ctrl Pts',(6.67937299859103,1.09940401592867,76.3548970281707));
#28059=CARTESIAN_POINT('Ctrl Pts',(6.64878638990511,1.27138856782977,76.3630987931365));
#28060=CARTESIAN_POINT('Ctrl Pts',(6.61157055828366,1.4420207185879,76.3713005581023));
#28061=CARTESIAN_POINT('Ctrl Pts',(6.57437396569766,1.61256465962842,76.3794980830971));
#28062=CARTESIAN_POINT('Ctrl Pts',(6.53055505368496,1.78175724261241,76.3876956080918));
#28063=CARTESIAN_POINT('Ctrl Pts',(6.48023818676576,1.94905157519826,76.3958931330866));
#28064=CARTESIAN_POINT('Ctrl Pts',(6.42993041616303,2.11631566420407,76.4040891761274));
#28065=CARTESIAN_POINT('Ctrl Pts',(6.373127127617,2.28168184128613,76.4122852191682));
#28066=CARTESIAN_POINT('Ctrl Pts',(6.31000303726401,2.44461667132477,76.420481262209));
#28067=CARTESIAN_POINT('Ctrl Pts',(6.24688320746188,2.60754050410187,76.4286767520591));
#28068=CARTESIAN_POINT('Ctrl Pts',(6.17744355427624,2.76803298173554,76.4368722419091));
#28069=CARTESIAN_POINT('Ctrl Pts',(6.1019075782321,2.92557907203235,76.4450677317593));
#28070=CARTESIAN_POINT('Ctrl Pts',(6.02636295823757,3.08314319109718,76.4532641594593));
#28071=CARTESIAN_POINT('Ctrl Pts',(5.94472078066831,3.23775992746542,76.4614605871593));
#28072=CARTESIAN_POINT('Ctrl Pts',(5.8572513118581,3.38893730684659,76.4696570148593));
#28073=CARTESIAN_POINT('Ctrl Pts',(5.76975592011947,3.5401594899797,76.4778558716973));
#28074=CARTESIAN_POINT('Ctrl Pts',(5.6764299768004,3.68793997528957,76.4860547285353));
#28075=CARTESIAN_POINT('Ctrl Pts',(5.57758804065649,3.83181427638733,76.4942535853733));
#28076=CARTESIAN_POINT('Ctrl Pts',(5.4786422249977,3.9758397844847,76.5024610589311));
#28077=CARTESIAN_POINT('Ctrl Pts',(5.37416903822127,4.11595061054609,76.5106685324889));
#28078=CARTESIAN_POINT('Ctrl Pts',(5.26452505114972,4.25171318244976,76.5188760060467));
#28079=CARTESIAN_POINT('Ctrl Pts',(5.15482171308313,4.38754924350633,76.5270879223627));
#28080=CARTESIAN_POINT('Ctrl Pts',(5.03994223078305,4.51903208828505,76.5352998386787));
#28081=CARTESIAN_POINT('Ctrl Pts',(4.92028120311269,4.64576386424192,76.5435117549948));
#28082=CARTESIAN_POINT('Ctrl Pts',(4.80044402700788,4.77268219721208,76.5517357597595));
#28083=CARTESIAN_POINT('Ctrl Pts',(4.6758114953634,4.89483523347394,76.5599597645243));
#28084=CARTESIAN_POINT('Ctrl Pts',(4.54681350183855,5.01186352363057,76.5681837692891));
#28085=CARTESIAN_POINT('Ctrl Pts',(4.4298368382441,5.11798594115522,76.575641378609));
#28086=CARTESIAN_POINT('Ctrl Pts',(4.30927101176112,5.21989465020696,76.5830989879291));
#28087=CARTESIAN_POINT('Ctrl Pts',(4.18545737387484,5.31735230838401,76.590556597249));
#28088=CARTESIAN_POINT('Ctrl Pts',(4.04914339526347,5.42464938291518,76.5987671337835));
#28089=CARTESIAN_POINT('Ctrl Pts',(3.9085045758614,5.52685577924727,76.606977670318));
#28090=CARTESIAN_POINT('Ctrl Pts',(3.76395772984268,5.62360304501994,76.6151882068525));
#28091=CARTESIAN_POINT('Ctrl Pts',(3.6195985629453,5.72022469447976,76.623388082855));
#28092=CARTESIAN_POINT('Ctrl Pts',(3.47134177445127,5.81140113485322,76.6315879588575));
#28093=CARTESIAN_POINT('Ctrl Pts',(3.31963737148585,5.89680394127484,76.6397878348599));
#28094=CARTESIAN_POINT('Ctrl Pts',(3.24692434436106,5.93773812946241,76.6437180952514));
#28095=CARTESIAN_POINT('Ctrl Pts',(3.17341976708094,5.97734650173748,76.6476483556429));
#28096=CARTESIAN_POINT('Ctrl Pts',(3.09917575053257,6.0155962852664,76.6515786160344));
#28097=CARTESIAN_POINT('Origin',(0.,0.,-3.69717978381041));
#28098=CARTESIAN_POINT('',(3.09917575053265,6.01559628526636,79.0457515827422));
#28099=CARTESIAN_POINT('',(3.09917575053268,6.01559628526634,78.6513920151221));
#28100=CARTESIAN_POINT('',(3.09917575053259,6.01559628526639,-3.69717978381041));
#28101=CARTESIAN_POINT('',(-6.76699915081304,0.00184116009375152,77.6971797838099));
#28102=CARTESIAN_POINT('Ctrl Pts',(-6.767,3.94374831596175E-12,77.6971797838099));
#28103=CARTESIAN_POINT('Ctrl Pts',(-6.76700000000011,-0.186007249411788,
77.7059292956159));
#28104=CARTESIAN_POINT('Ctrl Pts',(-6.75932637295459,-0.372014355523699,
77.7146788074218));
#28105=CARTESIAN_POINT('Ctrl Pts',(-6.74400518266959,-0.557389537151275,
77.7234283192278));
#28106=CARTESIAN_POINT('Ctrl Pts',(-6.72868405709685,-0.742763935807823,
77.7321777940783));
#28107=CARTESIAN_POINT('Ctrl Pts',(-6.70571545653038,-0.927506129691662,
77.7409272689289));
#28108=CARTESIAN_POINT('Ctrl Pts',(-6.67517739415703,-1.11098863924659,
77.7496767437794));
#28109=CARTESIAN_POINT('Ctrl Pts',(-6.64463945823127,-1.29447038906366,
77.7584261824014));
#28110=CARTESIAN_POINT('Ctrl Pts',(-6.60653217027184,-1.47669218228099,
77.7671756210234));
#28111=CARTESIAN_POINT('Ctrl Pts',(-6.56098496116737,-1.6570351050402,77.7759250596454));
#28112=CARTESIAN_POINT('Ctrl Pts',(-6.51543793687542,-1.83737729603934,
77.7846744627656));
#28113=CARTESIAN_POINT('Ctrl Pts',(-6.46245112202662,-2.01584035396981,
77.7934238658859));
#28114=CARTESIAN_POINT('Ctrl Pts',(-6.40220448416263,-2.19181813638084,
77.8021732690061));
#28115=CARTESIAN_POINT('Ctrl Pts',(-6.34195808575208,-2.36779521935886,
77.8109226373514));
#28116=CARTESIAN_POINT('Ctrl Pts',(-6.27445201489257,-2.54128677544771,
77.8196720056967));
#28117=CARTESIAN_POINT('Ctrl Pts',(-6.19991555136207,-2.71170355237786,
77.8284213740419));
#28118=CARTESIAN_POINT('Ctrl Pts',(-6.12537937789061,-2.88211966613023,
77.837170708339));
#28119=CARTESIAN_POINT('Ctrl Pts',(-6.04381298133639,-3.04946076210402,
77.845920042636));
#28120=CARTESIAN_POINT('Ctrl Pts',(-5.95549339426327,-3.21315848206817,
77.8546693769331));
#28121=CARTESIAN_POINT('Ctrl Pts',(-5.86717414355185,-3.37685557859594,
77.8634186779087));
#28122=CARTESIAN_POINT('Ctrl Pts',(-5.77210188986266,-3.53690907467265,
77.8721679788842));
#28123=CARTESIAN_POINT('Ctrl Pts',(-5.67059953467101,-3.69277536784855,
77.8809172798598));
#28124=CARTESIAN_POINT('Ctrl Pts',(-5.56909755761804,-3.84864108035737,
77.8896665482405));
#28125=CARTESIAN_POINT('Ctrl Pts',(-5.46116568338115,-4.00031938104218,
77.8984158166213));
#28126=CARTESIAN_POINT('Ctrl Pts',(-5.34717048686166,-4.14729511663152,
77.9071650850021));
#28127=CARTESIAN_POINT('Ctrl Pts',(-5.23317570555561,-4.29427031687988,
77.9159143215147));
#28128=CARTESIAN_POINT('Ctrl Pts',(-5.1131178217884,-4.4365427598709,77.9246635580273));
#28129=CARTESIAN_POINT('Ctrl Pts',(-4.98740459172039,-4.57362924147623,
77.9334127945399));
#28130=CARTESIAN_POINT('Ctrl Pts',(-4.86169180910849,-4.71071523514417,
77.9421619999111));
#28131=CARTESIAN_POINT('Ctrl Pts',(-4.73032391415444,-4.84261509316512,
77.9509112052822));
#28132=CARTESIAN_POINT('Ctrl Pts',(-4.59374707237299,-4.96888084331518,
77.9596604106533));
#28133=CARTESIAN_POINT('Ctrl Pts',(-4.45717070537422,-5.09514615452706,
77.9684095856095));
#28134=CARTESIAN_POINT('Ctrl Pts',(-4.31538563819543,-5.21577720253604,
77.9771587605657));
#28135=CARTESIAN_POINT('Ctrl Pts',(-4.16887341290698,-5.33036429028611,
77.985907935522));
#28136=CARTESIAN_POINT('Ctrl Pts',(-4.02236168477371,-5.44495098921153,
77.9946570807899));
#28137=CARTESIAN_POINT('Ctrl Pts',(-3.87112305634454,-5.55349359238749,
78.0034062260578));
#28138=CARTESIAN_POINT('Ctrl Pts',(-3.71567117316729,-5.65562346102476,
78.0121553713258));
#28139=CARTESIAN_POINT('Ctrl Pts',(-3.56021980457292,-5.75775299158775,
78.0209044876319));
#28140=CARTESIAN_POINT('Ctrl Pts',(-3.40055544862373,-5.85346967275362,
78.0296536039381));
#28141=CARTESIAN_POINT('Ctrl Pts',(-3.23722036323383,-5.94244842803572,
78.0384027202443));
#28142=CARTESIAN_POINT('Ctrl Pts',(-3.07388580496003,-6.03142689616499,
78.0471518083152));
#28143=CARTESIAN_POINT('Ctrl Pts',(-2.90688079257638,-6.11366734484856,
78.0559008963862));
#28144=CARTESIAN_POINT('Ctrl Pts',(-2.7367725109452,-6.18889046787344,78.0646499844571));
#28145=CARTESIAN_POINT('Ctrl Pts',(-2.56666476416548,-6.2641133543831,78.0733990450194));
#28146=CARTESIAN_POINT('Ctrl Pts',(-2.39345402971993,-6.33231884350328,
78.0821481055816));
#28147=CARTESIAN_POINT('Ctrl Pts',(-2.21772856473936,-6.39327529621079,
78.0908971661438));
#28148=CARTESIAN_POINT('Ctrl Pts',(-2.04200363768182,-6.45423156232109,
78.0996461999238));
#28149=CARTESIAN_POINT('Ctrl Pts',(-1.8637642662002,-6.50793874252076,78.1083952337038));
#28150=CARTESIAN_POINT('Ctrl Pts',(-1.6836157819463,-6.55421443796138,78.1171442674838));
#28151=CARTESIAN_POINT('Ctrl Pts',(-1.50346783419841,-6.60048999558685,
78.125893275208));
#28152=CARTESIAN_POINT('Ctrl Pts',(-1.32141106257251,-6.63933404145494,
78.1346422829322));
#28153=CARTESIAN_POINT('Ctrl Pts',(-1.13806375959081,-6.67061465527024,
78.1433912906564));
#28154=CARTESIAN_POINT('Ctrl Pts',(-0.954716987419649,-6.70189517852473,
78.1521402730513));
#28155=CARTESIAN_POINT('Ctrl Pts',(-0.770079973810508,-6.7256122653582,
78.1608892554462));
#28156=CARTESIAN_POINT('Ctrl Pts',(-0.584779770553222,-6.74168536939775,
78.1696382378411));
#28157=CARTESIAN_POINT('Ctrl Pts',(-0.391490647554734,-6.75845143942389,
78.1787644185171));
#28158=CARTESIAN_POINT('Ctrl Pts',(-0.197480213105212,-6.76689975924024,
78.1878905991932));
#28159=CARTESIAN_POINT('Ctrl Pts',(-0.00346532629872835,-6.76699911271707,
78.1970167798692));
#28160=CARTESIAN_POINT('Ctrl Pts',(0.184486595295083,-6.76709536139776,
78.2058577673991));
#28161=CARTESIAN_POINT('Ctrl Pts',(0.372442378184217,-6.75935659726775,
78.2146987549291));
#28162=CARTESIAN_POINT('Ctrl Pts',(0.559750217721036,-6.74380965729025,
78.223539742459));
#28163=CARTESIAN_POINT('Ctrl Pts',(0.745129914456703,-6.72842275717265,
78.2322897210568));
#28164=CARTESIAN_POINT('Ctrl Pts',(0.929874656313132,-6.70538772273487,
78.2410396996546));
#28165=CARTESIAN_POINT('Ctrl Pts',(1.11335688289672,-6.6747828018076,78.2497896782523));
#28166=CARTESIAN_POINT('Ctrl Pts',(1.29683723118751,-6.64417819418044,78.2585395672773));
#28167=CARTESIAN_POINT('Ctrl Pts',(1.4790548073013,-6.60600390230099,78.2672894563022));
#28168=CARTESIAN_POINT('Ctrl Pts',(1.65939064804703,-6.56038959797161,78.2760393453271));
#28169=CARTESIAN_POINT('Ctrl Pts',(1.83972470264153,-6.51477574543287,78.2847891476881));
#28170=CARTESIAN_POINT('Ctrl Pts',(2.01817678125729,-6.46172209820137,78.293538950049));
#28171=CARTESIAN_POINT('Ctrl Pts',(2.19414072347555,-6.40140886724057,78.30228875241));
#28172=CARTESIAN_POINT('Ctrl Pts',(2.37010298131968,-6.34109621361422,78.3110384710155));
#28173=CARTESIAN_POINT('Ctrl Pts',(2.54357687926781,-6.27352420826024,78.3197881896209));
#28174=CARTESIAN_POINT('Ctrl Pts',(2.71397317789835,-6.19892237325556,78.3285379082264));
#28175=CARTESIAN_POINT('Ctrl Pts',(2.8843679020706,-6.1243212275703,78.3372875459847));
#28176=CARTESIAN_POINT('Ctrl Pts',(3.0516848212611,-6.04269049717491,78.3460371837429));
#28177=CARTESIAN_POINT('Ctrl Pts',(3.21535561997237,-5.95430745235011,78.3547868215012));
#28178=CARTESIAN_POINT('Ctrl Pts',(3.37902496075119,-5.86592519481609,78.3635363813202));
#28179=CARTESIAN_POINT('Ctrl Pts',(3.53904799384704,-5.77079087940336,78.3722859411392));
#28180=CARTESIAN_POINT('Ctrl Pts',(3.69488118814804,-5.66922763747141,78.3810355009582));
#28181=CARTESIAN_POINT('Ctrl Pts',(3.85071304610658,-5.56766526649173,78.3897849857457));
#28182=CARTESIAN_POINT('Ctrl Pts',(4.00235489705798,-5.45967423580838,78.3985344705331));
#28183=CARTESIAN_POINT('Ctrl Pts',(4.14929168607489,-5.34562133936456,78.4072839553205));
#28184=CARTESIAN_POINT('Ctrl Pts',(4.29622726385596,-5.23156938308663,78.4160333679838));
#28185=CARTESIAN_POINT('Ctrl Pts',(4.4384576309191,-5.11145583677338,78.4247827806471));
#28186=CARTESIAN_POINT('Ctrl Pts',(4.57549970660809,-4.98568866204352,78.4335321933104));
#28187=CARTESIAN_POINT('Ctrl Pts',(4.71254069815148,-4.85992248226304,78.4422815367568));
#28188=CARTESIAN_POINT('Ctrl Pts',(4.84439326931173,-4.72850295734146,78.4510308802031));
#28189=CARTESIAN_POINT('Ctrl Pts',(4.97060959434564,-4.59187644221827,78.4597802236494));
#28190=CARTESIAN_POINT('Ctrl Pts',(5.0968249628039,-4.45525096256808,78.4685295007857));
#28191=CARTESIAN_POINT('Ctrl Pts',(5.21740397615722,-4.31341878218468,78.477278777922));
#28192=CARTESIAN_POINT('Ctrl Pts',(5.33193710451825,-4.16686161438817,78.4860280550583));
#28193=CARTESIAN_POINT('Ctrl Pts',(5.44646940289274,-4.02030550864661,78.4947772687913));
#28194=CARTESIAN_POINT('Ctrl Pts',(5.55495572749557,-3.86902470980288,78.5035264825242));
#28195=CARTESIAN_POINT('Ctrl Pts',(5.65702762491349,-3.71353301465944,78.5122756962572));
#28196=CARTESIAN_POINT('Ctrl Pts',(5.75909881655046,-3.55804239467067,78.5210248494933));
#28197=CARTESIAN_POINT('Ctrl Pts',(5.85475551250674,-3.39834117619739,78.5297740027294));
#28198=CARTESIAN_POINT('Ctrl Pts',(5.94367283727987,-3.23497174692167,78.5385231559655));
#28199=CARTESIAN_POINT('Ctrl Pts',(6.03258957676211,-3.07160339301163,78.5472722516111));
#28200=CARTESIAN_POINT('Ctrl Pts',(6.11476689685191,-2.904567128297,78.5560213472566));
#28201=CARTESIAN_POINT('Ctrl Pts',(6.18992570525175,-2.734430244761,78.5647704429021));
#28202=CARTESIAN_POINT('Ctrl Pts',(6.26508404388619,-2.56429442463221,78.5735194838632));
#28203=CARTESIAN_POINT('Ctrl Pts',(6.33322384283244,-2.3910582865618,78.5822685248242));
#28204=CARTESIAN_POINT('Ctrl Pts',(6.39411368719969,-2.21531017132265,78.5910175657852));
#28205=CARTESIAN_POINT('Ctrl Pts',(6.45500317120838,-2.03956309619679,78.5997665549676));
#28206=CARTESIAN_POINT('Ctrl Pts',(6.50864269270032,-1.86130434438778,78.6085155441501));
#28207=CARTESIAN_POINT('Ctrl Pts',(6.55485008446302,-1.68113930720069,78.6172645333325));
#28208=CARTESIAN_POINT('Ctrl Pts',(6.60199664749377,-1.4973123921196,78.6261913468618));
#28209=CARTESIAN_POINT('Ctrl Pts',(6.64140563640884,-1.31150116499787,78.6351181603912));
#28210=CARTESIAN_POINT('Ctrl Pts',(6.67293772282154,-1.12436255155771,78.6440449739206));
#28211=CARTESIAN_POINT('Ctrl Pts',(6.70384494949854,-0.94093239505252,78.6527948880761));
#28212=CARTESIAN_POINT('Ctrl Pts',(6.72718449348916,-0.756227260507957,
78.6615448022316));
#28213=CARTESIAN_POINT('Ctrl Pts',(6.74287707373921,-0.570874564542999,
78.6702947163872));
#28214=CARTESIAN_POINT('Ctrl Pts',(6.75856934538663,-0.38552551363374,78.6790444584711));
#28215=CARTESIAN_POINT('Ctrl Pts',(6.766614930041,-0.19952921241945,78.6877942005551));
#28216=CARTESIAN_POINT('Ctrl Pts',(6.76698649908906,-0.0135174386016032,
78.6965439426391));
#28217=CARTESIAN_POINT('Ctrl Pts',(6.76735806132392,0.172490924444679,78.705293524285));
#28218=CARTESIAN_POINT('Ctrl Pts',(6.76005588896295,0.358514472900385,78.7140431059309));
#28219=CARTESIAN_POINT('Ctrl Pts',(6.74510478454592,0.543921359661268,78.7227926875768));
#28220=CARTESIAN_POINT('Ctrl Pts',(6.73015393440698,0.729325093149558,78.7315421204158));
#28221=CARTESIAN_POINT('Ctrl Pts',(6.70755443556909,0.914111900255522,78.7402915532549));
#28222=CARTESIAN_POINT('Ctrl Pts',(6.67738304682331,1.09765415591461,78.7490409860939));
#28223=CARTESIAN_POINT('Ctrl Pts',(6.64721213111874,1.28119353391204,78.7577902817553));
#28224=CARTESIAN_POINT('Ctrl Pts',(6.60946960955508,1.46348811672592,78.7665395774166));
#28225=CARTESIAN_POINT('Ctrl Pts',(6.56428366991196,1.64391876348169,78.7752888730779));
#28226=CARTESIAN_POINT('Ctrl Pts',(6.51909837867733,1.8243468210966,78.7840380431888));
#28227=CARTESIAN_POINT('Ctrl Pts',(6.46646995271939,2.00291071820387,78.7927872132996));
#28228=CARTESIAN_POINT('Ctrl Pts',(6.40657713281569,2.17900400212644,78.8015363834104));
#28229=CARTESIAN_POINT('Ctrl Pts',(6.34668509279078,2.3550949930961,78.8102854395962));
#28230=CARTESIAN_POINT('Ctrl Pts',(6.27952894037541,2.52871516398086,78.819034495782));
#28231=CARTESIAN_POINT('Ctrl Pts',(6.20533675061458,2.69927486771394,78.8277835519678));
#28232=CARTESIAN_POINT('Ctrl Pts',(6.12832117907928,2.87632521635899,78.83686555325));
#28233=CARTESIAN_POINT('Ctrl Pts',(6.04372366626091,3.05007728919975,78.8459475545323));
#28234=CARTESIAN_POINT('Ctrl Pts',(5.95185378007879,3.21989527478174,78.8550295558146));
#28235=CARTESIAN_POINT('Ctrl Pts',(5.86334450817379,3.38350129286738,78.8637793361217));
#28236=CARTESIAN_POINT('Ctrl Pts',(5.7680856205726,3.54345567124955,78.8725291164288));
#28237=CARTESIAN_POINT('Ctrl Pts',(5.66640068804484,3.69921508465309,78.8812788967359));
#28238=CARTESIAN_POINT('Ctrl Pts',(5.5647194110792,3.85496889852288,78.8900283624894));
#28239=CARTESIAN_POINT('Ctrl Pts',(5.45661270815107,4.00652780919646,78.8987778282429));
#28240=CARTESIAN_POINT('Ctrl Pts',(5.34244776449103,4.15337704569243,78.9075272939964));
#28241=CARTESIAN_POINT('Ctrl Pts',(5.22828631819585,4.30022178356262,78.916276491716));
#28242=CARTESIAN_POINT('Ctrl Pts',(5.1080671784406,4.4423569097269,78.9250256894356));
#28243=CARTESIAN_POINT('Ctrl Pts',(4.98219864544711,4.57929969070654,78.9337748871552));
#28244=CARTESIAN_POINT('Ctrl Pts',(4.85633329944008,4.71623900430018,78.9425238633454));
#28245=CARTESIAN_POINT('Ctrl Pts',(4.72481904033624,4.84798602483641,78.9512728395357));
#28246=CARTESIAN_POINT('Ctrl Pts',(4.58810250737165,4.97409332259156,78.9600218157259));
#28247=CARTESIAN_POINT('Ctrl Pts',(4.45137708685612,5.10020881822161,78.9687713606621));
#28248=CARTESIAN_POINT('Ctrl Pts',(4.30944892636025,5.22068366307955,78.9775209055983));
#28249=CARTESIAN_POINT('Ctrl Pts',(4.16280009466638,5.33510865604868,78.9862704505344));
#28250=CARTESIAN_POINT('Ctrl Pts',(4.01615988348763,5.44952692272911,78.9950194811427));
#28251=CARTESIAN_POINT('Ctrl Pts',(3.86479978232201,5.55789587288647,79.003768511751));
#28252=CARTESIAN_POINT('Ctrl Pts',(3.70923383581034,5.659847467139,79.0125175423593));
#28253=CARTESIAN_POINT('Ctrl Pts',(3.55366577799509,5.76180044505402,79.0212666917073));
#28254=CARTESIAN_POINT('Ctrl Pts',(3.39389200026811,5.85733573571076,79.0300158410553));
#28255=CARTESIAN_POINT('Ctrl Pts',(3.23045513626015,5.94612887621942,79.0387649904033));
#28256=CARTESIAN_POINT('Ctrl Pts',(3.18695122151563,5.96976399206696,79.0410938545163));
#28257=CARTESIAN_POINT('Ctrl Pts',(3.1431879126266,5.99292165435335,79.0434227186292));
#28258=CARTESIAN_POINT('Ctrl Pts',(3.09917575053266,6.01559628526635,79.0457515827422));
#28259=CARTESIAN_POINT('Ctrl Pts',(3.09917575053268,6.01559628526634,77.0459357433347));
#28260=CARTESIAN_POINT('Ctrl Pts',(2.94459599297447,6.09523424855869,77.0541212456873));
#28261=CARTESIAN_POINT('Ctrl Pts',(2.78680153118066,6.16898384532002,77.0623067480399));
#28262=CARTESIAN_POINT('Ctrl Pts',(2.62628284950005,6.23657978337662,77.0704922503925));
#28263=CARTESIAN_POINT('Ctrl Pts',(2.46587183064077,6.30413038359885,77.0786722625786));
#28264=CARTESIAN_POINT('Ctrl Pts',(2.30274056247645,6.3655354062191,77.0868522747648));
#28265=CARTESIAN_POINT('Ctrl Pts',(2.13740267681911,6.4205762044482,77.095032286951));
#28266=CARTESIAN_POINT('Ctrl Pts',(1.97214201399145,6.4755912952832,77.1032084785748));
#28267=CARTESIAN_POINT('Ctrl Pts',(1.80467712843983,6.5242479695393,77.1113846701988));
#28268=CARTESIAN_POINT('Ctrl Pts',(1.63554016630024,6.56637627344174,77.1195608618226));
#28269=CARTESIAN_POINT('Ctrl Pts',(1.4664221967583,6.60849984670508,77.1277361353319));
#28270=CARTESIAN_POINT('Ctrl Pts',(1.29563287264218,6.64409641530863,77.1359114088412));
#28271=CARTESIAN_POINT('Ctrl Pts',(1.12371828957322,6.67304624633148,77.1440866823505));
#28272=CARTESIAN_POINT('Ctrl Pts',(0.951806553853321,6.70199559787043,77.1522618204561));
#28273=CARTESIAN_POINT('Ctrl Pts',(0.778769952066066,6.72429837035717,77.1604369585617));
#28274=CARTESIAN_POINT('Ctrl Pts',(0.605163411855234,6.73988621899152,77.1686120966674));
#28275=CARTESIAN_POINT('Ctrl Pts',(0.4315277147346,6.75547668557733,77.176788607773));
#28276=CARTESIAN_POINT('Ctrl Pts',(0.257322247994863,6.7643499497148,77.1849651188785));
#28277=CARTESIAN_POINT('Ctrl Pts',(0.083105707101584,6.76648966905641,77.1931416299841));
#28278=CARTESIAN_POINT('Ctrl Pts',(-0.0911722384356991,6.76863014256697,
77.201321022996));
#28279=CARTESIAN_POINT('Ctrl Pts',(-0.265460905273268,6.76403233996544,
77.2095004160079));
#28280=CARTESIAN_POINT('Ctrl Pts',(-0.439202930077307,6.7527320238709,77.2176798090198));
#28281=CARTESIAN_POINT('Ctrl Pts',(-0.613132562637829,6.74141950562231,
77.2258680341929));
#28282=CARTESIAN_POINT('Ctrl Pts',(-0.786514013848733,6.72339004167877,
77.234056259366));
#28283=CARTESIAN_POINT('Ctrl Pts',(-0.958795441472268,6.69873124564734,
77.2422444845391));
#28284=CARTESIAN_POINT('Ctrl Pts',(-1.13117954412829,6.67405775364596,77.2504375896711));
#28285=CARTESIAN_POINT('Ctrl Pts',(-1.30246196237958,6.64274711990887,77.2586306948031));
#28286=CARTESIAN_POINT('Ctrl Pts',(-1.47210251455571,6.60493778824894,77.2668237999351));
#28287=CARTESIAN_POINT('Ctrl Pts',(-1.64198104633278,6.56707541591244,77.2750283987334));
#28288=CARTESIAN_POINT('Ctrl Pts',(-1.81021276293874,6.52269622631456,77.2832329975316));
#28289=CARTESIAN_POINT('Ctrl Pts',(-1.97627306419992,6.47198839428177,77.2914375963299));
#28290=CARTESIAN_POINT('Ctrl Pts',(-2.07599484862549,6.44153755530184,77.296364585059));
#28291=CARTESIAN_POINT('Ctrl Pts',(-2.17493394727849,6.40880542593423,77.301291573788));
#28292=CARTESIAN_POINT('Ctrl Pts',(-2.27298060169066,6.37384092869739,77.3062185625171));
#28293=CARTESIAN_POINT('Ctrl Pts',(-2.43661332190611,6.31548773114942,77.314441347609));
#28294=CARTESIAN_POINT('Ctrl Pts',(-2.59822931702284,6.25074650535034,77.3226641327008));
#28295=CARTESIAN_POINT('Ctrl Pts',(-2.75729380899212,6.17977506474902,77.3308869177927));
#28296=CARTESIAN_POINT('Ctrl Pts',(-2.91617773354826,6.10888418976783,77.3391003685132));
#28297=CARTESIAN_POINT('Ctrl Pts',(-3.07251559759457,6.03177732774177,77.3473138192338));
#28298=CARTESIAN_POINT('Ctrl Pts',(-3.22578865161336,5.94866174657145,77.3555272699543));
#28299=CARTESIAN_POINT('Ctrl Pts',(-3.37891855779665,5.8656237903667,77.3637330498047));
#28300=CARTESIAN_POINT('Ctrl Pts',(-3.52898904074577,5.77658846088174,77.3719388296551));
#28301=CARTESIAN_POINT('Ctrl Pts',(-3.6755021087829,5.68181073675747,77.3801446095055));
#28302=CARTESIAN_POINT('Ctrl Pts',(-3.82190781754906,5.58710246218812,77.3883443764688));
#28303=CARTESIAN_POINT('Ctrl Pts',(-3.96476100329072,5.48666036821466,77.396544143432));
#28304=CARTESIAN_POINT('Ctrl Pts',(-4.10358896683244,5.38078494192911,77.4047439103953));
#28305=CARTESIAN_POINT('Ctrl Pts',(-4.24234312501469,5.2749658023865,77.4129393181017));
#28306=CARTESIAN_POINT('Ctrl Pts',(-4.37707603927068,5.16371930204179,77.4211347258082));
#28307=CARTESIAN_POINT('Ctrl Pts',(-4.50734459841955,5.04738879729887,77.4293301335146));
#28308=CARTESIAN_POINT('Ctrl Pts',(-4.63758693772306,4.93108170701501,77.4375238916877));
#28309=CARTESIAN_POINT('Ctrl Pts',(-4.76336644023871,4.80969288494777,77.4457176498609));
#28310=CARTESIAN_POINT('Ctrl Pts',(-4.8842734404309,4.68360565794147,77.453911408034));
#28311=CARTESIAN_POINT('Ctrl Pts',(-5.00517072295319,4.55752856495593,77.4621045076495));
#28312=CARTESIAN_POINT('Ctrl Pts',(-5.12119603392262,4.42675407760548,77.4702976072649));
#28313=CARTESIAN_POINT('Ctrl Pts',(-5.23197696954709,4.29170199223209,77.4784907068804));
#28314=CARTESIAN_POINT('Ctrl Pts',(-5.34276918852648,4.1566361514178,77.4866846409864));
#28315=CARTESIAN_POINT('Ctrl Pts',(-5.44831574020577,4.01729212222537,77.4948785750925));
#28316=CARTESIAN_POINT('Ctrl Pts',(-5.54828485420199,3.87412237502028,77.5030725091986));
#28317=CARTESIAN_POINT('Ctrl Pts',(-5.64828236738323,3.73091195621196,77.5112687710341));
#28318=CARTESIAN_POINT('Ctrl Pts',(-5.74269908143153,3.58387394896211,77.5194650328696));
#28319=CARTESIAN_POINT('Ctrl Pts',(-5.83124683478272,3.43348938426151,77.5276612947051));
#28320=CARTESIAN_POINT('Ctrl Pts',(-5.91988642150887,3.28294885487978,77.5358660569301));
#28321=CARTESIAN_POINT('Ctrl Pts',(-6.0026447046072,3.12905514378719,77.544070819155));
#28322=CARTESIAN_POINT('Ctrl Pts',(-6.07927927952005,2.97231432415857,77.5522755813799));
#28323=CARTESIAN_POINT('Ctrl Pts',(-6.15595455676992,2.81549025597441,77.5604847013376));
#28324=CARTESIAN_POINT('Ctrl Pts',(-6.2264994970635,2.65581639285271,77.5686938212953));
#28325=CARTESIAN_POINT('Ctrl Pts',(-6.29072012717906,2.49381821340374,77.576902941253));
#28326=CARTESIAN_POINT('Ctrl Pts',(-6.35503500880818,2.33158228210496,77.5851241090835));
#28327=CARTESIAN_POINT('Ctrl Pts',(-6.41300691173094,2.16701555591936,77.593345276914));
#28328=CARTESIAN_POINT('Ctrl Pts',(-6.46449157378496,2.00065931444194,77.6015664447444));
#28329=CARTESIAN_POINT('Ctrl Pts',(-6.51226066621631,1.84630874946532,77.6091943034177));
#28330=CARTESIAN_POINT('Ctrl Pts',(-6.55444556182836,1.69041800057974,77.6168221620909));
#28331=CARTESIAN_POINT('Ctrl Pts',(-6.59097066947956,1.53342578368182,77.6244500207641));
#28332=CARTESIAN_POINT('Ctrl Pts',(-6.64384035882495,1.30618128610771,77.635491261827));
#28333=CARTESIAN_POINT('Ctrl Pts',(-6.68498080346422,1.07608419429346,77.6465325028899));
#28334=CARTESIAN_POINT('Ctrl Pts',(-6.71413982814934,0.844165486180697,
77.6575737439527));
#28335=CARTESIAN_POINT('Ctrl Pts',(-6.74253161918314,0.618349034201611,
77.668324467353));
#28336=CARTESIAN_POINT('Ctrl Pts',(-6.75956428101389,0.390805215452577,
77.6790751907532));
#28337=CARTESIAN_POINT('Ctrl Pts',(-6.7650483845779,0.162509551473162,77.6898259141535));
#28338=CARTESIAN_POINT('Ctrl Pts',(-6.76629882392945,0.110455486721055,
77.692277204039));
#28339=CARTESIAN_POINT('Ctrl Pts',(-6.766949042737,0.0583624462839173,77.6947284939244));
#28340=CARTESIAN_POINT('Ctrl Pts',(-6.76699712094732,0.00624220238653553,
77.6971797838099));
#28341=CARTESIAN_POINT('',(-6.767,3.76644462146691E-12,77.3028202161898));
#28342=CARTESIAN_POINT('Ctrl Pts',(3.09917575053257,6.0155962852664,76.6515786160344));
#28343=CARTESIAN_POINT('Ctrl Pts',(2.94447999371585,6.09529401023024,76.6597677554965));
#28344=CARTESIAN_POINT('Ctrl Pts',(2.78657234059765,6.16909059992118,76.6679568949587));
#28345=CARTESIAN_POINT('Ctrl Pts',(2.6259447762783,6.2367221384263,76.6761460344209));
#28346=CARTESIAN_POINT('Ctrl Pts',(2.46541858317967,6.30431099501909,76.6843300057597));
#28347=CARTESIAN_POINT('Ctrl Pts',(2.30217622891919,6.36574241074283,76.6925139770985));
#28348=CARTESIAN_POINT('Ctrl Pts',(2.13673265208952,6.42079921610188,76.7006979484374));
#28349=CARTESIAN_POINT('Ctrl Pts',(1.97135990103597,6.47583245184858,76.7088784162487));
#28350=CARTESIAN_POINT('Ctrl Pts',(1.80378814606259,6.52449640038739,76.71705888406));
#28351=CARTESIAN_POINT('Ctrl Pts',(1.63455064267454,6.56662266287109,76.7252393518714));
#28352=CARTESIAN_POINT('Ctrl Pts',(1.46532381932214,6.60874626690159,76.7334193034396));
#28353=CARTESIAN_POINT('Ctrl Pts',(1.29443180442709,6.64433291168642,76.7415992550078));
#28354=CARTESIAN_POINT('Ctrl Pts',(1.12242162302429,6.67326447101923,76.7497792065761));
#28355=CARTESIAN_POINT('Ctrl Pts',(0.950408413126966,6.70219653973508,76.7579593021645));
#28356=CARTESIAN_POINT('Ctrl Pts',(0.777277352866236,6.72447322915449,76.766139397753));
#28357=CARTESIAN_POINT('Ctrl Pts',(0.603584097146813,6.74002783656503,76.7743194933414));
#28358=CARTESIAN_POINT('Ctrl Pts',(0.429855836852966,6.75558557871106,76.7825012374727));
#28359=CARTESIAN_POINT('Ctrl Pts',(0.255565514406007,6.76441850834548,76.7906829816039));
#28360=CARTESIAN_POINT('Ctrl Pts',(0.0812723540308919,6.76651193780594,
76.7988647257352));
#28361=CARTESIAN_POINT('Ctrl Pts',(-0.0930879890354412,6.76860617419551,
76.807049623585));
#28362=CARTESIAN_POINT('Ctrl Pts',(-0.267450812114449,6.76395573194799,
76.8152345214349));
#28363=CARTESIAN_POINT('Ctrl Pts',(-0.441258415564034,6.75259801933255,
76.8234194192848));
#28364=CARTESIAN_POINT('Ctrl Pts',(-0.615256595147889,6.74122785324028,
76.8316132916914));
#28365=CARTESIAN_POINT('Ctrl Pts',(-0.788697979502679,6.72313575241151,
76.839807164098));
#28366=CARTESIAN_POINT('Ctrl Pts',(-0.961030600080398,6.69841094482185,
76.8480010365045));
#28367=CARTESIAN_POINT('Ctrl Pts',(-1.1334708175112,6.67367070015776,76.856200024802));
#28368=CARTESIAN_POINT('Ctrl Pts',(-1.3048005379438,6.64228956004986,76.8643990130995));
#28369=CARTESIAN_POINT('Ctrl Pts',(-1.47447963245551,6.60440752933023,76.872598001397));
#28370=CARTESIAN_POINT('Ctrl Pts',(-1.64439086219489,6.56647367281645,76.8808082065978));
#28371=CARTESIAN_POINT('Ctrl Pts',(-1.81264660864914,6.5220212548482,76.8890184117987));
#28372=CARTESIAN_POINT('Ctrl Pts',(-1.97872258860794,6.47123990571612,76.8972286169996));
#28373=CARTESIAN_POINT('Ctrl Pts',(-2.05377599510466,6.44829069150821,76.9009389902187));
#28374=CARTESIAN_POINT('Ctrl Pts',(-2.12838449552966,6.42404954884372,76.9046493634377));
#28375=CARTESIAN_POINT('Ctrl Pts',(-2.2025011858424,6.39853713956267,76.9083597366568));
#28376=CARTESIAN_POINT('Ctrl Pts',(-2.36615894309163,6.34220294995783,76.9165526464727));
#28377=CARTESIAN_POINT('Ctrl Pts',(-2.52789770493843,6.27950189926979,76.9247455562885));
#28378=CARTESIAN_POINT('Ctrl Pts',(-2.68718362870622,6.21058235156843,76.9329384661044));
#28379=CARTESIAN_POINT('Ctrl Pts',(-2.8462856811994,6.14174236096027,76.9411219184571));
#28380=CARTESIAN_POINT('Ctrl Pts',(-3.00294020397036,6.06669830728647,76.9493053708098));
#28381=CARTESIAN_POINT('Ctrl Pts',(-3.15662855968243,5.9856482636551,76.9574888231624));
#28382=CARTESIAN_POINT('Ctrl Pts',(-3.31017106484937,5.90467513667099,76.965664509403));
#28383=CARTESIAN_POINT('Ctrl Pts',(-3.46075269009441,5.81770753676374,76.9738401956437));
#28384=CARTESIAN_POINT('Ctrl Pts',(-3.60787479708822,5.72499156755149,76.9820158818843));
#28385=CARTESIAN_POINT('Ctrl Pts',(-3.75488748420434,5.6323445544616,76.9901854875799));
#28386=CARTESIAN_POINT('Ctrl Pts',(-3.8984454723192,5.53395787845469,76.9983550932755));
#28387=CARTESIAN_POINT('Ctrl Pts',(-4.03807472580735,5.43012352610839,77.0065246989712));
#28388=CARTESIAN_POINT('Ctrl Pts',(-4.17762878587552,5.32634509084158,77.0146899051547));
#28389=CARTESIAN_POINT('Ctrl Pts',(-4.3132580358509,5.21712503821022,77.0228551113383));
#28390=CARTESIAN_POINT('Ctrl Pts',(-4.44451741051006,5.10279864267374,77.0310203175218));
#28391=CARTESIAN_POINT('Ctrl Pts',(-4.57575070407425,4.9884949636677,77.0391839012878));
#28392=CARTESIAN_POINT('Ctrl Pts',(-4.70261557471194,4.86908719503985,77.0473474850537));
#28393=CARTESIAN_POINT('Ctrl Pts',(-4.82469985157451,4.74495103686191,77.0555110688196));
#28394=CARTESIAN_POINT('Ctrl Pts',(-4.94677460385563,4.62082456334592,77.0636740156918));
#28395=CARTESIAN_POINT('Ctrl Pts',(-5.06406925049367,4.49197069223053,77.071836962564));
#28396=CARTESIAN_POINT('Ctrl Pts',(-5.17620841174312,4.3588020691699,77.0799999094361));
#28397=CARTESIAN_POINT('Ctrl Pts',(-5.28835967056454,4.22561907987909,77.0881637369269));
#28398=CARTESIAN_POINT('Ctrl Pts',(-5.39535410282002,4.08812068833179,77.0963275644177));
#28399=CARTESIAN_POINT('Ctrl Pts',(-5.49685656544128,3.94675270304146,77.1044913919085));
#28400=CARTESIAN_POINT('Ctrl Pts',(-5.59838884747007,3.80534318664484,77.1126576177697));
#28401=CARTESIAN_POINT('Ctrl Pts',(-5.69442573548572,3.66006210641259,77.1208238436309));
#28402=CARTESIAN_POINT('Ctrl Pts',(-5.78467536991784,3.51138432312185,77.1289900694921));
#28403=CARTESIAN_POINT('Ctrl Pts',(-5.87502156397725,3.36254746692816,77.1371650325379));
#28404=CARTESIAN_POINT('Ctrl Pts',(-5.95956794621117,3.210306957146,77.1453399955838));
#28405=CARTESIAN_POINT('Ctrl Pts',(-6.03806813568016,3.05516320167743,77.1535149586297));
#28406=CARTESIAN_POINT('Ctrl Pts',(-6.11661113729133,2.89993483448296,77.1616943801066));
#28407=CARTESIAN_POINT('Ctrl Pts',(-6.1891012231642,2.74180039441464,77.1698738015835));
#28408=CARTESIAN_POINT('Ctrl Pts',(-6.2553402552646,2.58128016512471,77.1780532230604));
#28409=CARTESIAN_POINT('Ctrl Pts',(-6.32167987821284,2.42051616919978,77.186245065838));
#28410=CARTESIAN_POINT('Ctrl Pts',(-6.38174935182926,2.25735948336676,77.1944369086158));
#28411=CARTESIAN_POINT('Ctrl Pts',(-6.43540009344285,2.09234668191381,77.2026287513934));
#28412=CARTESIAN_POINT('Ctrl Pts',(-6.48677735071721,1.93432640299816,77.2104734596171));
#28413=CARTESIAN_POINT('Ctrl Pts',(-6.53226863502543,1.77460434834334,77.2183181678407));
#28414=CARTESIAN_POINT('Ctrl Pts',(-6.57178766936335,1.6136591426952,77.2261628760644));
#28415=CARTESIAN_POINT('Ctrl Pts',(-6.62724690738091,1.38779586902559,77.237171787285));
#28416=CARTESIAN_POINT('Ctrl Pts',(-6.67107997133574,1.15898350456572,77.2481806985057));
#28417=CARTESIAN_POINT('Ctrl Pts',(-6.70303305923548,0.928243937117981,
77.2591896097263));
#28418=CARTESIAN_POINT('Ctrl Pts',(-6.73420260589151,0.703162475960873,
77.2699285646906));
#28419=CARTESIAN_POINT('Ctrl Pts',(-6.75406775022714,0.476246829645958,
77.2806675196549));
#28420=CARTESIAN_POINT('Ctrl Pts',(-6.76243688553776,0.248468044461097,
77.2914064746192));
#28421=CARTESIAN_POINT('Ctrl Pts',(-6.76540188998257,0.16777092517219,77.2952110551427));
#28422=CARTESIAN_POINT('Ctrl Pts',(-6.76692439875737,0.0869657043062816,
77.2990156356663));
#28423=CARTESIAN_POINT('Ctrl Pts',(-6.76699725388582,0.00609638431824338,
77.3028202161898));
#28424=CARTESIAN_POINT('Ctrl Pts',(-6.767,3.76644436666148E-12,77.3028202161898));
#28425=CARTESIAN_POINT('Ctrl Pts',(-6.76700000000011,-0.186007249411994,
77.3115697279958));
#28426=CARTESIAN_POINT('Ctrl Pts',(-6.75932637295458,-0.372014355523931,
77.3203192398017));
#28427=CARTESIAN_POINT('Ctrl Pts',(-6.74400518266957,-0.557389537151535,
77.3290687516077));
#28428=CARTESIAN_POINT('Ctrl Pts',(-6.72868405709682,-0.742763935808111,
77.3378182264582));
#28429=CARTESIAN_POINT('Ctrl Pts',(-6.70571545653034,-0.927506129691979,
77.3465677013088));
#28430=CARTESIAN_POINT('Ctrl Pts',(-6.67517739415697,-1.11098863924693,
77.3553171761593));
#28431=CARTESIAN_POINT('Ctrl Pts',(-6.64463945823122,-1.29447038906391,
77.3640666147813));
#28432=CARTESIAN_POINT('Ctrl Pts',(-6.60653217027181,-1.47669218228113,
77.3728160534033));
#28433=CARTESIAN_POINT('Ctrl Pts',(-6.56098496116736,-1.65703510504025,
77.3815654920253));
#28434=CARTESIAN_POINT('Ctrl Pts',(-6.5154379368754,-1.83737729603941,77.3903148951455));
#28435=CARTESIAN_POINT('Ctrl Pts',(-6.46245112202659,-2.01584035396991,
77.3990642982658));
#28436=CARTESIAN_POINT('Ctrl Pts',(-6.40220448416258,-2.19181813638097,
77.407813701386));
#28437=CARTESIAN_POINT('Ctrl Pts',(-6.34195808575201,-2.36779521935908,
77.4165630697313));
#28438=CARTESIAN_POINT('Ctrl Pts',(-6.27445201489246,-2.54128677544801,
77.4253124380766));
#28439=CARTESIAN_POINT('Ctrl Pts',(-6.19991555136191,-2.71170355237824,
77.4340618064218));
#28440=CARTESIAN_POINT('Ctrl Pts',(-6.12537937789048,-2.88211966613052,
77.4428111407189));
#28441=CARTESIAN_POINT('Ctrl Pts',(-6.04381298133629,-3.04946076210421,
77.451560475016));
#28442=CARTESIAN_POINT('Ctrl Pts',(-5.95549339426321,-3.21315848206827,
77.460309809313));
#28443=CARTESIAN_POINT('Ctrl Pts',(-5.86717414355184,-3.37685557859595,
77.4690591102886));
#28444=CARTESIAN_POINT('Ctrl Pts',(-5.7721018898627,-3.53690907467258,77.4778084112641));
#28445=CARTESIAN_POINT('Ctrl Pts',(-5.67059953467111,-3.69277536784839,
77.4865577122397));
#28446=CARTESIAN_POINT('Ctrl Pts',(-5.56909755761813,-3.84864108035724,
77.4953069806204));
#28447=CARTESIAN_POINT('Ctrl Pts',(-5.46116568338122,-4.00031938104207,
77.5040562490012));
#28448=CARTESIAN_POINT('Ctrl Pts',(-5.34717048686172,-4.14729511663144,
77.5128055173819));
#28449=CARTESIAN_POINT('Ctrl Pts',(-5.2331757055557,-4.29427031687977,77.5215547538946));
#28450=CARTESIAN_POINT('Ctrl Pts',(-5.11311782178851,-4.43654275987077,
77.5303039904072));
#28451=CARTESIAN_POINT('Ctrl Pts',(-4.98740459172053,-4.57362924147608,
77.5390532269198));
#28452=CARTESIAN_POINT('Ctrl Pts',(-4.86169180910883,-4.71071523514381,
77.5478024322909));
#28453=CARTESIAN_POINT('Ctrl Pts',(-4.730323914155,-4.84261509316456,77.556551637662));
#28454=CARTESIAN_POINT('Ctrl Pts',(-4.59374707237378,-4.96888084331445,
77.5653008430331));
#28455=CARTESIAN_POINT('Ctrl Pts',(-4.45717070537482,-5.09514615452655,
77.5740500179894));
#28456=CARTESIAN_POINT('Ctrl Pts',(-4.31538563819583,-5.21577720253572,
77.5827991929456));
#28457=CARTESIAN_POINT('Ctrl Pts',(-4.16887341290716,-5.33036429028597,
77.5915483679019));
#28458=CARTESIAN_POINT('Ctrl Pts',(-4.02236168477423,-5.44495098921114,
77.6002975131698));
#28459=CARTESIAN_POINT('Ctrl Pts',(-3.87112305634541,-5.55349359238687,
77.6090466584377));
#28460=CARTESIAN_POINT('Ctrl Pts',(-3.71567117316853,-5.65562346102394,
77.6177958037056));
#28461=CARTESIAN_POINT('Ctrl Pts',(-3.56021980457443,-5.75775299158681,
77.6265449200117));
#28462=CARTESIAN_POINT('Ctrl Pts',(-3.40055544862552,-5.85346967275257,
77.6352940363179));
#28463=CARTESIAN_POINT('Ctrl Pts',(-3.23722036323591,-5.94244842803459,
77.644043152624));
#28464=CARTESIAN_POINT('Ctrl Pts',(-3.07388580496244,-6.03142689616374,
77.652792240695));
#28465=CARTESIAN_POINT('Ctrl Pts',(-2.90688079257915,-6.11366734484723,
77.6615413287659));
#28466=CARTESIAN_POINT('Ctrl Pts',(-2.73677251094833,-6.18889046787205,
77.6702904168369));
#28467=CARTESIAN_POINT('Ctrl Pts',(-2.56666476416886,-6.26411335438171,
77.6790394773991));
#28468=CARTESIAN_POINT('Ctrl Pts',(-2.39345402972357,-6.3323188435019,77.6877885379613));
#28469=CARTESIAN_POINT('Ctrl Pts',(-2.21772856474325,-6.39327529620944,
77.6965375985235));
#28470=CARTESIAN_POINT('Ctrl Pts',(-2.04200363768559,-6.4542315623199,77.7052866323035));
#28471=CARTESIAN_POINT('Ctrl Pts',(-1.86376426620386,-6.50793874251972,
77.7140356660835));
#28472=CARTESIAN_POINT('Ctrl Pts',(-1.68361578194983,-6.55421443796047,
77.7227846998635));
#28473=CARTESIAN_POINT('Ctrl Pts',(-1.50346783420193,-6.60048999558605,
77.7315337075877));
#28474=CARTESIAN_POINT('Ctrl Pts',(-1.32141106257603,-6.63933404145424,
77.7402827153119));
#28475=CARTESIAN_POINT('Ctrl Pts',(-1.13806375959431,-6.67061465526964,
77.7490317230362));
#28476=CARTESIAN_POINT('Ctrl Pts',(-0.954716987423268,-6.70189517852421,
77.757780705431));
#28477=CARTESIAN_POINT('Ctrl Pts',(-0.770079973814236,-6.72561226535777,
77.7665296878259));
#28478=CARTESIAN_POINT('Ctrl Pts',(-0.584779770557059,-6.74168536939742,
77.7752786702208));
#28479=CARTESIAN_POINT('Ctrl Pts',(-0.391490647558487,-6.75845143942367,
77.7844048508968));
#28480=CARTESIAN_POINT('Ctrl Pts',(-0.197480213108879,-6.76689975924013,
77.7935310315729));
#28481=CARTESIAN_POINT('Ctrl Pts',(-0.00346532630230147,-6.76699911271707,
77.8026572122489));
#28482=CARTESIAN_POINT('Ctrl Pts',(0.184486595291538,-6.76709536139786,
77.8114981997789));
#28483=CARTESIAN_POINT('Ctrl Pts',(0.372442378180706,-6.75935659726795,
77.8203391873088));
#28484=CARTESIAN_POINT('Ctrl Pts',(0.559750217717562,-6.74380965729054,
77.8291801748387));
#28485=CARTESIAN_POINT('Ctrl Pts',(0.745129914453265,-6.72842275717303,
77.8379301534365));
#28486=CARTESIAN_POINT('Ctrl Pts',(0.929874656309734,-6.70538772273535,
77.8466801320343));
#28487=CARTESIAN_POINT('Ctrl Pts',(1.11335688289337,-6.67478280180816,77.855430110632));
#28488=CARTESIAN_POINT('Ctrl Pts',(1.29683723118408,-6.64417819418111,77.864179999657));
#28489=CARTESIAN_POINT('Ctrl Pts',(1.47905480729778,-6.60600390230177,77.8729298886819));
#28490=CARTESIAN_POINT('Ctrl Pts',(1.65939064804344,-6.56038959797252,77.8816797777069));
#28491=CARTESIAN_POINT('Ctrl Pts',(1.839724702638,-6.51477574543387,77.8904295800678));
#28492=CARTESIAN_POINT('Ctrl Pts',(2.01817678125382,-6.46172209820245,77.8991793824287));
#28493=CARTESIAN_POINT('Ctrl Pts',(2.19414072347213,-6.40140886724174,77.9079291847897));
#28494=CARTESIAN_POINT('Ctrl Pts',(2.37010298131632,-6.34109621361548,77.9166789033952));
#28495=CARTESIAN_POINT('Ctrl Pts',(2.54357687926451,-6.27352420826158,77.9254286220007));
#28496=CARTESIAN_POINT('Ctrl Pts',(2.71397317789512,-6.19892237325697,77.9341783406061));
#28497=CARTESIAN_POINT('Ctrl Pts',(2.88436790206755,-6.12432122757174,77.9429279783644));
#28498=CARTESIAN_POINT('Ctrl Pts',(3.05168482125823,-6.04269049717636,77.9516776161227));
#28499=CARTESIAN_POINT('Ctrl Pts',(3.21535561996969,-5.95430745235157,77.960427253881));
#28500=CARTESIAN_POINT('Ctrl Pts',(3.37902496074868,-5.86592519481754,77.9691768137));
#28501=CARTESIAN_POINT('Ctrl Pts',(3.5390479938447,-5.7707908794048,77.977926373519));
#28502=CARTESIAN_POINT('Ctrl Pts',(3.69488118814588,-5.66922763747283,77.986675933338));
#28503=CARTESIAN_POINT('Ctrl Pts',(3.85071304610448,-5.56766526649318,77.9954254181254));
#28504=CARTESIAN_POINT('Ctrl Pts',(4.00235489705594,-5.45967423580988,78.0041749029129));
#28505=CARTESIAN_POINT('Ctrl Pts',(4.14929168607292,-5.34562133936609,78.0129243877003));
#28506=CARTESIAN_POINT('Ctrl Pts',(4.29622726385405,-5.2315693830882,78.0216738003636));
#28507=CARTESIAN_POINT('Ctrl Pts',(4.43845763091726,-5.11145583677499,78.0304232130269));
#28508=CARTESIAN_POINT('Ctrl Pts',(4.57549970660631,-4.98568866204515,78.0391726256902));
#28509=CARTESIAN_POINT('Ctrl Pts',(4.71254069814977,-4.8599224822647,78.0479219691366));
#28510=CARTESIAN_POINT('Ctrl Pts',(4.84439326931009,-4.72850295734315,78.0566713125829));
#28511=CARTESIAN_POINT('Ctrl Pts',(4.97060959434406,-4.59187644221998,78.0654206560292));
#28512=CARTESIAN_POINT('Ctrl Pts',(5.09682496280238,-4.45525096256981,78.0741699331655));
#28513=CARTESIAN_POINT('Ctrl Pts',(5.21740397615577,-4.31341878218643,78.0829192103018));
#28514=CARTESIAN_POINT('Ctrl Pts',(5.33193710451687,-4.16686161438993,78.0916684874381));
#28515=CARTESIAN_POINT('Ctrl Pts',(5.44646940289143,-4.02030550864839,78.1004177011711));
#28516=CARTESIAN_POINT('Ctrl Pts',(5.55495572749432,-3.86902470980468,78.109166914904));
#28517=CARTESIAN_POINT('Ctrl Pts',(5.65702762491231,-3.71353301466125,78.117916128637));
#28518=CARTESIAN_POINT('Ctrl Pts',(5.75909881654934,-3.55804239467248,78.1266652818731));
#28519=CARTESIAN_POINT('Ctrl Pts',(5.85475551250569,-3.3983411761992,78.1354144351092));
#28520=CARTESIAN_POINT('Ctrl Pts',(5.94367283727888,-3.23497174692349,78.1441635883453));
#28521=CARTESIAN_POINT('Ctrl Pts',(6.03258957676119,-3.07160339301345,78.1529126839909));
#28522=CARTESIAN_POINT('Ctrl Pts',(6.11476689685105,-2.90456712829882,78.1616617796364));
#28523=CARTESIAN_POINT('Ctrl Pts',(6.18992570525095,-2.73443024476281,78.1704108752819));
#28524=CARTESIAN_POINT('Ctrl Pts',(6.26508404388545,-2.56429442463402,78.179159916243));
#28525=CARTESIAN_POINT('Ctrl Pts',(6.33322384283176,-2.39105828656361,78.187908957204));
#28526=CARTESIAN_POINT('Ctrl Pts',(6.39411368719907,-2.21531017132444,78.196657998165));
#28527=CARTESIAN_POINT('Ctrl Pts',(6.45500317120774,-2.03956309619882,78.2054069873474));
#28528=CARTESIAN_POINT('Ctrl Pts',(6.50864269269967,-1.86130434439004,78.2141559765298));
#28529=CARTESIAN_POINT('Ctrl Pts',(6.55485008446237,-1.68113930720319,78.2229049657122));
#28530=CARTESIAN_POINT('Ctrl Pts',(6.6019966474932,-1.49731239212209,78.2318317792416));
#28531=CARTESIAN_POINT('Ctrl Pts',(6.64140563640835,-1.31150116500034,78.240758592771));
#28532=CARTESIAN_POINT('Ctrl Pts',(6.67293772282112,-1.12436255156017,78.2496854063004));
#28533=CARTESIAN_POINT('Ctrl Pts',(6.7038449494982,-0.940932395054963,78.2584353204559));
#28534=CARTESIAN_POINT('Ctrl Pts',(6.72718449348889,-0.756227260510381,
78.2671852346114));
#28535=CARTESIAN_POINT('Ctrl Pts',(6.74287707373901,-0.5708745645454,78.2759351487669));
#28536=CARTESIAN_POINT('Ctrl Pts',(6.75856934538649,-0.385525513636246,
78.2846848908509));
#28537=CARTESIAN_POINT('Ctrl Pts',(6.76661493004092,-0.199529212422058,
78.2934346329349));
#28538=CARTESIAN_POINT('Ctrl Pts',(6.76698649908906,-0.01351743860431,78.3021843750189));
#28539=CARTESIAN_POINT('Ctrl Pts',(6.76735806132399,0.172490924442,78.3109339566648));
#28540=CARTESIAN_POINT('Ctrl Pts',(6.76005588896309,0.358514472897737,78.3196835383107));
#28541=CARTESIAN_POINT('Ctrl Pts',(6.74510478454613,0.543921359658655,78.3284331199566));
#28542=CARTESIAN_POINT('Ctrl Pts',(6.73015393440725,0.729325093146978,78.3371825527956));
#28543=CARTESIAN_POINT('Ctrl Pts',(6.70755443556943,0.914111900252981,78.3459319856347));
#28544=CARTESIAN_POINT('Ctrl Pts',(6.67738304682373,1.09765415591211,78.3546814184737));
#28545=CARTESIAN_POINT('Ctrl Pts',(6.64721213111924,1.28119353390945,78.363430714135));
#28546=CARTESIAN_POINT('Ctrl Pts',(6.60946960955567,1.46348811672325,78.3721800097964));
#28547=CARTESIAN_POINT('Ctrl Pts',(6.56428366991265,1.64391876347894,78.3809293054577));
#28548=CARTESIAN_POINT('Ctrl Pts',(6.51909837867806,1.82434682109403,78.3896784755685));
#28549=CARTESIAN_POINT('Ctrl Pts',(6.46646995272014,2.00291071820147,78.3984276456793));
#28550=CARTESIAN_POINT('Ctrl Pts',(6.40657713281646,2.1790040021242,78.4071768157902));
#28551=CARTESIAN_POINT('Ctrl Pts',(6.34668509279168,2.35509499309367,78.4159258719759));
#28552=CARTESIAN_POINT('Ctrl Pts',(6.27952894037646,2.52871516397824,78.4246749281617));
#28553=CARTESIAN_POINT('Ctrl Pts',(6.20533675061579,2.69927486771115,78.4334239843475));
#28554=CARTESIAN_POINT('Ctrl Pts',(6.12832117908056,2.87632521635626,78.4425059856298));
#28555=CARTESIAN_POINT('Ctrl Pts',(6.04372366626226,3.05007728919708,78.451587986912));
#28556=CARTESIAN_POINT('Ctrl Pts',(5.9518537800802,3.21989527477914,78.4606699881943));
#28557=CARTESIAN_POINT('Ctrl Pts',(5.86334450817532,3.38350129286473,78.4694197685014));
#28558=CARTESIAN_POINT('Ctrl Pts',(5.76808562057425,3.54345567124686,78.4781695488086));
#28559=CARTESIAN_POINT('Ctrl Pts',(5.66640068804662,3.69921508465036,78.4869193291157));
#28560=CARTESIAN_POINT('Ctrl Pts',(5.56471941108111,3.85496889852012,78.4956687948692));
#28561=CARTESIAN_POINT('Ctrl Pts',(5.45661270815312,4.00652780919367,78.5044182606226));
#28562=CARTESIAN_POINT('Ctrl Pts',(5.34244776449322,4.15337704568962,78.5131677263761));
#28563=CARTESIAN_POINT('Ctrl Pts',(5.22828631819809,4.30022178355989,78.5219169240957));
#28564=CARTESIAN_POINT('Ctrl Pts',(5.10806717844289,4.44235690972426,78.5306661218153));
#28565=CARTESIAN_POINT('Ctrl Pts',(4.98219864544945,4.57929969070399,78.5394153195349));
#28566=CARTESIAN_POINT('Ctrl Pts',(4.8563332994424,4.71623900429781,78.5481642957252));
#28567=CARTESIAN_POINT('Ctrl Pts',(4.7248190403385,4.84798602483421,78.5569132719154));
#28568=CARTESIAN_POINT('Ctrl Pts',(4.58810250737386,4.97409332258953,78.5656622481057));
#28569=CARTESIAN_POINT('Ctrl Pts',(4.45137708685827,5.10020881821975,78.5744117930419));
#28570=CARTESIAN_POINT('Ctrl Pts',(4.30944892636232,5.22068366307784,78.583161337978));
#28571=CARTESIAN_POINT('Ctrl Pts',(4.16280009466838,5.33510865604713,78.5919108829142));
#28572=CARTESIAN_POINT('Ctrl Pts',(4.01615988348954,5.4495269227277,78.6006599135225));
#28573=CARTESIAN_POINT('Ctrl Pts',(3.86479978232383,5.55789587288521,78.6094089441308));
#28574=CARTESIAN_POINT('Ctrl Pts',(3.70923383581206,5.65984746713787,78.6181579747391));
#28575=CARTESIAN_POINT('Ctrl Pts',(3.55366577799671,5.76180044505303,78.6269071240871));
#28576=CARTESIAN_POINT('Ctrl Pts',(3.39389200026962,5.85733573570988,78.6356562734351));
#28577=CARTESIAN_POINT('Ctrl Pts',(3.23045513626155,5.94612887621866,78.6444054227832));
#28578=CARTESIAN_POINT('Ctrl Pts',(3.18695122151658,5.96976399206646,78.6467342868961));
#28579=CARTESIAN_POINT('Ctrl Pts',(3.14318791262709,5.9929216543531,78.6490631510091));
#28580=CARTESIAN_POINT('Ctrl Pts',(3.09917575053268,6.01559628526634,78.6513920151221));
#28581=CARTESIAN_POINT('Origin',(0.,0.,-3.69717978381041));
#28582=CARTESIAN_POINT('',(3.09917575053255,6.01559628526641,81.0455808655427));
#28583=CARTESIAN_POINT('',(3.09917575053259,6.01559628526639,80.651216691749));
#28584=CARTESIAN_POINT('',(3.09917575053259,6.01559628526639,-3.69717978381041));
#28585=CARTESIAN_POINT('',(-6.7669999925025,-0.000318545333296113,79.6971797838099));
#28586=CARTESIAN_POINT('Ctrl Pts',(-6.7669999925025,-0.000318545333296113,
79.6971797838099));
#28587=CARTESIAN_POINT('Ctrl Pts',(-6.76699126828019,-0.185651074678613,
79.7058520742601));
#28588=CARTESIAN_POINT('Ctrl Pts',(-6.7593645097331,-0.370812397315357,
79.7145243647103));
#28589=CARTESIAN_POINT('Ctrl Pts',(-6.74418751263934,-0.555179065130915,
79.7231966551606));
#28590=CARTESIAN_POINT('Ctrl Pts',(-6.728987169257,-0.739829338287013,79.7318822859174));
#28591=CARTESIAN_POINT('Ctrl Pts',(-6.70621341493911,-0.923682226209467,
79.7405679166743));
#28592=CARTESIAN_POINT('Ctrl Pts',(-6.67598545392258,-1.10612260577845,
79.7492535474312));
#28593=CARTESIAN_POINT('Ctrl Pts',(-6.64567895497579,-1.28903699978067,
79.757961745091));
#28594=CARTESIAN_POINT('Ctrl Pts',(-6.60787955356384,-1.47053125611473,
79.7666699427509));
#28595=CARTESIAN_POINT('Ctrl Pts',(-6.56275749079366,-1.65000094455482,
79.7753781404107));
#28596=CARTESIAN_POINT('Ctrl Pts',(-6.51757624396202,-1.82970603324961,
79.7840977601216));
#28597=CARTESIAN_POINT('Ctrl Pts',(-6.46505323702654,-2.00738097265852,
79.7928173798325));
#28598=CARTESIAN_POINT('Ctrl Pts',(-6.40540793799161,-2.18243857826839,
79.8015369995434));
#28599=CARTESIAN_POINT('Ctrl Pts',(-6.34562037681719,-2.3579137200447,79.8102774167317));
#28600=CARTESIAN_POINT('Ctrl Pts',(-6.2786766452146,-2.53075876779444,79.8190178339199));
#28601=CARTESIAN_POINT('Ctrl Pts',(-6.20484459315538,-2.70040600184314,
79.8277582511081));
#28602=CARTESIAN_POINT('Ctrl Pts',(-6.13638854804961,-2.85770054238756,
79.8358622435693));
#28603=CARTESIAN_POINT('Ctrl Pts',(-6.06201137532344,-3.01224609912074,
79.8439662360305));
#28604=CARTESIAN_POINT('Ctrl Pts',(-5.9819606965745,-3.16361110515152,79.8520702284916));
#28605=CARTESIAN_POINT('Ctrl Pts',(-5.9014453592497,-3.31585471770051,79.8602212610236));
#28606=CARTESIAN_POINT('Ctrl Pts',(-5.81498775513594,-3.46526172829884,
79.8683722935556));
#28607=CARTESIAN_POINT('Ctrl Pts',(-5.7228122671405,-3.61133060727847,79.8765233260876));
#28608=CARTESIAN_POINT('Ctrl Pts',(-5.63074384366015,-3.75722982299903,
79.8846648909578));
#28609=CARTESIAN_POINT('Ctrl Pts',(-5.53297094985115,-3.89979831914096,
79.892806455828));
#28610=CARTESIAN_POINT('Ctrl Pts',(-5.42976486685794,-4.03855698122921,
79.9009480206981));
#28611=CARTESIAN_POINT('Ctrl Pts',(-5.32665694302677,-4.17718367014688,
79.9090818421373));
#28612=CARTESIAN_POINT('Ctrl Pts',(-5.21812633448767,-4.31200744751291,
79.9172156635765));
#28613=CARTESIAN_POINT('Ctrl Pts',(-5.10448882341879,-4.44257615034258,
79.9253494850156));
#28614=CARTESIAN_POINT('Ctrl Pts',(-4.99093549321105,-4.57304812995348,
79.9334772810492));
#28615=CARTESIAN_POINT('Ctrl Pts',(-4.87228303231264,-4.69927103664301,
79.9416050770828));
#28616=CARTESIAN_POINT('Ctrl Pts',(-4.74888888196918,-4.82082393234907,
79.9497328731164));
#28617=CARTESIAN_POINT('Ctrl Pts',(-4.62556019810287,-4.94231233845131,
79.9578563569668));
#28618=CARTESIAN_POINT('Ctrl Pts',(-4.49749509479425,-5.05913541182123,
79.9659798408173));
#28619=CARTESIAN_POINT('Ctrl Pts',(-4.36508941462806,-5.17090740608475,
79.9741033246677));
#28620=CARTESIAN_POINT('Ctrl Pts',(-4.23184517865899,-5.28338727824497,
79.9822782564207));
#28621=CARTESIAN_POINT('Ctrl Pts',(-4.09420544734246,-5.39075159227332,
79.9904531881736));
#28622=CARTESIAN_POINT('Ctrl Pts',(-3.95260959059071,-5.49264657741333,
79.9986281199266));
#28623=CARTESIAN_POINT('Ctrl Pts',(-3.81193675626825,-5.59387733862141,
80.0067497616642));
#28624=CARTESIAN_POINT('Ctrl Pts',(-3.66735953678444,-5.68970967033223,
80.014871403402));
#28625=CARTESIAN_POINT('Ctrl Pts',(-3.51933978753285,-5.77983879185987,
80.0229930451396));
#28626=CARTESIAN_POINT('Ctrl Pts',(-3.37130049339222,-5.86997981425676,
80.0311157592787));
#28627=CARTESIAN_POINT('Ctrl Pts',(-3.21981807670386,-5.95441593614001,
80.0392384734178));
#28628=CARTESIAN_POINT('Ctrl Pts',(-3.06538091489876,-6.03288727282173,
80.0473611875569));
#28629=CARTESIAN_POINT('Ctrl Pts',(-2.91089395226344,-6.11138391389049,
80.0554865210002));
#28630=CARTESIAN_POINT('Ctrl Pts',(-2.75345067328943,-6.18391177388882,
80.0636118544435));
#28631=CARTESIAN_POINT('Ctrl Pts',(-2.59356139439414,-6.25025825814489,
80.0717371878868));
#28632=CARTESIAN_POINT('Ctrl Pts',(-2.43193308752715,-6.31732635671269,
80.0799508961245));
#28633=CARTESIAN_POINT('Ctrl Pts',(-2.26780561666465,-6.37807768298584,
80.0881646043621));
#28634=CARTESIAN_POINT('Ctrl Pts',(-2.10172306626406,-6.43234398588365,
80.0963783125997));
#28635=CARTESIAN_POINT('Ctrl Pts',(-1.93714316759201,-6.48611930791891,
80.1045177063302));
#28636=CARTESIAN_POINT('Ctrl Pts',(-1.77064379038275,-6.53352643507237,
80.1126571000606));
#28637=CARTESIAN_POINT('Ctrl Pts',(-1.60276547411663,-6.57445296849705,
80.1207964937911));
#28638=CARTESIAN_POINT('Ctrl Pts',(-1.43258800730884,-6.61594000469293,
80.1290473592823));
#28639=CARTESIAN_POINT('Ctrl Pts',(-1.26099394264601,-6.65076757655893,
80.1372982247735));
#28640=CARTESIAN_POINT('Ctrl Pts',(-1.08855215076031,-6.67887290005396,
80.1455490902648));
#28641=CARTESIAN_POINT('Ctrl Pts',(-0.916110358874604,-6.70697822354898,
80.153799955756));
#28642=CARTESIAN_POINT('Ctrl Pts',(-0.742821228910491,-6.72836131821488,
80.1620508212472));
#28643=CARTESIAN_POINT('Ctrl Pts',(-0.569253656216054,-6.74301410905277,
80.1703016867384));
#28644=CARTESIAN_POINT('Ctrl Pts',(-0.396087756160033,-6.75763299018583,
80.1785334579549));
#28645=CARTESIAN_POINT('Ctrl Pts',(-0.22210414601066,-6.76559849540422,
80.1867652291714));
#28646=CARTESIAN_POINT('Ctrl Pts',(-0.047855088193626,-6.76683078630861,
80.1949970003879));
#28647=CARTESIAN_POINT('Ctrl Pts',(0.126185899374362,-6.76806160573832,
80.2032189420725));
#28648=CARTESIAN_POINT('Ctrl Pts',(0.300491348675806,-6.7625752180599,80.211440883757));
#28649=CARTESIAN_POINT('Ctrl Pts',(0.474502880395008,-6.75034339989432,
80.2196628254415));
#28650=CARTESIAN_POINT('Ctrl Pts',(0.648341490250427,-6.73812373695072,
80.2278765966705));
#28651=CARTESIAN_POINT('Ctrl Pts',(0.821886409229279,-6.71917201784723,
80.2360903678995));
#28652=CARTESIAN_POINT('Ctrl Pts',(0.994578157988799,-6.69351202939471,
80.2443041391285));
#28653=CARTESIAN_POINT('Ctrl Pts',(1.16713288415996,-6.66787240090761,80.2525113931255));
#28654=CARTESIAN_POINT('Ctrl Pts',(1.33883543562522,-6.63553515713876,80.2607186471225));
#28655=CARTESIAN_POINT('Ctrl Pts',(1.50913026499436,-6.59657599389851,80.2689259011195));
#28656=CARTESIAN_POINT('Ctrl Pts',(1.67932407241606,-6.55763994193272,80.2771282864262));
#28657=CARTESIAN_POINT('Ctrl Pts',(1.84811147297831,-6.51208987571257,80.285330671733));
#28658=CARTESIAN_POINT('Ctrl Pts',(2.01494584904912,-6.4600528036077,80.2935330570397));
#28659=CARTESIAN_POINT('Ctrl Pts',(2.18173043001608,-6.4080312630226,80.3017329941781));
#28660=CARTESIAN_POINT('Ctrl Pts',(2.34656280485905,-6.34952667619528,80.3099329313165));
#28661=CARTESIAN_POINT('Ctrl Pts',(2.50891005003434,-6.28471633097602,80.3181328684549));
#28662=CARTESIAN_POINT('Ctrl Pts',(2.67123459541787,-6.21991504769889,80.3263316590579));
#28663=CARTESIAN_POINT('Ctrl Pts',(2.83107437011529,-6.14880989410969,80.3345304496609));
#28664=CARTESIAN_POINT('Ctrl Pts',(2.98791500502242,-6.07162687611499,80.342729240264));
#28665=CARTESIAN_POINT('Ctrl Pts',(3.14476216180441,-5.99444064863326,80.3509283717958));
#28666=CARTESIAN_POINT('Ctrl Pts',(3.29860960869036,-5.91117621143672,80.3591275033275));
#28667=CARTESIAN_POINT('Ctrl Pts',(3.44896617558892,-5.82210626145242,80.3673266348593));
#28668=CARTESIAN_POINT('Ctrl Pts',(3.59935627011023,-5.7330164499899,80.3755275946943));
#28669=CARTESIAN_POINT('Ctrl Pts',(3.74625362593384,-5.63811873000138,80.3837285545293));
#28670=CARTESIAN_POINT('Ctrl Pts',(3.8891946911901,-5.53773000912998,80.3919295143642));
#28671=CARTESIAN_POINT('Ctrl Pts',(4.03226972748446,-5.43724719926376,80.4001381605215));
#28672=CARTESIAN_POINT('Ctrl Pts',(4.17138077111078,-5.33126331254785,80.4083468066788));
#28673=CARTESIAN_POINT('Ctrl Pts',(4.30609535650516,-5.22013714194222,80.4165554528361));
#28674=CARTESIAN_POINT('Ctrl Pts',(4.44087425885037,-5.10895791623176,80.4247680180575));
#28675=CARTESIAN_POINT('Ctrl Pts',(4.5712522505928,-4.99263175010406,80.4329805832789));
#28676=CARTESIAN_POINT('Ctrl Pts',(4.69683267576492,-4.87155537953403,80.4411931485002));
#28677=CARTESIAN_POINT('Ctrl Pts',(4.82258541614656,-4.75031287399405,80.4494169825949));
#28678=CARTESIAN_POINT('Ctrl Pts',(4.94352718524975,-4.6243073961534,80.4576408166895));
#28679=CARTESIAN_POINT('Ctrl Pts',(5.05929985198646,-4.49397085078328,80.4658646507842));
#28680=CARTESIAN_POINT('Ctrl Pts',(5.16567326996443,-4.37421595345513,80.4734208155179));
#28681=CARTESIAN_POINT('Ctrl Pts',(5.26768317643285,-4.25080524346746,80.4809769802517));
#28682=CARTESIAN_POINT('Ctrl Pts',(5.36508391286331,-4.12409548967229,80.4885331449855));
#28683=CARTESIAN_POINT('Ctrl Pts',(5.47652852392743,-3.97911589560306,80.4971788069255));
#28684=CARTESIAN_POINT('Ctrl Pts',(5.58219275646772,-3.82948667938921,80.5058244688656));
#28685=CARTESIAN_POINT('Ctrl Pts',(5.68169250808639,-3.67568486728053,80.5144701308057));
#28686=CARTESIAN_POINT('Ctrl Pts',(5.78106452227576,-3.52208050539437,80.5231046934755));
#28687=CARTESIAN_POINT('Ctrl Pts',(5.87428767147399,-3.36431448412436,80.5317392561454));
#28688=CARTESIAN_POINT('Ctrl Pts',(5.96101936055093,-3.20289512521672,80.5403738188152));
#28689=CARTESIAN_POINT('Ctrl Pts',(6.05081494041197,-3.03577345275566,80.5493134067564));
#28690=CARTESIAN_POINT('Ctrl Pts',(6.13365183298998,-2.86473585119626,80.5582529946975));
#28691=CARTESIAN_POINT('Ctrl Pts',(6.20919844019825,-2.69037984869045,80.5671925826386));
#28692=CARTESIAN_POINT('Ctrl Pts',(6.28196482320838,-2.52244039876286,80.575803180839));
#28693=CARTESIAN_POINT('Ctrl Pts',(6.34796775239083,-2.35142273477379,80.5844137790394));
#28694=CARTESIAN_POINT('Ctrl Pts',(6.40695701572333,-2.17788677361189,80.5930243772399));
#28695=CARTESIAN_POINT('Ctrl Pts',(6.46589044563991,-2.00451506446723,80.6016268254977));
#28696=CARTESIAN_POINT('Ctrl Pts',(6.51782334714075,-1.82863009817014,80.6102292737555));
#28697=CARTESIAN_POINT('Ctrl Pts',(6.56255362652765,-1.65081158796176,80.6188317220133));
#28698=CARTESIAN_POINT('Ctrl Pts',(6.60723356820451,-1.47319318776229,80.6274244894117));
#28699=CARTESIAN_POINT('Ctrl Pts',(6.64472698384982,-1.29364587973253,80.6360172568102));
#28700=CARTESIAN_POINT('Ctrl Pts',(6.67488157492676,-1.11276455762361,80.6446100242086));
#28701=CARTESIAN_POINT('Ctrl Pts',(6.67843631935433,-1.09144154017072,80.6456229741753));
#28702=CARTESIAN_POINT('Ctrl Pts',(6.6818891359297,-1.07010000105353,80.646635924142));
#28703=CARTESIAN_POINT('Ctrl Pts',(6.68523982118511,-1.0487409276084,80.6476488741087));
#28704=CARTESIAN_POINT('Ctrl Pts',(6.71367175746758,-0.867500444258104,
80.656244169314));
#28705=CARTESIAN_POINT('Ctrl Pts',(6.73471237551699,-0.685209894751886,
80.6648394645192));
#28706=CARTESIAN_POINT('Ctrl Pts',(6.74831832548549,-0.502482614541714,
80.6734347597246));
#28707=CARTESIAN_POINT('Ctrl Pts',(6.76193701871019,-0.319584192988989,
80.682038105235));
#28708=CARTESIAN_POINT('Ctrl Pts',(6.76810712222662,-0.13624852877261,80.6906414507454));
#28709=CARTESIAN_POINT('Ctrl Pts',(6.76683740358844,0.0469100564533351,
80.6992447962559));
#28710=CARTESIAN_POINT('Ctrl Pts',(6.76551505072461,0.237661198026486,80.7082047801706));
#28711=CARTESIAN_POINT('Ctrl Pts',(6.75612293780566,0.428219885752169,80.7171647640853));
#28712=CARTESIAN_POINT('Ctrl Pts',(6.73873063703672,0.617898374704722,80.726124748));
#28713=CARTESIAN_POINT('Ctrl Pts',(6.72198491915971,0.800525302880217,80.7347516320915));
#28714=CARTESIAN_POINT('Ctrl Pts',(6.69782321040895,0.982336010378989,80.7433785161829));
#28715=CARTESIAN_POINT('Ctrl Pts',(6.66635996946198,1.1627268628336,80.7520054002744));
#28716=CARTESIAN_POINT('Ctrl Pts',(6.63486665545255,1.34329013571311,80.7606405300779));
#28717=CARTESIAN_POINT('Ctrl Pts',(6.59605794024985,1.52243054607268,80.7692756598815));
#28718=CARTESIAN_POINT('Ctrl Pts',(6.55009878553166,1.69955726581269,80.777910789685));
#28719=CARTESIAN_POINT('Ctrl Pts',(6.50407136954502,1.87694706468546,80.7865587448966));
#28720=CARTESIAN_POINT('Ctrl Pts',(6.45087237543878,2.05231690311487,80.7952067001081));
#28721=CARTESIAN_POINT('Ctrl Pts',(6.39071620493619,2.22509222010369,80.8038546553197));
#28722=CARTESIAN_POINT('Ctrl Pts',(6.38396889421377,2.24447125868193,80.8048246379572));
#28723=CARTESIAN_POINT('Ctrl Pts',(6.37713410730476,2.26381767877992,80.8057946205947));
#28724=CARTESIAN_POINT('Ctrl Pts',(6.37021218380461,2.28313068686557,80.8067646032322));
#28725=CARTESIAN_POINT('Ctrl Pts',(6.3115102399365,2.44691624683938,80.8149906210925));
#28726=CARTESIAN_POINT('Ctrl Pts',(6.24641018884347,2.60865229056004,80.8232166389527));
#28727=CARTESIAN_POINT('Ctrl Pts',(6.17507486429063,2.7678040791223,80.831442656813));
#28728=CARTESIAN_POINT('Ctrl Pts',(6.10381704099951,2.92678295945859,80.8396597376317));
#28729=CARTESIAN_POINT('Ctrl Pts',(6.02633758133013,3.08318285169219,80.8478768184504));
#28730=CARTESIAN_POINT('Ctrl Pts',(5.94284863313208,3.23648561308099,80.856093899269));
#28731=CARTESIAN_POINT('Ctrl Pts',(5.85944769074041,3.38962677783419,80.8643023184524));
#28732=CARTESIAN_POINT('Ctrl Pts',(5.77005005594519,3.53967700554285,80.8725107376357));
#28733=CARTESIAN_POINT('Ctrl Pts',(5.6749152518394,3.68613969952858,80.880719156819));
#28734=CARTESIAN_POINT('Ctrl Pts',(5.57983763741589,3.83251434839754,80.8889226415633));
#28735=CARTESIAN_POINT('Ctrl Pts',(5.47902991569958,3.97530545848919,80.8971261263077));
#28736=CARTESIAN_POINT('Ctrl Pts',(5.37279691093228,4.11404209432482,80.9053296110521));
#28737=CARTESIAN_POINT('Ctrl Pts',(5.26660849486966,4.25272049885185,80.9135296525844));
#28738=CARTESIAN_POINT('Ctrl Pts',(5.15499954851385,4.38734753453143,80.9217296941167));
#28739=CARTESIAN_POINT('Ctrl Pts',(5.0383175143484,4.51748222183665,80.9299297356491));
#28740=CARTESIAN_POINT('Ctrl Pts',(4.92166328754959,4.64758589577303,80.9381278229683));
#28741=CARTESIAN_POINT('Ctrl Pts',(4.79993862089678,4.77319908793876,80.9463259102875));
#28742=CARTESIAN_POINT('Ctrl Pts',(4.67353047667194,4.89391478099267,80.9545239976067));
#28743=CARTESIAN_POINT('Ctrl Pts',(4.54709857854369,5.01465315825678,80.9627236254642));
#28744=CARTESIAN_POINT('Ctrl Pts',(4.41598169958258,5.13049194577093,80.9709232533216));
#28745=CARTESIAN_POINT('Ctrl Pts',(4.28060315415918,5.24106149902885,80.979122881179));
#28746=CARTESIAN_POINT('Ctrl Pts',(4.14521328827664,5.35164029819871,80.9873231946957));
#28747=CARTESIAN_POINT('Ctrl Pts',(4.00556132715072,5.45694876292595,80.9955235082123));
#28748=CARTESIAN_POINT('Ctrl Pts',(3.86210276485753,5.55665827936898,81.003723821729));
#28749=CARTESIAN_POINT('Ctrl Pts',(3.71855185373349,5.65643198199317,81.0119294140478));
#28750=CARTESIAN_POINT('Ctrl Pts',(3.57118974338493,5.75059933539894,81.0201350063666));
#28751=CARTESIAN_POINT('Ctrl Pts',(3.42050050722433,5.83887534376939,81.0283405986854));
#28752=CARTESIAN_POINT('Ctrl Pts',(3.31496586926094,5.90069911314797,81.0340873543045));
#28753=CARTESIAN_POINT('Ctrl Pts',(3.2077999114992,5.95963419113215,81.0398341099236));
#28754=CARTESIAN_POINT('Ctrl Pts',(3.09917575053255,6.01559628526641,81.0455808655427));
#28755=CARTESIAN_POINT('Ctrl Pts',(3.09917575053266,6.01559628526635,79.0457515827422));
#28756=CARTESIAN_POINT('Ctrl Pts',(2.93382384459277,6.10078395293753,79.0545010306546));
#28757=CARTESIAN_POINT('Ctrl Pts',(2.76495772123002,6.17915010267041,79.063250478567));
#28758=CARTESIAN_POINT('Ctrl Pts',(2.59315093316735,6.25042856433167,79.0719999264794));
#28759=CARTESIAN_POINT('Ctrl Pts',(2.42134553245646,6.3217064504144,79.0807493037394));
#28760=CARTESIAN_POINT('Ctrl Pts',(2.24659977927624,6.38589665313445,79.0894986809994));
#28761=CARTESIAN_POINT('Ctrl Pts',(2.06950718689957,6.44278115439063,79.0982480582594));
#28762=CARTESIAN_POINT('Ctrl Pts',(1.89241596572904,6.49966521519711,79.1069973677741));
#28763=CARTESIAN_POINT('Ctrl Pts',(1.71297821457246,6.54924360009533,79.1157466772888));
#28764=CARTESIAN_POINT('Ctrl Pts',(1.53180337335897,6.59134792173544,79.1244959868034));
#28765=CARTESIAN_POINT('Ctrl Pts',(1.35062987477822,6.63345193135297,79.1332452314795));
#28766=CARTESIAN_POINT('Ctrl Pts',(1.16771959102978,6.66808192368234,79.1419944761557));
#28767=CARTESIAN_POINT('Ctrl Pts',(0.983693746906968,6.69512028363167,79.1507437208318));
#28768=CARTESIAN_POINT('Ctrl Pts',(0.799669205419977,6.72215845218866,79.159492903576));
#28769=CARTESIAN_POINT('Ctrl Pts',(0.614529402873566,6.74160505424578,79.1682420863201));
#28770=CARTESIAN_POINT('Ctrl Pts',(0.42890312736332,6.75339404354122,79.1769912690643));
#28771=CARTESIAN_POINT('Ctrl Pts',(0.243278104164084,6.76518295330329,79.1857403927829));
#28772=CARTESIAN_POINT('Ctrl Pts',(0.0571669005394561,6.76931433552275,
79.1944895165015));
#28773=CARTESIAN_POINT('Ctrl Pts',(-0.128798404777041,6.76577415902474,
79.2032386402201));
#28774=CARTESIAN_POINT('Ctrl Pts',(-0.314762517258607,6.76223400523444,
79.2119877078194));
#28775=CARTESIAN_POINT('Ctrl Pts',(-0.500580446819,6.75102239665093,79.2207367754186));
#28776=CARTESIAN_POINT('Ctrl Pts',(-0.685621118842083,6.73217741012503,
79.2294858430178));
#28777=CARTESIAN_POINT('Ctrl Pts',(-0.870660665414059,6.71333253821778,
79.2382348574036));
#28778=CARTESIAN_POINT('Ctrl Pts',(-1.05492267885453,6.68685441030618,79.2469838717893));
#28779=CARTESIAN_POINT('Ctrl Pts',(-1.23778137635229,6.65283295028182,79.2557328861751));
#28780=CARTESIAN_POINT('Ctrl Pts',(-1.42999922978822,6.61707018861871,79.2649296965425));
#28781=CARTESIAN_POINT('Ctrl Pts',(-1.6206660123367,6.57297172934419,79.2741265069099));
#28782=CARTESIAN_POINT('Ctrl Pts',(-1.80906628500359,6.52070304311301,79.2833233172773));
#28783=CARTESIAN_POINT('Ctrl Pts',(-1.98831342545491,6.47097374915042,79.292073315015));
#28784=CARTESIAN_POINT('Ctrl Pts',(-2.16550875896655,6.41384933989544,79.3008233127528));
#28785=CARTESIAN_POINT('Ctrl Pts',(-2.34005036713955,6.34952386240497,79.3095733104906));
#28786=CARTESIAN_POINT('Ctrl Pts',(-2.51458843547033,6.28519968948618,79.3183231307714));
#28787=CARTESIAN_POINT('Ctrl Pts',(-2.68647261718,6.21367483971123,79.3270729510523));
#28788=CARTESIAN_POINT('Ctrl Pts',(-2.85511905908677,6.13519226743869,79.3358227713332));
#28789=CARTESIAN_POINT('Ctrl Pts',(-3.02376230488837,6.05671118252961,79.3445724257917));
#28790=CARTESIAN_POINT('Ctrl Pts',(-3.18916767379864,5.97127275992654,79.3533220802502));
#28791=CARTESIAN_POINT('Ctrl Pts',(-3.35077334102754,5.87916720438015,79.3620717347088));
#28792=CARTESIAN_POINT('Ctrl Pts',(-3.51237616037333,5.78706327195664,79.3708212349772));
#28793=CARTESIAN_POINT('Ctrl Pts',(-3.67017916302264,5.68829258362321,79.3795707352457));
#28794=CARTESIAN_POINT('Ctrl Pts',(-3.82364636566425,5.58319061741067,79.3883202355141));
#28795=CARTESIAN_POINT('Ctrl Pts',(-3.97711106778758,5.47809036367731,79.3970695932225));
#28796=CARTESIAN_POINT('Ctrl Pts',(-4.12623987481884,5.36665920043257,79.4058189509309));
#28797=CARTESIAN_POINT('Ctrl Pts',(-4.27052628213884,5.24927559512371,79.4145683086394));
#28798=CARTESIAN_POINT('Ctrl Pts',(-4.41481053024921,5.13189374643084,79.4233175354159));
#28799=CARTESIAN_POINT('Ctrl Pts',(-4.55425230136462,5.00855981477414,79.4320667621924));
#28800=CARTESIAN_POINT('Ctrl Pts',(-4.6883780063047,4.87969268192151,79.4408159889689));
#28801=CARTESIAN_POINT('Ctrl Pts',(-4.82250188228825,4.7508273063188,79.4495650964398));
#28802=CARTESIAN_POINT('Ctrl Pts',(-4.95130963052905,4.61642907903591,79.4583142039106));
#28803=CARTESIAN_POINT('Ctrl Pts',(-5.07436379033314,4.47695444731749,79.4670633113815));
#28804=CARTESIAN_POINT('Ctrl Pts',(-5.19741643562745,4.33748153220658,79.4758123111712));
#28805=CARTESIAN_POINT('Ctrl Pts',(-5.31471544462706,4.19293255254673,79.484561310961));
#28806=CARTESIAN_POINT('Ctrl Pts',(-5.42586245275555,4.043798417797,79.4933103107507));
#28807=CARTESIAN_POINT('Ctrl Pts',(-5.53702160019085,3.89464799484439,79.5020602660928));
#28808=CARTESIAN_POINT('Ctrl Pts',(-5.64202723081188,3.74091164443946,79.510810221435));
#28809=CARTESIAN_POINT('Ctrl Pts',(-5.74052265232908,3.58311159163328,79.5195601767772));
#28810=CARTESIAN_POINT('Ctrl Pts',(-5.83901427066855,3.42531763191891,79.5283097942596));
#28811=CARTESIAN_POINT('Ctrl Pts',(-5.93099603115673,3.26346052695733,79.537059411742));
#28812=CARTESIAN_POINT('Ctrl Pts',(-6.01615550622685,3.0980900446721,79.5458090292245));
#28813=CARTESIAN_POINT('Ctrl Pts',(-6.10131214578748,2.93272506863936,79.5545583553756));
#28814=CARTESIAN_POINT('Ctrl Pts',(-6.17964682328712,2.76384720416976,79.5633076815267));
#28815=CARTESIAN_POINT('Ctrl Pts',(-6.25089348288541,2.59203002791648,79.5720570076778));
#28816=CARTESIAN_POINT('Ctrl Pts',(-6.32213814889314,2.42021765937072,79.5808060890094));
#28817=CARTESIAN_POINT('Ctrl Pts',(-6.38629508412575,2.24546640831948,79.5895551703409));
#28818=CARTESIAN_POINT('Ctrl Pts',(-6.44314639819806,2.06836976660059,79.5983042516725));
#28819=CARTESIAN_POINT('Ctrl Pts',(-6.50000285283698,1.89125711158283,79.6070541241069));
#28820=CARTESIAN_POINT('Ctrl Pts',(-6.5495522767325,1.71179891440252,79.6158039965413));
#28821=CARTESIAN_POINT('Ctrl Pts',(-6.59162635926388,1.53060476278419,79.6245538689757));
#28822=CARTESIAN_POINT('Ctrl Pts',(-6.633697520552,1.34942319164681,79.6333031338982));
#28823=CARTESIAN_POINT('Ctrl Pts',(-6.66829431424257,1.16650618642687,79.6420523988208));
#28824=CARTESIAN_POINT('Ctrl Pts',(-6.6952992374542,0.982474997618355,79.6508016637433));
#28825=CARTESIAN_POINT('Ctrl Pts',(-6.72230554731446,0.798434359177552,
79.659551377923));
#28826=CARTESIAN_POINT('Ctrl Pts',(-6.74171916496705,0.613279706240161,
79.6683010921026));
#28827=CARTESIAN_POINT('Ctrl Pts',(-6.75347414817276,0.427639953655215,
79.6770508062823));
#28828=CARTESIAN_POINT('Ctrl Pts',(-6.76248837758739,0.285283364199431,
79.6837604654582));
#28829=CARTESIAN_POINT('Ctrl Pts',(-6.76699999999991,0.142641701107,79.6904701246341));
#28830=CARTESIAN_POINT('Ctrl Pts',(-6.767,4.47431244915746E-12,79.6971797838099));
#28831=CARTESIAN_POINT('',(-6.767,4.30001371423856E-12,79.3028202161898));
#28832=CARTESIAN_POINT('Ctrl Pts',(3.09917575053268,6.01559628526634,78.6513920151221));
#28833=CARTESIAN_POINT('Ctrl Pts',(2.93382384459277,6.10078395293753,78.6601414630345));
#28834=CARTESIAN_POINT('Ctrl Pts',(2.76495772122999,6.17915010267042,78.6688909109469));
#28835=CARTESIAN_POINT('Ctrl Pts',(2.5931509331673,6.2504285643317,78.6776403588593));
#28836=CARTESIAN_POINT('Ctrl Pts',(2.42134553245638,6.32170645041443,78.6863897361194));
#28837=CARTESIAN_POINT('Ctrl Pts',(2.24659977927613,6.38589665313449,78.6951391133794));
#28838=CARTESIAN_POINT('Ctrl Pts',(2.06950718689943,6.44278115439067,78.7038884906394));
#28839=CARTESIAN_POINT('Ctrl Pts',(1.89241596572875,6.4996652151972,78.712637800154));
#28840=CARTESIAN_POINT('Ctrl Pts',(1.71297821457201,6.54924360009545,78.7213871096687));
#28841=CARTESIAN_POINT('Ctrl Pts',(1.53180337335837,6.59134792173558,78.7301364191833));
#28842=CARTESIAN_POINT('Ctrl Pts',(1.35062987477771,6.63345193135307,78.7388856638595));
#28843=CARTESIAN_POINT('Ctrl Pts',(1.16771959102937,6.6680819236824,78.7476349085356));
#28844=CARTESIAN_POINT('Ctrl Pts',(0.983693746906654,6.69512028363171,78.7563841532117));
#28845=CARTESIAN_POINT('Ctrl Pts',(0.799669205419761,6.72215845218868,78.7651333359559));
#28846=CARTESIAN_POINT('Ctrl Pts',(0.614529402873448,6.74160505424579,78.7738825187));
#28847=CARTESIAN_POINT('Ctrl Pts',(0.428903127363302,6.75339404354122,78.7826317014442));
#28848=CARTESIAN_POINT('Ctrl Pts',(0.24327810416391,6.7651829533033,78.7913808251628));
#28849=CARTESIAN_POINT('Ctrl Pts',(0.0571669005391258,6.76931433552276,
78.8001299488814));
#28850=CARTESIAN_POINT('Ctrl Pts',(-0.128798404777528,6.76577415902473,
78.8088790726));
#28851=CARTESIAN_POINT('Ctrl Pts',(-0.314762517258994,6.76223400523441,
78.8176281401992));
#28852=CARTESIAN_POINT('Ctrl Pts',(-0.500580446819287,6.7510223966509,78.8263772077985));
#28853=CARTESIAN_POINT('Ctrl Pts',(-0.68562111884227,6.73217741012501,78.8351262753977));
#28854=CARTESIAN_POINT('Ctrl Pts',(-0.870660665414274,6.71333253821775,
78.8438752897835));
#28855=CARTESIAN_POINT('Ctrl Pts',(-1.05492267885478,6.68685441030614,78.8526243041692));
#28856=CARTESIAN_POINT('Ctrl Pts',(-1.23778137635256,6.65283295028177,78.861373318555));
#28857=CARTESIAN_POINT('Ctrl Pts',(-1.42999922978852,6.61707018861864,78.8705701289224));
#28858=CARTESIAN_POINT('Ctrl Pts',(-1.62066601233703,6.57297172934411,78.8797669392898));
#28859=CARTESIAN_POINT('Ctrl Pts',(-1.80906628500394,6.52070304311292,78.8889637496572));
#28860=CARTESIAN_POINT('Ctrl Pts',(-1.98831342545541,6.47097374915027,78.897713747395));
#28861=CARTESIAN_POINT('Ctrl Pts',(-2.16550875896719,6.41384933989523,78.9064637451327));
#28862=CARTESIAN_POINT('Ctrl Pts',(-2.34005036714033,6.34952386240468,78.9152137428705));
#28863=CARTESIAN_POINT('Ctrl Pts',(-2.51458843547113,6.28519968948586,78.9239635631514));
#28864=CARTESIAN_POINT('Ctrl Pts',(-2.68647261718082,6.21367483971087,78.9327133834322));
#28865=CARTESIAN_POINT('Ctrl Pts',(-2.85511905908761,6.1351922674383,78.9414632037131));
#28866=CARTESIAN_POINT('Ctrl Pts',(-3.02376230488922,6.05671118252918,78.9502128581716));
#28867=CARTESIAN_POINT('Ctrl Pts',(-3.18916767379951,5.97127275992608,78.9589625126302));
#28868=CARTESIAN_POINT('Ctrl Pts',(-3.35077334102842,5.87916720437966,78.9677121670887));
#28869=CARTESIAN_POINT('Ctrl Pts',(-3.51237616037433,5.78706327195604,78.9764616673572));
#28870=CARTESIAN_POINT('Ctrl Pts',(-3.67017916302375,5.6882925836225,78.9852111676256));
#28871=CARTESIAN_POINT('Ctrl Pts',(-3.82364636566547,5.58319061740984,78.993960667894));
#28872=CARTESIAN_POINT('Ctrl Pts',(-3.9771110677888,5.47809036367642,79.0027100256025));
#28873=CARTESIAN_POINT('Ctrl Pts',(-4.12623987482006,5.36665920043164,79.0114593833109));
#28874=CARTESIAN_POINT('Ctrl Pts',(-4.27052628214005,5.24927559512273,79.0202087410194));
#28875=CARTESIAN_POINT('Ctrl Pts',(-4.41481053025052,5.13189374642973,79.0289579677959));
#28876=CARTESIAN_POINT('Ctrl Pts',(-4.55425230136601,5.00855981477288,79.0377071945724));
#28877=CARTESIAN_POINT('Ctrl Pts',(-4.68837800630617,4.87969268192011,79.0464564213489));
#28878=CARTESIAN_POINT('Ctrl Pts',(-4.8225018822897,4.75082730631733,79.0552055288198));
#28879=CARTESIAN_POINT('Ctrl Pts',(-4.95130963053048,4.61642907903439,79.0639546362906));
#28880=CARTESIAN_POINT('Ctrl Pts',(-5.07436379033454,4.47695444731591,79.0727037437615));
#28881=CARTESIAN_POINT('Ctrl Pts',(-5.19741643562883,4.33748153220493,79.0814527435512));
#28882=CARTESIAN_POINT('Ctrl Pts',(-5.31471544462841,4.19293255254502,79.0902017433409));
#28883=CARTESIAN_POINT('Ctrl Pts',(-5.42586245275687,4.04379841779524,79.0989507431307));
#28884=CARTESIAN_POINT('Ctrl Pts',(-5.53702160019206,3.89464799484267,79.1077006984728));
#28885=CARTESIAN_POINT('Ctrl Pts',(-5.64202723081298,3.74091164443779,79.116450653815));
#28886=CARTESIAN_POINT('Ctrl Pts',(-5.74052265233008,3.58311159163166,79.1252006091571));
#28887=CARTESIAN_POINT('Ctrl Pts',(-5.83901427066959,3.42531763191713,79.1339502266396));
#28888=CARTESIAN_POINT('Ctrl Pts',(-5.9309960311578,3.26346052695539,79.142699844122));
#28889=CARTESIAN_POINT('Ctrl Pts',(-6.01615550622794,3.09809004466999,79.1514494616045));
#28890=CARTESIAN_POINT('Ctrl Pts',(-6.10131214578846,2.93272506863731,79.1601987877556));
#28891=CARTESIAN_POINT('Ctrl Pts',(-6.179646823288,2.76384720416778,79.1689481139067));
#28892=CARTESIAN_POINT('Ctrl Pts',(-6.25089348288621,2.59203002791456,79.1776974400578));
#28893=CARTESIAN_POINT('Ctrl Pts',(-6.32213814889385,2.42021765936887,79.1864465213894));
#28894=CARTESIAN_POINT('Ctrl Pts',(-6.38629508412637,2.24546640831771,79.1951956027209));
#28895=CARTESIAN_POINT('Ctrl Pts',(-6.44314639819861,2.06836976659889,79.2039446840525));
#28896=CARTESIAN_POINT('Ctrl Pts',(-6.50000285283749,1.8912571115811,79.2126945564869));
#28897=CARTESIAN_POINT('Ctrl Pts',(-6.54955227673297,1.71179891440076,79.2214444289213));
#28898=CARTESIAN_POINT('Ctrl Pts',(-6.5916263592643,1.53060476278238,79.2301943013557));
#28899=CARTESIAN_POINT('Ctrl Pts',(-6.63369752055234,1.34942319164508,79.2389435662782));
#28900=CARTESIAN_POINT('Ctrl Pts',(-6.66829431424286,1.16650618642523,79.2476928312007));
#28901=CARTESIAN_POINT('Ctrl Pts',(-6.69529923745443,0.982474997616808,
79.2564420961232));
#28902=CARTESIAN_POINT('Ctrl Pts',(-6.72230554731464,0.798434359175971,
79.2651918103029));
#28903=CARTESIAN_POINT('Ctrl Pts',(-6.74171916496719,0.613279706238548,
79.2739415244826));
#28904=CARTESIAN_POINT('Ctrl Pts',(-6.75347414817286,0.427639953653572,
79.2826912386623));
#28905=CARTESIAN_POINT('Ctrl Pts',(-6.76248837758742,0.285283364198275,
79.2894008978381));
#28906=CARTESIAN_POINT('Ctrl Pts',(-6.76699999999991,0.142641701106334,
79.296110557014));
#28907=CARTESIAN_POINT('Ctrl Pts',(-6.767,4.30001365154025E-12,79.3028202161898));
#28908=CARTESIAN_POINT('Ctrl Pts',(-6.76699998814839,-0.000400499275143691,
79.3028202161898));
#28909=CARTESIAN_POINT('Ctrl Pts',(-6.76698906540322,-0.184955680925308,
79.3114483693845));
#28910=CARTESIAN_POINT('Ctrl Pts',(-6.759423854444,-0.369326019158339,79.3200765225791));
#28911=CARTESIAN_POINT('Ctrl Pts',(-6.74437525354799,-0.552893696228719,
79.3287046757738));
#28912=CARTESIAN_POINT('Ctrl Pts',(-6.72930224251752,-0.736759135975562,
79.3373468245805));
#28913=CARTESIAN_POINT('Ctrl Pts',(-6.70672162339215,-0.919819020312296,
79.3459889733872));
#28914=CARTESIAN_POINT('Ctrl Pts',(-6.67675560673779,-1.1014642835315,79.3546311221939));
#28915=CARTESIAN_POINT('Ctrl Pts',(-6.64670872982854,-1.28359969805948,
79.3632965909621));
#28916=CARTESIAN_POINT('Ctrl Pts',(-6.60923663947623,-1.46431256296585,
79.3719620597303));
#28917=CARTESIAN_POINT('Ctrl Pts',(-6.56451244123904,-1.64300499354625,
79.3806275284985));
#28918=CARTESIAN_POINT('Ctrl Pts',(-6.51972457954531,-1.82195178704953,
79.3893053322826));
#28919=CARTESIAN_POINT('Ctrl Pts',(-6.46766407913286,-1.9988721201907,79.3979831360666));
#28920=CARTESIAN_POINT('Ctrl Pts',(-6.40855305186145,-2.17318585985583,
79.4066609398507));
#28921=CARTESIAN_POINT('Ctrl Pts',(-6.34929707638161,-2.34792704031221,
79.4153600227796));
#28922=CARTESIAN_POINT('Ctrl Pts',(-6.28295609962157,-2.52004856631107,
79.4240591057085));
#28923=CARTESIAN_POINT('Ctrl Pts',(-6.20980027758688,-2.68899042625331,
79.4327581886375));
#28924=CARTESIAN_POINT('Ctrl Pts',(-6.15926792524473,-2.80568694273686,
79.4387670763977));
#28925=CARTESIAN_POINT('Ctrl Pts',(-6.10548494151629,-2.92086683827788,
79.444775964158));
#28926=CARTESIAN_POINT('Ctrl Pts',(-6.04855265123554,-3.03435327956907,
79.4507848519183));
#28927=CARTESIAN_POINT('Ctrl Pts',(-5.97061225014743,-3.18971640844865,
79.4590110293621));
#28928=CARTESIAN_POINT('Ctrl Pts',(-5.88657306186628,-3.34229182855461,
79.4672372068058));
#28929=CARTESIAN_POINT('Ctrl Pts',(-5.79665788956477,-3.49156788726019,
79.4754633842496));
#28930=CARTESIAN_POINT('Ctrl Pts',(-5.70684373200964,-3.64067624253122,
79.4836803200358));
#28931=CARTESIAN_POINT('Ctrl Pts',(-5.61116691886959,-3.78649231292714,
79.4918972558221));
#28932=CARTESIAN_POINT('Ctrl Pts',(-5.5098973481489,-3.92852646839267,79.5001141916083));
#28933=CARTESIAN_POINT('Ctrl Pts',(-5.40872122212924,-4.07042956435928,
79.5083235453628));
#28934=CARTESIAN_POINT('Ctrl Pts',(-5.30196282298704,-4.20855740507196,
79.5165328991172));
#28935=CARTESIAN_POINT('Ctrl Pts',(-5.18993683028937,-4.34244685604856,
79.5247422528716));
#28936=CARTESIAN_POINT('Ctrl Pts',(-5.07799172976975,-4.47623962759346,
79.532945678783));
#28937=CARTESIAN_POINT('Ctrl Pts',(-4.96078684111141,-4.60579983139573,
79.5411491046943));
#28938=CARTESIAN_POINT('Ctrl Pts',(-4.83867888205708,-4.73069505213925,
79.5493525306056));
#28939=CARTESIAN_POINT('Ctrl Pts',(-4.71663460008055,-4.85552514229876,
79.5575516785797));
#28940=CARTESIAN_POINT('Ctrl Pts',(-4.58969259155407,-4.97569483994611,
79.5657508265538));
#28941=CARTESIAN_POINT('Ctrl Pts',(-4.45824846587645,-5.0908063817543,79.5739499745278));
#28942=CARTESIAN_POINT('Ctrl Pts',(-4.32682909980619,-5.20589624045902,
79.582147578061));
#28943=CARTESIAN_POINT('Ctrl Pts',(-4.19090957123172,-5.31592960045705,
79.5903451815942));
#28944=CARTESIAN_POINT('Ctrl Pts',(-4.05092103613112,-5.42054681365546,
79.5985427851273));
#28945=CARTESIAN_POINT('Ctrl Pts',(-3.91094260070558,-5.52515647909393,
79.6067397972325));
#28946=CARTESIAN_POINT('Ctrl Pts',(-3.76689603018786,-5.62435056051894,
79.6149368093378));
#28947=CARTESIAN_POINT('Ctrl Pts',(-3.61924408083728,-5.71781088208803,
79.623133821443));
#28948=CARTESIAN_POINT('Ctrl Pts',(-3.47157594793389,-5.81128144747751,
79.6313317319906));
#28949=CARTESIAN_POINT('Ctrl Pts',(-3.32030195203603,-5.89901680906969,
79.6395296425383));
#28950=CARTESIAN_POINT('Ctrl Pts',(-3.16591227150854,-5.98074313853317,
79.647727553086));
#28951=CARTESIAN_POINT('Ctrl Pts',(-3.01147760811152,-6.06249327972296,
79.6559278521711));
#28952=CARTESIAN_POINT('Ctrl Pts',(-2.85392576881812,-6.13823073366157,
79.6641281512563));
#28953=CARTESIAN_POINT('Ctrl Pts',(-2.69376990979961,-6.20772846321891,
79.6723284503414));
#28954=CARTESIAN_POINT('Ctrl Pts',(-2.53344714983676,-6.27729861745533,
79.6805372950875));
#28955=CARTESIAN_POINT('Ctrl Pts',(-2.37051527807995,-6.34061591329752,
79.6887461398335));
#28956=CARTESIAN_POINT('Ctrl Pts',(-2.20550667459669,-6.39750180213413,
79.6969549845795));
#28957=CARTESIAN_POINT('Ctrl Pts',(-2.04040950560559,-6.45441822348558,
79.7051682352807));
#28958=CARTESIAN_POINT('Ctrl Pts',(-1.87323372583407,-6.50489625267868,
79.7133814859819));
#28959=CARTESIAN_POINT('Ctrl Pts',(-1.70452502200897,-6.54880778839518,
79.7215947366831));
#28960=CARTESIAN_POINT('Ctrl Pts',(-1.53556953674757,-6.59278355643406,
79.7298200014521));
#28961=CARTESIAN_POINT('Ctrl Pts',(-1.36507699665651,-6.63017355870686,
79.738045266221));
#28962=CARTESIAN_POINT('Ctrl Pts',(-1.19360264973322,-6.66090096867908,
79.74627053099));
#28963=CARTESIAN_POINT('Ctrl Pts',(-1.03851658083228,-6.68869167501855,
79.7537096844353));
#28964=CARTESIAN_POINT('Ctrl Pts',(-0.882627683050216,-6.71103310593623,
79.7611488378805));
#28965=CARTESIAN_POINT('Ctrl Pts',(-0.726348091822014,-6.7279051308343,
79.7685879913258));
#28966=CARTESIAN_POINT('Ctrl Pts',(-0.55353567822464,-6.74656204772279,
79.7768141330241));
#28967=CARTESIAN_POINT('Ctrl Pts',(-0.379762391741271,-6.75858249991527,
79.7850402747225));
#28968=CARTESIAN_POINT('Ctrl Pts',(-0.205578996589351,-6.7638765716238,
79.7932664164208));
#28969=CARTESIAN_POINT('Ctrl Pts',(-0.0315912802210126,-6.769164695937,
79.8014833168168));
#28970=CARTESIAN_POINT('Ctrl Pts',(0.142805272178604,-6.76774147593213,
79.8097002172129));
#28971=CARTESIAN_POINT('Ctrl Pts',(0.317052893303833,-6.75956851158768,
79.817917117609));
#28972=CARTESIAN_POINT('Ctrl Pts',(0.491139737944541,-6.75140308835322,
79.8261264363557));
#28973=CARTESIAN_POINT('Ctrl Pts',(0.665077568985269,-6.73650034060762,
79.8343357551025));
#28974=CARTESIAN_POINT('Ctrl Pts',(0.838306629016581,-6.71487386298111,
79.8425450738492));
#28975=CARTESIAN_POINT('Ctrl Pts',(1.01141061122818,-6.69326300047524,79.8507484651627));
#28976=CARTESIAN_POINT('Ctrl Pts',(1.18380648732817,-6.66493812222926,79.8589518564762));
#28977=CARTESIAN_POINT('Ctrl Pts',(1.35493754616958,-6.62996479975422,79.8671552477897));
#28978=CARTESIAN_POINT('Ctrl Pts',(1.52597937202656,-6.5950097134425,79.8753543616033));
#28979=CARTESIAN_POINT('Ctrl Pts',(1.69575734395096,-6.55341316082856,79.8835534754169));
#28980=CARTESIAN_POINT('Ctrl Pts',(1.86372280741979,-6.50529217615191,79.8917525892304));
#28981=CARTESIAN_POINT('Ctrl Pts',(2.0316566474713,-6.45718025137335,79.8999501593696));
#28982=CARTESIAN_POINT('Ctrl Pts',(2.19777831266497,-6.40254643402087,79.9081477295087));
#28983=CARTESIAN_POINT('Ctrl Pts',(2.36155192827467,-6.34155828563155,79.9163452996478));
#28984=CARTESIAN_POINT('Ctrl Pts',(2.52531373754777,-6.28057453383937,79.9245422788293));
#28985=CARTESIAN_POINT('Ctrl Pts',(2.68672749790332,-6.21323748764651,79.9327392580107));
#28986=CARTESIAN_POINT('Ctrl Pts',(2.84527507413101,-6.13976373751701,79.9409362371921));
#28987=CARTESIAN_POINT('Ctrl Pts',(3.00384003779941,-6.06628192974005,79.9491341153119));
#28988=CARTESIAN_POINT('Ctrl Pts',(3.15953786560464,-5.98666222807343,79.9573319934317));
#28989=CARTESIAN_POINT('Ctrl Pts',(3.31187284218944,-5.90116829764819,79.9655298715514));
#28990=CARTESIAN_POINT('Ctrl Pts',(3.4642522128568,-5.81564945223172,79.9737301387304));
#28991=CARTESIAN_POINT('Ctrl Pts',(3.61326646751699,-5.72425314367834,79.9819304059094));
#28992=CARTESIAN_POINT('Ctrl Pts',(3.75844677241995,-5.62728770002797,79.9901306730883));
#28993=CARTESIAN_POINT('Ctrl Pts',(3.90377838994009,-5.53022119518294,79.9983394869079));
#28994=CARTESIAN_POINT('Ctrl Pts',(4.04526777584407,-5.42757415846521,80.0065483007275));
#28995=CARTESIAN_POINT('Ctrl Pts',(4.18247643829757,-5.31969734506444,80.0147571145471));
#28996=CARTESIAN_POINT('Ctrl Pts',(4.31975875358718,-5.21176262399869,80.0229703348116));
#28997=CARTESIAN_POINT('Ctrl Pts',(4.45275549164056,-5.09859276199623,80.0311835550761));
#28998=CARTESIAN_POINT('Ctrl Pts',(4.5810633547436,-4.98057702880151,80.0393967753406));
#28999=CARTESIAN_POINT('Ctrl Pts',(4.70955892024492,-4.86238864963156,80.0476220107779));
#29000=CARTESIAN_POINT('Ctrl Pts',(4.83335164838529,-4.73934048509996,80.0558472462152));
#29001=CARTESIAN_POINT('Ctrl Pts',(4.95207616011753,-4.61185761970116,80.0640724816525));
#29002=CARTESIAN_POINT('Ctrl Pts',(5.0594599440381,-4.49655209204032,80.0715120313462));
#29003=CARTESIAN_POINT('Ctrl Pts',(5.16269790830587,-4.3776192024549,80.0789515810399));
#29004=CARTESIAN_POINT('Ctrl Pts',(5.26154981968509,-4.25539451695984,80.0863911307336));
#29005=CARTESIAN_POINT('Ctrl Pts',(5.36987625030378,-4.12145513502538,80.0945437284172));
#29006=CARTESIAN_POINT('Ctrl Pts',(5.47325436973728,-3.98316719419299,80.1026963261008));
#29007=CARTESIAN_POINT('Ctrl Pts',(5.57131138186526,-3.84093458500644,80.1108489237844));
#29008=CARTESIAN_POINT('Ctrl Pts',(5.66925479779108,-3.69886674816893,80.1189920769202));
#29009=CARTESIAN_POINT('Ctrl Pts',(5.76188917176911,-3.5528636374609,80.1271352300561));
#29010=CARTESIAN_POINT('Ctrl Pts',(5.84888078223282,-3.40336342391282,80.1352783831919));
#29011=CARTESIAN_POINT('Ctrl Pts',(5.93578990390099,-3.25400497222527,80.1434138146763));
#29012=CARTESIAN_POINT('Ctrl Pts',(6.01706673200033,-3.10115633339307,80.1515492461607));
#29013=CARTESIAN_POINT('Ctrl Pts',(6.09241984372683,-2.94528597045577,80.1596846776451));
#29014=CARTESIAN_POINT('Ctrl Pts',(6.16771733585885,-2.78953065845901,80.1678141042096));
#29015=CARTESIAN_POINT('Ctrl Pts',(6.23709965942037,-2.63075839119167,80.1759435307741));
#29016=CARTESIAN_POINT('Ctrl Pts',(6.30032049812378,-2.46946363020826,80.1840729573386));
#29017=CARTESIAN_POINT('Ctrl Pts',(6.36350795138381,-2.30825404520829,80.1921980909434));
#29018=CARTESIAN_POINT('Ctrl Pts',(6.42054026663406,-2.14452495895371,80.2003232245483));
#29019=CARTESIAN_POINT('Ctrl Pts',(6.47121859660633,-1.97879227685385,80.2084483581531));
#29020=CARTESIAN_POINT('Ctrl Pts',(6.52208994429173,-1.812428371442,80.2166044378193));
#29021=CARTESIAN_POINT('Ctrl Pts',(6.56655865586342,-1.64404591651449,80.2247605174854));
#29022=CARTESIAN_POINT('Ctrl Pts',(6.60447349218334,-1.47418414421252,80.2329165971516));
#29023=CARTESIAN_POINT('Ctrl Pts',(6.64223605159712,-1.30500458572629,80.241039919652));
#29024=CARTESIAN_POINT('Ctrl Pts',(6.6734972234809,-1.13435793474114,80.2491632421524));
#29025=CARTESIAN_POINT('Ctrl Pts',(6.69815844613823,-0.962788881545214,
80.2572865646528));
#29026=CARTESIAN_POINT('Ctrl Pts',(6.72282295310628,-0.791196979276123,
80.265410968994));
#29027=CARTESIAN_POINT('Ctrl Pts',(6.74088570806473,-0.618682792252615,
80.2735353733351));
#29028=CARTESIAN_POINT('Ctrl Pts',(6.75229985867353,-0.445797732786421,
80.2816597776763));
#29029=CARTESIAN_POINT('Ctrl Pts',(6.76371770093596,-0.27285675748553,80.2897868096757));
#29030=CARTESIAN_POINT('Ctrl Pts',(6.76848263274627,-0.0995450357197435,
80.297913841675));
#29031=CARTESIAN_POINT('Ctrl Pts',(6.76659990900356,0.0735844512996528,
80.3060408736744));
#29032=CARTESIAN_POINT('Ctrl Pts',(6.764705042075,0.247830588355886,80.31422032338));
#29033=CARTESIAN_POINT('Ctrl Pts',(6.75607647505621,0.421891756011707,80.3223997730855));
#29034=CARTESIAN_POINT('Ctrl Pts',(6.74077262160298,0.595208756528067,80.3305792227911));
#29035=CARTESIAN_POINT('Ctrl Pts',(6.72554061072609,0.767712135829498,80.3387202747988));
#29036=CARTESIAN_POINT('Ctrl Pts',(6.70369596187844,0.939477965526954,80.3468613268066));
#29037=CARTESIAN_POINT('Ctrl Pts',(6.67534771068181,1.10996483795442,80.3550023788144));
#29038=CARTESIAN_POINT('Ctrl Pts',(6.64679890047,1.28165787576388,80.3632010273688));
#29039=CARTESIAN_POINT('Ctrl Pts',(6.61165420335213,1.45205342352498,80.3713996759233));
#29040=CARTESIAN_POINT('Ctrl Pts',(6.57007602045649,1.62061410749833,80.3795983244777));
#29041=CARTESIAN_POINT('Ctrl Pts',(6.52849783756082,1.78917479147181,80.3877969730322));
#29042=CARTESIAN_POINT('Ctrl Pts',(6.48048633388413,1.95590027276036,80.3959956215866));
#29043=CARTESIAN_POINT('Ctrl Pts',(6.42625294640687,2.12027405511577,80.404194270141));
#29044=CARTESIAN_POINT('Ctrl Pts',(6.37178269870508,2.28536572755338,80.412428725674));
#29045=CARTESIAN_POINT('Ctrl Pts',(6.31086686766189,2.44859841521295,80.4206631812069));
#29046=CARTESIAN_POINT('Ctrl Pts',(6.24364890358894,2.60943238439179,80.4288976367398));
#29047=CARTESIAN_POINT('Ctrl Pts',(6.17651309793738,2.77006977122549,80.4371220275545));
#29048=CARTESIAN_POINT('Ctrl Pts',(6.10309063599951,2.92831395072693,80.4453464183692));
#29049=CARTESIAN_POINT('Ctrl Pts',(6.02357485675091,3.08363988577108,80.4535708091839));
#29050=CARTESIAN_POINT('Ctrl Pts',(5.94395413507908,3.23917081509647,80.4618060542908));
#29051=CARTESIAN_POINT('Ctrl Pts',(5.85822410089879,3.39177544385225,80.4700412993976));
#29052=CARTESIAN_POINT('Ctrl Pts',(5.76662812388039,3.5409446593913,80.4782765445045));
#29053=CARTESIAN_POINT('Ctrl Pts',(5.67533462049186,3.68962127956145,80.4864845947));
#29054=CARTESIAN_POINT('Ctrl Pts',(5.57821402459683,3.83488482288373,80.4946926448955));
#29055=CARTESIAN_POINT('Ctrl Pts',(5.47555411764076,3.9762540292073,80.5029006950909));
#29056=CARTESIAN_POINT('Ctrl Pts',(5.37295013608146,4.11754622271069,80.5111042738381));
#29057=CARTESIAN_POINT('Ctrl Pts',(5.26481306281275,4.25494801512752,80.5193078525853));
#29058=CARTESIAN_POINT('Ctrl Pts',(5.15147439772318,4.38800644138117,80.5275114313325));
#29059=CARTESIAN_POINT('Ctrl Pts',(5.03817693499965,4.52101649648116,80.5357120278066));
#29060=CARTESIAN_POINT('Ctrl Pts',(4.91968187919999,4.64968605846027,80.5439126242807));
#29061=CARTESIAN_POINT('Ctrl Pts',(4.79636151349017,4.77359458185446,80.5521132207548));
#29062=CARTESIAN_POINT('Ctrl Pts',(4.67216855260053,4.89837986213816,80.5603718433376));
#29063=CARTESIAN_POINT('Ctrl Pts',(4.54308196075631,5.01833617843895,80.5686304659205));
#29064=CARTESIAN_POINT('Ctrl Pts',(4.40952059185325,5.13307092781915,80.5768890885033));
#29065=CARTESIAN_POINT('Ctrl Pts',(4.27689665310766,5.24700038585605,80.5850897461078));
#29066=CARTESIAN_POINT('Ctrl Pts',(4.13986084765876,5.35578113020822,80.5932904037122));
#29067=CARTESIAN_POINT('Ctrl Pts',(3.99885715283741,5.45906864503471,80.6014910613166));
#29068=CARTESIAN_POINT('Ctrl Pts',(3.85635846642072,5.56345126567928,80.6097786663886));
#29069=CARTESIAN_POINT('Ctrl Pts',(3.70980756084845,5.66222327065163,80.6180662714607));
#29070=CARTESIAN_POINT('Ctrl Pts',(3.55969324529376,5.75507367454232,80.6263538765328));
#29071=CARTESIAN_POINT('Ctrl Pts',(3.40957892973918,5.84792407843294,80.6346414816049));
#29072=CARTESIAN_POINT('Ctrl Pts',(3.25590153894876,5.93485270808649,80.642929086677));
#29073=CARTESIAN_POINT('Ctrl Pts',(3.09917575053259,6.01559628526639,80.651216691749));
#29074=CARTESIAN_POINT('Origin',(0.,0.,-3.69717978381041));
#29075=CARTESIAN_POINT('',(3.09917575053248,6.01559628526645,83.0458432482751));
#29076=CARTESIAN_POINT('',(3.09917575053247,6.01559628526645,82.6513920151221));
#29077=CARTESIAN_POINT('',(3.09917575053259,6.01559628526639,-3.69717978381041));
#29078=CARTESIAN_POINT('',(-6.76699738887188,-0.00594466156221417,81.6971797837697));
#29079=CARTESIAN_POINT('Ctrl Pts',(-6.76699738887114,-0.00594466241648763,
81.6971797838099));
#29080=CARTESIAN_POINT('Ctrl Pts',(-6.76678155133687,-0.25163935935655,
81.7087532426108));
#29081=CARTESIAN_POINT('Ctrl Pts',(-6.75318140864,-0.49677316040071,81.7203267014117));
#29082=CARTESIAN_POINT('Ctrl Pts',(-6.72639980188629,-0.740158567594872,
81.7319001602126));
#29083=CARTESIAN_POINT('Ctrl Pts',(-6.70359956999444,-0.947362107477749,
81.7417530994659));
#29084=CARTESIAN_POINT('Ctrl Pts',(-6.67124650991105,-1.1532993901334,81.7516060387192));
#29085=CARTESIAN_POINT('Ctrl Pts',(-6.62949122889958,-1.3572527568377,81.7614589779725));
#29086=CARTESIAN_POINT('Ctrl Pts',(-6.5946355564979,-1.52750503542045,81.7696838255724));
#29087=CARTESIAN_POINT('Ctrl Pts',(-6.5531683641493,-1.69665270370569,81.7779086731722));
#29088=CARTESIAN_POINT('Ctrl Pts',(-6.50517151477902,-1.86414392236962,
81.786133520772));
#29089=CARTESIAN_POINT('Ctrl Pts',(-6.45722872055795,-2.03144650859345,
81.7943491053605));
#29090=CARTESIAN_POINT('Ctrl Pts',(-6.4027710106368,-2.19709601819849,81.8025646899489));
#29091=CARTESIAN_POINT('Ctrl Pts',(-6.34193145251597,-2.3605496079491,81.8107802745373));
#29092=CARTESIAN_POINT('Ctrl Pts',(-6.28114818941145,-2.52385195362786,
81.8189882572219));
#29093=CARTESIAN_POINT('Ctrl Pts',(-6.21399496268251,-2.68496209188757,
81.8271962399065));
#29094=CARTESIAN_POINT('Ctrl Pts',(-6.140654975692,-2.84335109852954,81.8354042225911));
#29095=CARTESIAN_POINT('Ctrl Pts',(-6.06736811968293,-3.0016253606274,81.8436062590219));
#29096=CARTESIAN_POINT('Ctrl Pts',(-5.98790358081624,-3.15718209335518,
81.8518082954528));
#29097=CARTESIAN_POINT('Ctrl Pts',(-5.90249314900087,-3.30951108564358,
81.8600103318836));
#29098=CARTESIAN_POINT('Ctrl Pts',(-5.81712744139058,-3.4617603125808,81.8682080734109));
#29099=CARTESIAN_POINT('Ctrl Pts',(-5.72582221846909,-3.61078485397099,
81.8764058149383));
#29100=CARTESIAN_POINT('Ctrl Pts',(-5.62885584206917,-3.7560978300896,81.8846035564656));
#29101=CARTESIAN_POINT('Ctrl Pts',(-5.53190790230778,-3.90138317722057,
81.8927997393208));
#29102=CARTESIAN_POINT('Ctrl Pts',(-5.4293011468347,-4.04295806315007,81.9009959221759));
#29103=CARTESIAN_POINT('Ctrl Pts',(-5.3213581806263,-4.18036315569372,81.909192105031));
#29104=CARTESIAN_POINT('Ctrl Pts',(-5.21342316058342,-4.31775813323269,
81.9173876845284));
#29105=CARTESIAN_POINT('Ctrl Pts',(-5.10015293308397,-4.45098364597748,
81.9255832640258));
#29106=CARTESIAN_POINT('Ctrl Pts',(-4.98191140900137,-4.57961217930754,
81.9337788435231));
#29107=CARTESIAN_POINT('Ctrl Pts',(-4.86365707654927,-4.70825464616727,
81.9419753107967));
#29108=CARTESIAN_POINT('Ctrl Pts',(-4.74043061752888,-4.83229887729244,
81.9501717780703));
#29109=CARTESIAN_POINT('Ctrl Pts',(-4.61263396174229,-4.95135304083456,
81.9583682453439));
#29110=CARTESIAN_POINT('Ctrl Pts',(-4.48480021133777,-5.07044176137415,
81.9665670917472));
#29111=CARTESIAN_POINT('Ctrl Pts',(-4.35239388431934,-5.18453728471014,
81.9747659381505));
#29112=CARTESIAN_POINT('Ctrl Pts',(-4.21585127287226,-5.29328697928059,
81.9829647845538));
#29113=CARTESIAN_POINT('Ctrl Pts',(-4.07916596111597,-5.40215032785894,
81.991172199549));
#29114=CARTESIAN_POINT('Ctrl Pts',(-3.93833600956304,-5.50565646190259,
81.9993796145442));
#29115=CARTESIAN_POINT('Ctrl Pts',(-3.79382889366723,-5.6034945637143,82.0075870295394));
#29116=CARTESIAN_POINT('Ctrl Pts',(-3.64924432705886,-5.70138510329458,
82.0157988434193));
#29117=CARTESIAN_POINT('Ctrl Pts',(-3.50097897162205,-5.79360136524906,
82.0240106572992));
#29118=CARTESIAN_POINT('Ctrl Pts',(-3.34952627567986,-5.8798777817681,82.0322224711791));
#29119=CARTESIAN_POINT('Ctrl Pts',(-3.19785054251053,-5.96628125348804,
82.0404463782092));
#29120=CARTESIAN_POINT('Ctrl Pts',(-3.04297840675532,-6.04672723307338,
82.0486702852393));
#29121=CARTESIAN_POINT('Ctrl Pts',(-2.88542590258064,-6.12099717045489,
82.0568941922693));
#29122=CARTESIAN_POINT('Ctrl Pts',(-2.7398501112934,-6.18962130918123,82.0644929402527));
#29123=CARTESIAN_POINT('Ctrl Pts',(-2.5919863963532,-6.25297313886653,82.0720916882361));
#29124=CARTESIAN_POINT('Ctrl Pts',(-2.4422535017986,-6.31091806577716,82.0796904362195));
#29125=CARTESIAN_POINT('Ctrl Pts',(-2.28163886038022,-6.37307410493908,
82.0878414185819));
#29126=CARTESIAN_POINT('Ctrl Pts',(-2.11839752773329,-6.42919224847301,
82.0959924009443));
#29127=CARTESIAN_POINT('Ctrl Pts',(-1.95302775807828,-6.47904094570915,
82.1041433833067));
#29128=CARTESIAN_POINT('Ctrl Pts',(-1.78785008071304,-6.52883173907076,
82.1122848975488));
#29129=CARTESIAN_POINT('Ctrl Pts',(-1.6205492343434,-6.57236747812648,82.1204264117909));
#29130=CARTESIAN_POINT('Ctrl Pts',(-1.45164418627425,-6.60946428664655,
82.1285679260331));
#29131=CARTESIAN_POINT('Ctrl Pts',(-1.28289979323479,-6.64652581031905,
82.136701696426));
#29132=CARTESIAN_POINT('Ctrl Pts',(-1.11255459095754,-6.6771605183777,82.144835466819));
#29133=CARTESIAN_POINT('Ctrl Pts',(-0.941143475441524,-6.70123406236746,
82.152969237212));
#29134=CARTESIAN_POINT('Ctrl Pts',(-0.769859347333846,-6.72528977182559,
82.1610969818206));
#29135=CARTESIAN_POINT('Ctrl Pts',(-0.597511238958798,-6.7427939450621,
82.1692247264292));
#29136=CARTESIAN_POINT('Ctrl Pts',(-0.424645027153775,-6.75366312462456,
82.1773524710378));
#29137=CARTESIAN_POINT('Ctrl Pts',(-0.251870536929661,-6.76452653707775,
82.185475903123));
#29138=CARTESIAN_POINT('Ctrl Pts',(-0.078578854923129,-6.76876194406958,
82.1935993352081));
#29139=CARTESIAN_POINT('Ctrl Pts',(0.0946782218924676,-6.7663376382131,
82.2017227672933));
#29140=CARTESIAN_POINT('Ctrl Pts',(0.269034366824355,-6.76389795360663,
82.2098977309255));
#29141=CARTESIAN_POINT('Ctrl Pts',(0.443355093589183,-6.75471372536158,
82.2180726945577));
#29142=CARTESIAN_POINT('Ctrl Pts',(0.617076688796914,-6.73880592984717,
82.2262476581899));
#29143=CARTESIAN_POINT('Ctrl Pts',(0.789664057197207,-6.72300199619345,
82.2343692475546));
#29144=CARTESIAN_POINT('Ctrl Pts',(0.961659728066461,-6.7005620903319,82.2424908369192));
#29145=CARTESIAN_POINT('Ctrl Pts',(1.13251514981973,-6.67155892092911,82.2506124262839));
#29146=CARTESIAN_POINT('Ctrl Pts',(1.30339312799251,-6.64255192251317,82.2587350878649));
#29147=CARTESIAN_POINT('Ctrl Pts',(1.47313019634748,-6.60697999592719,82.2668577494459));
#29148=CARTESIAN_POINT('Ctrl Pts',(1.64118721566619,-6.56496713800868,82.2749804110269));
#29149=CARTESIAN_POINT('Ctrl Pts',(1.80929842498212,-6.5229407330413,82.2831056917607));
#29150=CARTESIAN_POINT('Ctrl Pts',(1.97572815163149,-6.47446934975396,82.2912309724945));
#29151=CARTESIAN_POINT('Ctrl Pts',(2.13995169891577,-6.4197270756869,82.2993562532283));
#29152=CARTESIAN_POINT('Ctrl Pts',(2.30596441665834,-6.36438839957398,82.3075700566648));
#29153=CARTESIAN_POINT('Ctrl Pts',(2.46972223756801,-6.30264151435704,82.3157838601012));
#29154=CARTESIAN_POINT('Ctrl Pts',(2.63070401635478,-6.23471614256294,82.3239976635377));
#29155=CARTESIAN_POINT('Ctrl Pts',(2.79022641175924,-6.16740654952082,82.3321370045827));
#29156=CARTESIAN_POINT('Ctrl Pts',(2.94702258740959,-6.09403024458741,82.3402763456277));
#29157=CARTESIAN_POINT('Ctrl Pts',(3.10061072442964,-6.0148567842927,82.3484156866727));
#29158=CARTESIAN_POINT('Ctrl Pts',(3.25630650258359,-5.93459685179469,82.3566667213049));
#29159=CARTESIAN_POINT('Ctrl Pts',(3.40870521619962,-5.84837969843268,82.3649177559372));
#29160=CARTESIAN_POINT('Ctrl Pts',(3.55733614980349,-5.7565309447011,82.3731687905694));
#29161=CARTESIAN_POINT('Ctrl Pts',(3.70596708340735,-5.66468219096952,82.3814198252017));
#29162=CARTESIAN_POINT('Ctrl Pts',(3.85082995595522,-5.56720210682114,82.3896708598339));
#29163=CARTESIAN_POINT('Ctrl Pts',(3.99148990935795,-5.46445764037875,82.3979218944662));
#29164=CARTESIAN_POINT('Ctrl Pts',(4.13182148536352,-5.3619530358135,82.406153666663));
#29165=CARTESIAN_POINT('Ctrl Pts',(4.26840793867015,-5.25388874326233,82.4143854388598));
#29166=CARTESIAN_POINT('Ctrl Pts',(4.40077994327748,-5.14056659239491,82.4226172110565));
#29167=CARTESIAN_POINT('Ctrl Pts',(4.53299388251097,-5.02737975947629,82.4308391536964));
#29168=CARTESIAN_POINT('Ctrl Pts',(4.66100312434764,-4.90894780072468,82.4390610963364));
#29169=CARTESIAN_POINT('Ctrl Pts',(4.78436756753397,-4.78561552767553,82.4472830389763));
#29170=CARTESIAN_POINT('Ctrl Pts',(4.90760941842082,-4.66240581495707,82.455496811135));
#29171=CARTESIAN_POINT('Ctrl Pts',(5.02621541120786,-4.53430573739926,82.4637105832938));
#29172=CARTESIAN_POINT('Ctrl Pts',(5.13977871639818,-4.40170009728744,82.4719243554526));
#29173=CARTESIAN_POINT('Ctrl Pts',(5.25325191421958,-4.26919967377984,82.480131610353));
#29174=CARTESIAN_POINT('Ctrl Pts',(5.36169016183966,-4.1322010791893,82.4883388652534));
#29175=CARTESIAN_POINT('Ctrl Pts',(5.46472363448574,-3.99112573075479,82.4965461201539));
#29176=CARTESIAN_POINT('Ctrl Pts',(5.5676959854946,-3.85013407120357,82.504748506337));
#29177=CARTESIAN_POINT('Ctrl Pts',(5.66526973794926,-3.70507076416349,82.51295089252));
#29178=CARTESIAN_POINT('Ctrl Pts',(5.75711545423851,-3.55639011450771,82.5211532787031));
#29179=CARTESIAN_POINT('Ctrl Pts',(5.84893375682112,-3.40775384240023,82.5293532166739));
#29180=CARTESIAN_POINT('Ctrl Pts',(5.93502723747499,-3.25550268078992,82.5375531546448));
#29181=CARTESIAN_POINT('Ctrl Pts',(6.01510976560997,-3.10011991827148,82.5457530926156));
#29182=CARTESIAN_POINT('Ctrl Pts',(6.0951810961465,-2.94475888226221,82.553951884024));
#29183=CARTESIAN_POINT('Ctrl Pts',(6.16924298323341,-2.78626743555129,82.5621506754325));
#29184=CARTESIAN_POINT('Ctrl Pts',(6.23705524922844,-2.62515348466941,82.570349466841));
#29185=CARTESIAN_POINT('Ctrl Pts',(6.30487033481908,-2.46403283476073,82.5785485991505));
#29186=CARTESIAN_POINT('Ctrl Pts',(6.36643514249627,-2.30028979378828,82.5867477314601));
#29187=CARTESIAN_POINT('Ctrl Pts',(6.4215576252805,-2.13445231036017,82.5949468637696));
#29188=CARTESIAN_POINT('Ctrl Pts',(6.47669239949277,-1.96857784783767,82.6031478243539));
#29189=CARTESIAN_POINT('Ctrl Pts',(6.5253818746159,-1.80060835273854,82.6113487849383));
#29190=CARTESIAN_POINT('Ctrl Pts',(6.56748384468879,-1.63108704542453,82.6195497455226));
#29191=CARTESIAN_POINT('Ctrl Pts',(6.60962527443976,-1.46140685584918,82.6277583923806));
#29192=CARTESIAN_POINT('Ctrl Pts',(6.64516677720358,-1.29017229653161,82.6359670392386));
#29193=CARTESIAN_POINT('Ctrl Pts',(6.67401708183124,-1.11793782985677,82.6441756860966));
#29194=CARTESIAN_POINT('Ctrl Pts',(6.70288116040432,-0.945621133611937,
82.6523882519931));
#29195=CARTESIAN_POINT('Ctrl Pts',(6.72504762597267,-0.772303933532483,
82.6606008178896));
#29196=CARTESIAN_POINT('Ctrl Pts',(6.74047712353641,-0.598545860467189,
82.6688133837861));
#29197=CARTESIAN_POINT('Ctrl Pts',(6.75592779259387,-0.424549366290701,
82.6770372185062));
#29198=CARTESIAN_POINT('Ctrl Pts',(6.76462300101409,-0.250111148233967,
82.6852610532263));
#29199=CARTESIAN_POINT('Ctrl Pts',(6.76657554106495,-0.0757921306048062,
82.6934848879465));
#29200=CARTESIAN_POINT('Ctrl Pts',(6.76836955755702,0.0843742088110088,
82.7010410428687));
#29201=CARTESIAN_POINT('Ctrl Pts',(6.76447192498461,0.244439721655318,82.7085971977909));
#29202=CARTESIAN_POINT('Ctrl Pts',(6.75493109053418,0.403973962198986,82.716153352713));
#29203=CARTESIAN_POINT('Ctrl Pts',(6.74401451191755,0.586512301794816,82.7247990701999));
#29204=CARTESIAN_POINT('Ctrl Pts',(6.72568476538189,0.768771136426194,82.7334447876867));
#29205=CARTESIAN_POINT('Ctrl Pts',(6.69996462305992,0.950138437147746,82.7420905051736));
#29206=CARTESIAN_POINT('Ctrl Pts',(6.6742775001551,1.1312728992448,82.7507251233225));
#29207=CARTESIAN_POINT('Ctrl Pts',(6.64121894316698,1.3115178092047,82.7593597414714));
#29208=CARTESIAN_POINT('Ctrl Pts',(6.60086358361558,1.4902647249726,82.7679943596203));
#29209=CARTESIAN_POINT('Ctrl Pts',(6.55908302548745,1.67532430534764,82.776933919805));
#29210=CARTESIAN_POINT('Ctrl Pts',(6.50948085777193,1.85877783126783,82.7858734799897));
#29211=CARTESIAN_POINT('Ctrl Pts',(6.45219850249737,2.03995673590661,82.7948130401743));
#29212=CARTESIAN_POINT('Ctrl Pts',(6.39702369992608,2.21446964211677,82.8034236928945));
#29213=CARTESIAN_POINT('Ctrl Pts',(6.33472383417263,2.38687197320314,82.8120343456147));
#29214=CARTESIAN_POINT('Ctrl Pts',(6.26547711874044,2.55657690565725,82.8206449983349));
#29215=CARTESIAN_POINT('Ctrl Pts',(6.19629594990227,2.72612120117369,82.8292475005031));
#29216=CARTESIAN_POINT('Ctrl Pts',(6.12018115631522,2.89297290712752,82.8378500026712));
#29217=CARTESIAN_POINT('Ctrl Pts',(6.03736026261713,3.05656180362375,82.8464525048394));
#29218=CARTESIAN_POINT('Ctrl Pts',(5.95463258205344,3.2199665843357,82.8550453250764));
#29219=CARTESIAN_POINT('Ctrl Pts',(5.86521399602658,3.3801156100352,82.8636381453133));
#29220=CARTESIAN_POINT('Ctrl Pts',(5.76937957983948,3.5364598490201,82.8722309655503));
#29221=CARTESIAN_POINT('Ctrl Pts',(5.75808503033728,3.55488577382723,82.873243670979));
#29222=CARTESIAN_POINT('Ctrl Pts',(5.74670142053278,3.57325887594856,82.8742563764078));
#29223=CARTESIAN_POINT('Ctrl Pts',(5.7352292438198,3.59157827714143,82.8752690818365));
#29224=CARTESIAN_POINT('Ctrl Pts',(5.637860041778,3.74706276109426,82.8838643399086));
#29225=CARTESIAN_POINT('Ctrl Pts',(5.53422167700175,3.89849375004495,82.8924595979808));
#29226=CARTESIAN_POINT('Ctrl Pts',(5.42468356813408,4.04537973317909,82.9010548560529));
#29227=CARTESIAN_POINT('Ctrl Pts',(5.31504288136061,4.19240326895767,82.9096581632285));
#29228=CARTESIAN_POINT('Ctrl Pts',(5.19949160519025,4.33487305858242,82.9182614704041));
#29229=CARTESIAN_POINT('Ctrl Pts',(5.07843915550385,4.47233101903754,82.9268647775797));
#29230=CARTESIAN_POINT('Ctrl Pts',(4.95236783620994,4.61548802632587,82.9358247803614));
#29231=CARTESIAN_POINT('Ctrl Pts',(4.82032972472659,4.75320848801093,82.9447847831431));
#29232=CARTESIAN_POINT('Ctrl Pts',(4.68282829878418,4.88501874347541,82.9537447859248));
#29233=CARTESIAN_POINT('Ctrl Pts',(4.55043958001625,5.01192790621184,82.9623716294669));
#29234=CARTESIAN_POINT('Ctrl Pts',(4.41298675734103,5.13335829386179,82.970998473009));
#29235=CARTESIAN_POINT('Ctrl Pts',(4.27095204001356,5.24892919288344,82.9796253165512));
#29236=CARTESIAN_POINT('Ctrl Pts',(4.12878157333259,5.36461054852528,82.9882604051791));
#29237=CARTESIAN_POINT('Ctrl Pts',(3.98202071308302,5.47442105199867,82.9968954938071));
#29238=CARTESIAN_POINT('Ctrl Pts',(3.83118140321319,5.57802277296117,83.005530582435));
#29239=CARTESIAN_POINT('Ctrl Pts',(3.68011806664266,5.68177836330795,83.0141784959056));
#29240=CARTESIAN_POINT('Ctrl Pts',(3.52496443168327,5.77930657784367,83.0228264093763));
#29241=CARTESIAN_POINT('Ctrl Pts',(3.36625910512639,5.87031418555716,83.0314743228469));
#29242=CARTESIAN_POINT('Ctrl Pts',(3.34845481171687,5.88052383752905,83.0324444855512));
#29243=CARTESIAN_POINT('Ctrl Pts',(3.33060584155262,5.89065147415317,83.0334146482556));
#29244=CARTESIAN_POINT('Ctrl Pts',(3.3127129717843,5.90069671874195,83.03438481096));
#29245=CARTESIAN_POINT('Ctrl Pts',(3.24226969262992,5.94024431384009,83.038204290065));
#29246=CARTESIAN_POINT('Ctrl Pts',(3.17107508926453,5.97855445657467,83.0420237691701));
#29247=CARTESIAN_POINT('Ctrl Pts',(3.09917575053248,6.01559628526645,83.0458432482751));
#29248=CARTESIAN_POINT('Ctrl Pts',(3.09917575053255,6.01559628526641,81.0455808655427));
#29249=CARTESIAN_POINT('Ctrl Pts',(2.94387255360249,6.09560695737296,81.0537971731457));
#29250=CARTESIAN_POINT('Ctrl Pts',(2.78558799776598,6.16953832751457,81.0620134807487));
#29251=CARTESIAN_POINT('Ctrl Pts',(2.62484427732996,6.23718538443168,81.0702297883517));
#29252=CARTESIAN_POINT('Ctrl Pts',(2.46398711339998,6.30488018267562,81.0784518945429));
#29253=CARTESIAN_POINT('Ctrl Pts',(2.3006676600825,6.36628170274451,81.0866740007341));
#29254=CARTESIAN_POINT('Ctrl Pts',(2.13542368240621,6.42123467073262,81.0948961069253));
#29255=CARTESIAN_POINT('Ctrl Pts',(1.96995434617089,6.47626258318682,81.1031294263663));
#29256=CARTESIAN_POINT('Ctrl Pts',(1.80255558755721,6.5248242846923,81.1113627458073));
#29257=CARTESIAN_POINT('Ctrl Pts',(1.63377659615256,6.56681528854468,81.1195960652483));
#29258=CARTESIAN_POINT('Ctrl Pts',(1.5968775088955,6.57599551709247,81.1213960639919));
#29259=CARTESIAN_POINT('Ctrl Pts',(1.55991247486456,6.58486188688256,81.1231960627355));
#29260=CARTESIAN_POINT('Ctrl Pts',(1.52288726532626,6.59341363613016,81.1249960614791));
#29261=CARTESIAN_POINT('Ctrl Pts',(1.35516514076932,6.63215258103748,81.1331499549272));
#29262=CARTESIAN_POINT('Ctrl Pts',(1.18568915885699,6.66455107448763,81.1413038483754));
#29263=CARTESIAN_POINT('Ctrl Pts',(1.01498429781996,6.6904481072032,81.1494577418236));
#29264=CARTESIAN_POINT('Ctrl Pts',(0.844487744228896,6.71631353833046,81.1576016852521));
#29265=CARTESIAN_POINT('Ctrl Pts',(0.672765653975801,6.73569324650873,81.1657456286807));
#29266=CARTESIAN_POINT('Ctrl Pts',(0.500357038199068,6.74847626018827,81.1738895721092));
#29267=CARTESIAN_POINT('Ctrl Pts',(0.328122520375613,6.76124636560039,81.1820252917963));
#29268=CARTESIAN_POINT('Ctrl Pts',(0.15520321906578,6.76743301108239,81.1901610114834));
#29269=CARTESIAN_POINT('Ctrl Pts',(-0.017852813039725,6.76697645016344,
81.1982967311705));
#29270=CARTESIAN_POINT('Ctrl Pts',(-0.190770495782425,6.76652025424137,
81.2064259467697));
#29271=CARTESIAN_POINT('Ctrl Pts',(-0.363824327734731,6.75943142743707,
81.2145551623689));
#29272=CARTESIAN_POINT('Ctrl Pts',(-0.536462301573337,6.74570212794715,
81.2226843779682));
#29273=CARTESIAN_POINT('Ctrl Pts',(-0.708998559514368,6.73198091756989,
81.2308088039464));
#29274=CARTESIAN_POINT('Ctrl Pts',(-0.8811190837007,6.71162705495622,81.2389332299247));
#29275=CARTESIAN_POINT('Ctrl Pts',(-1.0522730425815,6.68468476772512,81.2470576559029));
#29276=CARTESIAN_POINT('Ctrl Pts',(-1.22446597091993,6.65757893058998,81.2552314002289));
#29277=CARTESIAN_POINT('Ctrl Pts',(-1.39568018537786,6.62380441962481,81.2634051445548));
#29278=CARTESIAN_POINT('Ctrl Pts',(-1.5653605731913,6.58345921806297,81.2715788888808));
#29279=CARTESIAN_POINT('Ctrl Pts',(-1.73395442124339,6.543372364954,81.2797002930493));
#29280=CARTESIAN_POINT('Ctrl Pts',(-1.90103367393275,6.49679883350736,81.2878216972178));
#29281=CARTESIAN_POINT('Ctrl Pts',(-2.06606496300445,6.44388582833723,81.2959431013864));
#29282=CARTESIAN_POINT('Ctrl Pts',(-2.23110901142692,6.39096873221201,81.3040651334591));
#29283=CARTESIAN_POINT('Ctrl Pts',(-2.39410443230724,6.33171129775786,81.3121871655319));
#29284=CARTESIAN_POINT('Ctrl Pts',(-2.55453415242879,6.26631025916168,81.3203091976047));
#29285=CARTESIAN_POINT('Ctrl Pts',(-2.71500682563224,6.20089171024282,81.3284334042515));
#29286=CARTESIAN_POINT('Ctrl Pts',(-2.87291209150143,6.12932642004497,81.3365576108983));
#29287=CARTESIAN_POINT('Ctrl Pts',(-3.02775399318628,6.05185878526131,81.3446818175451));
#29288=CARTESIAN_POINT('Ctrl Pts',(-3.18427188053063,5.97355265234789,81.3528939593935));
#29289=CARTESIAN_POINT('Ctrl Pts',(-3.33765935799626,5.88921582712286,81.3611061012419));
#29290=CARTESIAN_POINT('Ctrl Pts',(-3.48743157806289,5.79914735011362,81.3693182430903));
#29291=CARTESIAN_POINT('Ctrl Pts',(-3.63583660969516,5.70990105882087,81.3774554208008));
#29292=CARTESIAN_POINT('Ctrl Pts',(-3.78069184137684,5.61502757559133,81.3855925985113));
#29293=CARTESIAN_POINT('Ctrl Pts',(-3.92155680569367,5.51486003627632,81.3937297762218));
#29294=CARTESIAN_POINT('Ctrl Pts',(-4.06436835781731,5.41330829960881,81.4019794001391));
#29295=CARTESIAN_POINT('Ctrl Pts',(-4.20307824269482,5.30631535989489,81.4102290240565));
#29296=CARTESIAN_POINT('Ctrl Pts',(-4.33726443674413,5.19426859199201,81.4184786479738));
#29297=CARTESIAN_POINT('Ctrl Pts',(-4.47145063079335,5.08222182408921,81.4267282718911));
#29298=CARTESIAN_POINT('Ctrl Pts',(-4.60111289085595,4.96512153283837,81.4349778958085));
#29299=CARTESIAN_POINT('Ctrl Pts',(-4.72587030010071,4.84339126094785,81.4432275197258));
#29300=CARTESIAN_POINT('Ctrl Pts',(-4.84862596813934,4.72361415963656,81.4513447778604));
#29301=CARTESIAN_POINT('Ctrl Pts',(-4.967020259715,4.59897661286981,81.4594620359949));
#29302=CARTESIAN_POINT('Ctrl Pts',(-5.08063812871043,4.46983279386308,81.4675792941295));
#29303=CARTESIAN_POINT('Ctrl Pts',(-5.19412536666736,4.34083745670469,81.4756872195256));
#29304=CARTESIAN_POINT('Ctrl Pts',(-5.30284687153531,4.20734643475976,81.4837951449216));
#29305=CARTESIAN_POINT('Ctrl Pts',(-5.40642239704789,4.06975255570888,81.4919030703177));
#29306=CARTESIAN_POINT('Ctrl Pts',(-5.50990108083009,3.93228732509373,81.500003414912));
#29307=CARTESIAN_POINT('Ctrl Pts',(-5.60824314329255,3.79072716765027,81.5081037595063));
#29308=CARTESIAN_POINT('Ctrl Pts',(-5.70110683920205,3.64549993937782,81.5162041041006));
#29309=CARTESIAN_POINT('Ctrl Pts',(-5.79389713109863,3.50038750581859,81.5242980457859));
#29310=CARTESIAN_POINT('Ctrl Pts',(-5.88121748434763,3.35161408544836,81.5323919874712));
#29311=CARTESIAN_POINT('Ctrl Pts',(-5.96276803091265,3.19963848106721,81.5404859291564));
#29312=CARTESIAN_POINT('Ctrl Pts',(-6.04428338719127,3.04772845644327,81.5485763781842));
#29313=CARTESIAN_POINT('Ctrl Pts',(-6.12003371792392,2.89261932275003,81.556666827212));
#29314=CARTESIAN_POINT('Ctrl Pts',(-6.18976379603621,2.73479672906039,81.5647572762398));
#29315=CARTESIAN_POINT('Ctrl Pts',(-6.25947732487724,2.57701159193161,81.5728458051344));
#29316=CARTESIAN_POINT('Ctrl Pts',(-6.32317329671697,2.41651461460409,81.580934334029));
#29317=CARTESIAN_POINT('Ctrl Pts',(-6.38064360341805,2.25381370262947,81.5890228629236));
#29318=CARTESIAN_POINT('Ctrl Pts',(-6.43811142968165,2.0911198128801,81.5971110427147));
#29319=CARTESIAN_POINT('Ctrl Pts',(-6.48935400421463,1.92622252658037,81.6051992225057));
#29320=CARTESIAN_POINT('Ctrl Pts',(-6.53421233085119,1.75964718490734,81.6132874022967));
#29321=CARTESIAN_POINT('Ctrl Pts',(-6.57909237290122,1.59299120597718,81.621379497485));
#29322=CARTESIAN_POINT('Ctrl Pts',(-6.61758189679574,1.42465590580469,81.6294715926733));
#29323=CARTESIAN_POINT('Ctrl Pts',(-6.64957240512015,1.25517960032207,81.6375636878615));
#29324=CARTESIAN_POINT('Ctrl Pts',(-6.68157167014302,1.08565690442609,81.645657998083));
#29325=CARTESIAN_POINT('Ctrl Pts',(-6.707068317244,0.914992945643581,81.6537523083045));
#29326=CARTESIAN_POINT('Ctrl Pts',(-6.72600549102029,0.743733241669988,
81.6618466185259));
#29327=CARTESIAN_POINT('Ctrl Pts',(-6.74495917228062,0.572324251067659,
81.6699479845361));
#29328=CARTESIAN_POINT('Ctrl Pts',(-6.75734193290791,0.400318846176341,
81.6780493505463));
#29329=CARTESIAN_POINT('Ctrl Pts',(-6.76314897039875,0.228265205833898,
81.6861507165564));
#29330=CARTESIAN_POINT('Ctrl Pts',(-6.76578417235999,0.150188201649751,
81.6898270722942));
#29331=CARTESIAN_POINT('Ctrl Pts',(-6.76706595052292,0.0721012471304621,
81.6935034280319));
#29332=CARTESIAN_POINT('Ctrl Pts',(-6.76699738887189,-0.00594466156220883,
81.6971797837697));
#29333=CARTESIAN_POINT('',(-6.767,4.06094923584722E-12,81.3028202161898));
#29334=CARTESIAN_POINT('Ctrl Pts',(3.09917575053259,6.01559628526639,80.651216691749));
#29335=CARTESIAN_POINT('Ctrl Pts',(2.94383946288018,6.09562400538604,80.659430820505));
#29336=CARTESIAN_POINT('Ctrl Pts',(2.7855089613724,6.16957580012018,80.6676449492608));
#29337=CARTESIAN_POINT('Ctrl Pts',(2.62470545272606,6.2372438052741,80.6758590780168));
#29338=CARTESIAN_POINT('Ctrl Pts',(2.46368391518074,6.30500355954956,80.684084344076));
#29339=CARTESIAN_POINT('Ctrl Pts',(2.30018300496955,6.36646237140818,80.6923096101353));
#29340=CARTESIAN_POINT('Ctrl Pts',(2.13474098897898,6.42146166460356,80.7005348761945));
#29341=CARTESIAN_POINT('Ctrl Pts',(1.99084271420704,6.46929898910123,80.7076890539793));
#29342=CARTESIAN_POINT('Ctrl Pts',(1.84547632817944,6.51225032196516,80.714843231764));
#29343=CARTESIAN_POINT('Ctrl Pts',(1.69900208345931,6.55024281385056,80.7219974095488));
#29344=CARTESIAN_POINT('Ctrl Pts',(1.52198592333032,6.59615726823219,80.730643332815));
#29345=CARTESIAN_POINT('Ctrl Pts',(1.34294978917248,6.63493281563262,80.7392892560813));
#29346=CARTESIAN_POINT('Ctrl Pts',(1.16248299663846,6.66640249928899,80.7479351793476));
#29347=CARTESIAN_POINT('Ctrl Pts',(0.982247045968157,6.69783192888907,80.7565700432882));
#29348=CARTESIAN_POINT('Ctrl Pts',(0.800584385052222,6.72197407749631,80.7652049072287));
#29349=CARTESIAN_POINT('Ctrl Pts',(0.61809689604195,6.73871243095469,80.7738397711693));
#29350=CARTESIAN_POINT('Ctrl Pts',(0.429549570213807,6.75600661260222,80.7827613718429));
#29351=CARTESIAN_POINT('Ctrl Pts',(0.24012199781765,6.76539672476705,80.7916829725165));
#29352=CARTESIAN_POINT('Ctrl Pts',(0.0504896816497254,6.76681164153746,
80.8006045731902));
#29353=CARTESIAN_POINT('Ctrl Pts',(-0.132541039503159,6.76817730136851,
80.809215589699));
#29354=CARTESIAN_POINT('Ctrl Pts',(-0.315762144546805,6.76211363697309,
80.8178266062079));
#29355=CARTESIAN_POINT('Ctrl Pts',(-0.498560400104501,6.74860922912622,
80.8264376227167));
#29356=CARTESIAN_POINT('Ctrl Pts',(-0.681186277478519,6.73511755589375,
80.8350405190639));
#29357=CARTESIAN_POINT('Ctrl Pts',(-0.863389797227727,6.71419915086027,
80.8436434154111));
#29358=CARTESIAN_POINT('Ctrl Pts',(-1.04455831853247,6.68589462369731,80.8522463117583));
#29359=CARTESIAN_POINT('Ctrl Pts',(-1.2255239892674,6.65762178851607,80.860839575624));
#29360=CARTESIAN_POINT('Ctrl Pts',(-1.40545667279565,6.62197937676768,80.8694328394897));
#29361=CARTESIAN_POINT('Ctrl Pts',(-1.58374922023413,6.57905976621339,80.8780261033554));
#29362=CARTESIAN_POINT('Ctrl Pts',(-1.6036179751965,6.57427684489988,80.8789837286545));
#29363=CARTESIAN_POINT('Ctrl Pts',(-1.62346636815287,6.56940360340689,80.8799413539537));
#29364=CARTESIAN_POINT('Ctrl Pts',(-1.64329356408214,6.56444020935877,80.8808989792528));
#29365=CARTESIAN_POINT('Ctrl Pts',(-1.82126542019569,6.51988804704001,80.889494766199));
#29366=CARTESIAN_POINT('Ctrl Pts',(-1.99731995182512,6.46812021392288,80.8980905531452));
#29367=CARTESIAN_POINT('Ctrl Pts',(-2.1708754615811,6.40933606002253,80.9066863400914));
#29368=CARTESIAN_POINT('Ctrl Pts',(-2.3445929232905,6.35049705215316,80.9152901481283));
#29369=CARTESIAN_POINT('Ctrl Pts',(-2.51580641932027,6.28462875294149,80.9238939561653));
#29370=CARTESIAN_POINT('Ctrl Pts',(-2.68395367229331,6.21197888639226,80.9324977642022));
#29371=CARTESIAN_POINT('Ctrl Pts',(-2.85870835083578,6.13647420909016,80.9414396629317));
#29372=CARTESIAN_POINT('Ctrl Pts',(-3.03015059433496,6.05364437954267,80.9503815616612));
#29373=CARTESIAN_POINT('Ctrl Pts',(-3.19767795007734,5.96381964244302,80.9593234603907));
#29374=CARTESIAN_POINT('Ctrl Pts',(-3.35931003947585,5.87715582641876,80.9679506948411));
#29375=CARTESIAN_POINT('Ctrl Pts',(-3.51729784406443,5.7839812063096,80.9765779292915));
#29376=CARTESIAN_POINT('Ctrl Pts',(-3.67113009209778,5.68463656242808,80.9852051637419));
#29377=CARTESIAN_POINT('Ctrl Pts',(-3.82510885017376,5.58519730257237,80.9938406147821));
#29378=CARTESIAN_POINT('Ctrl Pts',(-3.97492390079849,5.47957646234283,81.0024760658224));
#29379=CARTESIAN_POINT('Ctrl Pts',(-4.12009545277081,5.36815633714754,81.0111115168626));
#29380=CARTESIAN_POINT('Ctrl Pts',(-4.26548148184185,5.25657159936208,81.0197597259567));
#29381=CARTESIAN_POINT('Ctrl Pts',(-4.40621006613223,5.1391706470642,81.0284079350509));
#29382=CARTESIAN_POINT('Ctrl Pts',(-4.54183567309202,5.01637495793813,81.037056144145));
#29383=CARTESIAN_POINT('Ctrl Pts',(-4.55618205641998,5.00338571448542,81.0379709457488));
#29384=CARTESIAN_POINT('Ctrl Pts',(-4.57047137642931,4.99033614058141,81.0388857473526));
#29385=CARTESIAN_POINT('Ctrl Pts',(-4.58470313105571,4.97722675795347,81.0398005489564));
#29386=CARTESIAN_POINT('Ctrl Pts',(-4.71032631150992,4.86151071430702,81.0478754694404));
#29387=CARTESIAN_POINT('Ctrl Pts',(-4.83176307243518,4.74085362904437,81.0559503899244));
#29388=CARTESIAN_POINT('Ctrl Pts',(-4.94859208424996,4.61559588609083,81.0640253104084));
#29389=CARTESIAN_POINT('Ctrl Pts',(-5.06529578359498,4.49047249638468,81.0720915696171));
#29390=CARTESIAN_POINT('Ctrl Pts',(-5.17740131799069,4.36075854015743,81.0801578288258));
#29391=CARTESIAN_POINT('Ctrl Pts',(-5.28452114638662,4.22683395148103,81.0882240880345));
#29392=CARTESIAN_POINT('Ctrl Pts',(-5.39154949671538,4.09302373156997,81.0962834588285));
#29393=CARTESIAN_POINT('Ctrl Pts',(-5.49360038454914,3.95501032620842,81.1043428296225));
#29394=CARTESIAN_POINT('Ctrl Pts',(-5.59032388366367,3.81320965536115,81.1124022004165));
#29395=CARTESIAN_POINT('Ctrl Pts',(-5.68698497174893,3.67150048167745,81.1204563708855));
#29396=CARTESIAN_POINT('Ctrl Pts',(-5.7783253060897,3.52600921521733,81.1285105413546));
#29397=CARTESIAN_POINT('Ctrl Pts',(-5.86403602602228,3.37718380984999,81.1365647118237));
#29398=CARTESIAN_POINT('Ctrl Pts',(-5.94971711686435,3.22840985150594,81.1446160980698));
#29399=CARTESIAN_POINT('Ctrl Pts',(-6.02977227964826,3.07630437018704,81.152667484316));
#29400=CARTESIAN_POINT('Ctrl Pts',(-6.10393667416835,2.92134319752792,81.1607188705622));
#29401=CARTESIAN_POINT('Ctrl Pts',(-6.17809008621871,2.76640497195007,81.1687690645367));
#29402=CARTESIAN_POINT('Ctrl Pts',(-6.24635430532472,2.60861223298746,81.1768192585112));
#29403=CARTESIAN_POINT('Ctrl Pts',(-6.308511115388,2.44846411185176,81.1848694524858));
#29404=CARTESIAN_POINT('Ctrl Pts',(-6.37067100353014,2.28830805999141,81.1929200451154));
#29405=CARTESIAN_POINT('Ctrl Pts',(-6.4267227466436,2.12579674180012,81.2009706377451));
#29406=CARTESIAN_POINT('Ctrl Pts',(-6.47649686715468,1.96144776370305,81.2090212303748));
#29407=CARTESIAN_POINT('Ctrl Pts',(-6.52630621734081,1.7969824608767,81.2170775211415));
#29408=CARTESIAN_POINT('Ctrl Pts',(-6.56982895997579,1.63067725702817,81.2251338119083));
#29409=CARTESIAN_POINT('Ctrl Pts',(-6.60694580497785,1.46306395283513,81.233190102675));
#29410=CARTESIAN_POINT('Ctrl Pts',(-6.64407584250108,1.29539107347988,81.2412492569068));
#29411=CARTESIAN_POINT('Ctrl Pts',(-6.67479537818248,1.12640953403713,81.2493084111385));
#29412=CARTESIAN_POINT('Ctrl Pts',(-6.69903664510372,0.956659305896044,
81.2573675653703));
#29413=CARTESIAN_POINT('Ctrl Pts',(-6.72330692248817,0.786705931081017,
81.2654363643041));
#29414=CARTESIAN_POINT('Ctrl Pts',(-6.74108340262473,0.615982400497209,
81.2735051632379));
#29415=CARTESIAN_POINT('Ctrl Pts',(-6.7523503267723,0.445032655586101,81.2815739621717));
#29416=CARTESIAN_POINT('Ctrl Pts',(-6.7621241711247,0.29673697373359,81.2885734931757));
#29417=CARTESIAN_POINT('Ctrl Pts',(-6.76700025229275,0.148271235916897,
81.2955730241797));
#29418=CARTESIAN_POINT('Ctrl Pts',(-6.76699999999021,-1.15140253983646E-5,
81.3025725551836));
#29419=CARTESIAN_POINT('Ctrl Pts',(-6.767,4.06094923160091E-12,81.3028202161898));
#29420=CARTESIAN_POINT('Ctrl Pts',(-6.76700000000011,-0.186007249411735,
81.3115697279958));
#29421=CARTESIAN_POINT('Ctrl Pts',(-6.75932637295459,-0.372014355523709,
81.3203192398017));
#29422=CARTESIAN_POINT('Ctrl Pts',(-6.74400518266958,-0.55738953715135,
81.3290687516077));
#29423=CARTESIAN_POINT('Ctrl Pts',(-6.72868405709685,-0.742763935807834,
81.3378182264582));
#29424=CARTESIAN_POINT('Ctrl Pts',(-6.70571545653039,-0.927506129691614,
81.3465677013088));
#29425=CARTESIAN_POINT('Ctrl Pts',(-6.67517739415705,-1.11098863924648,
81.3553171761593));
#29426=CARTESIAN_POINT('Ctrl Pts',(-6.6446394582313,-1.29447038906349,81.3640666147813));
#29427=CARTESIAN_POINT('Ctrl Pts',(-6.60653217027189,-1.47669218228075,
81.3728160534033));
#29428=CARTESIAN_POINT('Ctrl Pts',(-6.56098496116745,-1.65703510503991,
81.3815654920253));
#29429=CARTESIAN_POINT('Ctrl Pts',(-6.51543793687553,-1.83737729603892,
81.3903148951455));
#29430=CARTESIAN_POINT('Ctrl Pts',(-6.46245112202678,-2.01584035396928,
81.3990642982657));
#29431=CARTESIAN_POINT('Ctrl Pts',(-6.40220448416285,-2.1918181363802,81.407813701386));
#29432=CARTESIAN_POINT('Ctrl Pts',(-6.34195808575226,-2.36779521935841,
81.4165630697313));
#29433=CARTESIAN_POINT('Ctrl Pts',(-6.27445201489269,-2.54128677544744,
81.4253124380765));
#29434=CARTESIAN_POINT('Ctrl Pts',(-6.19991555136212,-2.71170355237777,
81.4340618064218));
#29435=CARTESIAN_POINT('Ctrl Pts',(-6.12537937789079,-2.88211966612984,
81.4428111407189));
#29436=CARTESIAN_POINT('Ctrl Pts',(-6.04381298133671,-3.04946076210335,
81.4515604750159));
#29437=CARTESIAN_POINT('Ctrl Pts',(-5.95549339426377,-3.21315848206723,
81.4603098093129));
#29438=CARTESIAN_POINT('Ctrl Pts',(-5.86717414355229,-3.37685557859519,
81.4690591102885));
#29439=CARTESIAN_POINT('Ctrl Pts',(-5.77210188986302,-3.53690907467208,
81.4778084112641));
#29440=CARTESIAN_POINT('Ctrl Pts',(-5.67059953467127,-3.69277536784814,
81.4865577122397));
#29441=CARTESIAN_POINT('Ctrl Pts',(-5.56909755761821,-3.84864108035713,
81.4953069806204));
#29442=CARTESIAN_POINT('Ctrl Pts',(-5.46116568338121,-4.0003193810421,81.5040562490012));
#29443=CARTESIAN_POINT('Ctrl Pts',(-5.34717048686161,-4.14729511663159,
81.512805517382));
#29444=CARTESIAN_POINT('Ctrl Pts',(-5.23317570555567,-4.2942703168798,81.5215547538946));
#29445=CARTESIAN_POINT('Ctrl Pts',(-5.11311782178858,-4.43654275987068,
81.5303039904072));
#29446=CARTESIAN_POINT('Ctrl Pts',(-4.98740459172071,-4.57362924147588,
81.5390532269198));
#29447=CARTESIAN_POINT('Ctrl Pts',(-4.86169180910878,-4.71071523514387,
81.5478024322909));
#29448=CARTESIAN_POINT('Ctrl Pts',(-4.73032391415469,-4.84261509316487,
81.5565516376621));
#29449=CARTESIAN_POINT('Ctrl Pts',(-4.5937470723732,-4.96888084331499,81.5653008430332));
#29450=CARTESIAN_POINT('Ctrl Pts',(-4.45717070537429,-5.09514615452701,
81.5740500179894));
#29451=CARTESIAN_POINT('Ctrl Pts',(-4.31538563819536,-5.21577720253611,
81.5827991929456));
#29452=CARTESIAN_POINT('Ctrl Pts',(-4.16887341290675,-5.33036429028629,
81.5915483679019));
#29453=CARTESIAN_POINT('Ctrl Pts',(-4.02236168477388,-5.44495098921139,
81.6002975131698));
#29454=CARTESIAN_POINT('Ctrl Pts',(-3.87112305634513,-5.55349359238706,
81.6090466584377));
#29455=CARTESIAN_POINT('Ctrl Pts',(-3.71567117316832,-5.65562346102408,
81.6177958037056));
#29456=CARTESIAN_POINT('Ctrl Pts',(-3.56021980457387,-5.75775299158717,
81.6265449200118));
#29457=CARTESIAN_POINT('Ctrl Pts',(-3.40055544862459,-5.85346967275312,
81.6352940363179));
#29458=CARTESIAN_POINT('Ctrl Pts',(-3.23722036323458,-5.94244842803531,
81.6440431526241));
#29459=CARTESIAN_POINT('Ctrl Pts',(-3.07388580496141,-6.03142689616426,
81.652792240695));
#29460=CARTESIAN_POINT('Ctrl Pts',(-2.90688079257841,-6.11366734484757,
81.6615413287659));
#29461=CARTESIAN_POINT('Ctrl Pts',(-2.73677251094791,-6.18889046787224,
81.6702904168369));
#29462=CARTESIAN_POINT('Ctrl Pts',(-2.5666647641681,-6.26411335438203,81.6790394773991));
#29463=CARTESIAN_POINT('Ctrl Pts',(-2.39345402972247,-6.33231884350233,
81.6877885379614));
#29464=CARTESIAN_POINT('Ctrl Pts',(-2.2177285647418,-6.39327529620994,81.6965375985236));
#29465=CARTESIAN_POINT('Ctrl Pts',(-2.04200363768409,-6.45423156232038,
81.7052866323036));
#29466=CARTESIAN_POINT('Ctrl Pts',(-1.86376426620231,-6.50793874252016,
81.7140356660836));
#29467=CARTESIAN_POINT('Ctrl Pts',(-1.68361578194824,-6.55421443796088,
81.7227846998636));
#29468=CARTESIAN_POINT('Ctrl Pts',(-1.50346783420042,-6.60048999558639,
81.7315337075878));
#29469=CARTESIAN_POINT('Ctrl Pts',(-1.3214110625746,-6.63933404145452,81.740282715312));
#29470=CARTESIAN_POINT('Ctrl Pts',(-1.13806375959297,-6.67061465526987,
81.7490317230362));
#29471=CARTESIAN_POINT('Ctrl Pts',(-0.95471698742188,-6.70189517852441,
81.7577807054311));
#29472=CARTESIAN_POINT('Ctrl Pts',(-0.770079973812807,-6.72561226535794,
81.766529687826));
#29473=CARTESIAN_POINT('Ctrl Pts',(-0.584779770555591,-6.74168536939755,
81.7752786702209));
#29474=CARTESIAN_POINT('Ctrl Pts',(-0.391490647557044,-6.75845143942376,
81.7844048508969));
#29475=CARTESIAN_POINT('Ctrl Pts',(-0.197480213107461,-6.76689975924017,
81.793531031573));
#29476=CARTESIAN_POINT('Ctrl Pts',(-0.00346532630091309,-6.76699911271707,
81.802657212249));
#29477=CARTESIAN_POINT('Ctrl Pts',(0.184486595292899,-6.76709536139782,
81.8114981997789));
#29478=CARTESIAN_POINT('Ctrl Pts',(0.372442378182036,-6.75935659726787,
81.8203391873089));
#29479=CARTESIAN_POINT('Ctrl Pts',(0.55975021771886,-6.74380965729043,81.8291801748388));
#29480=CARTESIAN_POINT('Ctrl Pts',(0.745129914454533,-6.72842275717289,
81.8379301534366));
#29481=CARTESIAN_POINT('Ctrl Pts',(0.929874656310971,-6.70538772273517,
81.8466801320343));
#29482=CARTESIAN_POINT('Ctrl Pts',(1.11335688289457,-6.67478280180796,81.8554301106321));
#29483=CARTESIAN_POINT('Ctrl Pts',(1.29683723118525,-6.64417819418088,81.864179999657));
#29484=CARTESIAN_POINT('Ctrl Pts',(1.47905480729892,-6.60600390230151,81.872929888682));
#29485=CARTESIAN_POINT('Ctrl Pts',(1.65939064804455,-6.56038959797224,81.8816797777069));
#29486=CARTESIAN_POINT('Ctrl Pts',(1.83972470263919,-6.51477574543354,81.8904295800679));
#29487=CARTESIAN_POINT('Ctrl Pts',(2.0181767812551,-6.46172209820206,81.8991793824288));
#29488=CARTESIAN_POINT('Ctrl Pts',(2.1941407234735,-6.40140886724127,81.9079291847898));
#29489=CARTESIAN_POINT('Ctrl Pts',(2.37010298131777,-6.34109621361494,81.9166789033953));
#29490=CARTESIAN_POINT('Ctrl Pts',(2.54357687926603,-6.27352420826097,81.9254286220008));
#29491=CARTESIAN_POINT('Ctrl Pts',(2.71397317789672,-6.19892237325628,81.9341783406062));
#29492=CARTESIAN_POINT('Ctrl Pts',(2.8843679020691,-6.12432122757101,81.9429279783645));
#29493=CARTESIAN_POINT('Ctrl Pts',(3.05168482125974,-6.0426904971756,81.9516776161228));
#29494=CARTESIAN_POINT('Ctrl Pts',(3.21535561997114,-5.95430745235078,81.960427253881));
#29495=CARTESIAN_POINT('Ctrl Pts',(3.37902496075009,-5.86592519481673,81.9691768137));
#29496=CARTESIAN_POINT('Ctrl Pts',(3.53904799384607,-5.77079087940396,81.9779263735191));
#29497=CARTESIAN_POINT('Ctrl Pts',(3.6948811881472,-5.66922763747197,81.9866759333381));
#29498=CARTESIAN_POINT('Ctrl Pts',(3.85071304610564,-5.56766526649237,81.9954254181255));
#29499=CARTESIAN_POINT('Ctrl Pts',(4.00235489705696,-5.45967423580913,82.004174902913));
#29500=CARTESIAN_POINT('Ctrl Pts',(4.14929168607379,-5.34562133936542,82.0129243877004));
#29501=CARTESIAN_POINT('Ctrl Pts',(4.29622726385489,-5.23156938308751,82.0216738003637));
#29502=CARTESIAN_POINT('Ctrl Pts',(4.43845763091805,-5.1114558367743,82.030423213027));
#29503=CARTESIAN_POINT('Ctrl Pts',(4.57549970660707,-4.98568866204446,82.0391726256903));
#29504=CARTESIAN_POINT('Ctrl Pts',(4.71254069815039,-4.85992248226409,82.0479219691366));
#29505=CARTESIAN_POINT('Ctrl Pts',(4.84439326931058,-4.72850295734264,82.0566713125829));
#29506=CARTESIAN_POINT('Ctrl Pts',(4.97060959434444,-4.59187644221957,82.0654206560292));
#29507=CARTESIAN_POINT('Ctrl Pts',(5.09682496280273,-4.45525096256941,82.0741699331655));
#29508=CARTESIAN_POINT('Ctrl Pts',(5.21740397615609,-4.31341878218604,82.0829192103018));
#29509=CARTESIAN_POINT('Ctrl Pts',(5.33193710451716,-4.16686161438956,82.0916684874381));
#29510=CARTESIAN_POINT('Ctrl Pts',(5.44646940289169,-4.02030550864803,82.1004177011711));
#29511=CARTESIAN_POINT('Ctrl Pts',(5.55495572749456,-3.86902470980433,82.1091669149041));
#29512=CARTESIAN_POINT('Ctrl Pts',(5.65702762491252,-3.71353301466092,82.117916128637));
#29513=CARTESIAN_POINT('Ctrl Pts',(5.7590988165496,-3.55804239467207,82.1266652818731));
#29514=CARTESIAN_POINT('Ctrl Pts',(5.85475551250599,-3.39834117619869,82.1354144351093));
#29515=CARTESIAN_POINT('Ctrl Pts',(5.94367283727921,-3.23497174692288,82.1441635883454));
#29516=CARTESIAN_POINT('Ctrl Pts',(6.03258957676142,-3.07160339301297,82.1529126839909));
#29517=CARTESIAN_POINT('Ctrl Pts',(6.11476689685121,-2.90456712829848,82.1616617796364));
#29518=CARTESIAN_POINT('Ctrl Pts',(6.18992570525104,-2.73443024476261,82.1704108752819));
#29519=CARTESIAN_POINT('Ctrl Pts',(6.26508404388558,-2.56429442463373,82.179159916243));
#29520=CARTESIAN_POINT('Ctrl Pts',(6.33322384283191,-2.39105828656321,82.187908957204));
#29521=CARTESIAN_POINT('Ctrl Pts',(6.39411368719924,-2.21531017132395,82.1966579981651));
#29522=CARTESIAN_POINT('Ctrl Pts',(6.45500317120789,-2.03956309619835,82.2054069873475));
#29523=CARTESIAN_POINT('Ctrl Pts',(6.5086426926998,-1.86130434438959,82.2141559765299));
#29524=CARTESIAN_POINT('Ctrl Pts',(6.55485008446248,-1.68113930720276,82.2229049657123));
#29525=CARTESIAN_POINT('Ctrl Pts',(6.60199664749329,-1.49731239212169,82.2318317792416));
#29526=CARTESIAN_POINT('Ctrl Pts',(6.64140563640842,-1.31150116499997,82.240758592771));
#29527=CARTESIAN_POINT('Ctrl Pts',(6.67293772282118,-1.12436255155982,82.2496854063004));
#29528=CARTESIAN_POINT('Ctrl Pts',(6.70384494949825,-0.940932395054639,
82.2584353204559));
#29529=CARTESIAN_POINT('Ctrl Pts',(6.72718449348892,-0.756227260510083,
82.2671852346114));
#29530=CARTESIAN_POINT('Ctrl Pts',(6.74287707373903,-0.57087456454513,82.2759351487669));
#29531=CARTESIAN_POINT('Ctrl Pts',(6.7585693453865,-0.385525513636003,82.2846848908509));
#29532=CARTESIAN_POINT('Ctrl Pts',(6.76661493004092,-0.199529212421841,
82.2934346329349));
#29533=CARTESIAN_POINT('Ctrl Pts',(6.76698649908906,-0.0135174386041215,
82.3021843750189));
#29534=CARTESIAN_POINT('Ctrl Pts',(6.76735806132399,0.172490924442033,82.3109339566648));
#29535=CARTESIAN_POINT('Ctrl Pts',(6.76005588896309,0.358514472897615,82.3196835383107));
#29536=CARTESIAN_POINT('Ctrl Pts',(6.74510478454615,0.543921359658378,82.3284331199566));
#29537=CARTESIAN_POINT('Ctrl Pts',(6.73015393440729,0.729325093146674,82.3371825527956));
#29538=CARTESIAN_POINT('Ctrl Pts',(6.70755443556948,0.914111900252648,82.3459319856346));
#29539=CARTESIAN_POINT('Ctrl Pts',(6.67738304682378,1.09765415591175,82.3546814184737));
#29540=CARTESIAN_POINT('Ctrl Pts',(6.64721213111929,1.28119353390919,82.363430714135));
#29541=CARTESIAN_POINT('Ctrl Pts',(6.60946960955571,1.46348811672309,82.3721800097964));
#29542=CARTESIAN_POINT('Ctrl Pts',(6.56428366991267,1.64391876347888,82.3809293054577));
#29543=CARTESIAN_POINT('Ctrl Pts',(6.51909837867808,1.82434682109394,82.3896784755685));
#29544=CARTESIAN_POINT('Ctrl Pts',(6.46646995272017,2.00291071820135,82.3984276456794));
#29545=CARTESIAN_POINT('Ctrl Pts',(6.4065771328165,2.17900400212406,82.4071768157902));
#29546=CARTESIAN_POINT('Ctrl Pts',(6.34668509279169,2.35509499309363,82.415925871976));
#29547=CARTESIAN_POINT('Ctrl Pts',(6.27952894037644,2.52871516397829,82.4246749281617));
#29548=CARTESIAN_POINT('Ctrl Pts',(6.20533675061573,2.69927486771129,82.4334239843475));
#29549=CARTESIAN_POINT('Ctrl Pts',(6.12832117908046,2.87632521635649,82.4425059856298));
#29550=CARTESIAN_POINT('Ctrl Pts',(6.0437236662621,3.0500772891974,82.4515879869121));
#29551=CARTESIAN_POINT('Ctrl Pts',(5.95185378007998,3.21989527477954,82.4606699881943));
#29552=CARTESIAN_POINT('Ctrl Pts',(5.86334450817511,3.3835012928651,82.4694197685015));
#29553=CARTESIAN_POINT('Ctrl Pts',(5.76808562057404,3.5434556712472,82.4781695488086));
#29554=CARTESIAN_POINT('Ctrl Pts',(5.66640068804642,3.69921508465067,82.4869193291157));
#29555=CARTESIAN_POINT('Ctrl Pts',(5.56471941108085,3.85496889852051,82.4956687948692));
#29556=CARTESIAN_POINT('Ctrl Pts',(5.45661270815278,4.00652780919414,82.5044182606227));
#29557=CARTESIAN_POINT('Ctrl Pts',(5.3424477644928,4.15337704569015,82.5131677263762));
#29558=CARTESIAN_POINT('Ctrl Pts',(5.22828631819768,4.30022178356039,82.5219169240957));
#29559=CARTESIAN_POINT('Ctrl Pts',(5.10806717844249,4.44235690972472,82.5306661218154));
#29560=CARTESIAN_POINT('Ctrl Pts',(4.98219864544905,4.57929969070442,82.539415319535));
#29561=CARTESIAN_POINT('Ctrl Pts',(4.85633329944209,4.71623900429811,82.5481642957252));
#29562=CARTESIAN_POINT('Ctrl Pts',(4.7248190403383,4.8479860248344,82.5569132719154));
#29563=CARTESIAN_POINT('Ctrl Pts',(4.58810250737377,4.97409332258961,82.5656622481057));
#29564=CARTESIAN_POINT('Ctrl Pts',(4.45137708685819,5.10020881821981,82.5744117930418));
#29565=CARTESIAN_POINT('Ctrl Pts',(4.30944892636227,5.22068366307788,82.583161337978));
#29566=CARTESIAN_POINT('Ctrl Pts',(4.16280009466835,5.33510865604715,82.5919108829142));
#29567=CARTESIAN_POINT('Ctrl Pts',(4.01615988348973,5.44952692272755,82.6006599135225));
#29568=CARTESIAN_POINT('Ctrl Pts',(3.86479978232426,5.5578958728849,82.6094089441308));
#29569=CARTESIAN_POINT('Ctrl Pts',(3.70923383581274,5.65984746713743,82.618157974739));
#29570=CARTESIAN_POINT('Ctrl Pts',(3.55366577799753,5.76180044505251,82.6269071240871));
#29571=CARTESIAN_POINT('Ctrl Pts',(3.3938920002706,5.85733573570932,82.6356562734351));
#29572=CARTESIAN_POINT('Ctrl Pts',(3.23045513626267,5.94612887621805,82.6444054227831));
#29573=CARTESIAN_POINT('Ctrl Pts',(3.18695122151726,5.9697639920661,82.6467342868961));
#29574=CARTESIAN_POINT('Ctrl Pts',(3.14318791262733,5.99292165435297,82.6490631510091));
#29575=CARTESIAN_POINT('Ctrl Pts',(3.09917575053247,6.01559628526645,82.6513920151221));
#29576=CARTESIAN_POINT('Origin',(0.,0.,-3.69717978381041));
#29577=CARTESIAN_POINT('',(3.09917575053258,6.01559628526639,85.045900138346));
#29578=CARTESIAN_POINT('',(3.0991757505325,6.01559628526643,84.6515000956437));
#29579=CARTESIAN_POINT('',(3.09917575053259,6.01559628526639,-3.69717978381041));
#29580=CARTESIAN_POINT('',(-6.76699958812818,0.00236098985609753,83.697179783854));
#29581=CARTESIAN_POINT('Ctrl Pts',(-6.76699958812818,0.00236098985609753,
83.697179783854));
#29582=CARTESIAN_POINT('Ctrl Pts',(-6.76705954036394,-0.169472342533521,
83.7053053883323));
#29583=CARTESIAN_POINT('Ctrl Pts',(-6.76057027671101,-0.341565259567424,
83.7134309928107));
#29584=CARTESIAN_POINT('Ctrl Pts',(-6.7474986903799,-0.513371623019327,
83.721556597289));
#29585=CARTESIAN_POINT('Ctrl Pts',(-6.73444109820115,-0.684994054363445,
83.7296735026742));
#29586=CARTESIAN_POINT('Ctrl Pts',(-6.714815238025,-0.856330178927854,83.7377904080594));
#29587=CARTESIAN_POINT('Ctrl Pts',(-6.68863998106626,-1.02683212049583,
83.7459073134446));
#29588=CARTESIAN_POINT('Ctrl Pts',(-6.66248716249329,-1.19718790157549,
83.7540172607222));
#29589=CARTESIAN_POINT('Ctrl Pts',(-6.62979617995887,-1.3667105614629,83.7621272079997));
#29590=CARTESIAN_POINT('Ctrl Pts',(-6.59063783953794,-1.53485565055829,
83.7702371552773));
#29591=CARTESIAN_POINT('Ctrl Pts',(-6.5515047181622,-1.70289244960474,83.7783418795264));
#29592=CARTESIAN_POINT('Ctrl Pts',(-6.50591261572719,-1.86955308703234,
83.7864466037756));
#29593=CARTESIAN_POINT('Ctrl Pts',(-6.4539837074203,-2.03430167486372,83.7945513280247));
#29594=CARTESIAN_POINT('Ctrl Pts',(-6.40205093456113,-2.19906252329428,
83.8026566554278));
#29595=CARTESIAN_POINT('Ctrl Pts',(-6.34378049746849,-2.36191067871605,
83.810761982831));
#29596=CARTESIAN_POINT('Ctrl Pts',(-6.27934513209687,-2.5223230784361,83.8188673102341));
#29597=CARTESIAN_POINT('Ctrl Pts',(-6.21494644312632,-2.68264417193828,
83.8269680241112));
#29598=CARTESIAN_POINT('Ctrl Pts',(-6.14438997264112,-2.84053193721467,
83.8350687379883));
#29599=CARTESIAN_POINT('Ctrl Pts',(-6.06789701064579,-2.99548240992932,
83.8431694518654));
#29600=CARTESIAN_POINT('Ctrl Pts',(-5.99140149515836,-3.1504380552088,83.8512704361609));
#29601=CARTESIAN_POINT('Ctrl Pts',(-5.90896925641487,-3.3024558822472,83.8593714204564));
#29602=CARTESIAN_POINT('Ctrl Pts',(-5.82086826400484,-3.45105515068961,
83.8674724047519));
#29603=CARTESIAN_POINT('Ctrl Pts',(-5.73274732437067,-3.59968806396205,
83.8755752232169));
#29604=CARTESIAN_POINT('Ctrl Pts',(-5.63895526377698,-3.7449005609918,83.8836780416819));
#29605=CARTESIAN_POINT('Ctrl Pts',(-5.53980417666195,-3.88623965862102,
83.8917808601469));
#29606=CARTESIAN_POINT('Ctrl Pts',(-5.44055444879911,-4.02771936786319,
83.8998917397244));
#29607=CARTESIAN_POINT('Ctrl Pts',(-5.33593525564391,-4.16531767772288,
83.908002619302));
#29608=CARTESIAN_POINT('Ctrl Pts',(-5.22630043182655,-4.29861289211876,
83.9161134988795));
#29609=CARTESIAN_POINT('Ctrl Pts',(-5.11661090070204,-4.43197462025528,
83.9242284257512));
#29610=CARTESIAN_POINT('Ctrl Pts',(-5.00190099635135,-4.56102869939972,
83.9323433526228));
#29611=CARTESIAN_POINT('Ctrl Pts',(-4.88256219763481,-4.68538956611161,
83.9404582794945));
#29612=CARTESIAN_POINT('Ctrl Pts',(-4.76304615833491,-4.80993513212333,
83.9485852585603));
#29613=CARTESIAN_POINT('Ctrl Pts',(-4.63888775218856,-4.92977330168086,
83.9567122376262));
#29614=CARTESIAN_POINT('Ctrl Pts',(-4.51051328349653,-5.0445573561415,83.964839216692));
#29615=CARTESIAN_POINT('Ctrl Pts',(-4.38288106340056,-5.15867774044919,
83.9729192063614));
#29616=CARTESIAN_POINT('Ctrl Pts',(-4.25108173245525,-5.26780214352434,
83.9809991960309));
#29617=CARTESIAN_POINT('Ctrl Pts',(-4.11556217166761,-5.37163262064138,
83.9890791857002));
#29618=CARTESIAN_POINT('Ctrl Pts',(-3.9776130062326,-5.47732457818439,83.9973040340184));
#29619=CARTESIAN_POINT('Ctrl Pts',(-3.83539619312975,-5.57784743904191,
84.0055288823365));
#29620=CARTESIAN_POINT('Ctrl Pts',(-3.68933537476457,-5.67283822195828,
84.0137537306546));
#29621=CARTESIAN_POINT('Ctrl Pts',(-3.54343905326622,-5.76772202419124,
84.0219693159699));
#29622=CARTESIAN_POINT('Ctrl Pts',(-3.39370764507189,-5.85708596087453,
84.0301849012852));
#29623=CARTESIAN_POINT('Ctrl Pts',(-3.24059755518394,-5.94060741720373,
84.0384004866005));
#29624=CARTESIAN_POINT('Ctrl Pts',(-3.08762913833998,-6.02405159097783,
84.0466084700197));
#29625=CARTESIAN_POINT('Ctrl Pts',(-2.93128857886769,-6.10166387994605,
84.054816453439));
#29626=CARTESIAN_POINT('Ctrl Pts',(-2.77206100954629,-6.17316505200964,
84.0630244368582));
#29627=CARTESIAN_POINT('Ctrl Pts',(-2.61294879211668,-6.244614425283,84.0712264740308));
#29628=CARTESIAN_POINT('Ctrl Pts',(-2.45095405664261,-6.30996135338351,
84.0794285112033));
#29629=CARTESIAN_POINT('Ctrl Pts',(-2.28658635047751,-6.36897259075669,
84.0876305483758));
#29630=CARTESIAN_POINT('Ctrl Pts',(-2.12230471346516,-6.42795292761223,
84.0958282906512));
#29631=CARTESIAN_POINT('Ctrl Pts',(-1.95565291804444,-6.48060406200328,
84.1040260329266));
#29632=CARTESIAN_POINT('Ctrl Pts',(-1.78716037693843,-6.52674090087092,
84.112223775202));
#29633=CARTESIAN_POINT('Ctrl Pts',(-1.61869987190167,-6.57286896758191,
84.1204199588123));
#29634=CARTESIAN_POINT('Ctrl Pts',(-1.44839966234766,-6.6124851052086,84.1286161424226));
#29635=CARTESIAN_POINT('Ctrl Pts',(-1.27680450356384,-6.64545402961145,
84.136812326033));
#29636=CARTESIAN_POINT('Ctrl Pts',(-1.10522197657826,-6.67842052704141,
84.1450079062898));
#29637=CARTESIAN_POINT('Ctrl Pts',(-0.932345042418501,-6.70474071717392,
84.1532034865466));
#29638=CARTESIAN_POINT('Ctrl Pts',(-0.758728781423026,-6.7243304228927,
84.1613990668035));
#29639=CARTESIAN_POINT('Ctrl Pts',(-0.585093713582004,-6.74392225065102,
84.1695955348401));
#29640=CARTESIAN_POINT('Ctrl Pts',(-0.410719515987915,-6.756782101216,84.1777920028767));
#29641=CARTESIAN_POINT('Ctrl Pts',(-0.236166577896974,-6.76287766764152,
84.1859884709134));
#29642=CARTESIAN_POINT('Ctrl Pts',(-0.0615629735190617,-6.7689750033854,
84.1941873180827));
#29643=CARTESIAN_POINT('Ctrl Pts',(0.113219116175861,-6.76830413158267,
84.202386165252));
#29644=CARTESIAN_POINT('Ctrl Pts',(0.287619060212619,-6.76088487375746,
84.2105850124214));
#29645=CARTESIAN_POINT('Ctrl Pts',(0.462201269150256,-6.75345786208634,
84.2187924281833));
#29646=CARTESIAN_POINT('Ctrl Pts',(0.636400175535817,-6.73926838925261,
84.2269998439452));
#29647=CARTESIAN_POINT('Ctrl Pts',(0.809659020699853,-6.71838829409252,
84.2352072597071));
#29648=CARTESIAN_POINT('Ctrl Pts',(0.983010726510958,-6.69749700793582,
84.2434190743552));
#29649=CARTESIAN_POINT('Ctrl Pts',(1.15542101269726,-6.66990800744151,84.2516308890033));
#29650=CARTESIAN_POINT('Ctrl Pts',(1.3263431798735,-6.63574432669034,84.2598427036514));
#29651=CARTESIAN_POINT('Ctrl Pts',(1.49751705592626,-6.60153033472536,84.268066611445));
#29652=CARTESIAN_POINT('Ctrl Pts',(1.66719808446835,-6.56072239677405,84.2762905192386));
#29653=CARTESIAN_POINT('Ctrl Pts',(1.83485334187446,-6.51349385612761,84.2845144270322));
#29654=CARTESIAN_POINT('Ctrl Pts',(1.98976370446868,-6.46985555650297,84.2921131660038));
#29655=CARTESIAN_POINT('Ctrl Pts',(2.14294455581183,-6.42073633812895,84.2997119049754));
#29656=CARTESIAN_POINT('Ctrl Pts',(2.29399148015313,-6.36630914180146,84.307310643947));
#29657=CARTESIAN_POINT('Ctrl Pts',(2.4560158360759,-6.307926414261,84.3154616261208));
#29658=CARTESIAN_POINT('Ctrl Pts',(2.61606447431989,-6.24326258603041,84.3236126082945));
#29659=CARTESIAN_POINT('Ctrl Pts',(2.77360937151675,-6.17246952639173,84.3317635904682));
#29660=CARTESIAN_POINT('Ctrl Pts',(2.93097126571379,-6.10175869945311,84.3399051045207));
#29661=CARTESIAN_POINT('Ctrl Pts',(3.085834877959,-6.02493296170729,84.3480466185731));
#29662=CARTESIAN_POINT('Ctrl Pts',(3.23768780522581,-5.94219375953798,84.3561881326256));
#29663=CARTESIAN_POINT('Ctrl Pts',(3.38939629666913,-5.85953325525758,84.3643219028281));
#29664=CARTESIAN_POINT('Ctrl Pts',(3.53809948528631,-5.7709706581231,84.3724556730306));
#29665=CARTESIAN_POINT('Ctrl Pts',(3.6833054159758,-5.67675525389666,84.3805894432331));
#29666=CARTESIAN_POINT('Ctrl Pts',(3.82840377296752,-5.58260964777952,84.3887171876505));
#29667=CARTESIAN_POINT('Ctrl Pts',(3.97000972541076,-5.48281977134684,84.3968449320678));
#29668=CARTESIAN_POINT('Ctrl Pts',(4.10765639577838,-5.37768053478644,84.4049726764852));
#29669=CARTESIAN_POINT('Ctrl Pts',(4.24523003179267,-5.27259708436407,84.4130961083786));
#29670=CARTESIAN_POINT('Ctrl Pts',(4.37884827947522,-5.16217014790846,84.4212195402721));
#29671=CARTESIAN_POINT('Ctrl Pts',(4.50807372315223,-5.04673759042655,84.4293429721656));
#29672=CARTESIAN_POINT('Ctrl Pts',(4.63811892223137,-4.93057277418906,84.4375179359167));
#29673=CARTESIAN_POINT('Ctrl Pts',(4.76371508083713,-4.80933881944455,84.4456928996679));
#29674=CARTESIAN_POINT('Ctrl Pts',(4.88445032991293,-4.68342118270538,84.4538678634191));
#29675=CARTESIAN_POINT('Ctrl Pts',(5.00439729499601,-4.55832566592044,84.4619894525915));
#29676=CARTESIAN_POINT('Ctrl Pts',(5.11954639866066,-4.42860773038687,84.4701110417639));
#29677=CARTESIAN_POINT('Ctrl Pts',(5.22953113968924,-4.29468195085743,84.4782326309363));
#29678=CARTESIAN_POINT('Ctrl Pts',(5.3395304009595,-4.16073849037818,84.486355292325));
#29679=CARTESIAN_POINT('Ctrl Pts',(5.44436370926848,-4.02258636226382,84.4944779537137));
#29680=CARTESIAN_POINT('Ctrl Pts',(5.54370529895975,-3.8806726940423,84.5026006151025));
#29681=CARTESIAN_POINT('Ctrl Pts',(5.64307892135534,-3.73871326574602,84.5107258956441));
#29682=CARTESIAN_POINT('Ctrl Pts',(5.73695708914281,-3.59299018173878,84.5188511761856));
#29683=CARTESIAN_POINT('Ctrl Pts',(5.82505778500283,-3.44397891999616,84.5269764567273));
#29684=CARTESIAN_POINT('Ctrl Pts',(5.91411831968266,-3.29334421144404,84.5351902605161));
#29685=CARTESIAN_POINT('Ctrl Pts',(5.99727456068421,-3.13934958800305,84.5434040643051));
#29686=CARTESIAN_POINT('Ctrl Pts',(6.07428365112252,-2.98251020546547,84.5516178680939));
#29687=CARTESIAN_POINT('Ctrl Pts',(6.1505946091245,-2.82709266364331,84.5597572089484));
#29688=CARTESIAN_POINT('Ctrl Pts',(6.22086932399302,-2.66888208901893,84.5678965498029));
#29689=CARTESIAN_POINT('Ctrl Pts',(6.28492075025478,-2.50839792756589,84.5760358906574));
#29690=CARTESIAN_POINT('Ctrl Pts',(6.34985114028735,-2.34571147692215,84.5842869259135));
#29691=CARTESIAN_POINT('Ctrl Pts',(6.40838607023891,-2.18068895703612,84.5925379611696));
#29692=CARTESIAN_POINT('Ctrl Pts',(6.46038363836647,-2.0138848639202,84.6007889964257));
#29693=CARTESIAN_POINT('Ctrl Pts',(6.51238120649402,-1.84708077080427,84.6090400316818));
#29694=CARTESIAN_POINT('Ctrl Pts',(6.55784137760392,-1.67849549255858,84.6172910669379));
#29695=CARTESIAN_POINT('Ctrl Pts',(6.59667642144928,-1.50869121780939,84.625542102194));
#29696=CARTESIAN_POINT('Ctrl Pts',(6.63542079932329,-1.33928337545691,84.6337738742267));
#29697=CARTESIAN_POINT('Ctrl Pts',(6.66769207561833,-1.16813340032523,84.6420056462593));
#29698=CARTESIAN_POINT('Ctrl Pts',(6.69333379840906,-0.995776914311138,
84.650237418292));
#29699=CARTESIAN_POINT('Ctrl Pts',(6.71894490242042,-0.823626239164798,
84.6584593607663));
#29700=CARTESIAN_POINT('Ctrl Pts',(6.73794216399962,-0.650272272811426,
84.6666813032406));
#29701=CARTESIAN_POINT('Ctrl Pts',(6.75021937948532,-0.476263927692286,
84.6749032457149));
#29702=CARTESIAN_POINT('Ctrl Pts',(6.76248439459687,-0.302428501824886,
84.6831170177067));
#29703=CARTESIAN_POINT('Ctrl Pts',(6.76804263775274,-0.127940347185809,
84.6913307896984));
#29704=CARTESIAN_POINT('Ctrl Pts',(6.76683924795597,0.0466432451993053,
84.6995445616902));
#29705=CARTESIAN_POINT('Ctrl Pts',(6.765636812995,0.221088313337655,84.7077518164225));
#29706=CARTESIAN_POINT('Ctrl Pts',(6.75768343356095,0.395628311704875,84.7159590711548));
#29707=CARTESIAN_POINT('Ctrl Pts',(6.74297619637966,0.569702567185123,84.724166325887));
#29708=CARTESIAN_POINT('Ctrl Pts',(6.72827768384473,0.743673558109239,84.7323687119009));
#29709=CARTESIAN_POINT('Ctrl Pts',(6.70683332513476,0.917179000461351,84.7405710979149));
#29710=CARTESIAN_POINT('Ctrl Pts',(6.67869226460581,1.08965987110408,84.7487734839288));
#29711=CARTESIAN_POINT('Ctrl Pts',(6.65055960350104,1.26208926038941,84.7569734217294));
#29712=CARTESIAN_POINT('Ctrl Pts',(6.61573427590793,1.43349433330917,84.76517335953));
#29713=CARTESIAN_POINT('Ctrl Pts',(6.57431712866856,1.60332257880166,84.7733732973307));
#29714=CARTESIAN_POINT('Ctrl Pts',(6.5329057726154,1.77312707792195,84.7815720885683));
#29715=CARTESIAN_POINT('Ctrl Pts',(6.48490451671685,1.94135484044307,84.7897708798059));
#29716=CARTESIAN_POINT('Ctrl Pts',(6.4304650454848,2.10746489859218,84.7979696710436));
#29717=CARTESIAN_POINT('Ctrl Pts',(6.37602331069314,2.27358186349499,84.8061688031819));
#29718=CARTESIAN_POINT('Ctrl Pts',(6.31514293880859,2.43758060795791,84.8143679353203));
#29719=CARTESIAN_POINT('Ctrl Pts',(6.24802509593879,2.59893659032287,84.8225670674586));
#29720=CARTESIAN_POINT('Ctrl Pts',(6.18089228687033,2.76032855247479,84.8307680278715));
#29721=CARTESIAN_POINT('Ctrl Pts',(6.10751937426341,2.91907624795365,84.8389689882843));
#29722=CARTESIAN_POINT('Ctrl Pts',(6.02815516936708,3.07467628442947,84.8471699486972));
#29723=CARTESIAN_POINT('Ctrl Pts',(5.94871658110543,3.23042215559701,84.8553785953841));
#29724=CARTESIAN_POINT('Ctrl Pts',(5.86327564463281,3.38301415390006,84.8635872420711));
#29725=CARTESIAN_POINT('Ctrl Pts',(5.77212699995609,3.53197379610579,84.871795888758));
#29726=CARTESIAN_POINT('Ctrl Pts',(5.68093483835623,3.68100455582867,84.8800084544835));
#29727=CARTESIAN_POINT('Ctrl Pts',(5.58402973400538,3.82639920367978,84.8882210202089));
#29728=CARTESIAN_POINT('Ctrl Pts',(5.48174891426729,3.96770939471749,84.8964335859344));
#29729=CARTESIAN_POINT('Ctrl Pts',(5.37932775048582,4.10921348372778,84.904657420485));
#29730=CARTESIAN_POINT('Ctrl Pts',(5.27151635082524,4.24662163302956,84.9128812550357));
#29731=CARTESIAN_POINT('Ctrl Pts',(5.15869216372487,4.37951871327475,84.9211050895863));
#29732=CARTESIAN_POINT('Ctrl Pts',(5.05502795934412,4.50162613050687,84.9286612465378));
#29733=CARTESIAN_POINT('Ctrl Pts',(4.94713247315765,4.61992548729601,84.9362174034893));
#29734=CARTESIAN_POINT('Ctrl Pts',(4.8353245216795,4.73412354824469,84.9437735604408));
#29735=CARTESIAN_POINT('Ctrl Pts',(4.70742503518454,4.86475713164338,84.9524172085999));
#29736=CARTESIAN_POINT('Ctrl Pts',(4.57411421330692,4.99032140237557,84.961060856759));
#29737=CARTESIAN_POINT('Ctrl Pts',(4.43581024301684,5.11036950600902,84.9697045049181));
#29738=CARTESIAN_POINT('Ctrl Pts',(4.29766488250379,5.2302799360608,84.9783382403676));
#29739=CARTESIAN_POINT('Ctrl Pts',(4.15453801777997,5.34468661122237,84.986971975817));
#29740=CARTESIAN_POINT('Ctrl Pts',(4.00688479438301,5.45317918690944,84.9956057112664));
#29741=CARTESIAN_POINT('Ctrl Pts',(3.85946199251083,5.56150245356185,85.0042259732647));
#29742=CARTESIAN_POINT('Ctrl Pts',(3.7075271693073,5.66392985430469,85.012846235263));
#29743=CARTESIAN_POINT('Ctrl Pts',(3.5515684951563,5.76009116457485,85.0214664972613));
#29744=CARTESIAN_POINT('Ctrl Pts',(3.4042165055845,5.8509457481065,85.0296110442896));
#29745=CARTESIAN_POINT('Ctrl Pts',(3.25327297297308,5.93620691929752,85.0377555913178));
#29746=CARTESIAN_POINT('Ctrl Pts',(3.09917575053258,6.01559628526639,85.045900138346));
#29747=CARTESIAN_POINT('Ctrl Pts',(3.09917575053248,6.01559628526645,83.0458432482751));
#29748=CARTESIAN_POINT('Ctrl Pts',(2.94443066306348,6.09531942489478,83.0540637081377));
#29749=CARTESIAN_POINT('Ctrl Pts',(2.78641930583546,6.16916464564878,83.0622841680003));
#29750=CARTESIAN_POINT('Ctrl Pts',(2.62562779814772,6.23685559120892,83.0705046278629));
#29751=CARTESIAN_POINT('Ctrl Pts',(2.46499034721999,6.30448168105682,83.0787172115794));
#29752=CARTESIAN_POINT('Ctrl Pts',(2.30157837857246,6.36596510034565,83.0869297952959));
#29753=CARTESIAN_POINT('Ctrl Pts',(2.13590237013809,6.4210754601732,83.0951423790124));
#29754=CARTESIAN_POINT('Ctrl Pts',(1.97035191792235,6.47614405506175,83.1033487388889));
#29755=CARTESIAN_POINT('Ctrl Pts',(1.80254118186197,6.52484909757285,83.1115550987655));
#29756=CARTESIAN_POINT('Ctrl Pts',(1.63300045841467,6.56700833734947,83.119761458642));
#29757=CARTESIAN_POINT('Ctrl Pts',(1.46355427379626,6.60914406840751,83.1279632425109));
#29758=CARTESIAN_POINT('Ctrl Pts',(1.29238037032785,6.6447411816277,83.1361650263798));
#29759=CARTESIAN_POINT('Ctrl Pts',(1.12002413070589,6.67366727868842,83.1443668102486));
#29760=CARTESIAN_POINT('Ctrl Pts',(0.94772949597837,6.70258303676078,83.1525656625727));
#29761=CARTESIAN_POINT('Ctrl Pts',(0.774253720049908,6.72483247038091,83.1607645148969));
#29762=CARTESIAN_POINT('Ctrl Pts',(0.600152393710189,6.74033427244702,83.168963367221));
#29763=CARTESIAN_POINT('Ctrl Pts',(0.426044884804798,6.75583662500239,83.1771625106971));
#29764=CARTESIAN_POINT('Ctrl Pts',(0.251312137196352,6.76459082661305,83.1853616541731));
#29765=CARTESIAN_POINT('Ctrl Pts',(0.0765152981278561,6.76656740224705,
83.1935607976492));
#29766=CARTESIAN_POINT('Ctrl Pts',(-0.0982951202571675,6.76854413143387,
83.2017605780863));
#29767=CARTESIAN_POINT('Ctrl Pts',(-0.273169281501512,6.7637421810302,83.2099603585233));
#29768=CARTESIAN_POINT('Ctrl Pts',(-0.447545774774762,6.75218422286309,
83.2181601389603));
#29769=CARTESIAN_POINT('Ctrl Pts',(-0.621967448440341,6.74062327006594,
83.2263620439343));
#29770=CARTESIAN_POINT('Ctrl Pts',(-0.795890839602391,6.72230284607982,
83.2345639489083));
#29771=CARTESIAN_POINT('Ctrl Pts',(-0.968759337792764,6.69729754045909,
83.2427658538822));
#29772=CARTESIAN_POINT('Ctrl Pts',(-1.14170398633059,6.67228121974463,83.2509713718795));
#29773=CARTESIAN_POINT('Ctrl Pts',(-1.31359246179592,6.64057420256431,83.2591768898768));
#29774=CARTESIAN_POINT('Ctrl Pts',(-1.48387796937551,6.60230226299902,83.2673824078741));
#29775=CARTESIAN_POINT('Ctrl Pts',(-1.65436318438348,6.56398543887052,83.2755975491383));
#29776=CARTESIAN_POINT('Ctrl Pts',(-1.8232413270061,6.51908839371184,83.2838126904025));
#29777=CARTESIAN_POINT('Ctrl Pts',(-1.98997945991885,6.46778716015772,83.2920278316668));
#29778=CARTESIAN_POINT('Ctrl Pts',(-2.15682885394968,6.41645169428671,83.3002484547352));
#29779=CARTESIAN_POINT('Ctrl Pts',(-2.32153505488385,6.35870364082029,83.3084690778037));
#29780=CARTESIAN_POINT('Ctrl Pts',(-2.48358487767961,6.29476728365403,83.3166897008721));
#29781=CARTESIAN_POINT('Ctrl Pts',(-2.64586607277502,6.23073963911865,83.3249220612226));
#29782=CARTESIAN_POINT('Ctrl Pts',(-2.80548298759804,6.16050618757545,83.333154421573));
#29783=CARTESIAN_POINT('Ctrl Pts',(-2.96194590614325,6.08433771655398,83.3413867819234));
#29784=CARTESIAN_POINT('Ctrl Pts',(-3.03308785002088,6.04970476236241,83.3451299443512));
#29785=CARTESIAN_POINT('Ctrl Pts',(-3.10357810974098,6.01384539589727,83.3488731067789));
#29786=CARTESIAN_POINT('Ctrl Pts',(-3.173372661103,5.97678801311909,83.3526162692066));
#29787=CARTESIAN_POINT('Ctrl Pts',(-3.32540914264454,5.89606431789096,83.3607701613693));
#29788=CARTESIAN_POINT('Ctrl Pts',(-3.4746125070392,5.80940338777875,83.368924053532));
#29789=CARTESIAN_POINT('Ctrl Pts',(-3.62048080640333,5.71702787560679,83.3770779456947));
#29790=CARTESIAN_POINT('Ctrl Pts',(-3.76617110568685,5.62476508736927,83.3852218878308));
#29791=CARTESIAN_POINT('Ctrl Pts',(-3.90853413530418,5.52680179125117,83.3933658299669));
#29792=CARTESIAN_POINT('Ctrl Pts',(-4.04709016103704,5.42340762145325,83.401509772103));
#29793=CARTESIAN_POINT('Ctrl Pts',(-4.18550627298595,5.32011785902022,83.4096454904916));
#29794=CARTESIAN_POINT('Ctrl Pts',(-4.32012274346839,5.21140835769521,83.4177812088803));
#29795=CARTESIAN_POINT('Ctrl Pts',(-4.45048659910675,5.09759335678821,83.4259169272689));
#29796=CARTESIAN_POINT('Ctrl Pts',(-4.5807462354779,4.98386934518137,83.4340461415648));
#29797=CARTESIAN_POINT('Ctrl Pts',(-4.70675975210336,4.86504820021443,83.4421753558607));
#29798=CARTESIAN_POINT('Ctrl Pts',(-4.82810522284315,4.74148594400054,83.4503045701566));
#29799=CARTESIAN_POINT('Ctrl Pts',(-4.94937919844588,4.61799648902423,83.4584289948276));
#29800=CARTESIAN_POINT('Ctrl Pts',(-5.06599034981524,4.48977174597194,83.4665534194986));
#29801=CARTESIAN_POINT('Ctrl Pts',(-5.17755177970986,4.35720628022398,83.4746778441695));
#29802=CARTESIAN_POINT('Ctrl Pts',(-5.28979045899961,4.22383605711877,83.4828515893064));
#29803=CARTESIAN_POINT('Ctrl Pts',(-5.39691762335385,4.08607248377964,83.4910253344432));
#29804=CARTESIAN_POINT('Ctrl Pts',(-5.49857838956078,3.94435352039536,83.4991990795801));
#29805=CARTESIAN_POINT('Ctrl Pts',(-5.59958814987847,3.80354208390882,83.5073204824376));
#29806=CARTESIAN_POINT('Ctrl Pts',(-5.69520112075932,3.65882608189352,83.5154418852951));
#29807=CARTESIAN_POINT('Ctrl Pts',(-5.78511111085763,3.51066638047987,83.5235632881526));
#29808=CARTESIAN_POINT('Ctrl Pts',(-5.87502805232226,3.36249522413938,83.5316853189141));
#29809=CARTESIAN_POINT('Ctrl Pts',(-5.95924094480983,3.21088015091966,83.5398073496757));
#29810=CARTESIAN_POINT('Ctrl Pts',(-6.03748837610024,3.05630873905999,83.5479293804373));
#29811=CARTESIAN_POINT('Ctrl Pts',(-6.11575675718707,2.90169594258798,83.5560535857736));
#29812=CARTESIAN_POINT('Ctrl Pts',(-6.18805633157849,2.74412555780631,83.5641777911099));
#29813=CARTESIAN_POINT('Ctrl Pts',(-6.2541728822409,2.58410730408832,83.5723019964463));
#29814=CARTESIAN_POINT('Ctrl Pts',(-6.32100509892106,2.42235696324146,83.5805141406969));
#29815=CARTESIAN_POINT('Ctrl Pts',(-6.38151950865884,2.25810580514608,83.5887262849475));
#29816=CARTESIAN_POINT('Ctrl Pts',(-6.43554611128877,2.0918975236555,83.5969384291981));
#29817=CARTESIAN_POINT('Ctrl Pts',(-6.48907951049594,1.92720654085356,83.6050756056096));
#29818=CARTESIAN_POINT('Ctrl Pts',(-6.53624302383644,1.76059438769159,83.6132127820211));
#29819=CARTESIAN_POINT('Ctrl Pts',(-6.57692251569119,1.59260140103992,83.6213499584327));
#29820=CARTESIAN_POINT('Ctrl Pts',(-6.61816417802968,1.42228683429307,83.6295995866028));
#29821=CARTESIAN_POINT('Ctrl Pts',(-6.65274121710189,1.25055337442426,83.6378492147729));
#29822=CARTESIAN_POINT('Ctrl Pts',(-6.6805889866268,1.07797021840157,83.6460988429431));
#29823=CARTESIAN_POINT('Ctrl Pts',(-6.70843675615168,0.905387062379014,
83.6543484711132));
#29824=CARTESIAN_POINT('Ctrl Pts',(-6.7295552724162,0.731954599804787,83.6625980992834));
#29825=CARTESIAN_POINT('Ctrl Pts',(-6.74393464102174,0.558242382506881,
83.6708477274535));
#29826=CARTESIAN_POINT('Ctrl Pts',(-6.7592338495307,0.373417895013728,83.6796250795723));
#29827=CARTESIAN_POINT('Ctrl Pts',(-6.76693482715002,0.187976924734993,
83.6884024316911));
#29828=CARTESIAN_POINT('Ctrl Pts',(-6.76699958812785,0.00236099078895365,
83.6971797838099));
#29829=CARTESIAN_POINT('',(-6.767,4.20685398138092E-12,83.3028202161898));
#29830=CARTESIAN_POINT('Ctrl Pts',(3.09917575053247,6.01559628526645,82.6513920151221));
#29831=CARTESIAN_POINT('Ctrl Pts',(2.93382384459258,6.10078395293762,82.6601414630345));
#29832=CARTESIAN_POINT('Ctrl Pts',(2.76495772122983,6.1791501026705,82.6688909109469));
#29833=CARTESIAN_POINT('Ctrl Pts',(2.59315093316715,6.25042856433176,82.6776403588593));
#29834=CARTESIAN_POINT('Ctrl Pts',(2.42134553245614,6.32170645041453,82.6863897361194));
#29835=CARTESIAN_POINT('Ctrl Pts',(2.2465997792758,6.38589665313461,82.6951391133794));
#29836=CARTESIAN_POINT('Ctrl Pts',(2.069507186899,6.44278115439081,82.7038884906394));
#29837=CARTESIAN_POINT('Ctrl Pts',(1.89241596572847,6.49966521519728,82.712637800154));
#29838=CARTESIAN_POINT('Ctrl Pts',(1.71297821457188,6.54924360009549,82.7213871096687));
#29839=CARTESIAN_POINT('Ctrl Pts',(1.53180337335839,6.59134792173557,82.7301364191834));
#29840=CARTESIAN_POINT('Ctrl Pts',(1.35062987477776,6.63345193135306,82.7388856638595));
#29841=CARTESIAN_POINT('Ctrl Pts',(1.16771959102944,6.66808192368239,82.7476349085356));
#29842=CARTESIAN_POINT('Ctrl Pts',(0.983693746906752,6.6951202836317,82.7563841532117));
#29843=CARTESIAN_POINT('Ctrl Pts',(0.79966920541976,6.72215845218868,82.7651333359559));
#29844=CARTESIAN_POINT('Ctrl Pts',(0.614529402873345,6.7416050542458,82.7738825187001));
#29845=CARTESIAN_POINT('Ctrl Pts',(0.428903127363098,6.75339404354123,82.7826317014442));
#29846=CARTESIAN_POINT('Ctrl Pts',(0.243278104163605,6.76518295330332,82.7913808251629));
#29847=CARTESIAN_POINT('Ctrl Pts',(0.0571669005387212,6.76931433552276,
82.8001299488815));
#29848=CARTESIAN_POINT('Ctrl Pts',(-0.128798404778032,6.76577415902472,
82.8088790726001));
#29849=CARTESIAN_POINT('Ctrl Pts',(-0.314762517259342,6.76223400523439,
82.8176281401993));
#29850=CARTESIAN_POINT('Ctrl Pts',(-0.500580446819479,6.75102239665088,
82.8263772077985));
#29851=CARTESIAN_POINT('Ctrl Pts',(-0.685621118842307,6.73217741012501,
82.8351262753977));
#29852=CARTESIAN_POINT('Ctrl Pts',(-0.870660665414156,6.71333253821776,
82.8438752897835));
#29853=CARTESIAN_POINT('Ctrl Pts',(-1.0549226788545,6.68685441030618,82.8526243041692));
#29854=CARTESIAN_POINT('Ctrl Pts',(-1.23778137635213,6.65283295028184,82.861373318555));
#29855=CARTESIAN_POINT('Ctrl Pts',(-1.42999922978807,6.61707018861874,82.8705701289224));
#29856=CARTESIAN_POINT('Ctrl Pts',(-1.62066601233655,6.57297172934423,82.8797669392898));
#29857=CARTESIAN_POINT('Ctrl Pts',(-1.80906628500344,6.52070304311305,82.8889637496572));
#29858=CARTESIAN_POINT('Ctrl Pts',(-1.98831342545476,6.47097374915046,82.8977137473949));
#29859=CARTESIAN_POINT('Ctrl Pts',(-2.16550875896641,6.41384933989549,82.9064637451327));
#29860=CARTESIAN_POINT('Ctrl Pts',(-2.3400503671394,6.34952386240502,82.9152137428704));
#29861=CARTESIAN_POINT('Ctrl Pts',(-2.51458843547019,6.28519968948624,82.9239635631513));
#29862=CARTESIAN_POINT('Ctrl Pts',(-2.68647261717986,6.21367483971129,82.9327133834322));
#29863=CARTESIAN_POINT('Ctrl Pts',(-2.85511905908664,6.13519226743875,82.941463203713));
#29864=CARTESIAN_POINT('Ctrl Pts',(-3.02376230488812,6.05671118252973,82.9502128581716));
#29865=CARTESIAN_POINT('Ctrl Pts',(-3.18916767379829,5.97127275992673,82.9589625126301));
#29866=CARTESIAN_POINT('Ctrl Pts',(-3.35077334102708,5.87916720438042,82.9677121670886));
#29867=CARTESIAN_POINT('Ctrl Pts',(-3.51237616037299,5.78706327195685,82.9764616673571));
#29868=CARTESIAN_POINT('Ctrl Pts',(-3.67017916302241,5.68829258362337,82.9852111676255));
#29869=CARTESIAN_POINT('Ctrl Pts',(-3.82364636566413,5.58319061741075,82.993960667894));
#29870=CARTESIAN_POINT('Ctrl Pts',(-3.97711106778746,5.47809036367739,83.0027100256024));
#29871=CARTESIAN_POINT('Ctrl Pts',(-4.12623987481873,5.36665920043266,83.0114593833109));
#29872=CARTESIAN_POINT('Ctrl Pts',(-4.27052628213873,5.2492755951238,83.0202087410193));
#29873=CARTESIAN_POINT('Ctrl Pts',(-4.41481053024921,5.13189374643086,83.0289579677958));
#29874=CARTESIAN_POINT('Ctrl Pts',(-4.55425230136471,5.00855981477407,83.0377071945723));
#29875=CARTESIAN_POINT('Ctrl Pts',(-4.68837800630488,4.87969268192134,83.0464564213488));
#29876=CARTESIAN_POINT('Ctrl Pts',(-4.82250188228852,4.75082730631854,83.0552055288197));
#29877=CARTESIAN_POINT('Ctrl Pts',(-4.9513096305294,4.61642907903555,83.0639546362905));
#29878=CARTESIAN_POINT('Ctrl Pts',(-5.07436379033356,4.47695444731702,83.0727037437614));
#29879=CARTESIAN_POINT('Ctrl Pts',(-5.19741643562803,4.3374815322059,83.0814527435511));
#29880=CARTESIAN_POINT('Ctrl Pts',(-5.31471544462778,4.19293255254584,83.0902017433409));
#29881=CARTESIAN_POINT('Ctrl Pts',(-5.42586245275639,4.04379841779588,83.0989507431306));
#29882=CARTESIAN_POINT('Ctrl Pts',(-5.5370216001915,3.89464799484345,83.1077006984728));
#29883=CARTESIAN_POINT('Ctrl Pts',(-5.64202723081236,3.74091164443871,83.1164506538149));
#29884=CARTESIAN_POINT('Ctrl Pts',(-5.74052265232941,3.58311159163274,83.1252006091571));
#29885=CARTESIAN_POINT('Ctrl Pts',(-5.83901427066893,3.42531763191825,83.1339502266395));
#29886=CARTESIAN_POINT('Ctrl Pts',(-5.93099603115716,3.26346052695655,83.142699844122));
#29887=CARTESIAN_POINT('Ctrl Pts',(-6.01615550622732,3.09809004467119,83.1514494616044));
#29888=CARTESIAN_POINT('Ctrl Pts',(-6.10131214578787,2.93272506863855,83.1601987877555));
#29889=CARTESIAN_POINT('Ctrl Pts',(-6.17964682328743,2.76384720416906,83.1689481139066));
#29890=CARTESIAN_POINT('Ctrl Pts',(-6.25089348288566,2.59203002791589,83.1776974400577));
#29891=CARTESIAN_POINT('Ctrl Pts',(-6.32213814889342,2.42021765937,83.1864465213893));
#29892=CARTESIAN_POINT('Ctrl Pts',(-6.38629508412605,2.24546640831863,83.1951956027209));
#29893=CARTESIAN_POINT('Ctrl Pts',(-6.44314639819838,2.06836976659961,83.2039446840525));
#29894=CARTESIAN_POINT('Ctrl Pts',(-6.50000285283727,1.89125711158184,83.2126945564869));
#29895=CARTESIAN_POINT('Ctrl Pts',(-6.54955227673276,1.71179891440153,83.2214444289213));
#29896=CARTESIAN_POINT('Ctrl Pts',(-6.59162635926411,1.53060476278319,83.2301943013557));
#29897=CARTESIAN_POINT('Ctrl Pts',(-6.63369752055217,1.34942319164592,83.2389435662782));
#29898=CARTESIAN_POINT('Ctrl Pts',(-6.6682943142427,1.1665061864261,83.2476928312007));
#29899=CARTESIAN_POINT('Ctrl Pts',(-6.6952992374543,0.982474997617712,83.2564420961232));
#29900=CARTESIAN_POINT('Ctrl Pts',(-6.72230554731453,0.798434359176906,
83.2651918103029));
#29901=CARTESIAN_POINT('Ctrl Pts',(-6.7417191649671,0.613279706239515,83.2739415244826));
#29902=CARTESIAN_POINT('Ctrl Pts',(-6.7534741481728,0.427639953654568,83.2826912386623));
#29903=CARTESIAN_POINT('Ctrl Pts',(-6.76248837758741,0.28528336419891,83.2894008978381));
#29904=CARTESIAN_POINT('Ctrl Pts',(-6.76699999999991,0.142641701106605,
83.296110557014));
#29905=CARTESIAN_POINT('Ctrl Pts',(-6.767,4.20685394936554E-12,83.3028202161898));
#29906=CARTESIAN_POINT('Ctrl Pts',(-6.7669999999934,9.4528375515739E-6,
83.3030260662099));
#29907=CARTESIAN_POINT('Ctrl Pts',(-6.76700024064021,-0.172262306021359,
83.3111539611311));
#29908=CARTESIAN_POINT('Ctrl Pts',(-6.76041772040418,-0.344752167752305,
83.3192818560524));
#29909=CARTESIAN_POINT('Ctrl Pts',(-6.74722842698908,-0.516911553392345,
83.3274097509736));
#29910=CARTESIAN_POINT('Ctrl Pts',(-6.73405087020116,-0.688917741248305,
83.3355304132047));
#29911=CARTESIAN_POINT('Ctrl Pts',(-6.71427827240309,-0.86059367454886,
83.3436510754358));
#29912=CARTESIAN_POINT('Ctrl Pts',(-6.68793865670865,-1.03139009307926,
83.3517717376669));
#29913=CARTESIAN_POINT('Ctrl Pts',(-6.66161689176405,-1.20207076033316,
83.3598868964042));
#29914=CARTESIAN_POINT('Ctrl Pts',(-6.62873702647889,-1.3718727380254,83.3680020551416));
#29915=CARTESIAN_POINT('Ctrl Pts',(-6.58937896398752,-1.54025123566215,
83.3761172138789));
#29916=CARTESIAN_POINT('Ctrl Pts',(-6.55003922871389,-1.70855132726992,
83.3842285937646));
#29917=CARTESIAN_POINT('Ctrl Pts',(-6.50422738748251,-1.87542890197709,
83.3923399736502));
#29918=CARTESIAN_POINT('Ctrl Pts',(-6.45207454880868,-2.04034874877197,
83.4004513535359));
#29919=CARTESIAN_POINT('Ctrl Pts',(-6.39992661755151,-2.20525307713245,
83.4085619701664));
#29920=CARTESIAN_POINT('Ctrl Pts',(-6.34143897963039,-2.3681996918337,83.416672586797));
#29921=CARTESIAN_POINT('Ctrl Pts',(-6.27679285263599,-2.52866772927915,
83.4247832034275));
#29922=CARTESIAN_POINT('Ctrl Pts',(-6.2121466358495,-2.68913598961127,83.4328938313236));
#29923=CARTESIAN_POINT('Ctrl Pts',(-6.14134204957303,-2.84712532466732,
83.4410044592196));
#29924=CARTESIAN_POINT('Ctrl Pts',(-6.06460870400489,-3.00213428535569,
83.4491150871156));
#29925=CARTESIAN_POINT('Ctrl Pts',(-5.98786051374254,-3.15717323379719,
83.457227284079));
#29926=CARTESIAN_POINT('Ctrl Pts',(-5.90518144343929,-3.30923033050929,
83.4653394810424));
#29927=CARTESIAN_POINT('Ctrl Pts',(-5.8168473212674,-3.45782825499826,83.4734516780058));
#29928=CARTESIAN_POINT('Ctrl Pts',(-5.72847914218544,-3.60648347089429,
83.4815670025983));
#29929=CARTESIAN_POINT('Ctrl Pts',(-5.63445175782866,-3.751676543635,83.4896823271907));
#29930=CARTESIAN_POINT('Ctrl Pts',(-5.53508456923408,-3.89295874771706,
83.4977976517831));
#29931=CARTESIAN_POINT('Ctrl Pts',(-5.43560601373181,-4.03439929543753,
83.5059220717179));
#29932=CARTESIAN_POINT('Ctrl Pts',(-5.33077591489073,-4.17191992138808,
83.5140464916528));
#29933=CARTESIAN_POINT('Ctrl Pts',(-5.22095475603217,-4.30510399821713,
83.5221709115876));
#29934=CARTESIAN_POINT('Ctrl Pts',(-5.11106353898663,-4.43837303713411,
83.5303005143318));
#29935=CARTESIAN_POINT('Ctrl Pts',(-4.99617516256445,-4.56729974242824,
83.538430117076));
#29936=CARTESIAN_POINT('Ctrl Pts',(-4.87668701817062,-4.69150431384286,
83.5465597198202));
#29937=CARTESIAN_POINT('Ctrl Pts',(-4.75703022003002,-4.81588419609222,
83.5547007972422));
#29938=CARTESIAN_POINT('Ctrl Pts',(-4.63276095352074,-4.93552838194434,
83.5628418746643));
#29939=CARTESIAN_POINT('Ctrl Pts',(-4.5043103695593,-5.05009674112096,83.5709829520863));
#29940=CARTESIAN_POINT('Ctrl Pts',(-4.44518089304723,-5.10283583263801,
83.5747305227969));
#29941=CARTESIAN_POINT('Ctrl Pts',(-4.38516580405952,-5.15449993889306,
83.5784780935075));
#29942=CARTESIAN_POINT('Ctrl Pts',(-4.32430916763142,-5.20505900281052,
83.582225664218));
#29943=CARTESIAN_POINT('Ctrl Pts',(-4.19187303624,-5.31508557057706,83.5903811226225));
#29944=CARTESIAN_POINT('Ctrl Pts',(-4.05501891968798,-5.42023379748667,
83.5985365810269));
#29945=CARTESIAN_POINT('Ctrl Pts',(-3.9141437135064,-5.52012391074859,83.6066920394314));
#29946=CARTESIAN_POINT('Ctrl Pts',(-3.7734399709696,-5.61989244461155,83.6148375715708));
#29947=CARTESIAN_POINT('Ctrl Pts',(-3.62872517580127,-5.71441539486231,
83.6229831037104));
#29948=CARTESIAN_POINT('Ctrl Pts',(-3.48043123136945,-5.80335139757263,
83.6311286358498));
#29949=CARTESIAN_POINT('Ctrl Pts',(-3.33228659692088,-5.8921978549335,83.6392659666479));
#29950=CARTESIAN_POINT('Ctrl Pts',(-3.18057029859005,-5.97546837700233,
83.647403297446));
#29951=CARTESIAN_POINT('Ctrl Pts',(-3.02574532241725,-6.0528633095313,83.6555406282441));
#29952=CARTESIAN_POINT('Ctrl Pts',(-2.87104369505901,-6.13019658163946,
83.6636714760435));
#29953=CARTESIAN_POINT('Ctrl Pts',(-2.71323864664276,-6.20166342213866,
83.6718023238429));
#29954=CARTESIAN_POINT('Ctrl Pts',(-2.55282000760788,-6.26700877682144,
83.6799331716424));
#29955=CARTESIAN_POINT('Ctrl Pts',(-2.39249547513759,-6.33231579788614,
83.6880592496336));
#29956=CARTESIAN_POINT('Ctrl Pts',(-2.22956074306105,-6.39150834710923,
83.6961853276247));
#29957=CARTESIAN_POINT('Ctrl Pts',(-2.06452797813734,-6.44437842056844,
83.7043114056159));
#29958=CARTESIAN_POINT('Ctrl Pts',(-1.89891003708618,-6.49743596167905,
83.7124662971996));
#29959=CARTESIAN_POINT('Ctrl Pts',(-1.73117949273514,-6.54412594728098,
83.7206211887834));
#29960=CARTESIAN_POINT('Ctrl Pts',(-1.56187240709269,-6.58428762919441,
83.7287760803671));
#29961=CARTESIAN_POINT('Ctrl Pts',(-1.39322555997764,-6.62429269456917,
83.7368991707206));
#29962=CARTESIAN_POINT('Ctrl Pts',(-1.22301480775866,-6.65782021271982,
83.7450222610741));
#29963=CARTESIAN_POINT('Ctrl Pts',(-1.05178294598792,-6.68476189811791,
83.7531453514276));
#29964=CARTESIAN_POINT('Ctrl Pts',(-0.880537638310403,-6.71170569910002,
83.7612690796432));
#29965=CARTESIAN_POINT('Ctrl Pts',(-0.708271422746935,-6.73206258032306,
83.7693928078588));
#29966=CARTESIAN_POINT('Ctrl Pts',(-0.53553480070528,-6.74577582470938,
83.7775165360745));
#29967=CARTESIAN_POINT('Ctrl Pts',(-0.362751751659414,-6.75949275485063,
83.7856424477319));
#29968=CARTESIAN_POINT('Ctrl Pts',(-0.189498408909942,-6.76656246368741,
83.7937683593893));
#29969=CARTESIAN_POINT('Ctrl Pts',(-0.016327835848695,-6.76698030156557,
83.8018942710468));
#29970=CARTESIAN_POINT('Ctrl Pts',(0.157950181193301,-6.7674008115608,83.8100721487617));
#29971=CARTESIAN_POINT('Ctrl Pts',(0.332143990632475,-6.76108407555866,
83.8182500264766));
#29972=CARTESIAN_POINT('Ctrl Pts',(0.505693297731611,-6.74807848862395,
83.8264279041915));
#29973=CARTESIAN_POINT('Ctrl Pts',(0.678414291462611,-6.73513497454738,
83.8345667506619));
#29974=CARTESIAN_POINT('Ctrl Pts',(0.850496564956195,-6.71556642097293,
83.8427055971324));
#29975=CARTESIAN_POINT('Ctrl Pts',(1.02139668540423,-6.68947216236418,83.8508444436028));
#29976=CARTESIAN_POINT('Ctrl Pts',(1.19352617743568,-6.66319019446686,83.8590418369399));
#29977=CARTESIAN_POINT('Ctrl Pts',(1.36445607369074,-6.63028835353182,83.8672392302771));
#29978=CARTESIAN_POINT('Ctrl Pts',(1.53364567701199,-6.59091950621326,83.8754366236142));
#29979=CARTESIAN_POINT('Ctrl Pts',(1.70283528033337,-6.55155065889467,83.8836340169514));
#29980=CARTESIAN_POINT('Ctrl Pts',(1.87028424783008,-6.5057149624111,83.8918314102885));
#29981=CARTESIAN_POINT('Ctrl Pts',(2.03547175042119,-6.45361478190613,83.9000288036257));
#29982=CARTESIAN_POINT('Ctrl Pts',(2.20123993080568,-6.40133145547683,83.9082550129701));
#29983=CARTESIAN_POINT('Ctrl Pts',(2.36522410994082,-6.34258403290148,83.9164812223145));
#29984=CARTESIAN_POINT('Ctrl Pts',(2.52688374619929,-6.2775112531316,83.9247074316589));
#29985=CARTESIAN_POINT('Ctrl Pts',(2.68836176478388,-6.21251157984128,83.9329243992096));
#29986=CARTESIAN_POINT('Ctrl Pts',(2.84752011107338,-6.14120083256944,83.9411413667603));
#29987=CARTESIAN_POINT('Ctrl Pts',(3.00383250907188,-6.06376774435194,83.9493583343111));
#29988=CARTESIAN_POINT('Ctrl Pts',(3.16000066993979,-5.98640610744987,83.9575677196621));
#29989=CARTESIAN_POINT('Ctrl Pts',(3.31332779313841,-5.90293353875851,83.9657771050131));
#29990=CARTESIAN_POINT('Ctrl Pts',(3.46330665181681,-5.81358719169855,83.9739864903641));
#29991=CARTESIAN_POINT('Ctrl Pts',(3.61317720992924,-5.72430536213152,83.9821899476724));
#29992=CARTESIAN_POINT('Ctrl Pts',(3.75970401250557,-5.62915838531564,83.9903934049807));
#29993=CARTESIAN_POINT('Ctrl Pts',(3.90240348740468,-5.52842979710259,83.9985968622889));
#29994=CARTESIAN_POINT('Ctrl Pts',(4.04502854338574,-5.42775373965433,84.0067960414286));
#29995=CARTESIAN_POINT('Ctrl Pts',(4.1838299557433,-5.32150207607723,84.0149952205683));
#29996=CARTESIAN_POINT('Ctrl Pts',(4.31835218954205,-5.21000224252134,84.0231943997079));
#29997=CARTESIAN_POINT('Ctrl Pts',(4.45284907645434,-5.09852341793581,84.0313920339456));
#29998=CARTESIAN_POINT('Ctrl Pts',(4.58306811105026,-4.98179861693386,84.0395896681833));
#29999=CARTESIAN_POINT('Ctrl Pts',(4.70858574603637,-4.8601964232141,84.047787302421));
#30000=CARTESIAN_POINT('Ctrl Pts',(4.83409432102289,-4.73860300687311,84.0559843449446));
#30001=CARTESIAN_POINT('Ctrl Pts',(4.95490191401302,-4.61213314789168,84.0641813874681));
#30002=CARTESIAN_POINT('Ctrl Pts',(5.07062090631274,-4.48119321436425,84.0723784299916));
#30003=CARTESIAN_POINT('Ctrl Pts',(5.18635257762259,-4.35023893411024,84.0805763706424));
#30004=CARTESIAN_POINT('Ctrl Pts',(5.29699429988119,-4.21481387235973,84.0887743112933));
#30005=CARTESIAN_POINT('Ctrl Pts',(5.40219788516575,-4.07535851300357,84.0969722519441));
#30006=CARTESIAN_POINT('Ctrl Pts',(5.50743211796276,-3.93586252803708,84.1051725807881));
#30007=CARTESIAN_POINT('Ctrl Pts',(5.60722484225888,-3.79233419308536,84.1133729096322));
#30008=CARTESIAN_POINT('Ctrl Pts',(5.70127041924144,-3.64524410796898,84.1215732384762));
#30009=CARTESIAN_POINT('Ctrl Pts',(5.79541399415545,-3.49800075116729,84.1297821122757));
#30010=CARTESIAN_POINT('Ctrl Pts',(5.88379826381659,-3.34718853190313,84.1379909860751));
#30011=CARTESIAN_POINT('Ctrl Pts',(5.96616241037227,-3.19330472912638,84.1461998598746));
#30012=CARTESIAN_POINT('Ctrl Pts',(6.04857076085715,-3.03933833860964,84.1544131392861));
#30013=CARTESIAN_POINT('Ctrl Pts',(6.124952390527,-2.88229740050623,84.1626264186976));
#30014=CARTESIAN_POINT('Ctrl Pts',(6.19509417591534,-2.72270034185545,84.1708396981091));
#30015=CARTESIAN_POINT('Ctrl Pts',(6.26533855468863,-2.56286984742335,84.1790649907326));
#30016=CARTESIAN_POINT('Ctrl Pts',(6.3293247184793,-2.40047609452752,84.1872902833561));
#30017=CARTESIAN_POINT('Ctrl Pts',(6.38688864992689,-2.23605509177101,84.1955155759796));
#30018=CARTESIAN_POINT('Ctrl Pts',(6.43894831037641,-2.08735604778603,84.2029543649975));
#30019=CARTESIAN_POINT('Ctrl Pts',(6.4857558052422,-1.93699928768334,84.2103931540153));
#30020=CARTESIAN_POINT('Ctrl Pts',(6.52722583053317,-1.78538846115365,84.2178319430332));
#30021=CARTESIAN_POINT('Ctrl Pts',(6.5730855482026,-1.61772929886722,84.2260581440487));
#30022=CARTESIAN_POINT('Ctrl Pts',(6.61254544186901,-1.44806772476172,84.2342843450642));
#30023=CARTESIAN_POINT('Ctrl Pts',(6.64542929212861,-1.27693324935919,84.2425105460797));
#30024=CARTESIAN_POINT('Ctrl Pts',(6.67827620431295,-1.10599100747197,84.250727506692));
#30025=CARTESIAN_POINT('Ctrl Pts',(6.70456171515487,-0.933579507830849,
84.2589444673044));
#30026=CARTESIAN_POINT('Ctrl Pts',(6.72415935584308,-0.760243353951828,
84.2671614279168));
#30027=CARTESIAN_POINT('Ctrl Pts',(6.74373891611447,-0.587067116767038,
84.275370807715));
#30028=CARTESIAN_POINT('Ctrl Pts',(6.75664285418664,-0.412968278389496,
84.2835801875132));
#30029=CARTESIAN_POINT('Ctrl Pts',(6.76279572049965,-0.238501662031088,
84.2917895673114));
#30030=CARTESIAN_POINT('Ctrl Pts',(6.76894414482621,-0.0641609997087456,
84.2999930204484));
#30031=CARTESIAN_POINT('Ctrl Pts',(6.76835119268485,0.11054655477672,84.3081964735854));
#30032=CARTESIAN_POINT('Ctrl Pts',(6.76099321579686,0.285060933747276,84.3163999267224));
#30033=CARTESIAN_POINT('Ctrl Pts',(6.7536390749184,0.459484331347476,84.3245991030691));
#30034=CARTESIAN_POINT('Ctrl Pts',(6.73952695053793,0.633714396599412,84.3327982794158));
#30035=CARTESIAN_POINT('Ctrl Pts',(6.71868528349019,0.807190845718842,84.3409974557625));
#30036=CARTESIAN_POINT('Ctrl Pts',(6.69784753811664,0.980634652626396,84.3491950893104));
#30037=CARTESIAN_POINT('Ctrl Pts',(6.67028280889954,1.15332476940956,84.3573927228583));
#30038=CARTESIAN_POINT('Ctrl Pts',(6.63607145211147,1.32470550782849,84.3655903564062));
#30039=CARTESIAN_POINT('Ctrl Pts',(6.60186255938082,1.49607390262771,84.3737873995233));
#30040=CARTESIAN_POINT('Ctrl Pts',(6.5610080618249,1.66613275496902,84.3819844426404));
#30041=CARTESIAN_POINT('Ctrl Pts',(6.5136395392399,1.83433610683828,84.3901814857575));
#30042=CARTESIAN_POINT('Ctrl Pts',(6.46626581920114,2.00255791461657,84.3983794282853));
#30043=CARTESIAN_POINT('Ctrl Pts',(6.41237674740521,2.16892347098477,84.406577370813));
#30044=CARTESIAN_POINT('Ctrl Pts',(6.35215394081282,2.3329014793206,84.4147753133407));
#30045=CARTESIAN_POINT('Ctrl Pts',(6.29191358091049,2.4969272827853,84.4229756453457));
#30046=CARTESIAN_POINT('Ctrl Pts',(6.22533593260335,2.65856381545149,84.4311759773506));
#30047=CARTESIAN_POINT('Ctrl Pts',(6.15265097727443,2.81729923008614,84.4393763093556));
#30048=CARTESIAN_POINT('Ctrl Pts',(6.07989026457699,2.97620008992537,84.4475851883229));
#30049=CARTESIAN_POINT('Ctrl Pts',(6.00100967714827,3.13219346419249,84.4557940672902));
#30050=CARTESIAN_POINT('Ctrl Pts',(5.91628590282751,3.28479072636363,84.4640029462574));
#30051=CARTESIAN_POINT('Ctrl Pts',(5.83151664681926,3.43746990628509,84.4722162319414));
#30052=CARTESIAN_POINT('Ctrl Pts',(5.74089813662695,3.58674903336307,84.4804295176253));
#30053=CARTESIAN_POINT('Ctrl Pts',(5.6447506740265,3.73216811358724,84.4886428033093));
#30054=CARTESIAN_POINT('Ctrl Pts',(5.54846255953812,3.87779992400336,84.4968681040179));
#30055=CARTESIAN_POINT('Ctrl Pts',(5.44662953819703,4.01956011156837,84.5050934047265));
#30056=CARTESIAN_POINT('Ctrl Pts',(5.3396132927531,4.15702043341796,84.5133187054352));
#30057=CARTESIAN_POINT('Ctrl Pts',(5.2428300073079,4.28133671373381,84.5207574977704));
#30058=CARTESIAN_POINT('Ctrl Pts',(5.1418079929839,4.40213642242927,84.5281962901057));
#30059=CARTESIAN_POINT('Ctrl Pts',(5.03684032101293,4.51912918388249,84.5356350824409));
#30060=CARTESIAN_POINT('Ctrl Pts',(4.92177755845788,4.64737352882208,84.5437892882083));
#30061=CARTESIAN_POINT('Ctrl Pts',(4.80163369204816,4.77142116902336,84.5519434939756));
#30062=CARTESIAN_POINT('Ctrl Pts',(4.67674849922026,4.89083964928733,84.5600976997429));
#30063=CARTESIAN_POINT('Ctrl Pts',(4.55204628327325,5.01008316228302,84.5682399582881));
#30064=CARTESIAN_POINT('Ctrl Pts',(4.42261684266922,5.12471077770117,84.5763822168333));
#30065=CARTESIAN_POINT('Ctrl Pts',(4.28883968130011,5.23432356547678,84.5845244753785));
#30066=CARTESIAN_POINT('Ctrl Pts',(4.1551752339486,5.34384399894047,84.5926598736595));
#30067=CARTESIAN_POINT('Ctrl Pts',(4.01717063548316,5.44835778210296,84.6007952719405));
#30068=CARTESIAN_POINT('Ctrl Pts',(3.87524213227022,5.5475028090374,84.6089306702215));
#30069=CARTESIAN_POINT('Ctrl Pts',(3.73342452133133,5.64657037149324,84.6170597121132));
#30070=CARTESIAN_POINT('Ctrl Pts',(3.58768941014001,5.74027732374158,84.6251887540049));
#30071=CARTESIAN_POINT('Ctrl Pts',(3.43848581699641,5.82830200712991,84.6333177958966));
#30072=CARTESIAN_POINT('Ctrl Pts',(3.32724415243864,5.89393053588032,84.639378562479));
#30073=CARTESIAN_POINT('Ctrl Pts',(3.21407517135522,5.95640123927637,84.6454393290614));
#30074=CARTESIAN_POINT('Ctrl Pts',(3.0991757505325,6.01559628526643,84.6515000956437));
#30075=CARTESIAN_POINT('Origin',(0.,0.,-3.69717978381041));
#30076=CARTESIAN_POINT('',(3.09917575053243,6.01559628526647,87.0457515827423));
#30077=CARTESIAN_POINT('',(3.09917575053262,6.01559628526637,86.651392015122));
#30078=CARTESIAN_POINT('',(3.09917575053259,6.01559628526639,-3.69717978381041));
#30079=CARTESIAN_POINT('',(-6.76699862563876,0.0030496394260042,85.6971797838099));
#30080=CARTESIAN_POINT('Ctrl Pts',(-6.767,4.52674774247449E-12,85.6971797838099));
#30081=CARTESIAN_POINT('Ctrl Pts',(-6.76700000000013,-0.186007249411268,
85.7059292956159));
#30082=CARTESIAN_POINT('Ctrl Pts',(-6.75932637295462,-0.372014355523239,
85.7146788074218));
#30083=CARTESIAN_POINT('Ctrl Pts',(-6.74400518266962,-0.557389537150879,
85.7234283192278));
#30084=CARTESIAN_POINT('Ctrl Pts',(-6.72868405709692,-0.742763935807108,
85.7321777940783));
#30085=CARTESIAN_POINT('Ctrl Pts',(-6.70571545653052,-0.927506129690636,
85.7409272689289));
#30086=CARTESIAN_POINT('Ctrl Pts',(-6.67517739415725,-1.11098863924525,
85.7496767437794));
#30087=CARTESIAN_POINT('Ctrl Pts',(-6.64463945823152,-1.2944703890624,85.7584261824014));
#30088=CARTESIAN_POINT('Ctrl Pts',(-6.60653217027211,-1.47669218227978,
85.7671756210234));
#30089=CARTESIAN_POINT('Ctrl Pts',(-6.56098496116766,-1.65703510503907,
85.7759250596454));
#30090=CARTESIAN_POINT('Ctrl Pts',(-6.51543793687577,-1.83737729603809,
85.7846744627656));
#30091=CARTESIAN_POINT('Ctrl Pts',(-6.46245112202704,-2.01584035396844,
85.7934238658858));
#30092=CARTESIAN_POINT('Ctrl Pts',(-6.40220448416313,-2.19181813637937,
85.8021732690061));
#30093=CARTESIAN_POINT('Ctrl Pts',(-6.34195808575257,-2.36779521935759,
85.8109226373514));
#30094=CARTESIAN_POINT('Ctrl Pts',(-6.27445201489302,-2.54128677544663,
85.8196720056966));
#30095=CARTESIAN_POINT('Ctrl Pts',(-6.19991555136247,-2.71170355237696,
85.8284213740419));
#30096=CARTESIAN_POINT('Ctrl Pts',(-6.12537937789111,-2.88211966612917,
85.837170708339));
#30097=CARTESIAN_POINT('Ctrl Pts',(-6.043812981337,-3.0494607621028,85.845920042636));
#30098=CARTESIAN_POINT('Ctrl Pts',(-5.95549339426401,-3.2131584820668,85.8546693769331));
#30099=CARTESIAN_POINT('Ctrl Pts',(-5.8671741435526,-3.37685557859464,85.8634186779086));
#30100=CARTESIAN_POINT('Ctrl Pts',(-5.77210188986342,-3.53690907467143,
85.8721679788842));
#30101=CARTESIAN_POINT('Ctrl Pts',(-5.67059953467176,-3.6927753678474,85.8809172798598));
#30102=CARTESIAN_POINT('Ctrl Pts',(-5.56909755761879,-3.84864108035629,
85.8896665482405));
#30103=CARTESIAN_POINT('Ctrl Pts',(-5.46116568338188,-4.00031938104117,
85.8984158166213));
#30104=CARTESIAN_POINT('Ctrl Pts',(-5.34717048686239,-4.14729511663058,
85.907165085002));
#30105=CARTESIAN_POINT('Ctrl Pts',(-5.23317570555648,-4.29427031687881,
85.9159143215146));
#30106=CARTESIAN_POINT('Ctrl Pts',(-5.11311782178942,-4.43654275986971,
85.9246635580273));
#30107=CARTESIAN_POINT('Ctrl Pts',(-4.98740459172158,-4.57362924147493,
85.9334127945399));
#30108=CARTESIAN_POINT('Ctrl Pts',(-4.86169180910993,-4.71071523514267,
85.942161999911));
#30109=CARTESIAN_POINT('Ctrl Pts',(-4.73032391415615,-4.84261509316343,
85.9509112052821));
#30110=CARTESIAN_POINT('Ctrl Pts',(-4.59374707237499,-4.96888084331333,
85.9596604106532));
#30111=CARTESIAN_POINT('Ctrl Pts',(-4.45717070537613,-5.0951461545254,85.9684095856095));
#30112=CARTESIAN_POINT('Ctrl Pts',(-4.31538563819724,-5.21577720253455,
85.9771587605657));
#30113=CARTESIAN_POINT('Ctrl Pts',(-4.16887341290867,-5.33036429028479,
85.9859079355219));
#30114=CARTESIAN_POINT('Ctrl Pts',(-4.02236168477565,-5.44495098921009,
85.9946570807898));
#30115=CARTESIAN_POINT('Ctrl Pts',(-3.87112305634672,-5.55349359238596,
86.0034062260577));
#30116=CARTESIAN_POINT('Ctrl Pts',(-3.71567117316973,-5.65562346102315,
86.0121553713256));
#30117=CARTESIAN_POINT('Ctrl Pts',(-3.5602198045754,-5.75775299158621,86.0209044876318));
#30118=CARTESIAN_POINT('Ctrl Pts',(-3.40055544862626,-5.85346967275215,
86.029653603938));
#30119=CARTESIAN_POINT('Ctrl Pts',(-3.2372203632364,-5.94244842803432,86.0384027202441));
#30120=CARTESIAN_POINT('Ctrl Pts',(-3.0738858049628,-6.03142689616357,86.0471518083151));
#30121=CARTESIAN_POINT('Ctrl Pts',(-2.90688079257937,-6.11366734484714,
86.055900896386));
#30122=CARTESIAN_POINT('Ctrl Pts',(-2.7367725109484,-6.18889046787202,86.064649984457));
#30123=CARTESIAN_POINT('Ctrl Pts',(-2.56666476416872,-6.26411335438177,
86.0733990450192));
#30124=CARTESIAN_POINT('Ctrl Pts',(-2.39345402972321,-6.33231884350204,
86.0821481055815));
#30125=CARTESIAN_POINT('Ctrl Pts',(-2.21772856474267,-6.39327529620964,
86.0908971661437));
#30126=CARTESIAN_POINT('Ctrl Pts',(-2.04200363768498,-6.4542315623201,86.0996461999237));
#30127=CARTESIAN_POINT('Ctrl Pts',(-1.8637642662032,-6.50793874251991,86.1083952337037));
#30128=CARTESIAN_POINT('Ctrl Pts',(-1.68361578194914,-6.55421443796065,
86.1171442674837));
#30129=CARTESIAN_POINT('Ctrl Pts',(-1.50346783420095,-6.60048999558628,
86.1258932752079));
#30130=CARTESIAN_POINT('Ctrl Pts',(-1.32141106257476,-6.6393340414545,86.1346422829321));
#30131=CARTESIAN_POINT('Ctrl Pts',(-1.13806375959275,-6.67061465526991,
86.1433912906564));
#30132=CARTESIAN_POINT('Ctrl Pts',(-0.954716987421285,-6.70189517852451,
86.1521402730513));
#30133=CARTESIAN_POINT('Ctrl Pts',(-0.770079973811828,-6.72561226535806,
86.1608892554462));
#30134=CARTESIAN_POINT('Ctrl Pts',(-0.584779770554227,-6.74168536939767,
86.1696382378411));
#30135=CARTESIAN_POINT('Ctrl Pts',(-0.391490647555678,-6.75845143942384,
86.1787644185171));
#30136=CARTESIAN_POINT('Ctrl Pts',(-0.197480213106098,-6.76689975924021,
86.1878905991932));
#30137=CARTESIAN_POINT('Ctrl Pts',(-0.00346532629955176,-6.76699911271707,
86.1970167798692));
#30138=CARTESIAN_POINT('Ctrl Pts',(0.184486595294258,-6.76709536139778,
86.2058577673991));
#30139=CARTESIAN_POINT('Ctrl Pts',(0.372442378183392,-6.7593565972678,86.2146987549291));
#30140=CARTESIAN_POINT('Ctrl Pts',(0.559750217720212,-6.74380965729032,
86.223539742459));
#30141=CARTESIAN_POINT('Ctrl Pts',(0.74512991445588,-6.72842275717274,86.2322897210568));
#30142=CARTESIAN_POINT('Ctrl Pts',(0.929874656312314,-6.70538772273499,
86.2410396996545));
#30143=CARTESIAN_POINT('Ctrl Pts',(1.11335688289591,-6.67478280180774,86.2497896782523));
#30144=CARTESIAN_POINT('Ctrl Pts',(1.2968372311867,-6.6441781941806,86.2585395672772));
#30145=CARTESIAN_POINT('Ctrl Pts',(1.47905480730049,-6.60600390230117,86.2672894563022));
#30146=CARTESIAN_POINT('Ctrl Pts',(1.65939064804622,-6.56038959797181,86.2760393453271));
#30147=CARTESIAN_POINT('Ctrl Pts',(1.83972470264086,-6.51477574543307,86.2847891476881));
#30148=CARTESIAN_POINT('Ctrl Pts',(2.01817678125675,-6.46172209820154,86.293538950049));
#30149=CARTESIAN_POINT('Ctrl Pts',(2.19414072347513,-6.40140886724072,86.30228875241));
#30150=CARTESIAN_POINT('Ctrl Pts',(2.37010298131926,-6.34109621361438,86.3110384710155));
#30151=CARTESIAN_POINT('Ctrl Pts',(2.54357687926739,-6.27352420826041,86.3197881896209));
#30152=CARTESIAN_POINT('Ctrl Pts',(2.71397317789794,-6.19892237325574,86.3285379082264));
#30153=CARTESIAN_POINT('Ctrl Pts',(2.88436790207019,-6.12432122757049,86.3372875459847));
#30154=CARTESIAN_POINT('Ctrl Pts',(3.0516848212607,-6.04269049717511,86.346037183743));
#30155=CARTESIAN_POINT('Ctrl Pts',(3.21535561997198,-5.95430745235033,86.3547868215012));
#30156=CARTESIAN_POINT('Ctrl Pts',(3.37902496075091,-5.86592519481626,86.3635363813202));
#30157=CARTESIAN_POINT('Ctrl Pts',(3.53904799384687,-5.77079087940347,86.3722859411393));
#30158=CARTESIAN_POINT('Ctrl Pts',(3.69488118814798,-5.66922763747145,86.3810355009583));
#30159=CARTESIAN_POINT('Ctrl Pts',(3.85071304610652,-5.56766526649177,86.3897849857457));
#30160=CARTESIAN_POINT('Ctrl Pts',(4.00235489705792,-5.45967423580842,86.3985344705331));
#30161=CARTESIAN_POINT('Ctrl Pts',(4.14929168607484,-5.34562133936461,86.4072839553206));
#30162=CARTESIAN_POINT('Ctrl Pts',(4.2962272638558,-5.23156938308675,86.4160333679839));
#30163=CARTESIAN_POINT('Ctrl Pts',(4.43845763091885,-5.1114558367736,86.4247827806471));
#30164=CARTESIAN_POINT('Ctrl Pts',(4.57549970660775,-4.98568866204383,86.4335321933104));
#30165=CARTESIAN_POINT('Ctrl Pts',(4.71254069815106,-4.85992248226345,86.4422815367568));
#30166=CARTESIAN_POINT('Ctrl Pts',(4.84439326931123,-4.72850295734197,86.4510308802031));
#30167=CARTESIAN_POINT('Ctrl Pts',(4.97060959434507,-4.59187644221889,86.4597802236494));
#30168=CARTESIAN_POINT('Ctrl Pts',(5.09682496280325,-4.45525096256881,86.4685295007857));
#30169=CARTESIAN_POINT('Ctrl Pts',(5.21740397615651,-4.31341878218553,86.477278777922));
#30170=CARTESIAN_POINT('Ctrl Pts',(5.33193710451749,-4.16686161438914,86.4860280550583));
#30171=CARTESIAN_POINT('Ctrl Pts',(5.44646940289209,-4.0203055086475,86.4947772687913));
#30172=CARTESIAN_POINT('Ctrl Pts',(5.55495572749501,-3.86902470980369,86.5035264825242));
#30173=CARTESIAN_POINT('Ctrl Pts',(5.65702762491302,-3.71353301466016,86.5122756962572));
#30174=CARTESIAN_POINT('Ctrl Pts',(5.75909881655015,-3.55804239467118,86.5210248494933));
#30175=CARTESIAN_POINT('Ctrl Pts',(5.85475551250658,-3.39834117619768,86.5297740027294));
#30176=CARTESIAN_POINT('Ctrl Pts',(5.94367283727983,-3.23497174692174,86.5385231559655));
#30177=CARTESIAN_POINT('Ctrl Pts',(6.03258957676214,-3.07160339301159,86.5472722516111));
#30178=CARTESIAN_POINT('Ctrl Pts',(6.11476689685199,-2.90456712829685,86.5560213472566));
#30179=CARTESIAN_POINT('Ctrl Pts',(6.18992570525187,-2.73443024476072,86.5647704429022));
#30180=CARTESIAN_POINT('Ctrl Pts',(6.2650840438863,-2.56429442463194,86.5735194838632));
#30181=CARTESIAN_POINT('Ctrl Pts',(6.33322384283255,-2.39105828656153,86.5822685248242));
#30182=CARTESIAN_POINT('Ctrl Pts',(6.39411368719979,-2.21531017132237,86.5910175657853));
#30183=CARTESIAN_POINT('Ctrl Pts',(6.45500317120843,-2.03956309619663,86.5997665549677));
#30184=CARTESIAN_POINT('Ctrl Pts',(6.50864269270033,-1.86130434438774,86.6085155441501));
#30185=CARTESIAN_POINT('Ctrl Pts',(6.55485008446299,-1.68113930720078,86.6172645333325));
#30186=CARTESIAN_POINT('Ctrl Pts',(6.60199664749375,-1.49731239211969,86.6261913468619));
#30187=CARTESIAN_POINT('Ctrl Pts',(6.64140563640882,-1.31150116499796,86.6351181603912));
#30188=CARTESIAN_POINT('Ctrl Pts',(6.67293772282152,-1.1243625515578,86.6440449739206));
#30189=CARTESIAN_POINT('Ctrl Pts',(6.70384494949855,-0.940932395052489,
86.6527948880761));
#30190=CARTESIAN_POINT('Ctrl Pts',(6.72718449348918,-0.756227260507799,
86.6615448022317));
#30191=CARTESIAN_POINT('Ctrl Pts',(6.74287707373924,-0.570874564542713,
86.6702947163872));
#30192=CARTESIAN_POINT('Ctrl Pts',(6.75856934538665,-0.385525513633454,
86.6790444584712));
#30193=CARTESIAN_POINT('Ctrl Pts',(6.766614930041,-0.199529212419166,86.6877942005552));
#30194=CARTESIAN_POINT('Ctrl Pts',(6.76698649908906,-0.0135174386013192,
86.6965439426391));
#30195=CARTESIAN_POINT('Ctrl Pts',(6.76735806132392,0.172490924444834,86.705293524285));
#30196=CARTESIAN_POINT('Ctrl Pts',(6.76005588896294,0.358514472900411,86.7140431059309));
#30197=CARTESIAN_POINT('Ctrl Pts',(6.74510478454593,0.543921359661166,86.7227926875768));
#30198=CARTESIAN_POINT('Ctrl Pts',(6.730153934407,0.729325093149327,86.7315421204159));
#30199=CARTESIAN_POINT('Ctrl Pts',(6.70755443556913,0.914111900255165,86.7402915532549));
#30200=CARTESIAN_POINT('Ctrl Pts',(6.67738304682339,1.09765415591413,86.7490409860939));
#30201=CARTESIAN_POINT('Ctrl Pts',(6.64721213111883,1.28119353391156,86.7577902817553));
#30202=CARTESIAN_POINT('Ctrl Pts',(6.60946960955518,1.46348811672544,86.7665395774166));
#30203=CARTESIAN_POINT('Ctrl Pts',(6.56428366991208,1.64391876348121,86.7752888730779));
#30204=CARTESIAN_POINT('Ctrl Pts',(6.51909837867743,1.82434682109625,86.7840380431888));
#30205=CARTESIAN_POINT('Ctrl Pts',(6.46646995271946,2.00291071820365,86.7927872132996));
#30206=CARTESIAN_POINT('Ctrl Pts',(6.40657713281573,2.17900400212633,86.8015363834104));
#30207=CARTESIAN_POINT('Ctrl Pts',(6.34668509279086,2.35509499309588,86.8102854395962));
#30208=CARTESIAN_POINT('Ctrl Pts',(6.27952894037554,2.52871516398052,86.819034495782));
#30209=CARTESIAN_POINT('Ctrl Pts',(6.20533675061478,2.69927486771349,86.8277835519678));
#30210=CARTESIAN_POINT('Ctrl Pts',(6.12832117907949,2.87632521635854,86.83686555325));
#30211=CARTESIAN_POINT('Ctrl Pts',(6.04372366626113,3.0500772891993,86.8459475545323));
#30212=CARTESIAN_POINT('Ctrl Pts',(5.95185378007903,3.2198952747813,86.8550295558146));
#30213=CARTESIAN_POINT('Ctrl Pts',(5.86334450817404,3.38350129286694,86.8637793361217));
#30214=CARTESIAN_POINT('Ctrl Pts',(5.76808562057286,3.54345567124912,86.8725291164288));
#30215=CARTESIAN_POINT('Ctrl Pts',(5.66640068804512,3.69921508465267,86.8812788967359));
#30216=CARTESIAN_POINT('Ctrl Pts',(5.56471941107956,3.85496889852236,86.8900283624894));
#30217=CARTESIAN_POINT('Ctrl Pts',(5.45661270815152,4.00652780919585,86.8987778282429));
#30218=CARTESIAN_POINT('Ctrl Pts',(5.34244776449158,4.15337704569173,86.9075272939964));
#30219=CARTESIAN_POINT('Ctrl Pts',(5.22828631819634,4.30022178356203,86.916276491716));
#30220=CARTESIAN_POINT('Ctrl Pts',(5.10806717844102,4.44235690972642,86.9250256894356));
#30221=CARTESIAN_POINT('Ctrl Pts',(4.98219864544745,4.57929969070617,86.9337748871552));
#30222=CARTESIAN_POINT('Ctrl Pts',(4.85633329944053,4.71623900429972,86.9425238633454));
#30223=CARTESIAN_POINT('Ctrl Pts',(4.72481904033678,4.84798602483587,86.9512728395357));
#30224=CARTESIAN_POINT('Ctrl Pts',(4.58810250737231,4.97409332259096,86.9600218157259));
#30225=CARTESIAN_POINT('Ctrl Pts',(4.4513770868568,5.10020881822102,86.9687713606621));
#30226=CARTESIAN_POINT('Ctrl Pts',(4.30944892636094,5.22068366307898,86.9775209055983));
#30227=CARTESIAN_POINT('Ctrl Pts',(4.16280009466709,5.33510865604813,86.9862704505344));
#30228=CARTESIAN_POINT('Ctrl Pts',(4.01615988348845,5.4495269227285,86.9950194811427));
#30229=CARTESIAN_POINT('Ctrl Pts',(3.86479978232295,5.55789587288581,87.003768511751));
#30230=CARTESIAN_POINT('Ctrl Pts',(3.70923383581141,5.6598474671383,87.0125175423592));
#30231=CARTESIAN_POINT('Ctrl Pts',(3.55366577799618,5.76180044505335,87.0212666917073));
#30232=CARTESIAN_POINT('Ctrl Pts',(3.39389200026922,5.85733573571011,87.0300158410553));
#30233=CARTESIAN_POINT('Ctrl Pts',(3.23045513626128,5.94612887621881,87.0387649904033));
#30234=CARTESIAN_POINT('Ctrl Pts',(3.18695122151632,5.9697639920666,87.0410938545163));
#30235=CARTESIAN_POINT('Ctrl Pts',(3.14318791262683,5.99292165435323,87.0434227186293));
#30236=CARTESIAN_POINT('Ctrl Pts',(3.09917575053243,6.01559628526647,87.0457515827423));
#30237=CARTESIAN_POINT('Ctrl Pts',(3.09917575053258,6.01559628526639,85.045900138346));
#30238=CARTESIAN_POINT('Ctrl Pts',(2.93640024297169,6.09945661795675,85.0545033613981));
#30239=CARTESIAN_POINT('Ctrl Pts',(2.7701058164934,6.17676461498262,85.0631065844503));
#30240=CARTESIAN_POINT('Ctrl Pts',(2.60083589136805,6.24723472155255,85.0717098075024));
#30241=CARTESIAN_POINT('Ctrl Pts',(2.43176061199912,6.3176237936021,85.080303137593));
#30242=CARTESIAN_POINT('Ctrl Pts',(2.25971694099547,6.3811905450431,85.0888964676836));
#30243=CARTESIAN_POINT('Ctrl Pts',(2.08527064437643,6.4376964311547,85.0974897977742));
#30244=CARTESIAN_POINT('Ctrl Pts',(2.04873372809135,6.44953131025782,85.0992896283709));
#30245=CARTESIAN_POINT('Ctrl Pts',(2.01209149180469,6.4610566140694,85.1010894589676));
#30246=CARTESIAN_POINT('Ctrl Pts',(1.97534925110199,6.47227041587191,85.1028892895643));
#30247=CARTESIAN_POINT('Ctrl Pts',(1.79988327660372,6.52582296529399,85.1114845473258));
#30248=CARTESIAN_POINT('Ctrl Pts',(1.62234168686871,6.57220438954524,85.1200798050874));
#30249=CARTESIAN_POINT('Ctrl Pts',(1.4433256820181,6.61128580350502,85.1286750628489));
#30250=CARTESIAN_POINT('Ctrl Pts',(1.26414203626826,6.65040381555213,85.137278369705));
#30251=CARTESIAN_POINT('Ctrl Pts',(1.0834815177399,6.68220810696158,85.145881676561));
#30252=CARTESIAN_POINT('Ctrl Pts',(0.901953607722654,6.7066212573483,85.1544849834171));
#30253=CARTESIAN_POINT('Ctrl Pts',(0.712899487659699,6.7320465854088,85.1634449863563));
#30254=CARTESIAN_POINT('Ctrl Pts',(0.52290489829983,6.74945479681724,85.1724049892955));
#30255=CARTESIAN_POINT('Ctrl Pts',(0.332660554966909,6.75881838453802,85.1813649922347));
#30256=CARTESIAN_POINT('Ctrl Pts',(0.149490065854732,6.76783380603551,85.189991835441));
#30257=CARTESIAN_POINT('Ctrl Pts',(-0.0339116426335964,6.76939210650464,
85.1986186786473));
#30258=CARTESIAN_POINT('Ctrl Pts',(-0.216930857746648,6.7635220117153,85.2072455218536));
#30259=CARTESIAN_POINT('Ctrl Pts',(-0.400124992964936,6.7576463065992,85.2158806101413));
#30260=CARTESIAN_POINT('Ctrl Pts',(-0.582935600874554,6.74432805375582,
85.224515698429));
#30261=CARTESIAN_POINT('Ctrl Pts',(-0.764754570328876,6.72364777833886,
85.2331507867167));
#30262=CARTESIAN_POINT('Ctrl Pts',(-0.946843577441532,6.70293678856265,
85.2417986998435));
#30263=CARTESIAN_POINT('Ctrl Pts',(-1.12793770097154,6.67484196857731,85.2504466129702));
#30264=CARTESIAN_POINT('Ctrl Pts',(-1.30743800710944,6.63949507549826,85.2590945260969));
#30265=CARTESIAN_POINT('Ctrl Pts',(-1.32757520874287,6.63552969221641,85.2600646902938));
#30266=CARTESIAN_POINT('Ctrl Pts',(-1.34769236653319,6.63147309036324,85.2610348544906));
#30267=CARTESIAN_POINT('Ctrl Pts',(-1.36778864671266,6.62732549509408,85.2620050186875));
#30268=CARTESIAN_POINT('Ctrl Pts',(-1.5381571931178,6.59216377507559,85.2702296982062));
#30269=CARTESIAN_POINT('Ctrl Pts',(-1.70739353262312,6.55038200664134,85.278454377725));
#30270=CARTESIAN_POINT('Ctrl Pts',(-1.87494565224324,6.50206642546308,85.2866790572437));
#30271=CARTESIAN_POINT('Ctrl Pts',(-2.04232165562978,6.45380162942678,85.2948950916937));
#30272=CARTESIAN_POINT('Ctrl Pts',(-2.20801662288681,6.39901679531064,85.3031111261437));
#30273=CARTESIAN_POINT('Ctrl Pts',(-2.37148799781839,6.33784929421672,85.3113271605938));
#30274=CARTESIAN_POINT('Ctrl Pts',(-2.53482028944595,6.27673383512803,85.3195362047483));
#30275=CARTESIAN_POINT('Ctrl Pts',(-2.69593242280624,6.20924664933658,85.3277452489029));
#30276=CARTESIAN_POINT('Ctrl Pts',(-2.85429620588865,6.13557512944383,85.3359542930574));
#30277=CARTESIAN_POINT('Ctrl Pts',(-3.01255696284828,6.06195153775099,85.3441579966854));
#30278=CARTESIAN_POINT('Ctrl Pts',(-3.16807260722118,5.98215177668911,85.3523617003134));
#30279=CARTESIAN_POINT('Ctrl Pts',(-3.32033408548818,5.89641166818815,85.3605654039413));
#30280=CARTESIAN_POINT('Ctrl Pts',(-3.47252699101504,5.81071017374932,85.3687654129353));
#30281=CARTESIAN_POINT('Ctrl Pts',(-3.62146833855935,5.71907383731397,85.3769654219293));
#30282=CARTESIAN_POINT('Ctrl Pts',(-3.76667280761687,5.62178485539598,85.3851654309232));
#30283=CARTESIAN_POINT('Ctrl Pts',(-3.91186566581762,5.52450365291098,85.3933647842271));
#30284=CARTESIAN_POINT('Ctrl Pts',(-4.05332193831789,5.42157089734255,85.401564137531));
#30285=CARTESIAN_POINT('Ctrl Pts',(-4.19058417650266,5.3133128328422,85.4097634908348));
#30286=CARTESIAN_POINT('Ctrl Pts',(-4.32784551977821,5.20505547415241,85.4179627906813));
#30287=CARTESIAN_POINT('Ctrl Pts',(-4.46091260103117,5.0914730968509,85.4261620905279));
#30288=CARTESIAN_POINT('Ctrl Pts',(-4.58936014499293,4.97293298361746,85.4343613903744));
#30289=CARTESIAN_POINT('Ctrl Pts',(-4.71783015315902,4.85437213889129,85.4425621241973));
#30290=CARTESIAN_POINT('Ctrl Pts',(-4.84167875093471,4.73085207391203,85.4507628580202));
#30291=CARTESIAN_POINT('Ctrl Pts',(-4.96051666765852,4.60277779062623,85.4589635918431));
#30292=CARTESIAN_POINT('Ctrl Pts',(-5.07939692655719,4.47465787423066,85.4671672476031));
#30293=CARTESIAN_POINT('Ctrl Pts',(-5.19326270426276,4.34198076971755,85.4753709033629));
#30294=CARTESIAN_POINT('Ctrl Pts',(-5.30176421555099,4.2051855134706,85.4835745591229));
#30295=CARTESIAN_POINT('Ctrl Pts',(-5.41039002229519,4.06823354946403,85.4917876126978));
#30296=CARTESIAN_POINT('Ctrl Pts',(-5.51363906262672,3.92715428986149,85.5000006662727));
#30297=CARTESIAN_POINT('Ctrl Pts',(-5.6112035853492,3.78241765591326,85.5082137198476));
#30298=CARTESIAN_POINT('Ctrl Pts',(-5.70882583918863,3.63759537805155,85.5164316332706));
#30299=CARTESIAN_POINT('Ctrl Pts',(-5.8007566819811,3.4891117162018,85.5246495466937));
#30300=CARTESIAN_POINT('Ctrl Pts',(-5.88673383057957,3.33746218074603,85.5328674601167));
#30301=CARTESIAN_POINT('Ctrl Pts',(-5.97284507452841,3.1855761231687,85.5410981907126));
#30302=CARTESIAN_POINT('Ctrl Pts',(-6.05298390287635,3.03051464266153,85.5493289213085));
#30303=CARTESIAN_POINT('Ctrl Pts',(-6.12693521146768,2.8727954877571,85.5575596519044));
#30304=CARTESIAN_POINT('Ctrl Pts',(-6.1948506440094,2.7279493068106,85.5651185935811));
#30305=CARTESIAN_POINT('Ctrl Pts',(-6.2575478694029,2.5808620072146,85.5726775352578));
#30306=CARTESIAN_POINT('Ctrl Pts',(-6.31489739915265,2.43194568980787,85.5802364769345));
#30307=CARTESIAN_POINT('Ctrl Pts',(-6.38883459767798,2.23995710033198,85.5899817525074));
#30308=CARTESIAN_POINT('Ctrl Pts',(-6.45408504329421,2.04440410320538,85.5997270280803));
#30309=CARTESIAN_POINT('Ctrl Pts',(-6.51033274202365,1.84603807873373,85.6094723036533));
#30310=CARTESIAN_POINT('Ctrl Pts',(-6.5637575996793,1.65762723063672,85.6187285038545));
#30311=CARTESIAN_POINT('Ctrl Pts',(-6.60906092362952,1.46667898193729,85.6279847040558));
#30312=CARTESIAN_POINT('Ctrl Pts',(-6.64601882907735,1.27386134392614,85.6372409042571));
#30313=CARTESIAN_POINT('Ctrl Pts',(-6.68284040545216,1.08175496510389,85.6464629604997));
#30314=CARTESIAN_POINT('Ctrl Pts',(-6.71137790879288,0.88779312340325,85.6556850167424));
#30315=CARTESIAN_POINT('Ctrl Pts',(-6.73145708710518,0.692657552085745,
85.6649070729851));
#30316=CARTESIAN_POINT('Ctrl Pts',(-6.75142263795899,0.498626247022922,
85.6740769418924));
#30317=CARTESIAN_POINT('Ctrl Pts',(-6.76302523036422,0.303434632015563,
85.6832468107997));
#30318=CARTESIAN_POINT('Ctrl Pts',(-6.76614176185295,0.107771325080025,
85.692416679707));
#30319=CARTESIAN_POINT('Ctrl Pts',(-6.76668136840097,0.0738935343331261,
85.6940043810747));
#30320=CARTESIAN_POINT('Ctrl Pts',(-6.76696669415284,0.0400016440156962,
85.6955920824423));
#30321=CARTESIAN_POINT('Ctrl Pts',(-6.76699725127752,0.00609927884748164,
85.6971797838099));
#30322=CARTESIAN_POINT('',(-6.767,4.35244939048229E-12,85.3028202161897));
#30323=CARTESIAN_POINT('Ctrl Pts',(3.0991757505325,6.01559628526643,84.6515000956437));
#30324=CARTESIAN_POINT('Ctrl Pts',(2.93966228093791,6.09777604823717,84.6599141842356));
#30325=CARTESIAN_POINT('Ctrl Pts',(2.77681272021419,6.17364026143562,84.6683282728275));
#30326=CARTESIAN_POINT('Ctrl Pts',(2.61117916232911,6.24291857885543,84.6767423614193));
#30327=CARTESIAN_POINT('Ctrl Pts',(2.4512708651572,6.30980223402163,84.6848656100904));
#30328=CARTESIAN_POINT('Ctrl Pts',(2.28876818650668,6.37054755109567,84.6929888587616));
#30329=CARTESIAN_POINT('Ctrl Pts',(2.12418928260589,6.42495983580149,84.7011121074327));
#30330=CARTESIAN_POINT('Ctrl Pts',(1.95959542423578,6.47937706468194,84.7092360942231));
#30331=CARTESIAN_POINT('Ctrl Pts',(1.79292531213377,6.52745999986657,84.7173600810136));
#30332=CARTESIAN_POINT('Ctrl Pts',(1.62471304845604,6.56906359462113,84.725484067804));
#30333=CARTESIAN_POINT('Ctrl Pts',(1.45645349744324,6.61067888485545,84.7336103383856));
#30334=CARTESIAN_POINT('Ctrl Pts',(1.2866512865693,6.64581111970828,84.7417366089673));
#30335=CARTESIAN_POINT('Ctrl Pts',(1.11585146793037,6.6743662247076,84.7498628795489));
#30336=CARTESIAN_POINT('Ctrl Pts',(0.944971136688856,6.70293479017685,84.7579929807388));
#30337=CARTESIAN_POINT('Ctrl Pts',(0.773092621512681,6.72491999178411,84.7661230819287));
#30338=CARTESIAN_POINT('Ctrl Pts',(0.600766820405878,6.74027953630259,84.7742531831185));
#30339=CARTESIAN_POINT('Ctrl Pts',(0.428235182212657,6.75565742725481,84.7823929954273));
#30340=CARTESIAN_POINT('Ctrl Pts',(0.255255555454282,6.76439382711683,84.7905328077361));
#30341=CARTESIAN_POINT('Ctrl Pts',(0.0823804065246283,6.76649853828558,
84.7986726200448));
#30342=CARTESIAN_POINT('Ctrl Pts',(-0.0906175152634459,6.76860474418279,
84.8068182131036));
#30343=CARTESIAN_POINT('Ctrl Pts',(-0.263510447505407,6.76406988825879,
84.8149638061625));
#30344=CARTESIAN_POINT('Ctrl Pts',(-0.435750638838326,6.7529556773869,84.8231093992213));
#30345=CARTESIAN_POINT('Ctrl Pts',(-0.608231588421889,6.74182593101227,
84.8312663782331));
#30346=CARTESIAN_POINT('Ctrl Pts',(-0.780057614198549,6.72409850849497,
84.839423357245));
#30347=CARTESIAN_POINT('Ctrl Pts',(-0.950689986302749,6.69988638336082,
84.8475803362569));
#30348=CARTESIAN_POINT('Ctrl Pts',(-0.991536191438923,6.69409045250774,
84.8495329647874));
#30349=CARTESIAN_POINT('Ctrl Pts',(-1.03231406068258,6.68792315174578,84.851485593318));
#30350=CARTESIAN_POINT('Ctrl Pts',(-1.07301633482434,6.68138645381332,84.8534382218486));
#30351=CARTESIAN_POINT('Ctrl Pts',(-1.24463313664217,6.65382516351021,84.8616712719821));
#30352=CARTESIAN_POINT('Ctrl Pts',(-1.41543824272571,6.61960716377652,84.8699043221155));
#30353=CARTESIAN_POINT('Ctrl Pts',(-1.58487627386707,6.57878835322533,84.878137372249));
#30354=CARTESIAN_POINT('Ctrl Pts',(-1.75411253035867,6.538018151603,84.8863606180853));
#30355=CARTESIAN_POINT('Ctrl Pts',(-1.92198460880699,6.4906628745298,84.8945838639217));
#30356=CARTESIAN_POINT('Ctrl Pts',(-2.08794366208133,6.43682998563535,84.902807109758));
#30357=CARTESIAN_POINT('Ctrl Pts',(-2.2537383006969,6.38305042866757,84.911022208873));
#30358=CARTESIAN_POINT('Ctrl Pts',(-2.41762335013413,6.32280614983077,84.919237307988));
#30359=CARTESIAN_POINT('Ctrl Pts',(-2.57906145728834,6.25625534961048,84.927452407103));
#30360=CARTESIAN_POINT('Ctrl Pts',(-2.74037192917028,6.18975716540296,84.9356610112433));
#30361=CARTESIAN_POINT('Ctrl Pts',(-2.89923898242252,6.11696252687464,84.9438696153837));
#30362=CARTESIAN_POINT('Ctrl Pts',(-3.05514161475003,6.03807905826204,84.9520782195241));
#30363=CARTESIAN_POINT('Ctrl Pts',(-3.21095217310614,5.95924217715167,84.9602819757746));
#30364=CARTESIAN_POINT('Ctrl Pts',(-3.36380147952,5.87432379091544,84.9684857320251));
#30365=CARTESIAN_POINT('Ctrl Pts',(-3.5131895866198,5.78357916246214,84.9766894882757));
#30366=CARTESIAN_POINT('Ctrl Pts',(-3.6625334935432,5.69286138305769,84.9848908172414));
#30367=CARTESIAN_POINT('Ctrl Pts',(-3.80841793334186,5.59632097767957,84.9930921462072));
#30368=CARTESIAN_POINT('Ctrl Pts',(-3.95036838552731,5.49425869600498,85.001293475173));
#30369=CARTESIAN_POINT('Ctrl Pts',(-4.09229926138989,5.39221048969365,85.0094936730973));
#30370=CARTESIAN_POINT('Ctrl Pts',(-4.23029693891469,5.28464213219884,85.0176938710215));
#30371=CARTESIAN_POINT('Ctrl Pts',(-4.36391666322163,5.17189717187577,85.0258940689457));
#30372=CARTESIAN_POINT('Ctrl Pts',(-4.49754217470596,5.05914732847808,85.0340946220271));
#30373=CARTESIAN_POINT('Ctrl Pts',(-4.62678908133326,4.94122066660374,85.0422951751084));
#30374=CARTESIAN_POINT('Ctrl Pts',(-4.75124641020018,4.81850044615126,85.0504957281898));
#30375=CARTESIAN_POINT('Ctrl Pts',(-4.87573168351915,4.69575267128035,85.0586981225445));
#30376=CARTESIAN_POINT('Ctrl Pts',(-4.99542498210598,4.56820944565328,85.0669005168992));
#30377=CARTESIAN_POINT('Ctrl Pts',(-5.1099528035355,4.43629026841568,85.0751029112539));
#30378=CARTESIAN_POINT('Ctrl Pts',(-5.22458772861137,4.30424772355674,85.0833129762893));
#30379=CARTESIAN_POINT('Ctrl Pts',(-5.33404729014861,4.16782132194593,85.0915230413246));
#30380=CARTESIAN_POINT('Ctrl Pts',(-5.43799826248202,4.02746370526695,85.09973310636));
#30381=CARTESIAN_POINT('Ctrl Pts',(-5.54199898390667,3.88703891592259,85.1079471005868));
#30382=CARTESIAN_POINT('Ctrl Pts',(-5.64048565794353,3.74267945609009,85.1161610948137));
#30383=CARTESIAN_POINT('Ctrl Pts',(-5.73316896334866,3.59486615017802,85.1243750890405));
#30384=CARTESIAN_POINT('Ctrl Pts',(-5.82597862696782,3.4468513254998,85.1326002816772));
#30385=CARTESIAN_POINT('Ctrl Pts',(-5.91296893139418,3.29537355503984,85.1408254743139));
#30386=CARTESIAN_POINT('Ctrl Pts',(-5.9938964313008,3.14093848568219,85.1490506669506));
#30387=CARTESIAN_POINT('Ctrl Pts',(-6.06667435844338,3.00205535894607,85.1564475650525));
#30388=CARTESIAN_POINT('Ctrl Pts',(-6.13454962914461,2.86078102512443,85.1638444631543));
#30389=CARTESIAN_POINT('Ctrl Pts',(-6.19737899166069,2.71749565477531,85.1712413612562));
#30390=CARTESIAN_POINT('Ctrl Pts',(-6.27351749308934,2.54385815571206,85.1802051437003));
#30391=CARTESIAN_POINT('Ctrl Pts',(-6.34240785676341,2.36689760305845,85.1891689261444));
#30392=CARTESIAN_POINT('Ctrl Pts',(-6.40377895071463,2.18721378707802,85.1981327085885));
#30393=CARTESIAN_POINT('Ctrl Pts',(-6.46499023798479,2.00799785707495,85.2070731498759));
#30394=CARTESIAN_POINT('Ctrl Pts',(-6.51872125062415,1.8260730545473,85.2160135911632));
#30395=CARTESIAN_POINT('Ctrl Pts',(-6.56474965271754,1.64205694089607,85.2249540324506));
#30396=CARTESIAN_POINT('Ctrl Pts',(-6.61070198134038,1.45834495999257,85.2338796974181));
#30397=CARTESIAN_POINT('Ctrl Pts',(-6.64897703290111,1.27254880623831,85.2428053623855));
#30398=CARTESIAN_POINT('Ctrl Pts',(-6.67940181839658,1.08530196185229,85.2517310273529));
#30399=CARTESIAN_POINT('Ctrl Pts',(-6.70974215523581,0.898574849787709,
85.2606319177689));
#30400=CARTESIAN_POINT('Ctrl Pts',(-6.732275662664,0.710405329823299,85.2695328081849));
#30401=CARTESIAN_POINT('Ctrl Pts',(-6.74688020335029,0.521436977630101,
85.2784336986009));
#30402=CARTESIAN_POINT('Ctrl Pts',(-6.76021796589159,0.348859485224565,
85.2865625377972));
#30403=CARTESIAN_POINT('Ctrl Pts',(-6.766943122425,0.175616043403798,85.2946913769935));
#30404=CARTESIAN_POINT('Ctrl Pts',(-6.76699964058907,0.00220550842528099,
85.3028202161898));
#30405=CARTESIAN_POINT('Ctrl Pts',(-6.767,4.35244894485728E-12,85.3028202161897));
#30406=CARTESIAN_POINT('Ctrl Pts',(-6.76700000000012,-0.186007249411442,
85.3115697279957));
#30407=CARTESIAN_POINT('Ctrl Pts',(-6.75932637295461,-0.37201435552342,
85.3203192398016));
#30408=CARTESIAN_POINT('Ctrl Pts',(-6.74400518266961,-0.557389537151059,
85.3290687516076));
#30409=CARTESIAN_POINT('Ctrl Pts',(-6.72868405709688,-0.742763935807543,
85.3378182264581));
#30410=CARTESIAN_POINT('Ctrl Pts',(-6.70571545653043,-0.927506129691318,
85.3465677013087));
#30411=CARTESIAN_POINT('Ctrl Pts',(-6.6751773941571,-1.11098863924618,85.3553171761592));
#30412=CARTESIAN_POINT('Ctrl Pts',(-6.64463945823134,-1.29447038906332,
85.3640666147812));
#30413=CARTESIAN_POINT('Ctrl Pts',(-6.60653217027191,-1.47669218228071,
85.3728160534032));
#30414=CARTESIAN_POINT('Ctrl Pts',(-6.56098496116743,-1.65703510503998,
85.3815654920252));
#30415=CARTESIAN_POINT('Ctrl Pts',(-6.51543793687551,-1.837377296039,85.3903148951455));
#30416=CARTESIAN_POINT('Ctrl Pts',(-6.46245112202676,-2.01584035396935,
85.3990642982657));
#30417=CARTESIAN_POINT('Ctrl Pts',(-6.40220448416282,-2.19181813638027,
85.4078137013859));
#30418=CARTESIAN_POINT('Ctrl Pts',(-6.34195808575224,-2.36779521935847,
85.4165630697312));
#30419=CARTESIAN_POINT('Ctrl Pts',(-6.27445201489266,-2.54128677544751,
85.4253124380765));
#30420=CARTESIAN_POINT('Ctrl Pts',(-6.19991555136209,-2.71170355237783,
85.4340618064218));
#30421=CARTESIAN_POINT('Ctrl Pts',(-6.1253793778906,-2.88211966613026,85.4428111407188));
#30422=CARTESIAN_POINT('Ctrl Pts',(-6.04381298133635,-3.0494607621041,85.4515604750159));
#30423=CARTESIAN_POINT('Ctrl Pts',(-5.95549339426319,-3.2131584820683,85.4603098093129));
#30424=CARTESIAN_POINT('Ctrl Pts',(-5.86717414355174,-3.37685557859613,
85.4690591102885));
#30425=CARTESIAN_POINT('Ctrl Pts',(-5.77210188986252,-3.53690907467289,
85.4778084112641));
#30426=CARTESIAN_POINT('Ctrl Pts',(-5.67059953467082,-3.69277536784884,
85.4865577122396));
#30427=CARTESIAN_POINT('Ctrl Pts',(-5.56909755761774,-3.84864108035781,
85.4953069806204));
#30428=CARTESIAN_POINT('Ctrl Pts',(-5.46116568338073,-4.00031938104276,
85.5040562490012));
#30429=CARTESIAN_POINT('Ctrl Pts',(-5.3471704868611,-4.14729511663224,85.5128055173819));
#30430=CARTESIAN_POINT('Ctrl Pts',(-5.23317570555531,-4.29427031688023,
85.5215547538945));
#30431=CARTESIAN_POINT('Ctrl Pts',(-5.11311782178838,-4.43654275987091,
85.5303039904071));
#30432=CARTESIAN_POINT('Ctrl Pts',(-4.98740459172068,-4.57362924147591,
85.5390532269197));
#30433=CARTESIAN_POINT('Ctrl Pts',(-4.86169180910883,-4.71071523514381,
85.5478024322909));
#30434=CARTESIAN_POINT('Ctrl Pts',(-4.73032391415484,-4.84261509316472,
85.556551637662));
#30435=CARTESIAN_POINT('Ctrl Pts',(-4.59374707237345,-4.96888084331476,
85.5653008430331));
#30436=CARTESIAN_POINT('Ctrl Pts',(-4.45717070537455,-5.09514615452678,
85.5740500179893));
#30437=CARTESIAN_POINT('Ctrl Pts',(-4.31538563819563,-5.21577720253588,
85.5827991929456));
#30438=CARTESIAN_POINT('Ctrl Pts',(-4.16887341290702,-5.33036429028608,
85.5915483679018));
#30439=CARTESIAN_POINT('Ctrl Pts',(-4.02236168477416,-5.44495098921118,
85.6002975131697));
#30440=CARTESIAN_POINT('Ctrl Pts',(-3.87112305634542,-5.55349359238686,
85.6090466584376));
#30441=CARTESIAN_POINT('Ctrl Pts',(-3.71567117316862,-5.65562346102388,
85.6177958037055));
#30442=CARTESIAN_POINT('Ctrl Pts',(-3.56021980457459,-5.7577529915867,85.6265449200117));
#30443=CARTESIAN_POINT('Ctrl Pts',(-3.40055544862578,-5.85346967275242,
85.6352940363178));
#30444=CARTESIAN_POINT('Ctrl Pts',(-3.23722036323625,-5.94244842803441,
85.644043152624));
#30445=CARTESIAN_POINT('Ctrl Pts',(-3.07388580496276,-6.03142689616358,
85.6527922406949));
#30446=CARTESIAN_POINT('Ctrl Pts',(-2.90688079257944,-6.1136673448471,85.6615413287658));
#30447=CARTESIAN_POINT('Ctrl Pts',(-2.73677251094859,-6.18889046787194,
85.6702904168368));
#30448=CARTESIAN_POINT('Ctrl Pts',(-2.5666647641688,-6.26411335438175,85.679039477399));
#30449=CARTESIAN_POINT('Ctrl Pts',(-2.39345402972317,-6.33231884350206,
85.6877885379612));
#30450=CARTESIAN_POINT('Ctrl Pts',(-2.21772856474251,-6.39327529620969,
85.6965375985235));
#30451=CARTESIAN_POINT('Ctrl Pts',(-2.04200363768457,-6.45423156232023,
85.7052866323035));
#30452=CARTESIAN_POINT('Ctrl Pts',(-1.86376426620255,-6.5079387425201,85.7140356660835));
#30453=CARTESIAN_POINT('Ctrl Pts',(-1.68361578194823,-6.55421443796088,
85.7227846998635));
#30454=CARTESIAN_POINT('Ctrl Pts',(-1.50346783420016,-6.60048999558646,
85.7315337075878));
#30455=CARTESIAN_POINT('Ctrl Pts',(-1.32141106257409,-6.63933404145463,
85.740282715312));
#30456=CARTESIAN_POINT('Ctrl Pts',(-1.1380637595922,-6.67061465527,85.7490317230362));
#30457=CARTESIAN_POINT('Ctrl Pts',(-0.954716987420987,-6.70189517852454,
85.7577807054311));
#30458=CARTESIAN_POINT('Ctrl Pts',(-0.770079973811785,-6.72561226535806,
85.766529687826));
#30459=CARTESIAN_POINT('Ctrl Pts',(-0.58477977055444,-6.74168536939765,
85.7752786702208));
#30460=CARTESIAN_POINT('Ctrl Pts',(-0.391490647555891,-6.75845143942382,
85.7844048508969));
#30461=CARTESIAN_POINT('Ctrl Pts',(-0.197480213106309,-6.76689975924021,
85.793531031573));
#30462=CARTESIAN_POINT('Ctrl Pts',(-0.00346532629976212,-6.76699911271707,
85.802657212249));
#30463=CARTESIAN_POINT('Ctrl Pts',(0.184486595294048,-6.76709536139779,
85.8114981997789));
#30464=CARTESIAN_POINT('Ctrl Pts',(0.372442378183182,-6.75935659726781,
85.8203391873088));
#30465=CARTESIAN_POINT('Ctrl Pts',(0.559750217720002,-6.74380965729034,
85.8291801748388));
#30466=CARTESIAN_POINT('Ctrl Pts',(0.745129914455671,-6.72842275717276,
85.8379301534365));
#30467=CARTESIAN_POINT('Ctrl Pts',(0.929874656312104,-6.70538772273502,
85.8466801320343));
#30468=CARTESIAN_POINT('Ctrl Pts',(1.1133568828957,-6.67478280180777,85.8554301106321));
#30469=CARTESIAN_POINT('Ctrl Pts',(1.29683723118637,-6.64417819418066,85.864179999657));
#30470=CARTESIAN_POINT('Ctrl Pts',(1.47905480730003,-6.60600390230127,85.872929888682));
#30471=CARTESIAN_POINT('Ctrl Pts',(1.65939064804565,-6.56038959797196,85.8816797777069));
#30472=CARTESIAN_POINT('Ctrl Pts',(1.83972470264028,-6.51477574543323,85.8904295800678));
#30473=CARTESIAN_POINT('Ctrl Pts',(2.01817678125618,-6.46172209820172,85.8991793824288));
#30474=CARTESIAN_POINT('Ctrl Pts',(2.19414072347456,-6.40140886724091,85.9079291847898));
#30475=CARTESIAN_POINT('Ctrl Pts',(2.3701029813187,-6.34109621361459,85.9166789033952));
#30476=CARTESIAN_POINT('Ctrl Pts',(2.54357687926684,-6.27352420826064,85.9254286220007));
#30477=CARTESIAN_POINT('Ctrl Pts',(2.7139731778974,-6.19892237325598,85.9341783406062));
#30478=CARTESIAN_POINT('Ctrl Pts',(2.88436790206977,-6.12432122757069,85.9429279783645));
#30479=CARTESIAN_POINT('Ctrl Pts',(3.05168482126039,-6.04269049717527,85.9516776161227));
#30480=CARTESIAN_POINT('Ctrl Pts',(3.21535561997179,-5.95430745235043,85.960427253881));
#30481=CARTESIAN_POINT('Ctrl Pts',(3.37902496075073,-5.86592519481636,85.9691768137));
#30482=CARTESIAN_POINT('Ctrl Pts',(3.53904799384669,-5.77079087940358,85.977926373519));
#30483=CARTESIAN_POINT('Ctrl Pts',(3.69488118814781,-5.66922763747157,85.986675933338));
#30484=CARTESIAN_POINT('Ctrl Pts',(3.85071304610635,-5.56766526649189,85.9954254181255));
#30485=CARTESIAN_POINT('Ctrl Pts',(4.00235489705775,-5.45967423580855,86.0041749029129));
#30486=CARTESIAN_POINT('Ctrl Pts',(4.14929168607467,-5.34562133936473,86.0129243877004));
#30487=CARTESIAN_POINT('Ctrl Pts',(4.29622726385584,-5.23156938308673,86.0216738003637));
#30488=CARTESIAN_POINT('Ctrl Pts',(4.43845763091908,-5.11145583677341,86.030423213027));
#30489=CARTESIAN_POINT('Ctrl Pts',(4.57549970660816,-4.98568866204345,86.0391726256903));
#30490=CARTESIAN_POINT('Ctrl Pts',(4.71254069815155,-4.85992248226297,86.0479219691366));
#30491=CARTESIAN_POINT('Ctrl Pts',(4.8443932693118,-4.72850295734139,86.0566713125829));
#30492=CARTESIAN_POINT('Ctrl Pts',(4.9706095943457,-4.5918764422182,86.0654206560293));
#30493=CARTESIAN_POINT('Ctrl Pts',(5.09682496280396,-4.45525096256801,86.0741699331656));
#30494=CARTESIAN_POINT('Ctrl Pts',(5.21740397615728,-4.3134187821846,86.0829192103019));
#30495=CARTESIAN_POINT('Ctrl Pts',(5.33193710451831,-4.16686161438809,86.0916684874382));
#30496=CARTESIAN_POINT('Ctrl Pts',(5.44646940289288,-4.02030550864643,86.1004177011711));
#30497=CARTESIAN_POINT('Ctrl Pts',(5.55495572749577,-3.8690247098026,86.1091669149041));
#30498=CARTESIAN_POINT('Ctrl Pts',(5.65702762491375,-3.71353301465905,86.117916128637));
#30499=CARTESIAN_POINT('Ctrl Pts',(5.75909881655071,-3.55804239467027,86.1266652818732));
#30500=CARTESIAN_POINT('Ctrl Pts',(5.85475551250698,-3.39834117619698,86.1354144351093));
#30501=CARTESIAN_POINT('Ctrl Pts',(5.9436728372801,-3.23497174692125,86.1441635883454));
#30502=CARTESIAN_POINT('Ctrl Pts',(6.03258957676226,-3.07160339301132,86.1529126839909));
#30503=CARTESIAN_POINT('Ctrl Pts',(6.114766896852,-2.90456712829681,86.1616617796364));
#30504=CARTESIAN_POINT('Ctrl Pts',(6.18992570525178,-2.73443024476092,86.170410875282));
#30505=CARTESIAN_POINT('Ctrl Pts',(6.26508404388622,-2.56429442463214,86.179159916243));
#30506=CARTESIAN_POINT('Ctrl Pts',(6.33322384283247,-2.39105828656172,86.187908957204));
#30507=CARTESIAN_POINT('Ctrl Pts',(6.39411368719972,-2.21531017132257,86.1966579981651));
#30508=CARTESIAN_POINT('Ctrl Pts',(6.45500317120833,-2.03956309619696,86.2054069873475));
#30509=CARTESIAN_POINT('Ctrl Pts',(6.5086426927002,-1.86130434438819,86.2141559765299));
#30510=CARTESIAN_POINT('Ctrl Pts',(6.55485008446285,-1.68113930720135,86.2229049657123));
#30511=CARTESIAN_POINT('Ctrl Pts',(6.60199664749362,-1.49731239212027,86.2318317792416));
#30512=CARTESIAN_POINT('Ctrl Pts',(6.64140563640871,-1.31150116499854,86.240758592771));
#30513=CARTESIAN_POINT('Ctrl Pts',(6.67293772282142,-1.12436255155839,86.2496854063004));
#30514=CARTESIAN_POINT('Ctrl Pts',(6.70384494949847,-0.940932395053078,
86.2584353204559));
#30515=CARTESIAN_POINT('Ctrl Pts',(6.72718449348912,-0.756227260508392,
86.2671852346114));
#30516=CARTESIAN_POINT('Ctrl Pts',(6.74287707373918,-0.570874564543308,
86.275935148767));
#30517=CARTESIAN_POINT('Ctrl Pts',(6.75856934538661,-0.38552551363405,86.284684890851));
#30518=CARTESIAN_POINT('Ctrl Pts',(6.76661493004099,-0.199529212419761,
86.2934346329349));
#30519=CARTESIAN_POINT('Ctrl Pts',(6.76698649908906,-0.0135174386019142,
86.3021843750189));
#30520=CARTESIAN_POINT('Ctrl Pts',(6.76735806132393,0.172490924444367,86.3109339566648));
#30521=CARTESIAN_POINT('Ctrl Pts',(6.76005588896296,0.358514472900072,86.3196835383107));
#30522=CARTESIAN_POINT('Ctrl Pts',(6.74510478454595,0.543921359660955,86.3284331199566));
#30523=CARTESIAN_POINT('Ctrl Pts',(6.73015393440701,0.729325093149245,86.3371825527957));
#30524=CARTESIAN_POINT('Ctrl Pts',(6.70755443556913,0.914111900255209,86.3459319856347));
#30525=CARTESIAN_POINT('Ctrl Pts',(6.67738304682337,1.0976541559143,86.3546814184737));
#30526=CARTESIAN_POINT('Ctrl Pts',(6.6472121311188,1.28119353391173,86.3634307141351));
#30527=CARTESIAN_POINT('Ctrl Pts',(6.60946960955515,1.46348811672561,86.3721800097964));
#30528=CARTESIAN_POINT('Ctrl Pts',(6.56428366991204,1.64391876348138,86.3809293054577));
#30529=CARTESIAN_POINT('Ctrl Pts',(6.51909837867742,1.82434682109629,86.3896784755686));
#30530=CARTESIAN_POINT('Ctrl Pts',(6.46646995271948,2.00291071820357,86.3984276456794));
#30531=CARTESIAN_POINT('Ctrl Pts',(6.4065771328158,2.17900400212613,86.4071768157902));
#30532=CARTESIAN_POINT('Ctrl Pts',(6.34668509279089,2.3550949930958,86.415925871976));
#30533=CARTESIAN_POINT('Ctrl Pts',(6.27952894037553,2.52871516398056,86.4246749281618));
#30534=CARTESIAN_POINT('Ctrl Pts',(6.20533675061471,2.69927486771364,86.4334239843476));
#30535=CARTESIAN_POINT('Ctrl Pts',(6.12832117907942,2.8763252163587,86.4425059856298));
#30536=CARTESIAN_POINT('Ctrl Pts',(6.04372366626106,3.05007728919946,86.4515879869121));
#30537=CARTESIAN_POINT('Ctrl Pts',(5.95185378007895,3.21989527478146,86.4606699881944));
#30538=CARTESIAN_POINT('Ctrl Pts',(5.86334450817396,3.38350129286709,86.4694197685015));
#30539=CARTESIAN_POINT('Ctrl Pts',(5.76808562057277,3.54345567124927,86.4781695488086));
#30540=CARTESIAN_POINT('Ctrl Pts',(5.66640068804502,3.69921508465281,86.4869193291158));
#30541=CARTESIAN_POINT('Ctrl Pts',(5.56471941107939,3.85496889852261,86.4956687948692));
#30542=CARTESIAN_POINT('Ctrl Pts',(5.45661270815127,4.00652780919619,86.5044182606227));
#30543=CARTESIAN_POINT('Ctrl Pts',(5.34244776449124,4.15337704569217,86.5131677263762));
#30544=CARTESIAN_POINT('Ctrl Pts',(5.22828631819606,4.30022178356236,86.5219169240958));
#30545=CARTESIAN_POINT('Ctrl Pts',(5.10806717844082,4.44235690972665,86.5306661218154));
#30546=CARTESIAN_POINT('Ctrl Pts',(4.98219864544733,4.5792996907063,86.539415319535));
#30547=CARTESIAN_POINT('Ctrl Pts',(4.8563332994404,4.71623900429985,86.5481642957252));
#30548=CARTESIAN_POINT('Ctrl Pts',(4.72481904033666,4.847986024836,86.5569132719155));
#30549=CARTESIAN_POINT('Ctrl Pts',(4.58810250737218,4.97409332259108,86.5656622481057));
#30550=CARTESIAN_POINT('Ctrl Pts',(4.45137708685657,5.10020881822122,86.5744117930419));
#30551=CARTESIAN_POINT('Ctrl Pts',(4.30944892636061,5.22068366307925,86.5831613379781));
#30552=CARTESIAN_POINT('Ctrl Pts',(4.16280009466665,5.33510865604847,86.5919108829142));
#30553=CARTESIAN_POINT('Ctrl Pts',(4.0161598834881,5.44952692272875,86.6006599135225));
#30554=CARTESIAN_POINT('Ctrl Pts',(3.86479978232271,5.55789587288598,86.6094089441308));
#30555=CARTESIAN_POINT('Ctrl Pts',(3.70923383581127,5.65984746713839,86.618157974739));
#30556=CARTESIAN_POINT('Ctrl Pts',(3.55366577799604,5.76180044505344,86.6269071240871));
#30557=CARTESIAN_POINT('Ctrl Pts',(3.39389200026908,5.8573357357102,86.6356562734351));
#30558=CARTESIAN_POINT('Ctrl Pts',(3.23045513626113,5.94612887621889,86.6444054227831));
#30559=CARTESIAN_POINT('Ctrl Pts',(3.18695122151628,5.96976399206662,86.6467342868961));
#30560=CARTESIAN_POINT('Ctrl Pts',(3.14318791262691,5.99292165435319,86.6490631510091));
#30561=CARTESIAN_POINT('Ctrl Pts',(3.09917575053262,6.01559628526637,86.6513920151221));
#30562=CARTESIAN_POINT('Origin',(0.,0.,-3.69717978381041));
#30563=CARTESIAN_POINT('',(3.09917575053266,6.01559628526635,89.0455129651334));
#30564=CARTESIAN_POINT('',(3.10355585847744,6.02401335114973,88.6512963024177));
#30565=CARTESIAN_POINT('',(3.09917575053259,6.01559628526639,-3.69717978381041));
#30566=CARTESIAN_POINT('',(-6.76699876913485,-0.00288604624860754,87.6971797838098));
#30567=CARTESIAN_POINT('Ctrl Pts',(-6.7669975382697,-0.00577209250227239,
87.6971797838098));
#30568=CARTESIAN_POINT('Ctrl Pts',(-6.7668219844602,-0.211585183032179,
87.7068360010219));
#30569=CARTESIAN_POINT('Ctrl Pts',(-6.75725319663902,-0.416988477787186,
87.7164922182341));
#30570=CARTESIAN_POINT('Ctrl Pts',(-6.73842610194962,-0.621210647497327,
87.7261484354462));
#30571=CARTESIAN_POINT('Ctrl Pts',(-6.7194757805851,-0.826769487542093,
87.7358678543133));
#30572=CARTESIAN_POINT('Ctrl Pts',(-6.69114566347315,-1.03113163631452,
87.7455872731803));
#30573=CARTESIAN_POINT('Ctrl Pts',(-6.65362223626317,-1.23353157118262,
87.7553066920473));
#30574=CARTESIAN_POINT('Ctrl Pts',(-6.61579460887123,-1.43757235022714,
87.7651049056622));
#30575=CARTESIAN_POINT('Ctrl Pts',(-6.56862406942557,-1.6396189176202,87.7749031192772));
#30576=CARTESIAN_POINT('Ctrl Pts',(-6.51234997735823,-1.83890912565093,
87.7847013328921));
#30577=CARTESIAN_POINT('Ctrl Pts',(-6.46802059077958,-1.99589811203143,
87.7924197834821));
#30578=CARTESIAN_POINT('Ctrl Pts',(-6.41804309218314,-2.15117711307301,
87.800138234072));
#30579=CARTESIAN_POINT('Ctrl Pts',(-6.36255499057615,-2.30438342987763,
87.807856684662));
#30580=CARTESIAN_POINT('Ctrl Pts',(-6.30393649042945,-2.46623298399817,
87.8160105768287));
#30581=CARTESIAN_POINT('Ctrl Pts',(-6.23904228599784,-2.62610950829824,
87.8241644689955));
#30582=CARTESIAN_POINT('Ctrl Pts',(-6.16802248275564,-2.78348480366266,
87.8323183611622));
#30583=CARTESIAN_POINT('Ctrl Pts',(-6.09708934351528,-2.9406680571984,87.8404623033024));
#30584=CARTESIAN_POINT('Ctrl Pts',(-6.02004563327546,-3.09535582767633,
87.8486062454426));
#30585=CARTESIAN_POINT('Ctrl Pts',(-5.93709108849273,-3.24703532579186,
87.8567501875828));
#30586=CARTESIAN_POINT('Ctrl Pts',(-5.85422031115392,-3.3985616580515,87.8648859059757));
#30587=CARTESIAN_POINT('Ctrl Pts',(-5.7654507560255,-3.54708544711929,87.8730216243686));
#30588=CARTESIAN_POINT('Ctrl Pts',(-5.67103007503556,-3.69211414883698,
87.8811573427614));
#30589=CARTESIAN_POINT('Ctrl Pts',(-5.57668487857314,-3.837026907491,87.8892865570617));
#30590=CARTESIAN_POINT('Ctrl Pts',(-5.47669775020504,-3.97844983723052,
87.8974157713619));
#30591=CARTESIAN_POINT('Ctrl Pts',(-5.37136206363486,-4.11591527868885,
87.9055449856621));
#30592=CARTESIAN_POINT('Ctrl Pts',(-5.26608843944813,-4.2532997273401,87.9136694103375));
#30593=CARTESIAN_POINT('Ctrl Pts',(-5.15547275458676,-4.38673104168613,
87.9217938350129));
#30594=CARTESIAN_POINT('Ctrl Pts',(-5.03985145501215,-4.51577084354509,
87.9299182596883));
#30595=CARTESIAN_POINT('Ctrl Pts',(-4.92352826013205,-4.6455939996085,87.9380920048226));
#30596=CARTESIAN_POINT('Ctrl Pts',(-4.80213868188773,-4.77097183557626,
87.9462657499568));
#30597=CARTESIAN_POINT('Ctrl Pts',(-4.67606661960873,-4.89149158938058,
87.954439495091));
#30598=CARTESIAN_POINT('Ctrl Pts',(-4.55080188592547,-5.01123956994793,
87.9625608979531));
#30599=CARTESIAN_POINT('Ctrl Pts',(-4.42091474696742,-5.12619126677077,
87.9706823008152));
#30600=CARTESIAN_POINT('Ctrl Pts',(-4.28681860625293,-5.23597891870123,
87.9788037036774));
#30601=CARTESIAN_POINT('Ctrl Pts',(-4.15271209793107,-5.34577505883473,
87.9869257344436));
#30602=CARTESIAN_POINT('Ctrl Pts',(-4.01439622280726,-5.45040612690525,
87.9950477652099));
#30603=CARTESIAN_POINT('Ctrl Pts',(-3.87231710880319,-5.5495449551175,88.0031697959761));
#30604=CARTESIAN_POINT('Ctrl Pts',(-3.73019995484619,-5.64871032654397,
88.0112940013172));
#30605=CARTESIAN_POINT('Ctrl Pts',(-3.58431785579056,-5.74238032078009,
88.0194182066583));
#30606=CARTESIAN_POINT('Ctrl Pts',(-3.43514547672217,-5.83027139623493,
88.0275424119994));
#30607=CARTESIAN_POINT('Ctrl Pts',(-3.28435840986844,-5.91911383176637,
88.0357545562419));
#30608=CARTESIAN_POINT('Ctrl Pts',(-3.13020974698006,-6.00205131654749,
88.0439667004844));
#30609=CARTESIAN_POINT('Ctrl Pts',(-2.9732139894315,-6.07883932778691,88.0521788447269));
#30610=CARTESIAN_POINT('Ctrl Pts',(-2.81765143011832,-6.15492634911473,
88.0603160211433));
#30611=CARTESIAN_POINT('Ctrl Pts',(-2.65929390137479,-6.22497561527429,
88.0684531975598));
#30612=CARTESIAN_POINT('Ctrl Pts',(-2.4986604103372,-6.28879838711765,88.0765903739762));
#30613=CARTESIAN_POINT('Ctrl Pts',(-2.33580704418711,-6.35350315798818,
88.0848400021317));
#30614=CARTESIAN_POINT('Ctrl Pts',(-2.17061471981748,-6.41180794955711,
88.0930896302872));
#30615=CARTESIAN_POINT('Ctrl Pts',(-2.00363795570425,-6.46356897870374,
88.1013392584427));
#30616=CARTESIAN_POINT('Ctrl Pts',(-1.83666119159103,-6.51533000785037,
88.1095888865982));
#30617=CARTESIAN_POINT('Ctrl Pts',(-1.66790037577361,-6.56054723609679,
88.1178385147536));
#30618=CARTESIAN_POINT('Ctrl Pts',(-1.49791805174984,-6.59913104205713,
88.1260881429091));
#30619=CARTESIAN_POINT('Ctrl Pts',(-1.32844591357875,-6.63759904237675,
88.1343130105867));
#30620=CARTESIAN_POINT('Ctrl Pts',(-1.15725305690841,-6.66958853701086,
88.1425378782643));
#30621=CARTESIAN_POINT('Ctrl Pts',(-0.984875954207333,-6.69494647886181,
88.1507627459419));
#30622=CARTESIAN_POINT('Ctrl Pts',(-0.81269305360654,-6.72027585215297,
88.1589783473854));
#30623=CARTESIAN_POINT('Ctrl Pts',(-0.639328915393011,-6.7389884979571,
88.167193948829));
#30624=CARTESIAN_POINT('Ctrl Pts',(-0.465332937994383,-6.75098172540983,
88.1754095502725));
#30625=CARTESIAN_POINT('Ctrl Pts',(-0.291498027256431,-6.76296385082949,
88.1836175466006));
#30626=CARTESIAN_POINT('Ctrl Pts',(-0.117032797816354,-6.76823892085928,
88.1918255429288));
#30627=CARTESIAN_POINT('Ctrl Pts',(0.0575053513952854,-6.76675565796201,
88.2000335392569));
#30628=CARTESIAN_POINT('Ctrl Pts',(0.231916988957002,-6.76527347018808,
88.2082355861284));
#30629=CARTESIAN_POINT('Ctrl Pts',(0.406401083709792,-6.75704270978331,
88.2164376329998));
#30630=CARTESIAN_POINT('Ctrl Pts',(0.580397242535718,-6.74206407866737,
88.2246396798713));
#30631=CARTESIAN_POINT('Ctrl Pts',(0.754302222551982,-6.72709329676928,
88.2328374286428));
#30632=CARTESIAN_POINT('Ctrl Pts',(0.927719419418191,-6.70538171927751,
88.2410351774144));
#30633=CARTESIAN_POINT('Ctrl Pts',(1.10009048385972,-6.67698209727429,88.249232926186));
#30634=CARTESIAN_POINT('Ctrl Pts',(1.27242867198254,-6.64858789192859,88.2574291114016));
#30635=CARTESIAN_POINT('Ctrl Pts',(1.44372077046563,-6.61350823505483,88.2656252966172));
#30636=CARTESIAN_POINT('Ctrl Pts',(1.6134152756098,-6.57184754452117,88.2738214818329));
#30637=CARTESIAN_POINT('Ctrl Pts',(1.78309722713759,-6.53018993595135,88.2820170607132));
#30638=CARTESIAN_POINT('Ctrl Pts',(1.95118147200846,-6.48195234798002,88.2902126395935));
#30639=CARTESIAN_POINT('Ctrl Pts',(2.11712845311619,-6.42728995090512,88.2984082184739));
#30640=CARTESIAN_POINT('Ctrl Pts',(2.28309334992864,-6.37262165245521,88.3066046821523));
#30641=CARTESIAN_POINT('Ctrl Pts',(2.44692018238773,-6.31152727527567,88.3148011458308));
#30642=CARTESIAN_POINT('Ctrl Pts',(2.608086216873,-6.24421134214379,88.3229976095092));
#30643=CARTESIAN_POINT('Ctrl Pts',(2.76929897328441,-6.17687589416768,88.331196449337));
#30644=CARTESIAN_POINT('Ctrl Pts',(2.92784906423909,-6.10331543591301,88.3393952891648));
#30645=CARTESIAN_POINT('Ctrl Pts',(3.08323529220617,-6.02378196259579,88.3475941289926));
#30646=CARTESIAN_POINT('Ctrl Pts',(3.23878382550873,-5.94416541430314,88.3558015327418));
#30647=CARTESIAN_POINT('Ctrl Pts',(3.39116157352667,-5.85856354998363,88.364008936491));
#30648=CARTESIAN_POINT('Ctrl Pts',(3.53989256732983,-5.7672740191327,88.3722163402403));
#30649=CARTESIAN_POINT('Ctrl Pts',(3.68870322932408,-5.67593558877802,88.3804281403093));
#30650=CARTESIAN_POINT('Ctrl Pts',(3.83386294492437,-5.57890361760862,88.3886399403783));
#30651=CARTESIAN_POINT('Ctrl Pts',(3.97492625272948,-5.47651808043779,88.3968517404473));
#30652=CARTESIAN_POINT('Ctrl Pts',(4.11619722543429,-5.37398181745003,88.4050756294335));
#30653=CARTESIAN_POINT('Ctrl Pts',(4.25335945656462,-5.26607645997574,88.4132995184196));
#30654=CARTESIAN_POINT('Ctrl Pts',(4.38600100006403,-5.15318195171074,88.4215234074058));
#30655=CARTESIAN_POINT('Ctrl Pts',(4.50855949317275,-5.04886937777519,88.4291221386558));
#30656=CARTESIAN_POINT('Ctrl Pts',(4.62725871104192,-4.94029791892675,88.4367208699058));
#30657=CARTESIAN_POINT('Ctrl Pts',(4.74180331890803,-4.82779352135039,88.4443196011557));
#30658=CARTESIAN_POINT('Ctrl Pts',(4.86578612535438,-4.70601903358597,88.4525444494778));
#30659=CARTESIAN_POINT('Ctrl Pts',(4.9852489806452,-4.5792945540232,88.4607692977998));
#30660=CARTESIAN_POINT('Ctrl Pts',(5.09977311128348,-4.44798867055999,88.4689941461218));
#30661=CARTESIAN_POINT('Ctrl Pts',(5.21416826235842,-4.31683066663464,88.477209731441));
#30662=CARTESIAN_POINT('Ctrl Pts',(5.32363553066573,-4.18110180095576,88.4854253167602));
#30663=CARTESIAN_POINT('Ctrl Pts',(5.42779151894399,-4.04120875814152,88.4936409020794));
#30664=CARTESIAN_POINT('Ctrl Pts',(5.53185113149757,-3.90144515861328,88.5018488855027));
#30665=CARTESIAN_POINT('Ctrl Pts',(5.63060903851758,-3.75752534147557,88.5100568689259));
#30666=CARTESIAN_POINT('Ctrl Pts',(5.72372077095539,-3.60989051580983,88.5182648523491));
#30667=CARTESIAN_POINT('Ctrl Pts',(5.81676504890371,-3.46236264370985,88.5264668895257));
#30668=CARTESIAN_POINT('Ctrl Pts',(5.90417110886795,-3.31112542592446,88.5346689267022));
#30669=CARTESIAN_POINT('Ctrl Pts',(5.98563659266067,-3.15665069030476,88.5428709638787));
#30670=CARTESIAN_POINT('Ctrl Pts',(6.06705941804239,-3.00225684350394,88.5510687061581));
#30671=CARTESIAN_POINT('Ctrl Pts',(6.14254769732389,-2.844629172746,88.5592664484375));
#30672=CARTESIAN_POINT('Ctrl Pts',(6.21184396533849,-2.68426592391436,88.5674641907169));
#30673=CARTESIAN_POINT('Ctrl Pts',(6.28112705781444,-2.5239331655008,88.5756603743312));
#30674=CARTESIAN_POINT('Ctrl Pts',(6.34422033618203,-2.36086619156955,88.5838565579456));
#30675=CARTESIAN_POINT('Ctrl Pts',(6.40091350225666,-2.19558542002547,88.59205274156));
#30676=CARTESIAN_POINT('Ctrl Pts',(6.45760249492325,-2.03031681545225,88.6002483218208));
#30677=CARTESIAN_POINT('Ctrl Pts',(6.5078921963106,-1.86283507694031,88.6084439020817));
#30678=CARTESIAN_POINT('Ctrl Pts',(6.55162146372919,-1.69367800836019,88.6166394823426));
#30679=CARTESIAN_POINT('Ctrl Pts',(6.59535546808648,-1.52450261597294,88.6248359503833));
#30680=CARTESIAN_POINT('Ctrl Pts',(6.63252753280762,-1.35365187943672,88.633032418424));
#30681=CARTESIAN_POINT('Ctrl Pts',(6.66302712934105,-1.18167612892247,88.6412288864647));
#30682=CARTESIAN_POINT('Ctrl Pts',(6.69353557878362,-1.00965046018414,88.6494277336381));
#30683=CARTESIAN_POINT('Ctrl Pts',(6.71736763959185,-0.836499480249944,
88.6576265808115));
#30684=CARTESIAN_POINT('Ctrl Pts',(6.73446436328804,-0.662781064608349,
88.6658254279849));
#30685=CARTESIAN_POINT('Ctrl Pts',(6.75157895472304,-0.48888109632954,88.6740328437509));
#30686=CARTESIAN_POINT('Ctrl Pts',(6.76194411068771,-0.314412865139171,
88.6822402595168));
#30687=CARTESIAN_POINT('Ctrl Pts',(6.76555292931201,-0.139937702845619,
88.6904476752827));
#30688=CARTESIAN_POINT('Ctrl Pts',(6.76916368213616,0.0346309719982851,
88.6986594899349));
#30689=CARTESIAN_POINT('Ctrl Pts',(6.76601088522337,0.209206226919585,88.706871304587));
#30690=CARTESIAN_POINT('Ctrl Pts',(6.75613973648387,0.3832295149173,88.7150831192392));
#30691=CARTESIAN_POINT('Ctrl Pts',(6.7462540509772,0.557509078662265,88.7233070270368));
#30692=CARTESIAN_POINT('Ctrl Pts',(6.72963027535547,0.731234693812542,88.7315309348344));
#30693=CARTESIAN_POINT('Ctrl Pts',(6.70636535089734,0.903854402148699,88.739754842632));
#30694=CARTESIAN_POINT('Ctrl Pts',(6.6848689903614,1.06335182466049,88.7473535815555));
#30695=CARTESIAN_POINT('Ctrl Pts',(6.65770341198288,1.22190497617399,88.7549523204789));
#30696=CARTESIAN_POINT('Ctrl Pts',(6.62498316933598,1.37908919436523,88.7625510594024));
#30697=CARTESIAN_POINT('Ctrl Pts',(6.58988221675236,1.54771006460649,88.7707026791055));
#30698=CARTESIAN_POINT('Ctrl Pts',(6.54828423870661,1.7152548674017,88.7788542988085));
#30699=CARTESIAN_POINT('Ctrl Pts',(6.50026562115968,1.88117937857333,88.7870059185115));
#30700=CARTESIAN_POINT('Ctrl Pts',(6.45230358230907,2.0469083865629,88.7951479334396));
#30701=CARTESIAN_POINT('Ctrl Pts',(6.3979360646495,2.21102055561252,88.8032899483676));
#30702=CARTESIAN_POINT('Ctrl Pts',(6.33729074034879,2.37298020899658,88.8114319632957));
#30703=CARTESIAN_POINT('Ctrl Pts',(6.27670410897857,2.53478311679824,88.8195660983299));
#30704=CARTESIAN_POINT('Ctrl Pts',(6.20985189507299,2.69443731640079,88.8277002333642));
#30705=CARTESIAN_POINT('Ctrl Pts',(6.13691200674627,2.85142070229096,88.8358343683984));
#30706=CARTESIAN_POINT('Ctrl Pts',(6.0640273681515,3.00828517807325,88.8439623420744));
#30707=CARTESIAN_POINT('Ctrl Pts',(5.98506439115894,3.1624825384342,88.8520903157505));
#30708=CARTESIAN_POINT('Ctrl Pts',(5.90024966940371,3.3135091426917,88.8602182894265));
#30709=CARTESIAN_POINT('Ctrl Pts',(5.8154800593316,3.46445541815515,88.8683419399548));
#30710=CARTESIAN_POINT('Ctrl Pts',(5.72486508178144,3.61223397800653,88.8764655904831));
#30711=CARTESIAN_POINT('Ctrl Pts',(5.62867799410391,3.75636433785255,88.8845892410114));
#30712=CARTESIAN_POINT('Ctrl Pts',(5.53251724504356,3.90045523092123,88.8927106670652));
#30713=CARTESIAN_POINT('Ctrl Pts',(5.4307876259904,4.04089960855886,88.900832093119));
#30714=CARTESIAN_POINT('Ctrl Pts',(5.32380661113034,4.17724456637206,88.9089535191728));
#30715=CARTESIAN_POINT('Ctrl Pts',(5.21683452069907,4.31357815019644,88.9170742677317));
#30716=CARTESIAN_POINT('Ctrl Pts',(5.10461213274398,4.44581270751718,88.9251950162907));
#30717=CARTESIAN_POINT('Ctrl Pts',(4.98749819833177,4.57352716419586,88.9333157648496));
#30718=CARTESIAN_POINT('Ctrl Pts',(4.87037173414231,4.7012552847797,88.9414373822306));
#30719=CARTESIAN_POINT('Ctrl Pts',(4.7483529294541,4.82446207291372,88.9495589996116));
#30720=CARTESIAN_POINT('Ctrl Pts',(4.62183845456009,4.94276221357548,88.9576806169926));
#30721=CARTESIAN_POINT('Ctrl Pts',(4.49523238084849,5.06114800572506,88.9658081145747));
#30722=CARTESIAN_POINT('Ctrl Pts',(4.3641244028324,5.17461980434966,88.9739356121568));
#30723=CARTESIAN_POINT('Ctrl Pts',(4.22894592839778,5.2828311855186,88.9820631097388));
#30724=CARTESIAN_POINT('Ctrl Pts',(4.09371401733998,5.3910853431046,88.9901938201551));
#30725=CARTESIAN_POINT('Ctrl Pts',(3.95440869625667,5.49407472060417,88.9983245305714));
#30726=CARTESIAN_POINT('Ctrl Pts',(3.81149139010395,5.59149554083373,89.0064552409876));
#30727=CARTESIAN_POINT('Ctrl Pts',(3.66841558133587,5.6890244057446,89.0145949687783));
#30728=CARTESIAN_POINT('Ctrl Pts',(3.52172009509385,5.78097218249617,89.022734696569));
#30729=CARTESIAN_POINT('Ctrl Pts',(3.37189273683585,5.86708005495695,89.0308744243598));
#30730=CARTESIAN_POINT('Ctrl Pts',(3.28207589654922,5.91869904576178,89.035753937951));
#30731=CARTESIAN_POINT('Ctrl Pts',(3.19113403238152,5.968220287335,89.0406334515422));
#30732=CARTESIAN_POINT('Ctrl Pts',(3.09917575053266,6.01559628526635,89.0455129651334));
#30733=CARTESIAN_POINT('Ctrl Pts',(3.09917575053243,6.01559628526647,87.0457515827423));
#30734=CARTESIAN_POINT('Ctrl Pts',(2.93382384459255,6.10078395293764,87.0545010306547));
#30735=CARTESIAN_POINT('Ctrl Pts',(2.76495772122979,6.17915010267051,87.0632504785671));
#30736=CARTESIAN_POINT('Ctrl Pts',(2.59315093316712,6.25042856433177,87.0719999264795));
#30737=CARTESIAN_POINT('Ctrl Pts',(2.42134553245623,6.32170645041449,87.0807493037395));
#30738=CARTESIAN_POINT('Ctrl Pts',(2.24659977927601,6.38589665313454,87.0894986809995));
#30739=CARTESIAN_POINT('Ctrl Pts',(2.06950718689934,6.4427811543907,87.0982480582595));
#30740=CARTESIAN_POINT('Ctrl Pts',(1.89241596572869,6.49966521519722,87.1069973677741));
#30741=CARTESIAN_POINT('Ctrl Pts',(1.71297821457197,6.54924360009546,87.1157466772888));
#30742=CARTESIAN_POINT('Ctrl Pts',(1.53180337335836,6.59134792173558,87.1244959868035));
#30743=CARTESIAN_POINT('Ctrl Pts',(1.35062987477773,6.63345193135307,87.1332452314796));
#30744=CARTESIAN_POINT('Ctrl Pts',(1.16771959102941,6.6680819236824,87.1419944761557));
#30745=CARTESIAN_POINT('Ctrl Pts',(0.983693746906729,6.6951202836317,87.1507437208318));
#30746=CARTESIAN_POINT('Ctrl Pts',(0.799669205419738,6.72215845218869,87.159492903576));
#30747=CARTESIAN_POINT('Ctrl Pts',(0.614529402873325,6.74160505424581,87.1682420863202));
#30748=CARTESIAN_POINT('Ctrl Pts',(0.42890312736308,6.75339404354123,87.1769912690644));
#30749=CARTESIAN_POINT('Ctrl Pts',(0.243278104163717,6.76518295330331,87.185740392783));
#30750=CARTESIAN_POINT('Ctrl Pts',(0.0571669005389611,6.76931433552276,
87.1944895165016));
#30751=CARTESIAN_POINT('Ctrl Pts',(-0.128798404777663,6.76577415902473,
87.2032386402202));
#30752=CARTESIAN_POINT('Ctrl Pts',(-0.314762517259356,6.7622340052344,87.2119877078194));
#30753=CARTESIAN_POINT('Ctrl Pts',(-0.500580446819875,6.75102239665086,
87.2207367754186));
#30754=CARTESIAN_POINT('Ctrl Pts',(-0.685621118843082,6.73217741012493,
87.2294858430178));
#30755=CARTESIAN_POINT('Ctrl Pts',(-0.870660665414926,6.71333253821766,
87.2382348574036));
#30756=CARTESIAN_POINT('Ctrl Pts',(-1.05492267885527,6.68685441030606,87.2469838717894));
#30757=CARTESIAN_POINT('Ctrl Pts',(-1.23778137635289,6.6528329502817,87.2557328861752));
#30758=CARTESIAN_POINT('Ctrl Pts',(-1.42999922978883,6.61707018861857,87.2649296965426));
#30759=CARTESIAN_POINT('Ctrl Pts',(-1.6206660123373,6.57297172934404,87.2741265069099));
#30760=CARTESIAN_POINT('Ctrl Pts',(-1.80906628500419,6.52070304311285,87.2833233172773));
#30761=CARTESIAN_POINT('Ctrl Pts',(-1.98831342545562,6.4709737491502,87.2920733150151));
#30762=CARTESIAN_POINT('Ctrl Pts',(-2.16550875896737,6.41384933989517,87.3008233127529));
#30763=CARTESIAN_POINT('Ctrl Pts',(-2.34005036714048,6.34952386240462,87.3095733104906));
#30764=CARTESIAN_POINT('Ctrl Pts',(-2.51458843547125,6.28519968948581,87.3183231307715));
#30765=CARTESIAN_POINT('Ctrl Pts',(-2.68647261718091,6.21367483971083,87.3270729510524));
#30766=CARTESIAN_POINT('Ctrl Pts',(-2.85511905908767,6.13519226743827,87.3358227713332));
#30767=CARTESIAN_POINT('Ctrl Pts',(-3.02376230488914,6.05671118252922,87.3445724257918));
#30768=CARTESIAN_POINT('Ctrl Pts',(-3.18916767379929,5.9712727599262,87.3533220802503));
#30769=CARTESIAN_POINT('Ctrl Pts',(-3.35077334102807,5.87916720437986,87.3620717347088));
#30770=CARTESIAN_POINT('Ctrl Pts',(-3.51237616037396,5.78706327195626,87.3708212349773));
#30771=CARTESIAN_POINT('Ctrl Pts',(-3.67017916302336,5.68829258362275,87.3795707352457));
#30772=CARTESIAN_POINT('Ctrl Pts',(-3.82364636566507,5.58319061741011,87.3883202355142));
#30773=CARTESIAN_POINT('Ctrl Pts',(-3.97711106778838,5.47809036367673,87.3970695932226));
#30774=CARTESIAN_POINT('Ctrl Pts',(-4.12623987481963,5.36665920043197,87.405818950931));
#30775=CARTESIAN_POINT('Ctrl Pts',(-4.27052628213961,5.24927559512309,87.4145683086395));
#30776=CARTESIAN_POINT('Ctrl Pts',(-4.41481053025006,5.13189374643012,87.423317535416));
#30777=CARTESIAN_POINT('Ctrl Pts',(-4.55425230136554,5.00855981477331,87.4320667621925));
#30778=CARTESIAN_POINT('Ctrl Pts',(-4.68837800630569,4.87969268192057,87.440815988969));
#30779=CARTESIAN_POINT('Ctrl Pts',(-4.82250188228921,4.75082730631783,87.4495650964399));
#30780=CARTESIAN_POINT('Ctrl Pts',(-4.95130963052998,4.61642907903491,87.4583142039107));
#30781=CARTESIAN_POINT('Ctrl Pts',(-5.07436379033404,4.47695444731647,87.4670633113816));
#30782=CARTESIAN_POINT('Ctrl Pts',(-5.19741643562824,4.33748153220563,87.4758123111713));
#30783=CARTESIAN_POINT('Ctrl Pts',(-5.31471544462775,4.19293255254586,87.484561310961));
#30784=CARTESIAN_POINT('Ctrl Pts',(-5.42586245275613,4.04379841779622,87.4933103107508));
#30785=CARTESIAN_POINT('Ctrl Pts',(-5.53702160019141,3.8946479948436,87.5020602660929));
#30786=CARTESIAN_POINT('Ctrl Pts',(-5.64202723081242,3.74091164443865,87.5108102214351));
#30787=CARTESIAN_POINT('Ctrl Pts',(-5.74052265232959,3.58311159163245,87.5195601767772));
#30788=CARTESIAN_POINT('Ctrl Pts',(-5.83901427066911,3.42531763191796,87.5283097942597));
#30789=CARTESIAN_POINT('Ctrl Pts',(-5.93099603115732,3.26346052695626,87.5370594117421));
#30790=CARTESIAN_POINT('Ctrl Pts',(-6.01615550622747,3.0980900446709,87.5458090292246));
#30791=CARTESIAN_POINT('Ctrl Pts',(-6.10131214578789,2.93272506863849,87.5545583553757));
#30792=CARTESIAN_POINT('Ctrl Pts',(-6.17964682328735,2.76384720416922,87.5633076815268));
#30793=CARTESIAN_POINT('Ctrl Pts',(-6.25089348288549,2.59203002791629,87.5720570076779));
#30794=CARTESIAN_POINT('Ctrl Pts',(-6.32213814889317,2.42021765937065,87.5808060890094));
#30795=CARTESIAN_POINT('Ctrl Pts',(-6.38629508412572,2.24546640831953,87.589555170341));
#30796=CARTESIAN_POINT('Ctrl Pts',(-6.443146398198,2.06836976660077,87.5983042516726));
#30797=CARTESIAN_POINT('Ctrl Pts',(-6.50000285283693,1.89125711158301,87.607054124107));
#30798=CARTESIAN_POINT('Ctrl Pts',(-6.54955227673245,1.71179891440271,87.6158039965413));
#30799=CARTESIAN_POINT('Ctrl Pts',(-6.59162635926384,1.53060476278437,87.6245538689758));
#30800=CARTESIAN_POINT('Ctrl Pts',(-6.63369752055196,1.349423191647,87.6333031338983));
#30801=CARTESIAN_POINT('Ctrl Pts',(-6.66829431424254,1.16650618642705,87.6420523988208));
#30802=CARTESIAN_POINT('Ctrl Pts',(-6.69529923745417,0.982474997618545,
87.6508016637433));
#30803=CARTESIAN_POINT('Ctrl Pts',(-6.72230554731443,0.798434359177744,
87.659551377923));
#30804=CARTESIAN_POINT('Ctrl Pts',(-6.74171916496703,0.613279706240354,
87.6683010921027));
#30805=CARTESIAN_POINT('Ctrl Pts',(-6.75347414817275,0.42763995365541,87.6770508062824));
#30806=CARTESIAN_POINT('Ctrl Pts',(-6.76248837758737,0.285283364199755,
87.6837604654582));
#30807=CARTESIAN_POINT('Ctrl Pts',(-6.76699999999989,0.142641701107454,
87.6904701246341));
#30808=CARTESIAN_POINT('Ctrl Pts',(-6.767,5.05731187567021E-12,87.6971797838099));
#30809=CARTESIAN_POINT('',(-6.76192617641306,-0.00322362460917852,87.3028202161898));
#30810=CARTESIAN_POINT('Ctrl Pts',(3.09917575053262,6.01559628526637,86.6513920151221));
#30811=CARTESIAN_POINT('Ctrl Pts',(2.93382384459274,6.10078395293755,86.6601414630345));
#30812=CARTESIAN_POINT('Ctrl Pts',(2.76495772122998,6.17915010267042,86.6688909109469));
#30813=CARTESIAN_POINT('Ctrl Pts',(2.59315093316732,6.25042856433169,86.6776403588593));
#30814=CARTESIAN_POINT('Ctrl Pts',(2.4213455324563,6.32170645041446,86.6863897361193));
#30815=CARTESIAN_POINT('Ctrl Pts',(2.24659977927596,6.38589665313456,86.6951391133793));
#30816=CARTESIAN_POINT('Ctrl Pts',(2.06950718689917,6.44278115439076,86.7038884906393));
#30817=CARTESIAN_POINT('Ctrl Pts',(1.89241596572852,6.49966521519727,86.712637800154));
#30818=CARTESIAN_POINT('Ctrl Pts',(1.7129782145718,6.54924360009551,86.7213871096686));
#30819=CARTESIAN_POINT('Ctrl Pts',(1.53180337335819,6.59134792173562,86.7301364191833));
#30820=CARTESIAN_POINT('Ctrl Pts',(1.35062987477756,6.6334519313531,86.7388856638594));
#30821=CARTESIAN_POINT('Ctrl Pts',(1.16771959102924,6.66808192368243,86.7476349085355));
#30822=CARTESIAN_POINT('Ctrl Pts',(0.983693746906558,6.69512028363173,86.7563841532116));
#30823=CARTESIAN_POINT('Ctrl Pts',(0.799669205419693,6.72215845218869,86.7651333359558));
#30824=CARTESIAN_POINT('Ctrl Pts',(0.61452940287341,6.74160505424579,86.7738825187));
#30825=CARTESIAN_POINT('Ctrl Pts',(0.428903127363293,6.75339404354122,86.7826317014442));
#30826=CARTESIAN_POINT('Ctrl Pts',(0.243278104164058,6.76518295330329,86.7913808251628));
#30827=CARTESIAN_POINT('Ctrl Pts',(0.0571669005394312,6.76931433552275,
86.8001299488814));
#30828=CARTESIAN_POINT('Ctrl Pts',(-0.128798404777065,6.76577415902474,
86.8088790726));
#30829=CARTESIAN_POINT('Ctrl Pts',(-0.314762517258374,6.76223400523444,
86.8176281401992));
#30830=CARTESIAN_POINT('Ctrl Pts',(-0.50058044681851,6.75102239665096,86.8263772077984));
#30831=CARTESIAN_POINT('Ctrl Pts',(-0.685621118841339,6.73217741012511,
86.8351262753976));
#30832=CARTESIAN_POINT('Ctrl Pts',(-0.870660665413061,6.7133325382179,86.8438752897833));
#30833=CARTESIAN_POINT('Ctrl Pts',(-1.05492267885329,6.68685441030637,86.8526243041691));
#30834=CARTESIAN_POINT('Ctrl Pts',(-1.23778137635079,6.65283295028209,86.8613733185549));
#30835=CARTESIAN_POINT('Ctrl Pts',(-1.42999922978674,6.61707018861903,86.8705701289223));
#30836=CARTESIAN_POINT('Ctrl Pts',(-1.62066601233522,6.57297172934456,86.8797669392896));
#30837=CARTESIAN_POINT('Ctrl Pts',(-1.80906628500213,6.52070304311342,86.888963749657));
#30838=CARTESIAN_POINT('Ctrl Pts',(-1.98831342545345,6.47097374915086,86.8977137473948));
#30839=CARTESIAN_POINT('Ctrl Pts',(-2.16550875896511,6.41384933989593,86.9064637451326));
#30840=CARTESIAN_POINT('Ctrl Pts',(-2.34005036713811,6.34952386240549,86.9152137428703));
#30841=CARTESIAN_POINT('Ctrl Pts',(-2.51458843546891,6.28519968948675,86.9239635631512));
#30842=CARTESIAN_POINT('Ctrl Pts',(-2.6864726171786,6.21367483971184,86.932713383432));
#30843=CARTESIAN_POINT('Ctrl Pts',(-2.85511905908539,6.13519226743933,86.9414632037129));
#30844=CARTESIAN_POINT('Ctrl Pts',(-3.02376230488701,6.05671118253029,86.9502128581715));
#30845=CARTESIAN_POINT('Ctrl Pts',(-3.1891676737973,5.97127275992727,86.95896251263));
#30846=CARTESIAN_POINT('Ctrl Pts',(-3.35077334102621,5.87916720438091,86.9677121670885));
#30847=CARTESIAN_POINT('Ctrl Pts',(-3.51237616037203,5.78706327195743,86.976461667357));
#30848=CARTESIAN_POINT('Ctrl Pts',(-3.67017916302135,5.68829258362404,86.9852111676254));
#30849=CARTESIAN_POINT('Ctrl Pts',(-3.82364636566299,5.58319061741154,86.9939606678938));
#30850=CARTESIAN_POINT('Ctrl Pts',(-3.97711106778634,5.47809036367821,87.0027100256023));
#30851=CARTESIAN_POINT('Ctrl Pts',(-4.12623987481763,5.36665920043351,87.0114593833107));
#30852=CARTESIAN_POINT('Ctrl Pts',(-4.27052628213765,5.24927559512468,87.0202087410192));
#30853=CARTESIAN_POINT('Ctrl Pts',(-4.41481053024835,5.1318937464316,87.0289579677957));
#30854=CARTESIAN_POINT('Ctrl Pts',(-4.55425230136406,5.00855981477467,87.0377071945722));
#30855=CARTESIAN_POINT('Ctrl Pts',(-4.68837800630443,4.87969268192178,87.0464564213487));
#30856=CARTESIAN_POINT('Ctrl Pts',(-4.82250188228808,4.75082730631899,87.0552055288196));
#30857=CARTESIAN_POINT('Ctrl Pts',(-4.95130963052897,4.61642907903601,87.0639546362904));
#30858=CARTESIAN_POINT('Ctrl Pts',(-5.07436379033314,4.4769544473175,87.0727037437613));
#30859=CARTESIAN_POINT('Ctrl Pts',(-5.19741643562762,4.33748153220639,87.081452743551));
#30860=CARTESIAN_POINT('Ctrl Pts',(-5.31471544462738,4.19293255254634,87.0902017433408));
#30861=CARTESIAN_POINT('Ctrl Pts',(-5.42586245275601,4.04379841779639,87.0989507431305));
#30862=CARTESIAN_POINT('Ctrl Pts',(-5.53702160019121,3.89464799484387,87.1077006984727));
#30863=CARTESIAN_POINT('Ctrl Pts',(-5.64202723081216,3.74091164443904,87.1164506538148));
#30864=CARTESIAN_POINT('Ctrl Pts',(-5.74052265232928,3.58311159163296,87.125200609157));
#30865=CARTESIAN_POINT('Ctrl Pts',(-5.83901427066881,3.42531763191847,87.1339502266394));
#30866=CARTESIAN_POINT('Ctrl Pts',(-5.93099603115704,3.26346052695678,87.1426998441219));
#30867=CARTESIAN_POINT('Ctrl Pts',(-6.0161555062272,3.09809004467143,87.1514494616043));
#30868=CARTESIAN_POINT('Ctrl Pts',(-6.10131214578775,2.93272506863879,87.1601987877554));
#30869=CARTESIAN_POINT('Ctrl Pts',(-6.17964682328732,2.76384720416931,87.1689481139066));
#30870=CARTESIAN_POINT('Ctrl Pts',(-6.25089348288555,2.59203002791614,87.1776974400577));
#30871=CARTESIAN_POINT('Ctrl Pts',(-6.32213814889313,2.42021765937072,87.1864465213892));
#30872=CARTESIAN_POINT('Ctrl Pts',(-6.38629508412561,2.24546640831985,87.1951956027208));
#30873=CARTESIAN_POINT('Ctrl Pts',(-6.44314639819782,2.06836976660133,87.2039446840523));
#30874=CARTESIAN_POINT('Ctrl Pts',(-6.50000285283673,1.89125711158371,87.2126945564867));
#30875=CARTESIAN_POINT('Ctrl Pts',(-6.54955227673223,1.71179891440353,87.2214444289211));
#30876=CARTESIAN_POINT('Ctrl Pts',(-6.59162635926361,1.53060476278533,87.2301943013555));
#30877=CARTESIAN_POINT('Ctrl Pts',(-6.63369752055176,1.34942319164796,87.238943566278));
#30878=CARTESIAN_POINT('Ctrl Pts',(-6.66829431424237,1.16650618642802,87.2476928312005));
#30879=CARTESIAN_POINT('Ctrl Pts',(-6.69529923745403,0.982474997619514,
87.256442096123));
#30880=CARTESIAN_POINT('Ctrl Pts',(-6.72230554731432,0.798434359178717,
87.2651918103027));
#30881=CARTESIAN_POINT('Ctrl Pts',(-6.74171916496694,0.613279706241331,
87.2739415244824));
#30882=CARTESIAN_POINT('Ctrl Pts',(-6.75347414817269,0.427639953656388,
87.2826912386621));
#30883=CARTESIAN_POINT('Ctrl Pts',(-6.76248837758735,0.28528336420035,87.289400897838));
#30884=CARTESIAN_POINT('Ctrl Pts',(-6.7669999999999,0.142641701107664,87.2961105570138));
#30885=CARTESIAN_POINT('Ctrl Pts',(-6.767,4.88301307805299E-12,87.3028202161897));
#30886=CARTESIAN_POINT('Ctrl Pts',(-6.75952464934065,-0.00474942101288033,
87.3028202161898));
#30887=CARTESIAN_POINT('Ctrl Pts',(-6.76474205737662,-0.664932310615616,
87.3338345898298));
#30888=CARTESIAN_POINT('Ctrl Pts',(-6.52475900416391,-2.44944862935725,
87.4178161533712));
#30889=CARTESIAN_POINT('Ctrl Pts',(-4.9434562315809,-5.00423164848898,87.5547649068138));
#30890=CARTESIAN_POINT('Ctrl Pts',(-0.961442134084449,-7.40213597015891,
87.7666336664189));
#30891=CARTESIAN_POINT('Ctrl Pts',(5.26255964958237,-6.02988092025636,88.0314696159252));
#30892=CARTESIAN_POINT('Ctrl Pts',(7.87321604513668,1.04812428378684,88.3440128912255));
#30893=CARTESIAN_POINT('Ctrl Pts',(4.99392233188169,5.04013769176598,88.5506217867228));
#30894=CARTESIAN_POINT('Ctrl Pts',(3.10355585847744,6.02401335114973,88.6512963024177));
#30895=CARTESIAN_POINT('Origin',(0.,0.,-3.69717978381041));
#30896=CARTESIAN_POINT('',(3.09917575053275,6.01559628526631,91.0459618091817));
#30897=CARTESIAN_POINT('',(3.09917575053247,6.01559628526645,90.6515381108923));
#30898=CARTESIAN_POINT('',(3.09917575053259,6.01559628526639,-3.69717978381041));
#30899=CARTESIAN_POINT('',(-6.76699988295537,-0.00125860319137315,89.6971797837778));
#30900=CARTESIAN_POINT('Ctrl Pts',(-6.76699988295525,-0.00125860387117534,
89.6971797838099));
#30901=CARTESIAN_POINT('Ctrl Pts',(-6.76697355887306,-0.142792461478475,
89.703868333921));
#30902=CARTESIAN_POINT('Ctrl Pts',(-6.76250695607499,-0.284257024204317,
89.710556884032));
#30903=CARTESIAN_POINT('Ctrl Pts',(-6.7536127253551,-0.425445831947712,
89.7172454341431));
#30904=CARTESIAN_POINT('Ctrl Pts',(-6.74267579642089,-0.599060842084828,
89.7254701136619));
#30905=CARTESIAN_POINT('Ctrl Pts',(-6.72502547760636,-0.772482642989311,
89.7336947931806));
#30906=CARTESIAN_POINT('Ctrl Pts',(-6.70066978690113,-0.945152583930449,
89.7419194726994));
#30907=CARTESIAN_POINT('Ctrl Pts',(-6.67633969678227,-1.11764102922893,
89.7501355071496));
#30908=CARTESIAN_POINT('Ctrl Pts',(-6.64531831969244,-1.28937883632884,
89.7583515415997));
#30909=CARTESIAN_POINT('Ctrl Pts',(-6.60766562973601,-1.45980955114203,
89.7665675760498));
#30910=CARTESIAN_POINT('Ctrl Pts',(-6.57004497511633,-1.6300952615651,89.7747766202044));
#30911=CARTESIAN_POINT('Ctrl Pts',(-6.52580432121743,-1.7990757465476,89.782985664359));
#30912=CARTESIAN_POINT('Ctrl Pts',(-6.47505518311067,-1.96620176372407,
89.7911947085136));
#30913=CARTESIAN_POINT('Ctrl Pts',(-6.42433906067716,-2.13321905436489,
89.7993984121416));
#30914=CARTESIAN_POINT('Ctrl Pts',(-6.367122991954,-2.29838393861884,89.8076021157697));
#30915=CARTESIAN_POINT('Ctrl Pts',(-6.30356912565913,-2.46115933617413,
89.8158058193977));
#30916=CARTESIAN_POINT('Ctrl Pts',(-6.2400438815928,-2.62386142592137,89.8240058283917));
#30917=CARTESIAN_POINT('Ctrl Pts',(-6.17018665659501,-2.78417583974394,
89.8322058373856));
#30918=CARTESIAN_POINT('Ctrl Pts',(-6.09420884250469,-2.94158249653781,
89.8404058463796));
#30919=CARTESIAN_POINT('Ctrl Pts',(-6.0182371037608,-3.09897656676307,89.8486051996835));
#30920=CARTESIAN_POINT('Ctrl Pts',(-5.93614589857633,-3.25346301675257,
89.8568045529875));
#30921=CARTESIAN_POINT('Ctrl Pts',(-5.84819413800976,-3.40454318876239,
89.8650039062914));
#30922=CARTESIAN_POINT('Ctrl Pts',(-5.76024295086259,-3.55562237577426,
89.873203206138));
#30923=CARTESIAN_POINT('Ctrl Pts',(-5.66643146387409,-3.70329501865751,
89.8814025059846));
#30924=CARTESIAN_POINT('Ctrl Pts',(-5.56706373077756,-3.84708856376624,
89.8896018058312));
#30925=CARTESIAN_POINT('Ctrl Pts',(-5.46767861924757,-3.99090725694346,
89.8978025396542));
#30926=CARTESIAN_POINT('Ctrl Pts',(-5.36273552941765,-4.13084520576755,
89.9060032734772));
#30927=CARTESIAN_POINT('Ctrl Pts',(-5.25258090816052,-4.26646021934198,
89.9142040073002));
#30928=CARTESIAN_POINT('Ctrl Pts',(-5.14238703860357,-4.40212355280216,
89.9224076630601));
#30929=CARTESIAN_POINT('Ctrl Pts',(-5.02697816451822,-4.53346060460891,
89.9306113188201));
#30930=CARTESIAN_POINT('Ctrl Pts',(-4.90673996530744,-4.66006350953018,
89.9388149745801));
#30931=CARTESIAN_POINT('Ctrl Pts',(-4.78636402550986,-4.78681144621781,
89.9470280281551));
#30932=CARTESIAN_POINT('Ctrl Pts',(-4.6611479550591,-4.90881414094584,89.9552410817301));
#30933=CARTESIAN_POINT('Ctrl Pts',(-4.53151390459832,-5.02570101900542,
89.9634541353051));
#30934=CARTESIAN_POINT('Ctrl Pts',(-4.40180314676163,-5.14265706165303,
89.9716720487282));
#30935=CARTESIAN_POINT('Ctrl Pts',(-4.26766947270954,-5.25449102419909,
89.9798899621513));
#30936=CARTESIAN_POINT('Ctrl Pts',(-4.12956674215047,-5.36087376480036,
89.9881078755744));
#30937=CARTESIAN_POINT('Ctrl Pts',(-3.99124861791615,-5.46742242659224,
89.9963386061704));
#30938=CARTESIAN_POINT('Ctrl Pts',(-3.84894935823525,-5.56850266818713,
90.0045693367663));
#30939=CARTESIAN_POINT('Ctrl Pts',(-3.70315145376962,-5.66382894431355,
90.0128000673623));
#30940=CARTESIAN_POINT('Ctrl Pts',(-3.56925351561354,-5.75137472813128,
90.0203590090382));
#30941=CARTESIAN_POINT('Ctrl Pts',(-3.43240522942697,-5.83406791005637,
90.0279179507141));
#30942=CARTESIAN_POINT('Ctrl Pts',(-3.29299648027131,-5.91172252232129,
90.0354768923899));
#30943=CARTESIAN_POINT('Ctrl Pts',(-3.1426151231373,-5.99548918726047,90.0436307845567));
#30944=CARTESIAN_POINT('Ctrl Pts',(-2.9887890810726,-6.073651259737,90.0517846767234));
#30945=CARTESIAN_POINT('Ctrl Pts',(-2.83197802127408,-6.14590835328844,
90.0599385688901));
#30946=CARTESIAN_POINT('Ctrl Pts',(-2.67535831477922,-6.21807727299817,
90.0680825110304));
#30947=CARTESIAN_POINT('Ctrl Pts',(-2.51576116957472,-6.284355405633,90.0762264531705));
#30948=CARTESIAN_POINT('Ctrl Pts',(-2.35367362196189,-6.34448654197334,
90.0843703953107));
#30949=CARTESIAN_POINT('Ctrl Pts',(-2.1917497502459,-6.40455695793254,90.0925061137036));
#30950=CARTESIAN_POINT('Ctrl Pts',(-2.02734082285004,-6.45849260875372,
90.1006418320966));
#30951=CARTESIAN_POINT('Ctrl Pts',(-1.86095677945185,-6.50608398846896,
90.1087775504895));
#30952=CARTESIAN_POINT('Ctrl Pts',(-1.69470575162617,-6.55363732129888,
90.1169067647897));
#30953=CARTESIAN_POINT('Ctrl Pts',(-1.52648310167053,-6.59485638166404,
90.1250359790899));
#30954=CARTESIAN_POINT('Ctrl Pts',(-1.35681697417567,-6.62958043156494,
90.1331651933901));
#30955=CARTESIAN_POINT('Ctrl Pts',(-1.18725081170344,-6.66428402251811,
90.1412896180655));
#30956=CARTESIAN_POINT('Ctrl Pts',(-1.0162432227095,-6.69250015074158,90.1494140427409));
#30957=CARTESIAN_POINT('Ctrl Pts',(-0.844335673570511,-6.71411842838181,
90.1575384674163));
#30958=CARTESIAN_POINT('Ctrl Pts',(-0.671384535558887,-6.7358679428066,
90.1657122125505));
#30959=CARTESIAN_POINT('Ctrl Pts',(-0.497522835850102,-6.75093913494648,
90.1738859576847));
#30960=CARTESIAN_POINT('Ctrl Pts',(-0.323311073628327,-6.75927207246974,
90.1820597028189));
#30961=CARTESIAN_POINT('Ctrl Pts',(-0.15021491255361,-6.7675516482995,90.190181105681));
#30962=CARTESIAN_POINT('Ctrl Pts',(0.0232264698307039,-6.76917902219835,
90.1983025085432));
#30963=CARTESIAN_POINT('Ctrl Pts',(0.19645980411135,-6.76414758453484,90.2064239114053));
#30964=CARTESIAN_POINT('Ctrl Pts',(0.369706531881311,-6.75911575786707,
90.2145459421716));
#30965=CARTESIAN_POINT('Ctrl Pts',(0.542744813668747,-6.74742410473295,
90.2226679729378));
#30966=CARTESIAN_POINT('Ctrl Pts',(0.715023288481733,-6.72911812178452,
90.2307900037041));
#30967=CARTESIAN_POINT('Ctrl Pts',(0.887347888759076,-6.710807237632,90.2389142090452));
#30968=CARTESIAN_POINT('Ctrl Pts',(1.05891191321258,-6.68587853612958,90.2470384143864));
#30969=CARTESIAN_POINT('Ctrl Pts',(1.22917105937705,-6.65442916460833,90.2551626197275));
#30970=CARTESIAN_POINT('Ctrl Pts',(1.40127314298828,-6.62263937540169,90.2633747639699));
#30971=CARTESIAN_POINT('Ctrl Pts',(1.57204155703373,-6.58418699685215,90.2715869082123));
#30972=CARTESIAN_POINT('Ctrl Pts',(1.74092750534122,-6.53922475689178,90.2797990524548));
#30973=CARTESIAN_POINT('Ctrl Pts',(1.90827171107745,-6.49467297262735,90.2879362288712));
#30974=CARTESIAN_POINT('Ctrl Pts',(2.07376734684281,-6.44372985590002,90.2960734052877));
#30975=CARTESIAN_POINT('Ctrl Pts',(2.23689879097849,-6.38659320756528,90.3042105817041));
#30976=CARTESIAN_POINT('Ctrl Pts',(2.40228463069688,-6.32866695911207,90.3124602098595));
#30977=CARTESIAN_POINT('Ctrl Pts',(2.56524009130338,-6.26437488644009,90.3207098380149));
#30978=CARTESIAN_POINT('Ctrl Pts',(2.72525221586998,-6.1939720180104,90.3289594661703));
#30979=CARTESIAN_POINT('Ctrl Pts',(2.88526434043657,-6.12356914958071,90.3372090943257));
#30980=CARTESIAN_POINT('Ctrl Pts',(3.04233281075082,-6.04705571077292,90.3454587224811));
#30981=CARTESIAN_POINT('Ctrl Pts',(3.19597412377447,-5.96473288590227,90.3537083506365));
#30982=CARTESIAN_POINT('Ctrl Pts',(3.34915429694435,-5.88265714519587,90.3619332183141));
#30983=CARTESIAN_POINT('Ctrl Pts',(3.4993858102387,-5.79456166088951,90.3701580859917));
#30984=CARTESIAN_POINT('Ctrl Pts',(3.64616325782922,-5.70068263432163,90.3783829536693));
#30985=CARTESIAN_POINT('Ctrl Pts',(3.7927753441963,-5.60690937298502,90.3865985551129));
#30986=CARTESIAN_POINT('Ctrl Pts',(3.93594081413043,-5.50736573556886,90.3948141565564));
#30987=CARTESIAN_POINT('Ctrl Pts',(4.07517752010596,-5.40233441945453,90.403029758));
#30988=CARTESIAN_POINT('Ctrl Pts',(4.21428533579547,-5.29740032997508,90.4112377543281));
#30989=CARTESIAN_POINT('Ctrl Pts',(4.34947134572244,-5.18698889321526,90.4194457506562));
#30990=CARTESIAN_POINT('Ctrl Pts',(4.48028107267301,-5.07142687119197,90.4276537469844));
#30991=CARTESIAN_POINT('Ctrl Pts',(4.61099598393749,-4.9559486127592,90.4358557938558));
#30992=CARTESIAN_POINT('Ctrl Pts',(4.73734066264471,-4.83532744172815,90.4440578407273));
#30993=CARTESIAN_POINT('Ctrl Pts',(4.85889245303521,-4.70993132963077,90.4522598875987));
#30994=CARTESIAN_POINT('Ctrl Pts',(4.98038054691856,-4.58460092857167,90.4604576363703));
#30995=CARTESIAN_POINT('Ctrl Pts',(5.09708050688783,-4.45450082822877,90.4686553851419));
#30996=CARTESIAN_POINT('Ctrl Pts',(5.20860534822872,-4.32003695891635,90.4768531339134));
#30997=CARTESIAN_POINT('Ctrl Pts',(5.32010891844612,-4.18559873588628,90.4850493191291));
#30998=CARTESIAN_POINT('Ctrl Pts',(5.42643910252046,-4.04679867362448,90.4932455043447));
#30999=CARTESIAN_POINT('Ctrl Pts',(5.52724796153608,-3.90407722409473,90.5014416895603));
#31000=CARTESIAN_POINT('Ctrl Pts',(5.62804936293984,-3.7613663327757,90.5096372684407));
#31001=CARTESIAN_POINT('Ctrl Pts',(5.72333004498768,-3.61473492449087,90.517832847321));
#31002=CARTESIAN_POINT('Ctrl Pts',(5.8127843664756,-3.46465393782076,90.5260284262013));
#31003=CARTESIAN_POINT('Ctrl Pts',(5.90224834548913,-3.31455674834513,90.5342248898798));
#31004=CARTESIAN_POINT('Ctrl Pts',(5.98588452699447,-3.16100954680833,90.5424213535582));
#31005=CARTESIAN_POINT('Ctrl Pts',(6.06343233179332,-3.00450950368997,90.5506178172367));
#31006=CARTESIAN_POINT('Ctrl Pts',(6.14100261764907,-2.8479640913135,90.5588166570645));
#31007=CARTESIAN_POINT('Ctrl Pts',(6.21248085183368,-2.68846445370207,90.5670154968923));
#31008=CARTESIAN_POINT('Ctrl Pts',(6.27765384261681,-2.52652948375403,90.5752143367201));
#31009=CARTESIAN_POINT('Ctrl Pts',(6.34289490844288,-2.36442536812308,90.5834217404693));
#31010=CARTESIAN_POINT('Ctrl Pts',(6.40181743873401,-2.1998811713549,90.5916291442185));
#31011=CARTESIAN_POINT('Ctrl Pts',(6.45425722505974,-2.03343371486855,90.5998365479678));
#31012=CARTESIAN_POINT('Ctrl Pts',(6.50672510091013,-1.86689710031616,90.6080483480368));
#31013=CARTESIAN_POINT('Ctrl Pts',(6.55270321587474,-1.69845553951099,90.6162601481058));
#31014=CARTESIAN_POINT('Ctrl Pts',(6.59207814784328,-1.52865780759695,90.6244719481749));
#31015=CARTESIAN_POINT('Ctrl Pts',(6.6315110452135,-1.35861010969589,90.632695837161));
#31016=CARTESIAN_POINT('Ctrl Pts',(6.66432126536162,-1.18720260322624,90.6409197261471));
#31017=CARTESIAN_POINT('Ctrl Pts',(6.6904468984214,-1.01499226568656,90.6491436151333));
#31018=CARTESIAN_POINT('Ctrl Pts',(6.71458653171343,-0.855872890940896,
90.6567423463834));
#31019=CARTESIAN_POINT('Ctrl Pts',(6.73301979156511,-0.69606838245863,90.6643410776335));
#31020=CARTESIAN_POINT('Ctrl Pts',(6.74573740825346,-0.536018487451575,
90.6719398088836));
#31021=CARTESIAN_POINT('Ctrl Pts',(6.7595029257901,-0.362780868293384,90.6801646572056));
#31022=CARTESIAN_POINT('Ctrl Pts',(6.7666100882802,-0.188769501549492,90.6883895055277));
#31023=CARTESIAN_POINT('Ctrl Pts',(6.76698438507566,-0.0145372673548326,
90.6966143538497));
#31024=CARTESIAN_POINT('Ctrl Pts',(6.76735826032995,0.159498742713185,90.7048299391689));
#31025=CARTESIAN_POINT('Ctrl Pts',(6.76101436821537,0.333754769415102,90.7130455244881));
#31026=CARTESIAN_POINT('Ctrl Pts',(6.74792988781481,0.507672363966806,90.7212611098073));
#31027=CARTESIAN_POINT('Ctrl Pts',(6.73485751450766,0.681429032253275,90.7294690932306));
#31028=CARTESIAN_POINT('Ctrl Pts',(6.71505700093106,0.854847536531307,90.7376770766538));
#31029=CARTESIAN_POINT('Ctrl Pts',(6.68855755548671,1.02736888552345,90.745885060077));
#31030=CARTESIAN_POINT('Ctrl Pts',(6.66207730747878,1.19976525198954,90.7540870972535));
#31031=CARTESIAN_POINT('Ctrl Pts',(6.62890784815014,1.37126540455445,90.7622891344301));
#31032=CARTESIAN_POINT('Ctrl Pts',(6.58913025732375,1.54131484519571,90.7704911716066));
#31033=CARTESIAN_POINT('Ctrl Pts',(6.54937349554961,1.71127524151301,90.778688913886));
#31034=CARTESIAN_POINT('Ctrl Pts',(6.50301557720924,1.87978609073229,90.7868866561654));
#31035=CARTESIAN_POINT('Ctrl Pts',(6.45018879981069,2.04630238400798,90.7950843984448));
#31036=CARTESIAN_POINT('Ctrl Pts',(6.39737206654969,2.212787016966,90.8032805820591));
#31037=CARTESIAN_POINT('Ctrl Pts',(6.33808902656848,2.37727750584865,90.8114767656735));
#31038=CARTESIAN_POINT('Ctrl Pts',(6.27252212793175,2.53924302787396,90.8196729492878));
#31039=CARTESIAN_POINT('Ctrl Pts',(6.20696005593358,2.70119662697704,90.8278685295487));
#31040=CARTESIAN_POINT('Ctrl Pts',(6.13511518033477,2.86062529645276,90.8360641098096));
#31041=CARTESIAN_POINT('Ctrl Pts',(6.05721846300543,3.01701731705771,90.8442596900705));
#31042=CARTESIAN_POINT('Ctrl Pts',(5.97931330757512,3.17342627870596,90.8524561581112));
#31043=CARTESIAN_POINT('Ctrl Pts',(5.89535516435128,3.32679761487085,90.8606526261519));
#31044=CARTESIAN_POINT('Ctrl Pts',(5.80562142392341,3.47664333547195,90.8688490941926));
#31045=CARTESIAN_POINT('Ctrl Pts',(5.71586163709679,3.62653255076492,90.877047941366));
#31046=CARTESIAN_POINT('Ctrl Pts',(5.62032309811326,3.77289380432431,90.8852467885394));
#31047=CARTESIAN_POINT('Ctrl Pts',(5.51932708963897,3.91526722939539,90.8934456357128));
#31048=CARTESIAN_POINT('Ctrl Pts',(5.41822553051475,4.05778944854036,90.9016530514787));
#31049=CARTESIAN_POINT('Ctrl Pts',(5.31165531477073,4.1963152196775,90.9098604672447));
#31050=CARTESIAN_POINT('Ctrl Pts',(5.19997928830277,4.33041619261039,90.9180678830107));
#31051=CARTESIAN_POINT('Ctrl Pts',(5.08824340741248,4.46458903894817,90.9262796976628));
#31052=CARTESIAN_POINT('Ctrl Pts',(4.97139650035427,4.59433209298243,90.9344915123149));
#31053=CARTESIAN_POINT('Ctrl Pts',(4.84983892418515,4.71925326820448,90.9427033269671));
#31054=CARTESIAN_POINT('Ctrl Pts',(4.72810233600539,4.84435840884812,90.9509272347647));
#31055=CARTESIAN_POINT('Ctrl Pts',(4.60164147498368,4.96462723234345,90.9591511425623));
#31056=CARTESIAN_POINT('Ctrl Pts',(4.47089144602487,5.07970655430623,90.9673750503599));
#31057=CARTESIAN_POINT('Ctrl Pts',(4.35008083399665,5.18603772248131,90.9749737892834));
#31058=CARTESIAN_POINT('Ctrl Pts',(4.22560891298427,5.28793871061637,90.9825725282069));
#31059=CARTESIAN_POINT('Ctrl Pts',(4.09784061972497,5.38516399521241,90.9901712671303));
#31060=CARTESIAN_POINT('Ctrl Pts',(3.96075565233607,5.48947880312157,90.9983240948073));
#31061=CARTESIAN_POINT('Ctrl Pts',(3.81946952411304,5.58871963443161,91.0064769224842));
#31062=CARTESIAN_POINT('Ctrl Pts',(3.67439693588874,5.68252550874446,91.0146297501611));
#31063=CARTESIAN_POINT('Ctrl Pts',(3.52951465418826,5.77620832831572,91.0227718829417));
#31064=CARTESIAN_POINT('Ctrl Pts',(3.38085610879501,5.86447019286279,91.0309140157223));
#31065=CARTESIAN_POINT('Ctrl Pts',(3.2288689564537,5.94699035328372,91.0390561485029));
#31066=CARTESIAN_POINT('Ctrl Pts',(3.18590021063501,5.9703198764929,91.0413580353959));
#31067=CARTESIAN_POINT('Ctrl Pts',(3.14266561864551,5.99319073505027,91.0436599222888));
#31068=CARTESIAN_POINT('Ctrl Pts',(3.09917575053275,6.01559628526631,91.0459618091817));
#31069=CARTESIAN_POINT('Ctrl Pts',(3.09917575053266,6.01559628526635,89.0455129651334));
#31070=CARTESIAN_POINT('Ctrl Pts',(2.94549603082524,6.09477055795357,89.0536675572585));
#31071=CARTESIAN_POINT('Ctrl Pts',(2.78897690056007,6.16795072432149,89.0618221493837));
#31072=CARTESIAN_POINT('Ctrl Pts',(2.63013819161377,6.23495485893961,89.0699767415088));
#31073=CARTESIAN_POINT('Ctrl Pts',(2.55997831502702,6.26455093062009,89.073578666889));
#31074=CARTESIAN_POINT('Ctrl Pts',(2.48936606853457,6.29294269471233,89.0771805922693));
#31075=CARTESIAN_POINT('Ctrl Pts',(2.41834701719733,6.32011761792554,89.0807825176495));
#31076=CARTESIAN_POINT('Ctrl Pts',(2.25604142262126,6.38222267264861,89.0890142896803));
#31077=CARTESIAN_POINT('Ctrl Pts',(2.09110366302185,6.43816268252841,89.0972460617112));
#31078=CARTESIAN_POINT('Ctrl Pts',(1.92404214632294,6.48770767060085,89.105477833742));
#31079=CARTESIAN_POINT('Ctrl Pts',(1.75718011777019,6.53719349700626,89.1136997762144));
#31080=CARTESIAN_POINT('Ctrl Pts',(1.58819972197526,6.58029940635646,89.1219217186869));
#31081=CARTESIAN_POINT('Ctrl Pts',(1.41762956869311,6.61684331127517,89.1301436611593));
#31082=CARTESIAN_POINT('Ctrl Pts',(1.24722891798956,6.65335090101215,89.1383574331492));
#31083=CARTESIAN_POINT('Ctrl Pts',(1.07524200392315,6.68330939818465,89.1465712051391));
#31084=CARTESIAN_POINT('Ctrl Pts',(0.902212927985894,6.7065863770308,89.154784977129));
#31085=CARTESIAN_POINT('Ctrl Pts',(0.729321142857274,6.72984488663859,89.1629922318594));
#31086=CARTESIAN_POINT('Ctrl Pts',(0.555389196392874,6.7464323897719,89.1711994865897));
#31087=CARTESIAN_POINT('Ctrl Pts',(0.380971819444985,6.75626742164553,89.1794067413201));
#31088=CARTESIAN_POINT('Ctrl Pts',(0.206657910601496,6.7660966191687,89.1876091273321));
#31089=CARTESIAN_POINT('Ctrl Pts',(0.0318595017268982,6.76918130516252,
89.1958115133441));
#31090=CARTESIAN_POINT('Ctrl Pts',(-0.142863013963399,6.76549178990273,
89.2040138993561));
#31091=CARTESIAN_POINT('Ctrl Pts',(-0.317533379220613,6.76180337587377,
89.2122138371548));
#31092=CARTESIAN_POINT('Ctrl Pts',(-0.492127538551597,6.75134479187953,
89.2204137749534));
#31093=CARTESIAN_POINT('Ctrl Pts',(-0.666084300259802,6.73413845305748,
89.2286137127521));
#31094=CARTESIAN_POINT('Ctrl Pts',(-0.840016738322924,6.7169345201257,89.2368125039879));
#31095=CARTESIAN_POINT('Ctrl Pts',(-1.01331159962821,6.692984745948,89.2450112952237));
#31096=CARTESIAN_POINT('Ctrl Pts',(-1.18541199675908,6.66236349938516,89.2532100864595));
#31097=CARTESIAN_POINT('Ctrl Pts',(-1.357519549718,6.63174097960983,89.2614092185959));
#31098=CARTESIAN_POINT('Ctrl Pts',(-1.52843218663935,6.59444649752415,89.2696083507323));
#31099=CARTESIAN_POINT('Ctrl Pts',(-1.69760234907644,6.55060571736768,89.2778074828688));
#31100=CARTESIAN_POINT('Ctrl Pts',(-1.86681023373675,6.50675516142291,89.2860084432797));
#31101=CARTESIAN_POINT('Ctrl Pts',(-2.03427452314954,6.45635548996661,89.2942094036906));
#31102=CARTESIAN_POINT('Ctrl Pts',(-2.19946192181757,6.39958250626356,89.3024103641015));
#31103=CARTESIAN_POINT('Ctrl Pts',(-2.36480414084381,6.34275631260779,89.3106190107866));
#31104=CARTESIAN_POINT('Ctrl Pts',(-2.52786486612134,6.27954498901384,89.3188276574716));
#31105=CARTESIAN_POINT('Ctrl Pts',(-2.68812904233416,6.21017320626081,89.3270363041567));
#31106=CARTESIAN_POINT('Ctrl Pts',(-2.84846973316572,6.14076830347038,89.3352488698802));
#31107=CARTESIAN_POINT('Ctrl Pts',(-3.00601088986818,6.06519723225535,89.3434614356037));
#31108=CARTESIAN_POINT('Ctrl Pts',(-3.16026132918106,5.98373105439096,89.3516740013272));
#31109=CARTESIAN_POINT('Ctrl Pts',(-3.31472342235522,5.90215309317486,89.359897835876));
#31110=CARTESIAN_POINT('Ctrl Pts',(-3.4658854636801,5.81466403877044,89.3681216704247));
#31111=CARTESIAN_POINT('Ctrl Pts',(-3.61328352052205,5.72157943231795,89.3763455049735));
#31112=CARTESIAN_POINT('Ctrl Pts',(-3.74871460788017,5.6360521890268,89.3839016619477));
#31113=CARTESIAN_POINT('Ctrl Pts',(-3.88096824980724,5.54580171474602,89.391457818922));
#31114=CARTESIAN_POINT('Ctrl Pts',(-4.00970942196484,5.4511025812588,89.3990139758962));
#31115=CARTESIAN_POINT('Ctrl Pts',(-4.15701444487575,5.34274829339431,89.4076596939486));
#31116=CARTESIAN_POINT('Ctrl Pts',(-4.30005656548543,5.22832269101837,89.4163054120009));
#31117=CARTESIAN_POINT('Ctrl Pts',(-4.43833437284333,5.1081774631308,89.4249511300533));
#31118=CARTESIAN_POINT('Ctrl Pts',(-4.57643465967659,4.98818647723112,89.4335857487656));
#31119=CARTESIAN_POINT('Ctrl Pts',(-4.70978260057282,4.86249070688326,89.442220367478));
#31120=CARTESIAN_POINT('Ctrl Pts',(-4.83790797572715,4.73148342683303,89.4508549861903));
#31121=CARTESIAN_POINT('Ctrl Pts',(-4.97055824140488,4.59584947857377,89.4597945460927));
#31122=CARTESIAN_POINT('Ctrl Pts',(-5.09761005166698,4.45452217666433,89.4687341059952));
#31123=CARTESIAN_POINT('Ctrl Pts',(-5.2185790068843,4.30798353628545,89.4776736658976));
#31124=CARTESIAN_POINT('Ctrl Pts',(-5.3350972405823,4.16683638398692,89.4862843191681));
#31125=CARTESIAN_POINT('Ctrl Pts',(-5.44597198202418,4.02085476569849,89.4948949724386));
#31126=CARTESIAN_POINT('Ctrl Pts',(-5.5508074454288,3.87050716363788,89.5035056257091));
#31127=CARTESIAN_POINT('Ctrl Pts',(-5.65554367505331,3.72030187564161,89.5121081284202));
#31128=CARTESIAN_POINT('Ctrl Pts',(-5.75425185009584,3.56573909271019,89.5207106311313));
#31129=CARTESIAN_POINT('Ctrl Pts',(-5.84657691847434,3.40731967041003,89.5293131338424));
#31130=CARTESIAN_POINT('Ctrl Pts',(-5.93879807684676,3.2490785459809,89.5379059546098));
#31131=CARTESIAN_POINT('Ctrl Pts',(-6.02465030729407,3.0869897044384,89.5464987753773));
#31132=CARTESIAN_POINT('Ctrl Pts',(-6.1038221834623,2.9215824055935,89.5550915961447));
#31133=CARTESIAN_POINT('Ctrl Pts',(-6.11315294868852,2.90208840410054,89.5561042991031));
#31134=CARTESIAN_POINT('Ctrl Pts',(-6.12239097611867,2.88254834210267,89.5571170020614));
#31135=CARTESIAN_POINT('Ctrl Pts',(-6.13153579659713,2.86296311101768,89.5581297050197));
#31136=CARTESIAN_POINT('Ctrl Pts',(-6.20694943739315,2.70145162094188,89.5664810572756));
#31137=CARTESIAN_POINT('Ctrl Pts',(-6.2759495415789,2.53701859353149,89.5748324095315));
#31138=CARTESIAN_POINT('Ctrl Pts',(-6.3383282268765,2.37020764668006,89.5831837617874));
#31139=CARTESIAN_POINT('Ctrl Pts',(-6.400741841753,2.20330329234334,89.5915397904679));
#31140=CARTESIAN_POINT('Ctrl Pts',(-6.45652652657995,2.03401868138721,89.5998958191483));
#31141=CARTESIAN_POINT('Ctrl Pts',(-6.50552402217737,1.86291336268577,89.6082518478288));
#31142=CARTESIAN_POINT('Ctrl Pts',(-6.55458494958711,1.69158653224517,89.6166186941651));
#31143=CARTESIAN_POINT('Ctrl Pts',(-6.59684103795359,1.51843461103407,89.6249855405014));
#31144=CARTESIAN_POINT('Ctrl Pts',(-6.63218470330744,1.34402941233246,89.6333523868377));
#31145=CARTESIAN_POINT('Ctrl Pts',(-6.66755368113727,1.16949930787032,89.6417252253537));
#31146=CARTESIAN_POINT('Ctrl Pts',(-6.69600030669519,0.993714469902181,
89.6500980638698));
#31147=CARTESIAN_POINT('Ctrl Pts',(-6.7174687628772,0.817252971710188,89.6584709023859));
#31148=CARTESIAN_POINT('Ctrl Pts',(-6.73896903306949,0.64052997600431,89.6668561485743));
#31149=CARTESIAN_POINT('Ctrl Pts',(-6.75347044137896,0.463128654103991,
89.6752413947628));
#31150=CARTESIAN_POINT('Ctrl Pts',(-6.76096921623424,0.285629580283465,
89.6836266409512));
#31151=CARTESIAN_POINT('Ctrl Pts',(-6.76500932685846,0.189998506171939,
89.6881443552268));
#31152=CARTESIAN_POINT('Ctrl Pts',(-6.76701766328379,0.0943390253482907,
89.6926620695022));
#31153=CARTESIAN_POINT('Ctrl Pts',(-6.76699988295537,-0.00125860319118299,
89.6971797837778));
#31154=CARTESIAN_POINT('',(-6.77442561751979,-0.00144966683613033,89.3028202190345));
#31155=CARTESIAN_POINT('Ctrl Pts',(3.10355585847744,6.02401335114973,88.6512963024177));
#31156=CARTESIAN_POINT('Ctrl Pts',(3.00479133306508,6.07541714714956,88.6565561665253));
#31157=CARTESIAN_POINT('Ctrl Pts',(0.888771830976022,7.10662707875989,88.7677504104355));
#31158=CARTESIAN_POINT('Ctrl Pts',(-4.32981959233283,6.73089174556964,88.9849250483597));
#31159=CARTESIAN_POINT('Ctrl Pts',(-6.77955107493284,2.23990816749953,89.1968398221759));
#31160=CARTESIAN_POINT('Ctrl Pts',(-6.7788200090861,-0.00145054709842048,
89.3028202161897));
#31161=CARTESIAN_POINT('Ctrl Pts',(-6.76699984504039,-0.00144817934294948,
89.3028202238418));
#31162=CARTESIAN_POINT('Ctrl Pts',(-6.76696265070365,-0.175248525353057,
89.311052552929));
#31163=CARTESIAN_POINT('Ctrl Pts',(-6.76022539825672,-0.349301770394149,
89.3192848820163));
#31164=CARTESIAN_POINT('Ctrl Pts',(-6.74675528548857,-0.523050779305459,
89.3275172111035));
#31165=CARTESIAN_POINT('Ctrl Pts',(-6.73330121635344,-0.696592843747613,
89.3357397350415));
#31166=CARTESIAN_POINT('Ctrl Pts',(-6.71313028247931,-0.869831039932917,
89.3439622589794));
#31167=CARTESIAN_POINT('Ctrl Pts',(-6.68626163023778,-1.0422065112107,89.3521847829174));
#31168=CARTESIAN_POINT('Ctrl Pts',(-6.65941959930036,-1.21441119387581,
89.3603991600265));
#31169=CARTESIAN_POINT('Ctrl Pts',(-6.62589312054883,-1.38575450239281,
89.3686135371357));
#31170=CARTESIAN_POINT('Ctrl Pts',(-6.58575325746878,-1.55568089007332,
89.3768279142448));
#31171=CARTESIAN_POINT('Ctrl Pts',(-6.54564512923008,-1.72547293282737,
89.385035797013));
#31172=CARTESIAN_POINT('Ctrl Pts',(-6.49893411291866,-1.89384993891608,
89.3932436797813));
#31173=CARTESIAN_POINT('Ctrl Pts',(-6.44574266198897,-2.06026467605874,
89.4014515625496));
#31174=CARTESIAN_POINT('Ctrl Pts',(-6.39258261907043,-2.22658115011907,
89.4096545988008));
#31175=CARTESIAN_POINT('Ctrl Pts',(-6.33294987322123,-2.39093732310856,
89.417857635052));
#31176=CARTESIAN_POINT('Ctrl Pts',(-6.26701725032542,-2.55279920560228,
89.4260606713032));
#31177=CARTESIAN_POINT('Ctrl Pts',(-6.20110411656765,-2.71461324306219,
89.4342612828047));
#31178=CARTESIAN_POINT('Ctrl Pts',(-6.12889494656976,-2.87393412585758,
89.4424618943062));
#31179=CARTESIAN_POINT('Ctrl Pts',(-6.05061150614224,-3.03024576589741,
89.4506625058077));
#31180=CARTESIAN_POINT('Ctrl Pts',(-5.97233883730244,-3.18653589788224,
89.4588619889275));
#31181=CARTESIAN_POINT('Ctrl Pts',(-5.88799372235747,-3.33981729111234,
89.4670614720472));
#31182=CARTESIAN_POINT('Ctrl Pts',(-5.79784489959881,-3.48959646953571,
89.475260955167));
#31183=CARTESIAN_POINT('Ctrl Pts',(-5.70769213553479,-3.6393821963028,89.4834607967681));
#31184=CARTESIAN_POINT('Ctrl Pts',(-5.61173534291087,-3.78566509613694,
89.4916606383692));
#31185=CARTESIAN_POINT('Ctrl Pts',(-5.51028781984356,-3.92797876044203,
89.4998604799702));
#31186=CARTESIAN_POINT('Ctrl Pts',(-5.40881746737885,-4.07032445051868,
89.5080621668351));
#31187=CARTESIAN_POINT('Ctrl Pts',(-5.30185413145434,-4.20869883427915,
89.5162638537));
#31188=CARTESIAN_POINT('Ctrl Pts',(-5.18975282496585,-4.34266676314899,
89.5244655405648));
#31189=CARTESIAN_POINT('Ctrl Pts',(-5.07754666409169,-4.47675999943338,
89.5326748989089));
#31190=CARTESIAN_POINT('Ctrl Pts',(-4.96019316133644,-4.60643827107466,
89.5408842572529));
#31191=CARTESIAN_POINT('Ctrl Pts',(-4.83808642973629,-4.73130095200058,
89.549093615597));
#31192=CARTESIAN_POINT('Ctrl Pts',(-4.71592118302453,-4.85622346872436,
89.5573069079708));
#31193=CARTESIAN_POINT('Ctrl Pts',(-4.58899842606424,-4.97632554743034,
89.5655202003446));
#31194=CARTESIAN_POINT('Ctrl Pts',(-4.45774704878049,-5.09124545166395,
89.5737334927185));
#31195=CARTESIAN_POINT('Ctrl Pts',(-4.32631686568479,-5.20632191308736,
89.5819579741895));
#31196=CARTESIAN_POINT('Ctrl Pts',(-4.19054655584925,-5.31620186561755,
89.5901824556604));
#31197=CARTESIAN_POINT('Ctrl Pts',(-4.05089677684706,-5.42056494318905,
89.5984069371314));
#31198=CARTESIAN_POINT('Ctrl Pts',(-3.92593488445409,-5.51395146884251,
89.6057663957422));
#31199=CARTESIAN_POINT('Ctrl Pts',(-3.79786722402444,-5.60292107817416,
89.6131258543529));
#31200=CARTESIAN_POINT('Ctrl Pts',(-3.66704116395306,-5.68727510341058,
89.6204853129636));
#31201=CARTESIAN_POINT('Ctrl Pts',(-3.51334538395874,-5.78637506634838,
89.6291312794545));
#31202=CARTESIAN_POINT('Ctrl Pts',(-3.35549317856629,-5.87932933795801,
89.6377772459454));
#31203=CARTESIAN_POINT('Ctrl Pts',(-3.19399180898765,-5.96579460961571,
89.6464232124363));
#31204=CARTESIAN_POINT('Ctrl Pts',(-3.03269702161607,-6.0521492804364,89.6550581195607));
#31205=CARTESIAN_POINT('Ctrl Pts',(-2.86776264543916,-6.13203135937298,
89.6636930266851));
#31206=CARTESIAN_POINT('Ctrl Pts',(-2.69972368964322,-6.20514149714406,
89.6723279338095));
#31207=CARTESIAN_POINT('Ctrl Pts',(-2.5261059761421,-6.28067883248063,89.681249512881));
#31208=CARTESIAN_POINT('Ctrl Pts',(-2.34917425510513,-6.34898665526861,
89.6901710919525));
#31209=CARTESIAN_POINT('Ctrl Pts',(-2.16954766146866,-6.40978563952149,
89.699092671024));
#31210=CARTESIAN_POINT('Ctrl Pts',(-1.99617306275606,-6.46846848421379,
89.7077037299997));
#31211=CARTESIAN_POINT('Ctrl Pts',(-1.82028833657608,-6.52015622982342,
89.7163147889754));
#31212=CARTESIAN_POINT('Ctrl Pts',(-1.64247222101487,-6.56464576372515,
89.7249258479511));
#31213=CARTESIAN_POINT('Ctrl Pts',(-1.46482379425947,-6.60909334194255,
89.7335287863006));
#31214=CARTESIAN_POINT('Ctrl Pts',(-1.28524790436,-6.64635616866093,89.7421317246502));
#31215=CARTESIAN_POINT('Ctrl Pts',(-1.10433903936368,-6.67628072253836,
89.7507346629997));
#31216=CARTESIAN_POINT('Ctrl Pts',(-0.923632750445762,-6.70617176783801,
89.7593279680485));
#31217=CARTESIAN_POINT('Ctrl Pts',(-0.741596764402537,-6.72874088365617,
89.7679212730972));
#31218=CARTESIAN_POINT('Ctrl Pts',(-0.558836585141634,-6.74388542837935,
89.776514578146));
#31219=CARTESIAN_POINT('Ctrl Pts',(-0.538474109691523,-6.74557277855254,
89.7774720129865));
#31220=CARTESIAN_POINT('Ctrl Pts',(-0.518102655000697,-6.74716801521932,
89.7784294478271));
#31221=CARTESIAN_POINT('Ctrl Pts',(-0.497723066033231,-6.74867103580686,
89.7793868826677));
#31222=CARTESIAN_POINT('Ctrl Pts',(-0.314757084158314,-6.76216500950856,
89.7879826402152));
#31223=CARTESIAN_POINT('Ctrl Pts',(-0.131349403861584,-6.76820605441165,
89.7965783977628));
#31224=CARTESIAN_POINT('Ctrl Pts',(0.0518851096250705,-6.76680108584545,
89.8051741553104));
#31225=CARTESIAN_POINT('Ctrl Pts',(0.23529058714254,-6.76539480639581,89.813777932992));
#31226=CARTESIAN_POINT('Ctrl Pts',(0.418522270053867,-6.75652864858688,
89.8223817106736));
#31227=CARTESIAN_POINT('Ctrl Pts',(0.600968566963205,-6.74026155141788,
89.8309854883552));
#31228=CARTESIAN_POINT('Ctrl Pts',(0.790585162880118,-6.72335514310549,
89.8399274020232));
#31229=CARTESIAN_POINT('Ctrl Pts',(0.979353017731205,-6.69845435117792,
89.8488693156912));
#31230=CARTESIAN_POINT('Ctrl Pts',(1.16659650727857,-6.66568388008353,89.8578112293592));
#31231=CARTESIAN_POINT('Ctrl Pts',(1.34724994785157,-6.63406676823249,89.8664384316899));
#31232=CARTESIAN_POINT('Ctrl Pts',(1.52648421520364,-6.5951245947866,89.8750656340206));
#31233=CARTESIAN_POINT('Ctrl Pts',(1.70370697552198,-6.5490206551482,89.8836928363513));
#31234=CARTESIAN_POINT('Ctrl Pts',(1.88109851339277,-6.50287280856423,89.8923282547717));
#31235=CARTESIAN_POINT('Ctrl Pts',(2.05647442793163,-6.44954966720732,89.9009636731921));
#31236=CARTESIAN_POINT('Ctrl Pts',(2.22925926219645,-6.38926381846229,89.9095990916125));
#31237=CARTESIAN_POINT('Ctrl Pts',(2.40229936144318,-6.32888890596259,89.9182472676337));
#31238=CARTESIAN_POINT('Ctrl Pts',(2.57274044573925,-6.2615308383996,89.9268954436548));
#31239=CARTESIAN_POINT('Ctrl Pts',(2.74002730451484,-6.18745015095177,89.9355436196759));
#31240=CARTESIAN_POINT('Ctrl Pts',(2.75772561987258,-6.17961269511115,89.9364585639077));
#31241=CARTESIAN_POINT('Ctrl Pts',(2.77538865371704,-6.17170003616697,89.9373735081395));
#31242=CARTESIAN_POINT('Ctrl Pts',(2.79301576541894,-6.16371251228683,89.9382884523713));
#31243=CARTESIAN_POINT('Ctrl Pts',(2.95149590480565,-6.09189905133607,89.9465144449126));
#31244=CARTESIAN_POINT('Ctrl Pts',(3.1074125902076,-6.01387519699057,89.954740437454));
#31245=CARTESIAN_POINT('Ctrl Pts',(3.26024624044715,-5.92984683205648,89.9629664299953));
#31246=CARTESIAN_POINT('Ctrl Pts',(3.41291966435877,-5.84590656000202,89.9711837986467));
#31247=CARTESIAN_POINT('Ctrl Pts',(3.56251617815635,-5.75597448414214,89.9794011672981));
#31248=CARTESIAN_POINT('Ctrl Pts',(3.70853670240629,-5.66030427865018,89.9876185359495));
#31249=CARTESIAN_POINT('Ctrl Pts',(3.85443336108473,-5.56471522780917,89.9958289340119));
#31250=CARTESIAN_POINT('Ctrl Pts',(3.99675977367483,-5.4633979368922,90.0040393320743));
#31251=CARTESIAN_POINT('Ctrl Pts',(4.13504190170056,-5.35665170336664,90.0122497301367));
#31252=CARTESIAN_POINT('Ctrl Pts',(4.27323439030631,-5.24997466656659,90.0204548059255));
#31253=CARTESIAN_POINT('Ctrl Pts',(4.40738753388358,-5.13787591537142,90.0286598817142));
#31254=CARTESIAN_POINT('Ctrl Pts',(4.53705663900844,-5.02069776569248,90.036864957503));
#31255=CARTESIAN_POINT('Ctrl Pts',(4.66666762163094,-4.90357213960638,90.0450663554725));
#31256=CARTESIAN_POINT('Ctrl Pts',(4.7917983048632,-4.78137189075798,90.0532677534419));
#31257=CARTESIAN_POINT('Ctrl Pts',(4.91203736727252,-4.65447933742524,90.0614691514114));
#31258=CARTESIAN_POINT('Ctrl Pts',(5.03226701155738,-4.52759672337376,90.0696699069791));
#31259=CARTESIAN_POINT('Ctrl Pts',(5.14760554564225,-4.39602279080391,90.0778706625469));
#31260=CARTESIAN_POINT('Ctrl Pts',(5.25767854304365,-4.26017667920222,90.0860714181146));
#31261=CARTESIAN_POINT('Ctrl Pts',(5.36775098132661,-4.12433125763411,90.0942721320263));
#31262=CARTESIAN_POINT('Ctrl Pts',(5.47255770975845,-3.98421397802927,90.1024728459381));
#31263=CARTESIAN_POINT('Ctrl Pts',(5.57176472796013,-3.84027691921551,90.1106735598499));
#31264=CARTESIAN_POINT('Ctrl Pts',(5.67098922101932,-3.69631450655443,90.1188757182795));
#31265=CARTESIAN_POINT('Ctrl Pts',(5.76461183530915,-3.54853126925179,90.1270778767091));
#31266=CARTESIAN_POINT('Ctrl Pts',(5.85234200095878,-3.39740814501494,90.1352800351387));
#31267=CARTESIAN_POINT('Ctrl Pts',(5.94010351892995,-3.24623101357602,90.1434851247916));
#31268=CARTESIAN_POINT('Ctrl Pts',(6.02196821358159,-3.09171192725364,90.1516902144446));
#31269=CARTESIAN_POINT('Ctrl Pts',(6.0976915279016,-2.93435632303868,90.1598953040975));
#31270=CARTESIAN_POINT('Ctrl Pts',(6.17350134715538,-2.7768209586502,90.1681097670953));
#31271=CARTESIAN_POINT('Ctrl Pts',(6.24315561418344,-2.6164429259011,90.1763242300931));
#31272=CARTESIAN_POINT('Ctrl Pts',(6.30645757824187,-2.45374852294113,90.1845386930908));
#31273=CARTESIAN_POINT('Ctrl Pts',(6.36979704671332,-2.29095772868938,90.1927580228983));
#31274=CARTESIAN_POINT('Ctrl Pts',(6.42677659332348,-2.12584816675173,90.2009773527058));
#31275=CARTESIAN_POINT('Ctrl Pts',(6.47724945315914,-1.95896108219372,90.2091966825133));
#31276=CARTESIAN_POINT('Ctrl Pts',(6.527800517631,-1.79181541621639,90.217428747674));
#31277=CARTESIAN_POINT('Ctrl Pts',(6.57182465781303,-1.62288707027252,90.2256608128347));
#31278=CARTESIAN_POINT('Ctrl Pts',(6.60922602780241,-1.45272857527453,90.2338928779953));
#31279=CARTESIAN_POINT('Ctrl Pts',(6.64284506471496,-1.29977790191831,90.2412924492566));
#31280=CARTESIAN_POINT('Ctrl Pts',(6.6711137667923,-1.14583359882521,90.2486920205178));
#31281=CARTESIAN_POINT('Ctrl Pts',(6.69399839447839,-0.991299397115065,
90.256091591779));
#31282=CARTESIAN_POINT('Ctrl Pts',(6.7192207516475,-0.820979089359053,90.2642470501858));
#31283=CARTESIAN_POINT('Ctrl Pts',(6.73797962917,-0.649417720235256,90.2724025085926));
#31284=CARTESIAN_POINT('Ctrl Pts',(6.75015668295053,-0.477151711322865,
90.2805579669994));
#31285=CARTESIAN_POINT('Ctrl Pts',(6.76231891565596,-0.305095372787335,
90.2887034991413));
#31286=CARTESIAN_POINT('Ctrl Pts',(6.76791524528198,-0.132336462220329,
90.2968490312831));
#31287=CARTESIAN_POINT('Ctrl Pts',(6.7668783330469,0.0405786365024204,90.304994563425));
#31288=CARTESIAN_POINT('Ctrl Pts',(6.76584246482847,0.213319635397034,90.3131318942256));
#31289=CARTESIAN_POINT('Ctrl Pts',(6.75818665301157,0.386216146611542,90.3212692250261));
#31290=CARTESIAN_POINT('Ctrl Pts',(6.74389534570866,0.558716892646988,90.3294065558267));
#31291=CARTESIAN_POINT('Ctrl Pts',(6.7296154242676,0.731080207611699,90.3375374036287));
#31292=CARTESIAN_POINT('Ctrl Pts',(6.70871056343421,0.903048022650518,90.3456682514307));
#31293=CARTESIAN_POINT('Ctrl Pts',(6.68121726641431,1.07406928964906,90.3537990992328));
#31294=CARTESIAN_POINT('Ctrl Pts',(6.65374009781757,1.24499023025313,90.3619251772266));
#31295=CARTESIAN_POINT('Ctrl Pts',(6.61968224793648,1.41496536867099,90.3700512552204));
#31296=CARTESIAN_POINT('Ctrl Pts',(6.57913202703983,1.58344901110798,90.3781773332142));
#31297=CARTESIAN_POINT('Ctrl Pts',(6.53843802246611,1.75253006576861,90.3863322247964));
#31298=CARTESIAN_POINT('Ctrl Pts',(6.4912055576777,1.9201086578375,90.3944871163785));
#31299=CARTESIAN_POINT('Ctrl Pts',(6.43757573536627,2.08564322246723,90.4026420079607));
#31300=CARTESIAN_POINT('Ctrl Pts',(6.38415505061073,2.25053226017239,90.410765098317));
#31301=CARTESIAN_POINT('Ctrl Pts',(6.3243869434986,2.41339283868552,90.4188881886733));
#31302=CARTESIAN_POINT('Ctrl Pts',(6.25846084365304,2.57370489148652,90.4270112790296));
#31303=CARTESIAN_POINT('Ctrl Pts',(6.19252956698909,2.73402953272194,90.435135007248));
#31304=CARTESIAN_POINT('Ctrl Pts',(6.12043947350541,2.89180491126887,90.4432587354665));
#31305=CARTESIAN_POINT('Ctrl Pts',(6.04242806073999,3.04653116359935,90.4513824636849));
#31306=CARTESIAN_POINT('Ctrl Pts',(5.96439568058366,3.20129900222728,90.4595083753453));
#31307=CARTESIAN_POINT('Ctrl Pts',(5.88043897681269,3.35301575629469,90.4676342870056));
#31308=CARTESIAN_POINT('Ctrl Pts',(5.79084126922772,3.50120641988003,90.4757601986659));
#31309=CARTESIAN_POINT('Ctrl Pts',(5.70067057498911,3.65034477816333,90.4839380763759));
#31310=CARTESIAN_POINT('Ctrl Pts',(5.60478667122776,3.79591146857661,90.492115954086));
#31311=CARTESIAN_POINT('Ctrl Pts',(5.50352196063604,3.93745286051742,90.5002938317961));
#31312=CARTESIAN_POINT('Ctrl Pts',(5.40274056454492,4.07831870609307,90.5084326782695));
#31313=CARTESIAN_POINT('Ctrl Pts',(5.29662988469172,4.21519734130055,90.516571524743));
#31314=CARTESIAN_POINT('Ctrl Pts',(5.18555709224255,4.34767600484362,90.5247103712164));
#31315=CARTESIAN_POINT('Ctrl Pts',(5.07368529680328,4.48110765467579,90.5329077645448));
#31316=CARTESIAN_POINT('Ctrl Pts',(4.95677998332856,4.61007551183414,90.5411051578731));
#31317=CARTESIAN_POINT('Ctrl Pts',(4.83525264498751,4.73419696032403,90.5493025512015));
#31318=CARTESIAN_POINT('Ctrl Pts',(4.71372530664655,4.85831840881383,90.5574999445299));
#31319=CARTESIAN_POINT('Ctrl Pts',(4.58757625589913,4.97759323730456,90.5656973378583));
#31320=CARTESIAN_POINT('Ctrl Pts',(4.45724896156953,5.09168151935953,90.5738947311867));
#31321=CARTESIAN_POINT('Ctrl Pts',(4.32646157626755,5.20617256423481,90.5821210635542));
#31322=CARTESIAN_POINT('Ctrl Pts',(4.19107721989538,5.31578121746848,90.5903473959217));
#31323=CARTESIAN_POINT('Ctrl Pts',(4.05149525096489,5.42011763999721,90.5985737282891));
#31324=CARTESIAN_POINT('Ctrl Pts',(3.91205160760407,5.52435066525198,90.6067919083708));
#31325=CARTESIAN_POINT('Ctrl Pts',(3.76841891532853,5.62332164540642,90.6150100884524));
#31326=CARTESIAN_POINT('Ctrl Pts',(3.62103201932383,5.71667876612212,90.623228268534));
#31327=CARTESIAN_POINT('Ctrl Pts',(3.47379502011576,5.80994093990756,90.6314380904854));
#31328=CARTESIAN_POINT('Ctrl Pts',(3.32281172514781,5.89760043816214,90.6396479124369));
#31329=CARTESIAN_POINT('Ctrl Pts',(3.16854834407815,5.97934698702456,90.6478577343883));
#31330=CARTESIAN_POINT('Ctrl Pts',(3.14549679572227,5.99156235862449,90.6490845265563));
#31331=CARTESIAN_POINT('Ctrl Pts',(3.12237206044821,6.00364577566048,90.6503113187243));
#31332=CARTESIAN_POINT('Ctrl Pts',(3.09917575053247,6.01559628526645,90.6515381108923));
#31333=CARTESIAN_POINT('Origin',(0.,0.,-3.69717978381041));
#31334=CARTESIAN_POINT('',(3.09917575053244,6.01559628526647,93.0458095097322));
#31335=CARTESIAN_POINT('',(3.09917575053273,6.01559628526632,92.651392015122));
#31336=CARTESIAN_POINT('',(3.09917575053259,6.01559628526639,-3.69717978381041));
#31337=CARTESIAN_POINT('',(-6.76699860320916,0.00434789205820069,91.6971797838561));
#31338=CARTESIAN_POINT('Ctrl Pts',(-6.76699860320916,0.00434789205818717,
91.6971797838561));
#31339=CARTESIAN_POINT('Ctrl Pts',(-6.76710755774317,-0.165227426188215,
91.705162465091));
#31340=CARTESIAN_POINT('Ctrl Pts',(-6.76083819870497,-0.335012369902362,
91.713145146326));
#31341=CARTESIAN_POINT('Ctrl Pts',(-6.74816981568796,-0.504473129748143,
91.7211278275609));
#31342=CARTESIAN_POINT('Ctrl Pts',(-6.73550943926403,-0.673826788052786,
91.729105463631));
#31343=CARTESIAN_POINT('Ctrl Pts',(-6.71645811032625,-0.842856292913908,
91.7370830997012));
#31344=CARTESIAN_POINT('Ctrl Pts',(-6.69104717862425,-1.01102752357418,
91.7450607357713));
#31345=CARTESIAN_POINT('Ctrl Pts',(-6.66564677156446,-1.17912910145453,
91.7530350676821));
#31346=CARTESIAN_POINT('Ctrl Pts',(-6.63389205724408,-1.34637273726657,
91.7610093995929));
#31347=CARTESIAN_POINT('Ctrl Pts',(-6.5958662380544,-1.51222933766481,91.7689837315038));
#31348=CARTESIAN_POINT('Ctrl Pts',(-6.56921624055413,-1.62846820063229,
91.774572458585));
#31349=CARTESIAN_POINT('Ctrl Pts',(-6.53948711408368,-1.74402586995437,
91.7801611856661));
#31350=CARTESIAN_POINT('Ctrl Pts',(-6.50672250975899,-1.85872299738174,
91.7857499127473));
#31351=CARTESIAN_POINT('Ctrl Pts',(-6.45633174716039,-2.03512298261142,
91.7943451705074));
#31352=CARTESIAN_POINT('Ctrl Pts',(-6.39879310470646,-2.2093686632292,91.8029404282674));
#31353=CARTESIAN_POINT('Ctrl Pts',(-6.33432507402493,-2.3808853094131,91.8115356860274));
#31354=CARTESIAN_POINT('Ctrl Pts',(-6.26979667176679,-2.55256257366203,
91.8201389928819));
#31355=CARTESIAN_POINT('Ctrl Pts',(-6.19832603626417,-2.72150541652671,
91.8287422997363));
#31356=CARTESIAN_POINT('Ctrl Pts',(-6.12017936261071,-2.88716012189728,
91.8373456065907));
#31357=CARTESIAN_POINT('Ctrl Pts',(-6.0387927007682,-3.05968292879758,91.8463056095307));
#31358=CARTESIAN_POINT('Ctrl Pts',(-5.95016479774376,-3.22863879470019,
91.8552656124707));
#31359=CARTESIAN_POINT('Ctrl Pts',(-5.85464789181539,-3.3934329318349,91.8642256154107));
#31360=CARTESIAN_POINT('Ctrl Pts',(-5.76268259042405,-3.55209952956248,
91.8728524586155));
#31361=CARTESIAN_POINT('Ctrl Pts',(-5.66433155353296,-3.70690808393633,
91.8814793018202));
#31362=CARTESIAN_POINT('Ctrl Pts',(-5.55995238299365,-3.85735900569849,
91.8901061450249));
#31363=CARTESIAN_POINT('Ctrl Pts',(-5.45547345235264,-4.00795372051034,
91.898741233311));
#31364=CARTESIAN_POINT('Ctrl Pts',(-5.34495506920274,-4.15418224439382,
91.9073763215971));
#31365=CARTESIAN_POINT('Ctrl Pts',(-5.22879527599012,-4.29557783793792,
91.9160114098832));
#31366=CARTESIAN_POINT('Ctrl Pts',(-5.11246296217296,-4.43718343231452,
91.9246593230084));
#31367=CARTESIAN_POINT('Ctrl Pts',(-4.99047269463205,-4.57394152202166,
91.9333072361335));
#31368=CARTESIAN_POINT('Ctrl Pts',(-4.86326053704181,-4.70542091091242,
91.9419551492587));
#31369=CARTESIAN_POINT('Ctrl Pts',(-4.8489892695319,-4.72017089681348,91.9429253134627));
#31370=CARTESIAN_POINT('Ctrl Pts',(-4.83465231767785,-4.73485448880977,
91.9438954776668));
#31371=CARTESIAN_POINT('Ctrl Pts',(-4.82025032355627,-4.74947110931898,
91.9448656418708));
#31372=CARTESIAN_POINT('Ctrl Pts',(-4.69815574864879,-4.87338520431105,
91.9530903213896));
#31373=CARTESIAN_POINT('Ctrl Pts',(-4.57111901890713,-4.99275154831081,
91.9613150009084));
#31374=CARTESIAN_POINT('Ctrl Pts',(-4.43951248728886,-5.10715359816075,
91.9695396804272));
#31375=CARTESIAN_POINT('Ctrl Pts',(-4.30804428902431,-5.2214353985137,91.9777557148773));
#31376=CARTESIAN_POINT('Ctrl Pts',(-4.17201612238669,-5.33076306246661,
91.9859717493275));
#31377=CARTESIAN_POINT('Ctrl Pts',(-4.0318381286734,-5.43475577226571,91.9941877837776));
#31378=CARTESIAN_POINT('Ctrl Pts',(-3.89177939999142,-5.53866000388458,
92.0023968279322));
#31379=CARTESIAN_POINT('Ctrl Pts',(-3.74757816231607,-5.63723810903598,
92.0106058720868));
#31380=CARTESIAN_POINT('Ctrl Pts',(-3.59967874351923,-5.73014850972083,
92.0188149162414));
#31381=CARTESIAN_POINT('Ctrl Pts',(-3.45187554308325,-5.82299846604062,
92.0270186198694));
#31382=CARTESIAN_POINT('Ctrl Pts',(-3.3003792563041,-5.91018787252385,92.0352223234975));
#31383=CARTESIAN_POINT('Ctrl Pts',(-3.14566446671059,-5.99141753367885,
92.0434260271255));
#31384=CARTESIAN_POINT('Ctrl Pts',(-2.99101935473563,-6.07261061210405,
92.0516260361195));
#31385=CARTESIAN_POINT('Ctrl Pts',(-2.83315894441096,-6.14784912628321,
92.0598260451135));
#31386=CARTESIAN_POINT('Ctrl Pts',(-2.67258385337681,-6.21687900370191,
92.0680260541075));
#31387=CARTESIAN_POINT('Ctrl Pts',(-2.51202160226596,-6.28590336134585,
92.0762254074114));
#31388=CARTESIAN_POINT('Ctrl Pts',(-2.34874542839318,-6.34871992161912,
92.0844247607154));
#31389=CARTESIAN_POINT('Ctrl Pts',(-2.18327778105369,-6.40512194503409,
92.0926241140193));
#31390=CARTESIAN_POINT('Ctrl Pts',(-2.01781121251409,-6.46152360072463,
92.1008234138659));
#31391=CARTESIAN_POINT('Ctrl Pts',(-1.85015353795974,-6.51151068615962,
92.1090227137125));
#31392=CARTESIAN_POINT('Ctrl Pts',(-1.68084417487681,-6.55492577073018,
92.1172220135591));
#31393=CARTESIAN_POINT('Ctrl Pts',(-1.51150520126126,-6.59834844816954,
92.1254227473822));
#31394=CARTESIAN_POINT('Ctrl Pts',(-1.34051431089039,-6.63519674574834,
92.1336234812052));
#31395=CARTESIAN_POINT('Ctrl Pts',(-1.1684230211126,-6.66536395433394,92.1418242150282));
#31396=CARTESIAN_POINT('Ctrl Pts',(-0.996270414882502,-6.69554191155306,
92.1500278707882));
#31397=CARTESIAN_POINT('Ctrl Pts',(-0.823016981123086,-6.71903397586791,
92.1582315265482));
#31398=CARTESIAN_POINT('Ctrl Pts',(-0.649221352251423,-6.73578507939356,
92.1664351823083));
#31399=CARTESIAN_POINT('Ctrl Pts',(-0.475226629315058,-6.75255537238508,
92.1746482358833));
#31400=CARTESIAN_POINT('Ctrl Pts',(-0.300688827600502,-6.76256924240023,
92.1828612894583));
#31401=CARTESIAN_POINT('Ctrl Pts',(-0.126169665710542,-6.76582369083429,
92.1910743430333));
#31402=CARTESIAN_POINT('Ctrl Pts',(0.0484527630829802,-6.7690800649985,
92.1992922564564));
#31403=CARTESIAN_POINT('Ctrl Pts',(0.223056172214694,-6.76556905187751,
92.2075101698795));
#31404=CARTESIAN_POINT('Ctrl Pts',(0.397082068574533,-6.75533972726884,
92.2157280833026));
#31405=CARTESIAN_POINT('Ctrl Pts',(0.571379386630653,-6.74509444836431,
92.2239588138986));
#31406=CARTESIAN_POINT('Ctrl Pts',(0.745097035285941,-6.72810995271888,
92.2321895444946));
#31407=CARTESIAN_POINT('Ctrl Pts',(0.917683489713388,-6.70448700593173,
92.2404202750906));
#31408=CARTESIAN_POINT('Ctrl Pts',(1.07618350715472,-6.68279215455884,92.2479792167663));
#31409=CARTESIAN_POINT('Ctrl Pts',(1.23372935843241,-6.65549892256677,92.2555381584418));
#31410=CARTESIAN_POINT('Ctrl Pts',(1.38990473063026,-6.62272253984505,92.2630971001175));
#31411=CARTESIAN_POINT('Ctrl Pts',(1.55837238108287,-6.58736638791305,92.2712509922842));
#31412=CARTESIAN_POINT('Ctrl Pts',(1.72576603746152,-6.54551994726072,92.2794048844509));
#31413=CARTESIAN_POINT('Ctrl Pts',(1.8915416762854,-6.49725781286809,92.2875587766177));
#31414=CARTESIAN_POINT('Ctrl Pts',(2.05711502251477,-6.44905457176311,92.2957027187579));
#31415=CARTESIAN_POINT('Ctrl Pts',(2.22107393415481,-6.39445132170594,92.3038466608981));
#31416=CARTESIAN_POINT('Ctrl Pts',(2.38288268948448,-6.33357395852888,92.3119906030383));
#31417=CARTESIAN_POINT('Ctrl Pts',(2.54452805044158,-6.27275806927232,92.3201263214312));
#31418=CARTESIAN_POINT('Ctrl Pts',(2.70402723791533,-6.20568080760949,92.3282620398241));
#31419=CARTESIAN_POINT('Ctrl Pts',(2.86085785998917,-6.13251834933563,92.336397758217));
#31420=CARTESIAN_POINT('Ctrl Pts',(3.0175631039645,-6.05941438072265,92.3445269725172));
#31421=CARTESIAN_POINT('Ctrl Pts',(3.17160370050919,-5.98023505569614,92.3526561868174));
#31422=CARTESIAN_POINT('Ctrl Pts',(3.32247548881616,-5.89520530823277,92.3607854011176));
#31423=CARTESIAN_POINT('Ctrl Pts',(3.47325838547474,-5.81022565916419,92.368909825793));
#31424=CARTESIAN_POINT('Ctrl Pts',(3.62087587424615,-5.71940263127901,92.3770342504684));
#31425=CARTESIAN_POINT('Ctrl Pts',(3.76484674977185,-5.62300790953848,92.3851586751439));
#31426=CARTESIAN_POINT('Ctrl Pts',(3.90969162067757,-5.52602801012816,92.393332420278));
#31427=CARTESIAN_POINT('Ctrl Pts',(4.0508451187565,-5.42340870668908,92.4015061654122));
#31428=CARTESIAN_POINT('Ctrl Pts',(4.18784475117516,-5.31547225936272,92.4096799105464));
#31429=CARTESIAN_POINT('Ctrl Pts',(4.32396707803633,-5.20822700546093,92.4178013134085));
#31430=CARTESIAN_POINT('Ctrl Pts',(4.45598830744837,-5.09573275470312,92.4259227162707));
#31431=CARTESIAN_POINT('Ctrl Pts',(4.58348636821586,-4.97834728724095,92.4340441191328));
#31432=CARTESIAN_POINT('Ctrl Pts',(4.71099428646251,-4.86095274415214,92.4421661498991));
#31433=CARTESIAN_POINT('Ctrl Pts',(4.83397807019475,-4.73866647895501,92.4502881806654));
#31434=CARTESIAN_POINT('Ctrl Pts',(4.9520512544675,-4.61188436250595,92.4584102114316));
#31435=CARTESIAN_POINT('Ctrl Pts',(5.07015605139785,-4.48506830168872,92.4665344167727));
#31436=CARTESIAN_POINT('Ctrl Pts',(5.18334738163508,-4.35375426053406,92.4746586221139));
#31437=CARTESIAN_POINT('Ctrl Pts',(5.29127797625718,-4.21837247975754,92.482782827455));
#31438=CARTESIAN_POINT('Ctrl Pts',(5.40037684488427,-4.08152528488055,92.4909949716974));
#31439=CARTESIAN_POINT('Ctrl Pts',(5.5041001850742,-3.94052207444959,92.4992071159399));
#31440=CARTESIAN_POINT('Ctrl Pts',(5.60213377838816,-3.79583800089551,92.5074192601824));
#31441=CARTESIAN_POINT('Ctrl Pts',(5.69927243304204,-3.65247473347069,92.5155564365988));
#31442=CARTESIAN_POINT('Ctrl Pts',(5.79082465098,-3.50549787138021,92.5236936130153));
#31443=CARTESIAN_POINT('Ctrl Pts',(5.87653081531274,-3.35539484661341,92.5318307894317));
#31444=CARTESIAN_POINT('Ctrl Pts',(5.96342139629414,-3.20321747255176,92.5400804175872));
#31445=CARTESIAN_POINT('Ctrl Pts',(6.04430298011276,-3.04782724715359,92.5483300457426));
#31446=CARTESIAN_POINT('Ctrl Pts',(6.11895548514497,-2.88975306398562,92.5565796738981));
#31447=CARTESIAN_POINT('Ctrl Pts',(6.19360799017718,-2.73167888081765,92.5648293020535));
#31448=CARTESIAN_POINT('Ctrl Pts',(6.2620313239398,-2.57092111869645,92.573078930209));
#31449=CARTESIAN_POINT('Ctrl Pts',(6.32405790722228,-2.40802420795542,92.5813285583644));
#31450=CARTESIAN_POINT('Ctrl Pts',(6.38589832358761,-2.24561621686919,92.589553426042));
#31451=CARTESIAN_POINT('Ctrl Pts',(6.44156534305441,-2.08059650627191,92.5977782937196));
#31452=CARTESIAN_POINT('Ctrl Pts',(6.49083224066949,-1.9134748034624,92.6060031613972));
#31453=CARTESIAN_POINT('Ctrl Pts',(6.54004363360991,-1.74654138195722,92.6142187628407));
#31454=CARTESIAN_POINT('Ctrl Pts',(6.58286916202593,-1.57751102478036,92.6224343642843));
#31455=CARTESIAN_POINT('Ctrl Pts',(6.61913014855371,-1.4069133152072,92.6306499657278));
#31456=CARTESIAN_POINT('Ctrl Pts',(6.65535756858123,-1.23647352654609,92.6388579620559));
#31457=CARTESIAN_POINT('Ctrl Pts',(6.68503247455617,-1.06446962367575,92.6470659583841));
#31458=CARTESIAN_POINT('Ctrl Pts',(6.70802597368386,-0.891446317162547,
92.6552739547122));
#31459=CARTESIAN_POINT('Ctrl Pts',(6.73100280628052,-0.718548424284471,
92.6634760015837));
#31460=CARTESIAN_POINT('Ctrl Pts',(6.74730783115768,-0.54463295371733,92.6716780484551));
#31461=CARTESIAN_POINT('Ctrl Pts',(6.75686320228404,-0.370254865761249,
92.6798800953266));
#31462=CARTESIAN_POINT('Ctrl Pts',(6.76641356613106,-0.195968156757047,
92.6880778440982));
#31463=CARTESIAN_POINT('Ctrl Pts',(6.76922130292415,-0.0212196706970898,
92.6962755928698));
#31464=CARTESIAN_POINT('Ctrl Pts',(6.76526038851042,0.153430360919473,92.7044733416414));
#31465=CARTESIAN_POINT('Ctrl Pts',(6.76130022956156,0.328047081550108,92.712669526857));
#31466=CARTESIAN_POINT('Ctrl Pts',(6.75057399279243,0.502565026684469,92.7208657120726));
#31467=CARTESIAN_POINT('Ctrl Pts',(6.7331077703053,0.676423501553901,92.7290618972882));
#31468=CARTESIAN_POINT('Ctrl Pts',(6.71564283992992,0.850269114765363,92.7372574761686));
#31469=CARTESIAN_POINT('Ctrl Pts',(6.69143895180731,1.02345499775442,92.7454530550489));
#31470=CARTESIAN_POINT('Ctrl Pts',(6.66057412388875,1.19542517130248,92.7536486339292));
#31471=CARTESIAN_POINT('Ctrl Pts',(6.62970596379054,1.36741391082199,92.7618450976076));
#31472=CARTESIAN_POINT('Ctrl Pts',(6.59217549459628,1.53818632615473,92.7700415612861));
#31473=CARTESIAN_POINT('Ctrl Pts',(6.54811195748699,1.70719617859692,92.7782380249646));
#31474=CARTESIAN_POINT('Ctrl Pts',(6.50403564638775,1.87625502688235,92.7864368647923));
#31475=CARTESIAN_POINT('Ctrl Pts',(6.45342258540803,2.04354994736245,92.7946357046201));
#31476=CARTESIAN_POINT('Ctrl Pts',(6.39645203796197,2.20854937143187,92.8028345444479));
#31477=CARTESIAN_POINT('Ctrl Pts',(6.33942198315822,2.37372114209419,92.8110419481971));
#31478=CARTESIAN_POINT('Ctrl Pts',(6.27602129215305,2.53659228639573,92.8192493519463));
#31479=CARTESIAN_POINT('Ctrl Pts',(6.20647796789813,2.69664981671614,92.8274567556956));
#31480=CARTESIAN_POINT('Ctrl Pts',(6.13689739255857,2.85679308231987,92.8356685557646));
#31481=CARTESIAN_POINT('Ctrl Pts',(6.06116778011801,3.01411940644195,92.8438803558336));
#31482=CARTESIAN_POINT('Ctrl Pts',(5.97956331682157,3.16814007583657,92.8520921559027));
#31483=CARTESIAN_POINT('Ctrl Pts',(5.89783872035261,3.32238748517779,92.8603160448888));
#31484=CARTESIAN_POINT('Ctrl Pts',(5.81022216919037,3.47331920411975,92.868539933875));
#31485=CARTESIAN_POINT('Ctrl Pts',(5.71703212125234,3.62047410218178,92.8767638228611));
#31486=CARTESIAN_POINT('Ctrl Pts',(5.63092612801164,3.75644268400171,92.8843625541111));
#31487=CARTESIAN_POINT('Ctrl Pts',(5.54006239522148,3.88918697978357,92.8919612853611));
#31488=CARTESIAN_POINT('Ctrl Pts',(5.44472225972871,4.01836888729926,92.8995600166111));
#31489=CARTESIAN_POINT('Ctrl Pts',(5.34152069359962,4.15820270547307,92.9077853139797));
#31490=CARTESIAN_POINT('Ctrl Pts',(5.23278390163382,4.29425453053385,92.9160106113483));
#31491=CARTESIAN_POINT('Ctrl Pts',(5.11881819253714,4.42605798784323,92.9242359087169));
#31492=CARTESIAN_POINT('Ctrl Pts',(5.00497706538544,4.5577173638215,92.9324522145779));
#31493=CARTESIAN_POINT('Ctrl Pts',(4.88591863435858,4.68513734956562,92.9406685204389));
#31494=CARTESIAN_POINT('Ctrl Pts',(4.76199193154249,4.80788122190266,92.9488848262999));
#31495=CARTESIAN_POINT('Ctrl Pts',(4.63820337581851,4.93048826570596,92.9570919730471));
#31496=CARTESIAN_POINT('Ctrl Pts',(4.50955761656096,5.04842933320243,92.9652991197944));
#31497=CARTESIAN_POINT('Ctrl Pts',(4.3764431142717,5.16130164469621,92.9735062665417));
#31498=CARTESIAN_POINT('Ctrl Pts',(4.24341509065272,5.27410062798577,92.9817080814646));
#31499=CARTESIAN_POINT('Ctrl Pts',(4.10592437625008,5.38183718013761,92.9899098963876));
#31500=CARTESIAN_POINT('Ctrl Pts',(3.96439573176304,5.48414582975134,92.9981117113106));
#31501=CARTESIAN_POINT('Ctrl Pts',(3.82293398255666,5.58640612190461,93.0063096495433));
#31502=CARTESIAN_POINT('Ctrl Pts',(3.6774383938496,5.68324341060657,93.0145075877761));
#31503=CARTESIAN_POINT('Ctrl Pts',(3.52836624268282,5.77433291883108,93.0227055260089));
#31504=CARTESIAN_POINT('Ctrl Pts',(3.38832450469249,5.85990445546354,93.0304068539166));
#31505=CARTESIAN_POINT('Ctrl Pts',(3.24512688595244,5.94040370281804,93.0381081818244));
#31506=CARTESIAN_POINT('Ctrl Pts',(3.09917575053244,6.01559628526647,93.0458095097322));
#31507=CARTESIAN_POINT('Ctrl Pts',(3.09917575053275,6.01559628526631,91.0459618091817));
#31508=CARTESIAN_POINT('Ctrl Pts',(2.94553883644237,6.0947485049227,91.0540936986117));
#31509=CARTESIAN_POINT('Ctrl Pts',(2.78871399936926,6.16809025739574,91.0622255880417));
#31510=CARTESIAN_POINT('Ctrl Pts',(2.62918527808529,6.23535674789338,91.0703574774717));
#31511=CARTESIAN_POINT('Ctrl Pts',(2.46976524118543,6.30257741079941,91.0784838267746));
#31512=CARTESIAN_POINT('Ctrl Pts',(2.30764532394961,6.3637309118955,91.0866101760775));
#31513=CARTESIAN_POINT('Ctrl Pts',(2.14333295264033,6.4185989790706,91.0947365253803));
#31514=CARTESIAN_POINT('Ctrl Pts',(1.9790979820844,6.47344120017153,91.1028590466966));
#31515=CARTESIAN_POINT('Ctrl Pts',(1.81267296063862,6.52200376861243,91.1109815680128));
#31516=CARTESIAN_POINT('Ctrl Pts',(1.64458401674675,6.56411703215757,91.1191040893291));
#31517=CARTESIAN_POINT('Ctrl Pts',(1.47651046575417,6.60622643914196,91.127225866818));
#31518=CARTESIAN_POINT('Ctrl Pts',(1.30677364815761,6.64188761962794,91.135347644307));
#31519=CARTESIAN_POINT('Ctrl Pts',(1.1359137972616,6.6709811006471,91.1434694217959));
#31520=CARTESIAN_POINT('Ctrl Pts',(0.965054922794803,6.70007441540294,91.1515911528705));
#31521=CARTESIAN_POINT('Ctrl Pts',(0.793073388439417,6.72260004293741,91.1597128839451));
#31522=CARTESIAN_POINT('Ctrl Pts',(0.620518326237572,6.7384898906805,91.1678346150197));
#31523=CARTESIAN_POINT('Ctrl Pts',(0.447931392235734,6.75438267335951,91.1759578462195));
#31524=CARTESIAN_POINT('Ctrl Pts',(0.274771083864169,6.76363720173535,91.1840810774192));
#31525=CARTESIAN_POINT('Ctrl Pts',(0.10159029898932,6.76623738950617,91.192204308619));
#31526=CARTESIAN_POINT('Ctrl Pts',(-0.0716554527820409,6.76883855270928,
91.200330587161));
#31527=CARTESIAN_POINT('Ctrl Pts',(-0.244921330711114,6.76478039895497,
91.208456865703));
#31528=CARTESIAN_POINT('Ctrl Pts',(-0.417655840659719,6.7540989479547,91.216583144245));
#31529=CARTESIAN_POINT('Ctrl Pts',(-0.590591764695115,6.7434050420333,91.2247188982935));
#31530=CARTESIAN_POINT('Ctrl Pts',(-0.76299471772106,6.72607243599861,91.232854652342));
#31531=CARTESIAN_POINT('Ctrl Pts',(-0.934318782378692,6.70218900157959,
91.2409904063905));
#31532=CARTESIAN_POINT('Ctrl Pts',(-1.10574976822514,6.67829066181026,91.2491312378605));
#31533=CARTESIAN_POINT('Ctrl Pts',(-1.27610016491944,6.64783341229592,91.2572720693306));
#31534=CARTESIAN_POINT('Ctrl Pts',(-1.44483593130785,6.61095591662823,91.2654129008006));
#31535=CARTESIAN_POINT('Ctrl Pts',(-1.61383281245392,6.57402135387541,91.273566330022));
#31536=CARTESIAN_POINT('Ctrl Pts',(-1.78120971858682,6.5306467894196,91.2817197592434));
#31537=CARTESIAN_POINT('Ctrl Pts',(-1.94644830628421,6.48102059794315,91.2898731884649));
#31538=CARTESIAN_POINT('Ctrl Pts',(-2.07162240693606,6.44342699481808,91.2960497007689));
#31539=CARTESIAN_POINT('Ctrl Pts',(-2.19556975145639,6.40224685692166,91.302226213073));
#31540=CARTESIAN_POINT('Ctrl Pts',(-2.31807371444179,6.35757998411456,91.3084027253771));
#31541=CARTESIAN_POINT('Ctrl Pts',(-2.48134137206542,6.29805002672488,91.3166344974079));
#31542=CARTESIAN_POINT('Ctrl Pts',(-2.64255407483943,6.2321393772728,91.3248662694387));
#31543=CARTESIAN_POINT('Ctrl Pts',(-2.80117716484146,6.16000775090184,91.3330980414696));
#31544=CARTESIAN_POINT('Ctrl Pts',(-2.95961084302233,6.0879622569011,91.341319983942));
#31545=CARTESIAN_POINT('Ctrl Pts',(-3.11546074286904,6.00971072463719,91.3495419264144));
#31546=CARTESIAN_POINT('Ctrl Pts',(-3.26820835388604,5.92546227357744,91.3577638688868));
#31547=CARTESIAN_POINT('Ctrl Pts',(-3.42080417331779,5.84129754366957,91.3659776408767));
#31548=CARTESIAN_POINT('Ctrl Pts',(-3.57030353185832,5.75114793491385,91.3741914128666));
#31549=CARTESIAN_POINT('Ctrl Pts',(-3.71620878461308,5.65527022070251,91.3824051848565));
#31550=CARTESIAN_POINT('Ctrl Pts',(-3.86199826809607,5.55946858115568,91.3906124395868));
#31551=CARTESIAN_POINT('Ctrl Pts',(-4.00419902778808,5.45794808468295,91.3988196943172));
#31552=CARTESIAN_POINT('Ctrl Pts',(-4.14233880762939,5.3510109514752,91.4070269490475));
#31553=CARTESIAN_POINT('Ctrl Pts',(-4.28039664000968,5.24413725565359,91.4152293350595));
#31554=CARTESIAN_POINT('Ctrl Pts',(-4.41439800909446,5.13185354304999,91.4234317210715));
#31555=CARTESIAN_POINT('Ctrl Pts',(-4.54390033169494,5.01450483852819,91.4316341070834));
#31556=CARTESIAN_POINT('Ctrl Pts',(-4.67336400099337,4.89719115974824,91.4398340448821));
#31557=CARTESIAN_POINT('Ctrl Pts',(-4.79833103093333,4.77481573787114,91.4480339826808));
#31558=CARTESIAN_POINT('Ctrl Pts',(-4.91839239984003,4.64776346226826,91.4562339204795));
#31559=CARTESIAN_POINT('Ctrl Pts',(-5.03843698106842,4.52072895185289,91.4644327117152));
#31560=CARTESIAN_POINT('Ctrl Pts',(-5.15357702071807,4.38901914998786,91.472631502951));
#31561=CARTESIAN_POINT('Ctrl Pts',(-5.26344081228832,4.25305535063179,91.4808302941867));
#31562=CARTESIAN_POINT('Ctrl Pts',(-5.37330917192722,4.11708589798484,91.4890294263232));
#31563=CARTESIAN_POINT('Ctrl Pts',(-5.47790062107777,3.97686237421657,91.4972285584596));
#31564=CARTESIAN_POINT('Ctrl Pts',(-5.57688413055956,3.83283868618456,91.505427690596));
#31565=CARTESIAN_POINT('Ctrl Pts',(-5.67588971177063,3.68878288318846,91.5136286510069));
#31566=CARTESIAN_POINT('Ctrl Pts',(-5.76928465974368,3.54092552353243,91.5218296114178));
#31567=CARTESIAN_POINT('Ctrl Pts',(-5.85678158973804,3.38974901874837,91.5300305718287));
#31568=CARTESIAN_POINT('Ctrl Pts',(-5.94436052541906,3.23843082518641,91.5382392185137));
#31569=CARTESIAN_POINT('Ctrl Pts',(-6.02603021900859,3.08378758185689,91.5464478651988));
#31570=CARTESIAN_POINT('Ctrl Pts',(-6.10154909944083,2.9263266371191,91.5546565118838));
#31571=CARTESIAN_POINT('Ctrl Pts',(-6.17710403470759,2.76879051610389,91.5628690776073));
#31572=CARTESIAN_POINT('Ctrl Pts',(-6.24650215950944,2.60843434025241,91.5710816433308));
#31573=CARTESIAN_POINT('Ctrl Pts',(-6.30955034489675,2.44578483215784,91.5792942090543));
#31574=CARTESIAN_POINT('Ctrl Pts',(-6.37268504149231,2.28291214546774,91.5875180436031));
#31575=CARTESIAN_POINT('Ctrl Pts',(-6.42945226869713,2.11774017661858,91.5957418781519));
#31576=CARTESIAN_POINT('Ctrl Pts',(-6.4797086371863,1.95081136381079,91.6039657127007));
#31577=CARTESIAN_POINT('Ctrl Pts',(-6.5258847861613,1.79743518562366,91.6115218696751));
#31578=CARTESIAN_POINT('Ctrl Pts',(-6.56656490163375,1.64257621069006,91.6190780266495));
#31579=CARTESIAN_POINT('Ctrl Pts',(-6.60167606144956,1.48666142066172,91.626634183624));
#31580=CARTESIAN_POINT('Ctrl Pts',(-6.65093877381793,1.26790517633836,91.6372358495785));
#31581=CARTESIAN_POINT('Ctrl Pts',(-6.68933642560366,1.046644544309,91.647837515533));
#31582=CARTESIAN_POINT('Ctrl Pts',(-6.71666652858663,0.82382021325287,91.6584391814875));
#31583=CARTESIAN_POINT('Ctrl Pts',(-6.74363790641983,0.603920594613034,
91.6689016937692));
#31584=CARTESIAN_POINT('Ctrl Pts',(-6.75983039058453,0.382497848912048,
91.6793642060509));
#31585=CARTESIAN_POINT('Ctrl Pts',(-6.76509698605697,0.160473578021119,
91.6898267183326));
#31586=CARTESIAN_POINT('Ctrl Pts',(-6.76633077581058,0.108460608368888,
91.6922777401583));
#31587=CARTESIAN_POINT('Ctrl Pts',(-6.76696514953633,0.0564147104294671,
91.6947287619841));
#31588=CARTESIAN_POINT('Ctrl Pts',(-6.76699860320852,0.00434789304140347,
91.6971797838098));
#31589=CARTESIAN_POINT('',(-6.76699927988566,0.00165422498013631,91.3028202161897));
#31590=CARTESIAN_POINT('Ctrl Pts',(3.09917575053247,6.01559628526645,90.6515381108923));
#31591=CARTESIAN_POINT('Ctrl Pts',(2.94407804857715,6.09550108839304,90.6597408227342));
#31592=CARTESIAN_POINT('Ctrl Pts',(2.785778374465,6.1694603469633,90.6679435345761));
#31593=CARTESIAN_POINT('Ctrl Pts',(2.62477392534936,6.23721499074756,90.6761462464181));
#31594=CARTESIAN_POINT('Ctrl Pts',(2.46384860630333,6.30493633464659,90.6843449268114));
#31595=CARTESIAN_POINT('Ctrl Pts',(2.30022149045008,6.36645900014936,90.6925436072047));
#31596=CARTESIAN_POINT('Ctrl Pts',(2.13441204498966,6.42157100888895,90.700742287598));
#31597=CARTESIAN_POINT('Ctrl Pts',(1.9686274665221,6.47667475229767,90.708939738408));
#31598=CARTESIAN_POINT('Ctrl Pts',(1.8006615482882,6.52536963460475,90.7171371892181));
#31599=CARTESIAN_POINT('Ctrl Pts',(1.63105160857606,6.56749264561152,90.7253346400281));
#31600=CARTESIAN_POINT('Ctrl Pts',(1.46144929665274,6.60961376223974,90.733531722178));
#31601=CARTESIAN_POINT('Ctrl Pts',(1.29020345843443,6.64516350893887,90.7417288043278));
#31602=CARTESIAN_POINT('Ctrl Pts',(1.11786430112426,6.67402939791787,90.7499258864777));
#31603=CARTESIAN_POINT('Ctrl Pts',(0.945501571982807,6.7028992350528,90.7581240897903));
#31604=CARTESIAN_POINT('Ctrl Pts',(0.77204557966371,6.72508333402019,90.7663222931029));
#31605=CARTESIAN_POINT('Ctrl Pts',(0.598054450501333,6.74052074206701,90.7745204964155));
#31606=CARTESIAN_POINT('Ctrl Pts',(0.424007900805846,6.75596306731499,90.7827213110612));
#31607=CARTESIAN_POINT('Ctrl Pts',(0.249426231884836,6.76465438943605,90.7909221257069));
#31608=CARTESIAN_POINT('Ctrl Pts',(0.074870443341808,6.76658580206546,90.7991229403526));
#31609=CARTESIAN_POINT('Ctrl Pts',(-0.0998690993695105,6.76851924788508,
90.8073323879625));
#31610=CARTESIAN_POINT('Ctrl Pts',(-0.274582348242346,6.76367856474909,
90.8155418355725));
#31611=CARTESIAN_POINT('Ctrl Pts',(-0.448709576780406,6.75210698343158,
90.8237512831824));
#31612=CARTESIAN_POINT('Ctrl Pts',(-0.622934508067399,6.7405289093024,90.8319653371116));
#31613=CARTESIAN_POINT('Ctrl Pts',(-0.796572407360125,6.72221244597446,
90.8401793910407));
#31614=CARTESIAN_POINT('Ctrl Pts',(-0.969071009046813,6.69725245002942,
90.8483934449698));
#31615=CARTESIAN_POINT('Ctrl Pts',(-1.14181493237204,6.67225695682791,90.8566191806468));
#31616=CARTESIAN_POINT('Ctrl Pts',(-1.31341596828111,6.64059911777658,90.8648449163238));
#31617=CARTESIAN_POINT('Ctrl Pts',(-1.48333318655589,6.60242468019606,90.8730706520008));
#31618=CARTESIAN_POINT('Ctrl Pts',(-1.61159264329477,6.57360928011416,90.8792797248653));
#31619=CARTESIAN_POINT('Ctrl Pts',(-1.73889295021271,6.5410819312111,90.8854887977298));
#31620=CARTESIAN_POINT('Ctrl Pts',(-1.86500840206443,6.50492372439747,90.8916978705944));
#31621=CARTESIAN_POINT('Ctrl Pts',(-2.03209470965791,6.457018878663,90.8999240716132));
#31622=CARTESIAN_POINT('Ctrl Pts',(-2.19756763433466,6.40260523918426,90.9081502726321));
#31623=CARTESIAN_POINT('Ctrl Pts',(-2.3608831728243,6.34180728533082,90.9163764736509));
#31624=CARTESIAN_POINT('Ctrl Pts',(-2.52401526072713,6.28107762516465,90.9245934342667));
#31625=CARTESIAN_POINT('Ctrl Pts',(-2.68499445497847,6.21397805487934,90.9328103948824));
#31626=CARTESIAN_POINT('Ctrl Pts',(-2.84328969871749,6.14068340571039,90.9410273554982));
#31627=CARTESIAN_POINT('Ctrl Pts',(-3.00143890222536,6.06745637681388,90.9492367352998));
#31628=CARTESIAN_POINT('Ctrl Pts',(-3.1569087631929,5.98804580133518,90.9574461151014));
#31629=CARTESIAN_POINT('Ctrl Pts',(-3.3091859943984,5.90267541496883,90.965655494903));
#31630=CARTESIAN_POINT('Ctrl Pts',(-3.46135329092207,5.81736666070723,90.9738589480434));
#31631=CARTESIAN_POINT('Ctrl Pts',(-3.61033223704725,5.72610684029319,90.9820624011838));
#31632=CARTESIAN_POINT('Ctrl Pts',(-3.75563197273801,5.62916667770177,90.9902658543242));
#31633=CARTESIAN_POINT('Ctrl Pts',(-3.90085595782944,5.53227705391815,90.9984650306743));
#31634=CARTESIAN_POINT('Ctrl Pts',(-4.04240425610001,5.42971318614278,91.0066642070245));
#31635=CARTESIAN_POINT('Ctrl Pts',(-4.17981288093117,5.32179042056354,91.0148633833746));
#31636=CARTESIAN_POINT('Ctrl Pts',(-4.31719565025572,5.21388796228148,91.023061016926));
#31637=CARTESIAN_POINT('Ctrl Pts',(-4.45044001211519,5.1006288311366,91.0312586504774));
#31638=CARTESIAN_POINT('Ctrl Pts',(-4.57911287462895,4.98237034767664,91.0394562840288));
#31639=CARTESIAN_POINT('Ctrl Pts',(-4.70777646953871,4.86412038172979,91.0476533271493));
#31640=CARTESIAN_POINT('Ctrl Pts',(-4.8318689561582,4.74087202263994,91.0558503702699));
#31641=CARTESIAN_POINT('Ctrl Pts',(-4.95099216549088,4.61302130682787,91.0640474133905));
#31642=CARTESIAN_POINT('Ctrl Pts',(-5.07012844547349,4.4851565627508,91.0722453559217));
#31643=CARTESIAN_POINT('Ctrl Pts',(-5.18429411731668,4.35268871834763,91.0804432984529));
#31644=CARTESIAN_POINT('Ctrl Pts',(-5.29312953230817,4.21604895064171,91.0886412409841));
#31645=CARTESIAN_POINT('Ctrl Pts',(-5.40199666986208,4.07936935616103,91.0968415729925));
#31646=CARTESIAN_POINT('Ctrl Pts',(-5.50553023251861,3.93851569673618,91.1050419050009));
#31647=CARTESIAN_POINT('Ctrl Pts',(-5.60341231425739,3.79395037347995,91.1132422370094));
#31648=CARTESIAN_POINT('Ctrl Pts',(-5.70139641558099,3.64923437408366,91.1214511159801));
#31649=CARTESIAN_POINT('Ctrl Pts',(-5.79371706655625,3.50079927946118,91.1296599949509));
#31650=CARTESIAN_POINT('Ctrl Pts',(-5.8801004651907,3.3491353390486,91.1378688739216));
#31651=CARTESIAN_POINT('Ctrl Pts',(-5.96653023643713,3.19738998191507,91.146082159609));
#31652=CARTESIAN_POINT('Ctrl Pts',(-6.04701623628843,3.04241264156358,91.1542954452964));
#31653=CARTESIAN_POINT('Ctrl Pts',(-6.12133178471444,2.88471596200471,91.1625087309838));
#31654=CARTESIAN_POINT('Ctrl Pts',(-6.1957560476286,2.72678859163935,91.1707340316959));
#31655=CARTESIAN_POINT('Ctrl Pts',(-6.26399167981509,2.566134262291,91.178959332408));
#31656=CARTESIAN_POINT('Ctrl Pts',(-6.32586062813689,2.40328448448943,91.1871846331201));
#31657=CARTESIAN_POINT('Ctrl Pts',(-6.38181362877759,2.25600650468158,91.1946234254141));
#31658=CARTESIAN_POINT('Ctrl Pts',(-6.43255989262885,2.10693325614759,91.2020622177081));
#31659=CARTESIAN_POINT('Ctrl Pts',(-6.47800353283848,1.95646600495182,91.2095010100021));
#31660=CARTESIAN_POINT('Ctrl Pts',(-6.5388554738026,1.75498073122464,91.2194620286932));
#31661=CARTESIAN_POINT('Ctrl Pts',(-6.59034529481158,1.5505156935588,91.2294230473842));
#31662=CARTESIAN_POINT('Ctrl Pts',(-6.63221952038937,1.34385759415431,91.2393840660753));
#31663=CARTESIAN_POINT('Ctrl Pts',(-6.67382360801738,1.13853268227768,91.2492808244934));
#31664=CARTESIAN_POINT('Ctrl Pts',(-6.70593570481504,0.931042901249972,
91.2591775829115));
#31665=CARTESIAN_POINT('Ctrl Pts',(-6.7283536306715,0.722181708872217,91.2690743413295));
#31666=CARTESIAN_POINT('Ctrl Pts',(-6.75051776729323,0.515684995818658,
91.2788590603573));
#31667=CARTESIAN_POINT('Ctrl Pts',(-6.76320592088888,0.30784775881192,91.288643779385));
#31668=CARTESIAN_POINT('Ctrl Pts',(-6.766269064769,0.0994582482758889,91.2984284984127));
#31669=CARTESIAN_POINT('Ctrl Pts',(-6.76672734614269,0.0682807930567607,
91.2998924043384));
#31670=CARTESIAN_POINT('Ctrl Pts',(-6.76697027192187,0.0370910152686651,
91.3013563102641));
#31671=CARTESIAN_POINT('Ctrl Pts',(-6.7669974352806,0.00589159620233154,
91.3028202161897));
#31672=CARTESIAN_POINT('Ctrl Pts',(-6.767,4.78819593890031E-12,91.3028202161897));
#31673=CARTESIAN_POINT('Ctrl Pts',(-6.76700000000013,-0.18600724941091,
91.3115697279957));
#31674=CARTESIAN_POINT('Ctrl Pts',(-6.75932637295464,-0.372014355522786,
91.3203192398016));
#31675=CARTESIAN_POINT('Ctrl Pts',(-6.74400518266967,-0.557389537150331,
91.3290687516076));
#31676=CARTESIAN_POINT('Ctrl Pts',(-6.72868405709696,-0.742763935806849,
91.3378182264581));
#31677=CARTESIAN_POINT('Ctrl Pts',(-6.70571545653052,-0.927506129690664,
91.3465677013087));
#31678=CARTESIAN_POINT('Ctrl Pts',(-6.6751773941572,-1.11098863924556,91.3553171761592));
#31679=CARTESIAN_POINT('Ctrl Pts',(-6.64463945823145,-1.29447038906274,
91.3640666147812));
#31680=CARTESIAN_POINT('Ctrl Pts',(-6.60653217027203,-1.47669218228016,
91.3728160534032));
#31681=CARTESIAN_POINT('Ctrl Pts',(-6.56098496116756,-1.65703510503947,
91.3815654920252));
#31682=CARTESIAN_POINT('Ctrl Pts',(-6.51543793687555,-1.83737729603889,
91.3903148951454));
#31683=CARTESIAN_POINT('Ctrl Pts',(-6.46245112202668,-2.01584035396964,
91.3990642982657));
#31684=CARTESIAN_POINT('Ctrl Pts',(-6.40220448416259,-2.19181813638095,
91.407813701386));
#31685=CARTESIAN_POINT('Ctrl Pts',(-6.34195808575197,-2.36779521935917,
91.4165630697312));
#31686=CARTESIAN_POINT('Ctrl Pts',(-6.27445201489237,-2.54128677544823,
91.4253124380765));
#31687=CARTESIAN_POINT('Ctrl Pts',(-6.19991555136176,-2.71170355237857,
91.4340618064218));
#31688=CARTESIAN_POINT('Ctrl Pts',(-6.12537937789035,-2.88211966613079,
91.4428111407189));
#31689=CARTESIAN_POINT('Ctrl Pts',(-6.04381298133618,-3.04946076210442,
91.4515604750159));
#31690=CARTESIAN_POINT('Ctrl Pts',(-5.95549339426313,-3.21315848206843,
91.4603098093129));
#31691=CARTESIAN_POINT('Ctrl Pts',(-5.86717414355159,-3.37685557859639,
91.4690591102885));
#31692=CARTESIAN_POINT('Ctrl Pts',(-5.77210188986228,-3.53690907467328,
91.4778084112641));
#31693=CARTESIAN_POINT('Ctrl Pts',(-5.67059953467048,-3.69277536784935,
91.4865577122397));
#31694=CARTESIAN_POINT('Ctrl Pts',(-5.56909755761758,-3.84864108035802,
91.4953069806204));
#31695=CARTESIAN_POINT('Ctrl Pts',(-5.46116568338077,-4.00031938104269,
91.5040562490012));
#31696=CARTESIAN_POINT('Ctrl Pts',(-5.34717048686137,-4.14729511663189,
91.5128055173819));
#31697=CARTESIAN_POINT('Ctrl Pts',(-5.23317570555541,-4.29427031688012,
91.5215547538945));
#31698=CARTESIAN_POINT('Ctrl Pts',(-5.11311782178829,-4.43654275987102,
91.5303039904072));
#31699=CARTESIAN_POINT('Ctrl Pts',(-4.98740459172039,-4.57362924147623,
91.5390532269198));
#31700=CARTESIAN_POINT('Ctrl Pts',(-4.86169180910834,-4.71071523514433,
91.5478024322909));
#31701=CARTESIAN_POINT('Ctrl Pts',(-4.73032391415413,-4.84261509316543,
91.556551637662));
#31702=CARTESIAN_POINT('Ctrl Pts',(-4.5937470723725,-4.96888084331563,91.5653008430332));
#31703=CARTESIAN_POINT('Ctrl Pts',(-4.45717070537355,-5.09514615452766,
91.5740500179894));
#31704=CARTESIAN_POINT('Ctrl Pts',(-4.31538563819458,-5.21577720253675,
91.5827991929456));
#31705=CARTESIAN_POINT('Ctrl Pts',(-4.16887341290592,-5.33036429028693,
91.5915483679019));
#31706=CARTESIAN_POINT('Ctrl Pts',(-4.02236168477282,-5.44495098921219,
91.6002975131698));
#31707=CARTESIAN_POINT('Ctrl Pts',(-3.87112305634381,-5.55349359238799,
91.6090466584377));
#31708=CARTESIAN_POINT('Ctrl Pts',(-3.71567117316673,-5.65562346102512,
91.6177958037056));
#31709=CARTESIAN_POINT('Ctrl Pts',(-3.56021980457233,-5.75775299158811,
91.6265449200118));
#31710=CARTESIAN_POINT('Ctrl Pts',(-3.40055544862311,-5.85346967275398,
91.635294036318));
#31711=CARTESIAN_POINT('Ctrl Pts',(-3.23722036323317,-5.94244842803608,
91.6440431526241));
#31712=CARTESIAN_POINT('Ctrl Pts',(-3.0738858049595,-6.03142689616525,91.6527922406951));
#31713=CARTESIAN_POINT('Ctrl Pts',(-2.90688079257599,-6.11366734484874,
91.661541328766));
#31714=CARTESIAN_POINT('Ctrl Pts',(-2.73677251094495,-6.18889046787355,
91.670290416837));
#31715=CARTESIAN_POINT('Ctrl Pts',(-2.56666476416543,-6.26411335438311,
91.6790394773992));
#31716=CARTESIAN_POINT('Ctrl Pts',(-2.3934540297201,-6.33231884350321,91.6877885379614));
#31717=CARTESIAN_POINT('Ctrl Pts',(-2.21772856473975,-6.39327529621065,
91.6965375985236));
#31718=CARTESIAN_POINT('Ctrl Pts',(-2.04200363768211,-6.454231562321,91.7052866323036));
#31719=CARTESIAN_POINT('Ctrl Pts',(-1.86376426620041,-6.50793874252071,
91.7140356660836));
#31720=CARTESIAN_POINT('Ctrl Pts',(-1.68361578194642,-6.55421443796135,
91.7227846998636));
#31721=CARTESIAN_POINT('Ctrl Pts',(-1.50346783419843,-6.60048999558685,
91.7315337075879));
#31722=CARTESIAN_POINT('Ctrl Pts',(-1.32141106257244,-6.63933404145495,
91.7402827153121));
#31723=CARTESIAN_POINT('Ctrl Pts',(-1.13806375959064,-6.67061465527026,
91.7490317230363));
#31724=CARTESIAN_POINT('Ctrl Pts',(-0.954716987419518,-6.70189517852475,
91.7577807054312));
#31725=CARTESIAN_POINT('Ctrl Pts',(-0.770079973810406,-6.72561226535821,
91.766529687826));
#31726=CARTESIAN_POINT('Ctrl Pts',(-0.584779770553154,-6.74168536939776,
91.7752786702209));
#31727=CARTESIAN_POINT('Ctrl Pts',(-0.391490647554569,-6.7584514394239,
91.784404850897));
#31728=CARTESIAN_POINT('Ctrl Pts',(-0.197480213104954,-6.76689975924025,
91.793531031573));
#31729=CARTESIAN_POINT('Ctrl Pts',(-0.00346532629837374,-6.76699911271707,
91.8026572122491));
#31730=CARTESIAN_POINT('Ctrl Pts',(0.184486595295469,-6.76709536139775,
91.811498199779));
#31731=CARTESIAN_POINT('Ctrl Pts',(0.372442378184638,-6.75935659726773,
91.8203391873089));
#31732=CARTESIAN_POINT('Ctrl Pts',(0.559750217721486,-6.74380965729021,
91.8291801748389));
#31733=CARTESIAN_POINT('Ctrl Pts',(0.745129914457184,-6.7284227571726,91.8379301534366));
#31734=CARTESIAN_POINT('Ctrl Pts',(0.92987465631364,-6.7053877227348,91.8466801320344));
#31735=CARTESIAN_POINT('Ctrl Pts',(1.11335688289726,-6.67478280180751,91.8554301106322));
#31736=CARTESIAN_POINT('Ctrl Pts',(1.29683723118795,-6.64417819418035,91.8641799996571));
#31737=CARTESIAN_POINT('Ctrl Pts',(1.47905480730164,-6.60600390230091,91.872929888682));
#31738=CARTESIAN_POINT('Ctrl Pts',(1.65939064804728,-6.56038959797155,91.881679777707));
#31739=CARTESIAN_POINT('Ctrl Pts',(1.83972470264193,-6.51477574543277,91.8904295800679));
#31740=CARTESIAN_POINT('Ctrl Pts',(2.01817678125785,-6.4617220982012,91.8991793824289));
#31741=CARTESIAN_POINT('Ctrl Pts',(2.19414072347625,-6.40140886724033,91.9079291847898));
#31742=CARTESIAN_POINT('Ctrl Pts',(2.37010298132052,-6.34109621361391,91.9166789033953));
#31743=CARTESIAN_POINT('Ctrl Pts',(2.54357687926878,-6.27352420825985,91.9254286220008));
#31744=CARTESIAN_POINT('Ctrl Pts',(2.71397317789946,-6.19892237325507,91.9341783406063));
#31745=CARTESIAN_POINT('Ctrl Pts',(2.88436790207172,-6.12432122756977,91.9429279783646));
#31746=CARTESIAN_POINT('Ctrl Pts',(3.05168482126224,-6.04269049717433,91.9516776161228));
#31747=CARTESIAN_POINT('Ctrl Pts',(3.21535561997352,-5.95430745234949,91.9604272538811));
#31748=CARTESIAN_POINT('Ctrl Pts',(3.37902496075246,-5.86592519481537,91.9691768137001));
#31749=CARTESIAN_POINT('Ctrl Pts',(3.53904799384842,-5.77079087940252,91.9779263735191));
#31750=CARTESIAN_POINT('Ctrl Pts',(3.69488118814954,-5.66922763747044,91.9866759333381));
#31751=CARTESIAN_POINT('Ctrl Pts',(3.85071304610807,-5.5676652664907,91.9954254181256));
#31752=CARTESIAN_POINT('Ctrl Pts',(4.00235489705947,-5.45967423580729,92.004174902913));
#31753=CARTESIAN_POINT('Ctrl Pts',(4.14929168607638,-5.34562133936341,92.0129243877005));
#31754=CARTESIAN_POINT('Ctrl Pts',(4.29622726385744,-5.23156938308542,92.0216738003638));
#31755=CARTESIAN_POINT('Ctrl Pts',(4.43845763092056,-5.11145583677211,92.030423213027));
#31756=CARTESIAN_POINT('Ctrl Pts',(4.57549970660954,-4.98568866204219,92.0391726256904));
#31757=CARTESIAN_POINT('Ctrl Pts',(4.71254069815292,-4.85992248226164,92.0479219691367));
#31758=CARTESIAN_POINT('Ctrl Pts',(4.84439326931316,-4.72850295734001,92.056671312583));
#31759=CARTESIAN_POINT('Ctrl Pts',(4.97060959434704,-4.59187644221675,92.0654206560293));
#31760=CARTESIAN_POINT('Ctrl Pts',(5.09682496280528,-4.4552509625665,92.0741699331656));
#31761=CARTESIAN_POINT('Ctrl Pts',(5.21740397615858,-4.31341878218304,92.0829192103019));
#31762=CARTESIAN_POINT('Ctrl Pts',(5.33193710451958,-4.16686161438647,92.0916684874382));
#31763=CARTESIAN_POINT('Ctrl Pts',(5.44646940289404,-4.02030550864485,92.1004177011712));
#31764=CARTESIAN_POINT('Ctrl Pts',(5.55495572749684,-3.86902470980106,92.1091669149042));
#31765=CARTESIAN_POINT('Ctrl Pts',(5.65702762491472,-3.71353301465756,92.1179161286371));
#31766=CARTESIAN_POINT('Ctrl Pts',(5.75909881655173,-3.55804239466862,92.1266652818733));
#31767=CARTESIAN_POINT('Ctrl Pts',(5.85475551250803,-3.39834117619517,92.1354144351094));
#31768=CARTESIAN_POINT('Ctrl Pts',(5.94367283728118,-3.23497174691927,92.1441635883455));
#31769=CARTESIAN_POINT('Ctrl Pts',(6.03258957676336,-3.07160339300917,92.152912683991));
#31770=CARTESIAN_POINT('Ctrl Pts',(6.11476689685311,-2.90456712829448,92.1616617796366));
#31771=CARTESIAN_POINT('Ctrl Pts',(6.18992570525289,-2.73443024475842,92.1704108752821));
#31772=CARTESIAN_POINT('Ctrl Pts',(6.26508404388732,-2.56429442462946,92.1791599162431));
#31773=CARTESIAN_POINT('Ctrl Pts',(6.33322384283356,-2.39105828655887,92.1879089572042));
#31774=CARTESIAN_POINT('Ctrl Pts',(6.39411368720077,-2.21531017131953,92.1966579981652));
#31775=CARTESIAN_POINT('Ctrl Pts',(6.45500317120931,-2.03956309619386,92.2054069873476));
#31776=CARTESIAN_POINT('Ctrl Pts',(6.5086426927011,-1.86130434438504,92.21415597653));
#31777=CARTESIAN_POINT('Ctrl Pts',(6.55485008446367,-1.68113930719815,92.2229049657124));
#31778=CARTESIAN_POINT('Ctrl Pts',(6.60199664749432,-1.49731239211713,92.2318317792418));
#31779=CARTESIAN_POINT('Ctrl Pts',(6.64140563640931,-1.31150116499548,92.2407585927711));
#31780=CARTESIAN_POINT('Ctrl Pts',(6.67293772282192,-1.12436255155541,92.2496854063005));
#31781=CARTESIAN_POINT('Ctrl Pts',(6.70384494949887,-0.940932395050179,
92.258435320456));
#31782=CARTESIAN_POINT('Ctrl Pts',(6.72718449348943,-0.756227260505578,
92.2671852346115));
#31783=CARTESIAN_POINT('Ctrl Pts',(6.74287707373942,-0.570874564540583,
92.2759351487671));
#31784=CARTESIAN_POINT('Ctrl Pts',(6.75856934538676,-0.385525513631416,
92.2846848908511));
#31785=CARTESIAN_POINT('Ctrl Pts',(6.76661493004106,-0.199529212417218,
92.293434632935));
#31786=CARTESIAN_POINT('Ctrl Pts',(6.76698649908907,-0.013517438599468,
92.302184375019));
#31787=CARTESIAN_POINT('Ctrl Pts',(6.76735806132387,0.172490924446717,92.3109339566649));
#31788=CARTESIAN_POINT('Ctrl Pts',(6.76005588896284,0.358514472902324,92.3196835383108));
#31789=CARTESIAN_POINT('Ctrl Pts',(6.74510478454577,0.543921359663106,92.3284331199567));
#31790=CARTESIAN_POINT('Ctrl Pts',(6.73015393440677,0.729325093151422,92.3371825527958));
#31791=CARTESIAN_POINT('Ctrl Pts',(6.70755443556883,0.914111900257411,92.3459319856348));
#31792=CARTESIAN_POINT('Ctrl Pts',(6.677383046823,1.09765415591652,92.3546814184739));
#31793=CARTESIAN_POINT('Ctrl Pts',(6.64721213111837,1.28119353391397,92.3634307141352));
#31794=CARTESIAN_POINT('Ctrl Pts',(6.60946960955465,1.46348811672787,92.3721800097965));
#31795=CARTESIAN_POINT('Ctrl Pts',(6.56428366991147,1.64391876348366,92.3809293054578));
#31796=CARTESIAN_POINT('Ctrl Pts',(6.51909837867677,1.82434682109859,92.3896784755687));
#31797=CARTESIAN_POINT('Ctrl Pts',(6.46646995271877,2.00291071820587,92.3984276456795));
#31798=CARTESIAN_POINT('Ctrl Pts',(6.40657713281501,2.17900400212845,92.4071768157903));
#31799=CARTESIAN_POINT('Ctrl Pts',(6.34668509279007,2.355094993098,92.4159258719761));
#31800=CARTESIAN_POINT('Ctrl Pts',(6.27952894037469,2.52871516398265,92.4246749281619));
#31801=CARTESIAN_POINT('Ctrl Pts',(6.20533675061385,2.69927486771562,92.4334239843476));
#31802=CARTESIAN_POINT('Ctrl Pts',(6.12832117907854,2.87632521636056,92.4425059856299));
#31803=CARTESIAN_POINT('Ctrl Pts',(6.04372366626017,3.05007728920121,92.4515879869122));
#31804=CARTESIAN_POINT('Ctrl Pts',(5.95185378007806,3.2198952747831,92.4606699881945));
#31805=CARTESIAN_POINT('Ctrl Pts',(5.86334450817307,3.38350129286863,92.4694197685016));
#31806=CARTESIAN_POINT('Ctrl Pts',(5.76808562057189,3.5434556712507,92.4781695488087));
#31807=CARTESIAN_POINT('Ctrl Pts',(5.66640068804416,3.69921508465414,92.4869193291158));
#31808=CARTESIAN_POINT('Ctrl Pts',(5.56471941107854,3.85496889852383,92.4956687948693));
#31809=CARTESIAN_POINT('Ctrl Pts',(5.45661270815044,4.00652780919732,92.5044182606228));
#31810=CARTESIAN_POINT('Ctrl Pts',(5.34244776449044,4.15337704569319,92.5131677263763));
#31811=CARTESIAN_POINT('Ctrl Pts',(5.22828631819522,4.30022178356339,92.5219169240959));
#31812=CARTESIAN_POINT('Ctrl Pts',(5.10806717843992,4.44235690972767,92.5306661218154));
#31813=CARTESIAN_POINT('Ctrl Pts',(4.98219864544639,4.57929969070732,92.539415319535));
#31814=CARTESIAN_POINT('Ctrl Pts',(4.85633329943941,4.71623900430087,92.5481642957253));
#31815=CARTESIAN_POINT('Ctrl Pts',(4.72481904033562,4.84798602483701,92.5569132719155));
#31816=CARTESIAN_POINT('Ctrl Pts',(4.58810250737109,4.97409332259208,92.5656622481058));
#31817=CARTESIAN_POINT('Ctrl Pts',(4.45137708685552,5.10020881822214,92.574411793042));
#31818=CARTESIAN_POINT('Ctrl Pts',(4.30944892635961,5.22068366308007,92.5831613379781));
#31819=CARTESIAN_POINT('Ctrl Pts',(4.16280009466571,5.33510865604921,92.5919108829143));
#31820=CARTESIAN_POINT('Ctrl Pts',(4.01615988348681,5.44952692272972,92.6006599135226));
#31821=CARTESIAN_POINT('Ctrl Pts',(3.86479978232104,5.55789587288715,92.6094089441309));
#31822=CARTESIAN_POINT('Ctrl Pts',(3.70923383580922,5.65984746713973,92.6181579747392));
#31823=CARTESIAN_POINT('Ctrl Pts',(3.55366577799393,5.76180044505474,92.6269071240872));
#31824=CARTESIAN_POINT('Ctrl Pts',(3.3938920002669,5.85733573571146,92.6356562734352));
#31825=CARTESIAN_POINT('Ctrl Pts',(3.23045513625889,5.9461288762201,92.6444054227832));
#31826=CARTESIAN_POINT('Ctrl Pts',(3.18695122151482,5.96976399206739,92.6467342868961));
#31827=CARTESIAN_POINT('Ctrl Pts',(3.14318791262623,5.99292165435354,92.6490631510091));
#31828=CARTESIAN_POINT('Ctrl Pts',(3.09917575053273,6.01559628526632,92.651392015122));
#31829=CARTESIAN_POINT('Origin',(0.,0.,-3.69717978381041));
#31830=CARTESIAN_POINT('',(3.09917575053266,6.01559628526635,95.0455637664379));
#31831=CARTESIAN_POINT('',(3.09917575053252,6.01559628526643,94.6512396476018));
#31832=CARTESIAN_POINT('',(3.09917575053259,6.01559628526639,-3.69717978381041));
#31833=CARTESIAN_POINT('',(-6.76699989852763,0.00117189038962358,93.6971797872887));
#31834=CARTESIAN_POINT('Ctrl Pts',(-6.7669998985405,0.00117181604119456,
93.6971797907676));
#31835=CARTESIAN_POINT('Ctrl Pts',(-6.76703136317471,-0.180530062912324,
93.7056818217919));
#31836=CARTESIAN_POINT('Ctrl Pts',(-6.75974012411332,-0.362125139993033,
93.7141838528163));
#31837=CARTESIAN_POINT('Ctrl Pts',(-6.74517804147444,-0.543012144257411,
93.7226858838406));
#31838=CARTESIAN_POINT('Ctrl Pts',(-6.73060282379904,-0.724062309071471,
93.7311955837191));
#31839=CARTESIAN_POINT('Ctrl Pts',(-6.70874370102569,-0.90440281033541,
93.7397052835976));
#31840=CARTESIAN_POINT('Ctrl Pts',(-6.67970414778261,-1.08343966056991,
93.7482149834761));
#31841=CARTESIAN_POINT('Ctrl Pts',(-6.64954898098444,-1.26935457588032,
93.7570516007991));
#31842=CARTESIAN_POINT('Ctrl Pts',(-6.611650843814,-1.45386331083921,93.765888218122));
#31843=CARTESIAN_POINT('Ctrl Pts',(-6.56618291935681,-1.63631624985726,
93.774724835445));
#31844=CARTESIAN_POINT('Ctrl Pts',(-6.52227459259335,-1.81251086091544,
93.7832583474874));
#31845=CARTESIAN_POINT('Ctrl Pts',(-6.47130730698831,-1.98678808993954,
93.7917918595299));
#31846=CARTESIAN_POINT('Ctrl Pts',(-6.41348694788727,-2.15858151786763,
93.8003253715723));
#31847=CARTESIAN_POINT('Ctrl Pts',(-6.35258597155414,-2.33952794661864,
93.8093135415355));
#31848=CARTESIAN_POINT('Ctrl Pts',(-6.28408193108863,-2.51771829154907,
93.8183017114988));
#31849=CARTESIAN_POINT('Ctrl Pts',(-6.20827160375272,-2.69251790969674,
93.827289881462));
#31850=CARTESIAN_POINT('Ctrl Pts',(-6.1324612764168,-2.86731752784441,93.8362780514252));
#31851=CARTESIAN_POINT('Ctrl Pts',(-6.04934489877415,-3.03872608388942,
93.8452662213884));
#31852=CARTESIAN_POINT('Ctrl Pts',(-5.95927365459807,-3.20614199773082,
93.8542543913516));
#31853=CARTESIAN_POINT('Ctrl Pts',(-5.87263415123288,-3.36717931617058,
93.8629001094041));
#31854=CARTESIAN_POINT('Ctrl Pts',(-5.77938579804812,-3.52484672363379,
93.8715458274565));
#31855=CARTESIAN_POINT('Ctrl Pts',(-5.67980653833225,-3.67859846777522,
93.8801915455089));
#31856=CARTESIAN_POINT('Ctrl Pts',(-5.58035511809212,-3.83215282601099,
93.8888261642213));
#31857=CARTESIAN_POINT('Ctrl Pts',(-5.47458916316032,-3.98180129009379,
93.8974607829336));
#31858=CARTESIAN_POINT('Ctrl Pts',(-5.36283216365784,-4.12702316257577,
93.906095401646));
#31859=CARTESIAN_POINT('Ctrl Pts',(-5.24712834107501,-4.27737370745086,
93.9150349615484));
#31860=CARTESIAN_POINT('Ctrl Pts',(-5.12500271662077,-4.42297899790175,
93.9239745214508));
#31861=CARTESIAN_POINT('Ctrl Pts',(-4.99686465761375,-4.56329185933692,
93.9329140813532));
#31862=CARTESIAN_POINT('Ctrl Pts',(-4.87344108767164,-4.69844229318401,
93.9415247346238));
#31863=CARTESIAN_POINT('Ctrl Pts',(-4.74443981405401,-4.8286825042295,93.9501353878943));
#31864=CARTESIAN_POINT('Ctrl Pts',(-4.61026922422516,-4.95355495378444,
93.9587460411649));
#31865=CARTESIAN_POINT('Ctrl Pts',(-4.47622563583541,-5.07830920321209,
93.967348543876));
#31866=CARTESIAN_POINT('Ctrl Pts',(-4.33702270929072,-5.19770561408688,
93.9759510465872));
#31867=CARTESIAN_POINT('Ctrl Pts',(-4.19310659484056,-5.3113224421329,93.9845535492984));
#31868=CARTESIAN_POINT('Ctrl Pts',(-4.04935245508128,-5.4248113967252,93.9931463700658));
#31869=CARTESIAN_POINT('Ctrl Pts',(-3.9008959488065,-5.53253355679588,94.0017391908333));
#31870=CARTESIAN_POINT('Ctrl Pts',(-3.7482174644504,-5.63410639224971,94.0103320116008));
#31871=CARTESIAN_POINT('Ctrl Pts',(-3.73022361156676,-5.64607721227611,
94.0113447145589));
#31872=CARTESIAN_POINT('Ctrl Pts',(-3.71217115528374,-5.65796266538561,
94.012357417517));
#31873=CARTESIAN_POINT('Ctrl Pts',(-3.69406091246685,-5.66976216211797,
94.0133701204751));
#31874=CARTESIAN_POINT('Ctrl Pts',(-3.54035127444973,-5.76990970789374,
94.0219653782351));
#31875=CARTESIAN_POINT('Ctrl Pts',(-3.382657288299,-5.86374391978502,94.0305606359951));
#31876=CARTESIAN_POINT('Ctrl Pts',(-3.2215207646025,-5.95097411885104,94.0391558937552));
#31877=CARTESIAN_POINT('Ctrl Pts',(-3.06023334338487,-6.03828600529932,
94.0477592006096));
#31878=CARTESIAN_POINT('Ctrl Pts',(-2.89549721833821,-6.11898138930087,
94.0563625074641));
#31879=CARTESIAN_POINT('Ctrl Pts',(-2.72787643941772,-6.19281673645117,
94.0649658143185));
#31880=CARTESIAN_POINT('Ctrl Pts',(-2.55330604487707,-6.26971332269832,
94.0739258172585));
#31881=CARTESIAN_POINT('Ctrl Pts',(-2.37560705618886,-6.33916877055169,
94.0828858201985));
#31882=CARTESIAN_POINT('Ctrl Pts',(-2.19543541894558,-6.40096495235205,
94.0918458231385));
#31883=CARTESIAN_POINT('Ctrl Pts',(-2.02196310260359,-6.46046336709713,
94.1004726663433));
#31884=CARTESIAN_POINT('Ctrl Pts',(-1.84619899975639,-6.5128617937432,94.109099509548));
#31885=CARTESIAN_POINT('Ctrl Pts',(-1.66874068540826,-6.55801749958501,
94.1177263527527));
#31886=CARTESIAN_POINT('Ctrl Pts',(-1.4911127657688,-6.60321636286733,94.1263614410388));
#31887=CARTESIAN_POINT('Ctrl Pts',(-1.31178770006376,-6.64115862191189,
94.134996529325));
#31888=CARTESIAN_POINT('Ctrl Pts',(-1.13137205816807,-6.67175286307853,
94.1436316176112));
#31889=CARTESIAN_POINT('Ctrl Pts',(-0.950688462838568,-6.70239254283292,
94.1522795307363));
#31890=CARTESIAN_POINT('Ctrl Pts',(-0.768911356462438,-6.72566235315488,
94.1609274438615));
#31891=CARTESIAN_POINT('Ctrl Pts',(-0.586652711046564,-6.74152264674841,
94.1695753569866));
#31892=CARTESIAN_POINT('Ctrl Pts',(-0.566206065584869,-6.7433019302457,
94.1705455211906));
#31893=CARTESIAN_POINT('Ctrl Pts',(-0.54575335970442,-6.74498801580856,
94.1715156853946));
#31894=CARTESIAN_POINT('Ctrl Pts',(-0.525295456907292,-6.74658088834282,
94.1724858495986));
#31895=CARTESIAN_POINT('Ctrl Pts',(-0.351861214087626,-6.76008464992711,
94.1807105291174));
#31896=CARTESIAN_POINT('Ctrl Pts',(-0.17767736880436,-6.76691420521858,
94.1889352086362));
#31897=CARTESIAN_POINT('Ctrl Pts',(-0.00329818154050613,-6.76699919624633,
94.197159888155));
#31898=CARTESIAN_POINT('Ctrl Pts',(0.170897713470069,-6.7670840979389,94.2053759226051));
#31899=CARTESIAN_POINT('Ctrl Pts',(0.34528818611701,-6.76043855250093,94.2135919570553));
#31900=CARTESIAN_POINT('Ctrl Pts',(0.519313869050381,-6.74704395312584,
94.2218079915054));
#31901=CARTESIAN_POINT('Ctrl Pts',(0.693191488953623,-6.73366075002822,
94.23001703566));
#31902=CARTESIAN_POINT('Ctrl Pts',(0.866704581925109,-6.71353995655838,
94.2382260798146));
#31903=CARTESIAN_POINT('Ctrl Pts',(1.03929369751265,-6.68671500890463,94.2464351239692));
#31904=CARTESIAN_POINT('Ctrl Pts',(1.21177053245603,-6.659907512655,94.2546388275972));
#31905=CARTESIAN_POINT('Ctrl Pts',(1.38332423446943,-6.62640460478376,94.2628425312252));
#31906=CARTESIAN_POINT('Ctrl Pts',(1.55340029863261,-6.58629155991504,94.2710462348532));
#31907=CARTESIAN_POINT('Ctrl Pts',(1.72339976704798,-6.54619658042597,94.2792462438471));
#31908=CARTESIAN_POINT('Ctrl Pts',(1.89192257529227,-6.49949747695438,94.2874462528411));
#31909=CARTESIAN_POINT('Ctrl Pts',(2.05842414827465,-6.44633066370317,94.295646261835));
#31910=CARTESIAN_POINT('Ctrl Pts',(2.22491240744009,-6.39316810178249,94.303845615139));
#31911=CARTESIAN_POINT('Ctrl Pts',(2.38937940944284,-6.33353896082529,94.3120449684429));
#31912=CARTESIAN_POINT('Ctrl Pts',(2.55129513111715,-6.2676297077873,94.3202443217468));
#31913=CARTESIAN_POINT('Ctrl Pts',(2.7132097971487,-6.2017208844582,94.3284436215934));
#31914=CARTESIAN_POINT('Ctrl Pts',(2.87257288351492,-6.12953216476514,94.33664292144));
#31915=CARTESIAN_POINT('Ctrl Pts',(3.02887388659421,-6.05129837135038,94.3448422212866));
#31916=CARTESIAN_POINT('Ctrl Pts',(3.18520222517252,-5.97305089561918,94.3530429551096));
#31917=CARTESIAN_POINT('Ctrl Pts',(3.33846709290998,-5.88875640029779,94.3612436889325));
#31918=CARTESIAN_POINT('Ctrl Pts',(3.48818210770356,-5.79869593818272,94.3694444227555));
#31919=CARTESIAN_POINT('Ctrl Pts',(3.63795046623988,-5.70860338735478,94.3776480785155));
#31920=CARTESIAN_POINT('Ctrl Pts',(3.78416614522528,-5.61274096190219,94.3858517342754));
#31921=CARTESIAN_POINT('Ctrl Pts',(3.92637125084586,-5.51143337077853,94.3940553900354));
#31922=CARTESIAN_POINT('Ctrl Pts',(4.0687392615568,-5.41000972529652,94.4022684436104));
#31923=CARTESIAN_POINT('Ctrl Pts',(4.2070872277713,-5.30312866025565,94.4104814971854));
#31924=CARTESIAN_POINT('Ctrl Pts',(4.34098906656382,-5.19115622226623,94.4186945507604));
#31925=CARTESIAN_POINT('Ctrl Pts',(4.47497013807854,-5.07911752767306,94.4269124641835));
#31926=CARTESIAN_POINT('Ctrl Pts',(4.60449957238568,-4.9619816948056,94.4351303776066));
#31927=CARTESIAN_POINT('Ctrl Pts',(4.72918786633991,-4.84015197332309,94.4433482910297));
#31928=CARTESIAN_POINT('Ctrl Pts',(4.85407063197312,-4.7181322385704,94.4515790216256));
#31929=CARTESIAN_POINT('Ctrl Pts',(4.9740969216564,-4.59140424509049,94.4598097522216));
#31930=CARTESIAN_POINT('Ctrl Pts',(5.08891638578258,-4.46040570111213,94.4680404828176));
#31931=CARTESIAN_POINT('Ctrl Pts',(5.19436433143749,-4.34009920559389,94.4755994244935));
#31932=CARTESIAN_POINT('Ctrl Pts',(5.29542107279306,-4.21619137373607,94.4831583661693));
#31933=CARTESIAN_POINT('Ctrl Pts',(5.39184783388915,-4.08904217833283,94.4907173078452));
#31934=CARTESIAN_POINT('Ctrl Pts',(5.49586416920154,-3.95188530203182,94.4988712000119));
#31935=CARTESIAN_POINT('Ctrl Pts',(5.5948140149615,-3.81053223763217,94.5070250921787));
#31936=CARTESIAN_POINT('Ctrl Pts',(5.68833552564354,-3.66539601512602,94.5151789843454));
#31937=CARTESIAN_POINT('Ctrl Pts',(5.78174291395415,-3.52043689936003,94.5233229264856));
#31938=CARTESIAN_POINT('Ctrl Pts',(5.86973495673427,-3.37170411874182,94.5314668686258));
#31939=CARTESIAN_POINT('Ctrl Pts',(5.95198971378876,-3.21964399382181,94.539610810766));
#31940=CARTESIAN_POINT('Ctrl Pts',(6.03416141004451,-3.06773741911438,94.5477465291589));
#31941=CARTESIAN_POINT('Ctrl Pts',(6.11060718164476,-2.912510508299,94.5558822475518));
#31942=CARTESIAN_POINT('Ctrl Pts',(6.18104812068848,-2.7544388048627,94.5640179659447));
#31943=CARTESIAN_POINT('Ctrl Pts',(6.2514327457875,-2.59649347170604,94.5721471802449));
#31944=CARTESIAN_POINT('Ctrl Pts',(6.31582194860431,-2.43570820665953,94.5802763945451));
#31945=CARTESIAN_POINT('Ctrl Pts',(6.37398255637531,-2.27258341343576,94.5884056088453));
#31946=CARTESIAN_POINT('Ctrl Pts',(6.43210889669107,-2.10955473116684,94.5965300335208));
#31947=CARTESIAN_POINT('Ctrl Pts',(6.48401382774071,-1.94418960933513,94.6046544581963));
#31948=CARTESIAN_POINT('Ctrl Pts',(6.52951216284625,-1.77700869869648,94.6127788828717));
#31949=CARTESIAN_POINT('Ctrl Pts',(6.57528670197219,-1.60881289290735,94.6209526280059));
#31950=CARTESIAN_POINT('Ctrl Pts',(6.61457645356851,-1.4387795230129,94.6291263731401));
#31951=CARTESIAN_POINT('Ctrl Pts',(6.64724352095938,-1.26745515623374,94.6373001182743));
#31952=CARTESIAN_POINT('Ctrl Pts',(6.67970139800974,-1.09722790056639,94.6454215211364));
#31953=CARTESIAN_POINT('Ctrl Pts',(6.70562111567153,-0.925726502013933,
94.6535429239986));
#31954=CARTESIAN_POINT('Ctrl Pts',(6.72491858694054,-0.753497842745212,
94.6616643268607));
#31955=CARTESIAN_POINT('Ctrl Pts',(6.74421755018839,-0.581255867663614,
94.669786357627));
#31956=CARTESIAN_POINT('Ctrl Pts',(6.75689320639271,-0.40828688357517,94.6779083883932));
#31957=CARTESIAN_POINT('Ctrl Pts',(6.76291332800492,-0.235143185938755,
94.6860304191595));
#31958=CARTESIAN_POINT('Ctrl Pts',(6.76893506143143,-0.061953131184593,
94.6941546245006));
#31959=CARTESIAN_POINT('Ctrl Pts',(6.76829769939601,0.111411364646957,94.7022788298417));
#31960=CARTESIAN_POINT('Ctrl Pts',(6.76102114450321,0.28439775593438,94.7104030351829));
#31961=CARTESIAN_POINT('Ctrl Pts',(6.75366582593869,0.459256605210039,94.7186151794253));
#31962=CARTESIAN_POINT('Ctrl Pts',(6.7395267607689,0.633728733321958,94.7268273236677));
#31963=CARTESIAN_POINT('Ctrl Pts',(6.71867825379905,0.807249355483022,94.7350394679102));
#31964=CARTESIAN_POINT('Ctrl Pts',(6.69802007071979,0.979185925608369,94.7431766443266));
#31965=CARTESIAN_POINT('Ctrl Pts',(6.67077455549188,1.15018793875211,94.7513138207431));
#31966=CARTESIAN_POINT('Ctrl Pts',(6.63706529048717,1.31971714007605,94.7594509971595));
#31967=CARTESIAN_POINT('Ctrl Pts',(6.60289018017261,1.49158915081183,94.7677006253149));
#31968=CARTESIAN_POINT('Ctrl Pts',(6.56207145162975,1.66194696293157,94.7759502534704));
#31969=CARTESIAN_POINT('Ctrl Pts',(6.51478972345904,1.83024693938072,94.7841998816258));
#31970=CARTESIAN_POINT('Ctrl Pts',(6.46750799528837,1.99854691582974,94.7924495097812));
#31971=CARTESIAN_POINT('Ctrl Pts',(6.41376344604637,2.16478870994882,94.8006991379366));
#31972=CARTESIAN_POINT('Ctrl Pts',(6.35378652268395,2.32845137895552,94.808948766092));
#31973=CARTESIAN_POINT('Ctrl Pts',(6.29397854994596,2.49165302214472,94.8171751556458));
#31974=CARTESIAN_POINT('Ctrl Pts',(6.22779462444683,2.65277802842965,94.8254015451996));
#31975=CARTESIAN_POINT('Ctrl Pts',(6.1553978770005,2.81129258097013,94.8336279347534));
#31976=CARTESIAN_POINT('Ctrl Pts',(6.08308532859357,2.96962277753435,94.8418447568319));
#31977=CARTESIAN_POINT('Ctrl Pts',(6.00457449590004,3.12534824290175,94.8500615789103));
#31978=CARTESIAN_POINT('Ctrl Pts',(5.92007781878808,3.2779517414833,94.8582784009887));
#31979=CARTESIAN_POINT('Ctrl Pts',(5.83567988021109,3.43037691534964,94.8664856213052));
#31980=CARTESIAN_POINT('Ctrl Pts',(5.74531021133635,3.57968708163405,94.8746928416218));
#31981=CARTESIAN_POINT('Ctrl Pts',(5.64922859225456,3.72538659905969,94.8829000619383));
#31982=CARTESIAN_POINT('Ctrl Pts',(5.553211520259,3.87098823637669,94.8911017686909));
#31983=CARTESIAN_POINT('Ctrl Pts',(5.45149033534239,4.01298375647365,94.8993034754434));
#31984=CARTESIAN_POINT('Ctrl Pts',(5.34437011223514,4.1509031671972,94.9075051821959));
#31985=CARTESIAN_POINT('Ctrl Pts',(5.23730236092207,4.28875501944559,94.9157028714225));
#31986=CARTESIAN_POINT('Ctrl Pts',(5.12484105804399,4.42253445618407,94.9239005606492));
#31987=CARTESIAN_POINT('Ctrl Pts',(5.007333890578,4.5518014355054,94.9320982498758));
#31988=CARTESIAN_POINT('Ctrl Pts',(4.88986290332839,4.68102861378834,94.9402934150508));
#31989=CARTESIAN_POINT('Ctrl Pts',(4.76734938775491,4.80574583753666,94.9484885802256));
#31990=CARTESIAN_POINT('Ctrl Pts',(4.64018054396985,4.92554702742382,94.9566837454005));
#31991=CARTESIAN_POINT('Ctrl Pts',(4.51300243034254,5.04535695009568,94.9648795079536));
#31992=CARTESIAN_POINT('Ctrl Pts',(4.38116856654943,5.16024987153774,94.9730752705067));
#31993=CARTESIAN_POINT('Ctrl Pts',(4.24510243737961,5.26985714191131,94.9812710330598));
#31994=CARTESIAN_POINT('Ctrl Pts',(4.10903283705908,5.37946720844994,94.989467004693));
#31995=CARTESIAN_POINT('Ctrl Pts',(3.96873103887808,5.48379113414139,94.9976629763261));
#31996=CARTESIAN_POINT('Ctrl Pts',(3.82465270478567,5.58250129312799,95.0058589479594));
#31997=CARTESIAN_POINT('Ctrl Pts',(3.68049870632419,5.68126329087263,95.0140592237999));
#31998=CARTESIAN_POINT('Ctrl Pts',(3.53256450856589,5.77440543321535,95.0222594996404));
#31999=CARTESIAN_POINT('Ctrl Pts',(3.38133426050597,5.86164376422933,95.030459775481));
#32000=CARTESIAN_POINT('Ctrl Pts',(3.28848452619887,5.9152048471473,95.0354944391333));
#32001=CARTESIAN_POINT('Ctrl Pts',(3.19439287092439,5.96654136592671,95.0405291027856));
#32002=CARTESIAN_POINT('Ctrl Pts',(3.09917575053267,6.01559628526635,95.0455637664379));
#32003=CARTESIAN_POINT('Ctrl Pts',(3.09917575053244,6.01559628526647,93.0458095097322));
#32004=CARTESIAN_POINT('Ctrl Pts',(2.94385794011429,6.09561448609764,93.0540050841243));
#32005=CARTESIAN_POINT('Ctrl Pts',(2.78542189912283,6.1696224327375,93.0622006585164));
#32006=CARTESIAN_POINT('Ctrl Pts',(2.62437621248653,6.23738234320575,93.0703962329085));
#32007=CARTESIAN_POINT('Ctrl Pts',(2.46331484877174,6.30514884979872,93.0785926051032));
#32008=CARTESIAN_POINT('Ctrl Pts',(2.29964366408314,6.36666596921278,93.0867889772979));
#32009=CARTESIAN_POINT('Ctrl Pts',(2.13389102361547,6.42174416333548,93.0949853494926));
#32010=CARTESIAN_POINT('Ctrl Pts',(1.96809209102169,6.47683773993837,93.1031840108061));
#32011=CARTESIAN_POINT('Ctrl Pts',(1.80021088518807,6.52548869614646,93.1113826721197));
#32012=CARTESIAN_POINT('Ctrl Pts',(1.63079076518772,6.56755742115579,93.1195813334332));
#32013=CARTESIAN_POINT('Ctrl Pts',(1.46119433501691,6.60966992575917,93.1277885268347));
#32014=CARTESIAN_POINT('Ctrl Pts',(1.29005613971564,6.64518642674827,93.1359957202363));
#32015=CARTESIAN_POINT('Ctrl Pts',(1.1179305662884,6.67401829851838,93.1442029136379));
#32016=CARTESIAN_POINT('Ctrl Pts',(0.945714434956046,6.70286533917859,93.1524144249698));
#32017=CARTESIAN_POINT('Ctrl Pts',(0.772510245545406,6.72502069396306,93.1606259363017));
#32018=CARTESIAN_POINT('Ctrl Pts',(0.598877237411706,6.74044768947213,93.1688374476336));
#32019=CARTESIAN_POINT('Ctrl Pts',(0.424985635592444,6.75589766058744,93.1770611884662));
#32020=CARTESIAN_POINT('Ctrl Pts',(0.250664297164476,6.76459922719533,93.1852849292987));
#32021=CARTESIAN_POINT('Ctrl Pts',(0.0764735428941643,6.76656787427993,
93.1935086701312));
#32022=CARTESIAN_POINT('Ctrl Pts',(-0.094974794195755,6.76850552746012,
93.2016029383735));
#32023=CARTESIAN_POINT('Ctrl Pts',(-0.2662963084587,6.7639207858022,93.2096972066159));
#32024=CARTESIAN_POINT('Ctrl Pts',(-0.436963125906042,6.7528773294499,93.2177914748582));
#32025=CARTESIAN_POINT('Ctrl Pts',(-0.608825750804297,6.74175649515391,
93.2259424570325));
#32026=CARTESIAN_POINT('Ctrl Pts',(-0.780533533911339,6.7240529782543,93.2340934392067));
#32027=CARTESIAN_POINT('Ctrl Pts',(-0.951537045940788,6.69976613399321,
93.242244421381));
#32028=CARTESIAN_POINT('Ctrl Pts',(-1.12234192154217,6.67550750115267,93.2503859354341));
#32029=CARTESIAN_POINT('Ctrl Pts',(-1.29244379615307,6.64468081407114,93.2585274494871));
#32030=CARTESIAN_POINT('Ctrl Pts',(-1.46129448753021,6.60733739268049,93.2666689635402));
#32031=CARTESIAN_POINT('Ctrl Pts',(-1.62998457555874,6.57002949070924,93.2748027337433));
#32032=CARTESIAN_POINT('Ctrl Pts',(-1.79742549499512,6.52621727301864,93.2829365039463));
#32033=CARTESIAN_POINT('Ctrl Pts',(-1.96307543085417,6.47600369462346,93.2910702741494));
#32034=CARTESIAN_POINT('Ctrl Pts',(-2.1286026473735,6.42582731622569,93.2991980185675));
#32035=CARTESIAN_POINT('Ctrl Pts',(-2.29234117372637,6.36925912553189,93.3073257629855));
#32036=CARTESIAN_POINT('Ctrl Pts',(-2.45376062469325,6.30645286961736,93.3154535074035));
#32037=CARTESIAN_POINT('Ctrl Pts',(-2.61509442763574,6.24367993826009,93.3235769392976));
#32038=CARTESIAN_POINT('Ctrl Pts',(-2.7741112656693,6.17467566567759,93.3317003711916));
#32039=CARTESIAN_POINT('Ctrl Pts',(-2.93029713630135,6.09964324309087,93.3398238030857));
#32040=CARTESIAN_POINT('Ctrl Pts',(-3.08747378866408,6.02413484432777,93.3479987668365));
#32041=CARTESIAN_POINT('Ctrl Pts',(-3.24178307511636,5.94252166554713,93.3561737305873));
#32042=CARTESIAN_POINT('Ctrl Pts',(-3.39272232760371,5.85505971000973,93.3643486943381));
#32043=CARTESIAN_POINT('Ctrl Pts',(-3.5426760932907,5.76816879614173,93.3724702835111));
#32044=CARTESIAN_POINT('Ctrl Pts',(-3.68930339320392,5.67550546036032,93.3805918726841));
#32045=CARTESIAN_POINT('Ctrl Pts',(-3.8321370633259,5.57736627162714,93.3887134618572));
#32046=CARTESIAN_POINT('Ctrl Pts',(-3.97498959042175,5.47921412650828,93.3968361232465));
#32047=CARTESIAN_POINT('Ctrl Pts',(-4.11404718847162,5.37558489577674,93.4049587846359));
#32048=CARTESIAN_POINT('Ctrl Pts',(-4.24887279397961,5.26681772805742,93.4130814460253));
#32049=CARTESIAN_POINT('Ctrl Pts',(-4.38374187401632,5.15801548835501,93.4212067265675));
#32050=CARTESIAN_POINT('Ctrl Pts',(-4.5143759594578,5.04407224228703,93.4293320071098));
#32051=CARTESIAN_POINT('Ctrl Pts',(-4.64037214806056,4.925366517073,93.4374572876521));
#32052=CARTESIAN_POINT('Ctrl Pts',(-4.767741038993,4.80536751761509,93.4456710914398));
#32053=CARTESIAN_POINT('Ctrl Pts',(-4.89037010359729,4.68050192199052,93.4538848952275));
#32054=CARTESIAN_POINT('Ctrl Pts',(-5.00788304941987,4.55119724504807,93.4620986990153));
#32055=CARTESIAN_POINT('Ctrl Pts',(-5.12433067169839,4.42306479058494,93.4702380398704));
#32056=CARTESIAN_POINT('Ctrl Pts',(-5.23575436939067,4.29057373024794,93.4783773807256));
#32057=CARTESIAN_POINT('Ctrl Pts',(-5.34183027815121,4.15417119043342,93.4865167215808));
#32058=CARTESIAN_POINT('Ctrl Pts',(-5.44936184346608,4.01589682832268,93.4947677568348));
#32059=CARTESIAN_POINT('Ctrl Pts',(-5.55139755368367,3.87360317450173,93.5030187920888));
#32060=CARTESIAN_POINT('Ctrl Pts',(-5.64764718687912,3.72778355762997,93.5112698273428));
#32061=CARTESIAN_POINT('Ctrl Pts',(-5.7438968200745,3.58196394075833,93.5195208625968));
#32062=CARTESIAN_POINT('Ctrl Pts',(-5.83436023472334,3.43261872392146,93.5277718978508));
#32063=CARTESIAN_POINT('Ctrl Pts',(-5.91879711720737,3.28026366094826,93.5360229331049));
#32064=CARTESIAN_POINT('Ctrl Pts',(-6.00834497308961,3.11868652995183,93.5447734043927));
#32065=CARTESIAN_POINT('Ctrl Pts',(-6.09136577186997,2.95327257986616,93.5535238756804));
#32066=CARTESIAN_POINT('Ctrl Pts',(-6.16753814020142,2.78455782650691,93.5622743469682));
#32067=CARTESIAN_POINT('Ctrl Pts',(-6.24357747062115,2.61613773982212,93.5710095352282));
#32068=CARTESIAN_POINT('Ctrl Pts',(-6.31279210425957,2.44442860806013,93.5797447234881));
#32069=CARTESIAN_POINT('Ctrl Pts',(-6.37490601256228,2.26999170284767,93.588479911748));
#32070=CARTESIAN_POINT('Ctrl Pts',(-6.43931765511321,2.08910198115318,93.5975382344198));
#32071=CARTESIAN_POINT('Ctrl Pts',(-6.49609301686329,1.90527905537716,93.6065965570917));
#32072=CARTESIAN_POINT('Ctrl Pts',(-6.54497677419722,1.71917655440589,93.6156548797635));
#32073=CARTESIAN_POINT('Ctrl Pts',(-6.59192178979746,1.54045492399483,93.6243539471497));
#32074=CARTESIAN_POINT('Ctrl Pts',(-6.63158894292493,1.35963136459074,93.633053014536));
#32075=CARTESIAN_POINT('Ctrl Pts',(-6.66380078958852,1.1773054135098,93.6417520819222));
#32076=CARTESIAN_POINT('Ctrl Pts',(-6.695965293044,0.995247435126455,93.6504383638956));
#32077=CARTESIAN_POINT('Ctrl Pts',(-6.72069628556325,0.811691750617424,
93.6591246458691));
#32078=CARTESIAN_POINT('Ctrl Pts',(-6.73786647902023,0.627251393697585,
93.6678109278425));
#32079=CARTESIAN_POINT('Ctrl Pts',(-6.75500384035646,0.443163715859861,
93.6764806002734));
#32080=CARTESIAN_POINT('Ctrl Pts',(-6.76460921398091,0.258195026906238,
93.6851502727042));
#32081=CARTESIAN_POINT('Ctrl Pts',(-6.76660659767924,0.0729667886354999,
93.6938199451351));
#32082=CARTESIAN_POINT('Ctrl Pts',(-6.76686461923086,0.0490390488214526,
93.6949398913601));
#32083=CARTESIAN_POINT('Ctrl Pts',(-6.76699575324996,0.0251069907190605,
93.696059837585));
#32084=CARTESIAN_POINT('Ctrl Pts',(-6.76699989851475,0.00117196473805261,
93.6971797838099));
#32085=CARTESIAN_POINT('',(-6.76718481463439,-0.000576657417987951,93.3031400867603));
#32086=CARTESIAN_POINT('Ctrl Pts',(3.09917575053273,6.01559628526632,92.651392015122));
#32087=CARTESIAN_POINT('Ctrl Pts',(2.93382384459271,6.10078395293757,92.6601414630344));
#32088=CARTESIAN_POINT('Ctrl Pts',(2.76495772122981,6.17915010267051,92.6688909109469));
#32089=CARTESIAN_POINT('Ctrl Pts',(2.59315093316699,6.25042856433183,92.6776403588593));
#32090=CARTESIAN_POINT('Ctrl Pts',(2.42134553245594,6.3217064504146,92.6863897361193));
#32091=CARTESIAN_POINT('Ctrl Pts',(2.24659977927557,6.38589665313469,92.6951391133793));
#32092=CARTESIAN_POINT('Ctrl Pts',(2.06950718689874,6.44278115439089,92.7038884906393));
#32093=CARTESIAN_POINT('Ctrl Pts',(1.89241596572818,6.49966521519737,92.712637800154));
#32094=CARTESIAN_POINT('Ctrl Pts',(1.71297821457155,6.54924360009557,92.7213871096686));
#32095=CARTESIAN_POINT('Ctrl Pts',(1.53180337335803,6.59134792173566,92.7301364191833));
#32096=CARTESIAN_POINT('Ctrl Pts',(1.35062987477737,6.63345193135314,92.7388856638594));
#32097=CARTESIAN_POINT('Ctrl Pts',(1.16771959102902,6.66808192368247,92.7476349085355));
#32098=CARTESIAN_POINT('Ctrl Pts',(0.9836937469063,6.69512028363176,92.7563841532116));
#32099=CARTESIAN_POINT('Ctrl Pts',(0.799669205419276,6.72215845218874,92.7651333359558));
#32100=CARTESIAN_POINT('Ctrl Pts',(0.614529402872833,6.74160505424585,92.7738825187));
#32101=CARTESIAN_POINT('Ctrl Pts',(0.428903127362555,6.75339404354126,92.7826317014442));
#32102=CARTESIAN_POINT('Ctrl Pts',(0.243278104163159,6.76518295330333,92.7913808251628));
#32103=CARTESIAN_POINT('Ctrl Pts',(0.0571669005383708,6.76931433552276,
92.8001299488814));
#32104=CARTESIAN_POINT('Ctrl Pts',(-0.128798404778285,6.76577415902471,
92.8088790726));
#32105=CARTESIAN_POINT('Ctrl Pts',(-0.314762517259753,6.76223400523438,
92.8176281401992));
#32106=CARTESIAN_POINT('Ctrl Pts',(-0.500580446820047,6.75102239665085,
92.8263772077984));
#32107=CARTESIAN_POINT('Ctrl Pts',(-0.685621118843031,6.73217741012493,
92.8351262753976));
#32108=CARTESIAN_POINT('Ctrl Pts',(-0.870660665414907,6.71333253821766,
92.8438752897834));
#32109=CARTESIAN_POINT('Ctrl Pts',(-1.05492267885528,6.68685441030605,92.8526243041692));
#32110=CARTESIAN_POINT('Ctrl Pts',(-1.23778137635294,6.6528329502817,92.861373318555));
#32111=CARTESIAN_POINT('Ctrl Pts',(-1.42999922978878,6.61707018861858,92.8705701289223));
#32112=CARTESIAN_POINT('Ctrl Pts',(-1.62066601233716,6.57297172934408,92.8797669392897));
#32113=CARTESIAN_POINT('Ctrl Pts',(-1.80906628500395,6.52070304311291,92.8889637496571));
#32114=CARTESIAN_POINT('Ctrl Pts',(-1.98831342545542,6.47097374915026,92.8977137473949));
#32115=CARTESIAN_POINT('Ctrl Pts',(-2.16550875896721,6.41384933989522,92.9064637451326));
#32116=CARTESIAN_POINT('Ctrl Pts',(-2.34005036714034,6.34952386240467,92.9152137428704));
#32117=CARTESIAN_POINT('Ctrl Pts',(-2.51458843547103,6.2851996894859,92.9239635631513));
#32118=CARTESIAN_POINT('Ctrl Pts',(-2.68647261718061,6.21367483971097,92.9327133834321));
#32119=CARTESIAN_POINT('Ctrl Pts',(-2.85511905908728,6.13519226743845,92.941463203713));
#32120=CARTESIAN_POINT('Ctrl Pts',(-3.02376230488879,6.0567111825294,92.9502128581715));
#32121=CARTESIAN_POINT('Ctrl Pts',(-3.18916767379896,5.97127275992637,92.9589625126301));
#32122=CARTESIAN_POINT('Ctrl Pts',(-3.35077334102777,5.87916720438002,92.9677121670886));
#32123=CARTESIAN_POINT('Ctrl Pts',(-3.51237616037348,5.78706327195655,92.976461667357));
#32124=CARTESIAN_POINT('Ctrl Pts',(-3.6701791630227,5.68829258362317,92.9852111676255));
#32125=CARTESIAN_POINT('Ctrl Pts',(-3.82364636566424,5.58319061741068,92.9939606678939));
#32126=CARTESIAN_POINT('Ctrl Pts',(-3.97711106778759,5.4780903636773,93.0027100256023));
#32127=CARTESIAN_POINT('Ctrl Pts',(-4.12623987481888,5.36665920043255,93.0114593833108));
#32128=CARTESIAN_POINT('Ctrl Pts',(-4.2705262821389,5.24927559512367,93.0202087410192));
#32129=CARTESIAN_POINT('Ctrl Pts',(-4.41481053024929,5.13189374643078,93.0289579677957));
#32130=CARTESIAN_POINT('Ctrl Pts',(-4.55425230136472,5.00855981477405,93.0377071945722));
#32131=CARTESIAN_POINT('Ctrl Pts',(-4.68837800630482,4.8796926819214,93.0464564213488));
#32132=CARTESIAN_POINT('Ctrl Pts',(-4.82250188228811,4.75082730631893,93.0552055288196));
#32133=CARTESIAN_POINT('Ctrl Pts',(-4.95130963052868,4.6164290790363,93.0639546362904));
#32134=CARTESIAN_POINT('Ctrl Pts',(-5.07436379033255,4.47695444731816,93.0727037437613));
#32135=CARTESIAN_POINT('Ctrl Pts',(-5.19741643562673,4.33748153220743,93.081452743551));
#32136=CARTESIAN_POINT('Ctrl Pts',(-5.31471544462622,4.19293255254778,93.0902017433407));
#32137=CARTESIAN_POINT('Ctrl Pts',(-5.42586245275461,4.04379841779826,93.0989507431304));
#32138=CARTESIAN_POINT('Ctrl Pts',(-5.53702160018989,3.89464799484576,93.1077006984726));
#32139=CARTESIAN_POINT('Ctrl Pts',(-5.6420272308109,3.74091164444093,93.1164506538148));
#32140=CARTESIAN_POINT('Ctrl Pts',(-5.74052265232809,3.58311159163486,93.1252006091569));
#32141=CARTESIAN_POINT('Ctrl Pts',(-5.83901427066769,3.42531763192038,93.1339502266394));
#32142=CARTESIAN_POINT('Ctrl Pts',(-5.93099603115599,3.26346052695869,93.1426998441218));
#32143=CARTESIAN_POINT('Ctrl Pts',(-6.01615550622621,3.09809004467333,93.1514494616042));
#32144=CARTESIAN_POINT('Ctrl Pts',(-6.10131214578678,2.93272506864081,93.1601987877553));
#32145=CARTESIAN_POINT('Ctrl Pts',(-6.17964682328636,2.76384720417144,93.1689481139064));
#32146=CARTESIAN_POINT('Ctrl Pts',(-6.25089348288462,2.59203002791839,93.1776974400575));
#32147=CARTESIAN_POINT('Ctrl Pts',(-6.32213814889227,2.42021765937297,93.1864465213891));
#32148=CARTESIAN_POINT('Ctrl Pts',(-6.38629508412482,2.24546640832209,93.1951956027207));
#32149=CARTESIAN_POINT('Ctrl Pts',(-6.44314639819711,2.06836976660356,93.2039446840522));
#32150=CARTESIAN_POINT('Ctrl Pts',(-6.50000285283612,1.8912571115858,93.2126945564866));
#32151=CARTESIAN_POINT('Ctrl Pts',(-6.54955227673173,1.71179891440549,93.221444428921));
#32152=CARTESIAN_POINT('Ctrl Pts',(-6.59162635926319,1.53060476278714,93.2301943013554));
#32153=CARTESIAN_POINT('Ctrl Pts',(-6.63369752055137,1.34942319164987,93.2389435662779));
#32154=CARTESIAN_POINT('Ctrl Pts',(-6.66829431424201,1.16650618643004,93.2476928312004));
#32155=CARTESIAN_POINT('Ctrl Pts',(-6.69529923745372,0.98247499762164,93.2564420961229));
#32156=CARTESIAN_POINT('Ctrl Pts',(-6.72230554731407,0.79843435918082,93.2651918103026));
#32157=CARTESIAN_POINT('Ctrl Pts',(-6.74171916496675,0.613279706243404,
93.2739415244823));
#32158=CARTESIAN_POINT('Ctrl Pts',(-6.75347414817256,0.427639953658433,
93.282691238662));
#32159=CARTESIAN_POINT('Ctrl Pts',(-6.76248837758731,0.285283364201734,
93.2894008978379));
#32160=CARTESIAN_POINT('Ctrl Pts',(-6.7669999999999,0.142641701108384,93.2961105570138));
#32161=CARTESIAN_POINT('Ctrl Pts',(-6.767,4.93710580834799E-12,93.3028202161897));
#32162=CARTESIAN_POINT('Ctrl Pts',(-6.76699943564324,-0.00276369392438207,
93.3028202161897));
#32163=CARTESIAN_POINT('Ctrl Pts',(-6.76692073666861,-0.19546083458944,
93.311844006505));
#32164=CARTESIAN_POINT('Ctrl Pts',(-6.75860706019009,-0.387883716665939,
93.3208677968202));
#32165=CARTESIAN_POINT('Ctrl Pts',(-6.74215322839483,-0.579360720833886,
93.3298915871354));
#32166=CARTESIAN_POINT('Ctrl Pts',(-6.72561737121243,-0.771792273194158,
93.3389603627103));
#32167=CARTESIAN_POINT('Ctrl Pts',(-6.70086007133121,-0.963268274798117,
93.348029138285));
#32168=CARTESIAN_POINT('Ctrl Pts',(-6.66802805393154,-1.15312222768533,
93.3570979138599));
#32169=CARTESIAN_POINT('Ctrl Pts',(-6.63511598923357,-1.34343906093151,
93.366188799894));
#32170=CARTESIAN_POINT('Ctrl Pts',(-6.59408989033998,-1.53212572130063,
93.375279685928));
#32171=CARTESIAN_POINT('Ctrl Pts',(-6.54514676617052,-1.71852925761759,
93.3843705719621));
#32172=CARTESIAN_POINT('Ctrl Pts',(-6.49602927726239,-1.90559687503779,
93.3934938451802));
#32173=CARTESIAN_POINT('Ctrl Pts',(-6.43893835629684,-2.09036486917792,
93.4026171183984));
#32174=CARTESIAN_POINT('Ctrl Pts',(-6.37412106298803,-2.27219490237356,
93.4117403916164));
#32175=CARTESIAN_POINT('Ctrl Pts',(-6.32111453265114,-2.42089255200888,
93.4192012563629));
#32176=CARTESIAN_POINT('Ctrl Pts',(-6.26294175426668,-2.56762573814302,
93.4266621211093));
#32177=CARTESIAN_POINT('Ctrl Pts',(-6.19976076501379,-2.71205742133084,
93.4341229858557));
#32178=CARTESIAN_POINT('Ctrl Pts',(-6.13072231116159,-2.86987926319289,
93.442275542069));
#32179=CARTESIAN_POINT('Ctrl Pts',(-6.05554564095145,-3.02531006094246,
93.4504280982822));
#32180=CARTESIAN_POINT('Ctrl Pts',(-5.97441769268714,-3.17783294609816,
93.4585806544955));
#32181=CARTESIAN_POINT('Ctrl Pts',(-5.89338373310665,-3.33017912981451,
93.4667237657758));
#32182=CARTESIAN_POINT('Ctrl Pts',(-5.80641238994543,-3.47962378758133,
93.4748668770562));
#32183=CARTESIAN_POINT('Ctrl Pts',(-5.71373902127651,-3.6256689585154,93.4830099883365));
#32184=CARTESIAN_POINT('Ctrl Pts',(-5.62115353351799,-3.77157563677606,
93.4911453776139));
#32185=CARTESIAN_POINT('Ctrl Pts',(-5.52287697972033,-3.91408893961336,
93.4992807668912));
#32186=CARTESIAN_POINT('Ctrl Pts',(-5.41919108118185,-4.05273451210897,
93.5074161561685));
#32187=CARTESIAN_POINT('Ctrl Pts',(-5.31558171967864,-4.19127774165127,
93.5155455402071));
#32188=CARTESIAN_POINT('Ctrl Pts',(-5.20657118215975,-4.32595863416734,
93.5236749242457));
#32189=CARTESIAN_POINT('Ctrl Pts',(-5.09248503410837,-4.45633090977121,
93.5318043082843));
#32190=CARTESIAN_POINT('Ctrl Pts',(-4.97845913661793,-4.58663433387233,
93.5399293990764));
#32191=CARTESIAN_POINT('Ctrl Pts',(-4.85936320713057,-4.7126333982141,93.5480544898686));
#32192=CARTESIAN_POINT('Ctrl Pts',(-4.7355636994504,-4.83391409195981,93.5561795806607));
#32193=CARTESIAN_POINT('Ctrl Pts',(-4.6112916222113,-4.95565774040562,93.5643356866858));
#32194=CARTESIAN_POINT('Ctrl Pts',(-4.4822802159272,-5.07264663169301,93.572491792711));
#32195=CARTESIAN_POINT('Ctrl Pts',(-4.34893856883504,-5.18449827124082,
93.5806478987361));
#32196=CARTESIAN_POINT('Ctrl Pts',(-4.21613359775723,-5.29589972816813,
93.5887711779095));
#32197=CARTESIAN_POINT('Ctrl Pts',(-4.07903347406898,-5.40220498938928,
93.5968944570829));
#32198=CARTESIAN_POINT('Ctrl Pts',(-3.93807637029669,-5.50307582191185,
93.6050177362563));
#32199=CARTESIAN_POINT('Ctrl Pts',(-3.79710049689509,-5.60396008623804,
93.613142097113));
#32200=CARTESIAN_POINT('Ctrl Pts',(-3.65226691796216,-5.69940826759409,
93.6212664579697));
#32201=CARTESIAN_POINT('Ctrl Pts',(-3.50404357691585,-5.78912494346726,
93.6293908188264));
#32202=CARTESIAN_POINT('Ctrl Pts',(-3.35577229842576,-5.87887063493322,
93.6375178072118));
#32203=CARTESIAN_POINT('Ctrl Pts',(-3.20410938755046,-5.96288094038789,
93.6456447955972));
#32204=CARTESIAN_POINT('Ctrl Pts',(-3.04954816703763,-6.04090597318957,
93.6537717839827));
#32205=CARTESIAN_POINT('Ctrl Pts',(-2.89398772583128,-6.11943542894502,
93.6619513124227));
#32206=CARTESIAN_POINT('Ctrl Pts',(-2.73549170607932,-6.19190178616823,
93.6701308408628));
#32207=CARTESIAN_POINT('Ctrl Pts',(-2.57458344338408,-6.25809947931899,
93.6783103693029));
#32208=CARTESIAN_POINT('Ctrl Pts',(-2.41443294957232,-6.32398542619154,
93.6864513777065));
#32209=CARTESIAN_POINT('Ctrl Pts',(-2.25189324911824,-6.38366155869766,
93.6945923861102));
#32210=CARTESIAN_POINT('Ctrl Pts',(-2.08749516385627,-6.43697544976495,
93.7027333945139));
#32211=CARTESIAN_POINT('Ctrl Pts',(-1.92193027838147,-6.49066773124564,
93.7109321829722));
#32212=CARTESIAN_POINT('Ctrl Pts',(-1.7544808950459,-6.5379070259825,93.7191309714305));
#32213=CARTESIAN_POINT('Ctrl Pts',(-1.58569885720144,-6.57859013271613,
93.7273297598887));
#32214=CARTESIAN_POINT('Ctrl Pts',(-1.41691681935687,-6.61927323944979,
93.735528548347));
#32215=CARTESIAN_POINT('Ctrl Pts',(-1.24680250385791,-6.6534001486529,93.7437273368052));
#32216=CARTESIAN_POINT('Ctrl Pts',(-1.07591179273701,-6.68092080586572,
93.7519261252635));
#32217=CARTESIAN_POINT('Ctrl Pts',(-0.904306951495498,-6.70855646833614,
93.7601591753955));
#32218=CARTESIAN_POINT('Ctrl Pts',(-0.731385791230929,-6.72961657496667,
93.7683922255275));
#32219=CARTESIAN_POINT('Ctrl Pts',(-0.557693213700642,-6.74398007703109,
93.7766252756595));
#32220=CARTESIAN_POINT('Ctrl Pts',(-0.384207477330789,-6.75832647437245,
93.7848485214944));
#32221=CARTESIAN_POINT('Ctrl Pts',(-0.209952506395458,-6.76599211737185,
93.7930717673292));
#32222=CARTESIAN_POINT('Ctrl Pts',(-0.0354831671871846,-6.76690697031121,
93.8012950131641));
#32223=CARTESIAN_POINT('Ctrl Pts',(0.138813326271391,-6.76782091691113,
93.8095101122776));
#32224=CARTESIAN_POINT('Ctrl Pts',(0.313323409343689,-6.76199739075653,
93.8177252113911));
#32225=CARTESIAN_POINT('Ctrl Pts',(0.48748722261307,-6.7494181384612,93.8259403105046));
#32226=CARTESIAN_POINT('Ctrl Pts',(0.661513339485855,-6.73684883150227,
93.8341489146435));
#32227=CARTESIAN_POINT('Ctrl Pts',(0.835193376198719,-6.71753446263811,
93.8423575187824));
#32228=CARTESIAN_POINT('Ctrl Pts',(1.00796750380458,-6.69150883667309,93.8505661229212));
#32229=CARTESIAN_POINT('Ctrl Pts',(1.18063959336153,-6.66549858108864,93.8587698791702));
#32230=CARTESIAN_POINT('Ctrl Pts',(1.35240648640268,-6.63278501759715,93.8669736354192));
#32231=CARTESIAN_POINT('Ctrl Pts',(1.5227134110507,-6.5934537890097,93.8751773916682));
#32232=CARTESIAN_POINT('Ctrl Pts',(1.69296994617221,-6.55413419754146,93.8833787206324));
#32233=CARTESIAN_POINT('Ctrl Pts',(1.86176702394338,-6.50820091797749,93.8915800495967));
#32234=CARTESIAN_POINT('Ctrl Pts',(2.02855975576241,-6.45579075848197,93.899781378561));
#32235=CARTESIAN_POINT('Ctrl Pts',(2.19532948527123,-6.40338782684784,93.9079815764837));
#32236=CARTESIAN_POINT('Ctrl Pts',(2.36009507742931,-6.34450990087382,93.9161817744064));
#32237=CARTESIAN_POINT('Ctrl Pts',(2.52232648966835,-6.27934376185262,93.9243819723291));
#32238=CARTESIAN_POINT('Ctrl Pts',(2.68456492827967,-6.21417480043378,93.9325825254089));
#32239=CARTESIAN_POINT('Ctrl Pts',(2.84426863580239,-6.14271721688352,93.9407830784887));
#32240=CARTESIAN_POINT('Ctrl Pts',(3.00092719746958,-6.06520609340585,93.9489836315686));
#32241=CARTESIAN_POINT('Ctrl Pts',(3.1576209337445,-5.98767756632549,93.9571860259218));
#32242=CARTESIAN_POINT('Ctrl Pts',(3.31126784130981,-5.90409295102151,93.965388420275));
#32243=CARTESIAN_POINT('Ctrl Pts',(3.46138172439311,-5.81473348985467,93.9735908146282));
#32244=CARTESIAN_POINT('Ctrl Pts',(3.61163599034558,-5.72529046188315,93.9818008796621));
#32245=CARTESIAN_POINT('Ctrl Pts',(3.75835032243735,-5.63006198181099,93.9900109446959));
#32246=CARTESIAN_POINT('Ctrl Pts',(3.90106637958895,-5.52937339144688,93.9982210097297));
#32247=CARTESIAN_POINT('Ctrl Pts',(4.0438507381137,-5.42863661330965,94.006435003955));
#32248=CARTESIAN_POINT('Ctrl Pts',(4.18263272211037,-5.32243473237826,94.0146489981803));
#32249=CARTESIAN_POINT('Ctrl Pts',(4.31698684499628,-5.21113361756624,94.0228629924056));
#32250=CARTESIAN_POINT('Ctrl Pts',(4.45152413729963,-5.09968076226482,94.0310881850408));
#32251=CARTESIAN_POINT('Ctrl Pts',(4.58162123725197,-4.9831150186645,94.039313377676));
#32252=CARTESIAN_POINT('Ctrl Pts',(4.7068884383998,-4.86184021009107,94.0475385703112));
#32253=CARTESIAN_POINT('Ctrl Pts',(4.81954096409286,-4.75277803448919,94.0549354684311));
#32254=CARTESIAN_POINT('Ctrl Pts',(4.92828775431794,-4.63990808496353,94.0623323665511));
#32255=CARTESIAN_POINT('Ctrl Pts',(5.03287358499152,-4.52354644913641,94.0697292646711));
#32256=CARTESIAN_POINT('Ctrl Pts',(5.15512017711148,-4.38753554458314,94.078375231162));
#32257=CARTESIAN_POINT('Ctrl Pts',(5.27195899930973,-4.24644513036207,94.0870211976529));
#32258=CARTESIAN_POINT('Ctrl Pts',(5.3829705552559,-4.10072152203098,94.0956671641438));
#32259=CARTESIAN_POINT('Ctrl Pts',(5.49384011233034,-3.9551843140056,94.1043020712681));
#32260=CARTESIAN_POINT('Ctrl Pts',(5.59889708268893,-3.8050259710503,94.1129369783925));
#32261=CARTESIAN_POINT('Ctrl Pts',(5.69776096585244,-3.65072718454943,94.1215718855169));
#32262=CARTESIAN_POINT('Ctrl Pts',(5.79990705014212,-3.49130580287416,94.1304934645884));
#32263=CARTESIAN_POINT('Ctrl Pts',(5.89544153356701,-3.32746455336801,94.1394150436598));
#32264=CARTESIAN_POINT('Ctrl Pts',(5.98399032744266,-3.15977036524377,94.1483366227313));
#32265=CARTESIAN_POINT('Ctrl Pts',(6.06945713552447,-2.99791285860198,94.156947681707));
#32266=CARTESIAN_POINT('Ctrl Pts',(6.14841614237943,-2.83246638633334,94.1655587406827));
#32267=CARTESIAN_POINT('Ctrl Pts',(6.22057492005191,-2.66397009443071,94.1741697996584));
#32268=CARTESIAN_POINT('Ctrl Pts',(6.29266564866576,-2.49563270231018,94.182772738008));
#32269=CARTESIAN_POINT('Ctrl Pts',(6.35796881414188,-2.3242515041962,94.1913756763575));
#32270=CARTESIAN_POINT('Ctrl Pts',(6.41623844991414,-2.15038907034132,94.1999786147071));
#32271=CARTESIAN_POINT('Ctrl Pts',(6.47444283717413,-1.97672132219192,94.2085719197558));
#32272=CARTESIAN_POINT('Ctrl Pts',(6.5256293102815,-1.800578169687,94.2171652248046));
#32273=CARTESIAN_POINT('Ctrl Pts',(6.56960038783988,-1.62254113787422,94.2257585298533));
#32274=CARTESIAN_POINT('Ctrl Pts',(6.57449948561295,-1.60270489836153,94.2267159646938));
#32275=CARTESIAN_POINT('Ctrl Pts',(6.57930906415589,-1.58284516773862,94.2276733995343));
#32276=CARTESIAN_POINT('Ctrl Pts',(6.58402888803372,-1.56296276396384,94.2286308343748));
#32277=CARTESIAN_POINT('Ctrl Pts',(6.6264030110611,-1.38446046272552,94.2372265919223));
#32278=CARTESIAN_POINT('Ctrl Pts',(6.66148888606537,-1.20433869060862,94.2458223494699));
#32279=CARTESIAN_POINT('Ctrl Pts',(6.68919571236195,-1.02320561067585,94.2544181070175));
#32280=CARTESIAN_POINT('Ctrl Pts',(6.71692839006948,-0.841903527421079,
94.2630218846991));
#32281=CARTESIAN_POINT('Ctrl Pts',(6.73726823038795,-0.659588554715393,
94.2716256623807));
#32282=CARTESIAN_POINT('Ctrl Pts',(6.75017631614964,-0.47687388363436,94.2802294400623));
#32283=CARTESIAN_POINT('Ctrl Pts',(6.76359170096919,-0.286978366205748,
94.2891713537304));
#32284=CARTESIAN_POINT('Ctrl Pts',(6.76897935589969,-0.0966514746789712,
94.2981132673984));
#32285=CARTESIAN_POINT('Ctrl Pts',(6.76635512778851,0.0934199371131073,
94.3070551810665));
#32286=CARTESIAN_POINT('Ctrl Pts',(6.76382325958695,0.276801770990058,94.3156823833972));
#32287=CARTESIAN_POINT('Ctrl Pts',(6.75383391928934,0.459945508383227,94.3243095857279));
#32288=CARTESIAN_POINT('Ctrl Pts',(6.73645427998343,0.642240401791198,94.3329367880586));
#32289=CARTESIAN_POINT('Ctrl Pts',(6.71905808923127,0.824708903182535,94.341572206479));
#32290=CARTESIAN_POINT('Ctrl Pts',(6.69425758892832,1.00632664457754,94.3502076248994));
#32291=CARTESIAN_POINT('Ctrl Pts',(6.66217129853548,1.18649171466561,94.3588430433199));
#32292=CARTESIAN_POINT('Ctrl Pts',(6.63003760521888,1.36692295298242,94.367491219341));
#32293=CARTESIAN_POINT('Ctrl Pts',(6.59059667366888,1.54589693265643,94.3761393953621));
#32294=CARTESIAN_POINT('Ctrl Pts',(6.54401757759243,1.72282411875424,94.3847875713833));
#32295=CARTESIAN_POINT('Ctrl Pts',(6.539089685841,1.74154234419046,94.3857025156151));
#32296=CARTESIAN_POINT('Ctrl Pts',(6.53408194301536,1.76023767644184,94.386617459847));
#32297=CARTESIAN_POINT('Ctrl Pts',(6.52899458127401,1.77890942931186,94.3875324040788));
#32298=CARTESIAN_POINT('Ctrl Pts',(6.48325069878245,1.94679968611338,94.3957592814969));
#32299=CARTESIAN_POINT('Ctrl Pts',(6.43096677510618,2.11314476249537,94.4039861589149));
#32300=CARTESIAN_POINT('Ctrl Pts',(6.37226362387557,2.27739880298383,94.412213036333));
#32301=CARTESIAN_POINT('Ctrl Pts',(6.31362342555486,2.44147669841715,94.4204310912968));
#32302=CARTESIAN_POINT('Ctrl Pts',(6.24857782899537,2.6034676890307,94.4286491462605));
#32303=CARTESIAN_POINT('Ctrl Pts',(6.17729809685386,2.76283861682251,94.4368672012242));
#32304=CARTESIAN_POINT('Ctrl Pts',(6.10608054068996,2.92207052833379,94.4450780877323));
#32305=CARTESIAN_POINT('Ctrl Pts',(6.02863982598939,3.07868660391034,94.4532889742403));
#32306=CARTESIAN_POINT('Ctrl Pts',(5.94519623557328,3.23217120841785,94.4614998607483));
#32307=CARTESIAN_POINT('Ctrl Pts',(5.86181360996178,3.38554367538576,94.4697047482924));
#32308=CARTESIAN_POINT('Ctrl Pts',(5.77243701925507,3.53578891695613,94.4779096358365));
#32309=CARTESIAN_POINT('Ctrl Pts',(5.6773338210649,3.68241356778305,94.4861145233806));
#32310=CARTESIAN_POINT('Ctrl Pts',(5.58226883254748,3.82897930913024,94.4943161144417));
#32311=CARTESIAN_POINT('Ctrl Pts',(5.4814820127794,3.97192705648257,94.5025177055029));
#32312=CARTESIAN_POINT('Ctrl Pts',(5.37528555289648,4.11078997576164,94.510719296564));
#32313=CARTESIAN_POINT('Ctrl Pts',(5.26911251457786,4.24962226890877,94.5189190787693));
#32314=CARTESIAN_POINT('Ctrl Pts',(5.15753243013563,4.38437124418564,94.5271188609746));
#32315=CARTESIAN_POINT('Ctrl Pts',(5.04089955210063,4.51460083569209,94.5353186431798));
#32316=CARTESIAN_POINT('Ctrl Pts',(4.92427126168953,4.64482530476311,94.5435181028558));
#32317=CARTESIAN_POINT('Ctrl Pts',(4.80259081330919,4.7705304781173,94.5517175625319));
#32318=CARTESIAN_POINT('Ctrl Pts',(4.67625133983461,4.89131499769694,94.5599170222079));
#32319=CARTESIAN_POINT('Ctrl Pts',(4.54984956301961,5.01215908123418,94.5681205253844));
#32320=CARTESIAN_POINT('Ctrl Pts',(4.41878442857251,5.1280774136718,94.5763240285609));
#32321=CARTESIAN_POINT('Ctrl Pts',(4.28348484926054,5.23870657187014,94.5845275317374));
#32322=CARTESIAN_POINT('Ctrl Pts',(4.14815093231874,5.34936380660134,94.5927331168779));
#32323=CARTESIAN_POINT('Ctrl Pts',(4.00858071140653,5.45472897168289,94.6009387020185));
#32324=CARTESIAN_POINT('Ctrl Pts',(3.86523446916498,5.55448030857784,94.609144287159));
#32325=CARTESIAN_POINT('Ctrl Pts',(3.72175727671629,5.65432277069536,94.6173573682971));
#32326=CARTESIAN_POINT('Ctrl Pts',(3.57449747044358,5.748540961385,94.6255704494351));
#32327=CARTESIAN_POINT('Ctrl Pts',(3.42394318831687,5.83685720599524,94.6337835305731));
#32328=CARTESIAN_POINT('Ctrl Pts',(3.31728028784536,5.89942644464998,94.6396022362494));
#32329=CARTESIAN_POINT('Ctrl Pts',(3.20896436658928,5.95903427537873,94.6454209419256));
#32330=CARTESIAN_POINT('Ctrl Pts',(3.09917575053252,6.01559628526642,94.6512396476019));
#32331=CARTESIAN_POINT('Origin',(0.,0.,-3.69717978381041));
#32332=CARTESIAN_POINT('',(3.09917575053274,6.01559628526631,97.0457515827422));
#32333=CARTESIAN_POINT('',(3.09917575053247,6.01559628526645,96.651556635143));
#32334=CARTESIAN_POINT('',(3.09917575053259,6.01559628526639,-3.69717978381041));
#32335=CARTESIAN_POINT('',(-6.767,5.25699960180013E-12,95.6971797838099));
#32336=CARTESIAN_POINT('Ctrl Pts',(-6.767,5.25699960145695E-12,95.6971797838099));
#32337=CARTESIAN_POINT('Ctrl Pts',(-6.76700000000015,-0.186007249410409,
95.7059292956159));
#32338=CARTESIAN_POINT('Ctrl Pts',(-6.75932637295467,-0.372014355522253,
95.7146788074218));
#32339=CARTESIAN_POINT('Ctrl Pts',(-6.74400518266972,-0.557389537149768,
95.7234283192278));
#32340=CARTESIAN_POINT('Ctrl Pts',(-6.72868405709704,-0.742763935806127,
95.7321777940783));
#32341=CARTESIAN_POINT('Ctrl Pts',(-6.70571545653064,-0.927506129689783,
95.7409272689288));
#32342=CARTESIAN_POINT('Ctrl Pts',(-6.67517739415737,-1.11098863924453,
95.7496767437794));
#32343=CARTESIAN_POINT('Ctrl Pts',(-6.64463945823168,-1.29447038906155,
95.7584261824014));
#32344=CARTESIAN_POINT('Ctrl Pts',(-6.60653217027232,-1.47669218227882,
95.7671756210234));
#32345=CARTESIAN_POINT('Ctrl Pts',(-6.56098496116793,-1.65703510503799,
95.7759250596454));
#32346=CARTESIAN_POINT('Ctrl Pts',(-6.51543793687604,-1.83737729603714,
95.7846744627656));
#32347=CARTESIAN_POINT('Ctrl Pts',(-6.4624511220273,-2.01584035396762,95.7934238658858));
#32348=CARTESIAN_POINT('Ctrl Pts',(-6.40220448416337,-2.19181813637868,
95.8021732690061));
#32349=CARTESIAN_POINT('Ctrl Pts',(-6.34195808575295,-2.36779521935654,
95.8109226373513));
#32350=CARTESIAN_POINT('Ctrl Pts',(-6.27445201489357,-2.54128677544523,
95.8196720056966));
#32351=CARTESIAN_POINT('Ctrl Pts',(-6.19991555136322,-2.71170355237524,
95.8284213740418));
#32352=CARTESIAN_POINT('Ctrl Pts',(-6.12537937789186,-2.88211966612758,
95.8371707083389));
#32353=CARTESIAN_POINT('Ctrl Pts',(-6.04381298133773,-3.04946076210134,
95.845920042636));
#32354=CARTESIAN_POINT('Ctrl Pts',(-5.95549339426472,-3.21315848206548,
95.854669376933));
#32355=CARTESIAN_POINT('Ctrl Pts',(-5.86717414355334,-3.37685557859334,
95.8634186779086));
#32356=CARTESIAN_POINT('Ctrl Pts',(-5.7721018898642,-3.53690907467015,95.8721679788841));
#32357=CARTESIAN_POINT('Ctrl Pts',(-5.67059953467257,-3.69277536784614,
95.8809172798597));
#32358=CARTESIAN_POINT('Ctrl Pts',(-5.56909755761964,-3.84864108035506,
95.8896665482405));
#32359=CARTESIAN_POINT('Ctrl Pts',(-5.46116568338277,-4.00031938103997,
95.8984158166212));
#32360=CARTESIAN_POINT('Ctrl Pts',(-5.3471704868633,-4.1472951166294,95.907165085002));
#32361=CARTESIAN_POINT('Ctrl Pts',(-5.23317570555735,-4.29427031687775,
95.9159143215146));
#32362=CARTESIAN_POINT('Ctrl Pts',(-5.11311782179024,-4.43654275986878,
95.9246635580272));
#32363=CARTESIAN_POINT('Ctrl Pts',(-4.98740459172233,-4.57362924147411,
95.9334127945399));
#32364=CARTESIAN_POINT('Ctrl Pts',(-4.86169180911071,-4.71071523514187,
95.942161999911));
#32365=CARTESIAN_POINT('Ctrl Pts',(-4.73032391415695,-4.84261509316265,
95.9509112052821));
#32366=CARTESIAN_POINT('Ctrl Pts',(-4.59374707237581,-4.96888084331257,
95.9596604106532));
#32367=CARTESIAN_POINT('Ctrl Pts',(-4.45717070537706,-5.09514615452458,
95.9684095856094));
#32368=CARTESIAN_POINT('Ctrl Pts',(-4.31538563819829,-5.21577720253367,
95.9771587605656));
#32369=CARTESIAN_POINT('Ctrl Pts',(-4.16887341290985,-5.33036429028386,
95.9859079355219));
#32370=CARTESIAN_POINT('Ctrl Pts',(-4.02236168477685,-5.4449509892092,95.9946570807898));
#32371=CARTESIAN_POINT('Ctrl Pts',(-3.87112305634796,-5.5534935923851,96.0034062260577));
#32372=CARTESIAN_POINT('Ctrl Pts',(-3.71567117317098,-5.65562346102233,
96.0121553713256));
#32373=CARTESIAN_POINT('Ctrl Pts',(-3.5602198045769,-5.75775299158528,96.0209044876318));
#32374=CARTESIAN_POINT('Ctrl Pts',(-3.400555448628,-5.85346967275113,96.0296536039379));
#32375=CARTESIAN_POINT('Ctrl Pts',(-3.23722036323839,-5.94244842803324,
96.0384027202441));
#32376=CARTESIAN_POINT('Ctrl Pts',(-3.07388580496494,-6.03142689616247,
96.047151808315));
#32377=CARTESIAN_POINT('Ctrl Pts',(-2.90688079258165,-6.11366734484605,
96.0559008963859));
#32378=CARTESIAN_POINT('Ctrl Pts',(-2.73677251095083,-6.18889046787095,
96.0646499844569));
#32379=CARTESIAN_POINT('Ctrl Pts',(-2.56666476417118,-6.26411335438077,
96.0733990450191));
#32380=CARTESIAN_POINT('Ctrl Pts',(-2.39345402972569,-6.3323188435011,96.0821481055814));
#32381=CARTESIAN_POINT('Ctrl Pts',(-2.21772856474518,-6.39327529620877,
96.0908971661436));
#32382=CARTESIAN_POINT('Ctrl Pts',(-2.04200363768799,-6.45423156231913,
96.0996461999236));
#32383=CARTESIAN_POINT('Ctrl Pts',(-1.86376426620674,-6.50793874251888,
96.1083952337035));
#32384=CARTESIAN_POINT('Ctrl Pts',(-1.6836157819532,-6.5542144379596,96.1171442674835));
#32385=CARTESIAN_POINT('Ctrl Pts',(-1.50346783420542,-6.60048999558525,
96.1258932752077));
#32386=CARTESIAN_POINT('Ctrl Pts',(-1.32141106257962,-6.63933404145352,
96.1346422829319));
#32387=CARTESIAN_POINT('Ctrl Pts',(-1.13806375959802,-6.67061465526901,
96.1433912906561));
#32388=CARTESIAN_POINT('Ctrl Pts',(-0.954716987426327,-6.70189517852379,
96.152140273051));
#32389=CARTESIAN_POINT('Ctrl Pts',(-0.770079973816635,-6.72561226535752,
96.1608892554459));
#32390=CARTESIAN_POINT('Ctrl Pts',(-0.58477977055879,-6.74168536939727,
96.1696382378408));
#32391=CARTESIAN_POINT('Ctrl Pts',(-0.391490647560252,-6.75845143942357,
96.1787644185169));
#32392=CARTESIAN_POINT('Ctrl Pts',(-0.197480213110674,-6.76689975924008,
96.187890599193));
#32393=CARTESIAN_POINT('Ctrl Pts',(-0.0034653263041271,-6.76699911271707,
96.197016779869));
#32394=CARTESIAN_POINT('Ctrl Pts',(0.184486595289811,-6.76709536139791,
96.205857767399));
#32395=CARTESIAN_POINT('Ctrl Pts',(0.372442378179076,-6.75935659726804,
96.2146987549289));
#32396=CARTESIAN_POINT('Ctrl Pts',(0.559750217716033,-6.74380965729067,
96.2235397424588));
#32397=CARTESIAN_POINT('Ctrl Pts',(0.745129914451711,-6.7284227571732,96.2322897210566));
#32398=CARTESIAN_POINT('Ctrl Pts',(0.929874656308157,-6.70538772273556,
96.2410396996544));
#32399=CARTESIAN_POINT('Ctrl Pts',(1.11335688289177,-6.67478280180843,96.2497896782521));
#32400=CARTESIAN_POINT('Ctrl Pts',(1.29683723118258,-6.6441781941814,96.2585395672771));
#32401=CARTESIAN_POINT('Ctrl Pts',(1.4790548072964,-6.60600390230208,96.267289456302));
#32402=CARTESIAN_POINT('Ctrl Pts',(1.65939064804216,-6.56038959797284,96.2760393453269));
#32403=CARTESIAN_POINT('Ctrl Pts',(1.8397247026367,-6.51477574543424,96.2847891476879));
#32404=CARTESIAN_POINT('Ctrl Pts',(2.0181767812525,-6.46172209820286,96.2935389500488));
#32405=CARTESIAN_POINT('Ctrl Pts',(2.1941407234708,-6.4014088672422,96.3022887524098));
#32406=CARTESIAN_POINT('Ctrl Pts',(2.3701029813151,-6.34109621361594,96.3110384710152));
#32407=CARTESIAN_POINT('Ctrl Pts',(2.54357687926338,-6.27352420826204,96.3197881896208));
#32408=CARTESIAN_POINT('Ctrl Pts',(2.7139731778941,-6.19892237325742,96.3285379082262));
#32409=CARTESIAN_POINT('Ctrl Pts',(2.88436790206651,-6.12432122757223,96.3372875459845));
#32410=CARTESIAN_POINT('Ctrl Pts',(3.05168482125718,-6.04269049717689,96.3460371837428));
#32411=CARTESIAN_POINT('Ctrl Pts',(3.21535561996863,-5.95430745235214,96.354786821501));
#32412=CARTESIAN_POINT('Ctrl Pts',(3.37902496074761,-5.86592519481816,96.36353638132));
#32413=CARTESIAN_POINT('Ctrl Pts',(3.53904799384362,-5.77079087940546,96.3722859411391));
#32414=CARTESIAN_POINT('Ctrl Pts',(3.69488118814479,-5.66922763747353,96.3810355009581));
#32415=CARTESIAN_POINT('Ctrl Pts',(3.85071304610328,-5.56766526649401,96.3897849857455));
#32416=CARTESIAN_POINT('Ctrl Pts',(4.00235489705464,-5.45967423581082,96.398534470533));
#32417=CARTESIAN_POINT('Ctrl Pts',(4.14929168607153,-5.34562133936718,96.4072839553204));
#32418=CARTESIAN_POINT('Ctrl Pts',(4.29622726385256,-5.23156938308942,96.4160333679837));
#32419=CARTESIAN_POINT('Ctrl Pts',(4.43845763091568,-5.11145583677635,96.424782780647));
#32420=CARTESIAN_POINT('Ctrl Pts',(4.57549970660466,-4.98568866204667,96.4335321933103));
#32421=CARTESIAN_POINT('Ctrl Pts',(4.71254069814814,-4.85992248226628,96.4422815367566));
#32422=CARTESIAN_POINT('Ctrl Pts',(4.84439326930848,-4.72850295734479,96.4510308802029));
#32423=CARTESIAN_POINT('Ctrl Pts',(4.97060959434248,-4.59187644222169,96.4597802236492));
#32424=CARTESIAN_POINT('Ctrl Pts',(5.09682496280083,-4.45525096257158,96.4685295007855));
#32425=CARTESIAN_POINT('Ctrl Pts',(5.21740397615425,-4.31341878218827,96.4772787779218));
#32426=CARTESIAN_POINT('Ctrl Pts',(5.33193710451538,-4.16686161439184,96.4860280550581));
#32427=CARTESIAN_POINT('Ctrl Pts',(5.44646940289005,-4.02030550865026,96.4947772687911));
#32428=CARTESIAN_POINT('Ctrl Pts',(5.55495572749305,-3.8690247098065,96.5035264825241));
#32429=CARTESIAN_POINT('Ctrl Pts',(5.65702762491114,-3.71353301466302,96.512275696257));
#32430=CARTESIAN_POINT('Ctrl Pts',(5.75909881654828,-3.5580423946742,96.5210248494931));
#32431=CARTESIAN_POINT('Ctrl Pts',(5.85475551250472,-3.39834117620087,96.5297740027293));
#32432=CARTESIAN_POINT('Ctrl Pts',(5.94367283727801,-3.23497174692509,96.5385231559654));
#32433=CARTESIAN_POINT('Ctrl Pts',(6.03258957676034,-3.0716033930151,96.5472722516109));
#32434=CARTESIAN_POINT('Ctrl Pts',(6.11476689685024,-2.90456712830052,96.5560213472564));
#32435=CARTESIAN_POINT('Ctrl Pts',(6.18992570525017,-2.73443024476456,96.564770442902));
#32436=CARTESIAN_POINT('Ctrl Pts',(6.26508404388482,-2.56429442463559,96.573519483863));
#32437=CARTESIAN_POINT('Ctrl Pts',(6.33322384283125,-2.39105828656497,96.5822685248241));
#32438=CARTESIAN_POINT('Ctrl Pts',(6.39411368719867,-2.2153101713256,96.5910175657851));
#32439=CARTESIAN_POINT('Ctrl Pts',(6.45500317120736,-2.03956309620002,96.5997665549675));
#32440=CARTESIAN_POINT('Ctrl Pts',(6.50864269269932,-1.86130434439128,96.6085155441499));
#32441=CARTESIAN_POINT('Ctrl Pts',(6.55485008446205,-1.68113930720447,96.6172645333323));
#32442=CARTESIAN_POINT('Ctrl Pts',(6.6019966474929,-1.49731239212341,96.6261913468617));
#32443=CARTESIAN_POINT('Ctrl Pts',(6.64140563640808,-1.3115011650017,96.6351181603911));
#32444=CARTESIAN_POINT('Ctrl Pts',(6.67293772282089,-1.12436255156156,96.6440449739204));
#32445=CARTESIAN_POINT('Ctrl Pts',(6.703844949498,-0.940932395056388,96.652794888076));
#32446=CARTESIAN_POINT('Ctrl Pts',(6.72718449348872,-0.756227260511841,
96.6615448022315));
#32447=CARTESIAN_POINT('Ctrl Pts',(6.74287707373888,-0.570874564546893,
96.670294716387));
#32448=CARTESIAN_POINT('Ctrl Pts',(6.75856934538641,-0.385525513637644,
96.679044458471));
#32449=CARTESIAN_POINT('Ctrl Pts',(6.76661493004088,-0.199529212423358,
96.687794200555));
#32450=CARTESIAN_POINT('Ctrl Pts',(6.76698649908906,-0.0135174386055113,
96.6965439426389));
#32451=CARTESIAN_POINT('Ctrl Pts',(6.76735806132402,0.172490924440769,96.7052935242848));
#32452=CARTESIAN_POINT('Ctrl Pts',(6.76005588896316,0.358514472896479,96.7140431059307));
#32453=CARTESIAN_POINT('Ctrl Pts',(6.74510478454623,0.54392135965737,96.7227926875766));
#32454=CARTESIAN_POINT('Ctrl Pts',(6.7301539344074,0.729325093145667,96.7315421204157));
#32455=CARTESIAN_POINT('Ctrl Pts',(6.70755443556962,0.914111900251644,96.7402915532547));
#32456=CARTESIAN_POINT('Ctrl Pts',(6.67738304682395,1.09765415591075,96.7490409860938));
#32457=CARTESIAN_POINT('Ctrl Pts',(6.6472121311195,1.28119353390807,96.7577902817551));
#32458=CARTESIAN_POINT('Ctrl Pts',(6.60946960955598,1.46348811672184,96.7665395774164));
#32459=CARTESIAN_POINT('Ctrl Pts',(6.56428366991301,1.64391876347752,96.7752888730777));
#32460=CARTESIAN_POINT('Ctrl Pts',(6.51909837867849,1.82434682109246,96.7840380431886));
#32461=CARTESIAN_POINT('Ctrl Pts',(6.46646995272066,2.00291071819976,96.7927872132994));
#32462=CARTESIAN_POINT('Ctrl Pts',(6.40657713281708,2.17900400212236,96.8015363834102));
#32463=CARTESIAN_POINT('Ctrl Pts',(6.34668509279232,2.35509499309194,96.810285439596));
#32464=CARTESIAN_POINT('Ctrl Pts',(6.27952894037711,2.52871516397663,96.8190344957818));
#32465=CARTESIAN_POINT('Ctrl Pts',(6.20533675061645,2.69927486770964,96.8277835519675));
#32466=CARTESIAN_POINT('Ctrl Pts',(6.12832117908122,2.87632521635486,96.8368655532498));
#32467=CARTESIAN_POINT('Ctrl Pts',(6.04372366626291,3.05007728919579,96.8459475545321));
#32468=CARTESIAN_POINT('Ctrl Pts',(5.95185378008084,3.21989527477796,96.8550295558144));
#32469=CARTESIAN_POINT('Ctrl Pts',(5.86334450817601,3.38350129286353,96.8637793361215));
#32470=CARTESIAN_POINT('Ctrl Pts',(5.76808562057499,3.54345567124565,96.8725291164286));
#32471=CARTESIAN_POINT('Ctrl Pts',(5.66640068804741,3.69921508464916,96.8812788967357));
#32472=CARTESIAN_POINT('Ctrl Pts',(5.56471941108188,3.85496889851902,96.8900283624892));
#32473=CARTESIAN_POINT('Ctrl Pts',(5.45661270815385,4.00652780919267,96.8987778282427));
#32474=CARTESIAN_POINT('Ctrl Pts',(5.34244776449392,4.15337704568872,96.9075272939962));
#32475=CARTESIAN_POINT('Ctrl Pts',(5.22828631819892,4.30022178355889,96.9162764917158));
#32476=CARTESIAN_POINT('Ctrl Pts',(5.10806717844385,4.44235690972315,96.9250256894354));
#32477=CARTESIAN_POINT('Ctrl Pts',(4.98219864545055,4.5792996907028,96.933774887155));
#32478=CARTESIAN_POINT('Ctrl Pts',(4.85633329944363,4.71623900429653,96.9425238633452));
#32479=CARTESIAN_POINT('Ctrl Pts',(4.72481904033988,4.84798602483286,96.9512728395354));
#32480=CARTESIAN_POINT('Ctrl Pts',(4.58810250737539,4.97409332258812,96.9600218157257));
#32481=CARTESIAN_POINT('Ctrl Pts',(4.45137708685986,5.10020881821835,96.9687713606619));
#32482=CARTESIAN_POINT('Ctrl Pts',(4.30944892636398,5.22068366307647,96.9775209055981));
#32483=CARTESIAN_POINT('Ctrl Pts',(4.16280009467009,5.33510865604578,96.9862704505342));
#32484=CARTESIAN_POINT('Ctrl Pts',(4.01615988349162,5.44952692272616,96.9950194811425));
#32485=CARTESIAN_POINT('Ctrl Pts',(3.86479978232629,5.55789587288348,97.0037685117508));
#32486=CARTESIAN_POINT('Ctrl Pts',(3.70923383581492,5.659847467136,97.012517542359));
#32487=CARTESIAN_POINT('Ctrl Pts',(3.55366577799975,5.76180044505114,97.0212666917071));
#32488=CARTESIAN_POINT('Ctrl Pts',(3.39389200027285,5.85733573570801,97.0300158410551));
#32489=CARTESIAN_POINT('Ctrl Pts',(3.23045513626497,5.9461288762168,97.0387649904031));
#32490=CARTESIAN_POINT('Ctrl Pts',(3.18695122151889,5.96976399206524,97.0410938545161));
#32491=CARTESIAN_POINT('Ctrl Pts',(3.14318791262828,5.99292165435248,97.0434227186292));
#32492=CARTESIAN_POINT('Ctrl Pts',(3.09917575053274,6.01559628526631,97.0457515827422));
#32493=CARTESIAN_POINT('Ctrl Pts',(3.09917575053267,6.01559628526635,95.0455637664379));
#32494=CARTESIAN_POINT('Ctrl Pts',(2.943906770375,6.09558932922995,95.0537737090146));
#32495=CARTESIAN_POINT('Ctrl Pts',(2.78564419716587,6.16951272082007,95.0619836515913));
#32496=CARTESIAN_POINT('Ctrl Pts',(2.62490874004041,6.23715825568499,95.070193594168));
#32497=CARTESIAN_POINT('Ctrl Pts',(2.46407107433121,6.30484680504367,95.0784087572891));
#32498=CARTESIAN_POINT('Ctrl Pts',(2.30075772543929,6.36624941518948,95.0866239204103));
#32499=CARTESIAN_POINT('Ctrl Pts',(2.13550538356776,6.42120749989853,95.0948390835315));
#32500=CARTESIAN_POINT('Ctrl Pts',(1.97003647291874,6.47623760903449,95.1030650129015));
#32501=CARTESIAN_POINT('Ctrl Pts',(1.80262383819817,6.52480622767291,95.1112909422715));
#32502=CARTESIAN_POINT('Ctrl Pts',(1.63381603663925,6.56680547590839,95.1195168716415));
#32503=CARTESIAN_POINT('Ctrl Pts',(1.58139506131994,6.57984777333096,95.1220713225407));
#32504=CARTESIAN_POINT('Ctrl Pts',(1.52883959571413,6.59225694302585,95.1246257734398));
#32505=CARTESIAN_POINT('Ctrl Pts',(1.47616617480197,6.60403077100422,95.127180224339));
#32506=CARTESIAN_POINT('Ctrl Pts',(1.30656773086973,6.64194026823597,95.1354050726611));
#32507=CARTESIAN_POINT('Ctrl Pts',(1.13526998503762,6.67336557312749,95.1436299209831));
#32508=CARTESIAN_POINT('Ctrl Pts',(0.962809917477377,6.69815542241349,95.1518547693052));
#32509=CARTESIAN_POINT('Ctrl Pts',(0.790544078190971,6.7229173528328,95.1600703546244));
#32510=CARTESIAN_POINT('Ctrl Pts',(0.617118875677853,6.74105865770386,95.1682859399436));
#32511=CARTESIAN_POINT('Ctrl Pts',(0.443084048288832,6.75247847283884,95.1765015252628));
#32512=CARTESIAN_POINT('Ctrl Pts',(0.269210255640676,6.76388772119821,95.184709508686));
#32513=CARTESIAN_POINT('Ctrl Pts',(0.0947283172537854,6.76858784255455,
95.1929174921093));
#32514=CARTESIAN_POINT('Ctrl Pts',(-0.0798041992942283,6.76652941246656,
95.2011254755325));
#32515=CARTESIAN_POINT('Ctrl Pts',(-0.254210276332712,6.76447247360149,
95.2093275127091));
#32516=CARTESIAN_POINT('Ctrl Pts',(-0.428666501257262,6.75566673983363,
95.2175295498856));
#32517=CARTESIAN_POINT('Ctrl Pts',(-0.602612485437827,6.7401147759066,95.2257315870622));
#32518=CARTESIAN_POINT('Ctrl Pts',(-0.77646738491674,6.72457095557656,95.2339293293416));
#32519=CARTESIAN_POINT('Ctrl Pts',(-0.949812219419549,6.70228797442919,
95.242127071621));
#32520=CARTESIAN_POINT('Ctrl Pts',(-1.12208881749832,6.67332043930495,95.2503248139004));
#32521=CARTESIAN_POINT('Ctrl Pts',(-1.29433266003202,6.6443584118783,95.2585209975147));
#32522=CARTESIAN_POINT('Ctrl Pts',(-1.46550831622571,6.60871441534547,95.2667171811291));
#32523=CARTESIAN_POINT('Ctrl Pts',(-1.63506463190266,6.56649470033298,95.2749133647434));
#32524=CARTESIAN_POINT('Ctrl Pts',(-1.80460846586917,6.52427809328054,95.2831089450043));
#32525=CARTESIAN_POINT('Ctrl Pts',(-1.97253284831188,6.47548681760763,95.2913045252652));
#32526=CARTESIAN_POINT('Ctrl Pts',(-2.13829874066011,6.42027783633165,95.2995001055261));
#32527=CARTESIAN_POINT('Ctrl Pts',(-2.30408258946872,6.36506287458604,95.3076965735667));
#32528=CARTESIAN_POINT('Ctrl Pts',(-2.46770714183432,6.30342893561063,95.3158930416074));
#32529=CARTESIAN_POINT('Ctrl Pts',(-2.62865034699279,6.23558227860516,95.3240895096481));
#32530=CARTESIAN_POINT('Ctrl Pts',(-2.78964026803451,6.16771592821465,95.3322883568215));
#32531=CARTESIAN_POINT('Ctrl Pts',(-2.94794696103396,6.09363340715741,95.3404872039949));
#32532=CARTESIAN_POINT('Ctrl Pts',(-3.10307006934435,6.01358837506686,95.3486860511683));
#32533=CARTESIAN_POINT('Ctrl Pts',(-3.25835529638719,5.93345968813414,95.3568934669343));
#32534=CARTESIAN_POINT('Ctrl Pts',(-3.41044997221247,5.84735620540302,95.3651008827003));
#32535=CARTESIAN_POINT('Ctrl Pts',(-3.55887912042718,5.75557715665314,95.3733082984662));
#32536=CARTESIAN_POINT('Ctrl Pts',(-3.70738782144522,5.66374891756092,95.3815201131184));
#32537=CARTESIAN_POINT('Ctrl Pts',(-3.85222678100859,5.56623924854325,95.3897319277705));
#32538=CARTESIAN_POINT('Ctrl Pts',(-3.99295167116383,5.46338960277866,95.3979437424227));
#32539=CARTESIAN_POINT('Ctrl Pts',(-4.13388380011314,5.36038849527525,95.4061676502203));
#32540=CARTESIAN_POINT('Ctrl Pts',(-4.27068947043723,5.25203191798305,95.4143915580179));
#32541=CARTESIAN_POINT('Ctrl Pts',(-4.40295800230478,5.13870118122666,95.4226154658155));
#32542=CARTESIAN_POINT('Ctrl Pts',(-4.52517168297585,5.03398567348949,95.4302142047389));
#32543=CARTESIAN_POINT('Ctrl Pts',(-4.6435120554334,4.92502408966409,95.4378129436624));
#32544=CARTESIAN_POINT('Ctrl Pts',(-4.75768487240652,4.81214335352493,95.4454116825858));
#32545=CARTESIAN_POINT('Ctrl Pts',(-4.87840941474031,4.6927850371587,95.4534464697021));
#32546=CARTESIAN_POINT('Ctrl Pts',(-4.99485389248265,4.56866854002903,95.4614812568183));
#32547=CARTESIAN_POINT('Ctrl Pts',(-5.10660816305721,4.44013987043173,95.4695160439346));
#32548=CARTESIAN_POINT('Ctrl Pts',(-5.21823051087443,4.31176292529563,95.4775413462118));
#32549=CARTESIAN_POINT('Ctrl Pts',(-5.32517342373367,4.17898445205639,95.485566648489));
#32550=CARTESIAN_POINT('Ctrl Pts',(-5.42706130152284,4.04218933617825,95.4935919507662));
#32551=CARTESIAN_POINT('Ctrl Pts',(-5.52885159927958,3.90552523168374,95.501609567053));
#32552=CARTESIAN_POINT('Ctrl Pts',(-5.62559627334275,3.76485243981903,95.5096271833397));
#32553=CARTESIAN_POINT('Ctrl Pts',(-5.71695805868633,3.62059105053601,95.5176447996264));
#32554=CARTESIAN_POINT('Ctrl Pts',(-5.80824657868332,3.47644534814162,95.5256559863821));
#32555=CARTESIAN_POINT('Ctrl Pts',(-5.89416060514533,3.32871709553155,95.5336671731378));
#32556=CARTESIAN_POINT('Ctrl Pts',(-5.97440465955954,3.17785744863317,95.5416783598935));
#32557=CARTESIAN_POINT('Ctrl Pts',(-6.05461363157628,3.02706375700254,95.5496860441886));
#32558=CARTESIAN_POINT('Ctrl Pts',(-6.1291573868748,2.87314172643022,95.5576937284837));
#32559=CARTESIAN_POINT('Ctrl Pts',(-6.19778506576384,2.71656939513695,95.5657014127788));
#32560=CARTESIAN_POINT('Ctrl Pts',(-6.26639652982033,2.56003405757821,95.5737072050784));
#32561=CARTESIAN_POINT('Ctrl Pts',(-6.32909454842009,2.40085001021319,95.581712997378));
#32562=CARTESIAN_POINT('Ctrl Pts',(-6.38567540637297,2.23951749366766,95.5897187896776));
#32563=CARTESIAN_POINT('Ctrl Pts',(-6.44225426242193,2.07819068527514,95.597724298722));
#32564=CARTESIAN_POINT('Ctrl Pts',(-6.49271626553911,1.91471591483534,95.6057298077663));
#32565=CARTESIAN_POINT('Ctrl Pts',(-6.53690686631789,1.74961070558169,95.6137353168106));
#32566=CARTESIAN_POINT('Ctrl Pts',(-6.58112025794606,1.58442034500872,95.6217449546141));
#32567=CARTESIAN_POINT('Ctrl Pts',(-6.61905568935104,1.41759823012135,95.6297545924177));
#32568=CARTESIAN_POINT('Ctrl Pts',(-6.65060917076422,1.2496746207501,95.6377642302212));
#32569=CARTESIAN_POINT('Ctrl Pts',(-6.68217182860439,1.0817021756031,95.6457761973987));
#32570=CARTESIAN_POINT('Ctrl Pts',(-6.70734878206237,0.912627969872602,
95.6537881645761));
#32571=CARTESIAN_POINT('Ctrl Pts',(-6.72608773376436,0.742989096625667,
95.6618001317536));
#32572=CARTESIAN_POINT('Ctrl Pts',(-6.74484382719967,0.573195043709559,
95.6698194279966));
#32573=CARTESIAN_POINT('Ctrl Pts',(-6.75715013196647,0.402835666939462,
95.6778387242395));
#32574=CARTESIAN_POINT('Ctrl Pts',(-6.7630064226757,0.232450267470704,95.6858580204825));
#32575=CARTESIAN_POINT('Ctrl Pts',(-6.7656701866882,0.15494959035367,95.6895056387102));
#32576=CARTESIAN_POINT('Ctrl Pts',(-6.76700020042621,0.0774435045898423,
95.6931532569379));
#32577=CARTESIAN_POINT('Ctrl Pts',(-6.76699999997734,-1.75112276718149E-5,
95.6968008751656));
#32578=CARTESIAN_POINT('',(-6.76699859668926,-0.00435802771595241,95.3028202161534));
#32579=CARTESIAN_POINT('Ctrl Pts',(3.09917575053252,6.01559628526642,94.6512396476019));
#32580=CARTESIAN_POINT('Ctrl Pts',(2.94401132479335,6.09553546382698,94.6594632335912));
#32581=CARTESIAN_POINT('Ctrl Pts',(2.78590477759022,6.16938874478998,94.6676868195806));
#32582=CARTESIAN_POINT('Ctrl Pts',(2.62538040155148,6.23695973589291,94.67591040557));
#32583=CARTESIAN_POINT('Ctrl Pts',(2.46463890552551,6.30462212129426,94.6841451145111));
#32584=CARTESIAN_POINT('Ctrl Pts',(2.30147338489664,6.36598512597349,94.6923798234522));
#32585=CARTESIAN_POINT('Ctrl Pts',(2.13642342298202,6.42090211401278,94.7006145323933));
#32586=CARTESIAN_POINT('Ctrl Pts',(2.10488202478951,6.431396867039,94.7021882027577));
#32587=CARTESIAN_POINT('Ctrl Pts',(2.07327183631911,6.44165636140993,94.7037618731221));
#32588=CARTESIAN_POINT('Ctrl Pts',(2.04159666135396,6.45167978687321,94.7053355434865));
#32589=CARTESIAN_POINT('Ctrl Pts',(1.87744184354736,6.50362562718925,94.7134910018933));
#32590=CARTESIAN_POINT('Ctrl Pts',(1.71103543735194,6.54938703930309,94.7216464603001));
#32591=CARTESIAN_POINT('Ctrl Pts',(1.54288826862621,6.58876200742868,94.7298019187068));
#32592=CARTESIAN_POINT('Ctrl Pts',(1.37494575710755,6.62808905104228,94.7379474508487));
#32593=CARTESIAN_POINT('Ctrl Pts',(1.20526705246651,6.66104504104213,94.7460929829906));
#32594=CARTESIAN_POINT('Ctrl Pts',(1.03438091509877,6.68747673808885,94.7542385151325));
#32595=CARTESIAN_POINT('Ctrl Pts',(0.86366683469625,6.71388182234152,94.762375845933));
#32596=CARTESIAN_POINT('Ctrl Pts',(0.691748100327034,6.73377563589263,94.7705131767336));
#32597=CARTESIAN_POINT('Ctrl Pts',(0.519166526651232,6.74705529231864,94.7786505075341));
#32598=CARTESIAN_POINT('Ctrl Pts',(0.346722448441673,6.76032436886341,94.7867813553361));
#32599=CARTESIAN_POINT('Ctrl Pts',(0.173616945133653,6.766989752579,94.7949122031381));
#32600=CARTESIAN_POINT('Ctrl Pts',(0.000399870219098874,6.76699998818559,
94.8030430509401));
#32601=CARTESIAN_POINT('Ctrl Pts',(-0.172715590171761,6.76701021778766,
94.8111691289339));
#32602=CARTESIAN_POINT('Ctrl Pts',(-0.345942127238149,6.76037307423085,
94.8192952069277));
#32603=CARTESIAN_POINT('Ctrl Pts',(-0.518726947958766,6.74708910223227,
94.8274212849215));
#32604=CARTESIAN_POINT('Ctrl Pts',(-0.692124432095885,6.73375802769519,
94.8355761765037));
#32605=CARTESIAN_POINT('Ctrl Pts',(-0.86507669044076,6.71373287892692,94.8437310680859));
#32606=CARTESIAN_POINT('Ctrl Pts',(-1.0370266241599,6.68706697893654,94.8518859596681));
#32607=CARTESIAN_POINT('Ctrl Pts',(-1.20830601325809,6.66050506663267,94.8600090500244));
#32608=CARTESIAN_POINT('Ctrl Pts',(-1.3785905197743,6.6273541767211,94.8681321403806));
#32609=CARTESIAN_POINT('Ctrl Pts',(-1.5473365971255,6.58771875957042,94.8762552307369));
#32610=CARTESIAN_POINT('Ctrl Pts',(-1.7160959251891,6.54808023006584,94.8843789589554));
#32611=CARTESIAN_POINT('Ctrl Pts',(-1.88331622730901,6.50195624267316,94.8925026871738));
#32612=CARTESIAN_POINT('Ctrl Pts',(-2.04846627137669,6.44950191371645,94.9006264153922));
#32613=CARTESIAN_POINT('Ctrl Pts',(-2.21366070337928,6.39703348643265,94.9087523270525));
#32614=CARTESIAN_POINT('Ctrl Pts',(-2.37678342085705,6.33823144041911,94.9168782387128));
#32615=CARTESIAN_POINT('Ctrl Pts',(-2.53732045830639,6.27330007985111,94.9250041503731));
#32616=CARTESIAN_POINT('Ctrl Pts',(-2.69888414679854,6.20795347648245,94.9331820280832));
#32617=CARTESIAN_POINT('Ctrl Pts',(-2.85782862088997,6.13639903207623,94.9413599057933));
#32618=CARTESIAN_POINT('Ctrl Pts',(-3.01365322584842,6.05889290500611,94.9495377835033));
#32619=CARTESIAN_POINT('Ctrl Pts',(-3.16873411376371,5.98175669787045,94.9576766299768));
#32620=CARTESIAN_POINT('Ctrl Pts',(-3.32072455663284,5.89872572514541,94.9658154764502));
#32621=CARTESIAN_POINT('Ctrl Pts',(-3.46915873002406,5.81009696183273,94.9739543229237));
#32622=CARTESIAN_POINT('Ctrl Pts',(-3.61866066578788,5.7208306468267,94.9821517162521));
#32623=CARTESIAN_POINT('Ctrl Pts',(-3.76455465845203,5.6258859081452,94.9903491095805));
#32624=CARTESIAN_POINT('Ctrl Pts',(-3.90639760901627,5.52560826699396,94.9985465029089));
#32625=CARTESIAN_POINT('Ctrl Pts',(-4.04824055958042,5.42533062584278,95.0067438962373));
#32626=CARTESIAN_POINT('Ctrl Pts',(-4.18603220978262,5.31972035716278,95.0149412895657));
#32627=CARTESIAN_POINT('Ctrl Pts',(-4.31936653152684,5.20916133041834,95.0231386828941));
#32628=CARTESIAN_POINT('Ctrl Pts',(-4.45143330188874,5.09965334023632,95.0312581471708));
#32629=CARTESIAN_POINT('Ctrl Pts',(-4.57954166030533,4.98494649229571,95.0393776114476));
#32630=CARTESIAN_POINT('Ctrl Pts',(-4.70324933048561,4.86536069940212,95.0474970757243));
#32631=CARTESIAN_POINT('Ctrl Pts',(-4.82681675105671,4.74591048307133,95.0556073348185));
#32632=CARTESIAN_POINT('Ctrl Pts',(-4.94599315118097,4.6215925855464,95.0637175939127));
#32633=CARTESIAN_POINT('Ctrl Pts',(-5.06036782651735,4.49276824022207,95.0718278530068));
#32634=CARTESIAN_POINT('Ctrl Pts',(-5.17463735853119,4.36406232163556,95.0799306564332));
#32635=CARTESIAN_POINT('Ctrl Pts',(-5.28411370980808,4.23085847657609,95.0880334598595));
#32636=CARTESIAN_POINT('Ctrl Pts',(-5.38842172690336,4.0935559472219,95.0961362632859));
#32637=CARTESIAN_POINT('Ctrl Pts',(-5.49265620418498,3.95635021965445,95.104233354029));
#32638=CARTESIAN_POINT('Ctrl Pts',(-5.59172938012883,3.81505185422318,95.1123304447722));
#32639=CARTESIAN_POINT('Ctrl Pts',(-5.68530527557364,3.67009440253716,95.1204275355154));
#32640=CARTESIAN_POINT('Ctrl Pts',(-5.77883951687644,3.52520147685166,95.1285210219396));
#32641=CARTESIAN_POINT('Ctrl Pts',(-5.86688114923733,3.37665301685795,95.1366145083639));
#32642=CARTESIAN_POINT('Ctrl Pts',(-5.94913655838172,3.22491289955653,95.1447079947882));
#32643=CARTESIAN_POINT('Ctrl Pts',(-6.0313740854861,3.07320577002914,95.1527997217166));
#32644=CARTESIAN_POINT('Ctrl Pts',(-6.107827717105,2.91830868845482,95.1608914486451));
#32645=CARTESIAN_POINT('Ctrl Pts',(-6.17824901137132,2.76071153029239,95.1689831755736));
#32646=CARTESIAN_POINT('Ctrl Pts',(-6.2486686519124,2.6031180730332,95.1770747124815));
#32647=CARTESIAN_POINT('Ctrl Pts',(-6.31305608682467,2.44282500258794,95.1851662493894));
#32648=CARTESIAN_POINT('Ctrl Pts',(-6.37121042519647,2.28034355259636,95.1932577862973));
#32649=CARTESIAN_POINT('Ctrl Pts',(-6.42937467534367,2.11783440940623,95.2013507023198));
#32650=CARTESIAN_POINT('Ctrl Pts',(-6.48130359055544,1.95313649195031,95.2094436183423));
#32651=CARTESIAN_POINT('Ctrl Pts',(-6.52684571990895,1.78677753190102,95.2175365343648));
#32652=CARTESIAN_POINT('Ctrl Pts',(-6.57242486755529,1.62028334926142,95.2256360286027));
#32653=CARTESIAN_POINT('Ctrl Pts',(-6.61160676440659,1.45212578406303,95.2337355228406));
#32654=CARTESIAN_POINT('Ctrl Pts',(-6.64429065493007,1.28284476567078,95.2418350170784));
#32655=CARTESIAN_POINT('Ctrl Pts',(-6.67698945208373,1.11348654075579,95.2499382053736));
#32656=CARTESIAN_POINT('Ctrl Pts',(-6.70318428156195,0.943004205998225,
95.2580413936688));
#32657=CARTESIAN_POINT('Ctrl Pts',(-6.72282616721505,0.771943861565483,
95.266144581964));
#32658=CARTESIAN_POINT('Ctrl Pts',(-6.74249097732885,0.600683868982252,
95.2742572276619));
#32659=CARTESIAN_POINT('Ctrl Pts',(-6.75558754225939,0.42884488681141,95.2823698733597));
#32660=CARTESIAN_POINT('Ctrl Pts',(-6.76211896818731,0.25697482382795,95.2904825190576));
#32661=CARTESIAN_POINT('Ctrl Pts',(-6.76542996181808,0.169848262164658,
95.2945950847562));
#32662=CARTESIAN_POINT('Ctrl Pts',(-6.76705467190439,0.0827136769254795,
95.2987076504548));
#32663=CARTESIAN_POINT('Ctrl Pts',(-6.76699859668926,-0.00435802771576677,
95.3028202161534));
#32664=CARTESIAN_POINT('Ctrl Pts',(-6.76699859668877,-0.00435802848384897,
95.3028202161897));
#32665=CARTESIAN_POINT('Ctrl Pts',(-6.76682533277866,-0.273396342687137,
95.3155274182271));
#32666=CARTESIAN_POINT('Ctrl Pts',(-6.75060771707868,-0.541919813427472,
95.3282346202645));
#32667=CARTESIAN_POINT('Ctrl Pts',(-6.71852819966011,-0.808497266768375,
95.3409418223019));
#32668=CARTESIAN_POINT('Ctrl Pts',(-6.69776103485891,-0.981070246392114,
95.3491680233207));
#32669=CARTESIAN_POINT('Ctrl Pts',(-6.67031147402146,-1.15308377659327,
95.3573942243396));
#32670=CARTESIAN_POINT('Ctrl Pts',(-6.63621604054561,-1.3239809904999,95.3656204253584));
#32671=CARTESIAN_POINT('Ctrl Pts',(-6.60215890610328,-1.49468623740521,
95.3738373859742));
#32672=CARTESIAN_POINT('Ctrl Pts',(-6.56147083387031,-1.66427731645193,
95.38205434659));
#32673=CARTESIAN_POINT('Ctrl Pts',(-6.51424011597687,-1.83220214807146,
95.3902713072057));
#32674=CARTESIAN_POINT('Ctrl Pts',(-6.4670529722603,-1.99997205538241,95.3984806870073));
#32675=CARTESIAN_POINT('Ctrl Pts',(-6.4133353005395,-2.16607843368287,95.4066900668089));
#32676=CARTESIAN_POINT('Ctrl Pts',(-6.35322649846421,-2.32997898256877,
95.4148994466105));
#32677=CARTESIAN_POINT('Ctrl Pts',(-6.29316109120236,-2.49376120546088,
95.4231028997509));
#32678=CARTESIAN_POINT('Ctrl Pts',(-6.22671386686271,-2.65534043552512,
95.4313063528913));
#32679=CARTESIAN_POINT('Ctrl Pts',(-6.1540741762698,-2.81418905423377,95.4395098060317));
#32680=CARTESIAN_POINT('Ctrl Pts',(-6.08147235567091,-2.97295485876479,
95.4477089823818));
#32681=CARTESIAN_POINT('Ctrl Pts',(-6.00268464912206,-3.12899256258344,
95.455908158732));
#32682=CARTESIAN_POINT('Ctrl Pts',(-5.91794873054344,-3.28179399454921,
95.4641073350821));
#32683=CARTESIAN_POINT('Ctrl Pts',(-5.8332287563066,-3.43456667461972,95.4723049686335));
#32684=CARTESIAN_POINT('Ctrl Pts',(-5.74256296776677,-3.5841039794754,95.4805026021849));
#32685=CARTESIAN_POINT('Ctrl Pts',(-5.64623538618265,-3.72992157609498,
95.4887002357363));
#32686=CARTESIAN_POINT('Ctrl Pts',(-5.54991474254855,-3.87572867026883,
95.4968972788568));
#32687=CARTESIAN_POINT('Ctrl Pts',(-5.44793331496594,-4.01781629000376,
95.5050943219774));
#32688=CARTESIAN_POINT('Ctrl Pts',(-5.34061889447139,-4.15572843482526,
95.513291365098));
#32689=CARTESIAN_POINT('Ctrl Pts',(-5.23329269903204,-4.29365571188979,
95.5214893076292));
#32690=CARTESIAN_POINT('Ctrl Pts',(-5.1206325651975,-4.4274063181409,95.5296872501603));
#32691=CARTESIAN_POINT('Ctrl Pts',(-5.00300709506265,-4.55655670509572,
95.5378851926915));
#32692=CARTESIAN_POINT('Ctrl Pts',(-4.88534734030277,-4.68574473587535,
95.5460855247));
#32693=CARTESIAN_POINT('Ctrl Pts',(-4.7627196079308,-4.81032961145549,95.5542858567084));
#32694=CARTESIAN_POINT('Ctrl Pts',(-4.63552995592562,-4.92992403873693,
95.5624861887169));
#32695=CARTESIAN_POINT('Ctrl Pts',(-4.50820773792677,-5.04964311573508,
95.5706950676877));
#32696=CARTESIAN_POINT('Ctrl Pts',(-4.3763143626688,-5.16436110680497,95.5789039466584));
#32697=CARTESIAN_POINT('Ctrl Pts',(-4.24029038600628,-5.2737298416152,95.5871128256291));
#32698=CARTESIAN_POINT('Ctrl Pts',(-4.10419338851791,-5.38315728809917,
95.5953261113166));
#32699=CARTESIAN_POINT('Ctrl Pts',(-3.96396165690328,-5.48722954013065,
95.603539397004));
#32700=CARTESIAN_POINT('Ctrl Pts',(-3.8200653395177,-5.58564139574101,95.6117526826914));
#32701=CARTESIAN_POINT('Ctrl Pts',(-3.67595851955472,-5.68419721576705,
95.6199779834034));
#32702=CARTESIAN_POINT('Ctrl Pts',(-3.52817670420056,-5.77707590056016,
95.6282032841155));
#32703=CARTESIAN_POINT('Ctrl Pts',(-3.37721638996576,-5.86401726253825,
95.6364285848276));
#32704=CARTESIAN_POINT('Ctrl Pts',(-3.24069099575598,-5.94264523689934,
95.6438673771215));
#32705=CARTESIAN_POINT('Ctrl Pts',(-3.10156638207696,-6.01641757989647,
95.6513061694154));
#32706=CARTESIAN_POINT('Ctrl Pts',(-2.96022349961675,-6.08517590808325,
95.6587449617093));
#32707=CARTESIAN_POINT('Ctrl Pts',(-2.80531854339851,-6.16053170691812,
95.6668975179225));
#32708=CARTESIAN_POINT('Ctrl Pts',(-2.64729201842329,-6.23008659198876,
95.6750500741358));
#32709=CARTESIAN_POINT('Ctrl Pts',(-2.48662143000296,-6.29356837285892,
95.683202630349));
#32710=CARTESIAN_POINT('Ctrl Pts',(-2.32613698233264,-6.35697660855556,
95.6913457416294));
#32711=CARTESIAN_POINT('Ctrl Pts',(-2.16301490534355,-6.41432561260147,
95.6994888529097));
#32712=CARTESIAN_POINT('Ctrl Pts',(-1.99775729792893,-6.4653889889605,95.7076319641901));
#32713=CARTESIAN_POINT('Ctrl Pts',(-1.8326564020831,-6.5164039426058,95.7157673534674));
#32714=CARTESIAN_POINT('Ctrl Pts',(-1.66542435438282,-6.56114502813015,
95.7239027427447));
#32715=CARTESIAN_POINT('Ctrl Pts',(-1.49658323480923,-6.5994338864245,95.7320381320221));
#32716=CARTESIAN_POINT('Ctrl Pts',(-1.32786674740724,-6.63769448132206,
95.7401675160607));
#32717=CARTESIAN_POINT('Ctrl Pts',(-1.15754390817,-6.66951225203777,95.7482969000992));
#32718=CARTESIAN_POINT('Ctrl Pts',(-0.986151962342344,-6.69475864442986,
95.7564262841378));
#32719=CARTESIAN_POINT('Ctrl Pts',(-0.814850531104618,-6.71999170383338,
95.76455137493));
#32720=CARTESIAN_POINT('Ctrl Pts',(-0.642481478574638,-6.73866024328767,
95.7726764657221));
#32721=CARTESIAN_POINT('Ctrl Pts',(-0.469592245319419,-6.7506867889968,
95.7808015565143));
#32722=CARTESIAN_POINT('Ctrl Pts',(-0.296043056380474,-6.76275924263811,
95.7889576625394));
#32723=CARTESIAN_POINT('Ctrl Pts',(-0.121970072306283,-6.76813881991057,
95.7971137685645));
#32724=CARTESIAN_POINT('Ctrl Pts',(0.0520672536939946,-6.76679968678642,
95.8052698745896));
#32725=CARTESIAN_POINT('Ctrl Pts',(0.225404110931855,-6.76546594343091,
95.813393153763));
#32726=CARTESIAN_POINT('Ctrl Pts',(0.398705228442972,-6.75746749683414,
95.8215164329364));
#32727=CARTESIAN_POINT('Ctrl Pts',(0.5714177203458,-6.7428310663159,95.8296397121098));
#32728=CARTESIAN_POINT('Ctrl Pts',(0.74415321037656,-6.72819268683324,95.8377640729665));
#32729=CARTESIAN_POINT('Ctrl Pts',(0.91629955412383,-6.70691459375123,95.8458884338232));
#32730=CARTESIAN_POINT('Ctrl Pts',(1.08730896929934,-6.67907540047881,95.8540127946799));
#32731=CARTESIAN_POINT('Ctrl Pts',(1.25837369124453,-6.65122720363283,95.8621397830653));
#32732=CARTESIAN_POINT('Ctrl Pts',(1.42830039152984,-6.61681373987404,95.8702667714507));
#32733=CARTESIAN_POINT('Ctrl Pts',(1.59655150175245,-6.57596474308158,95.8783937598361));
#32734=CARTESIAN_POINT('Ctrl Pts',(1.76589033624718,-6.53485166217554,95.8865732882762));
#32735=CARTESIAN_POINT('Ctrl Pts',(1.93353147535555,-6.48721963844231,95.8947528167163));
#32736=CARTESIAN_POINT('Ctrl Pts',(2.09894324979684,-6.43325160662416,95.9029323451564));
#32737=CARTESIAN_POINT('Ctrl Pts',(2.26357604686572,-6.37953772766642,95.9110733535601));
#32738=CARTESIAN_POINT('Ctrl Pts',(2.42600011122687,-6.31954757571661,95.9192143619638));
#32739=CARTESIAN_POINT('Ctrl Pts',(2.58571253791689,-6.25350938843618,95.9273553703674));
#32740=CARTESIAN_POINT('Ctrl Pts',(2.74655850879154,-6.18700250122608,95.9355541588257));
#32741=CARTESIAN_POINT('Ctrl Pts',(2.90465386627124,-6.1143615699947,95.943752947284));
#32742=CARTESIAN_POINT('Ctrl Pts',(3.059511629435,-6.03586593533621,95.9519517357423));
#32743=CARTESIAN_POINT('Ctrl Pts',(3.21436939259886,-5.95737030067766,95.9601505242005));
#32744=CARTESIAN_POINT('Ctrl Pts',(3.36598926841503,-5.87302019974696,95.9683493126588));
#32745=CARTESIAN_POINT('Ctrl Pts',(3.51391566987933,-5.7831380465087,95.9765481011171));
#32746=CARTESIAN_POINT('Ctrl Pts',(3.66246023659221,-5.69288028740801,95.9847811512491));
#32747=CARTESIAN_POINT('Ctrl Pts',(3.80774221389315,-5.59676367682404,95.9930142013811));
#32748=CARTESIAN_POINT('Ctrl Pts',(3.94926832976421,-5.49504946834161,96.0012472515131));
#32749=CARTESIAN_POINT('Ctrl Pts',(4.09062590978606,-5.39345638584642,96.009470497348));
#32750=CARTESIAN_POINT('Ctrl Pts',(4.22823624653368,-5.28627918585261,96.0176937431829));
#32751=CARTESIAN_POINT('Ctrl Pts',(4.36163156742462,-5.17382441430371,96.0259169890177));
#32752=CARTESIAN_POINT('Ctrl Pts',(4.49489473435468,-5.06148105103645,96.0341320881312));
#32753=CARTESIAN_POINT('Ctrl Pts',(4.62395092959647,-4.9438707580321,96.0423471872447));
#32754=CARTESIAN_POINT('Ctrl Pts',(4.74836216306603,-4.82134273500266,96.0505622863583));
#32755=CARTESIAN_POINT('Ctrl Pts',(4.87267503523879,-4.69891158437696,96.0587708904972));
#32756=CARTESIAN_POINT('Ctrl Pts',(4.99235000622279,-4.57157069810194,96.0669794946361));
#32757=CARTESIAN_POINT('Ctrl Pts',(5.10698287118173,-4.43970888161109,96.075188098775));
#32758=CARTESIAN_POINT('Ctrl Pts',(5.22154803553013,-4.30792494091517,96.083391855024));
#32759=CARTESIAN_POINT('Ctrl Pts',(5.33107679166752,-4.17162565859752,96.091595611273));
#32760=CARTESIAN_POINT('Ctrl Pts',(5.43520240333724,-4.0312360182402,96.0997993675219));
#32761=CARTESIAN_POINT('Ctrl Pts',(5.53929720686305,-3.89088791563881,96.1080006964862));
#32762=CARTESIAN_POINT('Ctrl Pts',(5.63799183417681,-3.74645215076367,96.1162020254505));
#32763=CARTESIAN_POINT('Ctrl Pts',(5.73096025495111,-3.5983862433278,96.1244033544148));
#32764=CARTESIAN_POINT('Ctrl Pts',(5.82391585449262,-3.45034075559415,96.1326035523375));
#32765=CARTESIAN_POINT('Ctrl Pts',(5.91114662916736,-3.29866642528091,96.1408037502602));
#32766=CARTESIAN_POINT('Ctrl Pts',(5.99237025890225,-3.14384918216886,96.149003948183));
#32767=CARTESIAN_POINT('Ctrl Pts',(6.07359740649754,-2.98902523379813,96.1572045012628));
#32768=CARTESIAN_POINT('Ctrl Pts',(6.14881672430619,-2.83105841870121,96.1654050543427));
#32769=CARTESIAN_POINT('Ctrl Pts',(6.21779215777247,-2.67045870268445,96.1736056074225));
#32770=CARTESIAN_POINT('Ctrl Pts',(6.28678307831959,-2.50982292715116,96.1818080017757));
#32771=CARTESIAN_POINT('Ctrl Pts',(6.34952718089141,-2.34655340240013,96.190010396129));
#32772=CARTESIAN_POINT('Ctrl Pts',(6.4058367827842,-2.18117952317754,96.1982127904822));
#32773=CARTESIAN_POINT('Ctrl Pts',(6.46219904405341,-2.01565099030683,96.206422855516));
#32774=CARTESIAN_POINT('Ctrl Pts',(6.51211466676788,-1.84801451078317,96.2146329205499));
#32775=CARTESIAN_POINT('Ctrl Pts',(6.55544577102335,-1.67881498181666,96.2228429855837));
#32776=CARTESIAN_POINT('Ctrl Pts',(6.59879761277662,-1.50953447695721,96.231056979809));
#32777=CARTESIAN_POINT('Ctrl Pts',(6.63555857770002,-1.33868978124384,96.2392709740343));
#32778=CARTESIAN_POINT('Ctrl Pts',(6.66564207759946,-1.16683533257079,96.2474849682597));
#32779=CARTESIAN_POINT('Ctrl Pts',(6.69576659132887,-0.994746589046405,
96.2557101608948));
#32780=CARTESIAN_POINT('Ctrl Pts',(6.71919539828306,-0.821645696495592,
96.2639353535301));
#32781=CARTESIAN_POINT('Ctrl Pts',(6.73589376039568,-0.648092777820142,
96.2721605461653));
#32782=CARTESIAN_POINT('Ctrl Pts',(6.75091056167843,-0.492017009776847,
96.2795574442851));
#32783=CARTESIAN_POINT('Ctrl Pts',(6.76048489711358,-0.335575896286213,
96.2869543424049));
#32784=CARTESIAN_POINT('Ctrl Pts',(6.76462749297208,-0.179175560069701,
96.2943512405248));
#32785=CARTESIAN_POINT('Ctrl Pts',(6.76946962333506,0.0036351322212177,
96.3029972070157));
#32786=CARTESIAN_POINT('Ctrl Pts',(6.76690119693744,0.186805049357144,96.3116431735065));
#32787=CARTESIAN_POINT('Ctrl Pts',(6.75689235845708,0.369722404277046,96.3202891399974));
#32788=CARTESIAN_POINT('Ctrl Pts',(6.74689632264179,0.552405783033099,96.3289240471218));
#32789=CARTESIAN_POINT('Ctrl Pts',(6.72947886938024,0.734836940739044,96.3375589542462));
#32790=CARTESIAN_POINT('Ctrl Pts',(6.70466212033849,0.916403214801301,96.3461938613706));
#32791=CARTESIAN_POINT('Ctrl Pts',(6.67902147525857,1.10399734261729,96.3551154404421));
#32792=CARTESIAN_POINT('Ctrl Pts',(6.64548175244634,1.29066785329551,96.3640370195136));
#32793=CARTESIAN_POINT('Ctrl Pts',(6.60412588314898,1.4757406003501,96.3729585985851));
#32794=CARTESIAN_POINT('Ctrl Pts',(6.56420942591019,1.65437179634198,96.3815696575608));
#32795=CARTESIAN_POINT('Ctrl Pts',(6.51701177788901,1.831514230476,96.3901807165365));
#32796=CARTESIAN_POINT('Ctrl Pts',(6.46266000992232,2.00656786482563,96.3987917755122));
#32797=CARTESIAN_POINT('Ctrl Pts',(6.40835949818211,2.18145641551627,96.4073947138618));
#32798=CARTESIAN_POINT('Ctrl Pts',(6.34691840770841,2.35425980347348,96.4159976522113));
#32799=CARTESIAN_POINT('Ctrl Pts',(6.27851436634138,2.52439029304997,96.4246005905608));
#32800=CARTESIAN_POINT('Ctrl Pts',(6.21018692167635,2.69433027583548,96.4331938956096));
#32801=CARTESIAN_POINT('Ctrl Pts',(6.13491219422502,2.86160304890591,96.4417872006583));
#32802=CARTESIAN_POINT('Ctrl Pts',(6.05291701063844,3.02563789345715,96.4503805057071));
#32803=CARTESIAN_POINT('Ctrl Pts',(6.04378140506187,3.04391406011823,96.4513379405476));
#32804=CARTESIAN_POINT('Ctrl Pts',(6.03456242450087,3.06215005045793,96.4522953753882));
#32805=CARTESIAN_POINT('Ctrl Pts',(6.02526042023025,3.08034508917538,96.4532528102288));
#32806=CARTESIAN_POINT('Ctrl Pts',(5.94174792410106,3.24369838984614,96.4618485677764));
#32807=CARTESIAN_POINT('Ctrl Pts',(5.8516374843168,3.40355764061782,96.4704443253239));
#32808=CARTESIAN_POINT('Ctrl Pts',(5.755254406341,3.55940103364211,96.4790400828715));
#32809=CARTESIAN_POINT('Ctrl Pts',(5.65878139967662,3.71538983385044,96.4876438605531));
#32810=CARTESIAN_POINT('Ctrl Pts',(5.55602423343683,3.86735503764123,96.4962476382347));
#32811=CARTESIAN_POINT('Ctrl Pts',(5.44735096650021,4.01480465873114,96.5048514159163));
#32812=CARTESIAN_POINT('Ctrl Pts',(5.33440674514439,4.16804917886619,96.5137933295843));
#32813=CARTESIAN_POINT('Ctrl Pts',(5.21507223743087,4.31641571057879,96.5227352432523));
#32814=CARTESIAN_POINT('Ctrl Pts',(5.08980496090979,4.45939171411282,96.5316771569203));
#32815=CARTESIAN_POINT('Ctrl Pts',(4.96894647579248,4.59733566623781,96.540304359251));
#32816=CARTESIAN_POINT('Ctrl Pts',(4.84256595275606,4.73026188209838,96.5489315615817));
#32817=CARTESIAN_POINT('Ctrl Pts',(4.71111061934437,4.85774903965826,96.5575587639125));
#32818=CARTESIAN_POINT('Ctrl Pts',(4.57953009484883,4.98535760922188,96.5661941823329));
#32819=CARTESIAN_POINT('Ctrl Pts',(4.44286533809791,5.10751657560102,96.5748296007532));
#32820=CARTESIAN_POINT('Ctrl Pts',(4.30159692963566,5.22384464307172,96.5834650191737));
#32821=CARTESIAN_POINT('Ctrl Pts',(4.16011981722177,5.34034456869268,96.5921131951948));
#32822=CARTESIAN_POINT('Ctrl Pts',(4.01402570236079,5.4509961935557,96.6007613712159));
#32823=CARTESIAN_POINT('Ctrl Pts',(3.8638256196798,5.55546042922691,96.6094095472371));
#32824=CARTESIAN_POINT('Ctrl Pts',(3.84793502044534,5.5665123492642,96.6103244914688));
#32825=CARTESIAN_POINT('Ctrl Pts',(3.83199848768264,5.57749505656461,96.6112394357006));
#32826=CARTESIAN_POINT('Ctrl Pts',(3.81601664313435,5.58840817937645,96.6121543799324));
#32827=CARTESIAN_POINT('Ctrl Pts',(3.67232792393951,5.68652530437489,96.6203804119402));
#32828=CARTESIAN_POINT('Ctrl Pts',(3.52466401370678,5.77922588014726,96.628606443948));
#32829=CARTESIAN_POINT('Ctrl Pts',(3.37347074535601,5.86617286910531,96.6368324759558));
#32830=CARTESIAN_POINT('Ctrl Pts',(3.28326144601996,5.9180496956257,96.6417405290182));
#32831=CARTESIAN_POINT('Ctrl Pts',(3.19179639537182,5.96787904446892,96.6466485820806));
#32832=CARTESIAN_POINT('Ctrl Pts',(3.09917575053247,6.01559628526645,96.651556635143));
#32833=CARTESIAN_POINT('Origin',(0.,0.,-3.69717978381041));
#32834=CARTESIAN_POINT('',(3.09917575053247,6.01559628526645,99.0459901976524));
#32835=CARTESIAN_POINT('',(3.09917575053261,6.01559628526638,98.651480357023));
#32836=CARTESIAN_POINT('',(3.09917575053259,6.01559628526639,-3.69717978381041));
#32837=CARTESIAN_POINT('',(-6.767,5.7875637604881E-12,97.6971797838098));
#32838=CARTESIAN_POINT('Ctrl Pts',(-6.76699999999471,8.46578452749734E-6,
97.6973614935111));
#32839=CARTESIAN_POINT('Ctrl Pts',(-6.76700021337811,-0.170556414612781,
97.7054249703505));
#32840=CARTESIAN_POINT('Ctrl Pts',(-6.76054739979175,-0.341397623773265,
97.7134884471898));
#32841=CARTESIAN_POINT('Ctrl Pts',(-6.74760473158323,-0.511975962634623,
97.7215519240292));
#32842=CARTESIAN_POINT('Ctrl Pts',(-6.73467609075469,-0.682369427161041,
97.7296066616));
#32843=CARTESIAN_POINT('Ctrl Pts',(-6.71527162008903,-0.852500219493756,
97.7376613991708));
#32844=CARTESIAN_POINT('Ctrl Pts',(-6.68940644912142,-1.02182697089708,
97.7457161367415));
#32845=CARTESIAN_POINT('Ctrl Pts',(-6.66356363433439,-1.19100736721027,
97.7537639123182));
#32846=CARTESIAN_POINT('Ctrl Pts',(-6.63127128930906,-1.35938473877313,
97.7618116878949));
#32847=CARTESIAN_POINT('Ctrl Pts',(-6.5925964979879,-1.52642078560198,97.7698594634716));
#32848=CARTESIAN_POINT('Ctrl Pts',(-6.55394665663113,-1.6933490737777,97.77790204725));
#32849=CARTESIAN_POINT('Ctrl Pts',(-6.508922649235,-1.85893739707862,97.7859446310284));
#32850=CARTESIAN_POINT('Ctrl Pts',(-6.45764297323504,-2.02265573695282,
97.7939872148069));
#32851=CARTESIAN_POINT('Ctrl Pts',(-6.40523311497251,-2.1899823594492,97.8022070537133));
#32852=CARTESIAN_POINT('Ctrl Pts',(-6.34628870140792,-2.35535522032763,
97.8104268926197));
#32853=CARTESIAN_POINT('Ctrl Pts',(-6.28099080763204,-2.51822228455747,
97.8186467315261));
#32854=CARTESIAN_POINT('Ctrl Pts',(-6.21713029979191,-2.67750419750625,
97.8266856292082));
#32855=CARTESIAN_POINT('Ctrl Pts',(-6.14719326565084,-2.83438912434916,
97.8347245268905));
#32856=CARTESIAN_POINT('Ctrl Pts',(-6.07139848128779,-2.98837907257703,
97.8427634245726));
#32857=CARTESIAN_POINT('Ctrl Pts',(-5.995599517674,-3.14237751166096,97.8508027655118));
#32858=CARTESIAN_POINT('Ctrl Pts',(-5.91394232559818,-3.29348031874414,
97.858842106451));
#32859=CARTESIAN_POINT('Ctrl Pts',(-5.82669233804939,-3.44121278006992,
97.8668814473902));
#32860=CARTESIAN_POINT('Ctrl Pts',(-5.73942023282579,-3.58898269124103,
97.8749228262842));
#32861=CARTESIAN_POINT('Ctrl Pts',(-5.64655270034893,-3.73338023438517,
97.8829642051781));
#32862=CARTESIAN_POINT('Ctrl Pts',(-5.54839922872049,-3.87395856956858,
97.8910055840721));
#32863=CARTESIAN_POINT('Ctrl Pts',(-5.4464199561355,-4.02001633120827,97.8993603977794));
#32864=CARTESIAN_POINT('Ctrl Pts',(-5.33873463199313,-4.16195079374431,
97.9077152114868));
#32865=CARTESIAN_POINT('Ctrl Pts',(-5.2257366285637,-4.29929827865987,97.9160700251941));
#32866=CARTESIAN_POINT('Ctrl Pts',(-5.11679902718726,-4.43171040195134,
97.9241246220684));
#32867=CARTESIAN_POINT('Ctrl Pts',(-5.0029242146891,-4.55985924051399,97.9321792189428));
#32868=CARTESIAN_POINT('Ctrl Pts',(-4.88450213959166,-4.68336714857212,
97.9402338158171));
#32869=CARTESIAN_POINT('Ctrl Pts',(-4.76599545906791,-4.8069632955773,97.9482941672148));
#32870=CARTESIAN_POINT('Ctrl Pts',(-4.64293531433775,-4.92591165192842,
97.9563545186125));
#32871=CARTESIAN_POINT('Ctrl Pts',(-4.51574499210935,-5.03987461810702,
97.9644148700102));
#32872=CARTESIAN_POINT('Ctrl Pts',(-4.38838244307443,-5.15399190009662,
97.9724861358278));
#32873=CARTESIAN_POINT('Ctrl Pts',(-4.25687884341894,-5.2631100865309,97.9805574016454));
#32874=CARTESIAN_POINT('Ctrl Pts',(-4.12168714011927,-5.36693433153187,
97.988628667463));
#32875=CARTESIAN_POINT('Ctrl Pts',(-4.10697705485094,-5.37823135242596,
97.9895068944954));
#32876=CARTESIAN_POINT('Ctrl Pts',(-4.09222332896915,-5.38946574072866,
97.9903851215279));
#32877=CARTESIAN_POINT('Ctrl Pts',(-4.07742656333619,-5.40063714950379,
97.9912633485603));
#32878=CARTESIAN_POINT('Ctrl Pts',(-3.93873395085177,-5.50534867272368,
97.9994951205912));
#32879=CARTESIAN_POINT('Ctrl Pts',(-3.79580153277411,-5.60486788247453,
98.007726892622));
#32880=CARTESIAN_POINT('Ctrl Pts',(-3.64905391587604,-5.69883273302786,
98.0159586646529));
#32881=CARTESIAN_POINT('Ctrl Pts',(-3.5024815302977,-5.79268538015929,98.0241806071252));
#32882=CARTESIAN_POINT('Ctrl Pts',(-3.35210331618632,-5.88099668353843,
98.0324025495976));
#32883=CARTESIAN_POINT('Ctrl Pts',(-3.1983765797827,-5.9634449988155,98.04062449207));
#32884=CARTESIAN_POINT('Ctrl Pts',(-3.04480260796148,-6.04581138180968,
98.0488382640599));
#32885=CARTESIAN_POINT('Ctrl Pts',(-2.88788705426437,-6.12232621155359,
98.0570520360498));
#32886=CARTESIAN_POINT('Ctrl Pts',(-2.72811589115529,-6.19271125472729,
98.0652658080397));
#32887=CARTESIAN_POINT('Ctrl Pts',(-2.56847149929502,-6.26304045052749,
98.0734730627701));
#32888=CARTESIAN_POINT('Ctrl Pts',(-2.40597633742626,-6.32724940341208,
98.0816803175005));
#32889=CARTESIAN_POINT('Ctrl Pts',(-2.24114073350772,-6.38510588891152,
98.0898875722309));
#32890=CARTESIAN_POINT('Ctrl Pts',(-2.07640291358334,-6.44292805271039,
98.0980899582428));
#32891=CARTESIAN_POINT('Ctrl Pts',(-1.90932775465298,-6.49440513791089,
98.1062923442547));
#32892=CARTESIAN_POINT('Ctrl Pts',(-1.74044539424744,-6.53935308953744,
98.1144947302666));
#32893=CARTESIAN_POINT('Ctrl Pts',(-1.5716134411293,-6.5842876252909,98.1226946680653));
#32894=CARTESIAN_POINT('Ctrl Pts',(-1.40097570583604,-6.62269681358711,
98.130894605864));
#32895=CARTESIAN_POINT('Ctrl Pts',(-1.22907755420387,-6.65444643571141,
98.1390945436627));
#32896=CARTESIAN_POINT('Ctrl Pts',(-1.05720343836997,-6.68619161841908,
98.1472933348984));
#32897=CARTESIAN_POINT('Ctrl Pts',(-0.884069609390594,-6.71127902364263,
98.1554921261342));
#32898=CARTESIAN_POINT('Ctrl Pts',(-0.710231717166204,-6.7296255399488,
98.1636909173699));
#32899=CARTESIAN_POINT('Ctrl Pts',(-0.536386596869409,-6.74797281909181,
98.1718900495063));
#32900=CARTESIAN_POINT('Ctrl Pts',(-0.361837711464924,-6.7595786132292,
98.1800891816428));
#32901=CARTESIAN_POINT('Ctrl Pts',(-0.187145984910275,-6.76441168028174,
98.1882883137792));
#32902=CARTESIAN_POINT('Ctrl Pts',(-0.0124153049127425,-6.76924582503042,
98.1964892741901));
#32903=CARTESIAN_POINT('Ctrl Pts',(0.162457921454999,-6.76730422488259,
98.204690234601));
#32904=CARTESIAN_POINT('Ctrl Pts',(0.336912557256312,-6.75860776556556,
98.2128911950119));
#32905=CARTESIAN_POINT('Ctrl Pts',(0.511530699047683,-6.74990315557265,
98.2210998416969));
#32906=CARTESIAN_POINT('Ctrl Pts',(0.68572910798653,-6.73443105547005,98.229308488382));
#32907=CARTESIAN_POINT('Ctrl Pts',(0.8589506080348,-6.71226436107493,98.237517135067));
#32908=CARTESIAN_POINT('Ctrl Pts',(1.03225480889225,-6.69008708367735,98.2457297007905));
#32909=CARTESIAN_POINT('Ctrl Pts',(1.20458081761655,-6.66120889854043,98.253942266514));
#32910=CARTESIAN_POINT('Ctrl Pts',(1.37538151702226,-6.625753895417,98.2621548322375));
#32911=CARTESIAN_POINT('Ctrl Pts',(1.54641657963445,-6.59025024291306,98.2703786667863));
#32912=CARTESIAN_POINT('Ctrl Pts',(1.71592180208878,-6.54815182324261,98.278602501335));
#32913=CARTESIAN_POINT('Ctrl Pts',(1.88336390244769,-6.49963302125258,98.2868263358838));
#32914=CARTESIAN_POINT('Ctrl Pts',(2.03721169533878,-6.45505336903916,98.2943824928582));
#32915=CARTESIAN_POINT('Ctrl Pts',(2.18931775827407,-6.40505417374424,98.3019386498325));
#32916=CARTESIAN_POINT('Ctrl Pts',(2.33928402396668,-6.34980623761184,98.3094948068069));
#32917=CARTESIAN_POINT('Ctrl Pts',(2.51087469564636,-6.28659181784823,98.3181405248593));
#32918=CARTESIAN_POINT('Ctrl Pts',(2.68005497109013,-6.21636147434551,98.3267862429117));
#32919=CARTESIAN_POINT('Ctrl Pts',(2.84624552993176,-6.13931391796701,98.3354319609641));
#32920=CARTESIAN_POINT('Ctrl Pts',(3.0122227339653,-6.06236527494869,98.3440665796765));
#32921=CARTESIAN_POINT('Ctrl Pts',(3.1752175995722,-5.97861699848319,98.3527011983889));
#32922=CARTESIAN_POINT('Ctrl Pts',(3.33466923044143,-5.8883164082399,98.3613358171013));
#32923=CARTESIAN_POINT('Ctrl Pts',(3.49975207349135,-5.79482675193983,98.3702753770037));
#32924=CARTESIAN_POINT('Ctrl Pts',(3.66103653636448,-5.69431361453289,98.3792149369062));
#32925=CARTESIAN_POINT('Ctrl Pts',(3.81792347095631,-5.58710563439791,98.3881544968086));
#32926=CARTESIAN_POINT('Ctrl Pts',(3.96903818031422,-5.48384207837845,98.3967651500791));
#32927=CARTESIAN_POINT('Ctrl Pts',(4.11607286612411,-5.3743676871414,98.4053758033496));
#32928=CARTESIAN_POINT('Ctrl Pts',(4.25851726878939,-5.25902269166264,98.4139864566201));
#32929=CARTESIAN_POINT('Ctrl Pts',(4.40082683829702,-5.1437868779395,98.4225889593312));
#32930=CARTESIAN_POINT('Ctrl Pts',(4.53855455119751,-5.02269173027942,98.4311914620423));
#32931=CARTESIAN_POINT('Ctrl Pts',(4.67122029642491,-4.89611988642721,98.4397939647534));
#32932=CARTESIAN_POINT('Ctrl Pts',(4.80373672902785,-4.76969049663619,98.4483867855209));
#32933=CARTESIAN_POINT('Ctrl Pts',(4.93120233938645,-4.63779691755874,98.4569796062884));
#32934=CARTESIAN_POINT('Ctrl Pts',(5.0531710449642,-4.50086118318877,98.4655724270559));
#32935=CARTESIAN_POINT('Ctrl Pts',(5.06754561092885,-4.48472268489698,98.4665851300141));
#32936=CARTESIAN_POINT('Ctrl Pts',(5.08184386603344,-4.46851419716626,98.4675978329723));
#32937=CARTESIAN_POINT('Ctrl Pts',(5.09606511214929,-4.45223644618464,98.4686105359305));
#32938=CARTESIAN_POINT('Ctrl Pts',(5.21676711568027,-4.31407997660005,98.4772057936906));
#32939=CARTESIAN_POINT('Ctrl Pts',(5.33177651931316,-4.17109364975173,98.4858010514507));
#32940=CARTESIAN_POINT('Ctrl Pts',(5.44072957655019,-4.02377318879332,98.4943963092107));
#32941=CARTESIAN_POINT('Ctrl Pts',(5.54978466370526,-3.87631476847024,98.5029996160652));
#32942=CARTESIAN_POINT('Ctrl Pts',(5.65277190234388,-3.72451435815284,98.5116029229197));
#32943=CARTESIAN_POINT('Ctrl Pts',(5.7493711082545,-3.56889630832397,98.5202062297742));
#32944=CARTESIAN_POINT('Ctrl Pts',(5.84997535073926,-3.40682628018653,98.5291662327142));
#32945=CARTESIAN_POINT('Ctrl Pts',(5.94365038361258,-3.2406156366243,98.5381262356541));
#32946=CARTESIAN_POINT('Ctrl Pts',(6.03008829914884,-3.0708832775715,98.5470862385941));
#32947=CARTESIAN_POINT('Ctrl Pts',(6.11331219419341,-2.90746207580094,98.5557130817989));
#32948=CARTESIAN_POINT('Ctrl Pts',(6.18982738122912,-2.74077662017317,98.5643399250036));
#32949=CARTESIAN_POINT('Ctrl Pts',(6.25940878415947,-2.57139858302585,98.5729667682084));
#32950=CARTESIAN_POINT('Ctrl Pts',(6.32905668932188,-2.40185866329124,98.5816018564945));
#32951=CARTESIAN_POINT('Ctrl Pts',(6.39175747526719,-2.22962131062627,98.5902369447806));
#32952=CARTESIAN_POINT('Ctrl Pts',(6.4473356177723,-2.05527429600155,98.5988720330667));
#32953=CARTESIAN_POINT('Ctrl Pts',(6.50299630497266,-1.8806683410715,98.6075199461918));
#32954=CARTESIAN_POINT('Ctrl Pts',(6.55151312418768,-1.70394675572282,98.616167859317));
#32955=CARTESIAN_POINT('Ctrl Pts',(6.59276104946669,-1.52570991496907,98.6248157724421));
#32956=CARTESIAN_POINT('Ctrl Pts',(6.59738843875867,-1.50571445476685,98.6257859366461));
#32957=CARTESIAN_POINT('Ctrl Pts',(6.60192439938738,-1.48569993195239,98.62675610085));
#32958=CARTESIAN_POINT('Ctrl Pts',(6.60636879538482,-1.46566719938933,98.627726265054));
#32959=CARTESIAN_POINT('Ctrl Pts',(6.64404667773131,-1.29583738651382,98.6359509445728));
#32960=CARTESIAN_POINT('Ctrl Pts',(6.67522128892439,-1.12432995693657,98.6441756240916));
#32961=CARTESIAN_POINT('Ctrl Pts',(6.69974528392764,-0.95168383956509,98.6524003036103));
#32962=CARTESIAN_POINT('Ctrl Pts',(6.72424350143763,-0.779219192795254,
98.6606163380605));
#32963=CARTESIAN_POINT('Ctrl Pts',(6.74210497342658,-0.60561859359595,98.6688323725106));
#32964=CARTESIAN_POINT('Ctrl Pts',(6.75323287948293,-0.431433280439463,
98.6770484069607));
#32965=CARTESIAN_POINT('Ctrl Pts',(6.76435131779029,-0.257396166127547,
98.6852574511153));
#32966=CARTESIAN_POINT('Ctrl Pts',(6.76874757741193,-0.0827756843283776,
98.6934664952699));
#32967=CARTESIAN_POINT('Ctrl Pts',(6.76637635560913,0.0918695501989991,
98.7016755394246));
#32968=CARTESIAN_POINT('Ctrl Pts',(6.76400667644305,0.266401166441519,98.7098792430526));
#32969=CARTESIAN_POINT('Ctrl Pts',(6.75487829047703,0.440957146231089,98.7180829466806));
#32970=CARTESIAN_POINT('Ctrl Pts',(6.73899791488554,0.614976506192181,98.7262866503086));
#32971=CARTESIAN_POINT('Ctrl Pts',(6.72312469120729,0.788917494495235,98.7344866593026));
#32972=CARTESIAN_POINT('Ctrl Pts',(6.700505568594,0.962321988254316,98.7426866682966));
#32973=CARTESIAN_POINT('Ctrl Pts',(6.67119929074061,1.13463166852598,98.7508866772905));
#32974=CARTESIAN_POINT('Ctrl Pts',(6.64189535627904,1.30692757055193,98.7590860305945));
#32975=CARTESIAN_POINT('Ctrl Pts',(6.60590538309038,1.47812847892829,98.7672853838984));
#32976=CARTESIAN_POINT('Ctrl Pts',(6.56333971309382,1.64768346794082,98.7754847372023));
#32977=CARTESIAN_POINT('Ctrl Pts',(6.52077432061295,1.81723735150458,98.7836840370488));
#32978=CARTESIAN_POINT('Ctrl Pts',(6.47163340295877,1.98514498908865,98.7918833368954));
#32979=CARTESIAN_POINT('Ctrl Pts',(6.41607791618785,2.15086800464523,98.800082636742));
#32980=CARTESIAN_POINT('Ctrl Pts',(6.36051271331179,2.31662000351808,98.808283370565));
#32981=CARTESIAN_POINT('Ctrl Pts',(6.29853082018612,2.48018627922513,98.816484104388));
#32982=CARTESIAN_POINT('Ctrl Pts',(6.23034234743438,2.6410458598377,98.824684838211));
#32983=CARTESIAN_POINT('Ctrl Pts',(6.16212957900082,2.80196275502311,98.832888493971));
#32984=CARTESIAN_POINT('Ctrl Pts',(6.08770596552259,2.96017070410215,98.841092149731));
#32985=CARTESIAN_POINT('Ctrl Pts',(6.00732883561685,3.11517082368949,98.849295805491));
#32986=CARTESIAN_POINT('Ctrl Pts',(5.92685962854182,3.2703485058779,98.857508859066));
#32987=CARTESIAN_POINT('Ctrl Pts',(5.84042344468821,3.42231069834952,98.865721912641));
#32988=CARTESIAN_POINT('Ctrl Pts',(5.74832300072423,3.5705842210127,98.873934966216));
#32989=CARTESIAN_POINT('Ctrl Pts',(5.65616805886127,3.71894548044576,98.8821528796391));
#32990=CARTESIAN_POINT('Ctrl Pts',(5.55834237625173,3.86361342269772,98.8903707930621));
#32991=CARTESIAN_POINT('Ctrl Pts',(5.4551906321931,4.00414587227197,98.8985887064852));
#32992=CARTESIAN_POINT('Ctrl Pts',(5.35187800620843,4.14489750506377,98.9068194370812));
#32993=CARTESIAN_POINT('Ctrl Pts',(5.24322294116174,4.28150047496693,98.9150501676772));
#32994=CARTESIAN_POINT('Ctrl Pts',(5.12960972230994,4.41354654408258,98.9232808982731));
#32995=CARTESIAN_POINT('Ctrl Pts',(5.02526956867612,4.53481506615697,98.930839839949));
#32996=CARTESIAN_POINT('Ctrl Pts',(4.91674818224055,4.6522404656876,98.9383987816248));
#32997=CARTESIAN_POINT('Ctrl Pts',(4.80436851752053,4.76553587205654,98.9459577233007));
#32998=CARTESIAN_POINT('Ctrl Pts',(4.68043564866504,4.89047862548467,98.95429376283));
#32999=CARTESIAN_POINT('Ctrl Pts',(4.55141798359906,5.01079282400249,98.9626298023593));
#33000=CARTESIAN_POINT('Ctrl Pts',(4.41769880299643,5.12603416746357,98.9709658418886));
#33001=CARTESIAN_POINT('Ctrl Pts',(4.28706592412992,5.23861568638195,98.9791094816952));
#33002=CARTESIAN_POINT('Ctrl Pts',(4.15194643805172,5.3463556469886,98.9872531215018));
#33003=CARTESIAN_POINT('Ctrl Pts',(4.01273794638276,5.44887356924896,98.9953967613083));
#33004=CARTESIAN_POINT('Ctrl Pts',(3.86859609398656,5.55502458806437,99.003829000699));
#33005=CARTESIAN_POINT('Ctrl Pts',(3.7200703367406,5.6555763442914,99.0122612400897));
#33006=CARTESIAN_POINT('Ctrl Pts',(3.56764291884306,5.75014895490795,99.0206934794804));
#33007=CARTESIAN_POINT('Ctrl Pts',(3.41521550094564,5.84472156552443,99.0291257188711));
#33008=CARTESIAN_POINT('Ctrl Pts',(3.25888676068621,5.93331475135205,99.0375579582617));
#33009=CARTESIAN_POINT('Ctrl Pts',(3.09917575053247,6.01559628526645,99.0459901976524));
#33010=CARTESIAN_POINT('Ctrl Pts',(3.09917575053274,6.01559628526631,97.0457515827422));
#33011=CARTESIAN_POINT('Ctrl Pts',(2.93382384459274,6.10078395293755,97.0545010306546));
#33012=CARTESIAN_POINT('Ctrl Pts',(2.76495772122987,6.17915010267048,97.063250478567));
#33013=CARTESIAN_POINT('Ctrl Pts',(2.59315093316709,6.25042856433178,97.0719999264794));
#33014=CARTESIAN_POINT('Ctrl Pts',(2.42134553245619,6.3217064504145,97.0807493037395));
#33015=CARTESIAN_POINT('Ctrl Pts',(2.24659977927597,6.38589665313455,97.0894986809995));
#33016=CARTESIAN_POINT('Ctrl Pts',(2.0695071868993,6.44278115439072,97.0982480582595));
#33017=CARTESIAN_POINT('Ctrl Pts',(1.89241596572865,6.49966521519723,97.1069973677741));
#33018=CARTESIAN_POINT('Ctrl Pts',(1.71297821457194,6.54924360009547,97.1157466772888));
#33019=CARTESIAN_POINT('Ctrl Pts',(1.53180337335832,6.59134792173559,97.1244959868035));
#33020=CARTESIAN_POINT('Ctrl Pts',(1.35062987477769,6.63345193135307,97.1332452314796));
#33021=CARTESIAN_POINT('Ctrl Pts',(1.16771959102938,6.6680819236824,97.1419944761557));
#33022=CARTESIAN_POINT('Ctrl Pts',(0.983693746906691,6.69512028363171,97.1507437208318));
#33023=CARTESIAN_POINT('Ctrl Pts',(0.799669205419827,6.72215845218867,97.159492903576));
#33024=CARTESIAN_POINT('Ctrl Pts',(0.614529402873543,6.74160505424578,97.1682420863202));
#33025=CARTESIAN_POINT('Ctrl Pts',(0.428903127363426,6.75339404354121,97.1769912690643));
#33026=CARTESIAN_POINT('Ctrl Pts',(0.243278104164192,6.76518295330329,97.1857403927829));
#33027=CARTESIAN_POINT('Ctrl Pts',(0.0571669005395649,6.76931433552275,
97.1944895165015));
#33028=CARTESIAN_POINT('Ctrl Pts',(-0.128798404776931,6.76577415902474,
97.2032386402201));
#33029=CARTESIAN_POINT('Ctrl Pts',(-0.314762517258624,6.76223400523444,
97.2119877078193));
#33030=CARTESIAN_POINT('Ctrl Pts',(-0.500580446819143,6.75102239665092,
97.2207367754186));
#33031=CARTESIAN_POINT('Ctrl Pts',(-0.685621118842352,6.732177410125,97.2294858430178));
#33032=CARTESIAN_POINT('Ctrl Pts',(-0.870660665414071,6.71333253821777,
97.2382348574035));
#33033=CARTESIAN_POINT('Ctrl Pts',(-1.05492267885429,6.68685441030621,97.2469838717893));
#33034=CARTESIAN_POINT('Ctrl Pts',(-1.23778137635179,6.65283295028191,97.2557328861751));
#33035=CARTESIAN_POINT('Ctrl Pts',(-1.42999922978773,6.61707018861881,97.2649296965425));
#33036=CARTESIAN_POINT('Ctrl Pts',(-1.62066601233621,6.57297172934431,97.2741265069099));
#33037=CARTESIAN_POINT('Ctrl Pts',(-1.80906628500311,6.52070304311315,97.2833233172773));
#33038=CARTESIAN_POINT('Ctrl Pts',(-1.98831342545455,6.47097374915053,97.292073315015));
#33039=CARTESIAN_POINT('Ctrl Pts',(-2.16550875896632,6.41384933989552,97.3008233127528));
#33040=CARTESIAN_POINT('Ctrl Pts',(-2.34005036713943,6.34952386240501,97.3095733104905));
#33041=CARTESIAN_POINT('Ctrl Pts',(-2.51458843547022,6.28519968948623,97.3183231307714));
#33042=CARTESIAN_POINT('Ctrl Pts',(-2.68647261717989,6.21367483971128,97.3270729510523));
#33043=CARTESIAN_POINT('Ctrl Pts',(-2.85511905908666,6.13519226743874,97.3358227713331));
#33044=CARTESIAN_POINT('Ctrl Pts',(-3.02376230488815,6.05671118252972,97.3445724257917));
#33045=CARTESIAN_POINT('Ctrl Pts',(-3.18916767379831,5.97127275992672,97.3533220802502));
#33046=CARTESIAN_POINT('Ctrl Pts',(-3.3507733410271,5.87916720438041,97.3620717347087));
#33047=CARTESIAN_POINT('Ctrl Pts',(-3.5123761603729,5.7870632719569,97.3708212349772));
#33048=CARTESIAN_POINT('Ctrl Pts',(-3.67017916302221,5.68829258362349,97.3795707352456));
#33049=CARTESIAN_POINT('Ctrl Pts',(-3.82364636566383,5.58319061741096,97.3883202355141));
#33050=CARTESIAN_POINT('Ctrl Pts',(-3.97711106778727,5.47809036367754,97.3970695932225));
#33051=CARTESIAN_POINT('Ctrl Pts',(-4.12623987481864,5.36665920043274,97.4058189509309));
#33052=CARTESIAN_POINT('Ctrl Pts',(-4.27052628213874,5.2492755951238,97.4145683086394));
#33053=CARTESIAN_POINT('Ctrl Pts',(-4.41481053024941,5.13189374643069,97.4233175354159));
#33054=CARTESIAN_POINT('Ctrl Pts',(-4.5542523013651,5.00855981477372,97.4320667621924));
#33055=CARTESIAN_POINT('Ctrl Pts',(-4.68837800630544,4.87969268192081,97.440815988969));
#33056=CARTESIAN_POINT('Ctrl Pts',(-4.82250188228888,4.75082730631816,97.4495650964398));
#33057=CARTESIAN_POINT('Ctrl Pts',(-4.95130963052957,4.61642907903535,97.4583142039106));
#33058=CARTESIAN_POINT('Ctrl Pts',(-5.07436379033356,4.47695444731702,97.4670633113815));
#33059=CARTESIAN_POINT('Ctrl Pts',(-5.19741643562794,4.33748153220599,97.4758123111712));
#33060=CARTESIAN_POINT('Ctrl Pts',(-5.31471544462761,4.19293255254604,97.484561310961));
#33061=CARTESIAN_POINT('Ctrl Pts',(-5.42586245275616,4.04379841779619,97.4933103107507));
#33062=CARTESIAN_POINT('Ctrl Pts',(-5.53702160019136,3.89464799484367,97.5020602660929));
#33063=CARTESIAN_POINT('Ctrl Pts',(-5.64202723081229,3.74091164443883,97.510810221435));
#33064=CARTESIAN_POINT('Ctrl Pts',(-5.74052265232941,3.58311159163275,97.5195601767772));
#33065=CARTESIAN_POINT('Ctrl Pts',(-5.83901427066893,3.42531763191826,97.5283097942596));
#33066=CARTESIAN_POINT('Ctrl Pts',(-5.93099603115716,3.26346052695656,97.5370594117421));
#33067=CARTESIAN_POINT('Ctrl Pts',(-6.01615550622731,3.09809004467121,97.5458090292245));
#33068=CARTESIAN_POINT('Ctrl Pts',(-6.10131214578774,2.9327250686388,97.5545583553756));
#33069=CARTESIAN_POINT('Ctrl Pts',(-6.1796468232872,2.76384720416954,97.5633076815267));
#33070=CARTESIAN_POINT('Ctrl Pts',(-6.25089348288535,2.59203002791662,97.5720570076778));
#33071=CARTESIAN_POINT('Ctrl Pts',(-6.32213814889309,2.42021765937085,97.5808060890094));
#33072=CARTESIAN_POINT('Ctrl Pts',(-6.3862950841257,2.24546640831962,97.5895551703409));
#33073=CARTESIAN_POINT('Ctrl Pts',(-6.44314639819802,2.06836976660073,97.5983042516725));
#33074=CARTESIAN_POINT('Ctrl Pts',(-6.5000028528369,1.8912571115831,97.6070541241069));
#33075=CARTESIAN_POINT('Ctrl Pts',(-6.5495522767324,1.71179891440292,97.6158039965413));
#33076=CARTESIAN_POINT('Ctrl Pts',(-6.59162635926376,1.53060476278471,97.6245538689757));
#33077=CARTESIAN_POINT('Ctrl Pts',(-6.63369752055186,1.34942319164746,97.6333031338982));
#33078=CARTESIAN_POINT('Ctrl Pts',(-6.66829431424243,1.16650618642765,97.6420523988207));
#33079=CARTESIAN_POINT('Ctrl Pts',(-6.69529923745407,0.982474997619267,
97.6508016637432));
#33080=CARTESIAN_POINT('Ctrl Pts',(-6.72230554731435,0.798434359178469,
97.6595513779229));
#33081=CARTESIAN_POINT('Ctrl Pts',(-6.74171916496696,0.613279706241085,
97.6683010921026));
#33082=CARTESIAN_POINT('Ctrl Pts',(-6.7534741481727,0.427639953656142,97.6770508062823));
#33083=CARTESIAN_POINT('Ctrl Pts',(-6.76248837758734,0.285283364200488,
97.6837604654581));
#33084=CARTESIAN_POINT('Ctrl Pts',(-6.76699999999988,0.142641701108184,
97.690470124634));
#33085=CARTESIAN_POINT('Ctrl Pts',(-6.767,5.78756373465266E-12,97.6971797838098));
#33086=CARTESIAN_POINT('',(-6.76699828620706,0.00481606382174074,97.3028202162221));
#33087=CARTESIAN_POINT('Ctrl Pts',(3.09917575053247,6.01559628526645,96.651556635143));
#33088=CARTESIAN_POINT('Ctrl Pts',(2.94418678798982,6.09544506692237,96.6597696426594));
#33089=CARTESIAN_POINT('Ctrl Pts',(2.7859605775845,6.16937712803934,96.6679826501758));
#33090=CARTESIAN_POINT('Ctrl Pts',(2.62498916978028,6.23712440620966,96.6761956576923));
#33091=CARTESIAN_POINT('Ctrl Pts',(2.46413507988091,6.30482230934598,96.6844026794697));
#33092=CARTESIAN_POINT('Ctrl Pts',(2.30054010645421,6.36634426930046,96.6926097012472));
#33093=CARTESIAN_POINT('Ctrl Pts',(2.13471964029275,6.42146876168906,96.7008167230246));
#33094=CARTESIAN_POINT('Ctrl Pts',(1.96898685975561,6.47656410432527,96.7090194049407));
#33095=CARTESIAN_POINT('Ctrl Pts',(1.80103127000067,6.52526860599149,96.7172220868568));
#33096=CARTESIAN_POINT('Ctrl Pts',(1.63138701126607,6.56740933850422,96.7254247687729));
#33097=CARTESIAN_POINT('Ctrl Pts',(1.45513466268568,6.61119156332967,96.7339469667132));
#33098=CARTESIAN_POINT('Ctrl Pts',(1.27705981573491,6.64788823092621,96.7424691646535));
#33099=CARTESIAN_POINT('Ctrl Pts',(1.09777802498692,6.67736268356421,96.7509913625938));
#33100=CARTESIAN_POINT('Ctrl Pts',(0.92526260422526,6.70572472511539,96.759191919702));
#33101=CARTESIAN_POINT('Ctrl Pts',(0.751630058849052,6.72739969300063,96.7673924768102));
#33102=CARTESIAN_POINT('Ctrl Pts',(0.577438170068366,6.74231815919036,96.7755930339184));
#33103=CARTESIAN_POINT('Ctrl Pts',(0.403227077395019,6.75723827007563,96.7837944951021));
#33104=CARTESIAN_POINT('Ctrl Pts',(0.228456875528297,6.76540036430465,96.7919959562857));
#33105=CARTESIAN_POINT('Ctrl Pts',(0.0536892855156084,6.76678701161939,
96.8001974174694));
#33106=CARTESIAN_POINT('Ctrl Pts',(-0.121129244273583,6.76817406310234,
96.8084012691455));
#33107=CARTESIAN_POINT('Ctrl Pts',(-0.295944802446117,6.76278173074403,
96.8166051208216));
#33108=CARTESIAN_POINT('Ctrl Pts',(-0.470196793716727,6.75064470811333,
96.8248089724977));
#33109=CARTESIAN_POINT('Ctrl Pts',(-0.644531154044458,6.73850194830222,
96.8330167021411));
#33110=CARTESIAN_POINT('Ctrl Pts',(-0.818301059778924,6.71960817195363,
96.8412244317846));
#33111=CARTESIAN_POINT('Ctrl Pts',(-0.990952093649598,6.69404981667238,
96.849432161428));
#33112=CARTESIAN_POINT('Ctrl Pts',(-1.16380661045559,6.66846133884255,96.8576495645317));
#33113=CARTESIAN_POINT('Ctrl Pts',(-1.33553926760618,6.63619264851488,96.8658669676354));
#33114=CARTESIAN_POINT('Ctrl Pts',(-1.5056059627311,6.59738127479294,96.8740843707391));
#33115=CARTESIAN_POINT('Ctrl Pts',(-1.67579101629611,6.55854289017598,96.8823074927698));
#33116=CARTESIAN_POINT('Ctrl Pts',(-1.84430745232475,6.51315283974987,96.8905306148005));
#33117=CARTESIAN_POINT('Ctrl Pts',(-2.01062746299856,6.46139816177861,96.8987537368312));
#33118=CARTESIAN_POINT('Ctrl Pts',(-2.17717562068841,6.40957249009289,96.906988138808));
#33119=CARTESIAN_POINT('Ctrl Pts',(-2.34152100074633,6.35136487683304,96.9152225407848));
#33120=CARTESIAN_POINT('Ctrl Pts',(-2.50315604394867,6.28701032444223,96.9234569427616));
#33121=CARTESIAN_POINT('Ctrl Pts',(-2.54568983406041,6.27007561170981,96.9256238016211));
#33122=CARTESIAN_POINT('Ctrl Pts',(-2.58803607787279,6.25271549130404,96.9277906604806));
#33123=CARTESIAN_POINT('Ctrl Pts',(-2.63018582661199,6.23493476449349,96.9299575193402));
#33124=CARTESIAN_POINT('Ctrl Pts',(-2.78882584194334,6.16801301861826,96.938112977747));
#33125=CARTESIAN_POINT('Ctrl Pts',(-2.94516883681524,6.09492357467407,96.9462684361538));
#33126=CARTESIAN_POINT('Ctrl Pts',(-3.09869496624633,6.01584395626745,96.9544238945606));
#33127=CARTESIAN_POINT('Ctrl Pts',(-3.25203423419721,5.93686058815129,96.9625694267025));
#33128=CARTESIAN_POINT('Ctrl Pts',(-3.40256313992362,5.85190172383188,96.9707149588443));
#33129=CARTESIAN_POINT('Ctrl Pts',(-3.54977982079,5.76119364575711,96.9788604909862));
#33130=CARTESIAN_POINT('Ctrl Pts',(-3.69684827631917,5.6705768972476,96.9869978217868));
#33131=CARTESIAN_POINT('Ctrl Pts',(-3.840610837371,5.57422264936697,96.9951351525874));
#33132=CARTESIAN_POINT('Ctrl Pts',(-3.98058836081621,5.47240397830191,97.0032724833879));
#33133=CARTESIAN_POINT('Ctrl Pts',(-4.12045436439032,5.37066642601072,97.01140333119));
#33134=CARTESIAN_POINT('Ctrl Pts',(-4.25654104045743,5.2634733328904,97.0195341789919));
#33135=CARTESIAN_POINT('Ctrl Pts',(-4.38839648230385,5.15114213685695,97.027665026794));
#33136=CARTESIAN_POINT('Ctrl Pts',(-4.52017457364671,5.03887683779716,97.0357911047877));
#33137=CARTESIAN_POINT('Ctrl Pts',(-4.64772609644033,4.92147967492004,97.0439171827815));
#33138=CARTESIAN_POINT('Ctrl Pts',(-4.77063063078348,4.79930957374396,97.0520432607753));
#33139=CARTESIAN_POINT('Ctrl Pts',(-4.89397096215797,4.67670627970242,97.0601981523575));
#33140=CARTESIAN_POINT('Ctrl Pts',(-5.01263099277457,4.5492963609996,97.0683530439397));
#33141=CARTESIAN_POINT('Ctrl Pts',(-5.12622125432085,4.41748170927161,97.0765079355219));
#33142=CARTESIAN_POINT('Ctrl Pts',(-5.23936855356286,4.28618108859761,97.0846310258782));
#33143=CARTESIAN_POINT('Ctrl Pts',(-5.34748532593959,4.15051031727124,97.0927541162345));
#33144=CARTESIAN_POINT('Ctrl Pts',(-5.45022557716558,4.0109014146461,97.1008772065908));
#33145=CARTESIAN_POINT('Ctrl Pts',(-5.55297389602525,3.87128154929244,97.1090009348093));
#33146=CARTESIAN_POINT('Ctrl Pts',(-5.65034463591282,3.7277232312892,97.1171246630277));
#33147=CARTESIAN_POINT('Ctrl Pts',(-5.74203403516257,3.58068905925029,97.1252483912461));
#33148=CARTESIAN_POINT('Ctrl Pts',(-5.83374807808185,3.43361536834032,97.1333743029065));
#33149=CARTESIAN_POINT('Ctrl Pts',(-5.91977754634236,3.28306427347978,97.1415002145668));
#33150=CARTESIAN_POINT('Ctrl Pts',(-5.99986372172797,3.12952461576716,97.1496261262271));
#33151=CARTESIAN_POINT('Ctrl Pts',(-6.08046205652998,2.97500305598333,97.1578040039371));
#33152=CARTESIAN_POINT('Ctrl Pts',(-6.1550406449525,2.81745490935106,97.1659818816472));
#33153=CARTESIAN_POINT('Ctrl Pts',(-6.22338453038556,2.65739985454912,97.1741597593573));
#33154=CARTESIAN_POINT('Ctrl Pts',(-6.29140222527644,2.49810870780968,97.1822986058307));
#33155=CARTESIAN_POINT('Ctrl Pts',(-6.35324452736506,2.33633489402152,97.1904374523042));
#33156=CARTESIAN_POINT('Ctrl Pts',(-6.40874946345606,2.17260657152915,97.1985762987776));
#33157=CARTESIAN_POINT('Ctrl Pts',(-6.46465367473332,2.00770046808498,97.206773692106));
#33158=CARTESIAN_POINT('Ctrl Pts',(-6.51412889310712,1.84081199255287,97.2149710854344));
#33159=CARTESIAN_POINT('Ctrl Pts',(-6.55706192782659,1.67249151706282,97.2231684787627));
#33160=CARTESIAN_POINT('Ctrl Pts',(-6.59999496254606,1.50417104157277,97.2313658720911));
#33161=CARTESIAN_POINT('Ctrl Pts',(-6.63638579533957,1.33441894289787,97.2395632654195));
#33162=CARTESIAN_POINT('Ctrl Pts',(-6.6661743235188,1.16379074083731,97.2477606587479));
#33163=CARTESIAN_POINT('Ctrl Pts',(-6.71425349866384,0.888394012197591,
97.2609913866038));
#33164=CARTESIAN_POINT('Ctrl Pts',(-6.74526879236158,0.609985568231809,
97.2742221144597));
#33165=CARTESIAN_POINT('Ctrl Pts',(-6.75893709278174,0.330239876179668,
97.2874528423156));
#33166=CARTESIAN_POINT('Ctrl Pts',(-6.76422896296622,0.221932490367087,
97.2925753002736));
#33167=CARTESIAN_POINT('Ctrl Pts',(-6.766920989389,0.11342495687927,97.2976977582316));
#33168=CARTESIAN_POINT('Ctrl Pts',(-6.76699828620657,0.00481606451017424,
97.3028202161896));
#33169=CARTESIAN_POINT('Ctrl Pts',(-6.76699828620706,0.00481606382155593,
97.3028202162221));
#33170=CARTESIAN_POINT('Ctrl Pts',(-6.76712025881665,-0.166566307894805,
97.3109033388349));
#33171=CARTESIAN_POINT('Ctrl Pts',(-6.76072737653059,-0.338175828425599,
97.3189864614477));
#33172=CARTESIAN_POINT('Ctrl Pts',(-6.74779449262844,-0.50946882657651,
97.3270695840605));
#33173=CARTESIAN_POINT('Ctrl Pts',(-6.73487283404632,-0.680613148010278,
97.3351456907874));
#33174=CARTESIAN_POINT('Ctrl Pts',(-6.71542250083884,-0.851441125803964,
97.3432217975143));
#33175=CARTESIAN_POINT('Ctrl Pts',(-6.68947038760751,-1.02140830881792,
97.3512979042412));
#33176=CARTESIAN_POINT('Ctrl Pts',(-6.66353517089355,-1.19126483211662,
97.3593687528961));
#33177=CARTESIAN_POINT('Ctrl Pts',(-6.63110665762757,-1.3602613105025,97.3674396015511));
#33178=CARTESIAN_POINT('Ctrl Pts',(-6.59226363117107,-1.52785772149739,
97.3755104502061));
#33179=CARTESIAN_POINT('Ctrl Pts',(-6.55343387311752,-1.69539688317585,
97.3835785419371));
#33180=CARTESIAN_POINT('Ctrl Pts',(-6.50819404361204,-1.86153656734075,
97.391646633668));
#33181=CARTESIAN_POINT('Ctrl Pts',(-6.45667416967614,-2.02574619995618,
97.399714725399));
#33182=CARTESIAN_POINT('Ctrl Pts',(-6.40516252369416,-2.18992960756005,
97.4077815286197));
#33183=CARTESIAN_POINT('Ctrl Pts',(-6.34737293978065,-2.35218322242499,
97.4158483318404));
#33184=CARTESIAN_POINT('Ctrl Pts',(-6.28348549366712,-2.51199105310406,
97.4239151350611));
#33185=CARTESIAN_POINT('Ctrl Pts',(-6.21959571070349,-2.67180472917167,
97.4319822333462));
#33186=CARTESIAN_POINT('Ctrl Pts',(-6.14960775937732,-2.82917209784169,
97.4400493316312));
#33187=CARTESIAN_POINT('Ctrl Pts',(-6.07375004952149,-2.98359671134316,
97.4481164299163));
#33188=CARTESIAN_POINT('Ctrl Pts',(-5.99787467369683,-3.13805728770739,
97.4561854068912));
#33189=CARTESIAN_POINT('Ctrl Pts',(-5.91612698246284,-3.28957341148217,
97.4642543838661));
#33190=CARTESIAN_POINT('Ctrl Pts',(-5.82878150112226,-3.43767293560265,
97.472323360841));
#33191=CARTESIAN_POINT('Ctrl Pts',(-5.74135010679053,-3.58591813037385,
97.4804002744595));
#33192=CARTESIAN_POINT('Ctrl Pts',(-5.64831011398757,-3.73073969288594,
97.4884771880779));
#33193=CARTESIAN_POINT('Ctrl Pts',(-5.54998000547121,-3.87169354919392,
97.4965541016963));
#33194=CARTESIAN_POINT('Ctrl Pts',(-5.45159966181049,-4.01271941637859,
97.5046351416696));
#33195=CARTESIAN_POINT('Ctrl Pts',(-5.34792404227063,-4.14987334519492,
97.5127161816428));
#33196=CARTESIAN_POINT('Ctrl Pts',(-5.23931186014527,-4.28274447429929,
97.520797221616));
#33197=CARTESIAN_POINT('Ctrl Pts',(-5.13054413930407,-4.41580588228756,
97.5288898340903));
#33198=CARTESIAN_POINT('Ctrl Pts',(-5.01682597900833,-4.54457196028276,
97.5369824465645));
#33199=CARTESIAN_POINT('Ctrl Pts',(-4.89855359269738,-4.66866808623954,
97.5450750590387));
#33200=CARTESIAN_POINT('Ctrl Pts',(-4.79874025159647,-4.77339624245397,
97.5519046387443));
#33201=CARTESIAN_POINT('Ctrl Pts',(-4.69568404062259,-4.87479898062165,
97.55873421845));
#33202=CARTESIAN_POINT('Ctrl Pts',(-4.5896407234342,-4.97267403212743,97.5655637981556));
#33203=CARTESIAN_POINT('Ctrl Pts',(-4.46191197854839,-5.09056413417182,
97.5737899991745));
#33204=CARTESIAN_POINT('Ctrl Pts',(-4.32945957728245,-5.20369456492042,
97.5820162001933));
#33205=CARTESIAN_POINT('Ctrl Pts',(-4.19267247336223,-5.31166513732847,
97.5902424012122));
#33206=CARTESIAN_POINT('Ctrl Pts',(-4.05603902092366,-5.41951442755457,
97.5984593618279));
#33207=CARTESIAN_POINT('Ctrl Pts',(-3.91508084053274,-5.52221518069341,
97.6066763224437));
#33208=CARTESIAN_POINT('Ctrl Pts',(-3.77022318628941,-5.61940442801243,
97.6148932830595));
#33209=CARTESIAN_POINT('Ctrl Pts',(-3.62549917500851,-5.71650401034968,
97.6231026628611));
#33210=CARTESIAN_POINT('Ctrl Pts',(-3.47688315053867,-5.80810201490232,
97.6313120426627));
#33211=CARTESIAN_POINT('Ctrl Pts',(-3.32483292508749,-5.89387606081551,
97.6395214224643));
#33212=CARTESIAN_POINT('Ctrl Pts',(-3.1728924704349,-5.97958818320646,97.6477248756047));
#33213=CARTESIAN_POINT('Ctrl Pts',(-3.01752306419753,-6.05948454617642,
97.6559283287451));
#33214=CARTESIAN_POINT('Ctrl Pts',(-2.85921101992569,-6.13328634123139,
97.6641317818855));
#33215=CARTESIAN_POINT('Ctrl Pts',(-2.70098151009317,-6.20704966044074,
97.6723309582356));
#33216=CARTESIAN_POINT('Ctrl Pts',(-2.53981274273586,-6.27472459039795,
97.6805301345857));
#33217=CARTESIAN_POINT('Ctrl Pts',(-2.37621520132246,-6.33607846518681,
97.6887293109359));
#33218=CARTESIAN_POINT('Ctrl Pts',(-2.21264844325523,-6.39742079531828,
97.6969269444872));
#33219=CARTESIAN_POINT('Ctrl Pts',(-2.04665415471598,-6.45244430781402,
97.7051245780386));
#33220=CARTESIAN_POINT('Ctrl Pts',(-1.87876263760626,-6.50096454009209,
97.71332221159));
#33221=CARTESIAN_POINT('Ctrl Pts',(-1.71088321280617,-6.54948127772265,
97.7215192547105));
#33222=CARTESIAN_POINT('Ctrl Pts',(-1.54110717590793,-6.59149556754008,
97.7297162978311));
#33223=CARTESIAN_POINT('Ctrl Pts',(-1.36997977043031,-6.62687289968743,
97.7379133409517));
#33224=CARTESIAN_POINT('Ctrl Pts',(-1.19883358820531,-6.66225411356973,
97.7461112834829));
#33225=CARTESIAN_POINT('Ctrl Pts',(-1.02633609331553,-6.69099684630272,
97.7543092260141));
#33226=CARTESIAN_POINT('Ctrl Pts',(-0.853042547145141,-6.71301775751861,
97.7625071685453));
#33227=CARTESIAN_POINT('Ctrl Pts',(-0.679698490620669,-6.73504508723101,
97.7707075005537));
#33228=CARTESIAN_POINT('Ctrl Pts',(-0.505558276374564,-6.75034664767691,
97.7789078325621));
#33229=CARTESIAN_POINT('Ctrl Pts',(-0.331182163106764,-6.75889098705105,
97.7871081645706));
#33230=CARTESIAN_POINT('Ctrl Pts',(-0.15662430279854,-6.76744423193618,
97.7953170435413));
#33231=CARTESIAN_POINT('Ctrl Pts',(0.0181695890206001,-6.76922616762182,
97.8035259225121));
#33232=CARTESIAN_POINT('Ctrl Pts',(0.192638367528336,-6.76425749505118,
97.8117348014828));
#33233=CARTESIAN_POINT('Ctrl Pts',(0.367200804923314,-6.75928615518185,
97.8199480871702));
#33234=CARTESIAN_POINT('Ctrl Pts',(0.541437423555891,-6.74755700678809,
97.8281613728576));
#33235=CARTESIAN_POINT('Ctrl Pts',(0.714792420378166,-6.72914264938483,
97.836374658545));
#33236=CARTESIAN_POINT('Ctrl Pts',(0.888401014194871,-6.71070135404626,
97.8445999592571));
#33237=CARTESIAN_POINT('Ctrl Pts',(1.06112505389687,-6.68555535740216,97.8528252599692));
#33238=CARTESIAN_POINT('Ctrl Pts',(1.2324178746684,-6.65382861082233,97.8610505606813));
#33239=CARTESIAN_POINT('Ctrl Pts',(1.38733156837646,-6.62513559566919,97.8684893529752));
#33240=CARTESIAN_POINT('Ctrl Pts',(1.54107463423423,-6.59106087741857,97.8759281452692));
#33241=CARTESIAN_POINT('Ctrl Pts',(1.69325438273099,-6.55173096176593,97.8833669375632));
#33242=CARTESIAN_POINT('Ctrl Pts',(1.86003601946873,-6.50862727832513,97.8915194937764));
#33243=CARTESIAN_POINT('Ctrl Pts',(2.02543157073591,-6.45908359806189,97.8996720499897));
#33244=CARTESIAN_POINT('Ctrl Pts',(2.18890104298948,-6.4032024194148,97.9078246062029));
#33245=CARTESIAN_POINT('Ctrl Pts',(2.3521811319184,-6.3473859804604,97.9159677174833));
#33246=CARTESIAN_POINT('Ctrl Pts',(2.5135392412929,-6.28524677540145,97.9241108287636));
#33247=CARTESIAN_POINT('Ctrl Pts',(2.6724463572164,-6.21693811034024,97.932253940044));
#33248=CARTESIAN_POINT('Ctrl Pts',(2.83120278365768,-6.14869422146799,97.9403893293213));
#33249=CARTESIAN_POINT('Ctrl Pts',(2.98751251038381,-6.07429266339949,97.9485247185987));
#33250=CARTESIAN_POINT('Ctrl Pts',(3.14086246844589,-5.99393626545261,97.9566601078761));
#33251=CARTESIAN_POINT('Ctrl Pts',(3.29409922932973,-5.91363918358,97.9647894919147));
#33252=CARTESIAN_POINT('Ctrl Pts',(3.44438024941538,-5.8273961832761,97.9729188759533));
#33253=CARTESIAN_POINT('Ctrl Pts',(3.59121321704769,-5.73545783958892,97.9810482599919));
#33254=CARTESIAN_POINT('Ctrl Pts',(3.73796864004484,-5.64356804988408,97.9891733507841));
#33255=CARTESIAN_POINT('Ctrl Pts',(3.88127932797551,-5.54598910051285,97.9972984415762));
#33256=CARTESIAN_POINT('Ctrl Pts',(4.02067833662184,-5.44301705981341,98.0054235323684));
#33257=CARTESIAN_POINT('Ctrl Pts',(4.16060946150365,-5.33965195251193,98.0135796383935));
#33258=CARTESIAN_POINT('Ctrl Pts',(4.29659865865841,-5.23085267910821,98.0217357444186));
#33259=CARTESIAN_POINT('Ctrl Pts',(4.42820333081417,-5.11696240566278,98.0298918504437));
#33260=CARTESIAN_POINT('Ctrl Pts',(4.55927831796567,-5.00353051997053,98.0380151296171));
#33261=CARTESIAN_POINT('Ctrl Pts',(4.68600374401133,-4.885048796181,98.0461384087905));
#33262=CARTESIAN_POINT('Ctrl Pts',(4.80797609376235,-4.7618961435346,98.0542616879639));
#33263=CARTESIAN_POINT('Ctrl Pts',(4.92996468516247,-4.63872709207181,98.0623860488206));
#33264=CARTESIAN_POINT('Ctrl Pts',(5.04719868216898,-4.51088613284269,98.0705104096772));
#33265=CARTESIAN_POINT('Ctrl Pts',(5.15931210995732,-4.37878836575231,98.0786347705339));
#33266=CARTESIAN_POINT('Ctrl Pts',(5.2714617967521,-4.24664787644852,98.0867617589193));
#33267=CARTESIAN_POINT('Ctrl Pts',(5.37848737999048,-4.11024811658775,98.0948887473047));
#33268=CARTESIAN_POINT('Ctrl Pts',(5.48006381332114,-3.97003647362694,98.1030157356901));
#33269=CARTESIAN_POINT('Ctrl Pts',(5.58229692672876,-3.82891837835755,98.1111952641302));
#33270=CARTESIAN_POINT('Ctrl Pts',(5.67900996920538,-3.68393924668254,98.1193747925702));
#33271=CARTESIAN_POINT('Ctrl Pts',(5.7699168878031,-3.5355831354735,98.1275543210103));
#33272=CARTESIAN_POINT('Ctrl Pts',(5.86039569641415,-3.38792568101986,98.135695329414));
#33273=CARTESIAN_POINT('Ctrl Pts',(5.94512282658121,-3.23692333524932,98.1438363378176));
#33274=CARTESIAN_POINT('Ctrl Pts',(6.0238635010454,-3.08307598361979,98.1519773462213));
#33275=CARTESIAN_POINT('Ctrl Pts',(6.10316303016758,-2.92813671463416,98.1601761346796));
#33276=CARTESIAN_POINT('Ctrl Pts',(6.17639065570741,-2.77031224946982,98.1683749231378));
#33277=CARTESIAN_POINT('Ctrl Pts',(6.24335686394399,-2.61013104449633,98.1765737115961));
#33278=CARTESIAN_POINT('Ctrl Pts',(6.31032307218052,-2.44994983952296,98.1847725000543));
#33279=CARTESIAN_POINT('Ctrl Pts',(6.37102779387041,-2.28741226530144,98.1929712885126));
#33280=CARTESIAN_POINT('Ctrl Pts',(6.4253333466101,-2.12305920429465,98.2011700769708));
#33281=CARTESIAN_POINT('Ctrl Pts',(6.47986583521257,-1.95801933315856,98.2094031271028));
#33282=CARTESIAN_POINT('Ctrl Pts',(6.52811519062759,-1.79063577524243,98.2176361772349));
#33283=CARTESIAN_POINT('Ctrl Pts',(6.56987538026672,-1.62142729956208,98.2258692273669));
#33284=CARTESIAN_POINT('Ctrl Pts',(6.61158583993922,-1.45242032516615,98.2340924732018));
#33285=CARTESIAN_POINT('Ctrl Pts',(6.64682243641483,-1.28159310471467,98.2423157190366));
#33286=CARTESIAN_POINT('Ctrl Pts',(6.67542792079323,-1.10948234519267,98.2505389648715));
#33287=CARTESIAN_POINT('Ctrl Pts',(6.70400506588621,-0.937542094789563,
98.258754063985));
#33288=CARTESIAN_POINT('Ctrl Pts',(6.72596412360857,-0.764321188618504,
98.2669691630985));
#33289=CARTESIAN_POINT('Ctrl Pts',(6.74119817767269,-0.590369485443122,
98.275184262212));
#33290=CARTESIAN_POINT('Ctrl Pts',(6.75642018747615,-0.416555310968091,
98.2833928663509));
#33291=CARTESIAN_POINT('Ctrl Pts',(6.76492775268185,-0.242011845518606,
98.2916014704897));
#33292=CARTESIAN_POINT('Ctrl Pts',(6.76666535962014,-0.0672971835734554,
98.2998100746286));
#33293=CARTESIAN_POINT('Ctrl Pts',(6.76840194035141,0.107314294270125,98.3080138308775));
#33294=CARTESIAN_POINT('Ctrl Pts',(6.7633765243107,0.282096409987835,98.3162175871265));
#33295=CARTESIAN_POINT('Ctrl Pts',(6.75158558117908,0.456487831179224,98.3244213433754));
#33296=CARTESIAN_POINT('Ctrl Pts',(6.73979812669032,0.630827654345044,98.3326226723397));
#33297=CARTESIAN_POINT('Ctrl Pts',(6.72124915280194,0.804776656076253,98.340824001304));
#33298=CARTESIAN_POINT('Ctrl Pts',(6.69598721473029,0.977775137835097,98.3490253302683));
#33299=CARTESIAN_POINT('Ctrl Pts',(6.67072876052111,1.15074976145157,98.357225528191));
#33300=CARTESIAN_POINT('Ctrl Pts',(6.63875923692142,1.32277377165659,98.3654257261137));
#33301=CARTESIAN_POINT('Ctrl Pts',(6.60017889556942,1.49329419287695,98.3736259240364));
#33302=CARTESIAN_POINT('Ctrl Pts',(6.56159688327189,1.66382199947359,98.3818264771163));
#33303=CARTESIAN_POINT('Ctrl Pts',(6.51640356181274,1.83284573786251,98.3900270301961));
#33304=CARTESIAN_POINT('Ctrl Pts',(6.46474998749758,1.99982414205601,98.398227583276));
#33305=CARTESIAN_POINT('Ctrl Pts',(6.41308481538515,2.166840037976,98.4064299776292));
#33306=CARTESIAN_POINT('Ctrl Pts',(6.35495660724463,2.33180934281354,98.4146323719825));
#33307=CARTESIAN_POINT('Ctrl Pts',(6.29056583944162,2.49420737302459,98.4228347663357));
#33308=CARTESIAN_POINT('Ctrl Pts',(6.22611485495184,2.65675727394085,98.4310448313696));
#33309=CARTESIAN_POINT('Ctrl Pts',(6.15538974204171,2.81673076256253,98.4392548964034));
#33310=CARTESIAN_POINT('Ctrl Pts',(6.07863893984624,2.97362365456442,98.4474649614372));
#33311=CARTESIAN_POINT('Ctrl Pts',(6.00185140607834,3.13059163272124,98.4556789556625));
#33312=CARTESIAN_POINT('Ctrl Pts',(5.91903260292534,3.28447575938713,98.4638929498879));
#33313=CARTESIAN_POINT('Ctrl Pts',(5.83047619913612,3.43479785304859,98.4721069441132));
#33314=CARTESIAN_POINT('Ctrl Pts',(5.74179906347384,3.58532488579015,98.4803321367484));
#33315=CARTESIAN_POINT('Ctrl Pts',(5.64736888802309,3.7322798787694,98.4885573293835));
#33316=CARTESIAN_POINT('Ctrl Pts',(5.54752249562304,3.8752139502944,98.4967825220187));
#33317=CARTESIAN_POINT('Ctrl Pts',(5.45773084879053,4.00375425467799,98.5041794201387));
#33318=CARTESIAN_POINT('Ctrl Pts',(5.36355958090421,4.12904297003078,98.5115763182586));
#33319=CARTESIAN_POINT('Ctrl Pts',(5.26528024522293,4.25077792165919,98.5189732163786));
#33320=CARTESIAN_POINT('Ctrl Pts',(5.15038784002089,4.39309086356896,98.5276204809347));
#33321=CARTESIAN_POINT('Ctrl Pts',(5.02961995337024,4.53086980111672,98.5362677454909));
#33322=CARTESIAN_POINT('Ctrl Pts',(4.90335080295773,4.66362947747072,98.544915010047));
#33323=CARTESIAN_POINT('Ctrl Pts',(4.77367669485546,4.79996913420325,98.5537954556283));
#33324=CARTESIAN_POINT('Ctrl Pts',(4.63820061448258,4.93101474878858,98.5626759012097));
#33325=CARTESIAN_POINT('Ctrl Pts',(4.49737371021885,5.05627518145841,98.571556346791));
#33326=CARTESIAN_POINT('Ctrl Pts',(4.36064724662039,5.17788842061395,98.5801782214666));
#33327=CARTESIAN_POINT('Ctrl Pts',(4.21887741583759,5.29404839263359,98.5888000961422));
#33328=CARTESIAN_POINT('Ctrl Pts',(4.07251623075589,5.40434089878034,98.5974219708178));
#33329=CARTESIAN_POINT('Ctrl Pts',(3.91957096524828,5.5195949302826,98.606431701852));
#33330=CARTESIAN_POINT('Ctrl Pts',(3.76161192035452,5.62844114554434,98.6154414328862));
#33331=CARTESIAN_POINT('Ctrl Pts',(3.59919627489112,5.73045156814102,98.6244511639204));
#33332=CARTESIAN_POINT('Ctrl Pts',(3.43678062942783,5.83246199073764,98.6334608949546));
#33333=CARTESIAN_POINT('Ctrl Pts',(3.2699086754152,5.92763636981966,98.6424706259888));
#33334=CARTESIAN_POINT('Ctrl Pts',(3.09917575053261,6.01559628526638,98.651480357023));
#33335=CARTESIAN_POINT('Origin',(0.,0.,-3.69717978381041));
#33336=CARTESIAN_POINT('',(3.09917575053253,6.01559628526642,101.045648756765));
#33337=CARTESIAN_POINT('',(3.0991757505325,6.01559628526644,100.651392015122));
#33338=CARTESIAN_POINT('',(3.09917575053259,6.01559628526639,-3.69717978381041));
#33339=CARTESIAN_POINT('',(-6.76699843452386,0.00460295031038521,99.6971797837795));
#33340=CARTESIAN_POINT('Ctrl Pts',(-6.76699843452431,0.00460294966435506,
99.6971797838098));
#33341=CARTESIAN_POINT('Ctrl Pts',(-6.76712147278358,-0.176280998367531,
99.7056577969028));
#33342=CARTESIAN_POINT('Ctrl Pts',(-6.75998706702004,-0.357203135436458,
99.7141358099958));
#33343=CARTESIAN_POINT('Ctrl Pts',(-6.74561582556332,-0.537546401634019,
99.7226138230887));
#33344=CARTESIAN_POINT('Ctrl Pts',(-6.73162618285362,-0.713101023467001,
99.7308667199882));
#33345=CARTESIAN_POINT('Ctrl Pts',(-6.71077918971529,-0.888106761828978,
99.7391196168876));
#33346=CARTESIAN_POINT('Ctrl Pts',(-6.68314655339852,-1.06199865621265,
99.747372513787));
#33347=CARTESIAN_POINT('Ctrl Pts',(-6.65550828022493,-1.23592602327798,
99.7556270942174));
#33348=CARTESIAN_POINT('Ctrl Pts',(-6.62108166028766,-1.40873874611643,
99.7638816746477));
#33349=CARTESIAN_POINT('Ctrl Pts',(-6.57998975001323,-1.57988097327644,
99.7721362550781));
#33350=CARTESIAN_POINT('Ctrl Pts',(-6.53888239501195,-1.75108752562679,
99.7803939380592));
#33351=CARTESIAN_POINT('Ctrl Pts',(-6.49110483947996,-1.92062198926723,
99.7886516210404));
#33352=CARTESIAN_POINT('Ctrl Pts',(-6.43683037080898,-2.08794247464608,
99.7969093040216));
#33353=CARTESIAN_POINT('Ctrl Pts',(-6.38000869095953,-2.2631156506395,99.8055545368565));
#33354=CARTESIAN_POINT('Ctrl Pts',(-6.31606570320358,-2.43586160856736,
99.8141997696915));
#33355=CARTESIAN_POINT('Ctrl Pts',(-6.24525690462115,-2.60558154646557,
99.8228450025265));
#33356=CARTESIAN_POINT('Ctrl Pts',(-6.17749876946579,-2.76798942120558,
99.8311177718236));
#33357=CARTESIAN_POINT('Ctrl Pts',(-6.1034542234713,-2.92762626111469,99.8393905411208));
#33358=CARTESIAN_POINT('Ctrl Pts',(-6.02339433608997,-3.08399248895961,
99.8476633104179));
#33359=CARTESIAN_POINT('Ctrl Pts',(-5.94327424283882,-3.24047630583778,
99.8559423009238));
#33360=CARTESIAN_POINT('Ctrl Pts',(-5.85712996145528,-3.39368430193884,
99.8642212914297));
#33361=CARTESIAN_POINT('Ctrl Pts',(-5.76527650926265,-3.54314489849685,
99.8725002819356));
#33362=CARTESIAN_POINT('Ctrl Pts',(-5.67329733532742,-3.69281006490175,
99.8807906040691));
#33363=CARTESIAN_POINT('Ctrl Pts',(-5.57559358157656,-3.83871729907965,
99.8890809262026));
#33364=CARTESIAN_POINT('Ctrl Pts',(-5.47252174286387,-3.98042645628357,
99.8973712483361));
#33365=CARTESIAN_POINT('Ctrl Pts',(-5.45892503712293,-3.99911999794697,
99.8984648649045));
#33366=CARTESIAN_POINT('Ctrl Pts',(-5.44523497269768,-4.01774053746264,
99.8995584814728));
#33367=CARTESIAN_POINT('Ctrl Pts',(-5.43145241659336,-4.03628711147784,
99.9006520980411));
#33368=CARTESIAN_POINT('Ctrl Pts',(-5.32872777582496,-4.1745191011593,99.9088030802154));
#33369=CARTESIAN_POINT('Ctrl Pts',(-5.22056125470119,-4.3090441211298,99.9169540623897));
#33370=CARTESIAN_POINT('Ctrl Pts',(-5.10725086796601,-4.43940058697798,
99.925105044564));
#33371=CARTESIAN_POINT('Ctrl Pts',(-4.99407210174695,-4.56960563170927,
99.933246558617));
#33372=CARTESIAN_POINT('Ctrl Pts',(-4.87576160121589,-4.69565148783513,
99.9413880726701));
#33373=CARTESIAN_POINT('Ctrl Pts',(-4.75266032672034,-4.81710585505639,
99.9495295867231));
#33374=CARTESIAN_POINT('Ctrl Pts',(-4.6296761407412,-4.93844470022698,99.9576633569261));
#33375=CARTESIAN_POINT('Ctrl Pts',(-4.50191051119424,-5.05520049591546,
99.9657971271292));
#33376=CARTESIAN_POINT('Ctrl Pts',(-4.36974428504397,-5.16697434513909,
99.9739308973322));
#33377=CARTESIAN_POINT('Ctrl Pts',(-4.2376759723153,-5.27866538833625,99.9820586417502));
#33378=CARTESIAN_POINT('Ctrl Pts',(-4.10121383244336,-5.38538159887556,
99.9901863861682));
#33379=CARTESIAN_POINT('Ctrl Pts',(-3.96077514037961,-5.48676127486433,
99.9983141305862));
#33380=CARTESIAN_POINT('Ctrl Pts',(-3.82041096409603,-5.58808715951158,
100.00643756248));
#33381=CARTESIAN_POINT('Ctrl Pts',(-3.67607473345162,-5.68408193508003,
100.014560994374));
#33382=CARTESIAN_POINT('Ctrl Pts',(-3.52821632843498,-5.77442452022406,
100.022684426268));
#33383=CARTESIAN_POINT('Ctrl Pts',(-3.3794199678544,-5.86534020319357,100.030859390019));
#33384=CARTESIAN_POINT('Ctrl Pts',(-3.22705688234896,-5.95053149976472,
100.03903435377));
#33385=CARTESIAN_POINT('Ctrl Pts',(-3.07161512742359,-6.02971554129899,
100.047209317521));
#33386=CARTESIAN_POINT('Ctrl Pts',(-2.91718825626933,-6.10838258790662,
100.055330906694));
#33387=CARTESIAN_POINT('Ctrl Pts',(-2.75972313929371,-6.18112044471976,
100.063452495867));
#33388=CARTESIAN_POINT('Ctrl Pts',(-2.59972259339031,-6.24769809109051,
100.07157408504));
#33389=CARTESIAN_POINT('Ctrl Pts',(-2.43970092413312,-6.31428452707614,
100.079696746429));
#33390=CARTESIAN_POINT('Ctrl Pts',(-2.27714349716172,-6.37470899210375,
100.087819407819));
#33391=CARTESIAN_POINT('Ctrl Pts',(-2.1125725176687,-6.42878887175422,100.095942069208));
#33392=CARTESIAN_POINT('Ctrl Pts',(-1.94794847224879,-6.48288618946667,
100.10406734975));
#33393=CARTESIAN_POINT('Ctrl Pts',(-1.78130992892538,-6.53063473376461,
100.112192630293));
#33394=CARTESIAN_POINT('Ctrl Pts',(-1.61319358738926,-6.57190196591567,
100.120317910835));
#33395=CARTESIAN_POINT('Ctrl Pts',(-1.44324565319637,-6.61361879599802,
100.128531714623));
#33396=CARTESIAN_POINT('Ctrl Pts',(-1.27178790456063,-6.64871216986633,
100.13674551841));
#33397=CARTESIAN_POINT('Ctrl Pts',(-1.09938370566036,-6.67709850666654,
100.144959322198));
#33398=CARTESIAN_POINT('Ctrl Pts',(-0.928542451599543,-6.70522750473082,
100.153098663053));
#33399=CARTESIAN_POINT('Ctrl Pts',(-0.75677220700001,-6.72677059055827,
100.161238003909));
#33400=CARTESIAN_POINT('Ctrl Pts',(-0.584624310447284,-6.74169885233938,
100.169377344764));
#33401=CARTESIAN_POINT('Ctrl Pts',(-0.410114065865435,-6.7568319714002,
100.177628380018));
#33402=CARTESIAN_POINT('Ctrl Pts',(-0.235216121394139,-6.76516738364924,
100.185879415272));
#33403=CARTESIAN_POINT('Ctrl Pts',(-0.0605023203693838,-6.766729525349,
100.194130450526));
#33404=CARTESIAN_POINT('Ctrl Pts',(0.114211480655372,-6.76829166704876,
100.20238148578));
#33405=CARTESIAN_POINT('Ctrl Pts',(0.288740756527682,-6.76308061669069,
100.210632521034));
#33406=CARTESIAN_POINT('Ctrl Pts',(0.462521958286907,-6.75117489316508,
100.218883556288));
#33407=CARTESIAN_POINT('Ctrl Pts',(0.635897442947746,-6.73929696525575,
100.227115328319));
#33408=CARTESIAN_POINT('Ctrl Pts',(0.809069602165128,-6.72071868441591,
100.23534710035));
#33409=CARTESIAN_POINT('Ctrl Pts',(0.981480455201753,-6.69544510216139,
100.243578872381));
#33410=CARTESIAN_POINT('Ctrl Pts',(1.15368543245004,-6.67020169908979,100.251800814853));
#33411=CARTESIAN_POINT('Ctrl Pts',(1.32513056266644,-6.6382789656706,100.260022757325));
#33412=CARTESIAN_POINT('Ctrl Pts',(1.49525966648751,-6.59973389840649,100.268244699798));
#33413=CARTESIAN_POINT('Ctrl Pts',(1.66521970601936,-6.56122713496138,100.276458471788));
#33414=CARTESIAN_POINT('Ctrl Pts',(1.83386597656863,-6.5161112221054,100.284672243778));
#33415=CARTESIAN_POINT('Ctrl Pts',(2.00064911876799,-6.46449472917821,100.292886015768));
#33416=CARTESIAN_POINT('Ctrl Pts',(2.16729992602677,-6.41291919162237,100.301093270498));
#33417=CARTESIAN_POINT('Ctrl Pts',(2.33209020865481,-6.35485345290745,100.309300525228));
#33418=CARTESIAN_POINT('Ctrl Pts',(2.49448238538121,-6.29045679017215,100.317507779959));
#33419=CARTESIAN_POINT('Ctrl Pts',(2.65677822760844,-6.22609832890922,100.325710165971));
#33420=CARTESIAN_POINT('Ctrl Pts',(2.8166784657489,-6.15541655703321,100.333912551983));
#33421=CARTESIAN_POINT('Ctrl Pts',(2.97366214565786,-6.07862011014683,100.342114937995));
#33422=CARTESIAN_POINT('Ctrl Pts',(3.13059896974563,-6.00184658513734,100.350314875793));
#33423=CARTESIAN_POINT('Ctrl Pts',(3.28462064648304,-5.91896217437964,100.358514813592));
#33424=CARTESIAN_POINT('Ctrl Pts',(3.43522740073952,-5.83022312653714,100.366714751391));
#33425=CARTESIAN_POINT('Ctrl Pts',(3.58581309628472,-5.74149648670379,100.374913542626));
#33426=CARTESIAN_POINT('Ctrl Pts',(3.7329845112302,-5.64691702137982,100.383112333862));
#33427=CARTESIAN_POINT('Ctrl Pts',(3.87626761592042,-5.54678631008683,100.391311125098));
#33428=CARTESIAN_POINT('Ctrl Pts',(4.01955667823318,-5.44665143542102,100.399510257234));
#33429=CARTESIAN_POINT('Ctrl Pts',(4.1589568143405,-5.34096506020348,100.407709389371));
#33430=CARTESIAN_POINT('Ctrl Pts',(4.29402402246869,-5.23007138521663,100.415908521507));
#33431=CARTESIAN_POINT('Ctrl Pts',(4.42912134841042,-5.11915298272507,100.424109481918));
#33432=CARTESIAN_POINT('Ctrl Pts',(4.55988354506914,-5.0030251951959,100.432310442329));
#33433=CARTESIAN_POINT('Ctrl Pts',(4.68590062930382,-4.8820717213382,100.44051140274));
#33434=CARTESIAN_POINT('Ctrl Pts',(4.8120358218826,-4.76100488495828,100.448720049425));
#33435=CARTESIAN_POINT('Ctrl Pts',(4.93341675764953,-4.63510357443739,100.45692869611));
#33436=CARTESIAN_POINT('Ctrl Pts',(5.04967054633178,-4.50478816078063,100.465137342795));
#33437=CARTESIAN_POINT('Ctrl Pts',(5.16597983783781,-4.37441053088539,100.473349908519));
#33438=CARTESIAN_POINT('Ctrl Pts',(5.27715687373246,-4.23961487238904,100.481562474242));
#33439=CARTESIAN_POINT('Ctrl Pts',(5.38286992563477,-4.10085361402925,100.489775039966));
#33440=CARTESIAN_POINT('Ctrl Pts',(5.48872803109883,-3.96190195519954,100.497998874514));
#33441=CARTESIAN_POINT('Ctrl Pts',(5.58910696261734,-3.81897411506567,100.506222709063));
#33442=CARTESIAN_POINT('Ctrl Pts',(5.68371841565184,-3.67255142531458,100.514446543612));
#33443=CARTESIAN_POINT('Ctrl Pts',(5.77064854373808,-3.5380165168384,100.522002700586));
#33444=CARTESIAN_POINT('Ctrl Pts',(5.85271009104159,-3.40053169453125,100.52955885756));
#33445=CARTESIAN_POINT('Ctrl Pts',(5.92971449565611,-3.26048692682639,100.537115014535));
#33446=CARTESIAN_POINT('Ctrl Pts',(6.01782256082213,-3.10024838487717,100.545760732587));
#33447=CARTESIAN_POINT('Ctrl Pts',(6.0995104558487,-2.93629304170823,100.554406450639));
#33448=CARTESIAN_POINT('Ctrl Pts',(6.17447106581951,-2.76915078270537,100.563052168692));
#33449=CARTESIAN_POINT('Ctrl Pts',(6.24933544164374,-2.60222310030022,100.571686787404));
#33450=CARTESIAN_POINT('Ctrl Pts',(6.31748962976128,-2.43211693737029,100.580321406116));
#33451=CARTESIAN_POINT('Ctrl Pts',(6.3786722981306,-2.25938680023173,100.588956024829));
#33452=CARTESIAN_POINT('Ctrl Pts',(6.44201570067107,-2.08055650565231,100.597895584731));
#33453=CARTESIAN_POINT('Ctrl Pts',(6.49788600240192,-1.8989137845199,100.606835144634));
#33454=CARTESIAN_POINT('Ctrl Pts',(6.54604630935398,-1.71509962270219,100.615774704536));
#33455=CARTESIAN_POINT('Ctrl Pts',(6.5924346896645,-1.53804839972416,100.624385357806));
#33456=CARTESIAN_POINT('Ctrl Pts',(6.63167015877937,-1.35898299510614,100.632996011077));
#33457=CARTESIAN_POINT('Ctrl Pts',(6.66359053769349,-1.17849486463109,100.641606664347));
#33458=CARTESIAN_POINT('Ctrl Pts',(6.69548070183318,-0.998177578247951,
100.650209167058));
#33459=CARTESIAN_POINT('Ctrl Pts',(6.7200695278703,-0.816440550316719,100.658811669769));
#33460=CARTESIAN_POINT('Ctrl Pts',(6.73724540547018,-0.633887487233368,
100.66741417248));
#33461=CARTESIAN_POINT('Ctrl Pts',(6.75440195196575,-0.451539883945666,
100.676006993248));
#33462=CARTESIAN_POINT('Ctrl Pts',(6.76416216579936,-0.268378380753643,
100.684599814015));
#33463=CARTESIAN_POINT('Ctrl Pts',(6.76646596088498,-0.0850141175624732,
100.693192634783));
#33464=CARTESIAN_POINT('Ctrl Pts',(6.76673747360029,-0.0634038062546583,
100.694205337741));
#33465=CARTESIAN_POINT('Ctrl Pts',(6.76690547795264,-0.041790686436373,
100.6952180407));
#33466=CARTESIAN_POINT('Ctrl Pts',(6.76696992298183,-0.0201757641571949,
100.696230743658));
#33467=CARTESIAN_POINT('Ctrl Pts',(6.76751689643798,0.163279637956664,100.704826001418));
#33468=CARTESIAN_POINT('Ctrl Pts',(6.76059889533746,0.346649193364827,100.713421259178));
#33469=CARTESIAN_POINT('Ctrl Pts',(6.74626631702619,0.529320110857158,100.722016516938));
#33470=CARTESIAN_POINT('Ctrl Pts',(6.73192031686319,0.712162091916675,100.730619823793));
#33471=CARTESIAN_POINT('Ctrl Pts',(6.71014590400629,0.894303824750037,100.739223130647));
#33472=CARTESIAN_POINT('Ctrl Pts',(6.68104513733997,1.07513946668602,100.747826437502));
#33473=CARTESIAN_POINT('Ctrl Pts',(6.65073784279662,1.26347261704365,100.756786440442));
#33474=CARTESIAN_POINT('Ctrl Pts',(6.61248381678592,1.45038869262551,100.765746443382));
#33475=CARTESIAN_POINT('Ctrl Pts',(6.56645638204994,1.63521851219818,100.774706446322));
#33476=CARTESIAN_POINT('Ctrl Pts',(6.52214038514164,1.81317580570644,100.783333289527));
#33477=CARTESIAN_POINT('Ctrl Pts',(6.47061876047074,1.98919892111022,100.791960132731));
#33478=CARTESIAN_POINT('Ctrl Pts',(6.41209640505305,2.16270864711494,100.800586975936));
#33479=CARTESIAN_POINT('Ctrl Pts',(6.35351811705737,2.33638420455647,100.809222064222));
#33480=CARTESIAN_POINT('Ctrl Pts',(6.28792584884988,2.50754129194284,100.817857152508));
#33481=CARTESIAN_POINT('Ctrl Pts',(6.21557246644582,2.67562103339778,100.826492240794));
#33482=CARTESIAN_POINT('Ctrl Pts',(6.14311162474885,2.84395040699941,100.83514015392));
#33483=CARTESIAN_POINT('Ctrl Pts',(6.06386973016573,3.00919302443718,100.843788067045));
#33484=CARTESIAN_POINT('Ctrl Pts',(5.97814604092336,3.17081360432813,100.85243598017));
#33485=CARTESIAN_POINT('Ctrl Pts',(5.96852914797797,3.18894497301187,100.853406144374));
#33486=CARTESIAN_POINT('Ctrl Pts',(5.95883072418472,3.20703078618554,100.854376308578));
#33487=CARTESIAN_POINT('Ctrl Pts',(5.94905122609331,3.22507031075567,100.855346472781));
#33488=CARTESIAN_POINT('Ctrl Pts',(5.86615315497012,3.37798631696225,100.863570283494));
#33489=CARTESIAN_POINT('Ctrl Pts',(5.77724617322386,3.52790551519329,100.871794094208));
#33490=CARTESIAN_POINT('Ctrl Pts',(5.68257231884336,3.67432454215944,100.880017904921));
#33491=CARTESIAN_POINT('Ctrl Pts',(5.58799266104182,3.82059788823486,100.888233533281));
#33492=CARTESIAN_POINT('Ctrl Pts',(5.48765774697219,3.96337769808229,100.896449161642));
#33493=CARTESIAN_POINT('Ctrl Pts',(5.38185586416934,4.10218435194057,100.904664790003));
#33494=CARTESIAN_POINT('Ctrl Pts',(5.27614004912307,4.24087808930834,100.912873735111));
#33495=CARTESIAN_POINT('Ctrl Pts',(5.16496633698996,4.37560482318377,100.921082680219));
#33496=CARTESIAN_POINT('Ctrl Pts',(5.0486667791945,4.50591308756149,100.929291625327));
#33497=CARTESIAN_POINT('Ctrl Pts',(4.93244072621485,4.6361389931998,100.937495382135));
#33498=CARTESIAN_POINT('Ctrl Pts',(4.81109551777379,4.76195172485433,100.945699138944));
#33499=CARTESIAN_POINT('Ctrl Pts',(4.68500405485413,4.88293211154941,100.953902895752));
#33500=CARTESIAN_POINT('Ctrl Pts',(4.55896454466797,5.00386265139806,100.962103272414));
#33501=CARTESIAN_POINT('Ctrl Pts',(4.42818293267857,5.11996456382018,100.970303649076));
#33502=CARTESIAN_POINT('Ctrl Pts',(4.2930697041237,5.23085475955271,100.978504025737));
#33503=CARTESIAN_POINT('Ctrl Pts',(4.15799079295077,5.34171679030657,100.986702319587));
#33504=CARTESIAN_POINT('Ctrl Pts',(4.01858273469258,5.44736951538114,100.994900613437));
#33505=CARTESIAN_POINT('Ctrl Pts',(3.87528989711106,5.54746944230872,101.003098907287));
#33506=CARTESIAN_POINT('Ctrl Pts',(3.7319796150341,5.64758155541913,101.011298199198));
#33507=CARTESIAN_POINT('Ctrl Pts',(3.58478390008576,5.74213931093279,101.01949749111));
#33508=CARTESIAN_POINT('Ctrl Pts',(3.43417727668268,5.83084174303473,101.027696783022));
#33509=CARTESIAN_POINT('Ctrl Pts',(3.32426184422437,5.8955783792084,101.033680774269));
#33510=CARTESIAN_POINT('Ctrl Pts',(3.21253028801932,5.95719714790205,101.039664765517));
#33511=CARTESIAN_POINT('Ctrl Pts',(3.09917575053253,6.01559628526642,101.045648756765));
#33512=CARTESIAN_POINT('Ctrl Pts',(3.09917575053247,6.01559628526645,99.0459901976524));
#33513=CARTESIAN_POINT('Ctrl Pts',(2.9453019261631,6.09487055875705,99.054114251979));
#33514=CARTESIAN_POINT('Ctrl Pts',(2.78828904708904,6.16828618756218,99.0622383063056));
#33515=CARTESIAN_POINT('Ctrl Pts',(2.62862901059509,6.23559127305967,99.0703623606321));
#33516=CARTESIAN_POINT('Ctrl Pts',(2.46900589338129,6.30288079514278,99.0784845363782));
#33517=CARTESIAN_POINT('Ctrl Pts',(2.30673717191679,6.36406243989334,99.0866067121242));
#33518=CARTESIAN_POINT('Ctrl Pts',(2.14233674687458,6.41893155151158,99.0947288878703));
#33519=CARTESIAN_POINT('Ctrl Pts',(1.97795210363151,6.47379539590926,99.1028502839191));
#33520=CARTESIAN_POINT('Ctrl Pts',(1.81143651095054,6.52234779680194,99.110971679968));
#33521=CARTESIAN_POINT('Ctrl Pts',(1.64332100676458,6.56443333949902,99.1190930760168));
#33522=CARTESIAN_POINT('Ctrl Pts',(1.47518962954841,6.60652285580397,99.1272152388669));
#33523=CARTESIAN_POINT('Ctrl Pts',(1.30545839498646,6.64214420889851,99.1353374017169));
#33524=CARTESIAN_POINT('Ctrl Pts',(1.13467051781992,6.6711926831707,99.143459564567));
#33525=CARTESIAN_POINT('Ctrl Pts',(0.963833993153826,6.70024943165803,99.1515840409472));
#33526=CARTESIAN_POINT('Ctrl Pts',(0.791940587215222,6.7227295120575,99.1597085173274));
#33527=CARTESIAN_POINT('Ctrl Pts',(0.619540608498186,6.73857985293799,99.1678329937077));
#33528=CARTESIAN_POINT('Ctrl Pts',(0.446956624270756,6.75444711116431,99.1759661414836));
#33529=CARTESIAN_POINT('Ctrl Pts',(0.273865352014489,6.76367046088517,99.1840992892594));
#33530=CARTESIAN_POINT('Ctrl Pts',(0.100820022460005,6.76624891081249,99.1922324370353));
#33531=CARTESIAN_POINT('Ctrl Pts',(-0.0723196613544442,6.76882876665891,
99.2003700194708));
#33532=CARTESIAN_POINT('Ctrl Pts',(-0.245412987278003,6.76475651143226,
99.2085076019064));
#33533=CARTESIAN_POINT('Ctrl Pts',(-0.417910158476497,6.75408321679872,
99.2166451843419));
#33534=CARTESIAN_POINT('Ctrl Pts',(-0.590670436730441,6.74339364236707,
99.224795178896));
#33535=CARTESIAN_POINT('Ctrl Pts',(-0.762832379482159,6.72608294650915,
99.2329451734502));
#33536=CARTESIAN_POINT('Ctrl Pts',(-0.933853479637257,6.70225385065124,
99.2410951680044));
#33537=CARTESIAN_POINT('Ctrl Pts',(-1.09538993126271,6.67974629113467,99.2487931725187));
#33538=CARTESIAN_POINT('Ctrl Pts',(-1.2559084081125,6.65142379097088,99.2564911770331));
#33539=CARTESIAN_POINT('Ctrl Pts',(-1.41496405507995,6.61741382436007,99.2641891815474));
#33540=CARTESIAN_POINT('Ctrl Pts',(-1.58490571297841,6.58107616379215,99.272414049225));
#33541=CARTESIAN_POINT('Ctrl Pts',(-1.75368527277329,6.5381368794794,99.2806389169026));
#33542=CARTESIAN_POINT('Ctrl Pts',(-1.92075162863111,6.48868262292979,99.2888637845802));
#33543=CARTESIAN_POINT('Ctrl Pts',(-2.08762976553951,6.43928408213554,99.2970793860238));
#33544=CARTESIAN_POINT('Ctrl Pts',(-2.25279820098518,6.38338528551219,99.3052949874673));
#33545=CARTESIAN_POINT('Ctrl Pts',(-2.41571526919148,6.32112400908218,99.3135105889108));
#33546=CARTESIAN_POINT('Ctrl Pts',(-2.57848152639321,6.25892036740921,99.321718585239));
#33547=CARTESIAN_POINT('Ctrl Pts',(-2.73900023380844,6.19036610264663,99.3299265815671));
#33548=CARTESIAN_POINT('Ctrl Pts',(-2.89674407920975,6.11564900395398,99.3381345778952));
#33549=CARTESIAN_POINT('Ctrl Pts',(-3.05437358608738,6.04098606295437,99.3463366247666));
#33550=CARTESIAN_POINT('Ctrl Pts',(-3.20923191420068,5.96016933849633,99.3545386716381));
#33551=CARTESIAN_POINT('Ctrl Pts',(-3.36081088534313,5.87343504203112,99.3627407185095));
#33552=CARTESIAN_POINT('Ctrl Pts',(-3.51231042490358,5.78674619674117,99.370938467281));
#33553=CARTESIAN_POINT('Ctrl Pts',(-3.66053372030914,5.69414613483585,99.3791362160525));
#33554=CARTESIAN_POINT('Ctrl Pts',(-3.80499632793892,5.59591743544983,99.387333964824));
#33555=CARTESIAN_POINT('Ctrl Pts',(-3.94943138222869,5.4977074712147,99.3955301500396));
#33556=CARTESIAN_POINT('Ctrl Pts',(-4.09010687758579,5.39387120425928,99.4037263352552));
#33557=CARTESIAN_POINT('Ctrl Pts',(-4.22656630109052,5.28473521592956,99.4119225204709));
#33558=CARTESIAN_POINT('Ctrl Pts',(-4.36301562963498,5.17560730123402,99.4201180993512));
#33559=CARTESIAN_POINT('Ctrl Pts',(-4.49524922669044,5.06118066938256,99.4283136782316));
#33560=CARTESIAN_POINT('Ctrl Pts',(-4.62284275408058,4.94182292995659,99.4365092571119));
#33561=CARTESIAN_POINT('Ctrl Pts',(-4.7504500565209,4.82245230461952,99.4447057207904));
#33562=CARTESIAN_POINT('Ctrl Pts',(-4.87341602916203,4.6981497562585,99.4529021844689));
#33563=CARTESIAN_POINT('Ctrl Pts',(-4.9913523451223,4.56932060232614,99.4610986481473));
#33564=CARTESIAN_POINT('Ctrl Pts',(-5.10932285074251,4.44045410090732,99.4692974879751));
#33565=CARTESIAN_POINT('Ctrl Pts',(-5.22226055311114,4.30705864467148,99.477496327803));
#33566=CARTESIAN_POINT('Ctrl Pts',(-5.32981662230743,4.16957357203053,99.4856951676308));
#33567=CARTESIAN_POINT('Ctrl Pts',(-5.43748503687707,4.03194489232089,99.49390257138));
#33568=CARTESIAN_POINT('Ctrl Pts',(-5.53976036631841,3.89021834486554,99.5021099751293));
#33569=CARTESIAN_POINT('Ctrl Pts',(-5.63633586376882,3.74486408709227,99.5103173788785));
#33570=CARTESIAN_POINT('Ctrl Pts',(-5.73296309216669,3.59943196988601,99.5185291789475));
#33571=CARTESIAN_POINT('Ctrl Pts',(-5.82388421540091,3.45036857460691,99.5267409790165));
#33572=CARTESIAN_POINT('Ctrl Pts',(-5.90883796009994,3.29816963803895,99.5349527790856));
#33573=CARTESIAN_POINT('Ctrl Pts',(-5.99391676858159,3.1457466433699,99.5431766680717));
#33574=CARTESIAN_POINT('Ctrl Pts',(-6.07301047969293,2.99017920242219,99.5514005570579));
#33575=CARTESIAN_POINT('Ctrl Pts',(-6.14590503211473,2.83198522881508,99.5596244460441));
#33576=CARTESIAN_POINT('Ctrl Pts',(-6.21325833836466,2.68581673203086,99.5672231772942));
#33577=CARTESIAN_POINT('Ctrl Pts',(-6.27531960375733,2.53740626967087,99.5748219085443));
#33578=CARTESIAN_POINT('Ctrl Pts',(-6.33195787521391,2.38717374032905,99.5824206397944));
#33579=CARTESIAN_POINT('Ctrl Pts',(-6.40323906825369,2.19810098705693,99.5919839017931));
#33580=CARTESIAN_POINT('Ctrl Pts',(-6.46610086863492,2.00569185012578,99.6015471637919));
#33581=CARTESIAN_POINT('Ctrl Pts',(-6.52026103456438,1.81065873127475,99.6111104257907));
#33582=CARTESIAN_POINT('Ctrl Pts',(-6.57312998749973,1.6202753267113,99.6204456935072));
#33583=CARTESIAN_POINT('Ctrl Pts',(-6.61770733335403,1.42739178948677,99.6297809612236));
#33584=CARTESIAN_POINT('Ctrl Pts',(-6.65377763927682,1.23269303845678,99.6391162289401));
#33585=CARTESIAN_POINT('Ctrl Pts',(-6.69116935725116,1.03086162610188,99.64879348808));
#33586=CARTESIAN_POINT('Ctrl Pts',(-6.71941885109214,0.827079589550037,
99.6584707472199));
#33587=CARTESIAN_POINT('Ctrl Pts',(-6.73834104999955,0.622132537238636,
99.6681480063598));
#33588=CARTESIAN_POINT('Ctrl Pts',(-6.75726324890696,0.417185484927235,
99.6778252654997));
#33589=CARTESIAN_POINT('Ctrl Pts',(-6.76685799203185,0.211073596220982,
99.6875025246397));
#33590=CARTESIAN_POINT('Ctrl Pts',(-6.76699843452387,0.0046029503101877,
99.6971797837796));
#33591=CARTESIAN_POINT('',(-6.767,5.7588601855979E-12,99.3028202161897));
#33592=CARTESIAN_POINT('Ctrl Pts',(3.09917575053261,6.01559628526638,98.651480357023));
#33593=CARTESIAN_POINT('Ctrl Pts',(2.93245238380909,6.10149051597834,98.6602785000427));
#33594=CARTESIAN_POINT('Ctrl Pts',(2.76204767700999,6.18050514918712,98.6690766430624));
#33595=CARTESIAN_POINT('Ctrl Pts',(2.58854694694294,6.25233665947959,98.6778747860822));
#33596=CARTESIAN_POINT('Ctrl Pts',(2.41903728943524,6.3225158149404,98.6864705436297));
#33597=CARTESIAN_POINT('Ctrl Pts',(2.24677147783188,6.38575632069298,98.6950663011773));
#33598=CARTESIAN_POINT('Ctrl Pts',(2.07233554270395,6.4418719638352,98.7036620587248));
#33599=CARTESIAN_POINT('Ctrl Pts',(1.89773685291709,6.4980399647806,98.7122658364065));
#33600=CARTESIAN_POINT('Ctrl Pts',(1.72096428866876,6.5470697404895,98.7208696140881));
#33601=CARTESIAN_POINT('Ctrl Pts',(1.54261708282097,6.58882550503418,98.7294733917698));
#33602=CARTESIAN_POINT('Ctrl Pts',(1.35726067582878,6.63222230763853,98.7384153054378));
#33603=CARTESIAN_POINT('Ctrl Pts',(1.17020372440459,6.66776171376448,98.7473572191058));
#33604=CARTESIAN_POINT('Ctrl Pts',(0.982126885110365,6.69535031059193,98.7562991327739));
#33605=CARTESIAN_POINT('Ctrl Pts',(0.800669424599743,6.72196792463811,98.7649263351046));
#33606=CARTESIAN_POINT('Ctrl Pts',(0.618262942848151,6.74118486718215,98.7735535374353));
#33607=CARTESIAN_POINT('Ctrl Pts',(0.43552110515076,6.75297048468067,98.782180739766));
#33608=CARTESIAN_POINT('Ctrl Pts',(0.252605233822827,6.76476732617599,98.7908161581865));
#33609=CARTESIAN_POINT('Ctrl Pts',(0.0693536736601038,6.76911870559685,
98.7994515766069));
#33610=CARTESIAN_POINT('Ctrl Pts',(-0.113620481361248,6.76604606740268,
98.8080869950274));
#33611=CARTESIAN_POINT('Ctrl Pts',(-0.296864954634215,6.76296888982324,
98.8167351710485));
#33612=CARTESIAN_POINT('Ctrl Pts',(-0.47983089916059,6.75244579019949,98.8253833470697));
#33613=CARTESIAN_POINT('Ctrl Pts',(-0.661909413332708,6.73455009102624,
98.8340315230909));
#33614=CARTESIAN_POINT('Ctrl Pts',(-0.681172629746129,6.73265679390873,
98.8349464673227));
#33615=CARTESIAN_POINT('Ctrl Pts',(-0.700425922149364,6.73068102372902,
98.8358614115545));
#33616=CARTESIAN_POINT('Ctrl Pts',(-0.71966857618888,6.72862290074621,98.8367763557863));
#33617=CARTESIAN_POINT('Ctrl Pts',(-0.892673578136568,6.7101189267144,98.8450023483276));
#33618=CARTESIAN_POINT('Ctrl Pts',(-1.06519153420927,6.68491397747257,98.853228340869));
#33619=CARTESIAN_POINT('Ctrl Pts',(-1.23666451091438,6.65304064976646,98.8614543334104));
#33620=CARTESIAN_POINT('Ctrl Pts',(-1.4079577203671,6.62120073712467,98.8696717020618));
#33621=CARTESIAN_POINT('Ctrl Pts',(-1.57820778268713,6.58270643249318,98.8778890707133));
#33622=CARTESIAN_POINT('Ctrl Pts',(-1.74686124829024,6.53764214218107,98.8861064393647));
#33623=CARTESIAN_POINT('Ctrl Pts',(-1.91537164936142,6.4926160787834,98.8943168374271));
#33624=CARTESIAN_POINT('Ctrl Pts',(-2.08228780689118,6.44103122136321,98.9025272354895));
#33625=CARTESIAN_POINT('Ctrl Pts',(-2.2470657452993,6.38302315022455,98.9107376335518));
#33626=CARTESIAN_POINT('Ctrl Pts',(-2.4117368687555,6.3250526819919,98.9189427093406));
#33627=CARTESIAN_POINT('Ctrl Pts',(-2.57427219729211,6.26066741249165,98.9271477851294));
#33628=CARTESIAN_POINT('Ctrl Pts',(-2.73414213310794,6.19005297198368,98.9353528609181));
#33629=CARTESIAN_POINT('Ctrl Pts',(-2.89394040928929,6.11947018348689,98.9435542588876));
#33630=CARTESIAN_POINT('Ctrl Pts',(-3.05107534594188,6.04266393121495,98.9517556568572));
#33631=CARTESIAN_POINT('Ctrl Pts',(-3.20503649257048,5.95986829395512,98.9599570548266));
#33632=CARTESIAN_POINT('Ctrl Pts',(-3.35898557968034,5.87707914193888,98.9681578103944));
#33633=CARTESIAN_POINT('Ctrl Pts',(-3.50976105251121,5.78830170128249,98.9763585659621));
#33634=CARTESIAN_POINT('Ctrl Pts',(-3.65687595058967,5.69381658310126,98.9845593215298));
#33635=CARTESIAN_POINT('Ctrl Pts',(-3.80399010139447,5.59933194485946,98.9927600354416));
#33636=CARTESIAN_POINT('Ctrl Pts',(-3.94744341236865,5.49913987960917,99.0009607493534));
#33637=CARTESIAN_POINT('Ctrl Pts',(-4.08677698325455,5.39356495178661,99.0091614632652));
#33638=CARTESIAN_POINT('Ctrl Pts',(-4.22613509710495,5.28797142742848,99.0173636216948));
#33639=CARTESIAN_POINT('Ctrl Pts',(-4.36137173944622,5.1769933678733,99.0255657801245));
#33640=CARTESIAN_POINT('Ctrl Pts',(-4.49206020250443,5.06099635813699,99.0337679385541));
#33641=CARTESIAN_POINT('Ctrl Pts',(-4.62279536998506,4.94495789429513,99.0419730282071));
#33642=CARTESIAN_POINT('Ctrl Pts',(-4.74897885245106,4.82389714499411,99.05017811786));
#33643=CARTESIAN_POINT('Ctrl Pts',(-4.87021995362528,4.69821738570175,99.058383207513));
#33644=CARTESIAN_POINT('Ctrl Pts',(-4.9915995584228,4.57239405214399,99.0665976705108));
#33645=CARTESIAN_POINT('Ctrl Pts',(-5.10802525297673,4.44194142491324,99.0748121335086));
#33646=CARTESIAN_POINT('Ctrl Pts',(-5.21914519615482,4.30729757753677,99.0830265965063));
#33647=CARTESIAN_POINT('Ctrl Pts',(-5.33033097438728,4.17257395793616,99.0912459263138));
#33648=CARTESIAN_POINT('Ctrl Pts',(-5.43620451819687,4.03365445283905,99.0994652561213));
#33649=CARTESIAN_POINT('Ctrl Pts',(-5.5364567655613,3.89100700115928,99.1076845859288));
#33650=CARTESIAN_POINT('Ctrl Pts',(-5.63686434770489,3.74813852590161,99.1159166510895));
#33651=CARTESIAN_POINT('Ctrl Pts',(-5.7316330332971,3.60153086166351,99.1241487162502));
#33652=CARTESIAN_POINT('Ctrl Pts',(-5.82049857341232,3.45167862885657,99.1323807814109));
#33653=CARTESIAN_POINT('Ctrl Pts',(-5.90037730176227,3.31698068203152,99.1397803526719));
#33654=CARTESIAN_POINT('Ctrl Pts',(-5.97548700482453,3.17966170855554,99.1471799239329));
#33655=CARTESIAN_POINT('Ctrl Pts',(-6.04566906188862,3.04009450414338,99.1545794951939));
#33656=CARTESIAN_POINT('Ctrl Pts',(-6.12835566695495,2.87566019152554,99.163297470302));
#33657=CARTESIAN_POINT('Ctrl Pts',(-6.20443031847366,2.7076506828572,99.1720154454101));
#33658=CARTESIAN_POINT('Ctrl Pts',(-6.27358858800675,2.53660703074629,99.1807334205182));
#33659=CARTESIAN_POINT('Ctrl Pts',(-6.34261135922391,2.36589849585226,99.1894343149365));
#33660=CARTESIAN_POINT('Ctrl Pts',(-6.40474465693939,2.19216793913221,99.1981352093549));
#33661=CARTESIAN_POINT('Ctrl Pts',(-6.45972999030447,2.01598051884464,99.2068361037733));
#33662=CARTESIAN_POINT('Ctrl Pts',(-6.51456218618164,1.84028379120709,99.215512765673));
#33663=CARTESIAN_POINT('Ctrl Pts',(-6.56228603910053,1.66214412621012,99.2241894275727));
#33664=CARTESIAN_POINT('Ctrl Pts',(-6.6026914331339,1.48214535009902,99.2328660894725));
#33665=CARTESIAN_POINT('Ctrl Pts',(-6.64302991800459,1.30244464229498,99.2415283832861));
#33666=CARTESIAN_POINT('Ctrl Pts',(-6.67607403775892,1.12089124316773,99.2501906770997));
#33667=CARTESIAN_POINT('Ctrl Pts',(-6.7016628272348,0.93808547055124,99.2588529709132));
#33668=CARTESIAN_POINT('Ctrl Pts',(-6.72719076008196,0.755714456407419,
99.2674946635961));
#33669=CARTESIAN_POINT('Ctrl Pts',(-6.74529868753324,0.572097297730524,
99.2761363562789));
#33670=CARTESIAN_POINT('Ctrl Pts',(-6.75587633535769,0.387845254391387,
99.2847780489617));
#33671=CARTESIAN_POINT('Ctrl Pts',(-6.76323768989523,0.259617822565879,
99.2907921047043));
#33672=CARTESIAN_POINT('Ctrl Pts',(-6.76695297056617,0.131083220982737,
99.296806160447));
#33673=CARTESIAN_POINT('Ctrl Pts',(-6.76699955621847,0.00245074255190249,
99.3028202161897));
#33674=CARTESIAN_POINT('Ctrl Pts',(-6.767,5.7588599325272E-12,99.3028202161897));
#33675=CARTESIAN_POINT('Ctrl Pts',(-6.76700000000016,-0.186007249409913,
99.3115697279957));
#33676=CARTESIAN_POINT('Ctrl Pts',(-6.7593263729547,-0.372014355521765,
99.3203192398016));
#33677=CARTESIAN_POINT('Ctrl Pts',(-6.74400518266976,-0.557389537149286,
99.3290687516076));
#33678=CARTESIAN_POINT('Ctrl Pts',(-6.72868405709709,-0.742763935805651,
99.3378182264581));
#33679=CARTESIAN_POINT('Ctrl Pts',(-6.7057154565307,-0.927506129689313,
99.3465677013087));
#33680=CARTESIAN_POINT('Ctrl Pts',(-6.67517739415745,-1.11098863924406,
99.3553171761592));
#33681=CARTESIAN_POINT('Ctrl Pts',(-6.64463945823175,-1.29447038906122,
99.3640666147812));
#33682=CARTESIAN_POINT('Ctrl Pts',(-6.60653217027237,-1.47669218227862,
99.3728160534032));
#33683=CARTESIAN_POINT('Ctrl Pts',(-6.56098496116795,-1.65703510503792,
99.3815654920252));
#33684=CARTESIAN_POINT('Ctrl Pts',(-6.51543793687602,-1.8373772960372,99.3903148951455));
#33685=CARTESIAN_POINT('Ctrl Pts',(-6.46245112202725,-2.01584035396781,
99.3990642982657));
#33686=CARTESIAN_POINT('Ctrl Pts',(-6.40220448416326,-2.19181813637899,
99.4078137013859));
#33687=CARTESIAN_POINT('Ctrl Pts',(-6.34195808575275,-2.36779521935709,
99.4165630697312));
#33688=CARTESIAN_POINT('Ctrl Pts',(-6.27445201489326,-2.54128677544603,
99.4253124380765));
#33689=CARTESIAN_POINT('Ctrl Pts',(-6.19991555136278,-2.71170355237626,
99.4340618064218));
#33690=CARTESIAN_POINT('Ctrl Pts',(-6.12537937789138,-2.88211966612859,
99.4428111407188));
#33691=CARTESIAN_POINT('Ctrl Pts',(-6.04381298133723,-3.04946076210234,
99.4515604750159));
#33692=CARTESIAN_POINT('Ctrl Pts',(-5.95549339426418,-3.21315848206647,
99.4603098093129));
#33693=CARTESIAN_POINT('Ctrl Pts',(-5.86717414355284,-3.37685557859421,
99.4690591102885));
#33694=CARTESIAN_POINT('Ctrl Pts',(-5.77210188986374,-3.5369090746709,99.4778084112641));
#33695=CARTESIAN_POINT('Ctrl Pts',(-5.67059953467216,-3.69277536784678,
99.4865577122396));
#33696=CARTESIAN_POINT('Ctrl Pts',(-5.56909755761921,-3.84864108035569,
99.4953069806204));
#33697=CARTESIAN_POINT('Ctrl Pts',(-5.46116568338232,-4.00031938104058,
99.5040562490011));
#33698=CARTESIAN_POINT('Ctrl Pts',(-5.34717048686283,-4.14729511663001,
99.5128055173819));
#33699=CARTESIAN_POINT('Ctrl Pts',(-5.23317570555686,-4.29427031687835,
99.5215547538945));
#33700=CARTESIAN_POINT('Ctrl Pts',(-5.11311782178972,-4.43654275986937,
99.5303039904071));
#33701=CARTESIAN_POINT('Ctrl Pts',(-4.98740459172179,-4.57362924147469,
99.5390532269198));
#33702=CARTESIAN_POINT('Ctrl Pts',(-4.86169180910972,-4.71071523514291,
99.5478024322909));
#33703=CARTESIAN_POINT('Ctrl Pts',(-4.73032391415547,-4.84261509316412,
99.5565516376621));
#33704=CARTESIAN_POINT('Ctrl Pts',(-4.59374707237381,-4.96888084331443,
99.5653008430332));
#33705=CARTESIAN_POINT('Ctrl Pts',(-4.45717070537491,-5.09514615452647,
99.5740500179894));
#33706=CARTESIAN_POINT('Ctrl Pts',(-4.31538563819599,-5.21577720253558,
99.5827991929456));
#33707=CARTESIAN_POINT('Ctrl Pts',(-4.16887341290739,-5.33036429028579,
99.5915483679019));
#33708=CARTESIAN_POINT('Ctrl Pts',(-4.02236168477423,-5.44495098921114,
99.6002975131698));
#33709=CARTESIAN_POINT('Ctrl Pts',(-3.87112305634517,-5.55349359238705,
99.6090466584377));
#33710=CARTESIAN_POINT('Ctrl Pts',(-3.71567117316803,-5.65562346102427,
99.6177958037056));
#33711=CARTESIAN_POINT('Ctrl Pts',(-3.56021980457389,-5.75775299158714,
99.6265449200118));
#33712=CARTESIAN_POINT('Ctrl Pts',(-3.40055544862494,-5.85346967275291,
99.635294036318));
#33713=CARTESIAN_POINT('Ctrl Pts',(-3.23722036323528,-5.94244842803493,
99.6440431526241));
#33714=CARTESIAN_POINT('Ctrl Pts',(-3.07388580496189,-6.03142689616402,
99.6527922406951));
#33715=CARTESIAN_POINT('Ctrl Pts',(-2.90688079257867,-6.11366734484746,
99.661541328766));
#33716=CARTESIAN_POINT('Ctrl Pts',(-2.73677251094793,-6.18889046787223,
99.6702904168369));
#33717=CARTESIAN_POINT('Ctrl Pts',(-2.56666476416847,-6.26411335438187,
99.6790394773992));
#33718=CARTESIAN_POINT('Ctrl Pts',(-2.39345402972319,-6.33231884350204,
99.6877885379614));
#33719=CARTESIAN_POINT('Ctrl Pts',(-2.2177285647429,-6.39327529620956,99.6965375985236));
#33720=CARTESIAN_POINT('Ctrl Pts',(-2.04200363768508,-6.45423156232007,
99.7052866323036));
#33721=CARTESIAN_POINT('Ctrl Pts',(-1.86376426620317,-6.50793874251992,
99.7140356660836));
#33722=CARTESIAN_POINT('Ctrl Pts',(-1.68361578194898,-6.55421443796069,
99.7227846998636));
#33723=CARTESIAN_POINT('Ctrl Pts',(-1.50346783420054,-6.60048999558638,
99.7315337075879));
#33724=CARTESIAN_POINT('Ctrl Pts',(-1.32141106257408,-6.63933404145464,
99.7402827153121));
#33725=CARTESIAN_POINT('Ctrl Pts',(-1.13806375959181,-6.67061465527006,
99.7490317230363));
#33726=CARTESIAN_POINT('Ctrl Pts',(-0.95471698742034,-6.70189517852464,
99.7577807054312));
#33727=CARTESIAN_POINT('Ctrl Pts',(-0.770079973810876,-6.72561226535817,
99.7665296878261));
#33728=CARTESIAN_POINT('Ctrl Pts',(-0.584779770553267,-6.74168536939775,
99.775278670221));
#33729=CARTESIAN_POINT('Ctrl Pts',(-0.391490647554711,-6.75845143942389,
99.7844048508971));
#33730=CARTESIAN_POINT('Ctrl Pts',(-0.197480213105126,-6.76689975924024,
99.7935310315731));
#33731=CARTESIAN_POINT('Ctrl Pts',(-0.00346532629857358,-6.76699911271707,
99.8026572122492));
#33732=CARTESIAN_POINT('Ctrl Pts',(0.184486595295242,-6.76709536139775,
99.8114981997791));
#33733=CARTESIAN_POINT('Ctrl Pts',(0.372442378184379,-6.75935659726775,
99.820339187309));
#33734=CARTESIAN_POINT('Ctrl Pts',(0.559750217721202,-6.74380965729024,
99.829180174839));
#33735=CARTESIAN_POINT('Ctrl Pts',(0.745129914456873,-6.72842275717263,
99.8379301534367));
#33736=CARTESIAN_POINT('Ctrl Pts',(0.929874656313306,-6.70538772273485,
99.8466801320345));
#33737=CARTESIAN_POINT('Ctrl Pts',(1.1133568828969,-6.67478280180757,99.8554301106323));
#33738=CARTESIAN_POINT('Ctrl Pts',(1.29683723118757,-6.64417819418043,99.8641799996572));
#33739=CARTESIAN_POINT('Ctrl Pts',(1.47905480730123,-6.606003902301,99.8729298886822));
#33740=CARTESIAN_POINT('Ctrl Pts',(1.65939064804684,-6.56038959797166,99.8816797777071));
#33741=CARTESIAN_POINT('Ctrl Pts',(1.83972470264148,-6.51477574543289,99.8904295800681));
#33742=CARTESIAN_POINT('Ctrl Pts',(2.01817678125737,-6.46172209820135,99.899179382429));
#33743=CARTESIAN_POINT('Ctrl Pts',(2.19414072347575,-6.4014088672405,99.9079291847899));
#33744=CARTESIAN_POINT('Ctrl Pts',(2.37010298132,-6.34109621361411,99.9166789033954));
#33745=CARTESIAN_POINT('Ctrl Pts',(2.54357687926824,-6.27352420826007,99.9254286220009));
#33746=CARTESIAN_POINT('Ctrl Pts',(2.71397317789891,-6.19892237325532,99.9341783406064));
#33747=CARTESIAN_POINT('Ctrl Pts',(2.88436790207115,-6.12432122757004,99.9429279783647));
#33748=CARTESIAN_POINT('Ctrl Pts',(3.05168482126165,-6.04269049717463,99.9516776161229));
#33749=CARTESIAN_POINT('Ctrl Pts',(3.21535561997292,-5.95430745234982,99.9604272538812));
#33750=CARTESIAN_POINT('Ctrl Pts',(3.37902496075184,-5.86592519481572,99.9691768137002));
#33751=CARTESIAN_POINT('Ctrl Pts',(3.53904799384779,-5.77079087940291,99.9779263735192));
#33752=CARTESIAN_POINT('Ctrl Pts',(3.69488118814889,-5.66922763747086,99.9866759333382));
#33753=CARTESIAN_POINT('Ctrl Pts',(3.85071304610742,-5.56766526649115,99.9954254181257));
#33754=CARTESIAN_POINT('Ctrl Pts',(4.00235489705881,-5.45967423580778,100.004174902913));
#33755=CARTESIAN_POINT('Ctrl Pts',(4.14929168607571,-5.34562133936393,100.012924387701));
#33756=CARTESIAN_POINT('Ctrl Pts',(4.29622726385676,-5.23156938308597,100.021673800364));
#33757=CARTESIAN_POINT('Ctrl Pts',(4.43845763091988,-5.11145583677271,100.030423213027));
#33758=CARTESIAN_POINT('Ctrl Pts',(4.57549970660886,-4.98568866204282,100.03917262569));
#33759=CARTESIAN_POINT('Ctrl Pts',(4.71254069815223,-4.85992248226231,100.047921969137));
#33760=CARTESIAN_POINT('Ctrl Pts',(4.84439326931247,-4.72850295734071,100.056671312583));
#33761=CARTESIAN_POINT('Ctrl Pts',(4.97060959434635,-4.59187644221749,100.065420656029));
#33762=CARTESIAN_POINT('Ctrl Pts',(5.09682496280459,-4.45525096256728,100.074169933166));
#33763=CARTESIAN_POINT('Ctrl Pts',(5.2174039761579,-4.31341878218386,100.082919210302));
#33764=CARTESIAN_POINT('Ctrl Pts',(5.3319371045189,-4.16686161438733,100.091668487438));
#33765=CARTESIAN_POINT('Ctrl Pts',(5.44646940289338,-4.02030550864575,100.100417701171));
#33766=CARTESIAN_POINT('Ctrl Pts',(5.55495572749618,-3.869024709802,100.109166914904));
#33767=CARTESIAN_POINT('Ctrl Pts',(5.65702762491408,-3.71353301465854,100.117916128637));
#33768=CARTESIAN_POINT('Ctrl Pts',(5.7590988165511,-3.55804239466964,100.126665281873));
#33769=CARTESIAN_POINT('Ctrl Pts',(5.85475551250742,-3.39834117619623,100.135414435109));
#33770=CARTESIAN_POINT('Ctrl Pts',(5.94367283728058,-3.23497174692037,100.144163588346));
#33771=CARTESIAN_POINT('Ctrl Pts',(6.03258957676285,-3.0716033930102,100.152912683991));
#33772=CARTESIAN_POINT('Ctrl Pts',(6.11476689685266,-2.90456712829543,100.161661779637));
#33773=CARTESIAN_POINT('Ctrl Pts',(6.1899257052525,-2.73443024475929,100.170410875282));
#33774=CARTESIAN_POINT('Ctrl Pts',(6.2650840438869,-2.56429442463048,100.179159916243));
#33775=CARTESIAN_POINT('Ctrl Pts',(6.33322384283311,-2.39105828656004,100.187908957204));
#33776=CARTESIAN_POINT('Ctrl Pts',(6.39411368720031,-2.21531017132087,100.196657998165));
#33777=CARTESIAN_POINT('Ctrl Pts',(6.45500317120883,-2.03956309619536,100.205406987348));
#33778=CARTESIAN_POINT('Ctrl Pts',(6.50864269270062,-1.8613043443867,100.21415597653));
#33779=CARTESIAN_POINT('Ctrl Pts',(6.5548500844632,-1.68113930719997,100.222904965713));
#33780=CARTESIAN_POINT('Ctrl Pts',(6.60199664749393,-1.49731239211887,100.231831779242));
#33781=CARTESIAN_POINT('Ctrl Pts',(6.64140563640898,-1.31150116499713,100.240758592771));
#33782=CARTESIAN_POINT('Ctrl Pts',(6.67293772282166,-1.12436255155696,100.249685406301));
#33783=CARTESIAN_POINT('Ctrl Pts',(6.70384494949865,-0.940932395051767,
100.258435320456));
#33784=CARTESIAN_POINT('Ctrl Pts',(6.72718449348925,-0.756227260507198,
100.267185234612));
#33785=CARTESIAN_POINT('Ctrl Pts',(6.74287707373928,-0.570874564542234,
100.275935148767));
#33786=CARTESIAN_POINT('Ctrl Pts',(6.75856934538666,-0.385525513633097,
100.284684890851));
#33787=CARTESIAN_POINT('Ctrl Pts',(6.76661493004101,-0.199529212418929,
100.293434632935));
#33788=CARTESIAN_POINT('Ctrl Pts',(6.76698649908906,-0.0135174386012057,
100.302184375019));
#33789=CARTESIAN_POINT('Ctrl Pts',(6.76735806132391,0.17249092444508,100.310933956665));
#33790=CARTESIAN_POINT('Ctrl Pts',(6.76005588896293,0.35851447290079,100.319683538311));
#33791=CARTESIAN_POINT('Ctrl Pts',(6.74510478454589,0.543921359661676,100.328433119957));
#33792=CARTESIAN_POINT('Ctrl Pts',(6.73015393440693,0.729325093149969,100.337182552796));
#33793=CARTESIAN_POINT('Ctrl Pts',(6.70755443556903,0.914111900255936,100.345931985635));
#33794=CARTESIAN_POINT('Ctrl Pts',(6.67738304682325,1.09765415591502,100.354681418474));
#33795=CARTESIAN_POINT('Ctrl Pts',(6.64721213111866,1.28119353391246,100.363430714135));
#33796=CARTESIAN_POINT('Ctrl Pts',(6.60946960955499,1.46348811672634,100.372180009797));
#33797=CARTESIAN_POINT('Ctrl Pts',(6.56428366991186,1.64391876348211,100.380929305458));
#33798=CARTESIAN_POINT('Ctrl Pts',(6.51909837867721,1.82434682109703,100.389678475569));
#33799=CARTESIAN_POINT('Ctrl Pts',(6.46646995271926,2.0029107182043,100.39842764568));
#33800=CARTESIAN_POINT('Ctrl Pts',(6.40657713281555,2.17900400212686,100.40717681579));
#33801=CARTESIAN_POINT('Ctrl Pts',(6.34668509279062,2.35509499309652,100.415925871976));
#33802=CARTESIAN_POINT('Ctrl Pts',(6.27952894037524,2.52871516398128,100.424674928162));
#33803=CARTESIAN_POINT('Ctrl Pts',(6.2053367506144,2.69927486771436,100.433423984348));
#33804=CARTESIAN_POINT('Ctrl Pts',(6.12832117907908,2.87632521635941,100.44250598563));
#33805=CARTESIAN_POINT('Ctrl Pts',(6.0437236662607,3.05007728920016,100.451587986912));
#33806=CARTESIAN_POINT('Ctrl Pts',(5.95185378007857,3.21989527478216,100.460669988195));
#33807=CARTESIAN_POINT('Ctrl Pts',(5.86334450817362,3.38350129286768,100.469419768502));
#33808=CARTESIAN_POINT('Ctrl Pts',(5.76808562057248,3.54345567124974,100.478169548809));
#33809=CARTESIAN_POINT('Ctrl Pts',(5.66640068804479,3.69921508465317,100.486919329116));
#33810=CARTESIAN_POINT('Ctrl Pts',(5.56471941107921,3.85496889852286,100.495668794869));
#33811=CARTESIAN_POINT('Ctrl Pts',(5.45661270815116,4.00652780919634,100.504418260623));
#33812=CARTESIAN_POINT('Ctrl Pts',(5.3424477644912,4.15337704569221,100.513167726376));
#33813=CARTESIAN_POINT('Ctrl Pts',(5.22828631819602,4.30022178356241,100.521916924096));
#33814=CARTESIAN_POINT('Ctrl Pts',(5.10806717844077,4.4423569097267,100.530666121816));
#33815=CARTESIAN_POINT('Ctrl Pts',(4.98219864544728,4.57929969070635,100.539415319535));
#33816=CARTESIAN_POINT('Ctrl Pts',(4.85633329944035,4.7162390042999,100.548164295725));
#33817=CARTESIAN_POINT('Ctrl Pts',(4.7248190403366,4.84798602483605,100.556913271916));
#33818=CARTESIAN_POINT('Ctrl Pts',(4.58810250737212,4.97409332259114,100.565662248106));
#33819=CARTESIAN_POINT('Ctrl Pts',(4.45137708685659,5.1002088182212,100.574411793042));
#33820=CARTESIAN_POINT('Ctrl Pts',(4.30944892636073,5.22068366307915,100.583161337978));
#33821=CARTESIAN_POINT('Ctrl Pts',(4.16280009466687,5.3351086560483,100.591910882914));
#33822=CARTESIAN_POINT('Ctrl Pts',(4.01615988348822,5.44952692272866,100.600659913523));
#33823=CARTESIAN_POINT('Ctrl Pts',(3.86479978232272,5.55789587288597,100.609408944131));
#33824=CARTESIAN_POINT('Ctrl Pts',(3.70923383581116,5.65984746713846,100.618157974739));
#33825=CARTESIAN_POINT('Ctrl Pts',(3.55366577799593,5.7618004450535,100.626907124087));
#33826=CARTESIAN_POINT('Ctrl Pts',(3.39389200026896,5.85733573571026,100.635656273435));
#33827=CARTESIAN_POINT('Ctrl Pts',(3.23045513626101,5.94612887621895,100.644405422783));
#33828=CARTESIAN_POINT('Ctrl Pts',(3.18695122151616,5.96976399206668,100.646734286896));
#33829=CARTESIAN_POINT('Ctrl Pts',(3.14318791262679,5.99292165435326,100.649063151009));
#33830=CARTESIAN_POINT('Ctrl Pts',(3.0991757505325,6.01559628526644,100.651392015122));
#33831=CARTESIAN_POINT('Origin',(0.,0.,-3.69717978381041));
#33832=CARTESIAN_POINT('',(3.09917575053265,6.01559628526636,103.045648009871));
#33833=CARTESIAN_POINT('',(3.09917575053253,6.01559628526642,102.651329234227));
#33834=CARTESIAN_POINT('',(3.09917575053259,6.01559628526639,-3.69717978381041));
#33835=CARTESIAN_POINT('',(-6.76699833621906,-0.00474527222232697,101.69717978384));
#33836=CARTESIAN_POINT('Ctrl Pts',(-6.76699833621906,-0.00474527222232863,
101.69717978384));
#33837=CARTESIAN_POINT('Ctrl Pts',(-6.76685764347592,-0.20538024407743,
101.70658487248));
#33838=CARTESIAN_POINT('Ctrl Pts',(-6.75778988930074,-0.405671385327906,
101.715989961121));
#33839=CARTESIAN_POINT('Ctrl Pts',(-6.73991149079066,-0.604881886245581,
101.725395049761));
#33840=CARTESIAN_POINT('Ctrl Pts',(-6.72212131116182,-0.80310940608071,
101.734753730083));
#33841=CARTESIAN_POINT('Ctrl Pts',(-6.69560740036752,-1.0002668010555,101.744112410406));
#33842=CARTESIAN_POINT('Ctrl Pts',(-6.6605344896149,-1.19564598132158,101.753471090728));
#33843=CARTESIAN_POINT('Ctrl Pts',(-6.62520069676219,-1.39247844646671,
101.762899383527));
#33844=CARTESIAN_POINT('Ctrl Pts',(-6.58118016988564,-1.58750599058811,
101.772327676326));
#33845=CARTESIAN_POINT('Ctrl Pts',(-6.52869054886016,-1.78002492039412,
101.781755969125));
#33846=CARTESIAN_POINT('Ctrl Pts',(-6.47620092783464,-1.97254385020025,
101.791184261924));
#33847=CARTESIAN_POINT('Ctrl Pts',(-6.41524233215604,-2.16255404287778,
101.800612554723));
#33848=CARTESIAN_POINT('Ctrl Pts',(-6.34607992290035,-2.3493740894462,101.810040847522));
#33849=CARTESIAN_POINT('Ctrl Pts',(-6.28574552961825,-2.51234808477026,
101.818265695844));
#33850=CARTESIAN_POINT('Ctrl Pts',(-6.21904440781394,-2.67322514300025,
101.826490544166));
#33851=CARTESIAN_POINT('Ctrl Pts',(-6.1461413664766,-2.83147228545241,101.834715392488));
#33852=CARTESIAN_POINT('Ctrl Pts',(-6.07332043012784,-2.9895412065357,101.842930977807));
#33853=CARTESIAN_POINT('Ctrl Pts',(-5.99431163138863,-3.14498578679159,
101.851146563126));
#33854=CARTESIAN_POINT('Ctrl Pts',(-5.90932902089302,-3.29728972382343,
101.859362148446));
#33855=CARTESIAN_POINT('Ctrl Pts',(-5.82442504496082,-3.44945273374648,
101.867570131869));
#33856=CARTESIAN_POINT('Ctrl Pts',(-5.73355843927315,-3.59848057656376,
101.875778115292));
#33857=CARTESIAN_POINT('Ctrl Pts',(-5.63699069137025,-3.74387832940724,
101.883986098715));
#33858=CARTESIAN_POINT('Ctrl Pts',(-5.54049290165615,-3.88917074932472,
101.892188135892));
#33859=CARTESIAN_POINT('Ctrl Pts',(-5.43830239394184,-4.03083801969773,
101.900390173068));
#33860=CARTESIAN_POINT('Ctrl Pts',(-5.33072583250882,-4.1684111000024,101.908592210245));
#33861=CARTESIAN_POINT('Ctrl Pts',(-5.22320560223558,-4.3059121418345,101.916789952524));
#33862=CARTESIAN_POINT('Ctrl Pts',(-5.11030515729286,-4.43932298258219,
101.924987694804));
#33863=CARTESIAN_POINT('Ctrl Pts',(-4.99237364538065,-4.56820472230708,
101.933185437083));
#33864=CARTESIAN_POINT('Ctrl Pts',(-4.87446455619357,-4.69706195730227,
101.941381620697));
#33865=CARTESIAN_POINT('Ctrl Pts',(-4.75152654276489,-4.82139153791958,
101.949577804312));
#33866=CARTESIAN_POINT('Ctrl Pts',(-4.62394829350515,-4.94078851793829,
101.957773987926));
#33867=CARTESIAN_POINT('Ctrl Pts',(-4.49637943578457,-5.0601767086734,101.965969568187));
#33868=CARTESIAN_POINT('Ctrl Pts',(-4.36417128388756,-5.17463277610796,
101.974165148448));
#33869=CARTESIAN_POINT('Ctrl Pts',(-4.22774851464978,-5.28378950156765,
101.982360728709));
#33870=CARTESIAN_POINT('Ctrl Pts',(-4.09131096752224,-5.39295805134425,
101.990557196749));
#33871=CARTESIAN_POINT('Ctrl Pts',(-3.95065817371479,-5.49682589124071,
101.99875366479));
#33872=CARTESIAN_POINT('Ctrl Pts',(-3.80624696209212,-5.59506685067878,
102.006950132831));
#33873=CARTESIAN_POINT('Ctrl Pts',(-3.66179383321541,-5.69333632584778,
102.015148980004));
#33874=CARTESIAN_POINT('Ctrl Pts',(-3.51358041014197,-5.78597546549938,
102.023347827178));
#33875=CARTESIAN_POINT('Ctrl Pts',(-3.36209152494934,-5.87270206786142,
102.031546674351));
#33876=CARTESIAN_POINT('Ctrl Pts',(-3.21044431914049,-5.95951930795647,
102.039754090117));
#33877=CARTESIAN_POINT('Ctrl Pts',(-3.05551512397921,-6.04041148705646,
102.047961505883));
#33878=CARTESIAN_POINT('Ctrl Pts',(-2.89781323524833,-6.11514247206225,
102.056168921649));
#33879=CARTESIAN_POINT('Ctrl Pts',(-2.74002682385167,-6.18991351024763,
102.064380736301));
#33880=CARTESIAN_POINT('Ctrl Pts',(-2.57946508603522,-6.25851663050186,
102.072592550953));
#33881=CARTESIAN_POINT('Ctrl Pts',(-2.41665610906984,-6.32076437232835,
102.080804365605));
#33882=CARTESIAN_POINT('Ctrl Pts',(-2.25360737113515,-6.38310378341778,
102.089028273403));
#33883=CARTESIAN_POINT('Ctrl Pts',(-2.08830512018977,-6.43906899678869,
102.097252181201));
#33884=CARTESIAN_POINT('Ctrl Pts',(-1.92129261856777,-6.4885224569109,102.105476088998));
#33885=CARTESIAN_POINT('Ctrl Pts',(-1.76697615150164,-6.53421654074378,
102.113074827922));
#33886=CARTESIAN_POINT('Ctrl Pts',(-1.61119992339602,-6.5743517779,102.120673566845));
#33887=CARTESIAN_POINT('Ctrl Pts',(-1.45439827161408,-6.60885880220829,
102.128272305769));
#33888=CARTESIAN_POINT('Ctrl Pts',(-1.28620095868867,-6.64587364675711,
102.136423287943));
#33889=CARTESIAN_POINT('Ctrl Pts',(-1.11632544544517,-6.67652144097375,
102.144574270118));
#33890=CARTESIAN_POINT('Ctrl Pts',(-0.94529939735952,-6.70064907672024,
102.152725252292));
#33891=CARTESIAN_POINT('Ctrl Pts',(-0.774472011879651,-6.72474868598162,
102.160866766345));
#33892=CARTESIAN_POINT('Ctrl Pts',(-0.602497110271949,-6.74234316237416,
102.169008280398));
#33893=CARTESIAN_POINT('Ctrl Pts',(-0.429915582250584,-6.75332966707077,
102.177149794451));
#33894=CARTESIAN_POINT('Ctrl Pts',(-0.257498206185753,-6.76430572188747,
102.185283564654));
#33895=CARTESIAN_POINT('Ctrl Pts',(-0.0844757148706075,-6.76868629486567,
102.193417334857));
#33896=CARTESIAN_POINT('Ctrl Pts',(0.0886027882839978,-6.76641992089674,
102.20155110506));
#33897=CARTESIAN_POINT('Ctrl Pts',(0.261553068752986,-6.76415522593793,
102.209678849478));
#33898=CARTESIAN_POINT('Ctrl Pts',(0.434558914306283,-6.75525339383574,
102.217806593896));
#33899=CARTESIAN_POINT('Ctrl Pts',(0.607068105430911,-6.7397149283459,102.225934338314));
#33900=CARTESIAN_POINT('Ctrl Pts',(0.779485764393722,-6.72418470745641,
102.234057770208));
#33901=CARTESIAN_POINT('Ctrl Pts',(0.951406930313782,-6.70202489875823,
102.242181202102));
#33902=CARTESIAN_POINT('Ctrl Pts',(1.12228140005599,-6.67328805455664,102.250304633996));
#33903=CARTESIAN_POINT('Ctrl Pts',(1.29423983022416,-6.64436891511851,102.258479597747));
#33904=CARTESIAN_POINT('Ctrl Pts',(1.46513786356506,-6.60878901859909,102.266654561498));
#33905=CARTESIAN_POINT('Ctrl Pts',(1.63442152863352,-6.56665480033322,102.274829525249));
#33906=CARTESIAN_POINT('Ctrl Pts',(1.80259993569434,-6.52479567761254,102.282951114422));
#33907=CARTESIAN_POINT('Ctrl Pts',(1.96918463951716,-6.47646768023862,102.291072703595));
#33908=CARTESIAN_POINT('Ctrl Pts',(2.13364451927077,-6.42182606938134,102.299194292768));
#33909=CARTESIAN_POINT('Ctrl Pts',(2.29812611110159,-6.36717724471073,102.307316954157));
#33910=CARTESIAN_POINT('Ctrl Pts',(2.46048197276391,-6.30621326172673,102.315439615547));
#33911=CARTESIAN_POINT('Ctrl Pts',(2.62019808385182,-6.23913864258355,102.323562276936));
#33912=CARTESIAN_POINT('Ctrl Pts',(2.77996569541401,-6.17204239522343,102.331687557478));
#33913=CARTESIAN_POINT('Ctrl Pts',(2.93709152416275,-6.09883172971941,102.339812838021));
#33914=CARTESIAN_POINT('Ctrl Pts',(3.09108343974382,-6.01975848091446,102.347938118563));
#33915=CARTESIAN_POINT('Ctrl Pts',(3.24675306529124,-5.93982374547177,102.356151922351));
#33916=CARTESIAN_POINT('Ctrl Pts',(3.39921974923869,-5.85389811051584,102.364365726138));
#33917=CARTESIAN_POINT('Ctrl Pts',(3.54800332959427,-5.76228785927846,102.372579529926));
#33918=CARTESIAN_POINT('Ctrl Pts',(3.69543809982491,-5.67150810851784,102.380718870781));
#33919=CARTESIAN_POINT('Ctrl Pts',(3.83925600355025,-5.57514664295843,102.388858211636));
#33920=CARTESIAN_POINT('Ctrl Pts',(3.9790218042045,-5.47354313782811,102.396997552492));
#33921=CARTESIAN_POINT('Ctrl Pts',(4.12070558044972,-5.37054534996278,102.405248587746));
#33922=CARTESIAN_POINT('Ctrl Pts',(4.25822492660954,-5.2621608514902,102.413499623));
#33923=CARTESIAN_POINT('Ctrl Pts',(4.39116410387866,-5.14878304192433,102.421750658254));
#33924=CARTESIAN_POINT('Ctrl Pts',(4.52410328114777,-5.03540523235846,102.430001693508));
#33925=CARTESIAN_POINT('Ctrl Pts',(4.65246205279082,-4.917034421242,102.438252728762));
#33926=CARTESIAN_POINT('Ctrl Pts',(4.7758664037268,-4.79409940382484,102.446503764016));
#33927=CARTESIAN_POINT('Ctrl Pts',(4.89898264953621,-4.67145139580793,102.454735536047));
#33928=CARTESIAN_POINT('Ctrl Pts',(5.01755205440472,-4.54387770935175,102.462967308077));
#33929=CARTESIAN_POINT('Ctrl Pts',(5.13115663596937,-4.41174801831967,102.471199080108));
#33930=CARTESIAN_POINT('Ctrl Pts',(5.24462556231068,-4.27977610334292,102.479421022581));
#33931=CARTESIAN_POINT('Ctrl Pts',(5.35314123905025,-4.1432592857504,102.487642965053));
#33932=CARTESIAN_POINT('Ctrl Pts',(5.45632110349104,-4.00260527851527,102.495864907526));
#33933=CARTESIAN_POINT('Ctrl Pts',(5.55939843385556,-3.86209104495386,102.504078679515));
#33934=CARTESIAN_POINT('Ctrl Pts',(5.65715030118557,-3.71744809629668,102.512292451505));
#33935=CARTESIAN_POINT('Ctrl Pts',(5.74923310766844,-3.56911861300366,102.520506223495));
#33936=CARTESIAN_POINT('Ctrl Pts',(5.84124285057581,-3.42090682250058,102.528713478226));
#33937=CARTESIAN_POINT('Ctrl Pts',(5.92759230383383,-3.26901462657528,102.536920732956));
#33938=CARTESIAN_POINT('Ctrl Pts',(6.00798001085715,-3.11391476908745,102.545127987686));
#33939=CARTESIAN_POINT('Ctrl Pts',(6.0883200301798,-2.95890692013986,102.553330373698));
#33940=CARTESIAN_POINT('Ctrl Pts',(6.16270518422332,-2.80069551760968,102.56153275971));
#33941=CARTESIAN_POINT('Ctrl Pts',(6.23087893407393,-2.63977967052438,102.569735145722));
#33942=CARTESIAN_POINT('Ctrl Pts',(6.29903233571379,-2.47891185291634,102.577935083521));
#33943=CARTESIAN_POINT('Ctrl Pts',(6.360977882988,-2.31534152668179,102.586135021319));
#33944=CARTESIAN_POINT('Ctrl Pts',(6.41650624705025,-2.14958986357051,102.594334959118));
#33945=CARTESIAN_POINT('Ctrl Pts',(6.472026846814,-1.98386137681988,102.602533750354));
#33946=CARTESIAN_POINT('Ctrl Pts',(6.52113193584389,-1.81595250013607,102.61073254159));
#33947=CARTESIAN_POINT('Ctrl Pts',(6.56366134678883,-1.64640175068854,102.618931332825));
#33948=CARTESIAN_POINT('Ctrl Pts',(6.60619252608039,-1.47684395142562,102.627130464962));
#33949=CARTESIAN_POINT('Ctrl Pts',(6.64214739529731,-1.30564449104982,102.635329597098));
#33950=CARTESIAN_POINT('Ctrl Pts',(6.67141640530415,-1.13335437840009,102.643528729235));
#33951=CARTESIAN_POINT('Ctrl Pts',(6.70069194182912,-0.961025847828328,
102.651729689645));
#33952=CARTESIAN_POINT('Ctrl Pts',(6.72327858980431,-0.787606533896339,
102.659930650056));
#33953=CARTESIAN_POINT('Ctrl Pts',(6.739118383539,-0.613654962211398,102.668131610467));
#33954=CARTESIAN_POINT('Ctrl Pts',(6.75497302297354,-0.43954035602845,102.676340257152));
#33955=CARTESIAN_POINT('Ctrl Pts',(6.7640681418017,-0.264892852834303,102.684548903837));
#33956=CARTESIAN_POINT('Ctrl Pts',(6.76639782620604,-0.090274345825458,
102.692757550522));
#33957=CARTESIAN_POINT('Ctrl Pts',(6.76872862286714,0.0844275289629238,
102.700970116246));
#33958=CARTESIAN_POINT('Ctrl Pts',(6.76428755412174,0.25910002184057,102.709182681969));
#33959=CARTESIAN_POINT('Ctrl Pts',(6.75312080457621,0.433184024174481,102.717395247693));
#33960=CARTESIAN_POINT('Ctrl Pts',(6.74193873263893,0.60750689488003,102.725619082242));
#33961=CARTESIAN_POINT('Ctrl Pts',(6.72401257287093,0.781239304562182,102.73384291679));
#33962=CARTESIAN_POINT('Ctrl Pts',(6.69944024760741,0.953828794248695,102.742066751339));
#33963=CARTESIAN_POINT('Ctrl Pts',(6.67686290296134,1.11240606966546,102.749622908314));
#33964=CARTESIAN_POINT('Ctrl Pts',(6.64867539778419,1.27001837395876,102.757179065288));
#33965=CARTESIAN_POINT('Ctrl Pts',(6.61499105796768,1.42624763032497,102.764735222263));
#33966=CARTESIAN_POINT('Ctrl Pts',(6.57644960021108,1.60500438546353,102.773380940315));
#33967=CARTESIAN_POINT('Ctrl Pts',(6.53062364198936,1.78235784131071,102.782026658367));
#33968=CARTESIAN_POINT('Ctrl Pts',(6.4776287391073,1.9577065454994,102.79067237642));
#33969=CARTESIAN_POINT('Ctrl Pts',(6.42470187088049,2.13283013768694,102.799306995132));
#33970=CARTESIAN_POINT('Ctrl Pts',(6.36462449798613,2.30595381975003,102.807941613845));
#33971=CARTESIAN_POINT('Ctrl Pts',(6.29756288745097,2.4764875688362,102.816576232557));
#33972=CARTESIAN_POINT('Ctrl Pts',(6.22813292134587,2.65304390746782,102.825515792459));
#33973=CARTESIAN_POINT('Ctrl Pts',(6.15121644127757,2.82682372174258,102.834455352362));
#33974=CARTESIAN_POINT('Ctrl Pts',(6.06705486922959,2.99718771747075,102.843394912264));
#33975=CARTESIAN_POINT('Ctrl Pts',(5.98598979180754,3.1612836363987,102.852005565535));
#33976=CARTESIAN_POINT('Ctrl Pts',(5.89820335204383,3.32221027235961,102.860616218805));
#33977=CARTESIAN_POINT('Ctrl Pts',(5.80396090812787,3.47941471758161,102.869226872076));
#33978=CARTESIAN_POINT('Ctrl Pts',(5.70980767099022,3.63647035827869,102.877829374787));
#33979=CARTESIAN_POINT('Ctrl Pts',(5.60921076977305,3.78981057203066,102.886431877498));
#33980=CARTESIAN_POINT('Ctrl Pts',(5.50248177629145,3.93890635856967,102.895034380209));
#33981=CARTESIAN_POINT('Ctrl Pts',(5.39587290414377,4.08783434080192,102.903627200977));
#33982=CARTESIAN_POINT('Ctrl Pts',(5.28314588526197,4.23252717835655,102.912220021744));
#33983=CARTESIAN_POINT('Ctrl Pts',(5.16465606807672,4.37248404210677,102.920812842512));
#33984=CARTESIAN_POINT('Ctrl Pts',(5.15069150491236,4.38897859421726,102.92182554547));
#33985=CARTESIAN_POINT('Ctrl Pts',(5.13664694788962,4.40540739793204,102.922838248428));
#33986=CARTESIAN_POINT('Ctrl Pts',(5.12252301818374,4.42176966023534,102.923850951386));
#33987=CARTESIAN_POINT('Ctrl Pts',(5.00267607501209,4.56060971121688,102.932444123144));
#33988=CARTESIAN_POINT('Ctrl Pts',(4.87725181832151,4.69449267907582,102.941037294903));
#33989=CARTESIAN_POINT('Ctrl Pts',(4.74668977369564,4.82298923825186,102.949630466662));
#33990=CARTESIAN_POINT('Ctrl Pts',(4.61591887935909,4.9516913431459,102.958237384233));
#33991=CARTESIAN_POINT('Ctrl Pts',(4.47999398472752,5.07498959902972,102.966844301804));
#33992=CARTESIAN_POINT('Ctrl Pts',(4.33938998624165,5.19249299925438,102.975451219376));
#33993=CARTESIAN_POINT('Ctrl Pts',(4.19867056023672,5.31009286278104,102.984065202715));
#33994=CARTESIAN_POINT('Ctrl Pts',(4.05326460314171,5.42188818637733,102.992679186054));
#33995=CARTESIAN_POINT('Ctrl Pts',(3.90367773266319,5.52753011384918,103.001293169392));
#33996=CARTESIAN_POINT('Ctrl Pts',(3.75385609914769,5.63333783675246,103.009920671597));
#33997=CARTESIAN_POINT('Ctrl Pts',(3.59984068853573,5.73297268666424,103.018548173802));
#33998=CARTESIAN_POINT('Ctrl Pts',(3.44216516994388,5.82612975677895,103.027175676007));
#33999=CARTESIAN_POINT('Ctrl Pts',(3.32963221999344,5.89261591774023,103.033333120628));
#34000=CARTESIAN_POINT('Ctrl Pts',(3.21523547777787,5.9558034608754,103.03949056525));
#34001=CARTESIAN_POINT('Ctrl Pts',(3.09917575053265,6.01559628526636,103.045648009871));
#34002=CARTESIAN_POINT('Ctrl Pts',(3.09917575053253,6.01559628526642,101.045648756765));
#34003=CARTESIAN_POINT('Ctrl Pts',(2.94379194180815,6.09564848777267,101.053851475175));
#34004=CARTESIAN_POINT('Ctrl Pts',(2.78535787451797,6.16964896183388,101.062054193584));
#34005=CARTESIAN_POINT('Ctrl Pts',(2.62438968426278,6.23737667494397,101.070256911994));
#34006=CARTESIAN_POINT('Ctrl Pts',(2.45542743074839,6.30846790740621,101.078866996914));
#34007=CARTESIAN_POINT('Ctrl Pts',(2.28367335026463,6.37264727895645,101.087477081833));
#34008=CARTESIAN_POINT('Ctrl Pts',(2.10974435081307,6.42971755011154,101.096087166753));
#34009=CARTESIAN_POINT('Ctrl Pts',(1.94376157595981,6.48418047462568,101.104303886168));
#34010=CARTESIAN_POINT('Ctrl Pts',(1.77579854635092,6.53216938358717,101.112520605583));
#34011=CARTESIAN_POINT('Ctrl Pts',(1.60640334848402,6.57356503595875,101.120737324999));
#34012=CARTESIAN_POINT('Ctrl Pts',(1.43688644648369,6.61499042956304,101.12895994782));
#34013=CARTESIAN_POINT('Ctrl Pts',(1.26593567524199,6.64981305445053,101.137182570642));
#34014=CARTESIAN_POINT('Ctrl Pts',(1.09410655370616,6.67796524767367,101.145405193464));
#34015=CARTESIAN_POINT('Ctrl Pts',(0.922046649230749,6.70615525198407,101.153638860054));
#34016=CARTESIAN_POINT('Ctrl Pts',(0.749106392946738,6.72765689459352,101.161872526645));
#34017=CARTESIAN_POINT('Ctrl Pts',(0.575844420042956,6.74245446435535,101.170106193235));
#34018=CARTESIAN_POINT('Ctrl Pts',(0.551492363644704,6.74453427013938,101.171263439166));
#34019=CARTESIAN_POINT('Ctrl Pts',(0.527133948188128,6.74648172474415,101.172420685098));
#34020=CARTESIAN_POINT('Ctrl Pts',(0.502770719782657,6.74829686686421,101.173577931029));
#34021=CARTESIAN_POINT('Ctrl Pts',(0.331108731698954,6.7610862599527,101.181731823195));
#34022=CARTESIAN_POINT('Ctrl Pts',(0.15867722880418,6.76734226510693,101.189885715362));
#34023=CARTESIAN_POINT('Ctrl Pts',(-0.0139804348075886,6.7669855583888,
101.198039607529));
#34024=CARTESIAN_POINT('Ctrl Pts',(-0.186427407832123,6.76662928695253,
101.206183549669));
#34025=CARTESIAN_POINT('Ctrl Pts',(-0.359099630619685,6.75967636665673,
101.214327491809));
#34026=CARTESIAN_POINT('Ctrl Pts',(-0.531447486644818,6.74609906308371,
101.22247143395));
#34027=CARTESIAN_POINT('Ctrl Pts',(-0.703621305920052,6.73253546986277,
101.230607152342));
#34028=CARTESIAN_POINT('Ctrl Pts',(-0.875471048730543,6.71236083894149,
101.238742870735));
#34029=CARTESIAN_POINT('Ctrl Pts',(-1.04644594997033,6.68559944012433,101.246878589128));
#34030=CARTESIAN_POINT('Ctrl Pts',(-1.21728416548072,6.65885943568313,101.255007803428));
#34031=CARTESIAN_POINT('Ctrl Pts',(-1.38724857241814,6.62554320435573,101.263137017728));
#34032=CARTESIAN_POINT('Ctrl Pts',(-1.5557923882042,6.58572691848105,101.271266232029));
#34033=CARTESIAN_POINT('Ctrl Pts',(-1.72423690021901,6.54593409183165,101.279390656704));
#34034=CARTESIAN_POINT('Ctrl Pts',(-1.89126213295922,6.49964892127365,101.28751508138));
#34035=CARTESIAN_POINT('Ctrl Pts',(-2.05633038219051,6.44699886453226,101.295639506055));
#34036=CARTESIAN_POINT('Ctrl Pts',(-2.22240070136559,6.39402918824172,101.303813251189));
#34037=CARTESIAN_POINT('Ctrl Pts',(-2.38648982816899,6.3346171530717,101.311986996323));
#34038=CARTESIAN_POINT('Ctrl Pts',(-2.54806399910648,6.26894399851024,101.320160741457));
#34039=CARTESIAN_POINT('Ctrl Pts',(-2.70860349633345,6.20369139561318,101.32828214432));
#34040=CARTESIAN_POINT('Ctrl Pts',(-2.86665981931489,6.13225778843294,101.336403547182));
#34041=CARTESIAN_POINT('Ctrl Pts',(-3.02172817996081,6.05486975965881,101.344524950044));
#34042=CARTESIAN_POINT('Ctrl Pts',(-3.17680852967557,5.97747574764993,101.35264698081));
#34043=CARTESIAN_POINT('Ctrl Pts',(-3.32890012940004,5.89412656043081,101.360769011576));
#34044=CARTESIAN_POINT('Ctrl Pts',(-3.47752182676671,5.80509525713068,101.368891042343));
#34045=CARTESIAN_POINT('Ctrl Pts',(-3.62618331578456,5.71604011678235,101.377015247684));
#34046=CARTESIAN_POINT('Ctrl Pts',(-3.77137273875985,5.62130001913802,101.385139453025));
#34047=CARTESIAN_POINT('Ctrl Pts',(-3.91263706047693,5.52119192140451,101.393263658366));
#34048=CARTESIAN_POINT('Ctrl Pts',(-4.05543047072851,5.42000022278301,101.401475802608));
#34049=CARTESIAN_POINT('Ctrl Pts',(-4.19421299676689,5.31332385652425,101.409687946851));
#34050=CARTESIAN_POINT('Ctrl Pts',(-4.32855089063314,5.20153209998737,101.417900091093));
#34051=CARTESIAN_POINT('Ctrl Pts',(-4.46166242758833,5.09076087897687,101.42603726751));
#34052=CARTESIAN_POINT('Ctrl Pts',(-4.59040991419057,4.97496756616058,101.434174443926));
#34053=CARTESIAN_POINT('Ctrl Pts',(-4.71440865088442,4.85454839016629,101.442311620343));
#34054=CARTESIAN_POINT('Ctrl Pts',(-4.84012098856856,4.73246508093375,101.450561248498));
#34055=CARTESIAN_POINT('Ctrl Pts',(-4.96095209377052,4.60562740212507,101.458810876654));
#34056=CARTESIAN_POINT('Ctrl Pts',(-5.07654374176494,4.47448238771226,101.467060504809));
#34057=CARTESIAN_POINT('Ctrl Pts',(-5.19213538975946,4.34333737329935,101.475310132964));
#34058=CARTESIAN_POINT('Ctrl Pts',(-5.30248738655973,4.20788536154887,101.48355976112));
#34059=CARTESIAN_POINT('Ctrl Pts',(-5.40728763516789,4.06860288435238,101.491809389275));
#34060=CARTESIAN_POINT('Ctrl Pts',(-5.51599389035984,3.92412921457607,101.500366489047));
#34061=CARTESIAN_POINT('Ctrl Pts',(-5.61906258002938,3.77508792084405,101.50892358882));
#34062=CARTESIAN_POINT('Ctrl Pts',(-5.71609298988985,3.62195664398846,101.517480688592));
#34063=CARTESIAN_POINT('Ctrl Pts',(-5.80982120828065,3.47403681369791,101.525746568509));
#34064=CARTESIAN_POINT('Ctrl Pts',(-5.89791512808572,3.32230111885043,101.534012448427));
#34065=CARTESIAN_POINT('Ctrl Pts',(-5.9800536091311,3.16721452256051,101.542278328344));
#34066=CARTESIAN_POINT('Ctrl Pts',(-6.06211347227962,3.01227636561197,101.550536296671));
#34067=CARTESIAN_POINT('Ctrl Pts',(-6.13822908460589,2.85399400400668,101.558794264997));
#34068=CARTESIAN_POINT('Ctrl Pts',(-6.2081229015865,2.6928607536962,101.567052233323));
#34069=CARTESIAN_POINT('Ctrl Pts',(-6.27796196947152,2.53185372198564,101.575303733033));
#34070=CARTESIAN_POINT('Ctrl Pts',(-6.34158880976767,2.36800057174501,101.583555232742));
#34071=CARTESIAN_POINT('Ctrl Pts',(-6.39877202886701,2.20181868522118,101.591806732452));
#34072=CARTESIAN_POINT('Ctrl Pts',(-6.45592039237351,2.03573809359239,101.600053202523));
#34073=CARTESIAN_POINT('Ctrl Pts',(-6.50663284512085,1.86733192623631,101.608299672594));
#34074=CARTESIAN_POINT('Ctrl Pts',(-6.55072626635181,1.69713711388575,101.616546142666));
#34075=CARTESIAN_POINT('Ctrl Pts',(-6.59480081166407,1.52701516010118,101.624789082512));
#34076=CARTESIAN_POINT('Ctrl Pts',(-6.63226188359202,1.35510642812366,101.633032022358));
#34077=CARTESIAN_POINT('Ctrl Pts',(-6.66297629917446,1.18196270526588,101.641274962204));
#34078=CARTESIAN_POINT('Ctrl Pts',(-6.6936832034107,1.00886132547147,101.649515886203));
#34079=CARTESIAN_POINT('Ctrl Pts',(-6.71764667896215,0.834525903982359,
101.657756810202));
#34080=CARTESIAN_POINT('Ctrl Pts',(-6.73478467878672,0.659518256289958,
101.665997734201));
#34081=CARTESIAN_POINT('Ctrl Pts',(-6.75192301453384,0.484507178266194,
101.67423881973));
#34082=CARTESIAN_POINT('Ctrl Pts',(-6.76223557122643,0.308824198567568,
101.68247990526));
#34083=CARTESIAN_POINT('Ctrl Pts',(-6.76569215398912,0.133036376416896,
101.690720990789));
#34084=CARTESIAN_POINT('Ctrl Pts',(-6.7665951641789,0.0871129296084177,
101.692873921796));
#34085=CARTESIAN_POINT('Ctrl Pts',(-6.76703054237299,0.0411823393665977,
101.695026852803));
#34086=CARTESIAN_POINT('Ctrl Pts',(-6.76699833621951,-0.00474527158081274,
101.69717978381));
#34087=CARTESIAN_POINT('',(-6.76699858504056,-0.0030292735211277,101.30282021619));
#34088=CARTESIAN_POINT('Ctrl Pts',(3.0991757505325,6.01559628526644,100.651392015122));
#34089=CARTESIAN_POINT('Ctrl Pts',(2.93382384459261,6.10078395293761,100.660141463035));
#34090=CARTESIAN_POINT('Ctrl Pts',(2.76495772122985,6.17915010267049,100.668890910947));
#34091=CARTESIAN_POINT('Ctrl Pts',(2.59315093316717,6.25042856433175,100.67764035886));
#34092=CARTESIAN_POINT('Ctrl Pts',(2.42134553245627,6.32170645041447,100.68638973612));
#34093=CARTESIAN_POINT('Ctrl Pts',(2.24659977927605,6.38589665313452,100.69513911338));
#34094=CARTESIAN_POINT('Ctrl Pts',(2.06950718689938,6.44278115439069,100.70388849064));
#34095=CARTESIAN_POINT('Ctrl Pts',(1.89241596572884,6.49966521519717,100.712637800154));
#34096=CARTESIAN_POINT('Ctrl Pts',(1.71297821457225,6.54924360009539,100.721387109669));
#34097=CARTESIAN_POINT('Ctrl Pts',(1.53180337335876,6.59134792173549,100.730136419183));
#34098=CARTESIAN_POINT('Ctrl Pts',(1.35062987477813,6.63345193135298,100.73888566386));
#34099=CARTESIAN_POINT('Ctrl Pts',(1.16771959102981,6.66808192368233,100.747634908536));
#34100=CARTESIAN_POINT('Ctrl Pts',(0.983693746907121,6.69512028363164,100.756384153212));
#34101=CARTESIAN_POINT('Ctrl Pts',(0.799669205420127,6.72215845218864,100.765133335956));
#34102=CARTESIAN_POINT('Ctrl Pts',(0.61452940287371,6.74160505424577,100.7738825187));
#34103=CARTESIAN_POINT('Ctrl Pts',(0.428903127363461,6.75339404354121,100.782631701444));
#34104=CARTESIAN_POINT('Ctrl Pts',(0.243278104164221,6.76518295330329,100.791380825163));
#34105=CARTESIAN_POINT('Ctrl Pts',(0.0571669005395895,6.76931433552275,
100.800129948882));
#34106=CARTESIAN_POINT('Ctrl Pts',(-0.128798404776912,6.76577415902474,
100.8088790726));
#34107=CARTESIAN_POINT('Ctrl Pts',(-0.31476251725861,6.76223400523444,100.817628140199));
#34108=CARTESIAN_POINT('Ctrl Pts',(-0.500580446819135,6.75102239665092,
100.826377207799));
#34109=CARTESIAN_POINT('Ctrl Pts',(-0.685621118842349,6.732177410125,100.835126275398));
#34110=CARTESIAN_POINT('Ctrl Pts',(-0.870660665414201,6.71333253821775,
100.843875289784));
#34111=CARTESIAN_POINT('Ctrl Pts',(-1.05492267885455,6.68685441030617,100.852624304169));
#34112=CARTESIAN_POINT('Ctrl Pts',(-1.23778137635218,6.65283295028183,100.861373318555));
#34113=CARTESIAN_POINT('Ctrl Pts',(-1.42999922978813,6.61707018861873,100.870570128923));
#34114=CARTESIAN_POINT('Ctrl Pts',(-1.62066601233661,6.57297172934421,100.87976693929));
#34115=CARTESIAN_POINT('Ctrl Pts',(-1.80906628500351,6.52070304311304,100.888963749657));
#34116=CARTESIAN_POINT('Ctrl Pts',(-1.98831342545495,6.47097374915041,100.897713747395));
#34117=CARTESIAN_POINT('Ctrl Pts',(-2.16550875896672,6.41384933989539,100.906463745133));
#34118=CARTESIAN_POINT('Ctrl Pts',(-2.34005036713983,6.34952386240486,100.915213742871));
#34119=CARTESIAN_POINT('Ctrl Pts',(-2.51458843547062,6.28519968948607,100.923963563152));
#34120=CARTESIAN_POINT('Ctrl Pts',(-2.68647261718029,6.2136748397111,100.932713383432));
#34121=CARTESIAN_POINT('Ctrl Pts',(-2.85511905908706,6.13519226743855,100.941463203713));
#34122=CARTESIAN_POINT('Ctrl Pts',(-3.02376230488855,6.05671118252952,100.950212858172));
#34123=CARTESIAN_POINT('Ctrl Pts',(-3.18916767379871,5.97127275992651,100.95896251263));
#34124=CARTESIAN_POINT('Ctrl Pts',(-3.3507733410275,5.87916720438018,100.967712167089));
#34125=CARTESIAN_POINT('Ctrl Pts',(-3.51237616037329,5.78706327195666,100.976461667357));
#34126=CARTESIAN_POINT('Ctrl Pts',(-3.6701791630226,5.68829258362324,100.985211167626));
#34127=CARTESIAN_POINT('Ctrl Pts',(-3.82364636566422,5.58319061741069,100.993960667894));
#34128=CARTESIAN_POINT('Ctrl Pts',(-3.97711106778766,5.47809036367725,101.002710025603));
#34129=CARTESIAN_POINT('Ctrl Pts',(-4.12623987481902,5.36665920043244,101.011459383311));
#34130=CARTESIAN_POINT('Ctrl Pts',(-4.27052628213912,5.24927559512349,101.02020874102));
#34131=CARTESIAN_POINT('Ctrl Pts',(-4.41481053024959,5.13189374643053,101.028957967796));
#34132=CARTESIAN_POINT('Ctrl Pts',(-4.55425230136508,5.00855981477373,101.037707194573));
#34133=CARTESIAN_POINT('Ctrl Pts',(-4.68837800630524,4.87969268192099,101.046456421349));
#34134=CARTESIAN_POINT('Ctrl Pts',(-4.8225018822886,4.75082730631844,101.05520552882));
#34135=CARTESIAN_POINT('Ctrl Pts',(-4.95130963052922,4.61642907903572,101.063954636291));
#34136=CARTESIAN_POINT('Ctrl Pts',(-5.07436379033314,4.47695444731749,101.072703743762));
#34137=CARTESIAN_POINT('Ctrl Pts',(-5.19741643562771,4.33748153220628,101.081452743551));
#34138=CARTESIAN_POINT('Ctrl Pts',(-5.31471544462755,4.19293255254613,101.090201743341));
#34139=CARTESIAN_POINT('Ctrl Pts',(-5.42586245275625,4.04379841779607,101.098950743131));
#34140=CARTESIAN_POINT('Ctrl Pts',(-5.53702160019144,3.89464799484354,101.107700698473));
#34141=CARTESIAN_POINT('Ctrl Pts',(-5.64202723081238,3.7409116444387,101.116450653815));
#34142=CARTESIAN_POINT('Ctrl Pts',(-5.74052265232949,3.58311159163261,101.125200609157));
#34143=CARTESIAN_POINT('Ctrl Pts',(-5.83901427066895,3.42531763191822,101.13395022664));
#34144=CARTESIAN_POINT('Ctrl Pts',(-5.93099603115711,3.26346052695663,101.142699844122));
#34145=CARTESIAN_POINT('Ctrl Pts',(-6.01615550622722,3.09809004467139,101.151449461605));
#34146=CARTESIAN_POINT('Ctrl Pts',(-6.10131214578771,2.93272506863886,101.160198787756));
#34147=CARTESIAN_POINT('Ctrl Pts',(-6.17964682328723,2.76384720416949,101.168948113907));
#34148=CARTESIAN_POINT('Ctrl Pts',(-6.25089348288543,2.59203002791644,101.177697440058));
#34149=CARTESIAN_POINT('Ctrl Pts',(-6.32213814889316,2.42021765937067,101.18644652139));
#34150=CARTESIAN_POINT('Ctrl Pts',(-6.38629508412577,2.24546640831943,101.195195602721));
#34151=CARTESIAN_POINT('Ctrl Pts',(-6.44314639819808,2.06836976660053,101.203944684053));
#34152=CARTESIAN_POINT('Ctrl Pts',(-6.500002852837,1.89125711158277,101.212694556487));
#34153=CARTESIAN_POINT('Ctrl Pts',(-6.54955227673252,1.71179891440246,101.221444428922));
#34154=CARTESIAN_POINT('Ctrl Pts',(-6.59162635926389,1.53060476278412,101.230194301356));
#34155=CARTESIAN_POINT('Ctrl Pts',(-6.63369752055195,1.34942319164699,101.238943566278));
#34156=CARTESIAN_POINT('Ctrl Pts',(-6.66829431424249,1.16650618642729,101.247692831201));
#34157=CARTESIAN_POINT('Ctrl Pts',(-6.6952992374541,0.98247499761903,101.256442096123));
#34158=CARTESIAN_POINT('Ctrl Pts',(-6.72230554731438,0.798434359178225,
101.265191810303));
#34159=CARTESIAN_POINT('Ctrl Pts',(-6.74171916496698,0.613279706240836,
101.273941524483));
#34160=CARTESIAN_POINT('Ctrl Pts',(-6.75347414817272,0.427639953655887,
101.282691238662));
#34161=CARTESIAN_POINT('Ctrl Pts',(-6.76248837758735,0.285283364200229,
101.289400897838));
#34162=CARTESIAN_POINT('Ctrl Pts',(-6.76699999999988,0.142641701107921,
101.296110557014));
#34163=CARTESIAN_POINT('Ctrl Pts',(-6.767,5.52010523486073E-12,101.30282021619));
#34164=CARTESIAN_POINT('Ctrl Pts',(-6.76699704717928,-0.00632166646298646,
101.30282021619));
#34165=CARTESIAN_POINT('Ctrl Pts',(-6.76677605484367,-0.24288183478154,
101.313959647533));
#34166=CARTESIAN_POINT('Ctrl Pts',(-6.75414753504645,-0.478876740857043,
101.325099078876));
#34167=CARTESIAN_POINT('Ctrl Pts',(-6.72930744162487,-0.713239339977983,
101.336238510219));
#34168=CARTESIAN_POINT('Ctrl Pts',(-6.70352641088801,-0.956479543183305,
101.347799900788));
#34169=CARTESIAN_POINT('Ctrl Pts',(-6.66459101458145,-1.19796201672306,
101.359361291358));
#34170=CARTESIAN_POINT('Ctrl Pts',(-6.61276709992077,-1.43652367965356,
101.370922681928));
#34171=CARTESIAN_POINT('Ctrl Pts',(-6.60039721361044,-1.49346612924997,
101.373682278301));
#34172=CARTESIAN_POINT('Ctrl Pts',(-6.58729323537896,-1.55024227680139,
101.376441874675));
#34173=CARTESIAN_POINT('Ctrl Pts',(-6.57345917388123,-1.60683648493453,
101.379201471048));
#34174=CARTESIAN_POINT('Ctrl Pts',(-6.53257525540682,-1.77408982494738,
101.387356929454));
#34175=CARTESIAN_POINT('Ctrl Pts',(-6.48523716147742,-1.94005459146327,
101.395512387861));
#34176=CARTESIAN_POINT('Ctrl Pts',(-6.43153762266074,-2.10418934706445,
101.403667846268));
#34177=CARTESIAN_POINT('Ctrl Pts',(-6.37790344324148,-2.26812432909289,
101.41181337841));
#34178=CARTESIAN_POINT('Ctrl Pts',(-6.31792334356615,-2.43023339030949,
101.419958910552));
#34179=CARTESIAN_POINT('Ctrl Pts',(-6.2517410497252,-2.58998510559055,101.428104442694));
#34180=CARTESIAN_POINT('Ctrl Pts',(-6.18562539162669,-2.74957597461595,
101.436241773494));
#34181=CARTESIAN_POINT('Ctrl Pts',(-6.11332011027605,-2.90681388777158,
101.444379104295));
#34182=CARTESIAN_POINT('Ctrl Pts',(-6.0350187392794,-3.0611824213115,101.452516435095));
#34183=CARTESIAN_POINT('Ctrl Pts',(-5.95677975086082,-3.21542796968561,
101.460647282897));
#34184=CARTESIAN_POINT('Ctrl Pts',(-5.87255434911937,-3.36680836576513,
101.468778130699));
#34185=CARTESIAN_POINT('Ctrl Pts',(-5.78258419121467,-3.51482703294404,
101.476908978501));
#34186=CARTESIAN_POINT('Ctrl Pts',(-5.69266681260293,-3.66275886776898,
101.485035056495));
#34187=CARTESIAN_POINT('Ctrl Pts',(-5.59701157858968,-3.80733258953256,
101.493161134489));
#34188=CARTESIAN_POINT('Ctrl Pts',(-5.49590610710017,-3.94807612159885,
101.501287212483));
#34189=CARTESIAN_POINT('Ctrl Pts',(-5.39444213407503,-4.08931870452396,
101.509442104065));
#34190=CARTESIAN_POINT('Ctrl Pts',(-5.28748937522943,-4.22670355676432,
101.517596995647));
#34191=CARTESIAN_POINT('Ctrl Pts',(-5.17538278403037,-4.35978233846165,
101.525751887229));
#34192=CARTESIAN_POINT('Ctrl Pts',(-5.06371336934004,-4.49234215944,101.533874977585));
#34193=CARTESIAN_POINT('Ctrl Pts',(-4.94693049683313,-4.62062916326516,
101.541998067942));
#34194=CARTESIAN_POINT('Ctrl Pts',(-4.82540576829853,-4.74423314891578,
101.550121158298));
#34195=CARTESIAN_POINT('Ctrl Pts',(-4.70387149708733,-4.86784684051576,
101.558244886516));
#34196=CARTESIAN_POINT('Ctrl Pts',(-4.57759488461345,-4.98677652056343,
101.566368614735));
#34197=CARTESIAN_POINT('Ctrl Pts',(-4.44698442969164,-5.10064882951964,
101.574492342953));
#34198=CARTESIAN_POINT('Ctrl Pts',(-4.31633887015681,-5.21455174432087,
101.582618254614));
#34199=CARTESIAN_POINT('Ctrl Pts',(-4.18135742442363,-5.32339434113196,
101.590744166274));
#34200=CARTESIAN_POINT('Ctrl Pts',(-4.0424816528769,-5.42684356566077,101.598870077934));
#34201=CARTESIAN_POINT('Ctrl Pts',(-3.90271775633498,-5.530954358734,101.607047955644));
#34202=CARTESIAN_POINT('Ctrl Pts',(-3.75900985307031,-5.62960233335927,
101.615225833354));
#34203=CARTESIAN_POINT('Ctrl Pts',(-3.6118368983089,-5.72249274530028,101.623403711064));
#34204=CARTESIAN_POINT('Ctrl Pts',(-3.46536636814058,-5.81493981145188,
101.631542557538));
#34205=CARTESIAN_POINT('Ctrl Pts',(-3.31546413734347,-5.90168402369238,
101.639681404011));
#34206=CARTESIAN_POINT('Ctrl Pts',(-3.16262594594144,-5.98248160265103,
101.647820250485));
#34207=CARTESIAN_POINT('Ctrl Pts',(-3.00868831182946,-6.06386039961777,
101.656017643813));
#34208=CARTESIAN_POINT('Ctrl Pts',(-2.85177265868612,-6.13920652292378,
101.664215037142));
#34209=CARTESIAN_POINT('Ctrl Pts',(-2.69240440419186,-6.20832082968401,
101.67241243047));
#34210=CARTESIAN_POINT('Ctrl Pts',(-2.5330361496976,-6.27743513644424,101.680609823798));
#34211=CARTESIAN_POINT('Ctrl Pts',(-2.37121566294458,-6.34031754879485,
101.688807217127));
#34212=CARTESIAN_POINT('Ctrl Pts',(-2.20748187330029,-6.39682052109098,
101.697004610455));
#34213=CARTESIAN_POINT('Ctrl Pts',(-2.04317251602129,-6.45352211629927,
101.705230819792));
#34214=CARTESIAN_POINT('Ctrl Pts',(-1.87644740536304,-6.50396820714166,
101.713457029129));
#34215=CARTESIAN_POINT('Ctrl Pts',(-1.70782342178583,-6.54794839319918,
101.721683238466));
#34216=CARTESIAN_POINT('Ctrl Pts',(-1.5393888800303,-6.59187916940179,101.729900206009));
#34217=CARTESIAN_POINT('Ctrl Pts',(-1.36906005721576,-6.62935841606095,
101.738117173552));
#34218=CARTESIAN_POINT('Ctrl Pts',(-1.19737214157202,-6.66022439220986,
101.746334141096));
#34219=CARTESIAN_POINT('Ctrl Pts',(-1.02584265080669,-6.69106188680549,
101.754543526439));
#34220=CARTESIAN_POINT('Ctrl Pts',(-0.852956915561639,-6.71529820096794,
101.762752911782));
#34221=CARTESIAN_POINT('Ctrl Pts',(-0.679263651728511,-6.73282183719727,
101.770962297126));
#34222=CARTESIAN_POINT('Ctrl Pts',(-0.505695812766533,-6.75033281951149,
101.779165754426));
#34223=CARTESIAN_POINT('Ctrl Pts',(-0.331321962072286,-6.76114074295263,
101.787369211727));
#34224=CARTESIAN_POINT('Ctrl Pts',(-0.156699429616982,-6.7651854585634,
101.795572669028));
#34225=CARTESIAN_POINT('Ctrl Pts',(0.017832035788296,-6.76922806482257,
101.803771848159));
#34226=CARTESIAN_POINT('Ctrl Pts',(0.192611566902767,-6.76651448151195,
101.811971027291));
#34227=CARTESIAN_POINT('Ctrl Pts',(0.367078218529337,-6.75703652361605,
101.820170206423));
#34228=CARTESIAN_POINT('Ctrl Pts',(0.541511996878627,-6.7475603515717,101.828367840653));
#34229=CARTESIAN_POINT('Ctrl Pts',(0.71563265509255,-6.73132235694608,101.836565474883));
#34230=CARTESIAN_POINT('Ctrl Pts',(0.888880445623995,-6.70836645938393,
101.844763109113));
#34231=CARTESIAN_POINT('Ctrl Pts',(1.06211573094008,-6.68541221880362,101.852960151628));
#34232=CARTESIAN_POINT('Ctrl Pts',(1.234477918364,-6.65574108724116,101.861157194144));
#34233=CARTESIAN_POINT('Ctrl Pts',(1.40541362672095,-6.6194487336807,101.869354236659));
#34234=CARTESIAN_POINT('Ctrl Pts',(1.57636806403,-6.58315240366759,101.877552177302));
#34235=CARTESIAN_POINT('Ctrl Pts',(1.74589535995426,-6.54023348082067,101.885750117945));
#34236=CARTESIAN_POINT('Ctrl Pts',(1.91345349777141,-6.4908385214752,101.893948058588));
#34237=CARTESIAN_POINT('Ctrl Pts',(2.08106044799347,-6.44142917257642,101.902148387424));
#34238=CARTESIAN_POINT('Ctrl Pts',(2.24669675351575,-6.38554013074687,101.91034871626));
#34239=CARTESIAN_POINT('Ctrl Pts',(2.40983664903004,-6.32336748299446,101.918549045096));
#34240=CARTESIAN_POINT('Ctrl Pts',(2.57314654054857,-6.26113004972985,101.926757918887));
#34241=CARTESIAN_POINT('Ctrl Pts',(2.73395448939905,-6.19259605716673,101.934966792679));
#34242=CARTESIAN_POINT('Ctrl Pts',(2.89175485330826,-6.11800971463499,101.94317566647));
#34243=CARTESIAN_POINT('Ctrl Pts',(3.04963990693204,-6.043383342436,101.951388945874));
#34244=CARTESIAN_POINT('Ctrl Pts',(3.20451383998295,-5.96269831037021,101.959602225277));
#34245=CARTESIAN_POINT('Ctrl Pts',(3.35589673515166,-5.87624421744012,101.96781550468));
#34246=CARTESIAN_POINT('Ctrl Pts',(3.5075010515976,-5.78966367181101,101.976040797296));
#34247=CARTESIAN_POINT('Ctrl Pts',(3.65560382144678,-5.69729739200272,101.984266089911));
#34248=CARTESIAN_POINT('Ctrl Pts',(3.7997541101936,-5.5994783419589,101.992491382527));
#34249=CARTESIAN_POINT('Ctrl Pts',(3.93012073039307,-5.51101276165242,101.999930171639));
#34250=CARTESIAN_POINT('Ctrl Pts',(4.05725485954066,-5.41808800326091,102.007368960751));
#34251=CARTESIAN_POINT('Ctrl Pts',(4.18084761357551,-5.32097756357419,102.014807749863));
#34252=CARTESIAN_POINT('Ctrl Pts',(4.31752292777657,-5.2135877739378,102.023033950882));
#34253=CARTESIAN_POINT('Ctrl Pts',(4.45024897394864,-5.10077851177387,102.031260151901));
#34254=CARTESIAN_POINT('Ctrl Pts',(4.5785688837601,-4.98287025484949,102.039486352919));
#34255=CARTESIAN_POINT('Ctrl Pts',(4.70674465319765,-4.86509444300137,102.047703313535));
#34256=CARTESIAN_POINT('Ctrl Pts',(4.83052388012345,-4.74223128214391,102.055920274151));
#34257=CARTESIAN_POINT('Ctrl Pts',(4.94948067859382,-4.61464299943414,102.064137234767));
#34258=CARTESIAN_POINT('Ctrl Pts',(5.06832772974694,-4.48717242728752,102.072346614568));
#34259=CARTESIAN_POINT('Ctrl Pts',(5.18236096992875,-4.35498567567921,102.08055599437));
#34260=CARTESIAN_POINT('Ctrl Pts',(5.29118941659963,-4.21848356138365,102.088765374171));
#34261=CARTESIAN_POINT('Ctrl Pts',(5.39993929590646,-4.08207999311752,102.096968827312));
#34262=CARTESIAN_POINT('Ctrl Pts',(5.50349164340634,-3.94136754683849,102.105172280452));
#34263=CARTESIAN_POINT('Ctrl Pts',(5.60149397071873,-3.79678209751385,102.113375733593));
#34264=CARTESIAN_POINT('Ctrl Pts',(5.6994452054739,-3.65227202640264,102.121574909943));
#34265=CARTESIAN_POINT('Ctrl Pts',(5.79185198356465,-3.50389327091828,102.129774086293));
#34266=CARTESIAN_POINT('Ctrl Pts',(5.87840353612408,-3.35211289584404,102.137973262643));
#34267=CARTESIAN_POINT('Ctrl Pts',(5.9649388027028,-3.2003610805378,102.146170896194));
#34268=CARTESIAN_POINT('Ctrl Pts',(6.04562085544122,-3.045209228725,102.154368529746));
#34269=CARTESIAN_POINT('Ctrl Pts',(6.1201833705286,-2.88715162592914,102.162566163297));
#34270=CARTESIAN_POINT('Ctrl Pts',(6.19474051528497,-2.72910540715973,102.170763206418));
#34271=CARTESIAN_POINT('Ctrl Pts',(6.26317884635147,-2.56815417822818,102.178960249538));
#34272=CARTESIAN_POINT('Ctrl Pts',(6.32527898651211,-2.40481490821818,102.187157292659));
#34273=CARTESIAN_POINT('Ctrl Pts',(6.38738594053535,-2.24145771600476,102.19535523519));
#34274=CARTESIAN_POINT('Ctrl Pts',(6.44315319062226,-2.07571229602015,102.203553177721));
#34275=CARTESIAN_POINT('Ctrl Pts',(6.49241028927303,-1.90811363281691,102.211751120252));
#34276=CARTESIAN_POINT('Ctrl Pts',(6.54168174502811,-1.74046611916255,102.219951452261));
#34277=CARTESIAN_POINT('Ctrl Pts',(6.58443916857949,-1.57096463037527,102.228151784269));
#34278=CARTESIAN_POINT('Ctrl Pts',(6.62056254925754,-1.40015732379206,102.236352116278));
#34279=CARTESIAN_POINT('Ctrl Pts',(6.65672358026163,-1.22917198982982,102.244560995248));
#34280=CARTESIAN_POINT('Ctrl Pts',(6.68623668002341,-1.05687847035063,102.252769874219));
#34281=CARTESIAN_POINT('Ctrl Pts',(6.70903318831306,-0.883834078384577,
102.26097875319));
#34282=CARTESIAN_POINT('Ctrl Pts',(6.73184193429711,-0.710696792175269,
102.269192038877));
#34283=CARTESIAN_POINT('Ctrl Pts',(6.74792686787206,-0.536808186722328,
102.277405324565));
#34284=CARTESIAN_POINT('Ctrl Pts',(6.75727141716096,-0.362728541501153,
102.285618610252));
#34285=CARTESIAN_POINT('Ctrl Pts',(6.76662963637377,-0.188394239213868,
102.293843910964));
#34286=CARTESIAN_POINT('Ctrl Pts',(6.76922776069267,-0.0138686972772417,
102.302069211676));
#34287=CARTESIAN_POINT('Ctrl Pts',(6.76510136961379,0.160288673491626,102.310294512388));
#34288=CARTESIAN_POINT('Ctrl Pts',(6.76136954664049,0.317793007128361,102.317733304682));
#34289=CARTESIAN_POINT('Ctrl Pts',(6.75213842063547,0.474996070190415,102.325172096976));
#34290=CARTESIAN_POINT('Ctrl Pts',(6.7374705412114,0.631490068258035,102.33261088927));
#34291=CARTESIAN_POINT('Ctrl Pts',(6.72139525549191,0.802999913654975,102.340763445483));
#34292=CARTESIAN_POINT('Ctrl Pts',(6.69874158818251,0.97416380000485,102.348916001697));
#34293=CARTESIAN_POINT('Ctrl Pts',(6.66952499726471,1.14443230942732,102.35706855791));
#34294=CARTESIAN_POINT('Ctrl Pts',(6.64034225447185,1.31450355867679,102.36521166919));
#34295=CARTESIAN_POINT('Ctrl Pts',(6.60461178436809,1.48368113926133,102.373354780471));
#34296=CARTESIAN_POINT('Ctrl Pts',(6.56240095140022,1.65141840641962,102.381497891751));
#34297=CARTESIAN_POINT('Ctrl Pts',(6.52023014639807,1.81899661058134,102.389633281028));
#34298=CARTESIAN_POINT('Ctrl Pts',(6.47159130151889,1.98513686843841,102.397768670306));
#34299=CARTESIAN_POINT('Ctrl Pts',(6.41660320791154,2.14930041460457,102.405904059583));
#34300=CARTESIAN_POINT('Ctrl Pts',(6.36165570444918,2.31334278140798,102.414033443622));
#34301=CARTESIAN_POINT('Ctrl Pts',(6.30036840007265,2.47541099674163,102.42216282766));
#34302=CARTESIAN_POINT('Ctrl Pts',(6.23291052180081,2.63497920812001,102.430292211699));
#34303=CARTESIAN_POINT('Ctrl Pts',(6.16548826901972,2.79446314919543,102.438417302491));
#34304=CARTESIAN_POINT('Ctrl Pts',(6.0919020743481,2.95144937976762,102.446542393283));
#34305=CARTESIAN_POINT('Ctrl Pts',(6.01237010880785,3.10542986955332,102.454667484075));
#34306=CARTESIAN_POINT('Ctrl Pts',(5.93253455251368,3.25999813624939,102.4628235901));
#34307=CARTESIAN_POINT('Ctrl Pts',(5.84670786880475,3.41153731929982,102.470979696125));
#34308=CARTESIAN_POINT('Ctrl Pts',(5.7551585947507,3.55955594832659,102.479135802151));
#34309=CARTESIAN_POINT('Ctrl Pts',(5.66397778996784,3.70697882914099,102.487259081324));
#34310=CARTESIAN_POINT('Ctrl Pts',(5.56712058616963,3.85090914058018,102.495382360497));
#34311=CARTESIAN_POINT('Ctrl Pts',(5.46489701561949,3.9908883232525,102.503505639671));
#34312=CARTESIAN_POINT('Ctrl Pts',(5.3626598331371,4.13088614533589,102.511630000528));
#34313=CARTESIAN_POINT('Ctrl Pts',(5.25505507636806,4.26693149524327,102.519754361384));
#34314=CARTESIAN_POINT('Ctrl Pts',(5.14243446978351,4.39859713135704,102.527878722241));
#34315=CARTESIAN_POINT('Ctrl Pts',(5.02977744016367,4.53030534992758,102.536005710626));
#34316=CARTESIAN_POINT('Ctrl Pts',(4.9121015680922,4.65763075622964,102.544132699012));
#34317=CARTESIAN_POINT('Ctrl Pts',(4.78979695461393,4.7801813912833,102.552259687397));
#34318=CARTESIAN_POINT('Ctrl Pts',(4.66670165573424,4.90352430223986,102.560439215837));
#34319=CARTESIAN_POINT('Ctrl Pts',(4.53891782486309,5.02203022519002,102.568618744277));
#34320=CARTESIAN_POINT('Ctrl Pts',(4.40687795864314,5.13533987751787,102.576798272717));
#34321=CARTESIAN_POINT('Ctrl Pts',(4.27545991072082,5.24811591816364,102.584939281121));
#34322=CARTESIAN_POINT('Ctrl Pts',(4.13982615344022,5.35574434796051,102.593080289525));
#34323=CARTESIAN_POINT('Ctrl Pts',(4.00043295278129,5.45791399623533,102.601221297929));
#34324=CARTESIAN_POINT('Ctrl Pts',(3.86005042176651,5.560808784144,102.609420086387));
#34325=CARTESIAN_POINT('Ctrl Pts',(3.71585519949623,5.65816680806154,102.617618874845));
#34326=CARTESIAN_POINT('Ctrl Pts',(3.56833894735471,5.74971705015051,102.625817663303));
#34327=CARTESIAN_POINT('Ctrl Pts',(3.4208226952133,5.84126729223942,102.634016451762));
#34328=CARTESIAN_POINT('Ctrl Pts',(3.26998576806624,5.92700962529715,102.64221524022));
#34329=CARTESIAN_POINT('Ctrl Pts',(3.11634032552883,6.00672223225636,102.650414028678));
#34330=CARTESIAN_POINT('Ctrl Pts',(3.1106233360721,6.00968825666964,102.650719097194));
#34331=CARTESIAN_POINT('Ctrl Pts',(3.10490180318934,6.01264627953154,102.65102416571));
#34332=CARTESIAN_POINT('Ctrl Pts',(3.09917575053253,6.01559628526642,102.651329234227));
#34333=CARTESIAN_POINT('Origin',(0.,0.,-3.69717978381041));
#34334=CARTESIAN_POINT('',(3.09917575053258,6.0155962852664,105.045751582742));
#34335=CARTESIAN_POINT('',(3.09917575053253,6.01559628526642,104.651558856765));
#34336=CARTESIAN_POINT('',(3.09917575053259,6.01559628526639,-3.69717978381041));
#34337=CARTESIAN_POINT('',(-6.767,5.83999903015602E-12,103.69717978381));
#34338=CARTESIAN_POINT('Ctrl Pts',(-6.767,5.83999902796969E-12,103.69717978381));
#34339=CARTESIAN_POINT('Ctrl Pts',(-6.76700000000016,-0.186007249409826,
103.705929295616));
#34340=CARTESIAN_POINT('Ctrl Pts',(-6.7593263729547,-0.372014355521671,
103.714678807422));
#34341=CARTESIAN_POINT('Ctrl Pts',(-6.74400518266976,-0.557389537149187,
103.723428319228));
#34342=CARTESIAN_POINT('Ctrl Pts',(-6.7286840570971,-0.742763935805548,
103.732177794078));
#34343=CARTESIAN_POINT('Ctrl Pts',(-6.70571545653072,-0.927506129689208,
103.740927268929));
#34344=CARTESIAN_POINT('Ctrl Pts',(-6.67517739415747,-1.11098863924396,
103.749676743779));
#34345=CARTESIAN_POINT('Ctrl Pts',(-6.64463945823177,-1.29447038906111,
103.758426182401));
#34346=CARTESIAN_POINT('Ctrl Pts',(-6.6065321702724,-1.4766921822785,103.767175621023));
#34347=CARTESIAN_POINT('Ctrl Pts',(-6.56098496116798,-1.65703510503779,
103.775925059645));
#34348=CARTESIAN_POINT('Ctrl Pts',(-6.51543793687612,-1.83737729603683,
103.784674462766));
#34349=CARTESIAN_POINT('Ctrl Pts',(-6.46245112202743,-2.01584035396719,
103.793423865886));
#34350=CARTESIAN_POINT('Ctrl Pts',(-6.40220448416355,-2.19181813637813,
103.802173269006));
#34351=CARTESIAN_POINT('Ctrl Pts',(-6.34195808575307,-2.36779521935624,
103.810922637351));
#34352=CARTESIAN_POINT('Ctrl Pts',(-6.2744520148936,-2.54128677544517,103.819672005697));
#34353=CARTESIAN_POINT('Ctrl Pts',(-6.19991555136315,-2.71170355237541,
103.828421374042));
#34354=CARTESIAN_POINT('Ctrl Pts',(-6.12537937789178,-2.88211966612775,
103.837170708339));
#34355=CARTESIAN_POINT('Ctrl Pts',(-6.04381298133765,-3.04946076210151,
103.845920042636));
#34356=CARTESIAN_POINT('Ctrl Pts',(-5.95549339426463,-3.21315848206564,
103.854669376933));
#34357=CARTESIAN_POINT('Ctrl Pts',(-5.86717414355331,-3.37685557859339,
103.863418677909));
#34358=CARTESIAN_POINT('Ctrl Pts',(-5.77210188986423,-3.53690907467009,
103.872167978884));
#34359=CARTESIAN_POINT('Ctrl Pts',(-5.67059953467268,-3.69277536784598,
103.88091727986));
#34360=CARTESIAN_POINT('Ctrl Pts',(-5.56909755761982,-3.84864108035479,
103.889666548241));
#34361=CARTESIAN_POINT('Ctrl Pts',(-5.46116568338304,-4.00031938103959,
103.898415816621));
#34362=CARTESIAN_POINT('Ctrl Pts',(-5.34717048686366,-4.14729511662894,
103.907165085002));
#34363=CARTESIAN_POINT('Ctrl Pts',(-5.23317570555772,-4.2942703168773,103.915914321515));
#34364=CARTESIAN_POINT('Ctrl Pts',(-5.11311782179062,-4.43654275986834,
103.924663558027));
#34365=CARTESIAN_POINT('Ctrl Pts',(-4.98740459172272,-4.57362924147368,
103.93341279454));
#34366=CARTESIAN_POINT('Ctrl Pts',(-4.86169180911094,-4.71071523514164,
103.942161999911));
#34367=CARTESIAN_POINT('Ctrl Pts',(-4.73032391415701,-4.84261509316261,
103.950911205282));
#34368=CARTESIAN_POINT('Ctrl Pts',(-4.59374707237567,-4.9688808433127,103.959660410653));
#34369=CARTESIAN_POINT('Ctrl Pts',(-4.45717070537701,-5.09514615452462,
103.96840958561));
#34370=CARTESIAN_POINT('Ctrl Pts',(-4.31538563819835,-5.21577720253362,
103.977158760566));
#34371=CARTESIAN_POINT('Ctrl Pts',(-4.16887341291001,-5.33036429028374,
103.985907935522));
#34372=CARTESIAN_POINT('Ctrl Pts',(-4.02236168477712,-5.444950989209,103.99465708079));
#34373=CARTESIAN_POINT('Ctrl Pts',(-3.87112305634832,-5.55349359238484,
104.003406226058));
#34374=CARTESIAN_POINT('Ctrl Pts',(-3.71567117317147,-5.65562346102201,
104.012155371326));
#34375=CARTESIAN_POINT('Ctrl Pts',(-3.56021980457718,-5.75775299158512,
104.020904487632));
#34376=CARTESIAN_POINT('Ctrl Pts',(-3.40055544862807,-5.8534696727511,104.029653603938));
#34377=CARTESIAN_POINT('Ctrl Pts',(-3.23722036323823,-5.94244842803333,
104.038402720244));
#34378=CARTESIAN_POINT('Ctrl Pts',(-3.073885804965,-6.03142689616243,104.047151808315));
#34379=CARTESIAN_POINT('Ctrl Pts',(-2.90688079258194,-6.1136673448459,104.055900896386));
#34380=CARTESIAN_POINT('Ctrl Pts',(-2.73677251095136,-6.18889046787072,
104.064649984457));
#34381=CARTESIAN_POINT('Ctrl Pts',(-2.56666476417183,-6.26411335438049,
104.073399045019));
#34382=CARTESIAN_POINT('Ctrl Pts',(-2.39345402972648,-6.3323188435008,104.082148105581));
#34383=CARTESIAN_POINT('Ctrl Pts',(-2.2177285647461,-6.39327529620845,104.090897166144));
#34384=CARTESIAN_POINT('Ctrl Pts',(-2.04200363768856,-6.45423156231896,
104.099646199924));
#34385=CARTESIAN_POINT('Ctrl Pts',(-1.86376426620693,-6.50793874251884,
104.108395233704));
#34386=CARTESIAN_POINT('Ctrl Pts',(-1.68361578195302,-6.55421443795965,
104.117144267484));
#34387=CARTESIAN_POINT('Ctrl Pts',(-1.50346783420474,-6.60048999558542,
104.125893275208));
#34388=CARTESIAN_POINT('Ctrl Pts',(-1.32141106257844,-6.63933404145377,
104.134642282932));
#34389=CARTESIAN_POINT('Ctrl Pts',(-1.13806375959632,-6.6706146552693,104.143391290656));
#34390=CARTESIAN_POINT('Ctrl Pts',(-0.954716987425001,-6.70189517852397,
104.152140273051));
#34391=CARTESIAN_POINT('Ctrl Pts',(-0.770079973815685,-6.72561226535761,
104.160889255446));
#34392=CARTESIAN_POINT('Ctrl Pts',(-0.584779770558221,-6.74168536939732,
104.169638237841));
#34393=CARTESIAN_POINT('Ctrl Pts',(-0.391490647559682,-6.7584514394236,
104.178764418517));
#34394=CARTESIAN_POINT('Ctrl Pts',(-0.197480213110104,-6.7668997592401,
104.187890599193));
#34395=CARTESIAN_POINT('Ctrl Pts',(-0.00346532630355763,-6.76699911271707,
104.197016779869));
#34396=CARTESIAN_POINT('Ctrl Pts',(0.184486595290381,-6.76709536139789,
104.205857767399));
#34397=CARTESIAN_POINT('Ctrl Pts',(0.372442378179646,-6.75935659726801,
104.214698754929));
#34398=CARTESIAN_POINT('Ctrl Pts',(0.559750217716602,-6.74380965729062,
104.223539742459));
#34399=CARTESIAN_POINT('Ctrl Pts',(0.745129914452278,-6.72842275717314,
104.232289721057));
#34400=CARTESIAN_POINT('Ctrl Pts',(0.929874656308724,-6.70538772273549,
104.241039699655));
#34401=CARTESIAN_POINT('Ctrl Pts',(1.11335688289233,-6.67478280180833,104.249789678252));
#34402=CARTESIAN_POINT('Ctrl Pts',(1.29683723118314,-6.64417819418129,104.258539567277));
#34403=CARTESIAN_POINT('Ctrl Pts',(1.47905480729695,-6.60600390230196,104.267289456302));
#34404=CARTESIAN_POINT('Ctrl Pts',(1.65939064804271,-6.5603895979727,104.276039345327));
#34405=CARTESIAN_POINT('Ctrl Pts',(1.83972470263724,-6.51477574543409,104.284789147688));
#34406=CARTESIAN_POINT('Ctrl Pts',(2.01817678125304,-6.46172209820269,104.293538950049));
#34407=CARTESIAN_POINT('Ctrl Pts',(2.19414072347134,-6.40140886724201,104.30228875241));
#34408=CARTESIAN_POINT('Ctrl Pts',(2.37010298131563,-6.34109621361574,104.311038471015));
#34409=CARTESIAN_POINT('Ctrl Pts',(2.54357687926391,-6.27352420826183,104.319788189621));
#34410=CARTESIAN_POINT('Ctrl Pts',(2.71397317789462,-6.19892237325719,104.328537908226));
#34411=CARTESIAN_POINT('Ctrl Pts',(2.88436790206691,-6.12432122757204,104.337287545985));
#34412=CARTESIAN_POINT('Ctrl Pts',(3.05168482125746,-6.04269049717674,104.346037183743));
#34413=CARTESIAN_POINT('Ctrl Pts',(3.21535561996879,-5.95430745235205,104.354786821501));
#34414=CARTESIAN_POINT('Ctrl Pts',(3.37902496074777,-5.86592519481807,104.36353638132));
#34415=CARTESIAN_POINT('Ctrl Pts',(3.53904799384378,-5.77079087940536,104.372285941139));
#34416=CARTESIAN_POINT('Ctrl Pts',(3.69488118814495,-5.66922763747343,104.381035500958));
#34417=CARTESIAN_POINT('Ctrl Pts',(3.85071304610354,-5.56766526649383,104.389784985746));
#34418=CARTESIAN_POINT('Ctrl Pts',(4.002354897055,-5.45967423581057,104.398534470533));
#34419=CARTESIAN_POINT('Ctrl Pts',(4.14929168607198,-5.34562133936683,104.407283955321));
#34420=CARTESIAN_POINT('Ctrl Pts',(4.296227263853,-5.23156938308905,104.416033367984));
#34421=CARTESIAN_POINT('Ctrl Pts',(4.43845763091611,-5.11145583677598,104.424782780647));
#34422=CARTESIAN_POINT('Ctrl Pts',(4.57549970660508,-4.98568866204628,104.43353219331));
#34423=CARTESIAN_POINT('Ctrl Pts',(4.71254069814855,-4.85992248226588,104.442281536757));
#34424=CARTESIAN_POINT('Ctrl Pts',(4.84439326930888,-4.72850295734439,104.451030880203));
#34425=CARTESIAN_POINT('Ctrl Pts',(4.97060959434287,-4.59187644222127,104.459780223649));
#34426=CARTESIAN_POINT('Ctrl Pts',(5.09682496280121,-4.45525096257115,104.468529500786));
#34427=CARTESIAN_POINT('Ctrl Pts',(5.21740397615462,-4.31341878218783,104.477278777922));
#34428=CARTESIAN_POINT('Ctrl Pts',(5.33193710451573,-4.16686161439139,104.486028055058));
#34429=CARTESIAN_POINT('Ctrl Pts',(5.44646940289039,-4.0203055086498,104.494777268791));
#34430=CARTESIAN_POINT('Ctrl Pts',(5.55495572749338,-3.86902470980603,104.503526482524));
#34431=CARTESIAN_POINT('Ctrl Pts',(5.65702762491146,-3.71353301466254,104.512275696257));
#34432=CARTESIAN_POINT('Ctrl Pts',(5.75909881654858,-3.55804239467372,104.521024849493));
#34433=CARTESIAN_POINT('Ctrl Pts',(5.85475551250501,-3.39834117620037,104.529774002729));
#34434=CARTESIAN_POINT('Ctrl Pts',(5.94367283727829,-3.23497174692459,104.538523155966));
#34435=CARTESIAN_POINT('Ctrl Pts',(6.03258957676073,-3.07160339301437,104.547272251611));
#34436=CARTESIAN_POINT('Ctrl Pts',(6.11476689685071,-2.90456712829955,104.556021347257));
#34437=CARTESIAN_POINT('Ctrl Pts',(6.18992570525071,-2.73443024476334,104.564770442902));
#34438=CARTESIAN_POINT('Ctrl Pts',(6.26508404388517,-2.5642944246347,104.573519483863));
#34439=CARTESIAN_POINT('Ctrl Pts',(6.33322384283144,-2.39105828656444,104.582268524824));
#34440=CARTESIAN_POINT('Ctrl Pts',(6.39411368719873,-2.21531017132543,104.591017565785));
#34441=CARTESIAN_POINT('Ctrl Pts',(6.45500317120733,-2.03956309620009,104.599766554968));
#34442=CARTESIAN_POINT('Ctrl Pts',(6.50864269269922,-1.86130434439159,104.60851554415));
#34443=CARTESIAN_POINT('Ctrl Pts',(6.5548500844619,-1.68113930720503,104.617264533332));
#34444=CARTESIAN_POINT('Ctrl Pts',(6.60199664749281,-1.49731239212385,104.626191346862));
#34445=CARTESIAN_POINT('Ctrl Pts',(6.64140563640802,-1.31150116500202,104.635118160391));
#34446=CARTESIAN_POINT('Ctrl Pts',(6.67293772282085,-1.12436255156176,104.644044973921));
#34447=CARTESIAN_POINT('Ctrl Pts',(6.70384494949799,-0.940932395056459,
104.652794888076));
#34448=CARTESIAN_POINT('Ctrl Pts',(6.72718449348873,-0.756227260511783,
104.661544802232));
#34449=CARTESIAN_POINT('Ctrl Pts',(6.7428770737389,-0.570874564546707,104.670294716387));
#34450=CARTESIAN_POINT('Ctrl Pts',(6.75856934538641,-0.385525513637585,
104.679044458471));
#34451=CARTESIAN_POINT('Ctrl Pts',(6.76661493004087,-0.19952921242343,104.687794200555));
#34452=CARTESIAN_POINT('Ctrl Pts',(6.76698649908906,-0.0135174386057119,
104.696543942639));
#34453=CARTESIAN_POINT('Ctrl Pts',(6.76735806132403,0.172490924440569,104.705293524285));
#34454=CARTESIAN_POINT('Ctrl Pts',(6.76005588896317,0.35851447289628,104.714043105931));
#34455=CARTESIAN_POINT('Ctrl Pts',(6.74510478454625,0.543921359657171,104.722792687577));
#34456=CARTESIAN_POINT('Ctrl Pts',(6.73015393440742,0.729325093145469,104.731542120416));
#34457=CARTESIAN_POINT('Ctrl Pts',(6.70755443556964,0.914111900251446,104.740291553255));
#34458=CARTESIAN_POINT('Ctrl Pts',(6.67738304682398,1.09765415591055,104.749040986094));
#34459=CARTESIAN_POINT('Ctrl Pts',(6.64721213111954,1.28119353390787,104.757790281755));
#34460=CARTESIAN_POINT('Ctrl Pts',(6.60946960955602,1.46348811672165,104.766539577417));
#34461=CARTESIAN_POINT('Ctrl Pts',(6.56428366991306,1.64391876347732,104.775288873078));
#34462=CARTESIAN_POINT('Ctrl Pts',(6.51909837867851,1.82434682109239,104.784038043189));
#34463=CARTESIAN_POINT('Ctrl Pts',(6.46646995272065,2.00291071819982,104.7927872133));
#34464=CARTESIAN_POINT('Ctrl Pts',(6.40657713281702,2.17900400212254,104.80153638341));
#34465=CARTESIAN_POINT('Ctrl Pts',(6.34668509279221,2.35509499309224,104.810285439596));
#34466=CARTESIAN_POINT('Ctrl Pts',(6.27952894037695,2.52871516397704,104.819034495782));
#34467=CARTESIAN_POINT('Ctrl Pts',(6.20533675061622,2.69927486771016,104.827783551968));
#34468=CARTESIAN_POINT('Ctrl Pts',(6.12832117908098,2.87632521635538,104.83686555325));
#34469=CARTESIAN_POINT('Ctrl Pts',(6.04372366626265,3.05007728919629,104.845947554532));
#34470=CARTESIAN_POINT('Ctrl Pts',(5.95185378008057,3.21989527477846,104.855029555815));
#34471=CARTESIAN_POINT('Ctrl Pts',(5.86334450817573,3.38350129286403,104.863779336122));
#34472=CARTESIAN_POINT('Ctrl Pts',(5.76808562057469,3.54345567124614,104.872529116429));
#34473=CARTESIAN_POINT('Ctrl Pts',(5.6664006880471,3.69921508464963,104.881278896736));
#34474=CARTESIAN_POINT('Ctrl Pts',(5.56471941108155,3.85496889851948,104.890028362489));
#34475=CARTESIAN_POINT('Ctrl Pts',(5.45661270815352,4.00652780919313,104.898777828243));
#34476=CARTESIAN_POINT('Ctrl Pts',(5.34244776449357,4.15337704568917,104.907527293996));
#34477=CARTESIAN_POINT('Ctrl Pts',(5.22828631819855,4.30022178355933,104.916276491716));
#34478=CARTESIAN_POINT('Ctrl Pts',(5.10806717844347,4.44235690972358,104.925025689436));
#34479=CARTESIAN_POINT('Ctrl Pts',(4.98219864545016,4.57929969070322,104.933774887155));
#34480=CARTESIAN_POINT('Ctrl Pts',(4.85633329944323,4.71623900429694,104.942523863345));
#34481=CARTESIAN_POINT('Ctrl Pts',(4.72481904033947,4.84798602483326,104.951272839536));
#34482=CARTESIAN_POINT('Ctrl Pts',(4.58810250737497,4.9740933225885,104.960021815726));
#34483=CARTESIAN_POINT('Ctrl Pts',(4.45137708685943,5.10020881821873,104.968771360662));
#34484=CARTESIAN_POINT('Ctrl Pts',(4.30944892636354,5.22068366307683,104.977520905598));
#34485=CARTESIAN_POINT('Ctrl Pts',(4.16280009466965,5.33510865604614,104.986270450534));
#34486=CARTESIAN_POINT('Ctrl Pts',(4.01615988349106,5.44952692272657,104.995019481143));
#34487=CARTESIAN_POINT('Ctrl Pts',(3.86479978232562,5.55789587288396,105.003768511751));
#34488=CARTESIAN_POINT('Ctrl Pts',(3.70923383581412,5.65984746713652,105.012517542359));
#34489=CARTESIAN_POINT('Ctrl Pts',(3.55366577799894,5.76180044505164,105.021266691707));
#34490=CARTESIAN_POINT('Ctrl Pts',(3.39389200027203,5.85733573570849,105.030015841055));
#34491=CARTESIAN_POINT('Ctrl Pts',(3.23045513626413,5.94612887621726,105.038764990403));
#34492=CARTESIAN_POINT('Ctrl Pts',(3.18695122151827,5.96976399206556,105.041093854516));
#34493=CARTESIAN_POINT('Ctrl Pts',(3.14318791262789,5.99292165435268,105.043422718629));
#34494=CARTESIAN_POINT('Ctrl Pts',(3.09917575053258,6.0155962852664,105.045751582742));
#34495=CARTESIAN_POINT('Ctrl Pts',(3.09917575053265,6.01559628526636,103.045648009871));
#34496=CARTESIAN_POINT('Ctrl Pts',(2.93620633558397,6.09955651712641,103.054294205853));
#34497=CARTESIAN_POINT('Ctrl Pts',(2.76995739107423,6.1768211836711,103.062940401836));
#34498=CARTESIAN_POINT('Ctrl Pts',(2.60100041795294,6.24716622364161,103.071586597819));
#34499=CARTESIAN_POINT('Ctrl Pts',(2.52687362550646,6.27802882777806,103.075379958716));
#34500=CARTESIAN_POINT('Ctrl Pts',(2.45222578995234,6.30756014579373,103.079173319613));
#34501=CARTESIAN_POINT('Ctrl Pts',(2.37710607410156,6.3357442903316,103.08296668051));
#34502=CARTESIAN_POINT('Ctrl Pts',(2.21423320088169,6.39685251668918,103.091191360028));
#34503=CARTESIAN_POINT('Ctrl Pts',(2.04878781355926,6.45175678425539,103.099416039547));
#34504=CARTESIAN_POINT('Ctrl Pts',(1.88128287079002,6.50023566957938,103.107640719066));
#34505=CARTESIAN_POINT('Ctrl Pts',(1.71395399466591,6.54866359811035,103.115856753516));
#34506=CARTESIAN_POINT('Ctrl Pts',(1.54457021548309,6.59067949479075,103.124072787966));
#34507=CARTESIAN_POINT('Ctrl Pts',(1.3736637611641,6.62611023687838,103.132288822416));
#34508=CARTESIAN_POINT('Ctrl Pts',(1.20290271599981,6.66151083408776,103.140497866571));
#34509=CARTESIAN_POINT('Ctrl Pts',(1.0306219248412,6.69033736284446,103.148706910725));
#34510=CARTESIAN_POINT('Ctrl Pts',(0.857368139471158,6.71246667577723,103.15691595488));
#34511=CARTESIAN_POINT('Ctrl Pts',(0.684227067155946,6.73458159212722,103.165119658508));
#34512=CARTESIAN_POINT('Ctrl Pts',(0.51011461576297,6.75000792612537,103.173323362136));
#34513=CARTESIAN_POINT('Ctrl Pts',(0.335587173082654,6.75867370489672,103.181527065764));
#34514=CARTESIAN_POINT('Ctrl Pts',(0.161138330881639,6.76733558093305,103.189727074758));
#34515=CARTESIAN_POINT('Ctrl Pts',(-0.0137247730234298,6.76924294987574,
103.197927083752));
#34516=CARTESIAN_POINT('Ctrl Pts',(-0.188441097279942,6.76437572528729,
103.206127092746));
#34517=CARTESIAN_POINT('Ctrl Pts',(-0.363143450850669,6.75950888989239,
103.21432644605));
#34518=CARTESIAN_POINT('Ctrl Pts',(-0.537698689905782,6.74786854120877,
103.222525799354));
#34519=CARTESIAN_POINT('Ctrl Pts',(-0.711545861680575,6.72948671792472,
103.230725152658));
#34520=CARTESIAN_POINT('Ctrl Pts',(-0.885391900023208,6.71110501448473,
103.238924452504));
#34521=CARTESIAN_POINT('Ctrl Pts',(-1.05852952363827,6.68598196060847,103.247123752351));
#34522=CARTESIAN_POINT('Ctrl Pts',(-1.23040311181431,6.65420146842863,103.255323052198));
#34523=CARTESIAN_POINT('Ctrl Pts',(-1.40230675898107,6.62241541815501,103.263523786021));
#34524=CARTESIAN_POINT('Ctrl Pts',(-1.57294557772301,6.58396967505265,103.271724519844));
#34525=CARTESIAN_POINT('Ctrl Pts',(-1.74177429048402,6.53899925990277,103.279925253667));
#34526=CARTESIAN_POINT('Ctrl Pts',(-1.91066315723398,6.4940128217091,103.288128909427));
#34527=CARTESIAN_POINT('Ctrl Pts',(-2.07774028702214,6.44249717266287,103.296332565187));
#34528=CARTESIAN_POINT('Ctrl Pts',(-2.2424756550531,6.38463718127304,103.304536220946));
#34529=CARTESIAN_POINT('Ctrl Pts',(-2.40739973803829,6.3267109075435,103.312749274521));
#34530=CARTESIAN_POINT('Ctrl Pts',(-2.56997636116366,6.26242589036879,103.320962328097));
#34531=CARTESIAN_POINT('Ctrl Pts',(-2.72969458793926,6.19201554072461,103.329175381672));
#34532=CARTESIAN_POINT('Ctrl Pts',(-2.88950732357304,6.12156352769684,103.337393295095));
#34533=CARTESIAN_POINT('Ctrl Pts',(-3.04645796963835,6.04497911418334,103.345611208518));
#34534=CARTESIAN_POINT('Ctrl Pts',(-3.20006040701181,5.96254160501002,103.353829121941));
#34535=CARTESIAN_POINT('Ctrl Pts',(-3.35390241237484,5.87997552112997,103.362059852537));
#34536=CARTESIAN_POINT('Ctrl Pts',(-3.50438546420654,5.7915382797772,103.370290583133));
#34537=CARTESIAN_POINT('Ctrl Pts',(-3.6510514950988,5.69755315728926,103.378521313729));
#34538=CARTESIAN_POINT('Ctrl Pts',(-3.78574670354945,5.61123906269109,103.386080255405));
#34539=CARTESIAN_POINT('Ctrl Pts',(-3.91722273601703,5.52024637806843,103.39363919708));
#34540=CARTESIAN_POINT('Ctrl Pts',(-4.04515029016871,5.42485466440789,103.401198138756));
#34541=CARTESIAN_POINT('Ctrl Pts',(-4.18180096016709,5.32295838670253,103.409272509061));
#34542=CARTESIAN_POINT('Ctrl Pts',(-4.31484209244109,5.21571408620643,103.417346879367));
#34543=CARTESIAN_POINT('Ctrl Pts',(-4.44381626277234,5.10340925487268,103.425421249672));
#34544=CARTESIAN_POINT('Ctrl Pts',(-4.57263330685397,4.99124124191827,103.433485783159));
#34545=CARTESIAN_POINT('Ctrl Pts',(-4.69739297015287,4.87402520797903,103.441550316645));
#34546=CARTESIAN_POINT('Ctrl Pts',(-4.8176665367021,4.75209197524004,103.449614850132));
#34547=CARTESIAN_POINT('Ctrl Pts',(-4.93781994293716,4.63028056091864,103.457671326679));
#34548=CARTESIAN_POINT('Ctrl Pts',(-5.05349591220563,4.5037615904889,103.465727803226));
#34549=CARTESIAN_POINT('Ctrl Pts',(-5.16429867510254,4.37290614972859,103.473784279773));
#34550=CARTESIAN_POINT('Ctrl Pts',(-5.27501499522651,4.2421527958374,103.481834471059));
#34551=CARTESIAN_POINT('Ctrl Pts',(-5.38086543664533,4.10706998908007,103.489884662346));
#34552=CARTESIAN_POINT('Ctrl Pts',(-5.48149107981123,3.96806559194148,103.497934853633));
#34553=CARTESIAN_POINT('Ctrl Pts',(-5.58517308236886,3.82483913587916,103.506229557919));
#34554=CARTESIAN_POINT('Ctrl Pts',(-5.68330758303456,3.67744937432671,103.514524262204));
#34555=CARTESIAN_POINT('Ctrl Pts',(-5.77554624560037,3.52637981007881,103.52281896649));
#34556=CARTESIAN_POINT('Ctrl Pts',(-5.86499462276928,3.37988020800635,103.530862750049));
#34557=CARTESIAN_POINT('Ctrl Pts',(-5.94889847941986,3.22992054412356,103.538906533607));
#34558=CARTESIAN_POINT('Ctrl Pts',(-6.02698405823563,3.07697126437242,103.546950317166));
#34559=CARTESIAN_POINT('Ctrl Pts',(-6.10506417863741,2.92403267623042,103.554993538441));
#34560=CARTESIAN_POINT('Ctrl Pts',(-6.17732666058445,2.76810522044496,103.563036759715));
#34561=CARTESIAN_POINT('Ctrl Pts',(-6.2435439618279,2.60968346676804,103.57107998099));
#34562=CARTESIAN_POINT('Ctrl Pts',(-6.30976974087697,2.4512414303431,103.579124232038));
#34563=CARTESIAN_POINT('Ctrl Pts',(-6.36994865513251,2.2903048050044,103.587168483087));
#34564=CARTESIAN_POINT('Ctrl Pts',(-6.42390157633086,2.12738749117643,103.595212734135));
#34565=CARTESIAN_POINT('Ctrl Pts',(-6.47787208641834,1.96441706558902,103.603259607645));
#34566=CARTESIAN_POINT('Ctrl Pts',(-6.52561244701796,1.7994650206104,103.611306481155));
#34567=CARTESIAN_POINT('Ctrl Pts',(-6.56699363240196,1.63305959229667,103.619353354665));
#34568=CARTESIAN_POINT('Ctrl Pts',(-6.60841604447854,1.4664883798138,103.627408245006));
#34569=CARTESIAN_POINT('Ctrl Pts',(-6.64346654456829,1.29846125577211,103.635463135347));
#34570=CARTESIAN_POINT('Ctrl Pts',(-6.67206727133515,1.12951641279722,103.643518025688));
#34571=CARTESIAN_POINT('Ctrl Pts',(-6.70068510948697,0.960470492662015,
103.651577735149));
#34572=CARTESIAN_POINT('Ctrl Pts',(-6.72284544161039,0.790506128862421,
103.659637444609));
#34573=CARTESIAN_POINT('Ctrl Pts',(-6.73852239184888,0.620165280027229,
103.66769715407));
#34574=CARTESIAN_POINT('Ctrl Pts',(-6.75421881387219,0.449612856854959,
103.675766874211));
#34575=CARTESIAN_POINT('Ctrl Pts',(-6.7634157636552,0.278683385992217,103.683836594351));
#34576=CARTESIAN_POINT('Ctrl Pts',(-6.76613942338065,0.107918040077253,
103.691906314492));
#34577=CARTESIAN_POINT('Ctrl Pts',(-6.76671336282573,0.0719337477086487,
103.693606795156));
#34578=CARTESIAN_POINT('Ctrl Pts',(-6.76700004258492,0.0359567218966393,
103.695307275821));
#34579=CARTESIAN_POINT('Ctrl Pts',(-6.76699999999526,-8.01352280423633E-6,
103.697007756485));
#34580=CARTESIAN_POINT('',(-6.76699950316282,0.00259310511624294,103.30282021622));
#34581=CARTESIAN_POINT('Ctrl Pts',(3.09917575053253,6.01559628526642,102.651329234227));
#34582=CARTESIAN_POINT('Ctrl Pts',(2.94465102080322,6.09520589876518,102.659561891668));
#34583=CARTESIAN_POINT('Ctrl Pts',(2.78683225452528,6.16897342073497,102.667794549109));
#34584=CARTESIAN_POINT('Ctrl Pts',(2.6261999455191,6.23661469437992,102.67602720655));
#34585=CARTESIAN_POINT('Ctrl Pts',(2.46575773407981,6.30417591911303,102.684250121193));
#34586=CARTESIAN_POINT('Ctrl Pts',(2.30250893698856,6.36562519448207,102.692473035836));
#34587=CARTESIAN_POINT('Ctrl Pts',(2.13695934262842,6.42072377290545,102.700695950479));
#34588=CARTESIAN_POINT('Ctrl Pts',(1.97157253052235,6.47576817378265,102.708910779662));
#34589=CARTESIAN_POINT('Ctrl Pts',(1.80388976419275,6.52447420150795,102.717125608845));
#34590=CARTESIAN_POINT('Ctrl Pts',(1.63443763868945,6.56665079056556,102.725340438028));
#34591=CARTESIAN_POINT('Ctrl Pts',(1.46511822916006,6.60879434665249,102.733548833305));
#34592=CARTESIAN_POINT('Ctrl Pts',(1.29403256669579,6.64441856386078,102.741757228583));
#34593=CARTESIAN_POINT('Ctrl Pts',(1.12172336251686,6.67338187862675,102.74996562386));
#34594=CARTESIAN_POINT('Ctrl Pts',(0.949514645628381,6.70232830256534,102.758169232165));
#34595=CARTESIAN_POINT('Ctrl Pts',(0.776084160813869,6.72462150336137,102.766372840469));
#34596=CARTESIAN_POINT('Ctrl Pts',(0.601985888318103,6.74017076862789,102.774576448774));
#34597=CARTESIAN_POINT('Ctrl Pts',(0.42793743962812,6.75571558397333,102.782777709353));
#34598=CARTESIAN_POINT('Ctrl Pts',(0.253221939909041,6.76452027247827,102.790978969932));
#34599=CARTESIAN_POINT('Ctrl Pts',(0.0783998453697731,6.76654582961248,
102.799180230511));
#34600=CARTESIAN_POINT('Ctrl Pts',(-0.0963993126394692,6.76857112099508,
102.807380415091));
#34601=CARTESIAN_POINT('Ctrl Pts',(-0.27130467947958,6.76381904749359,102.815580599671));
#34602=CARTESIAN_POINT('Ctrl Pts',(-0.445754415818094,6.75230271839013,
102.823780784251));
#34603=CARTESIAN_POINT('Ctrl Pts',(-0.620212878314131,6.74078581322788,
102.831981379012));
#34604=CARTESIAN_POINT('Ctrl Pts',(-0.794215307374695,6.72250400195956,
102.840181973774));
#34605=CARTESIAN_POINT('Ctrl Pts',(-0.967203545148345,6.69752240028001,
102.848382568535));
#34606=CARTESIAN_POINT('Ctrl Pts',(-1.14023178482971,6.67253502183935,102.856585059608));
#34607=CARTESIAN_POINT('Ctrl Pts',(-1.31224501159702,6.64084481848889,102.86478755068));
#34608=CARTESIAN_POINT('Ctrl Pts',(-1.48269377772703,6.60256830040323,102.872990041752));
#34609=CARTESIAN_POINT('Ctrl Pts',(-1.65330245823249,6.56425587143582,102.88120022837));
#34610=CARTESIAN_POINT('Ctrl Pts',(-1.82234339568558,6.51934486103658,102.889410414987));
#34611=CARTESIAN_POINT('Ctrl Pts',(-1.98927995375338,6.4680023396405,102.897620601605));
#34612=CARTESIAN_POINT('Ctrl Pts',(-2.15629740973563,6.41663493751757,102.905834766902));
#34613=CARTESIAN_POINT('Ctrl Pts',(-2.32120811518539,6.35882992870066,102.914048932198));
#34614=CARTESIAN_POINT('Ctrl Pts',(-2.48349410094345,6.29480309863455,102.922263097495));
#34615=CARTESIAN_POINT('Ctrl Pts',(-2.6459998187415,6.23068957749699,102.93048838461));
#34616=CARTESIAN_POINT('Ctrl Pts',(-2.80587338684529,6.16033754424743,102.938713671725));
#34617=CARTESIAN_POINT('Ctrl Pts',(-2.96261910462237,6.08400994747104,102.946938958841));
#34618=CARTESIAN_POINT('Ctrl Pts',(-3.09778229647575,6.01819199880167,102.954031695256));
#34619=CARTESIAN_POINT('Ctrl Pts',(-3.230619975244,5.94793158111742,102.961124431671));
#34620=CARTESIAN_POINT('Ctrl Pts',(-3.36083145644398,5.87342327108958,102.968217168086));
#34621=CARTESIAN_POINT('Ctrl Pts',(-3.51955779805292,5.782598473144,102.976863134577));
#34622=CARTESIAN_POINT('Ctrl Pts',(-3.67474162686808,5.68525477980905,102.985509101068));
#34623=CARTESIAN_POINT('Ctrl Pts',(-3.82584466453705,5.58168447718369,102.994155067559));
#34624=CARTESIAN_POINT('Ctrl Pts',(-3.97675442087866,5.47824665505559,103.002789974683));
#34625=CARTESIAN_POINT('Ctrl Pts',(-4.12359354450498,5.36859827726257,103.011424881808));
#34626=CARTESIAN_POINT('Ctrl Pts',(-4.26585000875932,5.25307649884981,103.020059788932));
#34627=CARTESIAN_POINT('Ctrl Pts',(-4.41282927280917,5.13371949063343,103.028981368004));
#34628=CARTESIAN_POINT('Ctrl Pts',(-4.55491607446304,5.00809252951917,103.037902947075));
#34629=CARTESIAN_POINT('Ctrl Pts',(-4.69157743729695,4.87661667038185,103.046824526147));
#34630=CARTESIAN_POINT('Ctrl Pts',(-4.82348223191121,4.74971689537142,103.055435585122));
#34631=CARTESIAN_POINT('Ctrl Pts',(-4.95033261604947,4.61736871822652,103.064046644098));
#34632=CARTESIAN_POINT('Ctrl Pts',(-5.0716818674175,4.47999241469319,103.072657703074));
#34633=CARTESIAN_POINT('Ctrl Pts',(-5.19291668083943,4.34274566335603,103.081260641423));
#34634=CARTESIAN_POINT('Ctrl Pts',(-5.3086605034215,4.20048046725272,103.089863579773));
#34635=CARTESIAN_POINT('Ctrl Pts',(-5.4185033873348,4.05365391239081,103.098466518122));
#34636=CARTESIAN_POINT('Ctrl Pts',(-5.52822327262892,3.90699176930382,103.107059823171));
#34637=CARTESIAN_POINT('Ctrl Pts',(-5.63205521911334,3.75577870077789,103.11565312822));
#34638=CARTESIAN_POINT('Ctrl Pts',(-5.72962937647881,3.6005049934962,103.124246433269));
#34639=CARTESIAN_POINT('Ctrl Pts',(-5.74050073473508,3.58320496093413,103.125203868109));
#34640=CARTESIAN_POINT('Ctrl Pts',(-5.75129445271447,3.56585455464649,103.12616130295));
#34641=CARTESIAN_POINT('Ctrl Pts',(-5.76201005039754,3.54845447753213,103.12711873779));
#34642=CARTESIAN_POINT('Ctrl Pts',(-5.85821365169512,3.39223826535554,103.135714495338));
#34643=CARTESIAN_POINT('Ctrl Pts',(-5.94800424912497,3.23219914504976,103.144310252885));
#34644=CARTESIAN_POINT('Ctrl Pts',(-6.03110494216396,3.06888614591767,103.152906010433));
#34645=CARTESIAN_POINT('Ctrl Pts',(-6.11428317097482,2.90542077020509,103.161509788114));
#34646=CARTESIAN_POINT('Ctrl Pts',(-6.1907588978608,2.73867569059632,103.170113565796));
#34647=CARTESIAN_POINT('Ctrl Pts',(-6.26030291329682,2.56922097799457,103.178717343477));
#34648=CARTESIAN_POINT('Ctrl Pts',(-6.33258006935235,2.39310654700761,103.187659257145));
#34649=CARTESIAN_POINT('Ctrl Pts',(-6.39736952032273,2.21406554749393,103.196601170813));
#34650=CARTESIAN_POINT('Ctrl Pts',(-6.45447096379186,2.03275516911598,103.205543084481));
#34651=CARTESIAN_POINT('Ctrl Pts',(-6.50956271757872,1.85782602341062,103.214170286812));
#34652=CARTESIAN_POINT('Ctrl Pts',(-6.55749837040686,1.68078481732085,103.222797489143));
#34653=CARTESIAN_POINT('Ctrl Pts',(-6.59815021984394,1.50223256401043,103.231424691473));
#34654=CARTESIAN_POINT('Ctrl Pts',(-6.63884078394521,1.32351026700897,103.240060109894));
#34655=CARTESIAN_POINT('Ctrl Pts',(-6.67223363982516,1.14327434944384,103.248695528314));
#34656=CARTESIAN_POINT('Ctrl Pts',(-6.69825261285262,0.962133532527059,
103.257330946734));
#34657=CARTESIAN_POINT('Ctrl Pts',(-6.72431002520673,0.78072510585407,103.265979122755));
#34658=CARTESIAN_POINT('Ctrl Pts',(-6.74297174975277,0.598409411195861,
103.274627298777));
#34659=CARTESIAN_POINT('Ctrl Pts',(-6.75421349743395,0.415799267773559,
103.283275474798));
#34660=CARTESIAN_POINT('Ctrl Pts',(-6.75540283171353,0.396479806998448,
103.284190419029));
#34661=CARTESIAN_POINT('Ctrl Pts',(-6.7565091634507,0.377157049266722,103.285105363261));
#34662=CARTESIAN_POINT('Ctrl Pts',(-6.7575324979539,0.357831718964357,103.286020307493));
#34663=CARTESIAN_POINT('Ctrl Pts',(-6.76379587649999,0.239549907070366,
103.291620277059));
#34664=CARTESIAN_POINT('Ctrl Pts',(-6.76695409214459,0.121098237013267,
103.297220246624));
#34665=CARTESIAN_POINT('Ctrl Pts',(-6.76699950316258,0.00259310574074797,
103.30282021619));
#34666=CARTESIAN_POINT('Ctrl Pts',(-6.76699950316282,0.00259310511624744,
103.30282021622));
#34667=CARTESIAN_POINT('Ctrl Pts',(-6.76706574277703,-0.170266619558,103.310988716493));
#34668=CARTESIAN_POINT('Ctrl Pts',(-6.7605043375378,-0.343364296386368,
103.319157216767));
#34669=CARTESIAN_POINT('Ctrl Pts',(-6.74728687381096,-0.516148081947727,
103.327325717041));
#34670=CARTESIAN_POINT('Ctrl Pts',(-6.73408283282203,-0.68875640030021,
103.335485921953));
#34671=CARTESIAN_POINT('Ctrl Pts',(-6.71423621859555,-0.861051102120788,
103.343646126866));
#34672=CARTESIAN_POINT('Ctrl Pts',(-6.68777061728648,-1.03247913807475,
103.351806331778));
#34673=CARTESIAN_POINT('Ctrl Pts',(-6.66132639162829,-1.20376871558966,
103.359959945883));
#34674=CARTESIAN_POINT('Ctrl Pts',(-6.62827387931158,-1.37419266334526,
103.368113559988));
#34675=CARTESIAN_POINT('Ctrl Pts',(-6.58868857281771,-1.54320183074715,
103.376267174092));
#34676=CARTESIAN_POINT('Ctrl Pts',(-6.54912701333018,-1.71210961048463,
103.384415896889));
#34677=CARTESIAN_POINT('Ctrl Pts',(-6.50304054736499,-1.87960394697185,
103.392564619686));
#34678=CARTESIAN_POINT('Ctrl Pts',(-6.45055597016453,-2.04514465888718,
103.400713342482));
#34679=CARTESIAN_POINT('Ctrl Pts',(-6.39604769413584,-2.21706828484309,
103.4091762635));
#34680=CARTESIAN_POINT('Ctrl Pts',(-6.33463814294162,-2.3868842279124,103.417639184517));
#34681=CARTESIAN_POINT('Ctrl Pts',(-6.26652689360036,-2.55400268045738,
103.426102105535));
#34682=CARTESIAN_POINT('Ctrl Pts',(-6.20097048049423,-2.71485256089052,
103.434247584463));
#34683=CARTESIAN_POINT('Ctrl Pts',(-6.12920615613764,-2.87320328257457,
103.442393063392));
#34684=CARTESIAN_POINT('Ctrl Pts',(-6.05146148877742,-3.02854797714082,
103.45053854232));
#34685=CARTESIAN_POINT('Ctrl Pts',(-5.9737115727459,-3.18390315928478,103.458684571164));
#34686=CARTESIAN_POINT('Ctrl Pts',(-5.88998067207161,-3.33625158434668,
103.466830600007));
#34687=CARTESIAN_POINT('Ctrl Pts',(-5.80054284650386,-3.48510999623726,
103.47497662885));
#34688=CARTESIAN_POINT('Ctrl Pts',(-5.71108215100214,-3.63400647235883,
103.483124740695));
#34689=CARTESIAN_POINT('Ctrl Pts',(-5.61591181184105,-3.77941084611467,
103.49127285254));
#34690=CARTESIAN_POINT('Ctrl Pts',(-5.51534982011552,-3.92086793475013,
103.499420964385));
#34691=CARTESIAN_POINT('Ctrl Pts',(-5.41474318760003,-4.0623878180466,103.507572693284));
#34692=CARTESIAN_POINT('Ctrl Pts',(-5.30874034676697,-4.19995663042744,
103.515724422183));
#34693=CARTESIAN_POINT('Ctrl Pts',(-5.19770022153839,-4.33315144058222,
103.523876151082));
#34694=CARTESIAN_POINT('Ctrl Pts',(-5.08653198099771,-4.46649992756902,
103.532037285241));
#34695=CARTESIAN_POINT('Ctrl Pts',(-4.97031508416509,-4.59546405607798,
103.540198419401));
#34696=CARTESIAN_POINT('Ctrl Pts',(-4.84944661176212,-4.7196564027129,103.54835955356));
#34697=CARTESIAN_POINT('Ctrl Pts',(-4.72849558309742,-4.84393357590077,
103.556526261983));
#34698=CARTESIAN_POINT('Ctrl Pts',(-4.60288691110054,-4.96343222345064,
103.564692970406));
#34699=CARTESIAN_POINT('Ctrl Pts',(-4.47305131585109,-5.07780473489902,
103.572859678829));
#34700=CARTESIAN_POINT('Ctrl Pts',(-4.34303828673217,-5.19233354830163,
103.58103754791));
#34701=CARTESIAN_POINT('Ctrl Pts',(-4.20878708258286,-5.30172201124552,
103.589215416991));
#34702=CARTESIAN_POINT('Ctrl Pts',(-4.07075860683747,-5.40566493272185,
103.597393286072));
#34703=CARTESIAN_POINT('Ctrl Pts',(-4.03458189261365,-5.43290795881143,
103.599536673015));
#34704=CARTESIAN_POINT('Ctrl Pts',(-3.99814583848349,-5.45977714901582,
103.601680059958));
#34705=CARTESIAN_POINT('Ctrl Pts',(-3.96145902307961,-5.48626752979301,
103.603823446901));
#34706=CARTESIAN_POINT('Ctrl Pts',(-3.82186789696318,-5.58706183541023,
103.611978905308));
#34707=CARTESIAN_POINT('Ctrl Pts',(-3.67819970009139,-5.68268948867638,
103.620134363715));
#34708=CARTESIAN_POINT('Ctrl Pts',(-3.53087616309073,-5.77279849994071,
103.628289822122));
#34709=CARTESIAN_POINT('Ctrl Pts',(-3.38373193819997,-5.86279783669369,
103.636435354264));
#34710=CARTESIAN_POINT('Ctrl Pts',(-3.23294153755421,-5.94729171315061,
103.644580886406));
#34711=CARTESIAN_POINT('Ctrl Pts',(-3.07895901496569,-6.02596883365335,
103.652726418548));
#34712=CARTESIAN_POINT('Ctrl Pts',(-2.92513152991245,-6.10456673797856,
103.660863749348));
#34713=CARTESIAN_POINT('Ctrl Pts',(-2.76811864444988,-6.17735938076264,
103.669001080149));
#34714=CARTESIAN_POINT('Ctrl Pts',(-2.60840259564971,-6.24407918743892,
103.677138410949));
#34715=CARTESIAN_POINT('Ctrl Pts',(-2.44881379237286,-6.3107458385508,103.685269258751));
#34716=CARTESIAN_POINT('Ctrl Pts',(-2.28652644954427,-6.37134914681978,
103.693400106553));
#34717=CARTESIAN_POINT('Ctrl Pts',(-2.12204656300972,-6.42566785512749,
103.701530954355));
#34718=CARTESIAN_POINT('Ctrl Pts',(-1.95766316549192,-6.47995469839159,
103.709657032349));
#34719=CARTESIAN_POINT('Ctrl Pts',(-1.79109013193453,-6.52796416943831,
103.717783110343));
#34720=CARTESIAN_POINT('Ctrl Pts',(-1.62285255312617,-6.56952346755926,
103.725909188337));
#34721=CARTESIAN_POINT('Ctrl Pts',(-1.45401843459086,-6.61123012736082,
103.734064079919));
#34722=CARTESIAN_POINT('Ctrl Pts',(-1.28350829025956,-6.64644065036041,
103.742218971501));
#34723=CARTESIAN_POINT('Ctrl Pts',(-1.11186784727553,-6.67503100293886,
103.750373863083));
#34724=CARTESIAN_POINT('Ctrl Pts',(-0.940896742006795,-6.70350986313857,
103.758496953439));
#34725=CARTESIAN_POINT('Ctrl Pts',(-0.768804503938351,-6.72542004930831,
103.766620043796));
#34726=CARTESIAN_POINT('Ctrl Pts',(-0.596140021328421,-6.7406903262923,
103.774743134152));
#34727=CARTESIAN_POINT('Ctrl Pts',(-0.423461980314886,-6.75596180236816,
103.78286686237));
#34728=CARTESIAN_POINT('Ctrl Pts',(-0.250211969660003,-6.76459229842574,
103.790990590589));
#34729=CARTESIAN_POINT('Ctrl Pts',(-0.0769430694369275,-6.76656255155198,
103.799114318807));
#34730=CARTESIAN_POINT('Ctrl Pts',(0.0963724008534442,-6.76853333422981,
103.807240230468));
#34731=CARTESIAN_POINT('Ctrl Pts',(0.269706405172214,-6.7638403054025,103.815366142128));
#34732=CARTESIAN_POINT('Ctrl Pts',(0.442506837496675,-6.75251632347296,
103.823492053788));
#34733=CARTESIAN_POINT('Ctrl Pts',(0.616412346548741,-6.74111992350183,
103.831669931498));
#34734=CARTESIAN_POINT('Ctrl Pts',(0.789777060626473,-6.72300748934226,
103.839847809208));
#34735=CARTESIAN_POINT('Ctrl Pts',(0.962045255402203,-6.69826529233936,
103.848025686919));
#34736=CARTESIAN_POINT('Ctrl Pts',(1.13349125144722,-6.67364118447647,103.856164533392));
#34737=CARTESIAN_POINT('Ctrl Pts',(1.30385082336201,-6.64245058633746,103.864303379865));
#34738=CARTESIAN_POINT('Ctrl Pts',(1.47258852360663,-6.60482944822514,103.872442226339));
#34739=CARTESIAN_POINT('Ctrl Pts',(1.64254003980044,-6.56693768216541,103.880639619667));
#34740=CARTESIAN_POINT('Ctrl Pts',(1.81084589720142,-6.52252260743711,103.888837012996));
#34741=CARTESIAN_POINT('Ctrl Pts',(1.97697700707738,-6.47177339787846,103.897034406324));
#34742=CARTESIAN_POINT('Ctrl Pts',(2.14310811695347,-6.42102418831978,103.905231799652));
#34743=CARTESIAN_POINT('Ctrl Pts',(2.30706414786201,-6.36394102403529,103.913429192981));
#34744=CARTESIAN_POINT('Ctrl Pts',(2.46833918939741,-6.30076111641165,103.921626586309));
#34745=CARTESIAN_POINT('Ctrl Pts',(2.63018115541685,-6.23735911467977,103.929852795646));
#34746=CARTESIAN_POINT('Ctrl Pts',(2.78980496348707,-6.16762884505108,103.938079004983));
#34747=CARTESIAN_POINT('Ctrl Pts',(2.94668072219698,-6.0917453756237,103.94630521432));
#34748=CARTESIAN_POINT('Ctrl Pts',(3.1033802377122,-6.01594715802353,103.954522181863));
#34749=CARTESIAN_POINT('Ctrl Pts',(3.2573375316345,-5.93400966074938,103.962739149406));
#34750=CARTESIAN_POINT('Ctrl Pts',(3.40804033492672,-5.84615686374498,103.97095611695));
#34751=CARTESIAN_POINT('Ctrl Pts',(3.55860407733491,-5.75838513283458,103.979165502293));
#34752=CARTESIAN_POINT('Ctrl Pts',(3.70591900196913,-5.66470915216056,103.987374887636));
#34753=CARTESIAN_POINT('Ctrl Pts',(3.84949512797683,-5.56539991911477,103.99558427298));
#34754=CARTESIAN_POINT('Ctrl Pts',(3.99296757686672,-5.46616239781758,104.00378773028));
#34755=CARTESIAN_POINT('Ctrl Pts',(4.13270631092355,-5.36129992970159,104.011991187581));
#34756=CARTESIAN_POINT('Ctrl Pts',(4.26824809427468,-5.25112818408773,104.020194644882));
#34757=CARTESIAN_POINT('Ctrl Pts',(4.40371919149893,-5.14101389392265,104.028393824013));
#34758=CARTESIAN_POINT('Ctrl Pts',(4.53499742074772,-5.02559606793333,104.036593003145));
#34759=CARTESIAN_POINT('Ctrl Pts',(4.6616504952531,-4.90523227381808,104.044792182277));
#34760=CARTESIAN_POINT('Ctrl Pts',(4.78827970558998,-4.78489115883538,104.052989816507));
#34761=CARTESIAN_POINT('Ctrl Pts',(4.91028523309642,-4.65960617432333,104.061187450737));
#34762=CARTESIAN_POINT('Ctrl Pts',(5.02726949482033,-4.52977377210484,104.069385084966));
#34763=CARTESIAN_POINT('Ctrl Pts',(5.14424531249196,-4.39995074133151,104.077582127482));
#34764=CARTESIAN_POINT('Ctrl Pts',(5.25620034544828,-4.26558121242906,104.085779169998));
#34765=CARTESIAN_POINT('Ctrl Pts',(5.36277541842275,-4.12709689873653,104.093976212513));
#34766=CARTESIAN_POINT('Ctrl Pts',(5.46936216853308,-3.98859741170093,104.102174153156));
#34767=CARTESIAN_POINT('Ctrl Pts',(5.57056756547256,-3.84598252596951,104.110372093799));
#34768=CARTESIAN_POINT('Ctrl Pts',(5.66607408704463,-3.69971531879432,104.118570034442));
#34769=CARTESIAN_POINT('Ctrl Pts',(5.76160843121589,-3.55340550160872,104.126770363278));
#34770=CARTESIAN_POINT('Ctrl Pts',(5.85144039710096,-3.40344154390989,104.134970692114));
#34771=CARTESIAN_POINT('Ctrl Pts',(5.93529695554827,-3.25031368477867,104.14317102095));
#34772=CARTESIAN_POINT('Ctrl Pts',(6.01924089470567,-3.09702626244435,104.151379894741));
#34773=CARTESIAN_POINT('Ctrl Pts',(6.09719681425231,-2.94056866704617,104.159588768533));
#34774=CARTESIAN_POINT('Ctrl Pts',(6.16893821169109,-2.78145471657144,104.167797642324));
#34775=CARTESIAN_POINT('Ctrl Pts',(6.24071811194648,-2.62225537139473,104.176010921727));
#34776=CARTESIAN_POINT('Ctrl Pts',(6.30627670660361,-2.46039716120847,104.184224201131));
#34777=CARTESIAN_POINT('Ctrl Pts',(6.36543651163292,-2.29641176977704,104.192437480534));
#34778=CARTESIAN_POINT('Ctrl Pts',(6.42468284717531,-2.13218652393684,104.20066277315));
#34779=CARTESIAN_POINT('Ctrl Pts',(6.47751158071383,-1.96582822088184,104.208888065765));
#34780=CARTESIAN_POINT('Ctrl Pts',(6.52379541334976,-1.79788275612082,104.217113358381));
#34781=CARTESIAN_POINT('Ctrl Pts',(6.56565358015001,-1.64599625759747,104.224552147493));
#34782=CARTESIAN_POINT('Ctrl Pts',(6.60215927446537,-1.49281195096278,104.231990936605));
#34783=CARTESIAN_POINT('Ctrl Pts',(6.63325475579004,-1.33873834067336,104.239429725717));
#34784=CARTESIAN_POINT('Ctrl Pts',(6.66764176102705,-1.16835570569849,104.247655926736));
#34785=CARTESIAN_POINT('Ctrl Pts',(6.69550790612459,-0.996409170636312,
104.255882127755));
#34786=CARTESIAN_POINT('Ctrl Pts',(6.71671327765216,-0.823438975159202,
104.264108328773));
#34787=CARTESIAN_POINT('Ctrl Pts',(6.73789482941407,-0.65066307524144,104.272325289389));
#34788=CARTESIAN_POINT('Ctrl Pts',(6.75243046300857,-0.47686615734503,104.280542250005));
#34789=CARTESIAN_POINT('Ctrl Pts',(6.76023092441601,-0.30260014634741,104.288759210621));
#34790=CARTESIAN_POINT('Ctrl Pts',(6.76802418926368,-0.128494909911465,
104.296968590422));
#34791=CARTESIAN_POINT('Ctrl Pts',(6.76909464089102,0.0460782017084419,
104.305177970224));
#34792=CARTESIAN_POINT('Ctrl Pts',(6.76340462002218,0.220560526528714,104.313387350026));
#34793=CARTESIAN_POINT('Ctrl Pts',(6.75771870699421,0.394916885971801,104.321590803166));
#34794=CARTESIAN_POINT('Ctrl Pts',(6.74528205451015,0.569182232170582,104.329794256306));
#34795=CARTESIAN_POINT('Ctrl Pts',(6.7261090409509,0.742796182837956,104.337997709447));
#34796=CARTESIAN_POINT('Ctrl Pts',(6.70694602305525,0.916319621565553,104.346196885797));
#34797=CARTESIAN_POINT('Ctrl Pts',(6.68105367976009,1.08919198568131,104.354396062147));
#34798=CARTESIAN_POINT('Ctrl Pts',(6.64849837335323,1.26085620889911,104.362595238497));
#34799=CARTESIAN_POINT('Ctrl Pts',(6.6159491927186,1.43248813090258,104.370792872049));
#34800=CARTESIAN_POINT('Ctrl Pts',(6.57673960692468,1.60291201167313,104.3789905056));
#34801=CARTESIAN_POINT('Ctrl Pts',(6.53098746266332,1.7715788897293,104.387188139151));
#34802=CARTESIAN_POINT('Ctrl Pts',(6.48523861367921,1.94023361963083,104.395385182272));
#34803=CARTESIAN_POINT('Ctrl Pts',(6.43294823774539,2.10713125244343,104.403582225392));
#34804=CARTESIAN_POINT('Ctrl Pts',(6.37428462750736,2.27173600744526,104.411779268513));
#34805=CARTESIAN_POINT('Ctrl Pts',(6.31561458047564,2.43635882350479,104.419977211044));
#34806=CARTESIAN_POINT('Ctrl Pts',(6.25057002637754,2.59868792259207,104.428175153575));
#34807=CARTESIAN_POINT('Ctrl Pts',(6.17936818585291,2.7582055441299,104.436373096107));
#34808=CARTESIAN_POINT('Ctrl Pts',(6.10814559192847,2.91776966071552,104.444573428115));
#34809=CARTESIAN_POINT('Ctrl Pts',(6.03076228294856,3.07452034001717,104.452773760124));
#34810=CARTESIAN_POINT('Ctrl Pts',(5.94748241403092,3.22796250517148,104.460974092132));
#34811=CARTESIAN_POINT('Ctrl Pts',(5.86411574498172,3.38156459853289,104.469182971103));
#34812=CARTESIAN_POINT('Ctrl Pts',(5.77484040891931,3.53185097277528,104.477391850074));
#34813=CARTESIAN_POINT('Ctrl Pts',(5.67996558559512,3.67835288498196,104.485600729044));
#34814=CARTESIAN_POINT('Ctrl Pts',(5.58503983126507,3.82493344281334,104.493814014732));
#34815=CARTESIAN_POINT('Ctrl Pts',(5.4845088035225,3.96772519557063,104.502027300419));
#34816=CARTESIAN_POINT('Ctrl Pts',(5.37872325443189,4.10629092396456,104.510240586106));
#34817=CARTESIAN_POINT('Ctrl Pts',(5.27278295412074,4.24505935694127,104.518465886818));
#34818=CARTESIAN_POINT('Ctrl Pts',(5.16157299957407,4.37958913449246,104.526691187531));
#34819=CARTESIAN_POINT('Ctrl Pts',(5.04548327590348,4.50947752101929,104.534916488243));
#34820=CARTESIAN_POINT('Ctrl Pts',(4.94049412449559,4.62694589847781,104.542355280536));
#34821=CARTESIAN_POINT('Ctrl Pts',(4.83151441907065,4.74061841286867,104.54979407283));
#34822=CARTESIAN_POINT('Ctrl Pts',(4.71885624377911,4.85022522678555,104.557232865124));
#34823=CARTESIAN_POINT('Ctrl Pts',(4.59540267829461,4.9703350363437,104.565384474443));
#34824=CARTESIAN_POINT('Ctrl Pts',(4.46716728355509,5.0859161893053,104.573536083762));
#34825=CARTESIAN_POINT('Ctrl Pts',(4.33451801718587,5.19656064707139,104.581687693081));
#34826=CARTESIAN_POINT('Ctrl Pts',(4.20200393016589,5.3070923500051,104.589830995312));
#34827=CARTESIAN_POINT('Ctrl Pts',(4.06508519780222,5.41269713461875,104.597974297542));
#34828=CARTESIAN_POINT('Ctrl Pts',(3.92416764446704,5.51300256648933,104.606117599772));
#34829=CARTESIAN_POINT('Ctrl Pts',(3.78339917756085,5.61320187830396,104.614252286639));
#34830=CARTESIAN_POINT('Ctrl Pts',(3.63864061179269,5.70811279368045,104.622386973507));
#34831=CARTESIAN_POINT('Ctrl Pts',(3.49033166315081,5.79740233908317,104.630521660374));
#34832=CARTESIAN_POINT('Ctrl Pts',(3.36248390330737,5.87437320605857,104.637534059171));
#34833=CARTESIAN_POINT('Ctrl Pts',(3.2319984966419,5.94716731923532,104.644546457968));
#34834=CARTESIAN_POINT('Ctrl Pts',(3.09917575053253,6.01559628526642,104.651558856765));
#34835=CARTESIAN_POINT('Origin',(0.,0.,-3.69717978381041));
#34836=CARTESIAN_POINT('',(3.0991757505325,6.01559628526643,107.045813349661));
#34837=CARTESIAN_POINT('',(3.09917575053261,6.01559628526638,106.651392015122));
#34838=CARTESIAN_POINT('',(3.09917575053259,6.01559628526639,-3.69717978381041));
#34839=CARTESIAN_POINT('',(-6.76699999997695,1.76623100267976E-5,105.69756051241));
#34840=CARTESIAN_POINT('Ctrl Pts',(-6.76699999997695,1.76623100267975E-5,
105.69756051241));
#34841=CARTESIAN_POINT('Ctrl Pts',(-6.76700044466366,-0.170356143476382,
105.705581476401));
#34842=CARTESIAN_POINT('Ctrl Pts',(-6.76056227767791,-0.340943091970037,
105.713602440391));
#34843=CARTESIAN_POINT('Ctrl Pts',(-6.747663184599,-0.511204995287844,105.721623404382));
#34844=CARTESIAN_POINT('Ctrl Pts',(-6.73477403793164,-0.681335610696416,
105.729638183456));
#34845=CARTESIAN_POINT('Ctrl Pts',(-6.71543390845697,-0.85114130644225,
105.737652962531));
#34846=CARTESIAN_POINT('Ctrl Pts',(-6.68967254174539,-1.02008346924053,
105.745667741605));
#34847=CARTESIAN_POINT('Ctrl Pts',(-6.66270217275019,-1.19695422771114,
105.754058660902));
#34848=CARTESIAN_POINT('Ctrl Pts',(-6.62869328459728,-1.37287802099367,
105.762449580199));
#34849=CARTESIAN_POINT('Ctrl Pts',(-6.5877410844805,-1.54724154670424,105.770840499496));
#34850=CARTESIAN_POINT('Ctrl Pts',(-6.54865406306637,-1.71366363987277,
105.778849252171));
#34851=CARTESIAN_POINT('Ctrl Pts',(-6.50324228412838,-1.87866403626064,
105.786858004846));
#34852=CARTESIAN_POINT('Ctrl Pts',(-6.45164093027403,-2.04171944860524,
105.794866757521));
#34853=CARTESIAN_POINT('Ctrl Pts',(-6.40004205710617,-2.20476702221444,
105.802875125183));
#34854=CARTESIAN_POINT('Ctrl Pts',(-6.34225431417973,-2.36586943871361,
105.810883492845));
#34855=CARTESIAN_POINT('Ctrl Pts',(-6.27846270017658,-2.52451879028288,
105.818891860507));
#34856=CARTESIAN_POINT('Ctrl Pts',(-6.21466134671133,-2.68319236383449,
105.826901450857));
#34857=CARTESIAN_POINT('Ctrl Pts',(-6.14485443867364,-2.83941177790795,
105.834911041206));
#34858=CARTESIAN_POINT('Ctrl Pts',(-6.06927496196964,-2.99268949876335,
105.842920631555));
#34859=CARTESIAN_POINT('Ctrl Pts',(-5.99366876803175,-3.14602140306771,
105.850933053283));
#34860=CARTESIAN_POINT('Ctrl Pts',(-5.91228611141086,-3.2964092076703,105.85894547501));
#34861=CARTESIAN_POINT('Ctrl Pts',(-5.82540562324274,-3.44339052747315,
105.866957896738));
#34862=CARTESIAN_POINT('Ctrl Pts',(-5.73843226888166,-3.59052895499829,
105.87497888291));
#34863=CARTESIAN_POINT('Ctrl Pts',(-5.6459495436579,-3.73425330528655,105.882999869082));
#34864=CARTESIAN_POINT('Ctrl Pts',(-5.54827940201112,-3.87413018330814,
105.891020855254));
#34865=CARTESIAN_POINT('Ctrl Pts',(-5.45054816258855,-4.01409456162396,
105.899046858972));
#34866=CARTESIAN_POINT('Ctrl Pts',(-5.34762327212463,-4.15020637693373,
105.90707286269));
#34867=CARTESIAN_POINT('Ctrl Pts',(-5.23986615537025,-4.28206628554549,
105.915098866407));
#34868=CARTESIAN_POINT('Ctrl Pts',(-5.13196415113807,-4.41410348963581,
105.923135661686));
#34869=CARTESIAN_POINT('Ctrl Pts',(-5.01921720128658,-4.54187709697175,
105.931172456964));
#34870=CARTESIAN_POINT('Ctrl Pts',(-4.90202308582014,-4.66502504452938,
105.939209252242));
#34871=CARTESIAN_POINT('Ctrl Pts',(-4.86391226420427,-4.70507201653861,
105.941822769738));
#34872=CARTESIAN_POINT('Ctrl Pts',(-4.8253314061741,-4.74463014141675,105.944436287234));
#34873=CARTESIAN_POINT('Ctrl Pts',(-4.78629490478964,-4.78368791670033,
105.94704980473));
#34874=CARTESIAN_POINT('Ctrl Pts',(-4.66344512132277,-4.9066046501706,105.955274672408));
#34875=CARTESIAN_POINT('Ctrl Pts',(-4.53568489280584,-5.02495855146323,
105.963499540086));
#34876=CARTESIAN_POINT('Ctrl Pts',(-4.40338642834206,-5.13833406491764,
105.971724407763));
#34877=CARTESIAN_POINT('Ctrl Pts',(-4.27123701290651,-5.25158184816615,
105.979940009207));
#34878=CARTESIAN_POINT('Ctrl Pts',(-4.13455981241164,-5.35986218062053,
105.98815561065));
#34879=CARTESIAN_POINT('Ctrl Pts',(-3.9937648242292,-5.46279521204571,105.996371212094));
#34880=CARTESIAN_POINT('Ctrl Pts',(-3.85310016882183,-5.56563295920115,
106.004579208422));
#34881=CARTESIAN_POINT('Ctrl Pts',(-3.70832560480854,-5.66313305285339,
106.01278720475));
#34882=CARTESIAN_POINT('Ctrl Pts',(-3.55988531489514,-5.75495486904927,
106.020995201078));
#34883=CARTESIAN_POINT('Ctrl Pts',(-3.41155261994671,-5.84671012942597,
106.02919724795));
#34884=CARTESIAN_POINT('Ctrl Pts',(-3.25955979532231,-5.93279512231752,
106.037399294821));
#34885=CARTESIAN_POINT('Ctrl Pts',(-3.10438127590678,-6.01291159870153,
106.045601341693));
#34886=CARTESIAN_POINT('Ctrl Pts',(-2.94928407433597,-6.09298609183161,
106.053799090464));
#34887=CARTESIAN_POINT('Ctrl Pts',(-2.79100482170631,-6.16709813507121,
106.061996839236));
#34888=CARTESIAN_POINT('Ctrl Pts',(-2.63004398036768,-6.23499459994407,
106.070194588007));
#34889=CARTESIAN_POINT('Ctrl Pts',(-2.46911383907699,-6.30287811492981,
106.078390773223));
#34890=CARTESIAN_POINT('Ctrl Pts',(-2.30550345565305,-6.36454826788074,
106.086586958439));
#34891=CARTESIAN_POINT('Ctrl Pts',(-2.13973505400837,-6.41979928803446,
106.094783143654));
#34892=CARTESIAN_POINT('Ctrl Pts',(-1.97397891553591,-6.47504622084242,
106.102978722534));
#34893=CARTESIAN_POINT('Ctrl Pts',(-1.80606541691134,-6.52387485226607,
106.111174301415));
#34894=CARTESIAN_POINT('Ctrl Pts',(-1.63653374083831,-6.56612871600137,
106.119369880295));
#34895=CARTESIAN_POINT('Ctrl Pts',(-1.46698376205527,-6.60838714148131,
106.127566343974));
#34896=CARTESIAN_POINT('Ctrl Pts',(-1.29581560601942,-6.6440692983082,106.135762807652));
#34897=CARTESIAN_POINT('Ctrl Pts',(-1.12358054209639,-6.673069441076,106.14395927133));
#34898=CARTESIAN_POINT('Ctrl Pts',(-0.951295547343085,-6.70207799096587,
106.152158111158));
#34899=CARTESIAN_POINT('Ctrl Pts',(-0.777943382385791,-6.7244006087548,
106.160356950986));
#34900=CARTESIAN_POINT('Ctrl Pts',(-0.604082414082601,-6.73998319263454,
106.168555790814));
#34901=CARTESIAN_POINT('Ctrl Pts',(-0.430039843051825,-6.75558205296647,
106.176763194563));
#34902=CARTESIAN_POINT('Ctrl Pts',(-0.255487764764599,-6.76442678199833,
106.184970598312));
#34903=CARTESIAN_POINT('Ctrl Pts',(-0.0809875503417063,-6.76651535257917,
106.193178002062));
#34904=CARTESIAN_POINT('Ctrl Pts',(0.0936061356304104,-6.76860504190894,
106.201389802131));
#34905=CARTESIAN_POINT('Ctrl Pts',(0.268147543993728,-6.76393136790142,
106.2096016022));
#34906=CARTESIAN_POINT('Ctrl Pts',(0.4420785402835,-6.75254437706416,106.217813402269));
#34907=CARTESIAN_POINT('Ctrl Pts',(0.616265587303113,-6.74114062298529,
106.226037291255));
#34908=CARTESIAN_POINT('Ctrl Pts',(0.789840069506157,-6.7230038385874,106.234261180241));
#34909=CARTESIAN_POINT('Ctrl Pts',(0.962250890148902,-6.69823575461536,
106.242485069227));
#34910=CARTESIAN_POINT('Ctrl Pts',(1.12155550781551,-6.67535047321139,106.250083800477));
#34911=CARTESIAN_POINT('Ctrl Pts',(1.27986654957716,-6.64680436916413,106.257682531727));
#34912=CARTESIAN_POINT('Ctrl Pts',(1.43676036062567,-6.61271568012226,106.265281262977));
#34913=CARTESIAN_POINT('Ctrl Pts',(1.6065818421427,-6.57581816557165,106.273506111299));
#34914=CARTESIAN_POINT('Ctrl Pts',(1.77521940266211,-6.53232287046059,106.281730959621));
#34915=CARTESIAN_POINT('Ctrl Pts',(1.94212222556167,-6.48231827828435,106.289955807943));
#34916=CARTESIAN_POINT('Ctrl Pts',(2.10883707887704,-6.43237000236589,106.298171393263));
#34917=CARTESIAN_POINT('Ctrl Pts',(2.27382074434021,-6.37592712912642,106.306386978582));
#34918=CARTESIAN_POINT('Ctrl Pts',(2.43653201563181,-6.31312923491997,106.314602563901));
#34919=CARTESIAN_POINT('Ctrl Pts',(2.59909272988927,-6.25038944771882,106.322810547324));
#34920=CARTESIAN_POINT('Ctrl Pts',(2.75938490484714,-6.18130647867979,106.331018530747));
#34921=CARTESIAN_POINT('Ctrl Pts',(2.91688185424882,-6.10606986926566,106.339226514171));
#34922=CARTESIAN_POINT('Ctrl Pts',(3.07426470550153,-6.03088776476672,106.347428551347));
#34923=CARTESIAN_POINT('Ctrl Pts',(3.22885604218162,-5.9495610533771,106.355630588524));
#34924=CARTESIAN_POINT('Ctrl Pts',(3.38014847323695,-5.86232763489673,106.3638326257));
#34925=CARTESIAN_POINT('Ctrl Pts',(3.53136168184899,-5.77513989513605,106.37203036798));
#34926=CARTESIAN_POINT('Ctrl Pts',(3.67927911608528,-5.68205178877099,106.380228110259));
#34927=CARTESIAN_POINT('Ctrl Pts',(3.8234172737882,-5.58334750400672,106.388425852539));
#34928=CARTESIAN_POINT('Ctrl Pts',(3.96752802600509,-5.48466198622921,106.396622036153));
#34929=CARTESIAN_POINT('Ctrl Pts',(4.10786063374422,-5.38036261438356,106.404818219767));
#34930=CARTESIAN_POINT('Ctrl Pts',(4.24395967166901,-5.27077748584088,106.413014403382));
#34931=CARTESIAN_POINT('Ctrl Pts',(4.3800486908057,-5.16120042429263,106.421209983642));
#34932=CARTESIAN_POINT('Ctrl Pts',(4.51190448073893,-5.04633860530262,106.429405563903));
#34933=CARTESIAN_POINT('Ctrl Pts',(4.63910392739835,-4.92656104709941,106.437601144164));
#34934=CARTESIAN_POINT('Ctrl Pts',(4.76631715283842,-4.80677051408582,106.445797612205));
#34935=CARTESIAN_POINT('Ctrl Pts',(4.88887276880498,-4.68206342701493,106.453994080246));
#34936=CARTESIAN_POINT('Ctrl Pts',(5.00638379795321,-4.55284639182914,106.462190548286));
#34937=CARTESIAN_POINT('Ctrl Pts',(5.12392893622362,-4.42359184969891,106.47038939546));
#34938=CARTESIAN_POINT('Ctrl Pts',(5.23642632970017,-4.2898250173541,106.478588242633));
#34939=CARTESIAN_POINT('Ctrl Pts',(5.34352861111647,-4.1519863899319,106.486787089807));
#34940=CARTESIAN_POINT('Ctrl Pts',(5.4507428248317,-4.01400370774033,106.494994505573));
#34941=CARTESIAN_POINT('Ctrl Pts',(5.55255044120691,-3.87194101242286,106.503201921339));
#34942=CARTESIAN_POINT('Ctrl Pts',(5.64864627826914,-3.72626947804318,106.511409337105));
#34943=CARTESIAN_POINT('Ctrl Pts',(5.74479361932023,-3.58051986884452,106.519621151757));
#34944=CARTESIAN_POINT('Ctrl Pts',(5.83522289259002,-3.43115787135136,106.527832966409));
#34945=CARTESIAN_POINT('Ctrl Pts',(5.91967447460793,-3.27868008727222,106.536044781061));
#34946=CARTESIAN_POINT('Ctrl Pts',(6.004250424419,-3.12597775647578,106.544268688859));
#34947=CARTESIAN_POINT('Ctrl Pts',(6.08283092874094,-2.97015078956756,106.552492596656));
#34948=CARTESIAN_POINT('Ctrl Pts',(6.15520364966004,-2.81171780789105,106.560716504454));
#34949=CARTESIAN_POINT('Ctrl Pts',(6.22207470718817,-2.66532865880982,106.568315243377));
#34950=CARTESIAN_POINT('Ctrl Pts',(6.28364637551961,-2.5167150653473,106.575913982301));
#34951=CARTESIAN_POINT('Ctrl Pts',(6.33978909926604,-2.36629735596088,106.583512721224));
#34952=CARTESIAN_POINT('Ctrl Pts',(6.40001203166125,-2.20494794255636,106.591663703398));
#34953=CARTESIAN_POINT('Ctrl Pts',(6.45416596335491,-2.04104452900994,106.599814685573));
#34954=CARTESIAN_POINT('Ctrl Pts',(6.50202534328628,-1.87508811399969,106.607965667747));
#34955=CARTESIAN_POINT('Ctrl Pts',(6.54982913011222,-1.70932447274641,106.6161071818));
#34956=CARTESIAN_POINT('Ctrl Pts',(6.59135281938823,-1.54151292483798,106.624248695853));
#34957=CARTESIAN_POINT('Ctrl Pts',(6.6264187797736,-1.37217460808156,106.632390209906));
#34958=CARTESIAN_POINT('Ctrl Pts',(6.66145138696019,-1.20299735848194,106.640523980109));
#34959=CARTESIAN_POINT('Ctrl Pts',(6.69003842004142,-1.03229658677865,106.648657750312));
#34960=CARTESIAN_POINT('Ctrl Pts',(6.71205196314816,-0.860608763608052,
106.656791520515));
#34961=CARTESIAN_POINT('Ctrl Pts',(6.73404919784243,-0.689048132858079,
106.664919264933));
#34962=CARTESIAN_POINT('Ctrl Pts',(6.74948259292692,-0.516502267864114,
106.673047009351));
#34963=CARTESIAN_POINT('Ctrl Pts',(6.75827525172114,-0.343518008223105,
106.681174753769));
#34964=CARTESIAN_POINT('Ctrl Pts',(6.7670632451925,-0.170625532812691,106.689298185663));
#34965=CARTESIAN_POINT('Ctrl Pts',(6.76921750103009,0.00270450957563728,
106.697421617557));
#34966=CARTESIAN_POINT('Ctrl Pts',(6.76471293997549,0.175919981037493,106.705545049451));
#34967=CARTESIAN_POINT('Ctrl Pts',(6.76017980375731,0.350234263320476,106.713720013202));
#34968=CARTESIAN_POINT('Ctrl Pts',(6.74890303522488,0.524432143122847,106.721894976953));
#34969=CARTESIAN_POINT('Ctrl Pts',(6.73091037817121,0.697950199532255,106.730069940704));
#34970=CARTESIAN_POINT('Ctrl Pts',(6.71303519570248,0.870335351468791,106.738191529877));
#34971=CARTESIAN_POINT('Ctrl Pts',(6.68853162470116,1.04204916537469,106.74631311905));
#34972=CARTESIAN_POINT('Ctrl Pts',(6.65747895546655,1.2125440023026,106.754434708223));
#34973=CARTESIAN_POINT('Ctrl Pts',(6.62642218664269,1.38306134804596,106.762557369612));
#34974=CARTESIAN_POINT('Ctrl Pts',(6.58881466301032,1.55235903616866,106.770680031002));
#34975=CARTESIAN_POINT('Ctrl Pts',(6.54478684632054,1.71989945526758,106.778802692391));
#34976=CARTESIAN_POINT('Ctrl Pts',(6.50074483285733,1.88749389778959,106.786927972933));
#34977=CARTESIAN_POINT('Ctrl Pts',(6.45027849685564,2.05332958916554,106.795053253476));
#34978=CARTESIAN_POINT('Ctrl Pts',(6.39356821373546,2.2168839609487,106.803178534018));
#34979=CARTESIAN_POINT('Ctrl Pts',(6.33624008384824,2.38222022367442,106.811392337806));
#34980=CARTESIAN_POINT('Ctrl Pts',(6.27253128256514,2.54522480365822,106.819606141593));
#34981=CARTESIAN_POINT('Ctrl Pts',(6.20267777368547,2.7053793515565,106.827819945381));
#34982=CARTESIAN_POINT('Ctrl Pts',(6.13345752769562,2.86408200486213,106.835959286236));
#34983=CARTESIAN_POINT('Ctrl Pts',(6.05820374328877,3.01998578739856,106.844098627091));
#34984=CARTESIAN_POINT('Ctrl Pts',(5.97719174312741,3.17261215182214,106.852237967947));
#34985=CARTESIAN_POINT('Ctrl Pts',(5.8950680329613,3.32733297454797,106.860489003201));
#34986=CARTESIAN_POINT('Ctrl Pts',(5.80702712091954,3.47868543698048,106.868740038455));
#34987=CARTESIAN_POINT('Ctrl Pts',(5.71340025635927,3.62620276744611,106.876991073709));
#34988=CARTESIAN_POINT('Ctrl Pts',(5.61977339179908,3.77372009791163,106.885242108963));
#34989=CARTESIAN_POINT('Ctrl Pts',(5.52056084802858,3.91740201862809,106.893493144217));
#34990=CARTESIAN_POINT('Ctrl Pts',(5.41613476850117,4.05681810899045,106.901744179471));
#34991=CARTESIAN_POINT('Ctrl Pts',(5.31194522147646,4.19591841198514,106.909976525543));
#34992=CARTESIAN_POINT('Ctrl Pts',(5.20224058843683,4.33120657113159,106.918208871615));
#34993=CARTESIAN_POINT('Ctrl Pts',(5.08732837871471,4.46221682206545,106.926441217687));
#34994=CARTESIAN_POINT('Ctrl Pts',(4.97254920912488,4.59307539528678,106.934664032723));
#34995=CARTESIAN_POINT('Ctrl Pts',(4.85257470073578,4.71966565437131,106.942886847759));
#34996=CARTESIAN_POINT('Ctrl Pts',(4.72775504148645,4.84155153516923,106.951109662795));
#34997=CARTESIAN_POINT('Ctrl Pts',(4.60308733443707,4.96328903527262,106.95932246759));
#34998=CARTESIAN_POINT('Ctrl Pts',(4.47358648596615,5.08033332166435,106.967535272385));
#34999=CARTESIAN_POINT('Ctrl Pts',(4.33964202266184,5.19228236088404,106.97574807718));
#35000=CARTESIAN_POINT('Ctrl Pts',(4.20579201884946,5.30415245208969,106.983955090192));
#35001=CARTESIAN_POINT('Ctrl Pts',(4.06750491228971,5.41093422083757,106.992162103203));
#35002=CARTESIAN_POINT('Ctrl Pts',(3.92520649450804,5.5122629632005,107.000369116215));
#35003=CARTESIAN_POINT('Ctrl Pts',(3.78299019264822,5.61353323194707,107.008571393218));
#35004=CARTESIAN_POINT('Ctrl Pts',(3.63676748146777,5.70935653508362,107.016773670221));
#35005=CARTESIAN_POINT('Ctrl Pts',(3.48699657130324,5.79940892778906,107.024975947225));
#35006=CARTESIAN_POINT('Ctrl Pts',(3.36016850770618,5.87566653066111,107.031921748037));
#35007=CARTESIAN_POINT('Ctrl Pts',(3.23079671185624,5.94778646687896,107.038867548849));
#35008=CARTESIAN_POINT('Ctrl Pts',(3.0991757505325,6.01559628526643,107.045813349661));
#35009=CARTESIAN_POINT('Ctrl Pts',(3.09917575053258,6.0155962852664,105.045751582742));
#35010=CARTESIAN_POINT('Ctrl Pts',(2.93382384459258,6.10078395293763,105.054501030655));
#35011=CARTESIAN_POINT('Ctrl Pts',(2.76495772122971,6.17915010267055,105.063250478567));
#35012=CARTESIAN_POINT('Ctrl Pts',(2.59315093316692,6.25042856433186,105.07199992648));
#35013=CARTESIAN_POINT('Ctrl Pts',(2.42134553245602,6.32170645041457,105.08074930374));
#35014=CARTESIAN_POINT('Ctrl Pts',(2.24659977927579,6.38589665313461,105.089498681));
#35015=CARTESIAN_POINT('Ctrl Pts',(2.06950718689912,6.44278115439077,105.09824805826));
#35016=CARTESIAN_POINT('Ctrl Pts',(1.89241596572847,6.49966521519728,105.106997367774));
#35017=CARTESIAN_POINT('Ctrl Pts',(1.71297821457175,6.54924360009552,105.115746677289));
#35018=CARTESIAN_POINT('Ctrl Pts',(1.53180337335814,6.59134792173563,105.124495986804));
#35019=CARTESIAN_POINT('Ctrl Pts',(1.35062987477751,6.63345193135311,105.13324523148));
#35020=CARTESIAN_POINT('Ctrl Pts',(1.16771959102919,6.66808192368244,105.141994476156));
#35021=CARTESIAN_POINT('Ctrl Pts',(0.983693746906509,6.69512028363173,105.150743720832));
#35022=CARTESIAN_POINT('Ctrl Pts',(0.799669205419644,6.72215845218869,105.159492903576));
#35023=CARTESIAN_POINT('Ctrl Pts',(0.614529402873359,6.7416050542458,105.16824208632));
#35024=CARTESIAN_POINT('Ctrl Pts',(0.428903127363242,6.75339404354122,105.176991269065));
#35025=CARTESIAN_POINT('Ctrl Pts',(0.243278104163879,6.7651829533033,105.185740392783));
#35026=CARTESIAN_POINT('Ctrl Pts',(0.0571669005391235,6.76931433552276,
105.194489516502));
#35027=CARTESIAN_POINT('Ctrl Pts',(-0.128798404777501,6.76577415902473,
105.20323864022));
#35028=CARTESIAN_POINT('Ctrl Pts',(-0.314762517259193,6.76223400523441,
105.21198770782));
#35029=CARTESIAN_POINT('Ctrl Pts',(-0.500580446819713,6.75102239665088,
105.220736775419));
#35030=CARTESIAN_POINT('Ctrl Pts',(-0.68562111884292,6.73217741012494,105.229485843018));
#35031=CARTESIAN_POINT('Ctrl Pts',(-0.870660665414765,6.71333253821768,
105.238234857404));
#35032=CARTESIAN_POINT('Ctrl Pts',(-1.05492267885511,6.68685441030608,105.24698387179));
#35033=CARTESIAN_POINT('Ctrl Pts',(-1.23778137635273,6.65283295028173,105.255732886175));
#35034=CARTESIAN_POINT('Ctrl Pts',(-1.42999922978854,6.61707018861863,105.264929696543));
#35035=CARTESIAN_POINT('Ctrl Pts',(-1.62066601233689,6.57297172934414,105.27412650691));
#35036=CARTESIAN_POINT('Ctrl Pts',(-1.80906628500366,6.520703043113,105.283323317277));
#35037=CARTESIAN_POINT('Ctrl Pts',(-1.9883134254551,6.47097374915036,105.292073315015));
#35038=CARTESIAN_POINT('Ctrl Pts',(-2.16550875896686,6.41384933989534,105.300823312753));
#35039=CARTESIAN_POINT('Ctrl Pts',(-2.34005036713997,6.34952386240481,105.309573310491));
#35040=CARTESIAN_POINT('Ctrl Pts',(-2.51458843547075,6.28519968948602,105.318323130772));
#35041=CARTESIAN_POINT('Ctrl Pts',(-2.68647261718042,6.21367483971105,105.327072951053));
#35042=CARTESIAN_POINT('Ctrl Pts',(-2.85511905908718,6.1351922674385,105.335822771333));
#35043=CARTESIAN_POINT('Ctrl Pts',(-3.02376230488877,6.05671118252941,105.344572425792));
#35044=CARTESIAN_POINT('Ctrl Pts',(-3.18916767379903,5.97127275992634,105.35332208025));
#35045=CARTESIAN_POINT('Ctrl Pts',(-3.35077334102792,5.87916720437994,105.362071734709));
#35046=CARTESIAN_POINT('Ctrl Pts',(-3.5123761603736,5.78706327195647,105.370821234977));
#35047=CARTESIAN_POINT('Ctrl Pts',(-3.67017916302279,5.68829258362311,105.379570735246));
#35048=CARTESIAN_POINT('Ctrl Pts',(-3.8236463656643,5.58319061741064,105.388320235514));
#35049=CARTESIAN_POINT('Ctrl Pts',(-3.97711106778763,5.47809036367727,105.397069593223));
#35050=CARTESIAN_POINT('Ctrl Pts',(-4.12623987481889,5.36665920043254,105.405818950931));
#35051=CARTESIAN_POINT('Ctrl Pts',(-4.27052628213889,5.24927559512368,105.41456830864));
#35052=CARTESIAN_POINT('Ctrl Pts',(-4.41481053024935,5.13189374643073,105.423317535416));
#35053=CARTESIAN_POINT('Ctrl Pts',(-4.55425230136485,5.00855981477394,105.432066762193));
#35054=CARTESIAN_POINT('Ctrl Pts',(-4.68837800630502,4.87969268192121,105.440815988969));
#35055=CARTESIAN_POINT('Ctrl Pts',(-4.82250188228837,4.75082730631867,105.44956509644));
#35056=CARTESIAN_POINT('Ctrl Pts',(-4.95130963052899,4.61642907903597,105.458314203911));
#35057=CARTESIAN_POINT('Ctrl Pts',(-5.07436379033292,4.47695444731775,105.467063311382));
#35058=CARTESIAN_POINT('Ctrl Pts',(-5.19741643562715,4.33748153220693,105.475812311171));
#35059=CARTESIAN_POINT('Ctrl Pts',(-5.31471544462669,4.19293255254719,105.484561310961));
#35060=CARTESIAN_POINT('Ctrl Pts',(-5.42586245275512,4.04379841779758,105.493310310751));
#35061=CARTESIAN_POINT('Ctrl Pts',(-5.53702160019036,3.89464799484509,105.502060266093));
#35062=CARTESIAN_POINT('Ctrl Pts',(-5.64202723081133,3.74091164444028,105.510810221435));
#35063=CARTESIAN_POINT('Ctrl Pts',(-5.74052265232849,3.58311159163422,105.519560176777));
#35064=CARTESIAN_POINT('Ctrl Pts',(-5.83901427066812,3.42531763191965,105.52830979426));
#35065=CARTESIAN_POINT('Ctrl Pts',(-5.93099603115644,3.26346052695786,105.537059411742));
#35066=CARTESIAN_POINT('Ctrl Pts',(-6.01615550622669,3.09809004467241,105.545809029225));
#35067=CARTESIAN_POINT('Ctrl Pts',(-6.10131214578715,2.93272506864002,105.554558355376));
#35068=CARTESIAN_POINT('Ctrl Pts',(-6.17964682328665,2.76384720417078,105.563307681527));
#35069=CARTESIAN_POINT('Ctrl Pts',(-6.25089348288484,2.59203002791787,105.572057007678));
#35070=CARTESIAN_POINT('Ctrl Pts',(-6.32213814889256,2.42021765937224,105.58080608901));
#35071=CARTESIAN_POINT('Ctrl Pts',(-6.38629508412516,2.24546640832114,105.589555170341));
#35072=CARTESIAN_POINT('Ctrl Pts',(-6.44314639819748,2.06836976660239,105.598304251673));
#35073=CARTESIAN_POINT('Ctrl Pts',(-6.50000285283646,1.89125711158465,105.607054124107));
#35074=CARTESIAN_POINT('Ctrl Pts',(-6.54955227673202,1.71179891440436,105.615803996541));
#35075=CARTESIAN_POINT('Ctrl Pts',(-6.59162635926345,1.53060476278603,105.624553868976));
#35076=CARTESIAN_POINT('Ctrl Pts',(-6.63369752055156,1.34942319164891,105.633303133898));
#35077=CARTESIAN_POINT('Ctrl Pts',(-6.66829431424215,1.16650618642923,105.642052398821));
#35078=CARTESIAN_POINT('Ctrl Pts',(-6.69529923745382,0.982474997620986,
105.650801663743));
#35079=CARTESIAN_POINT('Ctrl Pts',(-6.72230554731414,0.798434359180195,
105.659551377923));
#35080=CARTESIAN_POINT('Ctrl Pts',(-6.7417191649668,0.613279706242812,105.668301092103));
#35081=CARTESIAN_POINT('Ctrl Pts',(-6.75347414817259,0.427639953657873,
105.677050806282));
#35082=CARTESIAN_POINT('Ctrl Pts',(-6.76248837758729,0.285283364201837,
105.683760465458));
#35083=CARTESIAN_POINT('Ctrl Pts',(-6.76699999999987,0.142641701109152,
105.690470124634));
#35084=CARTESIAN_POINT('Ctrl Pts',(-6.767,6.37056316116541E-12,105.69717978381));
#35085=CARTESIAN_POINT('',(-6.767,5.80994670776325E-12,105.30282021619));
#35086=CARTESIAN_POINT('Ctrl Pts',(3.09917575053253,6.01559628526642,104.651558856765));
#35087=CARTESIAN_POINT('Ctrl Pts',(2.94526809315026,6.09488798919087,104.659684436931));
#35088=CARTESIAN_POINT('Ctrl Pts',(2.78822179244347,6.16831755058199,104.667810017098));
#35089=CARTESIAN_POINT('Ctrl Pts',(2.62852912535888,6.23563337898726,104.675935597265));
#35090=CARTESIAN_POINT('Ctrl Pts',(2.46549012587466,6.30435979901025,104.684231447567));
#35091=CARTESIAN_POINT('Ctrl Pts',(2.29969296126507,6.36671323073493,104.69252729787));
#35092=CARTESIAN_POINT('Ctrl Pts',(2.13168545729376,6.4224766337576,104.700823148173));
#35093=CARTESIAN_POINT('Ctrl Pts',(1.9671733892681,6.47707986596187,104.708946401344));
#35094=CARTESIAN_POINT('Ctrl Pts',(1.80054241571459,6.52536448150152,104.717069654515));
#35095=CARTESIAN_POINT('Ctrl Pts',(1.63232420764034,6.56717646185568,104.725192907685));
#35096=CARTESIAN_POINT('Ctrl Pts',(1.46408745371886,6.60899305192844,104.733317056435));
#35097=CARTESIAN_POINT('Ctrl Pts',(1.29426347175619,6.6443354970468,104.741441205184));
#35098=CARTESIAN_POINT('Ctrl Pts',(1.12339596380903,6.6731005168885,104.749565353933));
#35099=CARTESIAN_POINT('Ctrl Pts',(0.952477109807773,6.70187418068061,104.757691944007));
#35100=CARTESIAN_POINT('Ctrl Pts',(0.780514465980827,6.72406642256315,104.76581853408));
#35101=CARTESIAN_POINT('Ctrl Pts',(0.608058681233473,6.73962563056559,104.773945124154));
#35102=CARTESIAN_POINT('Ctrl Pts',(0.429286414833262,6.7557547205933,104.782369364185));
#35103=CARTESIAN_POINT('Ctrl Pts',(0.249984630161608,6.76475564082305,104.790793604217));
#35104=CARTESIAN_POINT('Ctrl Pts',(0.0707677718090432,6.76662995312092,
104.799217844248));
#35105=CARTESIAN_POINT('Ctrl Pts',(-0.102413384704881,6.76844114194766,
104.807358371009));
#35106=CARTESIAN_POINT('Ctrl Pts',(-0.275514882274292,6.76359801666385,
104.81549889777));
#35107=CARTESIAN_POINT('Ctrl Pts',(-0.44798701878902,6.75215496201002,104.823639424531));
#35108=CARTESIAN_POINT('Ctrl Pts',(-0.6294756419622,6.74011368812088,104.832205521198));
#35109=CARTESIAN_POINT('Ctrl Pts',(-0.81026685441072,6.72076398380431,104.840771617864));
#35110=CARTESIAN_POINT('Ctrl Pts',(-0.9897323476931,6.69423026791953,104.849337714531));
#35111=CARTESIAN_POINT('Ctrl Pts',(-1.16919784097561,6.66769655203473,104.857903811198));
#35112=CARTESIAN_POINT('Ctrl Pts',(-1.34733717515646,6.63397898833411,104.866469907865));
#35113=CARTESIAN_POINT('Ctrl Pts',(-1.52354118781109,6.5932625648493,104.875036004532));
#35114=CARTESIAN_POINT('Ctrl Pts',(-1.69289445640747,6.55412918020714,104.883269054664));
#35115=CARTESIAN_POINT('Ctrl Pts',(-1.86098657619945,6.50840943586728,104.891502104796));
#35116=CARTESIAN_POINT('Ctrl Pts',(-2.02726723581267,6.45619675618707,104.899735154928));
#35117=CARTESIAN_POINT('Ctrl Pts',(-2.19334988072036,6.40404625378242,104.907958400763));
#35118=CARTESIAN_POINT('Ctrl Pts',(-2.35762502253053,6.34541831878858,104.916181646598));
#35119=CARTESIAN_POINT('Ctrl Pts',(-2.51955236299189,6.28045737905624,104.924404892433));
#35120=CARTESIAN_POINT('Ctrl Pts',(-2.68131928298852,6.21556079574519,104.932619991546));
#35121=CARTESIAN_POINT('Ctrl Pts',(-2.84074270365649,6.14434383502938,104.94083509066));
#35122=CARTESIAN_POINT('Ctrl Pts',(-2.99729723425014,6.06700076558067,104.949050189773));
#35123=CARTESIAN_POINT('Ctrl Pts',(-3.15372799059706,5.98971884466675,104.957258793912));
#35124=CARTESIAN_POINT('Ctrl Pts',(-3.30729405495557,5.90632062001654,104.965467398051));
#35125=CARTESIAN_POINT('Ctrl Pts',(-3.4574897006659,5.81704856175271,104.97367600219));
#35126=CARTESIAN_POINT('Ctrl Pts',(-3.60759664286986,5.72782922635278,104.981879758439));
#35127=CARTESIAN_POINT('Ctrl Pts',(-3.75433682474402,5.63274315058797,104.990083514688));
#35128=CARTESIAN_POINT('Ctrl Pts',(-3.89722875597661,5.53207890612462,104.998287270937));
#35129=CARTESIAN_POINT('Ctrl Pts',(-4.04007840908963,5.43144444567306,105.006488599901));
#35130=CARTESIAN_POINT('Ctrl Pts',(-4.17908178494357,5.32523530700372,105.014689928865));
#35131=CARTESIAN_POINT('Ctrl Pts',(-4.31378584557687,5.21378371995815,105.02289125783));
#35132=CARTESIAN_POINT('Ctrl Pts',(-4.44847132923409,5.10234750315055,105.031091455752));
#35133=CARTESIAN_POINT('Ctrl Pts',(-4.57885840209157,4.98567050559777,105.039291653675));
#35134=CARTESIAN_POINT('Ctrl Pts',(-4.70452662502886,4.8641256392485,105.047491851598));
#35135=CARTESIAN_POINT('Ctrl Pts',(-4.83020029075708,4.74257550869415,105.055692404678));
#35136=CARTESIAN_POINT('Ctrl Pts',(-4.95115444180458,4.61615733837194,105.063892957758));
#35137=CARTESIAN_POINT('Ctrl Pts',(-5.06700503571259,4.48528136999936,105.072093510837));
#35138=CARTESIAN_POINT('Ctrl Pts',(-5.18288164159939,4.35437601599482,105.080295905191));
#35139=CARTESIAN_POINT('Ctrl Pts',(-5.29365217060191,4.21901113862904,105.088498299544));
#35140=CARTESIAN_POINT('Ctrl Pts',(-5.3989724215177,4.07963059500383,105.096700693897));
#35141=CARTESIAN_POINT('Ctrl Pts',(-5.50439116538272,3.94011970606813,105.104910758931));
#35142=CARTESIAN_POINT('Ctrl Pts',(-5.60434923156479,3.79658593421217,105.113120823965));
#35143=CARTESIAN_POINT('Ctrl Pts',(-5.69854484998727,3.64950347207446,105.121330888998));
#35144=CARTESIAN_POINT('Ctrl Pts',(-5.79278554876156,3.50235061887985,105.129544883224));
#35145=CARTESIAN_POINT('Ctrl Pts',(-5.88125811987639,3.35164599799604,105.137758877449));
#35146=CARTESIAN_POINT('Ctrl Pts',(-5.96370650742258,3.19788894324452,105.145972871674));
#35147=CARTESIAN_POINT('Ctrl Pts',(-6.04626729958135,3.04392226641688,105.15419806431));
#35148=CARTESIAN_POINT('Ctrl Pts',(-6.12278733745084,2.88689516110816,105.162423256945));
#35149=CARTESIAN_POINT('Ctrl Pts',(-6.1930580184258,2.72732861613922,105.17064844958));
#35150=CARTESIAN_POINT('Ctrl Pts',(-6.25625229131923,2.58383076401195,105.1780453477));
#35151=CARTESIAN_POINT('Ctrl Pts',(-6.31439306651561,2.43827960410804,105.18544224582));
#35152=CARTESIAN_POINT('Ctrl Pts',(-6.36736319722621,2.29106414458636,105.19283914394));
#35153=CARTESIAN_POINT('Ctrl Pts',(-6.43416671896371,2.10540269693046,105.202167775712));
#35154=CARTESIAN_POINT('Ctrl Pts',(-6.49288172649907,1.91671821912665,105.211496407485));
#35155=CARTESIAN_POINT('Ctrl Pts',(-6.54326425484908,1.72568302165095,105.220825039257));
#35156=CARTESIAN_POINT('Ctrl Pts',(-6.59352975588623,1.53509155609093,105.230132002711));
#35157=CARTESIAN_POINT('Ctrl Pts',(-6.63550135685087,1.34216043581957,105.239438966164));
#35158=CARTESIAN_POINT('Ctrl Pts',(-6.66898465358551,1.14757687770405,105.248745929617));
#35159=CARTESIAN_POINT('Ctrl Pts',(-6.70230957459399,0.95391369826447,105.258008871208));
#35160=CARTESIAN_POINT('Ctrl Pts',(-6.72722623341481,0.758613842922332,
105.267271812798));
#35161=CARTESIAN_POINT('Ctrl Pts',(-6.74359154643889,0.562371811880692,
105.276534754389));
#35162=CARTESIAN_POINT('Ctrl Pts',(-6.75907150336007,0.37674638680155,105.285296574989));
#35163=CARTESIAN_POINT('Ctrl Pts',(-6.76690063763709,0.190278218662405,
105.29405839559));
#35164=CARTESIAN_POINT('Ctrl Pts',(-6.7669990598182,0.00356713044430194,
105.30282021619));
#35165=CARTESIAN_POINT('Ctrl Pts',(-6.767,6.19460692657023E-12,105.30282021619));
#35166=CARTESIAN_POINT('Ctrl Pts',(-6.76700000000017,-0.186007249409504,
105.311569727996));
#35167=CARTESIAN_POINT('Ctrl Pts',(-6.75932637295472,-0.372014355521384,
105.320319239802));
#35168=CARTESIAN_POINT('Ctrl Pts',(-6.74400518266978,-0.557389537148933,
105.329068751608));
#35169=CARTESIAN_POINT('Ctrl Pts',(-6.72868405709711,-0.742763935805453,
105.337818226458));
#35170=CARTESIAN_POINT('Ctrl Pts',(-6.70571545653072,-0.927506129689267,
105.346567701309));
#35171=CARTESIAN_POINT('Ctrl Pts',(-6.67517739415743,-1.11098863924417,
105.35531717616));
#35172=CARTESIAN_POINT('Ctrl Pts',(-6.64463945823174,-1.29447038906123,
105.364066614782));
#35173=CARTESIAN_POINT('Ctrl Pts',(-6.60653217027239,-1.47669218227853,
105.372816053403));
#35174=CARTESIAN_POINT('Ctrl Pts',(-6.560984961168,-1.65703510503773,105.381565492025));
#35175=CARTESIAN_POINT('Ctrl Pts',(-6.51543793687604,-1.83737729603717,
105.390314895146));
#35176=CARTESIAN_POINT('Ctrl Pts',(-6.46245112202722,-2.01584035396792,
105.399064298266));
#35177=CARTESIAN_POINT('Ctrl Pts',(-6.40220448416317,-2.19181813637925,
105.407813701386));
#35178=CARTESIAN_POINT('Ctrl Pts',(-6.34195808575264,-2.36779521935737,
105.416563069732));
#35179=CARTESIAN_POINT('Ctrl Pts',(-6.27445201489314,-2.54128677544633,
105.425312438077));
#35180=CARTESIAN_POINT('Ctrl Pts',(-6.19991555136263,-2.71170355237658,
105.434061806422));
#35181=CARTESIAN_POINT('Ctrl Pts',(-6.12537937789112,-2.88211966612918,
105.442811140719));
#35182=CARTESIAN_POINT('Ctrl Pts',(-6.04381298133682,-3.04946076210317,
105.451560475016));
#35183=CARTESIAN_POINT('Ctrl Pts',(-5.95549339426361,-3.21315848206753,
105.460309809313));
#35184=CARTESIAN_POINT('Ctrl Pts',(-5.86717414355217,-3.37685557859539,
105.469059110289));
#35185=CARTESIAN_POINT('Ctrl Pts',(-5.77210188986295,-3.53690907467219,
105.477808411264));
#35186=CARTESIAN_POINT('Ctrl Pts',(-5.67059953467125,-3.69277536784817,
105.48655771224));
#35187=CARTESIAN_POINT('Ctrl Pts',(-5.56909755761831,-3.84864108035697,
105.495306980621));
#35188=CARTESIAN_POINT('Ctrl Pts',(-5.46116568338145,-4.00031938104177,
105.504056249001));
#35189=CARTESIAN_POINT('Ctrl Pts',(-5.347170486862,-4.14729511663109,105.512805517382));
#35190=CARTESIAN_POINT('Ctrl Pts',(-5.23317570555606,-4.29427031687933,
105.521554753895));
#35191=CARTESIAN_POINT('Ctrl Pts',(-5.11311782178896,-4.43654275987025,
105.530303990407));
#35192=CARTESIAN_POINT('Ctrl Pts',(-4.98740459172108,-4.57362924147547,
105.53905322692));
#35193=CARTESIAN_POINT('Ctrl Pts',(-4.86169180910923,-4.71071523514341,
105.547802432291));
#35194=CARTESIAN_POINT('Ctrl Pts',(-4.73032391415522,-4.84261509316435,
105.556551637662));
#35195=CARTESIAN_POINT('Ctrl Pts',(-4.59374707237382,-4.96888084331442,
105.565300843033));
#35196=CARTESIAN_POINT('Ctrl Pts',(-4.45717070537499,-5.09514615452639,
105.57405001799));
#35197=CARTESIAN_POINT('Ctrl Pts',(-4.31538563819616,-5.21577720253544,
105.582799192946));
#35198=CARTESIAN_POINT('Ctrl Pts',(-4.16887341290764,-5.33036429028559,
105.591548367902));
#35199=CARTESIAN_POINT('Ctrl Pts',(-4.02236168477457,-5.44495098921089,
105.60029751317));
#35200=CARTESIAN_POINT('Ctrl Pts',(-3.8711230563456,-5.55349359238675,105.609046658438));
#35201=CARTESIAN_POINT('Ctrl Pts',(-3.71567117316855,-5.65562346102392,
105.617795803706));
#35202=CARTESIAN_POINT('Ctrl Pts',(-3.5602198045744,-5.75775299158683,105.626544920012));
#35203=CARTESIAN_POINT('Ctrl Pts',(-3.40055544862543,-5.85346967275262,
105.635294036318));
#35204=CARTESIAN_POINT('Ctrl Pts',(-3.23722036323576,-5.94244842803467,
105.644043152624));
#35205=CARTESIAN_POINT('Ctrl Pts',(-3.07388580496235,-6.03142689616379,
105.652792240695));
#35206=CARTESIAN_POINT('Ctrl Pts',(-2.90688079257911,-6.11366734484725,
105.661541328766));
#35207=CARTESIAN_POINT('Ctrl Pts',(-2.73677251094835,-6.18889046787205,
105.670290416837));
#35208=CARTESIAN_POINT('Ctrl Pts',(-2.56666476416852,-6.26411335438186,
105.679039477399));
#35209=CARTESIAN_POINT('Ctrl Pts',(-2.39345402972286,-6.33231884350218,
105.687788537962));
#35210=CARTESIAN_POINT('Ctrl Pts',(-2.21772856474217,-6.39327529620981,
105.696537598524));
#35211=CARTESIAN_POINT('Ctrl Pts',(-2.04200363768468,-6.45423156232019,
105.705286632304));
#35212=CARTESIAN_POINT('Ctrl Pts',(-1.86376426620312,-6.50793874251993,
105.714035666084));
#35213=CARTESIAN_POINT('Ctrl Pts',(-1.68361578194927,-6.55421443796061,
105.722784699864));
#35214=CARTESIAN_POINT('Ctrl Pts',(-1.50346783420131,-6.60048999558619,
105.731533707588));
#35215=CARTESIAN_POINT('Ctrl Pts',(-1.32141106257533,-6.63933404145438,
105.740282715312));
#35216=CARTESIAN_POINT('Ctrl Pts',(-1.13806375959355,-6.67061465526977,
105.749031723037));
#35217=CARTESIAN_POINT('Ctrl Pts',(-0.954716987422054,-6.7018951785244,
105.757780705431));
#35218=CARTESIAN_POINT('Ctrl Pts',(-0.770079973812569,-6.72561226535797,
105.766529687826));
#35219=CARTESIAN_POINT('Ctrl Pts',(-0.584779770554938,-6.74168536939761,
105.775278670221));
#35220=CARTESIAN_POINT('Ctrl Pts',(-0.391490647556358,-6.7584514394238,
105.784404850897));
#35221=CARTESIAN_POINT('Ctrl Pts',(-0.197480213106745,-6.7668997592402,
105.793531031573));
#35222=CARTESIAN_POINT('Ctrl Pts',(-0.00346532630016481,-6.76699911271707,
105.802657212249));
#35223=CARTESIAN_POINT('Ctrl Pts',(0.184486595293678,-6.7670953613978,105.811498199779));
#35224=CARTESIAN_POINT('Ctrl Pts',(0.372442378182846,-6.75935659726783,
105.820339187309));
#35225=CARTESIAN_POINT('Ctrl Pts',(0.559750217719698,-6.74380965729036,
105.829180174839));
#35226=CARTESIAN_POINT('Ctrl Pts',(0.7451299144554,-6.72842275717279,105.837930153437));
#35227=CARTESIAN_POINT('Ctrl Pts',(0.929874656311867,-6.70538772273505,
105.846680132035));
#35228=CARTESIAN_POINT('Ctrl Pts',(1.11335688289549,-6.6747828018078,105.855430110632));
#35229=CARTESIAN_POINT('Ctrl Pts',(1.29683723118632,-6.64417819418067,105.864179999657));
#35230=CARTESIAN_POINT('Ctrl Pts',(1.47905480730014,-6.60600390230125,105.872929888682));
#35231=CARTESIAN_POINT('Ctrl Pts',(1.65939064804591,-6.56038959797189,105.881679777707));
#35232=CARTESIAN_POINT('Ctrl Pts',(1.83972470264045,-6.51477574543318,105.890429580068));
#35233=CARTESIAN_POINT('Ctrl Pts',(2.01817678125625,-6.46172209820169,105.899179382429));
#35234=CARTESIAN_POINT('Ctrl Pts',(2.19414072347455,-6.40140886724091,105.90792918479));
#35235=CARTESIAN_POINT('Ctrl Pts',(2.37010298131872,-6.34109621361458,105.916678903396));
#35236=CARTESIAN_POINT('Ctrl Pts',(2.54357687926688,-6.27352420826062,105.925428622001));
#35237=CARTESIAN_POINT('Ctrl Pts',(2.71397317789747,-6.19892237325595,105.934178340607));
#35238=CARTESIAN_POINT('Ctrl Pts',(2.88436790206987,-6.12432122757065,105.942927978365));
#35239=CARTESIAN_POINT('Ctrl Pts',(3.05168482126052,-6.0426904971752,105.951677616123));
#35240=CARTESIAN_POINT('Ctrl Pts',(3.21535561997194,-5.95430745235034,105.960427253881));
#35241=CARTESIAN_POINT('Ctrl Pts',(3.3790249607508,-5.86592519481632,105.9691768137));
#35242=CARTESIAN_POINT('Ctrl Pts',(3.53904799384668,-5.77079087940359,105.977926373519));
#35243=CARTESIAN_POINT('Ctrl Pts',(3.69488118814771,-5.66922763747163,105.986675933338));
#35244=CARTESIAN_POINT('Ctrl Pts',(3.85071304610628,-5.56766526649194,105.995425418126));
#35245=CARTESIAN_POINT('Ctrl Pts',(4.00235489705771,-5.45967423580858,106.004174902913));
#35246=CARTESIAN_POINT('Ctrl Pts',(4.14929168607466,-5.34562133936475,106.012924387701));
#35247=CARTESIAN_POINT('Ctrl Pts',(4.29622726385565,-5.23156938308688,106.021673800364));
#35248=CARTESIAN_POINT('Ctrl Pts',(4.43845763091873,-5.11145583677371,106.030423213027));
#35249=CARTESIAN_POINT('Ctrl Pts',(4.57549970660766,-4.98568866204392,106.039172625691));
#35250=CARTESIAN_POINT('Ctrl Pts',(4.71254069815118,-4.85992248226334,106.047921969137));
#35251=CARTESIAN_POINT('Ctrl Pts',(4.84439326931155,-4.72850295734166,106.056671312583));
#35252=CARTESIAN_POINT('Ctrl Pts',(4.97060959434556,-4.59187644221835,106.06542065603));
#35253=CARTESIAN_POINT('Ctrl Pts',(5.09682496280384,-4.45525096256814,106.074169933166));
#35254=CARTESIAN_POINT('Ctrl Pts',(5.21740397615719,-4.31341878218472,106.082919210302));
#35255=CARTESIAN_POINT('Ctrl Pts',(5.33193710451824,-4.16686161438818,106.091668487439));
#35256=CARTESIAN_POINT('Ctrl Pts',(5.44646940289275,-4.0203055086466,106.100417701171));
#35257=CARTESIAN_POINT('Ctrl Pts',(5.55495572749559,-3.86902470980285,106.109166914904));
#35258=CARTESIAN_POINT('Ctrl Pts',(5.65702762491353,-3.71353301465938,106.117916128637));
#35259=CARTESIAN_POINT('Ctrl Pts',(5.75909881655058,-3.55804239467048,106.126665281874));
#35260=CARTESIAN_POINT('Ctrl Pts',(5.85475551250694,-3.39834117619705,106.13541443511));
#35261=CARTESIAN_POINT('Ctrl Pts',(5.94367283728014,-3.23497174692119,106.144163588346));
#35262=CARTESIAN_POINT('Ctrl Pts',(6.03258957676244,-3.071603393011,106.152912683991));
#35263=CARTESIAN_POINT('Ctrl Pts',(6.11476689685229,-2.90456712829622,106.161661779637));
#35264=CARTESIAN_POINT('Ctrl Pts',(6.18992570525216,-2.73443024476006,106.170410875282));
#35265=CARTESIAN_POINT('Ctrl Pts',(6.2650840438867,-2.564294424631,106.179159916243));
#35266=CARTESIAN_POINT('Ctrl Pts',(6.33322384283302,-2.3910582865603,106.187908957204));
#35267=CARTESIAN_POINT('Ctrl Pts',(6.39411368720031,-2.21531017132086,106.196657998166));
#35268=CARTESIAN_POINT('Ctrl Pts',(6.45500317120888,-2.0395630961952,106.205406987348));
#35269=CARTESIAN_POINT('Ctrl Pts',(6.50864269270072,-1.86130434438639,106.21415597653));
#35270=CARTESIAN_POINT('Ctrl Pts',(6.55485008446332,-1.68113930719951,106.222904965713));
#35271=CARTESIAN_POINT('Ctrl Pts',(6.60199664749401,-1.49731239211851,106.231831779242));
#35272=CARTESIAN_POINT('Ctrl Pts',(6.64140563640903,-1.31150116499686,106.240758592771));
#35273=CARTESIAN_POINT('Ctrl Pts',(6.67293772282169,-1.1243625515568,106.249685406301));
#35274=CARTESIAN_POINT('Ctrl Pts',(6.70384494949868,-0.940932395051574,
106.258435320456));
#35275=CARTESIAN_POINT('Ctrl Pts',(6.72718449348927,-0.756227260506975,
106.267185234612));
#35276=CARTESIAN_POINT('Ctrl Pts',(6.7428770737393,-0.570874564541984,106.275935148767));
#35277=CARTESIAN_POINT('Ctrl Pts',(6.75856934538668,-0.38552551363282,106.284684890851));
#35278=CARTESIAN_POINT('Ctrl Pts',(6.76661493004102,-0.199529212418625,
106.293434632935));
#35279=CARTESIAN_POINT('Ctrl Pts',(6.76698649908907,-0.0135174386008752,
106.302184375019));
#35280=CARTESIAN_POINT('Ctrl Pts',(6.7673580613239,0.172490924445438,106.310933956665));
#35281=CARTESIAN_POINT('Ctrl Pts',(6.76005588896291,0.358514472901174,106.319683538311));
#35282=CARTESIAN_POINT('Ctrl Pts',(6.74510478454585,0.543921359662087,106.328433119957));
#35283=CARTESIAN_POINT('Ctrl Pts',(6.73015393440688,0.729325093150405,106.337182552796));
#35284=CARTESIAN_POINT('Ctrl Pts',(6.70755443556897,0.914111900256396,106.345931985635));
#35285=CARTESIAN_POINT('Ctrl Pts',(6.67738304682317,1.09765415591551,106.354681418474));
#35286=CARTESIAN_POINT('Ctrl Pts',(6.6472121311186,1.28119353391271,106.363430714135));
#35287=CARTESIAN_POINT('Ctrl Pts',(6.60946960955497,1.46348811672637,106.372180009797));
#35288=CARTESIAN_POINT('Ctrl Pts',(6.5642836699119,1.64391876348192,106.380929305458));
#35289=CARTESIAN_POINT('Ctrl Pts',(6.51909837867726,1.82434682109686,106.389678475569));
#35290=CARTESIAN_POINT('Ctrl Pts',(6.4664699527193,2.00291071820416,106.39842764568));
#35291=CARTESIAN_POINT('Ctrl Pts',(6.40657713281559,2.17900400212675,106.407176815791));
#35292=CARTESIAN_POINT('Ctrl Pts',(6.3466850927907,2.35509499309632,106.415925871976));
#35293=CARTESIAN_POINT('Ctrl Pts',(6.27952894037536,2.52871516398098,106.424674928162));
#35294=CARTESIAN_POINT('Ctrl Pts',(6.20533675061456,2.69927486771398,106.433423984348));
#35295=CARTESIAN_POINT('Ctrl Pts',(6.1283211790793,2.87632521635894,106.44250598563));
#35296=CARTESIAN_POINT('Ctrl Pts',(6.04372366626097,3.05007728919961,106.451587986912));
#35297=CARTESIAN_POINT('Ctrl Pts',(5.95185378007891,3.21989527478153,106.460669988195));
#35298=CARTESIAN_POINT('Ctrl Pts',(5.86334450817396,3.38350129286708,106.469419768502));
#35299=CARTESIAN_POINT('Ctrl Pts',(5.76808562057283,3.54345567124917,106.478169548809));
#35300=CARTESIAN_POINT('Ctrl Pts',(5.66640068804514,3.69921508465264,106.486919329116));
#35301=CARTESIAN_POINT('Ctrl Pts',(5.56471941107956,3.85496889852235,106.49566879487));
#35302=CARTESIAN_POINT('Ctrl Pts',(5.4566127081515,4.00652780919587,106.504418260623));
#35303=CARTESIAN_POINT('Ctrl Pts',(5.34244776449154,4.15337704569177,106.513167726377));
#35304=CARTESIAN_POINT('Ctrl Pts',(5.22828631819636,4.300221783562,106.521916924096));
#35305=CARTESIAN_POINT('Ctrl Pts',(5.1080671784411,4.44235690972632,106.530666121816));
#35306=CARTESIAN_POINT('Ctrl Pts',(4.9821986454476,4.579299690706,106.539415319535));
#35307=CARTESIAN_POINT('Ctrl Pts',(4.85633329944058,4.71623900429968,106.548164295726));
#35308=CARTESIAN_POINT('Ctrl Pts',(4.72481904033672,4.84798602483594,106.556913271916));
#35309=CARTESIAN_POINT('Ctrl Pts',(4.58810250737212,4.97409332259113,106.565662248106));
#35310=CARTESIAN_POINT('Ctrl Pts',(4.45137708685649,5.1002088182213,106.574411793042));
#35311=CARTESIAN_POINT('Ctrl Pts',(4.3094489263605,5.22068366307934,106.583161337978));
#35312=CARTESIAN_POINT('Ctrl Pts',(4.16280009466652,5.33510865604858,106.591910882915));
#35313=CARTESIAN_POINT('Ctrl Pts',(4.01615988348784,5.44952692272895,106.600659913523));
#35314=CARTESIAN_POINT('Ctrl Pts',(3.8647997823223,5.55789587288626,106.609408944131));
#35315=CARTESIAN_POINT('Ctrl Pts',(3.70923383581072,5.65984746713875,106.618157974739));
#35316=CARTESIAN_POINT('Ctrl Pts',(3.55366577799534,5.76180044505387,106.626907124087));
#35317=CARTESIAN_POINT('Ctrl Pts',(3.39389200026823,5.85733573571069,106.635656273435));
#35318=CARTESIAN_POINT('Ctrl Pts',(3.23045513626013,5.94612887621943,106.644405422784));
#35319=CARTESIAN_POINT('Ctrl Pts',(3.18695122151561,5.96976399206697,106.646734286896));
#35320=CARTESIAN_POINT('Ctrl Pts',(3.14318791262657,5.99292165435336,106.649063151009));
#35321=CARTESIAN_POINT('Ctrl Pts',(3.09917575053261,6.01559628526638,106.651392015122));
#35322=CARTESIAN_POINT('Origin',(0.,0.,-3.69717978381041));
#35323=CARTESIAN_POINT('',(3.09917575053271,6.01559628526633,109.0454843164));
#35324=CARTESIAN_POINT('',(3.09917575053272,6.01559628526632,108.651236765584));
#35325=CARTESIAN_POINT('',(3.09917575053259,6.01559628526639,-3.69717978381041));
#35326=CARTESIAN_POINT('',(-6.76699985827658,-0.00138494936151985,107.697179783846));
#35327=CARTESIAN_POINT('Ctrl Pts',(-6.76699985827658,-0.00138494936171985,
107.697179783846));
#35328=CARTESIAN_POINT('Ctrl Pts',(-6.76696181981259,-0.187244654813968,
107.70587655106));
#35329=CARTESIAN_POINT('Ctrl Pts',(-6.75926240779375,-0.372917032884847,
107.714573318273));
#35330=CARTESIAN_POINT('Ctrl Pts',(-6.74397327179888,-0.557775500772766,
107.723270085487));
#35331=CARTESIAN_POINT('Ctrl Pts',(-6.72865813208867,-0.742948375372715,
107.731981644135));
#35332=CARTESIAN_POINT('Ctrl Pts',(-6.70572750687344,-0.927304289991112,
107.740693202783));
#35333=CARTESIAN_POINT('Ctrl Pts',(-6.6753044046526,-1.11022524976944,107.749404761432));
#35334=CARTESIAN_POINT('Ctrl Pts',(-6.64415517569663,-1.29751209565452,
107.758324244163));
#35335=CARTESIAN_POINT('Ctrl Pts',(-6.60515146150567,-1.48329431660274,
107.767243726895));
#35336=CARTESIAN_POINT('Ctrl Pts',(-6.55847902962916,-1.66692585855356,
107.776163209626));
#35337=CARTESIAN_POINT('Ctrl Pts',(-6.51269760225618,-1.84705176507271,
107.784912414124));
#35338=CARTESIAN_POINT('Ctrl Pts',(-6.45953776308255,-2.0251081253126,107.793661618621));
#35339=CARTESIAN_POINT('Ctrl Pts',(-6.39922373482964,-2.20050553091626,
107.802410823119));
#35340=CARTESIAN_POINT('Ctrl Pts',(-6.33714894657369,-2.38102334955431,
107.811415444968));
#35341=CARTESIAN_POINT('Ctrl Pts',(-6.26749609692,-2.55872430725835,107.820420066816));
#35342=CARTESIAN_POINT('Ctrl Pts',(-6.19056070292071,-2.73299234968812,
107.829424688665));
#35343=CARTESIAN_POINT('Ctrl Pts',(-6.11362530892143,-2.9072603921179,107.838429310514));
#35344=CARTESIAN_POINT('Ctrl Pts',(-6.02940757291204,-3.07809525843261,
107.847433932363));
#35345=CARTESIAN_POINT('Ctrl Pts',(-5.93825196960901,-3.24491179316706,
107.856438554211));
#35346=CARTESIAN_POINT('Ctrl Pts',(-5.85570847447816,-3.3959680017122,107.864592446378));
#35347=CARTESIAN_POINT('Ctrl Pts',(-5.76726219193837,-3.54412000438498,
107.872746338545));
#35348=CARTESIAN_POINT('Ctrl Pts',(-5.67314178603937,-3.68886856305481,
107.880900230712));
#35349=CARTESIAN_POINT('Ctrl Pts',(-5.57913623333142,-3.83344048804244,
107.889044172852));
#35350=CARTESIAN_POINT('Ctrl Pts',(-5.47947053682363,-3.97461693282893,
107.897188114992));
#35351=CARTESIAN_POINT('Ctrl Pts',(-5.37442007181827,-4.11192143548937,
107.905332057132));
#35352=CARTESIAN_POINT('Ctrl Pts',(-5.26947568670199,-4.24908728815513,
107.913467775525));
#35353=CARTESIAN_POINT('Ctrl Pts',(-5.15915757866682,-4.38238869428596,
107.921603493918));
#35354=CARTESIAN_POINT('Ctrl Pts',(-5.04378540357022,-4.51137648647639,
107.929739212311));
#35355=CARTESIAN_POINT('Ctrl Pts',(-4.92850546265413,-4.64026115949359,
107.937868426611));
#35356=CARTESIAN_POINT('Ctrl Pts',(-4.80817974230355,-4.76483881366017,
107.945997640911));
#35357=CARTESIAN_POINT('Ctrl Pts',(-4.68316930535853,-4.88469182828842,
107.954126855212));
#35358=CARTESIAN_POINT('Ctrl Pts',(-4.55823252289801,-5.00447422711672,
107.962251279887));
#35359=CARTESIAN_POINT('Ctrl Pts',(-4.42861678389364,-5.11953727760574,
107.970375704562));
#35360=CARTESIAN_POINT('Ctrl Pts',(-4.2947212710546,-5.22949884825986,107.978500129238));
#35361=CARTESIAN_POINT('Ctrl Pts',(-4.16001292673718,-5.34012795604158,
107.986673874372));
#35362=CARTESIAN_POINT('Ctrl Pts',(-4.02097292685055,-5.44559316305205,
107.994847619506));
#35363=CARTESIAN_POINT('Ctrl Pts',(-3.8780434613653,-5.54554487059313,108.00302136464));
#35364=CARTESIAN_POINT('Ctrl Pts',(-3.73602927435292,-5.64485651664706,
108.011142767503));
#35365=CARTESIAN_POINT('Ctrl Pts',(-3.59017560674146,-5.73872487720309,
108.019264170365));
#35366=CARTESIAN_POINT('Ctrl Pts',(-3.44094696811195,-5.82684931696721,
108.027385573227));
#35367=CARTESIAN_POINT('Ctrl Pts',(-3.2917067919097,-5.91498057004909,108.035507603993));
#35368=CARTESIAN_POINT('Ctrl Pts',(-3.13909144005077,-5.99736683160999,
108.043629634759));
#35369=CARTESIAN_POINT('Ctrl Pts',(-2.98359159460155,-6.07375256300609,
108.051751665526));
#35370=CARTESIAN_POINT('Ctrl Pts',(-2.82805011596196,-6.15015874575175,
108.059875870867));
#35371=CARTESIAN_POINT('Ctrl Pts',(-2.66962293432441,-6.2205610380697,108.068000076208));
#35372=CARTESIAN_POINT('Ctrl Pts',(-2.50882230458387,-6.2847513589658,108.076124281549));
#35373=CARTESIAN_POINT('Ctrl Pts',(-2.34628111929146,-6.34963649566948,
108.084336425791));
#35374=CARTESIAN_POINT('Ctrl Pts',(-2.18131515985527,-6.40817425168384,
108.092548570034));
#35375=CARTESIAN_POINT('Ctrl Pts',(-2.01447012225202,-6.46020116765368,
108.100760714276));
#35376=CARTESIAN_POINT('Ctrl Pts',(-1.84914819595518,-6.51175313522176,
108.108897890693));
#35377=CARTESIAN_POINT('Ctrl Pts',(-1.68198172595676,-6.55691260718002,
108.117035067109));
#35378=CARTESIAN_POINT('Ctrl Pts',(-1.51351238068621,-6.59557194438129,
108.125172243526));
#35379=CARTESIAN_POINT('Ctrl Pts',(-1.34271487268815,-6.63476553443312,
108.133421871681));
#35380=CARTESIAN_POINT('Ctrl Pts',(-1.17057860116143,-6.66727794398844,
108.141671499836));
#35381=CARTESIAN_POINT('Ctrl Pts',(-0.997673498291688,-6.69305136621604,
108.149921127992));
#35382=CARTESIAN_POINT('Ctrl Pts',(-0.824768395421815,-6.71882478844367,
108.158170756147));
#35383=CARTESIAN_POINT('Ctrl Pts',(-0.651094850587449,-6.73785924430758,
108.166420384303));
#35384=CARTESIAN_POINT('Ctrl Pts',(-0.477222493360277,-6.75015167917218,
108.174670012458));
#35385=CARTESIAN_POINT('Ctrl Pts',(-0.303871997551408,-6.76240721945736,
108.182894880136));
#35386=CARTESIAN_POINT('Ctrl Pts',(-0.129805729764351,-6.76799795827916,
108.191119747813));
#35387=CARTESIAN_POINT('Ctrl Pts',(0.0444228056201317,-6.76685418893749,
108.199344615491));
#35388=CARTESIAN_POINT('Ctrl Pts',(0.21845505305805,-6.76571170818,108.207560216935));
#35389=CARTESIAN_POINT('Ctrl Pts',(0.392648848574959,-6.75784982959583,
108.215775818378));
#35390=CARTESIAN_POINT('Ctrl Pts',(0.566445567877577,-6.74325058251819,
108.223991419822));
#35391=CARTESIAN_POINT('Ctrl Pts',(0.740081404970989,-6.7286648498448,108.23219941615));
#35392=CARTESIAN_POINT('Ctrl Pts',(0.913320542615075,-6.70735419908896,
108.240407412478));
#35393=CARTESIAN_POINT('Ctrl Pts',(1.08560426551689,-6.67935269159307,108.248615408806));
#35394=CARTESIAN_POINT('Ctrl Pts',(1.25776311085951,-6.65137148061649,108.256817455677));
#35395=CARTESIAN_POINT('Ctrl Pts',(1.42896756813976,-6.61670913006465,108.265019502549));
#35396=CARTESIAN_POINT('Ctrl Pts',(1.59866386525474,-6.57545153171467,108.27322154942));
#35397=CARTESIAN_POINT('Ctrl Pts',(1.76827123680715,-6.53421555348962,108.281419298192));
#35398=CARTESIAN_POINT('Ctrl Pts',(1.93637167484358,-6.48639129711199,108.289617046963));
#35399=CARTESIAN_POINT('Ctrl Pts',(2.10242134051472,-6.43211578774421,108.297814795735));
#35400=CARTESIAN_POINT('Ctrl Pts',(2.26843933554701,-6.3778506303398,108.306010980951));
#35401=CARTESIAN_POINT('Ctrl Pts',(2.43240699471959,-6.31713677628173,108.314207166166));
#35402=CARTESIAN_POINT('Ctrl Pts',(2.59379510021734,-6.25016127616628,108.322403351382));
#35403=CARTESIAN_POINT('Ctrl Pts',(2.75517126658728,-6.18319073074718,108.330598930262));
#35404=CARTESIAN_POINT('Ctrl Pts',(2.91396792756327,-6.10995959850189,108.338794509143));
#35405=CARTESIAN_POINT('Ctrl Pts',(3.06967538907312,-6.03070327621239,108.346990088023));
#35406=CARTESIAN_POINT('Ctrl Pts',(3.22539966082515,-5.95143839737743,108.355186551701));
#35407=CARTESIAN_POINT('Ctrl Pts',(3.37803374880273,-5.86614719534679,108.36338301538));
#35408=CARTESIAN_POINT('Ctrl Pts',(3.52709209003971,-5.77511128796488,108.371579479058));
#35409=CARTESIAN_POINT('Ctrl Pts',(3.67619364319029,-5.6840489893342,108.379778318886));
#35410=CARTESIAN_POINT('Ctrl Pts',(3.82171707865581,-5.5872388550992,108.387977158714));
#35411=CARTESIAN_POINT('Ctrl Pts',(3.96320533657081,-5.48500614951129,108.396175998542));
#35412=CARTESIAN_POINT('Ctrl Pts',(4.10484138299643,-5.38266665895396,108.404383402291));
#35413=CARTESIAN_POINT('Ctrl Pts',(4.24243353989542,-5.27489349148692,108.41259080604));
#35414=CARTESIAN_POINT('Ctrl Pts',(4.37555662367105,-5.16205319936248,108.420798209789));
#35415=CARTESIAN_POINT('Ctrl Pts',(4.50875101521519,-5.0491524640061,108.429010009858));
#35416=CARTESIAN_POINT('Ctrl Pts',(4.63747129710633,-4.93117943534259,108.437221809927));
#35417=CARTESIAN_POINT('Ctrl Pts',(4.76132887346901,-4.80853786079202,108.445433609996));
#35418=CARTESIAN_POINT('Ctrl Pts',(4.88536878549057,-4.68571574070716,108.453657498983));
#35419=CARTESIAN_POINT('Ctrl Pts',(5.00453144074282,-4.55821160189771,108.461881387969));
#35420=CARTESIAN_POINT('Ctrl Pts',(5.11846744566802,-4.42646360062259,108.470105276955));
#35421=CARTESIAN_POINT('Ctrl Pts',(5.22374234451304,-4.30473072508094,108.477704008205));
#35422=CARTESIAN_POINT('Ctrl Pts',(5.32455534103403,-4.17937520772323,108.485302739455));
#35423=CARTESIAN_POINT('Ctrl Pts',(5.42066408803459,-4.05076410627577,108.492901470705));
#35424=CARTESIAN_POINT('Ctrl Pts',(5.52469196327979,-3.9115557612076,108.501126319027));
#35425=CARTESIAN_POINT('Ctrl Pts',(5.62349986955515,-3.76814214549343,108.509351167349));
#35426=CARTESIAN_POINT('Ctrl Pts',(5.71672993877672,-3.6209512295934,108.517576015671));
#35427=CARTESIAN_POINT('Ctrl Pts',(5.80985501026929,-3.47392608329998,108.52579160099));
#35428=CARTESIAN_POINT('Ctrl Pts',(5.89741456331119,-3.32313240810039,108.53400718631));
#35429=CARTESIAN_POINT('Ctrl Pts',(5.97909148676538,-3.16903044997831,108.542222771629));
#35430=CARTESIAN_POINT('Ctrl Pts',(6.06069283441437,-3.01507108267719,108.550430755052));
#35431=CARTESIAN_POINT('Ctrl Pts',(6.13642222577955,-2.85780984381845,108.558638738475));
#35432=CARTESIAN_POINT('Ctrl Pts',(6.20600627425849,-2.69773518416176,108.566846721898));
#35433=CARTESIAN_POINT('Ctrl Pts',(6.27553991280148,-2.53777649006781,108.575048759075));
#35434=CARTESIAN_POINT('Ctrl Pts',(6.33893693350134,-2.37500876252847,108.583250796252));
#35435=CARTESIAN_POINT('Ctrl Pts',(6.39597022614917,-2.20994431292134,108.591452833428));
#35436=CARTESIAN_POINT('Ctrl Pts',(6.4529736540061,-2.04496629730817,108.599650575707));
#35437=CARTESIAN_POINT('Ctrl Pts',(6.50361987537532,-1.87769429379751,108.607848317987));
#35438=CARTESIAN_POINT('Ctrl Pts',(6.54773016761079,-1.70865989950009,108.616046060266));
#35439=CARTESIAN_POINT('Ctrl Pts',(6.59183207300411,-1.53965764429559,108.624242243881));
#35440=CARTESIAN_POINT('Ctrl Pts',(6.62940042803424,-1.36889401098159,108.632438427495));
#35441=CARTESIAN_POINT('Ctrl Pts',(6.66030649961352,-1.19691534003282,108.640634611109));
#35442=CARTESIAN_POINT('Ctrl Pts',(6.69121029607473,-1.02494932911375,108.64883019137));
#35443=CARTESIAN_POINT('Ctrl Pts',(6.71545272145503,-0.851768811698276,
108.657025771631));
#35444=CARTESIAN_POINT('Ctrl Pts',(6.73295626998631,-0.677929838886081,
108.665221351892));
#35445=CARTESIAN_POINT('Ctrl Pts',(6.75046171457579,-0.504072035103136,
108.673417819933));
#35446=CARTESIAN_POINT('Ctrl Pts',(6.76122679201078,-0.329555990916877,
108.681614287973));
#35447=CARTESIAN_POINT('Ctrl Pts',(6.76522592670201,-0.154942443116709,
108.689810756014));
#35448=CARTESIAN_POINT('Ctrl Pts',(6.76922622219469,0.0197217885630407,
108.698009603188));
#35449=CARTESIAN_POINT('Ctrl Pts',(6.76645665488345,0.194483221583864,108.706208450361));
#35450=CARTESIAN_POINT('Ctrl Pts',(6.75694377679353,0.368781503401733,108.714407297534));
#35451=CARTESIAN_POINT('Ctrl Pts',(6.74742095682094,0.543261943873229,108.7226147133));
#35452=CARTESIAN_POINT('Ctrl Pts',(6.73114076583603,0.717277907320158,108.730822129066));
#35453=CARTESIAN_POINT('Ctrl Pts',(6.70818172292812,0.890273537837168,108.739029544832));
#35454=CARTESIAN_POINT('Ctrl Pts',(6.68521037478073,1.06336188792753,108.747241359484));
#35455=CARTESIAN_POINT('Ctrl Pts',(6.65555309952177,1.23542846162337,108.755453174136));
#35456=CARTESIAN_POINT('Ctrl Pts',(6.61933948700453,1.4059280763192,108.763664988789));
#35457=CARTESIAN_POINT('Ctrl Pts',(6.5830725444375,1.57667877761777,108.771888896586));
#35458=CARTESIAN_POINT('Ctrl Pts',(6.54023005705052,1.74585756041812,108.780112804384));
#35459=CARTESIAN_POINT('Ctrl Pts',(6.49099175486399,1.91293362098316,108.788336712181));
#35460=CARTESIAN_POINT('Ctrl Pts',(6.44549647299097,2.06730881533578,108.795935451105));
#35461=CARTESIAN_POINT('Ctrl Pts',(6.39454143517043,2.2198888095163,108.803534190028));
#35462=CARTESIAN_POINT('Ctrl Pts',(6.33830442585919,2.37027129357249,108.811132928952));
#35463=CARTESIAN_POINT('Ctrl Pts',(6.27796846008213,2.53161473133012,108.819285518452));
#35464=CARTESIAN_POINT('Ctrl Pts',(6.21137310086153,2.6909063624389,108.827438107952));
#35465=CARTESIAN_POINT('Ctrl Pts',(6.13867664551614,2.84761971509446,108.835590697453));
#35466=CARTESIAN_POINT('Ctrl Pts',(6.06606751590959,3.00414481772821,108.843733493753));
#35467=CARTESIAN_POINT('Ctrl Pts',(5.98737203330339,3.15809747915696,108.851876290054));
#35468=CARTESIAN_POINT('Ctrl Pts',(5.90279789406262,3.3089675159859,108.860019086354));
#35469=CARTESIAN_POINT('Ctrl Pts',(5.81832523890025,3.45965651749149,108.86815211177));
#35470=CARTESIAN_POINT('Ctrl Pts',(5.72798816050227,3.60726994791767,108.876285137186));
#35471=CARTESIAN_POINT('Ctrl Pts',(5.63204177845997,3.75131902211495,108.884418162601));
#35472=CARTESIAN_POINT('Ctrl Pts',(5.53616136407185,3.89526905579284,108.892545596179));
#35473=CARTESIAN_POINT('Ctrl Pts',(5.43467952445377,4.03565930826703,108.900673029757));
#35474=CARTESIAN_POINT('Ctrl Pts',(5.32789673113761,4.17202653662859,108.908800463335));
#35475=CARTESIAN_POINT('Ctrl Pts',(5.2211670204732,4.30832597565942,108.916923856695));
#35476=CARTESIAN_POINT('Ctrl Pts',(5.10914182745673,4.44060608494335,108.925047250055));
#35477=CARTESIAN_POINT('Ctrl Pts',(4.9921642495206,4.56843355055193,108.933170643416));
#35478=CARTESIAN_POINT('Ctrl Pts',(4.87522254724616,4.69622181296454,108.941291545426));
#35479=CARTESIAN_POINT('Ctrl Pts',(4.75333173178667,4.81955988195647,108.949412447436));
#35480=CARTESIAN_POINT('Ctrl Pts',(4.62687436706289,4.93804845980843,108.957533349446));
#35481=CARTESIAN_POINT('Ctrl Pts',(4.50040460057786,5.0565486579172,108.965655047878));
#35482=CARTESIAN_POINT('Ctrl Pts',(4.36936765185437,5.17019815898645,108.973776746311));
#35483=CARTESIAN_POINT('Ctrl Pts',(4.23418226466472,5.27863519762436,108.981898444743));
#35484=CARTESIAN_POINT('Ctrl Pts',(4.0989913839812,5.38707664279038,108.990020473215));
#35485=CARTESIAN_POINT('Ctrl Pts',(3.95965201809419,5.49030497918769,108.998142501687));
#35486=CARTESIAN_POINT('Ctrl Pts',(3.81661487679756,5.58799963155042,109.006264530159));
#35487=CARTESIAN_POINT('Ctrl Pts',(3.6734965061454,5.68574976372473,109.014391171049));
#35488=CARTESIAN_POINT('Ctrl Pts',(3.52667647083157,5.77795973283162,109.022517811939));
#35489=CARTESIAN_POINT('Ctrl Pts',(3.37663368089296,5.86435281894424,109.03064445283));
#35490=CARTESIAN_POINT('Ctrl Pts',(3.28530383696744,5.91693959818328,109.03559107402));
#35491=CARTESIAN_POINT('Ctrl Pts',(3.19278045746336,5.96737206540541,109.04053769521));
#35492=CARTESIAN_POINT('Ctrl Pts',(3.09917575053271,6.01559628526633,109.0454843164));
#35493=CARTESIAN_POINT('Ctrl Pts',(3.0991757505325,6.01559628526643,107.045813349661));
#35494=CARTESIAN_POINT('Ctrl Pts',(2.9438094780766,6.09563945326048,107.054012219891));
#35495=CARTESIAN_POINT('Ctrl Pts',(2.78530897263697,6.1696758601344,107.06221109012));
#35496=CARTESIAN_POINT('Ctrl Pts',(2.624181600378,6.23746422260181,107.07040996035));
#35497=CARTESIAN_POINT('Ctrl Pts',(2.46305199894301,6.30525352291231,107.07860894401));
#35498=CARTESIAN_POINT('Ctrl Pts',(2.29929578858001,6.36679446737404,107.086807927669));
#35499=CARTESIAN_POINT('Ctrl Pts',(2.13344051535257,6.4218938458567,107.095006911329));
#35500=CARTESIAN_POINT('Ctrl Pts',(1.96755286063483,6.47700398191103,107.103207495754));
#35501=CARTESIAN_POINT('Ctrl Pts',(1.79956566691533,6.52566993411948,107.111408080179));
#35502=CARTESIAN_POINT('Ctrl Pts',(1.63002189542284,6.56774829149551,107.119608664604));
#35503=CARTESIAN_POINT('Ctrl Pts',(1.45710134210579,6.61066471818628,107.12797257903));
#35504=CARTESIAN_POINT('Ctrl Pts',(1.28256193294628,6.64672828420124,107.136336493456));
#35505=CARTESIAN_POINT('Ctrl Pts',(1.10699027058011,6.67584163539257,107.144700407882));
#35506=CARTESIAN_POINT('Ctrl Pts',(0.934608297546703,6.70442607124254,107.152912371315));
#35507=CARTESIAN_POINT('Ctrl Pts',(0.761231620545215,6.72631067366722,107.161124334747));
#35508=CARTESIAN_POINT('Ctrl Pts',(0.587419989921386,6.74145583353038,107.169336298179));
#35509=CARTESIAN_POINT('Ctrl Pts',(0.408784144552109,6.75702135366099,107.177776188102));
#35510=CARTESIAN_POINT('Ctrl Pts',(0.229689264636626,6.76546789067559,107.186216078025));
#35511=CARTESIAN_POINT('Ctrl Pts',(0.0507419610713189,6.76680975448451,
107.194655967949));
#35512=CARTESIAN_POINT('Ctrl Pts',(-0.128205342493988,6.76815161829342,
107.203095857872));
#35513=CARTESIAN_POINT('Ctrl Pts',(-0.307004666234908,6.76238887731013,
107.211535747795));
#35514=CARTESIAN_POINT('Ctrl Pts',(-0.485056527264841,6.74959325925332,
107.219975637718));
#35515=CARTESIAN_POINT('Ctrl Pts',(-0.667450634673003,6.73648558758559,
107.228621355771));
#35516=CARTESIAN_POINT('Ctrl Pts',(-0.849476241434182,6.71596863773433,
107.237267073823));
#35517=CARTESIAN_POINT('Ctrl Pts',(-1.03052163609518,6.6880725293271,107.245912791875));
#35518=CARTESIAN_POINT('Ctrl Pts',(-1.2113346053658,6.66021223383793,107.254547410588));
#35519=CARTESIAN_POINT('Ctrl Pts',(-1.39116957185494,6.62499171633672,107.2631820293));
#35520=CARTESIAN_POINT('Ctrl Pts',(-1.56941903346027,6.58249290902867,107.271816648013));
#35521=CARTESIAN_POINT('Ctrl Pts',(-1.7539635736031,6.53849320894178,107.280756207915));
#35522=CARTESIAN_POINT('Ctrl Pts',(-1.93680825493122,6.48669174887171,107.289695767817));
#35523=CARTESIAN_POINT('Ctrl Pts',(-2.11728625709747,6.42723796863833,107.29863532772));
#35524=CARTESIAN_POINT('Ctrl Pts',(-2.29112406528735,6.36997162747587,107.30724598099));
#35525=CARTESIAN_POINT('Ctrl Pts',(-2.46276589402842,6.30560607927925,107.315856634261));
#35526=CARTESIAN_POINT('Ctrl Pts',(-2.63162710199824,6.23432657117257,107.324467287531));
#35527=CARTESIAN_POINT('Ctrl Pts',(-2.80032847153802,6.16311453388887,107.333069790242));
#35528=CARTESIAN_POINT('Ctrl Pts',(-2.96625418783669,6.08500170293773,107.341672292954));
#35529=CARTESIAN_POINT('Ctrl Pts',(-3.12883680410529,6.00022243364996,107.350274795665));
#35530=CARTESIAN_POINT('Ctrl Pts',(-3.29123643690934,5.91553858172459,107.358867616432));
#35531=CARTESIAN_POINT('Ctrl Pts',(-3.45030020608423,5.82420340032712,107.3674604372));
#35532=CARTESIAN_POINT('Ctrl Pts',(-3.60548242248394,5.72649853760213,107.376053257967));
#35533=CARTESIAN_POINT('Ctrl Pts',(-3.62377135156097,5.7149835757314,107.377065960925));
#35534=CARTESIAN_POINT('Ctrl Pts',(-3.64200639260673,5.70338019469417,107.378078663883));
#35535=CARTESIAN_POINT('Ctrl Pts',(-3.66018667337285,5.69168889839069,107.379091366841));
#35536=CARTESIAN_POINT('Ctrl Pts',(-3.81449075443639,5.59245969749119,107.387686624601));
#35537=CARTESIAN_POINT('Ctrl Pts',(-3.9646663544448,5.48701045969764,107.396281882361));
#35538=CARTESIAN_POINT('Ctrl Pts',(-4.11022643393577,5.37571647892406,107.404877140121));
#35539=CARTESIAN_POINT('Ctrl Pts',(-4.25592282426801,5.26431827605744,107.413480446976));
#35540=CARTESIAN_POINT('Ctrl Pts',(-4.3969948241579,5.14706459065193,107.42208375383));
#35541=CARTESIAN_POINT('Ctrl Pts',(-4.53298929980819,5.02437030958353,107.430687060684));
#35542=CARTESIAN_POINT('Ctrl Pts',(-4.67462215357932,4.89658908107391,107.439647063624));
#35543=CARTESIAN_POINT('Ctrl Pts',(-4.81074720568499,4.7629067710744,107.448607066565));
#35544=CARTESIAN_POINT('Ctrl Pts',(-4.9408968752471,4.6238325086635,107.457567069505));
#35545=CARTESIAN_POINT('Ctrl Pts',(-5.06620719043081,4.48992944371309,107.466193912709));
#35546=CARTESIAN_POINT('Ctrl Pts',(-5.18597831737321,4.3510284281807,107.474820755914));
#35547=CARTESIAN_POINT('Ctrl Pts',(-5.29983536026046,4.20761620803667,107.483447599119));
#35548=CARTESIAN_POINT('Ctrl Pts',(-5.41380122169928,4.06406692206274,107.492082687405));
#35549=CARTESIAN_POINT('Ctrl Pts',(-5.52184153431556,3.9159980696293,107.500717775691));
#35550=CARTESIAN_POINT('Ctrl Pts',(-5.62362453945761,3.76392561552565,107.509352863977));
#35551=CARTESIAN_POINT('Ctrl Pts',(-5.72555871278871,3.61162730330887,107.518000777102));
#35552=CARTESIAN_POINT('Ctrl Pts',(-5.82121684441455,3.45531376477537,107.526648690227));
#35553=CARTESIAN_POINT('Ctrl Pts',(-5.91031219195361,3.29552708889558,107.535296603353));
#35554=CARTESIAN_POINT('Ctrl Pts',(-5.92030733363478,3.27760145631995,107.536266767557));
#35555=CARTESIAN_POINT('Ctrl Pts',(-5.93021992915776,3.25963213489651,107.537236931761));
#35556=CARTESIAN_POINT('Ctrl Pts',(-5.94004961119222,3.24161990624674,107.538207095965));
#35557=CARTESIAN_POINT('Ctrl Pts',(-6.02650562242684,3.08319510297793,107.546740080759));
#35558=CARTESIAN_POINT('Ctrl Pts',(-6.10671679174137,2.9211319740975,107.555273065552));
#35559=CARTESIAN_POINT('Ctrl Pts',(-6.18037722501124,2.75594382318696,107.563806050346));
#35560=CARTESIAN_POINT('Ctrl Pts',(-6.25393679587604,2.59098186255866,107.572327351019));
#35561=CARTESIAN_POINT('Ctrl Pts',(-6.32096338049466,2.42290369930237,107.580848651693));
#35562=CARTESIAN_POINT('Ctrl Pts',(-6.38119643998813,2.25224798685288,107.589369952366));
#35563=CARTESIAN_POINT('Ctrl Pts',(-6.44135375726403,2.08180687154008,107.597880537625));
#35564=CARTESIAN_POINT('Ctrl Pts',(-6.49473447280367,1.90879496828615,107.606391122883));
#35565=CARTESIAN_POINT('Ctrl Pts',(-6.54112551533562,1.73377218590718,107.614901708142));
#35566=CARTESIAN_POINT('Ctrl Pts',(-6.58744621359749,1.55901479635409,107.623399388519));
#35567=CARTESIAN_POINT('Ctrl Pts',(-6.62679829947891,1.38225291815665,107.631897068896));
#35568=CARTESIAN_POINT('Ctrl Pts',(-6.6590180784668,1.20406280178914,107.640394749274));
#35569=CARTESIAN_POINT('Ctrl Pts',(-6.69120843705091,1.02603539371257,107.648884670281));
#35570=CARTESIAN_POINT('Ctrl Pts',(-6.71627941206488,0.84658266026334,107.657374591288));
#35571=CARTESIAN_POINT('Ctrl Pts',(-6.73411774491939,0.666293627135781,
107.665864512295));
#35572=CARTESIAN_POINT('Ctrl Pts',(-6.7519376287008,0.486191055690526,107.674345652707));
#35573=CARTESIAN_POINT('Ctrl Pts',(-6.76253975861578,0.305254227259429,
107.68282679312));
#35574=CARTESIAN_POINT('Ctrl Pts',(-6.76586233578067,0.124080027661641,
107.691307933532));
#35575=CARTESIAN_POINT('Ctrl Pts',(-6.7666291224273,0.0822685210896604,
107.693265216958));
#35576=CARTESIAN_POINT('Ctrl Pts',(-6.76700841916055,0.0404444015700853,
107.695222500384));
#35577=CARTESIAN_POINT('Ctrl Pts',(-6.76699985827674,-0.00138494859027308,
107.69717978381));
#35578=CARTESIAN_POINT('',(-6.76721124277169,-0.000653705868658438,107.303185781308));
#35579=CARTESIAN_POINT('Ctrl Pts',(3.09917575053261,6.01559628526638,106.651392015122));
#35580=CARTESIAN_POINT('Ctrl Pts',(2.9338238445927,6.10078395293757,106.660141463035));
#35581=CARTESIAN_POINT('Ctrl Pts',(2.76495772122992,6.17915010267045,106.668890910947));
#35582=CARTESIAN_POINT('Ctrl Pts',(2.59315093316722,6.25042856433173,106.67764035886));
#35583=CARTESIAN_POINT('Ctrl Pts',(2.4213455324563,6.32170645041446,106.68638973612));
#35584=CARTESIAN_POINT('Ctrl Pts',(2.24659977927605,6.38589665313452,106.69513911338));
#35585=CARTESIAN_POINT('Ctrl Pts',(2.06950718689935,6.4427811543907,106.70388849064));
#35586=CARTESIAN_POINT('Ctrl Pts',(1.89241596572879,6.49966521519719,106.712637800154));
#35587=CARTESIAN_POINT('Ctrl Pts',(1.71297821457217,6.54924360009541,106.721387109669));
#35588=CARTESIAN_POINT('Ctrl Pts',(1.53180337335866,6.59134792173551,106.730136419184));
#35589=CARTESIAN_POINT('Ctrl Pts',(1.350629874778,6.63345193135301,106.73888566386));
#35590=CARTESIAN_POINT('Ctrl Pts',(1.16771959102965,6.66808192368236,106.747634908536));
#35591=CARTESIAN_POINT('Ctrl Pts',(0.983693746906934,6.69512028363167,106.756384153212));
#35592=CARTESIAN_POINT('Ctrl Pts',(0.799669205419912,6.72215845218867,106.765133335956));
#35593=CARTESIAN_POINT('Ctrl Pts',(0.614529402873468,6.74160505424579,106.7738825187));
#35594=CARTESIAN_POINT('Ctrl Pts',(0.428903127363191,6.75339404354122,106.782631701445));
#35595=CARTESIAN_POINT('Ctrl Pts',(0.243278104163796,6.7651829533033,106.791380825163));
#35596=CARTESIAN_POINT('Ctrl Pts',(0.0571669005390081,6.76931433552276,
106.800129948882));
#35597=CARTESIAN_POINT('Ctrl Pts',(-0.128798404777648,6.76577415902473,
106.8088790726));
#35598=CARTESIAN_POINT('Ctrl Pts',(-0.314762517259244,6.76223400523441,
106.8176281402));
#35599=CARTESIAN_POINT('Ctrl Pts',(-0.500580446819668,6.75102239665088,
106.826377207799));
#35600=CARTESIAN_POINT('Ctrl Pts',(-0.68562111884278,6.73217741012496,106.835126275398));
#35601=CARTESIAN_POINT('Ctrl Pts',(-0.870660665414785,6.71333253821768,
106.843875289784));
#35602=CARTESIAN_POINT('Ctrl Pts',(-1.05492267885529,6.68685441030606,106.85262430417));
#35603=CARTESIAN_POINT('Ctrl Pts',(-1.23778137635307,6.65283295028167,106.861373318555));
#35604=CARTESIAN_POINT('Ctrl Pts',(-1.42999922978891,6.61707018861856,106.870570128923));
#35605=CARTESIAN_POINT('Ctrl Pts',(-1.62066601233729,6.57297172934404,106.87976693929));
#35606=CARTESIAN_POINT('Ctrl Pts',(-1.80906628500408,6.52070304311288,106.888963749658));
#35607=CARTESIAN_POINT('Ctrl Pts',(-1.98831342545542,6.47097374915026,106.897713747395));
#35608=CARTESIAN_POINT('Ctrl Pts',(-2.16550875896709,6.41384933989526,106.906463745133));
#35609=CARTESIAN_POINT('Ctrl Pts',(-2.34005036714011,6.34952386240476,106.915213742871));
#35610=CARTESIAN_POINT('Ctrl Pts',(-2.51458843547092,6.28519968948595,106.923963563152));
#35611=CARTESIAN_POINT('Ctrl Pts',(-2.68647261718061,6.21367483971097,106.932713383433));
#35612=CARTESIAN_POINT('Ctrl Pts',(-2.8551190590874,6.1351922674384,106.941463203713));
#35613=CARTESIAN_POINT('Ctrl Pts',(-3.02376230488902,6.05671118252928,106.950212858172));
#35614=CARTESIAN_POINT('Ctrl Pts',(-3.18916767379931,5.97127275992619,106.95896251263));
#35615=CARTESIAN_POINT('Ctrl Pts',(-3.35077334102822,5.87916720437977,106.967712167089));
#35616=CARTESIAN_POINT('Ctrl Pts',(-3.51237616037403,5.78706327195622,106.976461667357));
#35617=CARTESIAN_POINT('Ctrl Pts',(-3.67017916302335,5.68829258362275,106.985211167626));
#35618=CARTESIAN_POINT('Ctrl Pts',(-3.82364636566498,5.58319061741018,106.993960667894));
#35619=CARTESIAN_POINT('Ctrl Pts',(-3.97711106778832,5.47809036367677,107.002710025603));
#35620=CARTESIAN_POINT('Ctrl Pts',(-4.12623987481959,5.366659200432,107.011459383311));
#35621=CARTESIAN_POINT('Ctrl Pts',(-4.2705262821396,5.2492755951231,107.02020874102));
#35622=CARTESIAN_POINT('Ctrl Pts',(-4.41481053025027,5.13189374642995,107.028957967796));
#35623=CARTESIAN_POINT('Ctrl Pts',(-4.55425230136596,5.00855981477294,107.037707194573));
#35624=CARTESIAN_POINT('Ctrl Pts',(-4.6883780063063,4.87969268191998,107.046456421349));
#35625=CARTESIAN_POINT('Ctrl Pts',(-4.82250188228965,4.75082730631738,107.05520552882));
#35626=CARTESIAN_POINT('Ctrl Pts',(-4.95130963053026,4.61642907903461,107.063954636291));
#35627=CARTESIAN_POINT('Ctrl Pts',(-5.07436379033417,4.47695444731633,107.072703743762));
#35628=CARTESIAN_POINT('Ctrl Pts',(-5.19741643562863,4.33748153220517,107.081452743551));
#35629=CARTESIAN_POINT('Ctrl Pts',(-5.31471544462838,4.19293255254507,107.090201743341));
#35630=CARTESIAN_POINT('Ctrl Pts',(-5.42586245275699,4.04379841779507,107.098950743131));
#35631=CARTESIAN_POINT('Ctrl Pts',(-5.53702160019218,3.8946479948425,107.107700698473));
#35632=CARTESIAN_POINT('Ctrl Pts',(-5.6420272308131,3.74091164443761,107.116450653815));
#35633=CARTESIAN_POINT('Ctrl Pts',(-5.7405226523302,3.58311159163148,107.125200609157));
#35634=CARTESIAN_POINT('Ctrl Pts',(-5.83901427066977,3.42531763191684,107.13395022664));
#35635=CARTESIAN_POINT('Ctrl Pts',(-5.93099603115803,3.26346052695498,107.142699844122));
#35636=CARTESIAN_POINT('Ctrl Pts',(-6.01615550622821,3.09809004466946,107.151449461605));
#35637=CARTESIAN_POINT('Ctrl Pts',(-6.10131214578867,2.93272506863688,107.160198787756));
#35638=CARTESIAN_POINT('Ctrl Pts',(-6.17964682328814,2.76384720416745,107.168948113907));
#35639=CARTESIAN_POINT('Ctrl Pts',(-6.25089348288629,2.59203002791435,107.177697440058));
#35640=CARTESIAN_POINT('Ctrl Pts',(-6.32213814889398,2.42021765936854,107.18644652139));
#35641=CARTESIAN_POINT('Ctrl Pts',(-6.38629508412653,2.24546640831725,107.195195602721));
#35642=CARTESIAN_POINT('Ctrl Pts',(-6.44314639819879,2.06836976659831,107.203944684053));
#35643=CARTESIAN_POINT('Ctrl Pts',(-6.50000285283766,1.8912571115805,107.212694556487));
#35644=CARTESIAN_POINT('Ctrl Pts',(-6.54955227673312,1.71179891440015,107.221444428922));
#35645=CARTESIAN_POINT('Ctrl Pts',(-6.59162635926444,1.53060476278177,107.230194301356));
#35646=CARTESIAN_POINT('Ctrl Pts',(-6.63369752055244,1.34942319164459,107.238943566279));
#35647=CARTESIAN_POINT('Ctrl Pts',(-6.66829431424292,1.16650618642486,107.247692831201));
#35648=CARTESIAN_POINT('Ctrl Pts',(-6.69529923745447,0.982474997616562,
107.256442096124));
#35649=CARTESIAN_POINT('Ctrl Pts',(-6.72230554731467,0.798434359175721,
107.265191810303));
#35650=CARTESIAN_POINT('Ctrl Pts',(-6.74171916496722,0.613279706238294,
107.273941524483));
#35651=CARTESIAN_POINT('Ctrl Pts',(-6.75347414817288,0.427639953653314,
107.282691238663));
#35652=CARTESIAN_POINT('Ctrl Pts',(-6.76248837758739,0.285283364198783,
107.289400897838));
#35653=CARTESIAN_POINT('Ctrl Pts',(-6.76699999999987,0.142641701107611,
107.296110557014));
#35654=CARTESIAN_POINT('Ctrl Pts',(-6.767,6.34351679601791E-12,107.30282021619));
#35655=CARTESIAN_POINT('Ctrl Pts',(-6.76699921757691,-0.00325412254306615,
107.30282021619));
#35656=CARTESIAN_POINT('Ctrl Pts',(-6.7669011553275,-0.207176118798005,
107.312373624824));
#35657=CARTESIAN_POINT('Ctrl Pts',(-6.75758045334832,-0.410786772883343,
107.321927033457));
#35658=CARTESIAN_POINT('Ctrl Pts',(-6.73915089857601,-0.613297779404236,
107.331480442091));
#35659=CARTESIAN_POINT('Ctrl Pts',(-6.721475047404,-0.80752680208984,107.340643150104));
#35660=CARTESIAN_POINT('Ctrl Pts',(-6.69542064108127,-1.00074419645186,
107.349805858117));
#35661=CARTESIAN_POINT('Ctrl Pts',(-6.66113955109404,-1.19227047302647,
107.35896856613));
#35662=CARTESIAN_POINT('Ctrl Pts',(-6.62676727658224,-1.38430619175933,
107.368155646098));
#35663=CARTESIAN_POINT('Ctrl Pts',(-6.58412459563606,-1.57464159892993,
107.377342726066));
#35664=CARTESIAN_POINT('Ctrl Pts',(-6.53341363497359,-1.76261035806021,
107.386529806034));
#35665=CARTESIAN_POINT('Ctrl Pts',(-6.48254029096963,-1.95118101853107,
107.395746304273));
#35666=CARTESIAN_POINT('Ctrl Pts',(-6.42354701191558,-2.13736966837478,
107.404962802511));
#35667=CARTESIAN_POINT('Ctrl Pts',(-6.35668567204398,-2.32052499810513,
107.414179300749));
#35668=CARTESIAN_POINT('Ctrl Pts',(-6.34874965654843,-2.34226437002954,
107.41527324043));
#35669=CARTESIAN_POINT('Ctrl Pts',(-6.34070284853216,-2.36396103460376,
107.416367180112));
#35670=CARTESIAN_POINT('Ctrl Pts',(-6.3325457126643,-2.38561392455213,107.417461119793));
#35671=CARTESIAN_POINT('Ctrl Pts',(-6.26807568330373,-2.55674782170998,
107.426107086284));
#35672=CARTESIAN_POINT('Ctrl Pts',(-6.19660697721829,-2.72541921646342,
107.434753052775));
#35673=CARTESIAN_POINT('Ctrl Pts',(-6.11834270474009,-2.8910502498839,107.443399019266));
#35674=CARTESIAN_POINT('Ctrl Pts',(-6.04017854290617,-3.05646941869561,
107.45203392639));
#35675=CARTESIAN_POINT('Ctrl Pts',(-5.95523627760394,-3.21885570674108,
107.460668833514));
#35676=CARTESIAN_POINT('Ctrl Pts',(-5.86376748714751,-3.37765004946808,
107.469303740639));
#35677=CARTESIAN_POINT('Ctrl Pts',(-5.76926200667351,-3.54171623620877,
107.47822531971));
#35678=CARTESIAN_POINT('Ctrl Pts',(-5.66778928891598,-3.70194756933119,
107.487146898782));
#35679=CARTESIAN_POINT('Ctrl Pts',(-5.55968042126128,-3.85775097867191,
107.496068477853));
#35680=CARTESIAN_POINT('Ctrl Pts',(-5.45533433771433,-4.00813157113072,
107.504679536829));
#35681=CARTESIAN_POINT('Ctrl Pts',(-5.34480643133607,-4.15438697055638,
107.513290595805));
#35682=CARTESIAN_POINT('Ctrl Pts',(-5.22844071569663,-4.29600939040474,
107.52190165478));
#35683=CARTESIAN_POINT('Ctrl Pts',(-5.11218473829912,-4.43749825377312,
107.53050459313));
#35684=CARTESIAN_POINT('Ctrl Pts',(-4.99010212077704,-4.57436261358622,
107.53910753148));
#35685=CARTESIAN_POINT('Ctrl Pts',(-4.86257905903547,-4.7061251465117,107.547710469829));
#35686=CARTESIAN_POINT('Ctrl Pts',(-4.73519879362234,-4.83774013588175,
107.556303774878));
#35687=CARTESIAN_POINT('Ctrl Pts',(-4.6023904490695,-4.9642644767047,107.564897079927));
#35688=CARTESIAN_POINT('Ctrl Pts',(-4.46457936745683,-5.08525516288797,
107.573490384975));
#35689=CARTESIAN_POINT('Ctrl Pts',(-4.4492249572258,-5.09873550574613,107.574447819816));
#35690=CARTESIAN_POINT('Ctrl Pts',(-4.43380848458944,-5.11214719161138,
107.575405254657));
#35691=CARTESIAN_POINT('Ctrl Pts',(-4.41833056731215,-5.12548963494758,
107.576362689497));
#35692=CARTESIAN_POINT('Ctrl Pts',(-4.27937132056985,-5.24527680285168,
107.584958447045));
#35693=CARTESIAN_POINT('Ctrl Pts',(-4.13561940654779,-5.35933932355982,
107.593554204592));
#35694=CARTESIAN_POINT('Ctrl Pts',(-3.98757292330089,-5.46731663445219,
107.60214996214));
#35695=CARTESIAN_POINT('Ctrl Pts',(-3.83938830765185,-5.57539469184662,
107.610753739821));
#35696=CARTESIAN_POINT('Ctrl Pts',(-3.68690137136883,-5.67737602660814,
107.619357517503));
#35697=CARTESIAN_POINT('Ctrl Pts',(-3.53063855954867,-5.77294382112177,
107.627961295185));
#35698=CARTESIAN_POINT('Ctrl Pts',(-3.3682344825807,-5.87226751352861,107.636903208853));
#35699=CARTESIAN_POINT('Ctrl Pts',(-3.20175206593238,-5.9646631704105,107.645845122521));
#35700=CARTESIAN_POINT('Ctrl Pts',(-3.03180835814051,-6.04982868183136,
107.654787036189));
#35701=CARTESIAN_POINT('Ctrl Pts',(-2.86784583217706,-6.13199678654658,
107.663414238519));
#35702=CARTESIAN_POINT('Ctrl Pts',(-2.70066179391385,-6.20743492554849,
107.67204144085));
#35703=CARTESIAN_POINT('Ctrl Pts',(-2.53082935546811,-6.27592158758384,
107.680668643181));
#35704=CARTESIAN_POINT('Ctrl Pts',(-2.36083517762041,-6.34447347268177,
107.689304061601));
#35705=CARTESIAN_POINT('Ctrl Pts',(-2.188187851084,-6.406060560975,107.697939480022));
#35706=CARTESIAN_POINT('Ctrl Pts',(-2.01347627982301,-6.46051099144565,
107.706574898442));
#35707=CARTESIAN_POINT('Ctrl Pts',(-1.83850659710088,-6.51504186467157,
107.715223074463));
#35708=CARTESIAN_POINT('Ctrl Pts',(-1.66146686887881,-6.56241492782876,
107.723871250484));
#35709=CARTESIAN_POINT('Ctrl Pts',(-1.48295828353281,-6.60250889657117,
107.732519426505));
#35710=CARTESIAN_POINT('Ctrl Pts',(-1.46407275205353,-6.60675068643997,
107.733434370737));
#35711=CARTESIAN_POINT('Ctrl Pts',(-1.44517078630128,-6.61091105022795,
107.734349314969));
#35712=CARTESIAN_POINT('Ctrl Pts',(-1.42625310231533,-6.61498987815824,
107.735264259201));
#35713=CARTESIAN_POINT('Ctrl Pts',(-1.25616980984483,-6.65166141175181,
107.743490251742));
#35714=CARTESIAN_POINT('Ctrl Pts',(-1.0844480393287,-6.68181714361858,107.751716244283));
#35715=CARTESIAN_POINT('Ctrl Pts',(-0.91162781215005,-6.70531309724718,
107.759942236825));
#35716=CARTESIAN_POINT('Ctrl Pts',(-0.738988764641646,-6.72878441840537,
107.768159605476));
#35717=CARTESIAN_POINT('Ctrl Pts',(-0.56525390581976,-6.74560981703483,
107.776376974128));
#35718=CARTESIAN_POINT('Ctrl Pts',(-0.390975243171381,-6.75569591968341,
107.784594342779));
#35719=CARTESIAN_POINT('Ctrl Pts',(-0.216844416769153,-6.76577346654248,
107.792804740841));
#35720=CARTESIAN_POINT('Ctrl Pts',(-0.0421710609531744,-6.76912308256552,
107.801015138904));
#35721=CARTESIAN_POINT('Ctrl Pts',(0.132485768440468,-6.76570295838952,
107.809225536966));
#35722=CARTESIAN_POINT('Ctrl Pts',(0.307029379032054,-6.76228505126031,
107.817430612755));
#35723=CARTESIAN_POINT('Ctrl Pts',(0.481556127602511,-6.75210615227238,
107.825635688544));
#35724=CARTESIAN_POINT('Ctrl Pts',(0.655504918904233,-6.73517648627654,
107.833840764333));
#35725=CARTESIAN_POINT('Ctrl Pts',(0.82937573990617,-6.71825440878489,107.842042162302));
#35726=CARTESIAN_POINT('Ctrl Pts',(1.0026687639085,-6.69458762748705,107.850243560272));
#35727=CARTESIAN_POINT('Ctrl Pts',(1.17482588738742,-6.66423837616305,107.858444958241));
#35728=CARTESIAN_POINT('Ctrl Pts',(1.34696952608683,-6.63389150204515,107.866645713809));
#35729=CARTESIAN_POINT('Ctrl Pts',(1.51797708740693,-6.59686325407021,107.874846469377));
#35730=CARTESIAN_POINT('Ctrl Pts',(1.68729818408293,-6.55326741694481,107.883047224944));
#35731=CARTESIAN_POINT('Ctrl Pts',(1.85661842068835,-6.50967180126551,107.891247938856));
#35732=CARTESIAN_POINT('Ctrl Pts',(2.02425186239254,-6.45950875121017,107.899448652768));
#35733=CARTESIAN_POINT('Ctrl Pts',(2.18966098654431,-6.40294258634308,107.90764936668));
#35734=CARTESIAN_POINT('Ctrl Pts',(2.35509924674841,-6.34636645760763,107.915851525109));
#35735=CARTESIAN_POINT('Ctrl Pts',(2.51831206970158,-6.28338508291823,107.924053683539));
#35736=CARTESIAN_POINT('Ctrl Pts',(2.67877964078278,-6.21421182742653,107.932255841968));
#35737=CARTESIAN_POINT('Ctrl Pts',(2.83930455851148,-6.14501385133692,107.940460931621));
#35738=CARTESIAN_POINT('Ctrl Pts',(2.99708194111754,-6.06961972818204,107.948666021274));
#35739=CARTESIAN_POINT('Ctrl Pts',(3.1516143525597,-5.98828990386569,107.956871110927));
#35740=CARTESIAN_POINT('Ctrl Pts',(3.30632329901144,-5.90686716984075,107.965085573925));
#35741=CARTESIAN_POINT('Ctrl Pts',(3.45777955091906,-5.81949535480991,107.973300036923));
#35742=CARTESIAN_POINT('Ctrl Pts',(3.60551165794221,-5.72648013045036,107.981514499921));
#35743=CARTESIAN_POINT('Ctrl Pts',(3.75333129156968,-5.63340979751014,107.989733829728));
#35744=CARTESIAN_POINT('Ctrl Pts',(3.89742208688876,-5.53468959248881,107.997953159536));
#35745=CARTESIAN_POINT('Ctrl Pts',(4.03734385191801,-5.43066695916623,108.006172489343));
#35746=CARTESIAN_POINT('Ctrl Pts',(4.17748241723885,-5.32648314908012,108.014404554504));
#35747=CARTESIAN_POINT('Ctrl Pts',(4.31343876444354,-5.21698071697537,108.022636619664));
#35748=CARTESIAN_POINT('Ctrl Pts',(4.44480688958729,-5.10254649310297,108.030868684825));
#35749=CARTESIAN_POINT('Ctrl Pts',(4.56288999321656,-4.99968479585735,108.038268256086));
#35750=CARTESIAN_POINT('Ctrl Pts',(4.67726631022453,-4.89283899070071,108.045667827348));
#35751=CARTESIAN_POINT('Ctrl Pts',(4.78766833474416,-4.78231334361186,108.053067398609));
#35752=CARTESIAN_POINT('Ctrl Pts',(4.90934823851321,-4.66049718887831,108.061222857016));
#35753=CARTESIAN_POINT('Ctrl Pts',(5.02657439131357,-4.53383532421019,108.069378315422));
#35754=CARTESIAN_POINT('Ctrl Pts',(5.13893230645968,-4.40268824124819,108.077533773829));
#35755=CARTESIAN_POINT('Ctrl Pts',(5.25115346725375,-4.27170078152526,108.085679305971));
#35756=CARTESIAN_POINT('Ctrl Pts',(5.35851794975707,-4.13623924461395,108.093824838113));
#35757=CARTESIAN_POINT('Ctrl Pts',(5.46064631275775,-3.99670249667963,108.101970370255));
#35758=CARTESIAN_POINT('Ctrl Pts',(5.56267184766199,-3.85730624153059,108.110107701055));
#35759=CARTESIAN_POINT('Ctrl Pts',(5.65947154441353,-3.71384323670518,108.118245031856));
#35760=CARTESIAN_POINT('Ctrl Pts',(5.7507046533086,-3.56674711612903,108.126382362656));
#35761=CARTESIAN_POINT('Ctrl Pts',(5.84186507693061,-3.41976818679871,108.134513210459));
#35762=CARTESIAN_POINT('Ctrl Pts',(5.92746755136478,-3.26916221418646,108.14264405826));
#35763=CARTESIAN_POINT('Ctrl Pts',(6.0072132843546,-3.11539364387129,108.150774906062));
#35764=CARTESIAN_POINT('Ctrl Pts',(6.08691223601707,-2.96171527898222,108.158900984056));
#35765=CARTESIAN_POINT('Ctrl Pts',(6.16076112060873,-2.80487833479093,108.16702706205));
#35766=CARTESIAN_POINT('Ctrl Pts',(6.22850595567014,-2.6453738034882,108.175153140044));
#35767=CARTESIAN_POINT('Ctrl Pts',(6.29649100154348,-2.48530369825005,108.183308031626));
#35768=CARTESIAN_POINT('Ctrl Pts',(6.35832843998911,-2.32254737285463,108.191462923208));
#35769=CARTESIAN_POINT('Ctrl Pts',(6.41380916033727,-2.1576239372916,108.19961781479));
#35770=CARTESIAN_POINT('Ctrl Pts',(6.46907352527439,-1.99334364546333,108.207740905147));
#35771=CARTESIAN_POINT('Ctrl Pts',(6.51803055986769,-1.82691346963807,108.215863995503));
#35772=CARTESIAN_POINT('Ctrl Pts',(6.56052278018734,-1.65886402415721,108.223987085859));
#35773=CARTESIAN_POINT('Ctrl Pts',(6.60301833719015,-1.49080138266653,108.232110814078));
#35774=CARTESIAN_POINT('Ctrl Pts',(6.63904797902274,-1.32111957290623,108.240234542296));
#35775=CARTESIAN_POINT('Ctrl Pts',(6.66850486910148,-1.15036160000663,108.248358270515));
#35776=CARTESIAN_POINT('Ctrl Pts',(6.69796967640807,-0.979557731909891,
108.256484182175));
#35777=CARTESIAN_POINT('Ctrl Pts',(6.72085815220533,-0.807677485085201,
108.264610093835));
#35778=CARTESIAN_POINT('Ctrl Pts',(6.73711507467389,-0.635271178790456,
108.272736005496));
#35779=CARTESIAN_POINT('Ctrl Pts',(6.75347596185154,-0.461762316245421,
108.280913883206));
#35780=CARTESIAN_POINT('Ctrl Pts',(6.76312014708903,-0.287721016406869,
108.289091760916));
#35781=CARTESIAN_POINT('Ctrl Pts',(6.76604456939785,-0.11370965184142,108.297269638626));
#35782=CARTESIAN_POINT('Ctrl Pts',(6.76895503407326,0.0594711942219803,
108.305408485099));
#35783=CARTESIAN_POINT('Ctrl Pts',(6.76520980862204,0.232622025700009,108.313547331573));
#35784=CARTESIAN_POINT('Ctrl Pts',(6.75485810033358,0.405192601558612,108.321686178046));
#35785=CARTESIAN_POINT('Ctrl Pts',(6.74443192695163,0.57900456518686,108.329883571374));
#35786=CARTESIAN_POINT('Ctrl Pts',(6.7273039019828,0.752227517647732,108.338080964703));
#35787=CARTESIAN_POINT('Ctrl Pts',(6.70357679070904,0.924309045215469,108.346278358031));
#35788=CARTESIAN_POINT('Ctrl Pts',(6.67984967943529,1.09639057278308,108.354475751359));
#35789=CARTESIAN_POINT('Ctrl Pts',(6.64952360704994,1.26733031962272,108.362673144688));
#35790=CARTESIAN_POINT('Ctrl Pts',(6.61275244723277,1.43659112889404,108.370870538016));
#35791=CARTESIAN_POINT('Ctrl Pts',(6.57584906158015,1.60646058505126,108.379097408445));
#35792=CARTESIAN_POINT('Ctrl Pts',(6.53234442784925,1.77514463446334,108.387324278874));
#35793=CARTESIAN_POINT('Ctrl Pts',(6.48232728054897,1.94209217800047,108.395551149303));
#35794=CARTESIAN_POINT('Ctrl Pts',(6.43236715978589,2.10884937800911,108.403768639951));
#35795=CARTESIAN_POINT('Ctrl Pts',(6.37590941385774,2.27387367424087,108.411986130598));
#35796=CARTESIAN_POINT('Ctrl Pts',(6.31309387566238,2.43662363057452,108.420203621245));
#35797=CARTESIAN_POINT('Ctrl Pts',(6.25033734753254,2.5992206966224,108.428413392231));
#35798=CARTESIAN_POINT('Ctrl Pts',(6.1812350510357,2.7595473455245,108.436623163217));
#35799=CARTESIAN_POINT('Ctrl Pts',(6.10597678161969,2.91707671176492,108.444832934204));
#35800=CARTESIAN_POINT('Ctrl Pts',(6.02713985275013,3.08209686885243,108.453433093844));
#35801=CARTESIAN_POINT('Ctrl Pts',(5.94154727860017,3.24404682343997,108.462033253485));
#35802=CARTESIAN_POINT('Ctrl Pts',(5.84947474930506,3.40234245149463,108.470633413126));
#35803=CARTESIAN_POINT('Ctrl Pts',(5.7616953094453,3.55325718870524,108.478832570918));
#35804=CARTESIAN_POINT('Ctrl Pts',(5.66802666498871,3.70085028319838,108.48703172871));
#35805=CARTESIAN_POINT('Ctrl Pts',(5.56875541167771,3.84463940635663,108.495230886502));
#35806=CARTESIAN_POINT('Ctrl Pts',(5.4695108546408,3.98838986138372,108.503427839355));
#35807=CARTESIAN_POINT('Ctrl Pts',(5.36466689280645,4.12833808747981,108.511624792209));
#35808=CARTESIAN_POINT('Ctrl Pts',(5.25455380262281,4.26403017523823,108.519821745063));
#35809=CARTESIAN_POINT('Ctrl Pts',(5.14445031197702,4.39971043350999,108.528017983315));
#35810=CARTESIAN_POINT('Ctrl Pts',(5.02907883426714,4.53113501443973,108.536214221568));
#35811=CARTESIAN_POINT('Ctrl Pts',(4.90881036653292,4.65788254311108,108.54441045982));
#35812=CARTESIAN_POINT('Ctrl Pts',(4.78853052612792,4.78464205711777,108.552607473115));
#35813=CARTESIAN_POINT('Ctrl Pts',(4.66335302104256,4.90672337871442,108.560804486409));
#35814=CARTESIAN_POINT('Ctrl Pts',(4.53368621275221,5.02374146670592,108.569001499703));
#35815=CARTESIAN_POINT('Ctrl Pts',(4.4039367973248,5.14083410368463,108.577203735088));
#35816=CARTESIAN_POINT('Ctrl Pts',(4.2696926326895,5.25285682389974,108.585405970473));
#35817=CARTESIAN_POINT('Ctrl Pts',(4.13139621060566,5.35946399847906,108.593608205858));
#35818=CARTESIAN_POINT('Ctrl Pts',(3.99304832634251,5.46611084319195,108.601813493418));
#35819=CARTESIAN_POINT('Ctrl Pts',(3.85064546936945,5.56733791543589,108.610018780978));
#35820=CARTESIAN_POINT('Ctrl Pts',(3.70465965353445,5.66284255930482,108.618224068539));
#35821=CARTESIAN_POINT('Ctrl Pts',(3.55853625432459,5.75843721089912,108.626437089118));
#35822=CARTESIAN_POINT('Ctrl Pts',(3.40882345864226,5.84829847758847,108.634650109698));
#35823=CARTESIAN_POINT('Ctrl Pts',(3.25601903814054,5.93216899820516,108.642863130277));
#35824=CARTESIAN_POINT('Ctrl Pts',(3.20408814465992,5.96067256543187,108.645654342046));
#35825=CARTESIAN_POINT('Ctrl Pts',(3.15180035632282,5.98848460848285,108.648445553815));
#35826=CARTESIAN_POINT('Ctrl Pts',(3.09917575053272,6.01559628526632,108.651236765584));
#35827=CARTESIAN_POINT('Origin',(0.,0.,-3.69717978381041));
#35828=CARTESIAN_POINT('',(3.09917575053272,6.01559628526632,111.045835064059));
#35829=CARTESIAN_POINT('',(3.09917575053264,6.01559628526636,110.651392015122));
#35830=CARTESIAN_POINT('',(3.09917575053259,6.01559628526639,-3.69717978381041));
#35831=CARTESIAN_POINT('',(-6.76699862514327,-0.0043136190180686,109.697179783784));
#35832=CARTESIAN_POINT('Ctrl Pts',(-6.76699862514293,-0.00431361956973403,
109.69717978381));
#35833=CARTESIAN_POINT('Ctrl Pts',(-6.76685589271447,-0.228225378934505,
109.70772212165));
#35834=CARTESIAN_POINT('Ctrl Pts',(-6.75559591374126,-0.451750734100564,
109.718264459491));
#35835=CARTESIAN_POINT('Ctrl Pts',(-6.73335608618393,-0.673947191291592,
109.728806797331));
#35836=CARTESIAN_POINT('Ctrl Pts',(-6.71079662375845,-0.899337096593478,
109.739500651579));
#35837=CARTESIAN_POINT('Ctrl Pts',(-6.67693942269762,-1.12335988097693,
109.750194505826));
#35838=CARTESIAN_POINT('Ctrl Pts',(-6.63197761234058,-1.3450509095991,109.760888360074));
#35839=CARTESIAN_POINT('Ctrl Pts',(-6.62505575980767,-1.37918015385788,
109.762534674613));
#35840=CARTESIAN_POINT('Ctrl Pts',(-6.61787081791661,-1.41325416636877,
109.764180989153));
#35841=CARTESIAN_POINT('Ctrl Pts',(-6.61042359516057,-1.4472694609313,109.765827303692));
#35842=CARTESIAN_POINT('Ctrl Pts',(-6.57321866317101,-1.61720351047717,
109.774051983211));
#35843=CARTESIAN_POINT('Ctrl Pts',(-6.52940775532851,-1.78592594270599,
109.78227666273));
#35844=CARTESIAN_POINT('Ctrl Pts',(-6.47908372953471,-1.95288581992872,
109.790501342249));
#35845=CARTESIAN_POINT('Ctrl Pts',(-6.42881259998526,-2.11967020343201,
109.798717376699));
#35846=CARTESIAN_POINT('Ctrl Pts',(-6.37204208792575,-2.28469538085837,
109.806933411149));
#35847=CARTESIAN_POINT('Ctrl Pts',(-6.30891606944647,-2.44742048464913,
109.815149445599));
#35848=CARTESIAN_POINT('Ctrl Pts',(-6.24584375930155,-2.61000714007112,
109.823358489754));
#35849=CARTESIAN_POINT('Ctrl Pts',(-6.17642684098778,-2.77029728703645,
109.831567533908));
#35850=CARTESIAN_POINT('Ctrl Pts',(-6.10085903600665,-2.92776502178299,
109.839776578063));
#35851=CARTESIAN_POINT('Ctrl Pts',(-6.02534039288434,-3.08513031334561,
109.847980281691));
#35852=CARTESIAN_POINT('Ctrl Pts',(-5.94367898836081,-3.23967652818743,
109.856183985319));
#35853=CARTESIAN_POINT('Ctrl Pts',(-5.85611673996379,-3.39089748118634,
109.864387688947));
#35854=CARTESIAN_POINT('Ctrl Pts',(-5.76859392625178,-3.54205033005641,
109.872587697941));
#35855=CARTESIAN_POINT('Ctrl Pts',(-5.67517574239427,-3.68988059112708,
109.880787706935));
#35856=CARTESIAN_POINT('Ctrl Pts',(-5.57615019217884,-3.83390636743568,
109.888987715929));
#35857=CARTESIAN_POINT('Ctrl Pts',(-5.47713256025519,-3.97792062713955,
109.897187069233));
#35858=CARTESIAN_POINT('Ctrl Pts',(-5.37250865077825,-4.11813070796377,
109.905386422537));
#35859=CARTESIAN_POINT('Ctrl Pts',(-5.26261017731818,-4.25408311173949,
109.913585775841));
#35860=CARTESIAN_POINT('Ctrl Pts',(-5.15271242036359,-4.39003462914583,
109.921785075687));
#35861=CARTESIAN_POINT('Ctrl Pts',(-5.03754039245939,-4.52172824529911,
109.929984375534));
#35862=CARTESIAN_POINT('Ctrl Pts',(-4.91746645641509,-4.64874312583869,
109.938183675381));
#35863=CARTESIAN_POINT('Ctrl Pts',(-4.79737152062709,-4.77578022002449,
109.946384409204));
#35864=CARTESIAN_POINT('Ctrl Pts',(-4.67237321497657,-4.89813668780901,
109.954585143027));
#35865=CARTESIAN_POINT('Ctrl Pts',(-4.54288118648516,-5.0154281497674,109.96278587685));
#35866=CARTESIAN_POINT('Ctrl Pts',(-4.41334301973963,-5.13276140289502,
109.97098953261));
#35867=CARTESIAN_POINT('Ctrl Pts',(-4.27930820618762,-5.24502581466851,
109.979193188369));
#35868=CARTESIAN_POINT('Ctrl Pts',(-4.14121995070203,-5.35187689693135,
109.987396844129));
#35869=CARTESIAN_POINT('Ctrl Pts',(-4.00297350624245,-5.45885038397808,
109.995609897704));
#35870=CARTESIAN_POINT('Ctrl Pts',(-3.86066462674346,-5.56039793262255,
110.003822951279));
#35871=CARTESIAN_POINT('Ctrl Pts',(-3.71476689498273,-5.65621745656409,
110.012036004854));
#35872=CARTESIAN_POINT('Ctrl Pts',(-3.56878283226078,-5.75209367906774,
110.020253918278));
#35873=CARTESIAN_POINT('Ctrl Pts',(-3.41920599069867,-5.84223493578066,
110.028471831701));
#35874=CARTESIAN_POINT('Ctrl Pts',(-3.26653499439086,-5.92638491244198,
110.036689745124));
#35875=CARTESIAN_POINT('Ctrl Pts',(-3.11362588282745,-6.01066613468161,
110.04492047572));
#35876=CARTESIAN_POINT('Ctrl Pts',(-2.95761329268543,-6.08893724214638,
110.053151206316));
#35877=CARTESIAN_POINT('Ctrl Pts',(-2.79901751809191,-6.16098936319603,
110.061381936912));
#35878=CARTESIAN_POINT('Ctrl Pts',(-2.65336626681946,-6.22716061911135,
110.068940878587));
#35879=CARTESIAN_POINT('Ctrl Pts',(-2.50553671752515,-6.28808713324493,
110.076499820263));
#35880=CARTESIAN_POINT('Ctrl Pts',(-2.3559424962054,-6.34364437485058,110.084058761939));
#35881=CARTESIAN_POINT('Ctrl Pts',(-2.19457398699976,-6.40357442545274,
110.092212654106));
#35882=CARTESIAN_POINT('Ctrl Pts',(-2.03065291637443,-6.45744132991262,
110.100366546273));
#35883=CARTESIAN_POINT('Ctrl Pts',(-1.86467927664805,-6.50501807801019,
110.108520438439));
#35884=CARTESIAN_POINT('Ctrl Pts',(-1.69890817113248,-6.55253676918291,
110.11666438058));
#35885=CARTESIAN_POINT('Ctrl Pts',(-1.53108982981379,-6.59378048312874,
110.12480832272));
#35886=CARTESIAN_POINT('Ctrl Pts',(-1.36174457958176,-6.62857003432714,
110.13295226486));
#35887=CARTESIAN_POINT('Ctrl Pts',(-1.19257033406992,-6.66332445506005,
110.141087983253));
#35888=CARTESIAN_POINT('Ctrl Pts',(-1.02187260468566,-6.69163761489769,
110.149223701646));
#35889=CARTESIAN_POINT('Ctrl Pts',(-0.850187255037952,-6.71337997072794,
110.157359420039));
#35890=CARTESIAN_POINT('Ctrl Pts',(-0.678639159086851,-6.73510494465159,
110.165488634339));
#35891=CARTESIAN_POINT('Ctrl Pts',(-0.506105376010765,-6.7502695281621,
110.173617848639));
#35892=CARTESIAN_POINT('Ctrl Pts',(-0.333132348388015,-6.75879514695167,
110.181747062939));
#35893=CARTESIAN_POINT('Ctrl Pts',(-0.160261234169782,-6.76731574256019,
110.189871487615));
#35894=CARTESIAN_POINT('Ctrl Pts',(0.0130482449213397,-6.76920514526511,
110.19799591229));
#35895=CARTESIAN_POINT('Ctrl Pts',(0.186244134243564,-6.764436570954,110.206120336966));
#35896=CARTESIAN_POINT('Ctrl Pts',(0.360491433488215,-6.75963904834414,
110.2142940821));
#35897=CARTESIAN_POINT('Ctrl Pts',(0.534623386956937,-6.74810240067998,
110.222467827234));
#35898=CARTESIAN_POINT('Ctrl Pts',(0.708076899331325,-6.7298526064568,110.230641572368));
#35899=CARTESIAN_POINT('Ctrl Pts',(0.880419666168669,-6.71171967857554,
110.23876297523));
#35900=CARTESIAN_POINT('Ctrl Pts',(1.0520922897976,-6.68695939252059,110.246884378092));
#35901=CARTESIAN_POINT('Ctrl Pts',(1.22254692741619,-6.65564933047597,110.255005780955));
#35902=CARTESIAN_POINT('Ctrl Pts',(1.3930147436899,-6.6243368477022,110.263127811721));
#35903=CARTESIAN_POINT('Ctrl Pts',(1.5622640264011,-6.58647364632309,110.271249842487));
#35904=CARTESIAN_POINT('Ctrl Pts',(1.72975674083793,-6.5421885189534,110.279371873253));
#35905=CARTESIAN_POINT('Ctrl Pts',(1.89729429941005,-6.49789153477998,110.287496078594));
#35906=CARTESIAN_POINT('Ctrl Pts',(2.06307399957685,-6.44716929451148,110.295620283936));
#35907=CARTESIAN_POINT('Ctrl Pts',(2.22657263568775,-6.39020056790133,110.303744489277));
#35908=CARTESIAN_POINT('Ctrl Pts',(2.39184103140226,-6.33261519424493,110.311956633519));
#35909=CARTESIAN_POINT('Ctrl Pts',(2.55477833010648,-6.26864744187902,110.320168777762));
#35910=CARTESIAN_POINT('Ctrl Pts',(2.71486533474273,-6.19853169825018,110.328380922004));
#35911=CARTESIAN_POINT('Ctrl Pts',(2.8734909214655,-6.12905603408306,110.33651809842));
#35912=CARTESIAN_POINT('Ctrl Pts',(3.02931773612832,-6.05354437649771,110.344655274837));
#35913=CARTESIAN_POINT('Ctrl Pts',(3.18186622310238,-5.97227061830592,110.352792451253));
#35914=CARTESIAN_POINT('Ctrl Pts',(3.33652285444479,-5.88987369711838,110.361042079409));
#35915=CARTESIAN_POINT('Ctrl Pts',(3.48780954592197,-5.80155444818604,110.369291707564));
#35916=CARTESIAN_POINT('Ctrl Pts',(3.63525807612075,-5.70764292155692,110.37754133572));
#35917=CARTESIAN_POINT('Ctrl Pts',(3.78270660631943,-5.61373139492788,110.385790963875));
#35918=CARTESIAN_POINT('Ctrl Pts',(3.92631669499138,-5.51422786174043,110.39404059203));
#35919=CARTESIAN_POINT('Ctrl Pts',(4.06565624941997,-5.40950351340605,110.402290220186));
#35920=CARTESIAN_POINT('Ctrl Pts',(4.20457758936896,-5.30509348528763,110.410515087864));
#35921=CARTESIAN_POINT('Ctrl Pts',(4.3396693489863,-5.1951819825892,110.418739955541));
#35922=CARTESIAN_POINT('Ctrl Pts',(4.47046790784446,-5.08007929907918,110.426964823219));
#35923=CARTESIAN_POINT('Ctrl Pts',(4.60111910748573,-4.96510629162562,110.435180424662));
#35924=CARTESIAN_POINT('Ctrl Pts',(4.72748647073325,-4.84495398395998,110.443396026106));
#35925=CARTESIAN_POINT('Ctrl Pts',(4.84913643400935,-4.71997508937951,110.451611627549));
#35926=CARTESIAN_POINT('Ctrl Pts',(4.97067378690417,-4.59511188674494,110.459819623878));
#35927=CARTESIAN_POINT('Ctrl Pts',(5.08750218785014,-4.465431250643,110.468027620206));
#35928=CARTESIAN_POINT('Ctrl Pts',(5.19922212118798,-4.33132523998714,110.476235616534));
#35929=CARTESIAN_POINT('Ctrl Pts',(5.31086107582188,-4.19731643428483,110.484437663405));
#35930=CARTESIAN_POINT('Ctrl Pts',(5.41739870942876,-4.05888891764186,110.492639710277));
#35931=CARTESIAN_POINT('Ctrl Pts',(5.51847322308392,-3.91647064154779,110.500841757148));
#35932=CARTESIAN_POINT('Ctrl Pts',(5.61949477089273,-3.77412699657741,110.50903950592));
#35933=CARTESIAN_POINT('Ctrl Pts',(5.71505869480656,-3.6277970501811,110.517237254691));
#35934=CARTESIAN_POINT('Ctrl Pts',(5.80484422325914,-3.4779408482168,110.525435003463));
#35935=CARTESIAN_POINT('Ctrl Pts',(5.89461262692539,-3.32811322831338,110.533631188679));
#35936=CARTESIAN_POINT('Ctrl Pts',(5.97860464085945,-3.17476099675327,110.541827373894));
#35937=CARTESIAN_POINT('Ctrl Pts',(6.05654333382081,-3.01837238351246,110.55002355911));
#35938=CARTESIAN_POINT('Ctrl Pts',(6.13447626105363,-2.86199533954819,110.55821913799));
#35939=CARTESIAN_POINT('Ctrl Pts',(6.20635659828984,-2.70258268200196,110.566414716871));
#35940=CARTESIAN_POINT('Ctrl Pts',(6.27195385526933,-2.54064634244362,110.574610295751));
#35941=CARTESIAN_POINT('Ctrl Pts',(6.33755819415582,-2.37869252017109,110.582806759429));
#35942=CARTESIAN_POINT('Ctrl Pts',(6.39687796660829,-2.21421480571479,110.591003223108));
#35943=CARTESIAN_POINT('Ctrl Pts',(6.44973120865177,-2.04774420671707,110.599199686786));
#35944=CARTESIAN_POINT('Ctrl Pts',(6.50259977281488,-1.88122534800373,110.607398526614));
#35945=CARTESIAN_POINT('Ctrl Pts',(6.54899796396364,-1.71271279589424,110.615597366442));
#35946=CARTESIAN_POINT('Ctrl Pts',(6.58879395725007,-1.54275182349752,110.62379620627));
#35947=CARTESIAN_POINT('Ctrl Pts',(6.62863151858366,-1.37261332202989,110.632003610019));
#35948=CARTESIAN_POINT('Ctrl Pts',(6.66185302246366,-1.2010237275144,110.640211013768));
#35949=CARTESIAN_POINT('Ctrl Pts',(6.68837778365413,-1.02853858611231,110.648418417517));
#35950=CARTESIAN_POINT('Ctrl Pts',(6.71491675291036,-0.855961052540755,
110.656630217586));
#35951=CARTESIAN_POINT('Ctrl Pts',(6.73475178771678,-0.682487371953734,
110.664842017655));
#35952=CARTESIAN_POINT('Ctrl Pts',(6.74785421614684,-0.508677184105277,
110.673053817724));
#35953=CARTESIAN_POINT('Ctrl Pts',(6.76097593318235,-0.334611123373883,
110.681277706711));
#35954=CARTESIAN_POINT('Ctrl Pts',(6.76734522321404,-0.160207923962732,
110.689501595697));
#35955=CARTESIAN_POINT('Ctrl Pts',(6.76698557477953,0.0139724989077925,
110.697725484683));
#35956=CARTESIAN_POINT('Ctrl Pts',(6.76665326584358,0.174912198439788,110.705324215933));
#35957=CARTESIAN_POINT('Ctrl Pts',(6.76057675465688,0.335661512626722,110.712922947183));
#35958=CARTESIAN_POINT('Ctrl Pts',(6.74881373515992,0.495784396806563,110.720521678433));
#35959=CARTESIAN_POINT('Ctrl Pts',(6.7360814713138,0.669101019269499,110.728746526755));
#35960=CARTESIAN_POINT('Ctrl Pts',(6.71665061774589,0.842170107914227,110.736971375077));
#35961=CARTESIAN_POINT('Ctrl Pts',(6.69053158575722,1.0144338815246,110.745196223399));
#35962=CARTESIAN_POINT('Ctrl Pts',(6.66444196958966,1.18650364793164,110.753411808718));
#35963=CARTESIAN_POINT('Ctrl Pts',(6.63167922716819,1.35776955381536,110.761627394038));
#35964=CARTESIAN_POINT('Ctrl Pts',(6.59230570527272,1.52767617256695,110.769842979357));
#35965=CARTESIAN_POINT('Ctrl Pts',(6.5529686157684,1.69742557641634,110.77805096278));
#35966=CARTESIAN_POINT('Ctrl Pts',(6.50703300933812,1.86581785066255,110.786258946203));
#35967=CARTESIAN_POINT('Ctrl Pts',(6.45461273974146,2.03230494266172,110.794466929627));
#35968=CARTESIAN_POINT('Ctrl Pts',(6.40223044583732,2.19867142363268,110.802668966803));
#35969=CARTESIAN_POINT('Ctrl Pts',(6.343372953196,2.36313513063809,110.81087100398));
#35970=CARTESIAN_POINT('Ctrl Pts',(6.27820470089683,2.52516033820369,110.819073041156));
#35971=CARTESIAN_POINT('Ctrl Pts',(6.21307057316136,2.68710070323751,110.827270783436));
#35972=CARTESIAN_POINT('Ctrl Pts',(6.14163240252789,2.84660478053349,110.835468525715));
#35973=CARTESIAN_POINT('Ctrl Pts',(6.06410380771575,3.00315401024445,110.843666267994));
#35974=CARTESIAN_POINT('Ctrl Pts',(5.98658995368304,3.15967347470982,110.851862451609));
#35975=CARTESIAN_POINT('Ctrl Pts',(5.90298813552255,3.31323888670916,110.860058635223));
#35976=CARTESIAN_POINT('Ctrl Pts',(5.81355938279019,3.46335333207171,110.868254818837));
#35977=CARTESIAN_POINT('Ctrl Pts',(5.72413721326177,3.61345672691661,110.876450399098));
#35978=CARTESIAN_POINT('Ctrl Pts',(5.62888914629168,3.76010935232465,110.884645979359));
#35979=CARTESIAN_POINT('Ctrl Pts',(5.52812125693116,3.90284055127363,110.89284155962));
#35980=CARTESIAN_POINT('Ctrl Pts',(5.42734245196785,4.04558721146808,110.901038027661));
#35981=CARTESIAN_POINT('Ctrl Pts',(5.32104284035047,4.18441130570462,110.909234495702));
#35982=CARTESIAN_POINT('Ctrl Pts',(5.20957077853204,4.31887268896237,110.917430963742));
#35983=CARTESIAN_POINT('Ctrl Pts',(5.09806636048116,4.45337310140558,110.925629810916));
#35984=CARTESIAN_POINT('Ctrl Pts',(4.98138673064542,4.58350800431764,110.933828658089));
#35985=CARTESIAN_POINT('Ctrl Pts',(4.85991935166817,4.70887172210937,110.942027505262));
#35986=CARTESIAN_POINT('Ctrl Pts',(4.73832502746805,4.83436645717691,110.950234921028));
#35987=CARTESIAN_POINT('Ctrl Pts',(4.61193320749025,4.95507978699414,110.958442336794));
#35988=CARTESIAN_POINT('Ctrl Pts',(4.48116764291128,5.07064350513078,110.96664975256));
#35989=CARTESIAN_POINT('Ctrl Pts',(4.35033199258888,5.18626916135582,110.974861567212));
#35990=CARTESIAN_POINT('Ctrl Pts',(4.21511820211421,5.29673947693754,110.983073381865));
#35991=CARTESIAN_POINT('Ctrl Pts',(4.07598158451339,5.40172779050442,110.991285196517));
#35992=CARTESIAN_POINT('Ctrl Pts',(3.93664006709109,5.50687071532374,110.999509104314));
#35993=CARTESIAN_POINT('Ctrl Pts',(3.79336447204605,5.6065152994204,111.007733012112));
#35994=CARTESIAN_POINT('Ctrl Pts',(3.64663854193452,5.70037861413413,111.01595691991));
#35995=CARTESIAN_POINT('Ctrl Pts',(3.51106649228901,5.78710658343437,111.023555658833));
#35996=CARTESIAN_POINT('Ctrl Pts',(3.37254922635882,5.86889923311976,111.031154397756));
#35997=CARTESIAN_POINT('Ctrl Pts',(3.23148476624057,5.94556937606107,111.03875313668));
#35998=CARTESIAN_POINT('Ctrl Pts',(3.18766134271625,5.96938790656103,111.041113779139));
#35999=CARTESIAN_POINT('Ctrl Pts',(3.14355466612796,5.99273270657428,111.043474421599));
#36000=CARTESIAN_POINT('Ctrl Pts',(3.09917575053272,6.01559628526632,111.045835064059));
#36001=CARTESIAN_POINT('Ctrl Pts',(3.09917575053271,6.01559628526633,109.0454843164));
#36002=CARTESIAN_POINT('Ctrl Pts',(2.94519484763712,6.09492572455532,109.053621569559));
#36003=CARTESIAN_POINT('Ctrl Pts',(2.78828698403167,6.16827687821786,109.061758822718));
#36004=CARTESIAN_POINT('Ctrl Pts',(2.62896692083732,6.23544881537353,109.069896075877));
#36005=CARTESIAN_POINT('Ctrl Pts',(2.46953857203641,6.30266640750706,109.07803885971));
#36006=CARTESIAN_POINT('Ctrl Pts',(2.30769509834838,6.36369628735901,109.086181643543));
#36007=CARTESIAN_POINT('Ctrl Pts',(2.14396668018385,6.41838732660015,109.094324427376));
#36008=CARTESIAN_POINT('Ctrl Pts',(1.98000008270331,6.47315792609397,109.102479056695));
#36009=CARTESIAN_POINT('Ctrl Pts',(1.81414341501669,6.52157117023759,109.110633686014));
#36010=CARTESIAN_POINT('Ctrl Pts',(1.64693819141886,6.56352676490665,109.118788315333));
#36011=CARTESIAN_POINT('Ctrl Pts',(1.57465309658292,6.58166473975154,109.122313672622));
#36012=CARTESIAN_POINT('Ctrl Pts',(1.50211604506174,6.59859646835207,109.12583902991));
#36013=CARTESIAN_POINT('Ctrl Pts',(1.4293710483408,6.61431685105614,109.129364387199));
#36014=CARTESIAN_POINT('Ctrl Pts',(1.25951018591324,6.65102422454118,109.13759615923));
#36015=CARTESIAN_POINT('Ctrl Pts',(1.08798504384715,6.68123804399826,109.145827931261));
#36016=CARTESIAN_POINT('Ctrl Pts',(0.91533308406224,6.70480830040808,109.154059703292));
#36017=CARTESIAN_POINT('Ctrl Pts',(0.742887287971219,6.72835041157627,109.162281645764));
#36018=CARTESIAN_POINT('Ctrl Pts',(0.569317704949634,6.74526470829783,109.170503588236));
#36019=CARTESIAN_POINT('Ctrl Pts',(0.395174483133718,6.75545158578463,109.178725530709));
#36020=CARTESIAN_POINT('Ctrl Pts',(0.221204314601722,6.76562834015216,109.186939302699));
#36021=CARTESIAN_POINT('Ctrl Pts',(0.0466619977576692,6.76909096827847,
109.195153074688));
#36022=CARTESIAN_POINT('Ctrl Pts',(-0.127894557792987,6.7657913049463,109.203366846678));
#36023=CARTESIAN_POINT('Ctrl Pts',(-0.302312610548465,6.76249425974895,
109.211574101409));
#36024=CARTESIAN_POINT('Ctrl Pts',(-0.476744522874798,6.75244561689631,
109.219781356139));
#36025=CARTESIAN_POINT('Ctrl Pts',(-0.650629627096702,6.73564919576013,
109.227988610869));
#36026=CARTESIAN_POINT('Ctrl Pts',(-0.824411578969602,6.71886273861886,
109.236190996881));
#36027=CARTESIAN_POINT('Ctrl Pts',(-0.997647013240173,6.69533651185546,
109.244393382893));
#36028=CARTESIAN_POINT('Ctrl Pts',(-1.16977753718885,6.66512636890617,109.252595768905));
#36029=CARTESIAN_POINT('Ctrl Pts',(-1.34185668435149,6.63492524295175,109.260795706704));
#36030=CARTESIAN_POINT('Ctrl Pts',(-1.51283122497298,6.59804423278493,109.268995644503));
#36031=CARTESIAN_POINT('Ctrl Pts',(-1.68214989877164,6.55459081240489,109.277195582301));
#36032=CARTESIAN_POINT('Ctrl Pts',(-1.85144489744949,6.51114346793458,109.285394373537));
#36033=CARTESIAN_POINT('Ctrl Pts',(-2.01908414317863,6.46112563182285,109.293593164773));
#36034=CARTESIAN_POINT('Ctrl Pts',(-2.18452852858125,6.40469547346434,109.301791956009));
#36035=CARTESIAN_POINT('Ctrl Pts',(-2.34997979305907,6.34826296877476,109.309991088145));
#36036=CARTESIAN_POINT('Ctrl Pts',(-2.51323567611532,6.28541772630625,109.318190220281));
#36037=CARTESIAN_POINT('Ctrl Pts',(-2.67377408946657,6.21636719624068,109.326389352418));
#36038=CARTESIAN_POINT('Ctrl Pts',(-2.83434830030004,6.14730126901831,109.334590312829));
#36039=CARTESIAN_POINT('Ctrl Pts',(-2.99220350535078,6.07202743990208,109.34279127324));
#36040=CARTESIAN_POINT('Ctrl Pts',(-3.14683933625071,5.99080054682387,109.350992233651));
#36041=CARTESIAN_POINT('Ctrl Pts',(-3.30162009814966,5.90949752459311,109.359200880336));
#36042=CARTESIAN_POINT('Ctrl Pts',(-3.45317513972735,5.82223045789055,109.367409527021));
#36043=CARTESIAN_POINT('Ctrl Pts',(-3.60102955021838,5.72929971099907,109.375618173706));
#36044=CARTESIAN_POINT('Ctrl Pts',(-3.74895455055768,5.63632459635893,109.383830739429));
#36045=CARTESIAN_POINT('Ctrl Pts',(-3.89317510145142,5.53768061245887,109.392043305153));
#36046=CARTESIAN_POINT('Ctrl Pts',(-4.03324693963188,5.43371034597448,109.400255870876));
#36047=CARTESIAN_POINT('Ctrl Pts',(-4.17351097658677,5.3295974172815,109.408479705425));
#36048=CARTESIAN_POINT('Ctrl Pts',(-4.30961464440236,5.22014382444315,109.416703539974));
#36049=CARTESIAN_POINT('Ctrl Pts',(-4.44114737597533,5.10573197346546,109.424927374522));
#36050=CARTESIAN_POINT('Ctrl Pts',(-4.56200121382049,5.00060900429826,109.432483531497));
#36051=CARTESIAN_POINT('Ctrl Pts',(-4.67899645747007,4.8913007846865,109.440039688471));
#36052=CARTESIAN_POINT('Ctrl Pts',(-4.79184372094166,4.77812962926624,109.447595845445));
#36053=CARTESIAN_POINT('Ctrl Pts',(-4.92096301084992,4.64863974376593,109.456241563498));
#36054=CARTESIAN_POINT('Ctrl Pts',(-5.04494591497753,4.51379721994059,109.46488728155));
#36055=CARTESIAN_POINT('Ctrl Pts',(-5.16335031922437,4.3740258893799,109.473532999602));
#36056=CARTESIAN_POINT('Ctrl Pts',(-5.28160271634628,4.23443399672308,109.482167618315));
#36057=CARTESIAN_POINT('Ctrl Pts',(-5.39429069811321,4.08992614645227,109.490802237027));
#36058=CARTESIAN_POINT('Ctrl Pts',(-5.50100930137731,3.94096253041822,109.499436855739));
#36059=CARTESIAN_POINT('Ctrl Pts',(-5.61149679114026,3.78673809814296,109.508376415642));
#36060=CARTESIAN_POINT('Ctrl Pts',(-5.71558532953905,3.62773764238932,109.517315975544));
#36061=CARTESIAN_POINT('Ctrl Pts',(-5.81286942987335,3.46451121967355,109.526255535447));
#36062=CARTESIAN_POINT('Ctrl Pts',(-5.90657422807939,3.30729026630176,109.534866188717));
#36063=CARTESIAN_POINT('Ctrl Pts',(-5.9939661405276,3.14614904002357,109.543476841988));
#36064=CARTESIAN_POINT('Ctrl Pts',(-6.07472520682089,2.98161074951357,109.552087495258));
#36065=CARTESIAN_POINT('Ctrl Pts',(-6.15540782925466,2.81722820550418,109.560689997969));
#36066=CARTESIAN_POINT('Ctrl Pts',(-6.2294699891014,2.6494552810904,109.56929250068));
#36067=CARTESIAN_POINT('Ctrl Pts',(-6.29663690795752,2.47884098912116,109.577895003391));
#36068=CARTESIAN_POINT('Ctrl Pts',(-6.36372823179869,2.30841872010268,109.586487824159));
#36069=CARTESIAN_POINT('Ctrl Pts',(-6.42393968504066,2.13516174643677,109.595080644926));
#36070=CARTESIAN_POINT('Ctrl Pts',(-6.47704392625067,1.95964052249879,109.603673465694));
#36071=CARTESIAN_POINT('Ctrl Pts',(-6.48330250229116,1.93895454899262,109.604686168652));
#36072=CARTESIAN_POINT('Ctrl Pts',(-6.48946241587,1.91823714958004,109.60569887161));
#36073=CARTESIAN_POINT('Ctrl Pts',(-6.49552333880982,1.89748927664348,109.606711574569));
#36074=CARTESIAN_POINT('Ctrl Pts',(-6.54330971000693,1.73390601258575,109.614696068013));
#36075=CARTESIAN_POINT('Ctrl Pts',(-6.58490844078597,1.56852987082132,109.622680561458));
#36076=CARTESIAN_POINT('Ctrl Pts',(-6.6201971399517,1.40188402807626,109.630665054903));
#36077=CARTESIAN_POINT('Ctrl Pts',(-6.65549177944812,1.2352101329678,109.638650892419));
#36078=CARTESIAN_POINT('Ctrl Pts',(-6.6844742029827,1.06726648420744,109.646636729935));
#36079=CARTESIAN_POINT('Ctrl Pts',(-6.70707341085314,0.8985851442278,109.654622567451));
#36080=CARTESIAN_POINT('Ctrl Pts',(-6.72969228739623,0.72975699653351,109.662615355247));
#36081=CARTESIAN_POINT('Ctrl Pts',(-6.74591681128877,0.560190252371543,
109.670608143043));
#36082=CARTESIAN_POINT('Ctrl Pts',(-6.75572795343816,0.390421335398477,
109.678600930839));
#36083=CARTESIAN_POINT('Ctrl Pts',(-6.76332979699452,0.258881426190013,
109.684793881821));
#36084=CARTESIAN_POINT('Ctrl Pts',(-6.76708247132931,0.127220256194025,
109.690986832802));
#36085=CARTESIAN_POINT('Ctrl Pts',(-6.76699862514328,-0.00431361901788746,
109.697179783784));
#36086=CARTESIAN_POINT('',(-6.767,6.1014472012115E-12,109.30282021619));
#36087=CARTESIAN_POINT('Ctrl Pts',(3.09917575053272,6.01559628526632,108.651236765584));
#36088=CARTESIAN_POINT('Ctrl Pts',(2.94407565780403,6.09550232009573,108.659463282396));
#36089=CARTESIAN_POINT('Ctrl Pts',(2.78604865213012,6.16932092097397,108.667689799207));
#36090=CARTESIAN_POINT('Ctrl Pts',(2.6256200252445,6.2368588634853,108.675916316018));
#36091=CARTESIAN_POINT('Ctrl Pts',(2.54269120615467,6.27177059915835,108.68016876982));
#36092=CARTESIAN_POINT('Ctrl Pts',(2.4591209175279,6.30500491425731,108.684421223622));
#36093=CARTESIAN_POINT('Ctrl Pts',(2.37498311842477,6.33654039576782,108.688673677424));
#36094=CARTESIAN_POINT('Ctrl Pts',(2.21222192667147,6.39754451767114,108.696899878443));
#36095=CARTESIAN_POINT('Ctrl Pts',(2.04688129247107,6.4523588191325,108.705126079462));
#36096=CARTESIAN_POINT('Ctrl Pts',(1.87947238656043,6.50075938242271,108.713352280481));
#36097=CARTESIAN_POINT('Ctrl Pts',(1.7122515292724,6.54910557788098,108.721569241096));
#36098=CARTESIAN_POINT('Ctrl Pts',(1.54296736792889,6.59105228254896,108.729786201712));
#36099=CARTESIAN_POINT('Ctrl Pts',(1.37215065393314,6.62642374006605,108.738003162328));
#36100=CARTESIAN_POINT('Ctrl Pts',(1.20149153224268,6.66176256453804,108.74621254213));
#36101=CARTESIAN_POINT('Ctrl Pts',(1.02930302272316,6.69053815065911,108.754421921931));
#36102=CARTESIAN_POINT('Ctrl Pts',(0.856130720629171,6.71262461256363,108.762631301733));
#36103=CARTESIAN_POINT('Ctrl Pts',(0.68308343815763,6.7346951294175,108.770834754873));
#36104=CARTESIAN_POINT('Ctrl Pts',(0.509054132095454,6.7500860956666,108.779038208014));
#36105=CARTESIAN_POINT('Ctrl Pts',(0.334598358714759,6.75872272980224,108.787241661154));
#36106=CARTESIAN_POINT('Ctrl Pts',(0.160233536149645,6.76735486131292,108.795440837504));
#36107=CARTESIAN_POINT('Ctrl Pts',(-0.0145569534579787,6.76923965808673,
108.803640013854));
#36108=CARTESIAN_POINT('Ctrl Pts',(-0.189212573766721,6.76435418956818,
108.811839190204));
#36109=CARTESIAN_POINT('Ctrl Pts',(-0.363835329985134,6.75946964032425,
108.820036823756));
#36110=CARTESIAN_POINT('Ctrl Pts',(-0.538322909153748,6.74781736711494,
108.828234457307));
#36111=CARTESIAN_POINT('Ctrl Pts',(-0.712114602225867,6.72942655753792,
108.836432090859));
#36112=CARTESIAN_POINT('Ctrl Pts',(-0.885893778030626,6.71103707255057,
108.844629133979));
#36113=CARTESIAN_POINT('Ctrl Pts',(-1.05897681077719,6.68591005464264,108.8528261771));
#36114=CARTESIAN_POINT('Ctrl Pts',(-1.23080799516007,6.65412659024835,108.86102322022));
#36115=CARTESIAN_POINT('Ctrl Pts',(-1.40265803351161,6.6223396384519,108.869221162752));
#36116=CARTESIAN_POINT('Ctrl Pts',(-1.57325559707273,6.5838948503112,108.877419105283));
#36117=CARTESIAN_POINT('Ctrl Pts',(-1.74205500329311,6.53892448079204,108.885617047814));
#36118=CARTESIAN_POINT('Ctrl Pts',(-1.9109036099483,6.49394100363356,108.893817379822));
#36119=CARTESIAN_POINT('Ctrl Pts',(-2.07795266878711,6.44242824879675,108.902017711831));
#36120=CARTESIAN_POINT('Ctrl Pts',(-2.24267144095204,6.38456841203367,108.910218043839));
#36121=CARTESIAN_POINT('Ctrl Pts',(-2.40756189459754,6.3266482696824,108.91842692281));
#36122=CARTESIAN_POINT('Ctrl Pts',(-2.57011687036094,6.26236794791452,108.926635801781));
#36123=CARTESIAN_POINT('Ctrl Pts',(-2.72982448024864,6.19195827723631,108.934844680752));
#36124=CARTESIAN_POINT('Ctrl Pts',(-2.88961782488563,6.12151080901378,108.943057966439));
#36125=CARTESIAN_POINT('Ctrl Pts',(-3.04656043442922,6.04492758954581,108.951271252126));
#36126=CARTESIAN_POINT('Ctrl Pts',(-3.20016494375342,5.96248549958586,108.959484537814));
#36127=CARTESIAN_POINT('Ctrl Pts',(-3.35399415754354,5.879922807009,108.967709838526));
#36128=CARTESIAN_POINT('Ctrl Pts',(-3.50447520308935,5.79148429746885,108.975935139238));
#36129=CARTESIAN_POINT('Ctrl Pts',(-3.65114854795072,5.69749096364333,108.98416043995));
#36130=CARTESIAN_POINT('Ctrl Pts',(-3.7837968954922,5.61248533140895,108.991599232244));
#36131=CARTESIAN_POINT('Ctrl Pts',(-3.91333115437953,5.52293706231391,108.999038024538));
#36132=CARTESIAN_POINT('Ctrl Pts',(-4.03943535765225,5.4291114366302,109.006476816832));
#36133=CARTESIAN_POINT('Ctrl Pts',(-4.17630503008599,5.32727595200764,109.014550656071));
#36134=CARTESIAN_POINT('Ctrl Pts',(-4.30955446625834,5.22008766297068,109.02262449531));
#36135=CARTESIAN_POINT('Ctrl Pts',(-4.43872698616404,5.10783630731243,109.030698334549));
#36136=CARTESIAN_POINT('Ctrl Pts',(-4.56774945848193,4.99571534351429,109.038762795167));
#36137=CARTESIAN_POINT('Ctrl Pts',(-4.69270416004923,4.87854325839703,109.046827255785));
#36138=CARTESIAN_POINT('Ctrl Pts',(-4.81316335252528,4.75665297682179,109.054891716403));
#36139=CARTESIAN_POINT('Ctrl Pts',(-4.93350898604421,4.63487760331604,109.062948574515));
#36140=CARTESIAN_POINT('Ctrl Pts',(-5.04936728488339,4.50839314912137,109.071005432627));
#36141=CARTESIAN_POINT('Ctrl Pts',(-5.16034367133203,4.37757263717502,109.079062290739));
#36142=CARTESIAN_POINT('Ctrl Pts',(-5.27123969934389,4.24684685287458,109.087113314848));
#36143=CARTESIAN_POINT('Ctrl Pts',(-5.37726061152404,4.11179154395132,109.095164338958));
#36144=CARTESIAN_POINT('Ctrl Pts',(-5.4780488726118,3.97281632463377,109.103215363067));
#36145=CARTESIAN_POINT('Ctrl Pts',(-5.58205542573057,3.82940345716147,109.11152346619));
#36146=CARTESIAN_POINT('Ctrl Pts',(-5.68048931894931,3.68181647099154,109.119831569313));
#36147=CARTESIAN_POINT('Ctrl Pts',(-5.77300244067269,3.53054270898783,109.128139672436));
#36148=CARTESIAN_POINT('Ctrl Pts',(-5.86259408574589,3.38404602892933,109.136185413541));
#36149=CARTESIAN_POINT('Ctrl Pts',(-5.94663302008584,3.23409222921794,109.144231154646));
#36150=CARTESIAN_POINT('Ctrl Pts',(-6.02484723544011,3.08115315906394,109.152276895751));
#36151=CARTESIAN_POINT('Ctrl Pts',(-6.10306004457755,2.92821683860823,109.160322492202));
#36152=CARTESIAN_POINT('Ctrl Pts',(-6.17544817281757,2.77229568653904,109.168368088652));
#36153=CARTESIAN_POINT('Ctrl Pts',(-6.24178595625474,2.61388543672081,109.176413685103));
#36154=CARTESIAN_POINT('Ctrl Pts',(-6.30813566481878,2.45544671048642,109.184460727859));
#36155=CARTESIAN_POINT('Ctrl Pts',(-6.36843271982456,2.29451834012415,109.192507770616));
#36156=CARTESIAN_POINT('Ctrl Pts',(-6.42249997207323,2.13161514085432,109.200554813373));
#36157=CARTESIAN_POINT('Ctrl Pts',(-6.4765876377089,1.96865043659004,109.208604894335));
#36158=CARTESIAN_POINT('Ctrl Pts',(-6.52444070196857,1.80370977322121,109.216654975297));
#36159=CARTESIAN_POINT('Ctrl Pts',(-6.56593218968929,1.63732204541504,109.224705056259));
#36160=CARTESIAN_POINT('Ctrl Pts',(-6.60746819406486,1.47075579846052,109.232763774237));
#36161=CARTESIAN_POINT('Ctrl Pts',(-6.64262890681234,1.3027397496562,109.240822492216));
#36162=CARTESIAN_POINT('Ctrl Pts',(-6.67133855704832,1.13381253178844,109.248881210195));
#36163=CARTESIAN_POINT('Ctrl Pts',(-6.70006664361088,0.96477683480887,109.256945103198));
#36164=CARTESIAN_POINT('Ctrl Pts',(-6.72233536982622,0.794829171801602,
109.265008996202));
#36165=CARTESIAN_POINT('Ctrl Pts',(-6.73812096766818,0.624511669282851,
109.273072889206));
#36166=CARTESIAN_POINT('Ctrl Pts',(-6.75392720729867,0.453971453762943,
109.281147326832));
#36167=CARTESIAN_POINT('Ctrl Pts',(-6.76323338022855,0.283060803695495,
109.289221764458));
#36168=CARTESIAN_POINT('Ctrl Pts',(-6.76606776734014,0.112320825142991,
109.297296202085));
#36169=CARTESIAN_POINT('Ctrl Pts',(-6.76668951966931,0.0748672328258921,
109.299067414062));
#36170=CARTESIAN_POINT('Ctrl Pts',(-6.7670000537757,0.0374218287909141,
109.30083862604));
#36171=CARTESIAN_POINT('Ctrl Pts',(-6.76699999999302,-9.72301229749807E-6,
109.302609838017));
#36172=CARTESIAN_POINT('Ctrl Pts',(-6.767,6.4861066398266E-12,109.30282021619));
#36173=CARTESIAN_POINT('Ctrl Pts',(-6.76700000000018,-0.186007249409342,
109.311569727996));
#36174=CARTESIAN_POINT('Ctrl Pts',(-6.75932637295473,-0.372014355521354,
109.320319239802));
#36175=CARTESIAN_POINT('Ctrl Pts',(-6.74400518266978,-0.557389537149031,
109.329068751608));
#36176=CARTESIAN_POINT('Ctrl Pts',(-6.72868405709709,-0.742763935805681,
109.337818226458));
#36177=CARTESIAN_POINT('Ctrl Pts',(-6.70571545653067,-0.927506129689624,
109.346567701309));
#36178=CARTESIAN_POINT('Ctrl Pts',(-6.67517739415735,-1.11098863924465,
109.35531717616));
#36179=CARTESIAN_POINT('Ctrl Pts',(-6.64463945823167,-1.29447038906158,
109.364066614782));
#36180=CARTESIAN_POINT('Ctrl Pts',(-6.60653217027233,-1.47669218227876,
109.372816053403));
#36181=CARTESIAN_POINT('Ctrl Pts',(-6.56098496116797,-1.65703510503784,
109.381565492025));
#36182=CARTESIAN_POINT('Ctrl Pts',(-6.51543793687604,-1.83737729603715,
109.390314895146));
#36183=CARTESIAN_POINT('Ctrl Pts',(-6.46245112202726,-2.01584035396779,
109.399064298266));
#36184=CARTESIAN_POINT('Ctrl Pts',(-6.40220448416326,-2.19181813637899,
109.407813701386));
#36185=CARTESIAN_POINT('Ctrl Pts',(-6.34195808575274,-2.36779521935712,
109.416563069732));
#36186=CARTESIAN_POINT('Ctrl Pts',(-6.27445201489324,-2.54128677544608,
109.425312438077));
#36187=CARTESIAN_POINT('Ctrl Pts',(-6.19991555136274,-2.71170355237634,
109.434061806422));
#36188=CARTESIAN_POINT('Ctrl Pts',(-6.12537937789128,-2.88211966612882,
109.442811140719));
#36189=CARTESIAN_POINT('Ctrl Pts',(-6.04381298133705,-3.0494607621027,109.451560475016));
#36190=CARTESIAN_POINT('Ctrl Pts',(-5.95549339426392,-3.21315848206696,
109.460309809313));
#36191=CARTESIAN_POINT('Ctrl Pts',(-5.86717414355249,-3.37685557859483,
109.469059110289));
#36192=CARTESIAN_POINT('Ctrl Pts',(-5.77210188986328,-3.53690907467164,
109.477808411264));
#36193=CARTESIAN_POINT('Ctrl Pts',(-5.6705995346716,-3.69277536784764,109.48655771224));
#36194=CARTESIAN_POINT('Ctrl Pts',(-5.56909755761868,-3.84864108035645,
109.495306980621));
#36195=CARTESIAN_POINT('Ctrl Pts',(-5.46116568338183,-4.00031938104125,
109.504056249001));
#36196=CARTESIAN_POINT('Ctrl Pts',(-5.34717048686239,-4.14729511663058,
109.512805517382));
#36197=CARTESIAN_POINT('Ctrl Pts',(-5.23317570555654,-4.29427031687874,
109.521554753895));
#36198=CARTESIAN_POINT('Ctrl Pts',(-5.11311782178954,-4.43654275986957,
109.530303990407));
#36199=CARTESIAN_POINT('Ctrl Pts',(-4.98740459172177,-4.57362924147472,
109.53905322692));
#36200=CARTESIAN_POINT('Ctrl Pts',(-4.86169180911002,-4.71071523514258,
109.547802432291));
#36201=CARTESIAN_POINT('Ctrl Pts',(-4.73032391415613,-4.84261509316346,
109.556551637662));
#36202=CARTESIAN_POINT('Ctrl Pts',(-4.59374707237484,-4.96888084331347,
109.565300843033));
#36203=CARTESIAN_POINT('Ctrl Pts',(-4.45717070537614,-5.09514615452538,
109.57405001799));
#36204=CARTESIAN_POINT('Ctrl Pts',(-4.31538563819742,-5.21577720253439,
109.582799192946));
#36205=CARTESIAN_POINT('Ctrl Pts',(-4.16887341290903,-5.3303642902845,109.591548367902));
#36206=CARTESIAN_POINT('Ctrl Pts',(-4.02236168477599,-5.44495098920984,
109.60029751317));
#36207=CARTESIAN_POINT('Ctrl Pts',(-3.87112305634705,-5.55349359238573,
109.609046658438));
#36208=CARTESIAN_POINT('Ctrl Pts',(-3.71567117317003,-5.65562346102295,
109.617795803706));
#36209=CARTESIAN_POINT('Ctrl Pts',(-3.56021980457579,-5.75775299158597,
109.626544920012));
#36210=CARTESIAN_POINT('Ctrl Pts',(-3.40055544862674,-5.85346967275187,
109.635294036318));
#36211=CARTESIAN_POINT('Ctrl Pts',(-3.23722036323697,-5.94244842803401,
109.644043152624));
#36212=CARTESIAN_POINT('Ctrl Pts',(-3.07388580496369,-6.0314268961631,109.652792240695));
#36213=CARTESIAN_POINT('Ctrl Pts',(-2.90688079258058,-6.11366734484655,
109.661541328766));
#36214=CARTESIAN_POINT('Ctrl Pts',(-2.73677251094995,-6.18889046787134,
109.670290416837));
#36215=CARTESIAN_POINT('Ctrl Pts',(-2.5666647641705,-6.26411335438104,109.679039477399));
#36216=CARTESIAN_POINT('Ctrl Pts',(-2.39345402972522,-6.33231884350128,
109.687788537962));
#36217=CARTESIAN_POINT('Ctrl Pts',(-2.21772856474491,-6.39327529620886,
109.696537598524));
#36218=CARTESIAN_POINT('Ctrl Pts',(-2.04200363768733,-6.45423156231935,
109.705286632304));
#36219=CARTESIAN_POINT('Ctrl Pts',(-1.86376426620566,-6.5079387425192,109.714035666084));
#36220=CARTESIAN_POINT('Ctrl Pts',(-1.68361578195171,-6.55421443795999,
109.722784699864));
#36221=CARTESIAN_POINT('Ctrl Pts',(-1.50346783420376,-6.60048999558563,
109.731533707588));
#36222=CARTESIAN_POINT('Ctrl Pts',(-1.3214110625778,-6.63933404145389,109.740282715312));
#36223=CARTESIAN_POINT('Ctrl Pts',(-1.13806375959602,-6.67061465526935,
109.749031723036));
#36224=CARTESIAN_POINT('Ctrl Pts',(-0.954716987424667,-6.70189517852402,
109.757780705431));
#36225=CARTESIAN_POINT('Ctrl Pts',(-0.770079973815318,-6.72561226535766,
109.766529687826));
#36226=CARTESIAN_POINT('Ctrl Pts',(-0.58477977055782,-6.74168536939736,
109.775278670221));
#36227=CARTESIAN_POINT('Ctrl Pts',(-0.391490647559245,-6.75845143942363,
109.784404850897));
#36228=CARTESIAN_POINT('Ctrl Pts',(-0.197480213109634,-6.76689975924011,
109.793531031573));
#36229=CARTESIAN_POINT('Ctrl Pts',(-0.00346532630305276,-6.76699911271707,
109.802657212249));
#36230=CARTESIAN_POINT('Ctrl Pts',(0.184486595290791,-6.76709536139788,
109.811498199779));
#36231=CARTESIAN_POINT('Ctrl Pts',(0.372442378179965,-6.75935659726799,
109.820339187309));
#36232=CARTESIAN_POINT('Ctrl Pts',(0.559750217716826,-6.7438096572906,109.829180174839));
#36233=CARTESIAN_POINT('Ctrl Pts',(0.745129914452536,-6.72842275717311,
109.837930153437));
#36234=CARTESIAN_POINT('Ctrl Pts',(0.929874656309014,-6.70538772273545,
109.846680132035));
#36235=CARTESIAN_POINT('Ctrl Pts',(1.11335688289266,-6.67478280180828,109.855430110632));
#36236=CARTESIAN_POINT('Ctrl Pts',(1.2968372311835,-6.64417819418122,109.864179999657));
#36237=CARTESIAN_POINT('Ctrl Pts',(1.47905480729734,-6.60600390230188,109.872929888682));
#36238=CARTESIAN_POINT('Ctrl Pts',(1.65939064804312,-6.5603895979726,109.881679777707));
#36239=CARTESIAN_POINT('Ctrl Pts',(1.83972470263769,-6.51477574543396,109.890429580068));
#36240=CARTESIAN_POINT('Ctrl Pts',(2.01817678125352,-6.46172209820255,109.899179382429));
#36241=CARTESIAN_POINT('Ctrl Pts',(2.19414072347184,-6.40140886724184,109.90792918479));
#36242=CARTESIAN_POINT('Ctrl Pts',(2.37010298131603,-6.34109621361559,109.916678903395));
#36243=CARTESIAN_POINT('Ctrl Pts',(2.54357687926423,-6.2735242082617,109.925428622001));
#36244=CARTESIAN_POINT('Ctrl Pts',(2.71397317789485,-6.1989223732571,109.934178340606));
#36245=CARTESIAN_POINT('Ctrl Pts',(2.88436790206728,-6.12432122757187,109.942927978365));
#36246=CARTESIAN_POINT('Ctrl Pts',(3.05168482125797,-6.04269049717649,109.951677616123));
#36247=CARTESIAN_POINT('Ctrl Pts',(3.21535561996943,-5.9543074523517,109.960427253881));
#36248=CARTESIAN_POINT('Ctrl Pts',(3.37902496074832,-5.86592519481775,109.9691768137));
#36249=CARTESIAN_POINT('Ctrl Pts',(3.53904799384424,-5.77079087940508,109.977926373519));
#36250=CARTESIAN_POINT('Ctrl Pts',(3.69488118814532,-5.66922763747319,109.986675933338));
#36251=CARTESIAN_POINT('Ctrl Pts',(3.85071304610394,-5.56766526649356,109.995425418126));
#36252=CARTESIAN_POINT('Ctrl Pts',(4.00235489705542,-5.45967423581026,110.004174902913));
#36253=CARTESIAN_POINT('Ctrl Pts',(4.14929168607241,-5.34562133936649,110.012924387701));
#36254=CARTESIAN_POINT('Ctrl Pts',(4.29622726385356,-5.23156938308861,110.021673800364));
#36255=CARTESIAN_POINT('Ctrl Pts',(4.43845763091677,-5.11145583677541,110.030423213027));
#36256=CARTESIAN_POINT('Ctrl Pts',(4.57549970660584,-4.98568866204558,110.039172625691));
#36257=CARTESIAN_POINT('Ctrl Pts',(4.71254069814922,-4.85992248226523,110.047921969137));
#36258=CARTESIAN_POINT('Ctrl Pts',(4.84439326930947,-4.72850295734378,110.056671312583));
#36259=CARTESIAN_POINT('Ctrl Pts',(4.97060959434338,-4.59187644222072,110.06542065603));
#36260=CARTESIAN_POINT('Ctrl Pts',(5.09682496280164,-4.45525096257066,110.074169933166));
#36261=CARTESIAN_POINT('Ctrl Pts',(5.21740397615497,-4.31341878218739,110.082919210302));
#36262=CARTESIAN_POINT('Ctrl Pts',(5.33193710451602,-4.16686161439102,110.091668487438));
#36263=CARTESIAN_POINT('Ctrl Pts',(5.44646940289061,-4.0203055086495,110.100417701171));
#36264=CARTESIAN_POINT('Ctrl Pts',(5.55495572749354,-3.8690247098058,110.109166914904));
#36265=CARTESIAN_POINT('Ctrl Pts',(5.65702762491156,-3.71353301466239,110.117916128637));
#36266=CARTESIAN_POINT('Ctrl Pts',(5.7590988165487,-3.55804239467354,110.126665281873));
#36267=CARTESIAN_POINT('Ctrl Pts',(5.85475551250514,-3.39834117620016,110.135414435109));
#36268=CARTESIAN_POINT('Ctrl Pts',(5.94367283727842,-3.23497174692434,110.144163588346));
#36269=CARTESIAN_POINT('Ctrl Pts',(6.03258957676081,-3.0716033930142,110.152912683991));
#36270=CARTESIAN_POINT('Ctrl Pts',(6.11476689685075,-2.90456712829946,110.161661779637));
#36271=CARTESIAN_POINT('Ctrl Pts',(6.18992570525071,-2.73443024476334,110.170410875282));
#36272=CARTESIAN_POINT('Ctrl Pts',(6.26508404388529,-2.56429442463443,110.179159916243));
#36273=CARTESIAN_POINT('Ctrl Pts',(6.33322384283166,-2.3910582865639,110.187908957204));
#36274=CARTESIAN_POINT('Ctrl Pts',(6.39411368719901,-2.21531017132461,110.196657998165));
#36275=CARTESIAN_POINT('Ctrl Pts',(6.45500317120764,-2.03956309619911,110.205406987348));
#36276=CARTESIAN_POINT('Ctrl Pts',(6.50864269269955,-1.86130434439045,110.21415597653));
#36277=CARTESIAN_POINT('Ctrl Pts',(6.55485008446224,-1.68113930720372,110.222904965713));
#36278=CARTESIAN_POINT('Ctrl Pts',(6.60199664749308,-1.49731239212262,110.231831779242));
#36279=CARTESIAN_POINT('Ctrl Pts',(6.64140563640825,-1.31150116500087,110.240758592771));
#36280=CARTESIAN_POINT('Ctrl Pts',(6.67293772282103,-1.1243625515607,110.249685406301));
#36281=CARTESIAN_POINT('Ctrl Pts',(6.70384494949815,-0.940932395055363,
110.258435320456));
#36282=CARTESIAN_POINT('Ctrl Pts',(6.72718449348886,-0.756227260510651,
110.267185234612));
#36283=CARTESIAN_POINT('Ctrl Pts',(6.742877073739,-0.570874564545538,110.275935148767));
#36284=CARTESIAN_POINT('Ctrl Pts',(6.75856934538648,-0.385525513636381,
110.284684890851));
#36285=CARTESIAN_POINT('Ctrl Pts',(6.76661493004091,-0.199529212422189,
110.293434632935));
#36286=CARTESIAN_POINT('Ctrl Pts',(6.76698649908906,-0.013517438604437,
110.302184375019));
#36287=CARTESIAN_POINT('Ctrl Pts',(6.767358061324,0.172490924441749,110.310933956665));
#36288=CARTESIAN_POINT('Ctrl Pts',(6.76005588896311,0.358514472897364,110.319683538311));
#36289=CARTESIAN_POINT('Ctrl Pts',(6.74510478454617,0.543921359658159,110.328433119957));
#36290=CARTESIAN_POINT('Ctrl Pts',(6.73015393440731,0.729325093146488,110.337182552796));
#36291=CARTESIAN_POINT('Ctrl Pts',(6.7075544355695,0.914111900252494,110.345931985635));
#36292=CARTESIAN_POINT('Ctrl Pts',(6.6773830468238,1.09765415591163,110.354681418474));
#36293=CARTESIAN_POINT('Ctrl Pts',(6.64721213111933,1.28119353390898,110.363430714135));
#36294=CARTESIAN_POINT('Ctrl Pts',(6.60946960955577,1.46348811672278,110.372180009797));
#36295=CARTESIAN_POINT('Ctrl Pts',(6.56428366991276,1.64391876347848,110.380929305458));
#36296=CARTESIAN_POINT('Ctrl Pts',(6.51909837867821,1.82434682109345,110.389678475569));
#36297=CARTESIAN_POINT('Ctrl Pts',(6.46646995272035,2.00291071820077,110.39842764568));
#36298=CARTESIAN_POINT('Ctrl Pts',(6.40657713281673,2.1790040021234,110.40717681579));
#36299=CARTESIAN_POINT('Ctrl Pts',(6.34668509279197,2.35509499309288,110.415925871976));
#36300=CARTESIAN_POINT('Ctrl Pts',(6.27952894037677,2.52871516397746,110.424674928162));
#36301=CARTESIAN_POINT('Ctrl Pts',(6.20533675061613,2.69927486771038,110.433423984348));
#36302=CARTESIAN_POINT('Ctrl Pts',(6.12832117908086,2.87632521635563,110.44250598563));
#36303=CARTESIAN_POINT('Ctrl Pts',(6.04372366626251,3.05007728919657,110.451587986912));
#36304=CARTESIAN_POINT('Ctrl Pts',(5.95185378008041,3.21989527477876,110.460669988195));
#36305=CARTESIAN_POINT('Ctrl Pts',(5.86334450817554,3.38350129286435,110.469419768502));
#36306=CARTESIAN_POINT('Ctrl Pts',(5.76808562057448,3.54345567124649,110.478169548809));
#36307=CARTESIAN_POINT('Ctrl Pts',(5.66640068804685,3.69921508465001,110.486919329116));
#36308=CARTESIAN_POINT('Ctrl Pts',(5.56471941108135,3.85496889851977,110.495668794869));
#36309=CARTESIAN_POINT('Ctrl Pts',(5.45661270815336,4.00652780919334,110.504418260623));
#36310=CARTESIAN_POINT('Ctrl Pts',(5.34244776449347,4.1533770456893,110.513167726376));
#36311=CARTESIAN_POINT('Ctrl Pts',(5.22828631819835,4.30022178355958,110.521916924096));
#36312=CARTESIAN_POINT('Ctrl Pts',(5.10806717844316,4.44235690972396,110.530666121816));
#36313=CARTESIAN_POINT('Ctrl Pts',(4.98219864544972,4.5792996907037,110.539415319535));
#36314=CARTESIAN_POINT('Ctrl Pts',(4.85633329944276,4.71623900429743,110.548164295725));
#36315=CARTESIAN_POINT('Ctrl Pts',(4.72481904033896,4.84798602483376,110.556913271916));
#36316=CARTESIAN_POINT('Ctrl Pts',(4.58810250737442,4.97409332258901,110.565662248106));
#36317=CARTESIAN_POINT('Ctrl Pts',(4.45137708685884,5.10020881821924,110.574411793042));
#36318=CARTESIAN_POINT('Ctrl Pts',(4.30944892636291,5.22068366307735,110.583161337978));
#36319=CARTESIAN_POINT('Ctrl Pts',(4.16280009466898,5.33510865604666,110.591910882914));
#36320=CARTESIAN_POINT('Ctrl Pts',(4.01615988349045,5.44952692272702,110.600659913523));
#36321=CARTESIAN_POINT('Ctrl Pts',(3.86479978232507,5.55789587288433,110.609408944131));
#36322=CARTESIAN_POINT('Ctrl Pts',(3.70923383581365,5.65984746713683,110.618157974739));
#36323=CARTESIAN_POINT('Ctrl Pts',(3.55366577799854,5.76180044505189,110.626907124087));
#36324=CARTESIAN_POINT('Ctrl Pts',(3.3938920002717,5.85733573570867,110.635656273435));
#36325=CARTESIAN_POINT('Ctrl Pts',(3.23045513626388,5.94612887621739,110.644405422783));
#36326=CARTESIAN_POINT('Ctrl Pts',(3.18695122151813,5.96976399206564,110.646734286896));
#36327=CARTESIAN_POINT('Ctrl Pts',(3.14318791262785,5.9929216543527,110.649063151009));
#36328=CARTESIAN_POINT('Ctrl Pts',(3.09917575053264,6.01559628526636,110.651392015122));
#36329=CARTESIAN_POINT('Origin',(0.,0.,-3.69717978381041));
#36330=CARTESIAN_POINT('',(3.09917575053268,6.01559628526634,113.045920956904));
#36331=CARTESIAN_POINT('',(3.09917575053259,6.01559628526639,112.651392015122));
#36332=CARTESIAN_POINT('',(3.09917575053259,6.01559628526639,-3.69717978381041));
#36333=CARTESIAN_POINT('',(-6.76699984597165,0.00144382119762321,111.697179783846));
#36334=CARTESIAN_POINT('Ctrl Pts',(-6.76699984597165,0.00144382119763222,
111.697179783846));
#36335=CARTESIAN_POINT('Ctrl Pts',(-6.76703761583499,-0.175578555110342,
111.705544669951));
#36336=CARTESIAN_POINT('Ctrl Pts',(-6.76012485488847,-0.352817258443799,
111.713909556056));
#36337=CARTESIAN_POINT('Ctrl Pts',(-6.74623679069683,-0.529696293972878,
111.722274442161));
#36338=CARTESIAN_POINT('Ctrl Pts',(-6.7323648860999,-0.706369520147311,
111.73062959522));
#36339=CARTESIAN_POINT('Ctrl Pts',(-6.71153387447242,-0.882683574078368,
111.738984748279));
#36340=CARTESIAN_POINT('Ctrl Pts',(-6.68377098569768,-1.05806162899233,
111.747339901339));
#36341=CARTESIAN_POINT('Ctrl Pts',(-6.65604385526244,-1.23321379862183,
111.755684293039));
#36342=CARTESIAN_POINT('Ctrl Pts',(-6.62140270326974,-1.40743203735987,
111.76402868474));
#36343=CARTESIAN_POINT('Ctrl Pts',(-6.57992658499906,-1.58014402382271,
111.77237307644));
#36344=CARTESIAN_POINT('Ctrl Pts',(-6.53848165704011,-1.75272612974412,
111.780711193104));
#36345=CARTESIAN_POINT('Ctrl Pts',(-6.49021208107389,-1.92380390897833,
111.789049309767));
#36346=CARTESIAN_POINT('Ctrl Pts',(-6.43524822976081,-2.09281370918684,
111.797387426431));
#36347=CARTESIAN_POINT('Ctrl Pts',(-6.38032466717979,-2.26169962450751,
111.80571943122));
#36348=CARTESIAN_POINT('Ctrl Pts',(-6.31871671730963,-2.42852025879494,
111.814051436009));
#36349=CARTESIAN_POINT('Ctrl Pts',(-6.25060500568759,-2.59272560500977,
111.822383440798));
#36350=CARTESIAN_POINT('Ctrl Pts',(-6.21804693548716,-2.67121738068288,
111.826366221298));
#36351=CARTESIAN_POINT('Ctrl Pts',(-6.1840035340459,-2.74911179372773,111.830349001797));
#36352=CARTESIAN_POINT('Ctrl Pts',(-6.14849852039715,-2.82635011006671,
111.834331782297));
#36353=CARTESIAN_POINT('Ctrl Pts',(-6.0718749796016,-2.99303849220699,111.842927040057));
#36354=CARTESIAN_POINT('Ctrl Pts',(-5.988514174124,-3.15651090180509,111.851522297817));
#36355=CARTESIAN_POINT('Ctrl Pts',(-5.89871943339522,-3.31623250784465,
111.860117555577));
#36356=CARTESIAN_POINT('Ctrl Pts',(-5.8088406036998,-3.47610368639473,111.868720862432));
#36357=CARTESIAN_POINT('Ctrl Pts',(-5.71251596204545,-3.63221678419541,
111.877324169286));
#36358=CARTESIAN_POINT('Ctrl Pts',(-5.61009279203003,-3.78406499214967,
111.88592747614));
#36359=CARTESIAN_POINT('Ctrl Pts',(-5.50342312186914,-3.94220887946116,
111.89488747908));
#36360=CARTESIAN_POINT('Ctrl Pts',(-5.39013867774819,-4.09572638509883,
111.90384748202));
#36361=CARTESIAN_POINT('Ctrl Pts',(-5.27067803046966,-4.24408318711173,
111.91280748496));
#36362=CARTESIAN_POINT('Ctrl Pts',(-5.15565928771743,-4.38692363905136,
111.921434328165));
#36363=CARTESIAN_POINT('Ctrl Pts',(-5.03491558889029,-4.52498005563022,
111.93006117137));
#36364=CARTESIAN_POINT('Ctrl Pts',(-4.90887633273898,-4.65781302221065,
111.938688014575));
#36365=CARTESIAN_POINT('Ctrl Pts',(-4.78271661491865,-4.79077294352998,
111.947323102861));
#36366=CARTESIAN_POINT('Ctrl Pts',(-4.65125145363274,-4.91849923518474,
111.955958191147));
#36367=CARTESIAN_POINT('Ctrl Pts',(-4.51494522387686,-5.0405910988089,111.964593279433));
#36368=CARTESIAN_POINT('Ctrl Pts',(-4.37843655201575,-5.16286429335205,
111.973241192559));
#36369=CARTESIAN_POINT('Ctrl Pts',(-4.23707267610891,-5.27948613977851,
111.981889105684));
#36370=CARTESIAN_POINT('Ctrl Pts',(-4.09135014666724,-5.39009675027879,
111.990537018809));
#36371=CARTESIAN_POINT('Ctrl Pts',(-4.075002297227,-5.40250557692955,111.991507183013));
#36372=CARTESIAN_POINT('Ctrl Pts',(-4.05859962102883,-5.41483879531184,
111.992477347216));
#36373=CARTESIAN_POINT('Ctrl Pts',(-4.04214284049685,-5.42709593217405,
111.99344751142));
#36374=CARTESIAN_POINT('Ctrl Pts',(-3.90262857552527,-5.5310072310252,112.001672190939));
#36375=CARTESIAN_POINT('Ctrl Pts',(-3.75892101225209,-5.62967227570346,
112.009896870458));
#36376=CARTESIAN_POINT('Ctrl Pts',(-3.61145150334582,-5.7227359749495,112.018121549977));
#36377=CARTESIAN_POINT('Ctrl Pts',(-3.46413700157703,-5.81570185371909,
112.026337584427));
#36378=CARTESIAN_POINT('Ctrl Pts',(-3.31306872905993,-5.90307792174032,
112.034553618877));
#36379=CARTESIAN_POINT('Ctrl Pts',(-3.15870995610597,-5.98455014292612,
112.042769653327));
#36380=CARTESIAN_POINT('Ctrl Pts',(-3.00448251335135,-6.06595304661966,
112.050978697482));
#36381=CARTESIAN_POINT('Ctrl Pts',(-2.84697046107697,-6.14146194113349,
112.059187741636));
#36382=CARTESIAN_POINT('Ctrl Pts',(-2.6866648930447,-6.21080677146545,112.067396785791));
#36383=CARTESIAN_POINT('Ctrl Pts',(-2.52646361439533,-6.28010648839524,
112.075600489419));
#36384=CARTESIAN_POINT('Ctrl Pts',(-2.36347276780517,-6.3432499871764,112.083804193047));
#36385=CARTESIAN_POINT('Ctrl Pts',(-2.19820690746325,-6.40001370248384,
112.092007896675));
#36386=CARTESIAN_POINT('Ctrl Pts',(-2.03301547653896,-6.45675185358664,
112.100207905669));
#36387=CARTESIAN_POINT('Ctrl Pts',(-1.86555141138387,-6.5071158292534,112.108407914663));
#36388=CARTESIAN_POINT('Ctrl Pts',(-1.69634813750132,-6.55093062063672,
112.116607923657));
#36389=CARTESIAN_POINT('Ctrl Pts',(-1.52715839346855,-6.59474190849714,
112.124807276961));
#36390=CARTESIAN_POINT('Ctrl Pts',(-1.35623006223046,-6.63200495693902,
112.133006630265));
#36391=CARTESIAN_POINT('Ctrl Pts',(-1.18411095100026,-6.66259485904113,
112.141205983568));
#36392=CARTESIAN_POINT('Ctrl Pts',(-1.01199296193552,-6.69318456170617,
112.149405283415));
#36393=CARTESIAN_POINT('Ctrl Pts',(-0.838684561136643,-6.7171011408871,
112.157604583262));
#36394=CARTESIAN_POINT('Ctrl Pts',(-0.66474283020421,-6.73427100506745,
112.165803883108));
#36395=CARTESIAN_POINT('Ctrl Pts',(-0.490770678583724,-6.75144387208719,
112.174004616931));
#36396=CARTESIAN_POINT('Ctrl Pts',(-0.316165332940904,-6.76186763806699,
112.182205350754));
#36397=CARTESIAN_POINT('Ctrl Pts',(-0.141488122766108,-6.76552068292723,
112.190406084577));
#36398=CARTESIAN_POINT('Ctrl Pts',(0.0332513252284336,-6.76917502937426,
112.198609740337));
#36399=CARTESIAN_POINT('Ctrl Pts',(0.208062330549596,-6.76605384154532,
112.206813396097));
#36400=CARTESIAN_POINT('Ctrl Pts',(0.382384382500243,-6.75618762202619,
112.215017051857));
#36401=CARTESIAN_POINT('Ctrl Pts',(0.556906131567837,-6.74631010011835,
112.223230105432));
#36402=CARTESIAN_POINT('Ctrl Pts',(0.730937449902314,-6.72967212972754,
112.231443159007));
#36403=CARTESIAN_POINT('Ctrl Pts',(0.903922692723735,-6.70635614664022,
112.239656212582));
#36404=CARTESIAN_POINT('Ctrl Pts',(1.07701029479464,-6.68302636696256,112.247874126005));
#36405=CARTESIAN_POINT('Ctrl Pts',(1.24905023488409,-6.65301075922937,112.256092039428));
#36406=CARTESIAN_POINT('Ctrl Pts',(1.41949797321629,-6.61644273790946,112.264309952851));
#36407=CARTESIAN_POINT('Ctrl Pts',(1.5902115525251,-6.57981768281136,112.272540683447));
#36408=CARTESIAN_POINT('Ctrl Pts',(1.75932762023771,-6.53661987976473,112.280771414043));
#36409=CARTESIAN_POINT('Ctrl Pts',(1.92631638239284,-6.48703277276483,112.289002144639));
#36410=CARTESIAN_POINT('Ctrl Pts',(2.07967558896,-6.4414929454895,112.296561086315));
#36411=CARTESIAN_POINT('Ctrl Pts',(2.23124058478261,-6.39056488042854,112.304120027991));
#36412=CARTESIAN_POINT('Ctrl Pts',(2.3806174150803,-6.33442576111019,112.311678969667));
#36413=CARTESIAN_POINT('Ctrl Pts',(2.54175142281211,-6.27386803426412,112.319832861834));
#36414=CARTESIAN_POINT('Ctrl Pts',(2.70083718573265,-6.20705874728179,112.327986754001));
#36415=CARTESIAN_POINT('Ctrl Pts',(2.85734834524032,-6.13415433731109,112.336140646167));
#36416=CARTESIAN_POINT('Ctrl Pts',(3.01366851740659,-6.06133889108892,112.344284588308));
#36417=CARTESIAN_POINT('Ctrl Pts',(3.16742001207413,-5.98244327961086,112.352428530448));
#36418=CARTESIAN_POINT('Ctrl Pts',(3.31809247529859,-5.8976733823913,112.360572472588));
#36419=CARTESIAN_POINT('Ctrl Pts',(3.46861278957044,-5.81298908575728,112.368708190981));
#36420=CARTESIAN_POINT('Ctrl Pts',(3.61605994593148,-5.72244249047124,112.376843909374));
#36421=CARTESIAN_POINT('Ctrl Pts',(3.75994440948221,-5.62628714496545,112.384979627767));
#36422=CARTESIAN_POINT('Ctrl Pts',(3.90371384472922,-5.53020867076331,112.393108842067));
#36423=CARTESIAN_POINT('Ctrl Pts',(4.0439259556214,-5.42853057649233,112.401238056367));
#36424=CARTESIAN_POINT('Ctrl Pts',(4.18011663927345,-5.32155183025302,112.409367270667));
#36425=CARTESIAN_POINT('Ctrl Pts',(4.31622708118886,-5.21463611446596,112.417491695343));
#36426=CARTESIAN_POINT('Ctrl Pts',(4.44832052754707,-5.10242619148798,112.425616120018));
#36427=CARTESIAN_POINT('Ctrl Pts',(4.57596267173852,-4.98526374697023,112.433740544694));
#36428=CARTESIAN_POINT('Ctrl Pts',(4.70437968545728,-4.86739005141094,112.441914289828));
#36429=CARTESIAN_POINT('Ctrl Pts',(4.82829086358383,-4.74450371615169,112.450088034962));
#36430=CARTESIAN_POINT('Ctrl Pts',(4.9472880835852,-4.61699356919802,112.458261780096));
#36431=CARTESIAN_POINT('Ctrl Pts',(5.0655232802109,-4.49029995991316,112.466383182958));
#36432=CARTESIAN_POINT('Ctrl Pts',(5.17890703408709,-4.35904187130088,112.47450458582));
#36433=CARTESIAN_POINT('Ctrl Pts',(5.28707657463593,-4.22363709306754,112.482625988683));
#36434=CARTESIAN_POINT('Ctrl Pts',(5.39525447828405,-4.08822184604976,112.490748019449));
#36435=CARTESIAN_POINT('Ctrl Pts',(5.49821713712489,-3.94865955672577,112.498870050215));
#36436=CARTESIAN_POINT('Ctrl Pts',(5.59564276395386,-3.80540024941016,112.506992080981));
#36437=CARTESIAN_POINT('Ctrl Pts',(5.69309447530815,-3.66210258615933,112.515116286323));
#36438=CARTESIAN_POINT('Ctrl Pts',(5.78500599705682,-3.51510623649389,112.523240491664));
#36439=CARTESIAN_POINT('Ctrl Pts',(5.87109950772212,-3.36488923598164,112.531364697005));
#36440=CARTESIAN_POINT('Ctrl Pts',(5.95812492106859,-3.21304624038041,112.539576841247));
#36441=CARTESIAN_POINT('Ctrl Pts',(6.03920544410244,-3.05791279641549,112.54778898549));
#36442=CARTESIAN_POINT('Ctrl Pts',(6.11410274967759,-2.90000630454228,112.556001129732));
#36443=CARTESIAN_POINT('Ctrl Pts',(6.18831632540041,-2.74354132490426,112.564138306149));
#36444=CARTESIAN_POINT('Ctrl Pts',(6.25645901989143,-2.58435407734079,112.572275482565));
#36445=CARTESIAN_POINT('Ctrl Pts',(6.31834833973038,-2.42296579790684,112.580412658982));
#36446=CARTESIAN_POINT('Ctrl Pts',(6.38109293924895,-2.25934721256086,112.588662287137));
#36447=CARTESIAN_POINT('Ctrl Pts',(6.4374099351969,-2.09346668712922,112.596911915292));
#36448=CARTESIAN_POINT('Ctrl Pts',(6.48716221335219,-1.92588042662453,112.605161543448));
#36449=CARTESIAN_POINT('Ctrl Pts',(6.53691449150748,-1.75829416611984,112.613411171603));
#36450=CARTESIAN_POINT('Ctrl Pts',(6.58010201805447,-1.58900255901556,112.621660799759));
#36451=CARTESIAN_POINT('Ctrl Pts',(6.61664193296375,-1.41856918440578,112.629910427914));
#36452=CARTESIAN_POINT('Ctrl Pts',(6.65307217677808,-1.24864734943308,112.638135295592));
#36453=CARTESIAN_POINT('Ctrl Pts',(6.68300371998199,-1.07708271244946,112.646360163269));
#36454=CARTESIAN_POINT('Ctrl Pts',(6.70628996835202,-0.904413545000902,
112.654585030947));
#36455=CARTESIAN_POINT('Ctrl Pts',(6.72954998215683,-0.731938908696387,
112.66280063239));
#36456=CARTESIAN_POINT('Ctrl Pts',(6.74617956147946,-0.558362572109245,
112.671016233834));
#36457=CARTESIAN_POINT('Ctrl Pts',(6.75608261991125,-0.384235127146414,
112.679231835277));
#36458=CARTESIAN_POINT('Ctrl Pts',(6.76597651116243,-0.210268870542459,
112.687439831606));
#36459=CARTESIAN_POINT('Ctrl Pts',(6.76915626185056,-0.0357528774845146,
112.695647827934));
#36460=CARTESIAN_POINT('Ctrl Pts',(6.76557729125571,0.138754877553961,112.703855824262));
#36461=CARTESIAN_POINT('Ctrl Pts',(6.76200091482999,0.313136142972685,112.712057871133));
#36462=CARTESIAN_POINT('Ctrl Pts',(6.75167558226842,0.487508825024241,112.720259918005));
#36463=CARTESIAN_POINT('Ctrl Pts',(6.73460872451394,0.661312579421232,112.728461964876));
#36464=CARTESIAN_POINT('Ctrl Pts',(6.71755081026585,0.83502525583471,112.736659713648));
#36465=CARTESIAN_POINT('Ctrl Pts',(6.69375844359767,1.00816924231583,112.744857462419));
#36466=CARTESIAN_POINT('Ctrl Pts',(6.66329107632034,1.18018686326773,112.753055211191));
#36467=CARTESIAN_POINT('Ctrl Pts',(6.63282952008147,1.35217167531291,112.761251396407));
#36468=CARTESIAN_POINT('Ctrl Pts',(6.59569555551616,1.52303019574673,112.769447581622));
#36469=CARTESIAN_POINT('Ctrl Pts',(6.55200021529622,1.69221221445727,112.777643766838));
#36470=CARTESIAN_POINT('Ctrl Pts',(6.50830810755886,1.86138171746414,112.785839345718));
#36471=CARTESIAN_POINT('Ctrl Pts',(6.45805567970994,2.0288746180972,112.794034924599));
#36472=CARTESIAN_POINT('Ctrl Pts',(6.40140456973998,2.19415326139997,112.802230503479));
#36473=CARTESIAN_POINT('Ctrl Pts',(6.34474734369284,2.3594497482532,112.810426967157));
#36474=CARTESIAN_POINT('Ctrl Pts',(6.28169017560345,2.52253116199824,112.818623430836));
#36475=CARTESIAN_POINT('Ctrl Pts',(6.212443850371,2.68287726256488,112.826819894514));
#36476=CARTESIAN_POINT('Ctrl Pts',(6.14317745067534,2.84326984735842,112.835018734342));
#36477=CARTESIAN_POINT('Ctrl Pts',(6.06771846218382,3.00092521014654,112.84321757417));
#36478=CARTESIAN_POINT('Ctrl Pts',(5.98632488021125,3.15534521543425,112.851416413998));
#36479=CARTESIAN_POINT('Ctrl Pts',(5.90484628032631,3.30992651681139,112.859623817747));
#36480=CARTESIAN_POINT('Ctrl Pts',(5.81742087000417,3.46126539118293,112.867831221496));
#36481=CARTESIAN_POINT('Ctrl Pts',(5.72435199260824,3.60888947804198,112.876038625245));
#36482=CARTESIAN_POINT('Ctrl Pts',(5.63123326259646,3.75659264017408,112.884250425314));
#36483=CARTESIAN_POINT('Ctrl Pts',(5.53246524198986,3.90057675237968,112.892462225383));
#36484=CARTESIAN_POINT('Ctrl Pts',(5.42839323009073,4.0404004677142,112.900674025452));
#36485=CARTESIAN_POINT('Ctrl Pts',(5.3241680096483,4.180430023095,112.908897914438));
#36486=CARTESIAN_POINT('Ctrl Pts',(5.21462341864902,4.31628666225212,112.917121803425));
#36487=CARTESIAN_POINT('Ctrl Pts',(5.10014431995143,4.44756303110672,112.925345692411));
#36488=CARTESIAN_POINT('Ctrl Pts',(4.99436761184972,4.56886012644521,112.932944423661));
#36489=CARTESIAN_POINT('Ctrl Pts',(4.88437866718782,4.68624708505496,112.940543154911));
#36490=CARTESIAN_POINT('Ctrl Pts',(4.7705069549644,4.79943250735296,112.948141886161));
#36491=CARTESIAN_POINT('Ctrl Pts',(4.64726925939531,4.92192746543924,112.956365615393));
#36492=CARTESIAN_POINT('Ctrl Pts',(4.51913753642527,5.03984460659206,112.964589344625));
#36493=CARTESIAN_POINT('Ctrl Pts',(4.38648522069382,5.15276978028659,112.972813073857));
#36494=CARTESIAN_POINT('Ctrl Pts',(4.25396400993284,5.26558334604212,112.981028675286));
#36495=CARTESIAN_POINT('Ctrl Pts',(4.11693136867661,5.37341453291452,112.989244276716));
#36496=CARTESIAN_POINT('Ctrl Pts',(3.97579855336091,5.47588484750121,112.997459878146));
#36497=CARTESIAN_POINT('Ctrl Pts',(3.83481094650602,5.57824973262681,113.005667026723));
#36498=CARTESIAN_POINT('Ctrl Pts',(3.68973185875539,5.67526452497526,113.013874175301));
#36499=CARTESIAN_POINT('Ctrl Pts',(3.54100646168675,5.76659017429648,113.022081323878));
#36500=CARTESIAN_POINT('Ctrl Pts',(3.39700359011511,5.85501593082232,113.03002786822));
#36501=CARTESIAN_POINT('Ctrl Pts',(3.24958270126473,5.93810811080855,113.037974412562));
#36502=CARTESIAN_POINT('Ctrl Pts',(3.09917575053269,6.01559628526634,113.045920956904));
#36503=CARTESIAN_POINT('Ctrl Pts',(3.09917575053272,6.01559628526632,111.045835064059));
#36504=CARTESIAN_POINT('Ctrl Pts',(2.94599616846457,6.09451289198494,111.053983127627));
#36505=CARTESIAN_POINT('Ctrl Pts',(2.78957094525295,6.16769307570725,111.062131191196));
#36506=CARTESIAN_POINT('Ctrl Pts',(2.63037268791528,6.23485593439571,111.070279254764));
#36507=CARTESIAN_POINT('Ctrl Pts',(2.47134965376088,6.30194486959974,111.078418350083));
#36508=CARTESIAN_POINT('Ctrl Pts',(2.3095599951337,6.36302952309325,111.086557445403));
#36509=CARTESIAN_POINT('Ctrl Pts',(2.14550169665552,6.41787437315879,111.094696540722));
#36510=CARTESIAN_POINT('Ctrl Pts',(1.98158945302321,6.47267039694612,111.102828390115));
#36511=CARTESIAN_POINT('Ctrl Pts',(1.81541293534023,6.52123756183,111.110960239508));
#36512=CARTESIAN_POINT('Ctrl Pts',(1.64749092867358,6.56338804581432,111.119092088902));
#36513=CARTESIAN_POINT('Ctrl Pts',(1.47968310346446,6.60550986885185,111.127218408904));
#36514=CARTESIAN_POINT('Ctrl Pts',(1.31013250607494,6.6412236103714,111.135344728906));
#36515=CARTESIAN_POINT('Ctrl Pts',(1.13937393368256,6.67039099597953,111.143471048909));
#36516=CARTESIAN_POINT('Ctrl Pts',(0.968695573767828,6.69954468044086,111.151593551637));
#36517=CARTESIAN_POINT('Ctrl Pts',(0.79681072883332,6.7221580720476,111.159716054365));
#36518=CARTESIAN_POINT('Ctrl Pts',(0.624265257620319,6.7381438013839,111.167838557093));
#36519=CARTESIAN_POINT('Ctrl Pts',(0.451735300993305,6.75412809334853,111.175960329479));
#36520=CARTESIAN_POINT('Ctrl Pts',(0.278545199562873,6.76348586692237,111.184082101865));
#36521=CARTESIAN_POINT('Ctrl Pts',(0.105247092715271,6.7661814969357,111.192203874251));
#36522=CARTESIAN_POINT('Ctrl Pts',(-0.068050230422212,6.76887711475852,
111.200325609908));
#36523=CARTESIAN_POINT('Ctrl Pts',(-0.241455192060132,6.76491064225783,
111.208447345564));
#36524=CARTESIAN_POINT('Ctrl Pts',(-0.414414701403533,6.7542985909168,111.216569081221));
#36525=CARTESIAN_POINT('Ctrl Pts',(-0.587406363512533,6.74368456682041,
111.224692326689));
#36526=CARTESIAN_POINT('Ctrl Pts',(-0.759952043109946,6.72642252596304,
111.232815572157));
#36527=CARTESIAN_POINT('Ctrl Pts',(-0.931502866286227,6.70258095140227,
111.240938817626));
#36528=CARTESIAN_POINT('Ctrl Pts',(-1.1031182494974,6.67873040449816,111.24906512013));
#36529=CARTESIAN_POINT('Ctrl Pts',(-1.2737376685576,6.64829544362148,111.257191422634));
#36530=CARTESIAN_POINT('Ctrl Pts',(-1.44282159062039,6.61139583277538,111.265317725138));
#36531=CARTESIAN_POINT('Ctrl Pts',(-1.61210274199256,6.57445318007955,111.273453506633));
#36532=CARTESIAN_POINT('Ctrl Pts',(-1.7798444611894,6.53103089407988,111.281589288128));
#36533=CARTESIAN_POINT('Ctrl Pts',(-1.94552064297387,6.48129913117444,111.289725069624));
#36534=CARTESIAN_POINT('Ctrl Pts',(-2.1113003983228,6.43153627812741,111.297865937257));
#36535=CARTESIAN_POINT('Ctrl Pts',(-2.27501169824269,6.37545620752656,111.30600680489));
#36536=CARTESIAN_POINT('Ctrl Pts',(-2.4361479277498,6.31327745898439,111.314147672523));
#36537=CARTESIAN_POINT('Ctrl Pts',(-2.59753321811656,6.25100260361006,111.322301123121));
#36538=CARTESIAN_POINT('Ctrl Pts',(-2.75633515188049,6.18261038399618,111.330454573719));
#36539=CARTESIAN_POINT('Ctrl Pts',(-2.91207022012727,6.10836606901125,111.338608024316));
#36540=CARTESIAN_POINT('Ctrl Pts',(-3.02907084637388,6.05258780759409,111.344733547853));
#36541=CARTESIAN_POINT('Ctrl Pts',(-3.14434096578099,5.99350746075695,111.35085907139));
#36542=CARTESIAN_POINT('Ctrl Pts',(-3.25768657164231,5.93125342578964,111.356984594926));
#36543=CARTESIAN_POINT('Ctrl Pts',(-3.41000582771465,5.8475934707198,111.365216366957));
#36544=CARTESIAN_POINT('Ctrl Pts',(-3.55932394366084,5.75793941617028,111.373448138988));
#36545=CARTESIAN_POINT('Ctrl Pts',(-3.70513675860652,5.66253040610139,111.381679911019));
#36546=CARTESIAN_POINT('Ctrl Pts',(-3.85077545847961,5.56723532392505,111.389901853491));
#36547=CARTESIAN_POINT('Ctrl Pts',(-3.99291689512999,5.46619916420568,111.398123795963));
#36548=CARTESIAN_POINT('Ctrl Pts',(-4.1310803784713,5.35970744599082,111.406345738436));
#36549=CARTESIAN_POINT('Ctrl Pts',(-4.26910656307485,5.25332155297767,111.414559510426));
#36550=CARTESIAN_POINT('Ctrl Pts',(-4.40316238502532,5.14149111542185,111.422773282416));
#36551=CARTESIAN_POINT('Ctrl Pts',(-4.53279502223442,5.02454558009049,111.430987054406));
#36552=CARTESIAN_POINT('Ctrl Pts',(-4.66232480176227,4.90769283579428,111.439194309136));
#36553=CARTESIAN_POINT('Ctrl Pts',(-4.78743812205835,4.78573331650393,111.447401563866));
#36554=CARTESIAN_POINT('Ctrl Pts',(-4.90771416413068,4.65903752755771,111.455608818597));
#36555=CARTESIAN_POINT('Ctrl Pts',(-5.02791885589199,4.53241689725316,111.463811204609));
#36556=CARTESIAN_POINT('Ctrl Pts',(-5.14329173993053,4.40106585362844,111.472013590621));
#36557=CARTESIAN_POINT('Ctrl Pts',(-5.25344783289772,4.2653926978676,111.480215976633));
#36558=CARTESIAN_POINT('Ctrl Pts',(-5.36357104694305,4.12976003725293,111.488415914431));
#36559=CARTESIAN_POINT('Ctrl Pts',(-5.46848034298784,3.98980810959565,111.49661585223));
#36560=CARTESIAN_POINT('Ctrl Pts',(-5.56782996976534,3.84597951473782,111.504815790029));
#36561=CARTESIAN_POINT('Ctrl Pts',(-5.66716570490075,3.70217103082984,111.513014581264));
#36562=CARTESIAN_POINT('Ctrl Pts',(-5.76094311472714,3.55448725364313,111.5212133725));
#36563=CARTESIAN_POINT('Ctrl Pts',(-5.84885886406463,3.40340109129862,111.529412163736));
#36564=CARTESIAN_POINT('Ctrl Pts',(-5.93677826888471,3.25230864688473,111.537611295872));
#36565=CARTESIAN_POINT('Ctrl Pts',(-6.01883534731291,3.09781384524642,111.545810428009));
#36566=CARTESIAN_POINT('Ctrl Pts',(-6.09477192685879,2.94041564401599,111.554009560145));
#36567=CARTESIAN_POINT('Ctrl Pts',(-6.17072543903968,2.78298234552009,111.562210520556));
#36568=CARTESIAN_POINT('Ctrl Pts',(-6.24055557839082,2.62264468073213,111.570411480967));
#36569=CARTESIAN_POINT('Ctrl Pts',(-6.30405164315535,2.45992314522838,111.578612441378));
#36570=CARTESIAN_POINT('Ctrl Pts',(-6.36760721901788,2.29704910047418,111.586821088063));
#36571=CARTESIAN_POINT('Ctrl Pts',(-6.42481672895831,2.13178705543421,111.595029734748));
#36572=CARTESIAN_POINT('Ctrl Pts',(-6.47551854354318,1.96467518746191,111.603238381433));
#36573=CARTESIAN_POINT('Ctrl Pts',(-6.52624456459836,1.79748353559025,111.611450947157));
#36574=CARTESIAN_POINT('Ctrl Pts',(-6.5704566049084,1.62844064650194,111.61966351288));
#36575=CARTESIAN_POINT('Ctrl Pts',(-6.60804385955467,1.45809648178776,111.627876078604));
#36576=CARTESIAN_POINT('Ctrl Pts',(-6.64568268933818,1.28751858029882,111.636099913152));
#36577=CARTESIAN_POINT('Ctrl Pts',(-6.67667850267813,1.11563618756065,111.644323747701));
#36578=CARTESIAN_POINT('Ctrl Pts',(-6.70097204536584,0.943007236040943,
111.65254758225));
#36579=CARTESIAN_POINT('Ctrl Pts',(-6.72329324126598,0.784393702624233,
111.660103739224));
#36580=CARTESIAN_POINT('Ctrl Pts',(-6.73995685897951,0.625150185465986,
111.667659896199));
#36581=CARTESIAN_POINT('Ctrl Pts',(-6.75095573916353,0.465709789305583,
111.675216053173));
#36582=CARTESIAN_POINT('Ctrl Pts',(-6.76161267506723,0.311226236987937,
111.682537296719));
#36583=CARTESIAN_POINT('Ctrl Pts',(-6.76696678843674,0.156380053440347,
111.689858540264));
#36584=CARTESIAN_POINT('Ctrl Pts',(-6.76699984597149,0.00144382195464194,
111.69717978381));
#36585=CARTESIAN_POINT('',(-6.767,-6.60172908859006E-10,111.302820216221));
#36586=CARTESIAN_POINT('Ctrl Pts',(3.09917575053264,6.01559628526636,110.651392015122));
#36587=CARTESIAN_POINT('Ctrl Pts',(2.93382384459273,6.10078395293755,110.660141463035));
#36588=CARTESIAN_POINT('Ctrl Pts',(2.76495772122995,6.17915010267044,110.668890910947));
#36589=CARTESIAN_POINT('Ctrl Pts',(2.59315093316725,6.25042856433172,110.67764035886));
#36590=CARTESIAN_POINT('Ctrl Pts',(2.42134553245632,6.32170645041445,110.68638973612));
#36591=CARTESIAN_POINT('Ctrl Pts',(2.24659977927607,6.38589665313452,110.69513911338));
#36592=CARTESIAN_POINT('Ctrl Pts',(2.06950718689937,6.44278115439069,110.70388849064));
#36593=CARTESIAN_POINT('Ctrl Pts',(1.89241596572869,6.49966521519722,110.712637800154));
#36594=CARTESIAN_POINT('Ctrl Pts',(1.71297821457194,6.54924360009547,110.721387109669));
#36595=CARTESIAN_POINT('Ctrl Pts',(1.5318033733583,6.5913479217356,110.730136419184));
#36596=CARTESIAN_POINT('Ctrl Pts',(1.35062987477763,6.63345193135309,110.73888566386));
#36597=CARTESIAN_POINT('Ctrl Pts',(1.16771959102928,6.66808192368242,110.747634908536));
#36598=CARTESIAN_POINT('Ctrl Pts',(0.983693746906564,6.69512028363172,110.756384153212));
#36599=CARTESIAN_POINT('Ctrl Pts',(0.799669205419412,6.72215845218873,110.765133335956));
#36600=CARTESIAN_POINT('Ctrl Pts',(0.614529402872837,6.74160505424585,110.7738825187));
#36601=CARTESIAN_POINT('Ctrl Pts',(0.428903127362429,6.75339404354127,110.782631701445));
#36602=CARTESIAN_POINT('Ctrl Pts',(0.243278104162903,6.76518295330334,110.791380825163));
#36603=CARTESIAN_POINT('Ctrl Pts',(0.0571669005379851,6.76931433552277,
110.800129948882));
#36604=CARTESIAN_POINT('Ctrl Pts',(-0.1287984047788,6.7657741590247,110.8088790726));
#36605=CARTESIAN_POINT('Ctrl Pts',(-0.314762517260398,6.76223400523435,
110.8176281402));
#36606=CARTESIAN_POINT('Ctrl Pts',(-0.50058044682082,6.75102239665079,110.826377207799));
#36607=CARTESIAN_POINT('Ctrl Pts',(-0.685621118843931,6.73217741012484,
110.835126275398));
#36608=CARTESIAN_POINT('Ctrl Pts',(-0.870660665416062,6.71333253821752,
110.843875289784));
#36609=CARTESIAN_POINT('Ctrl Pts',(-1.05492267885669,6.68685441030584,110.85262430417));
#36610=CARTESIAN_POINT('Ctrl Pts',(-1.23778137635459,6.65283295028139,110.861373318555));
#36611=CARTESIAN_POINT('Ctrl Pts',(-1.42999922979042,6.61707018861823,110.870570128923));
#36612=CARTESIAN_POINT('Ctrl Pts',(-1.62066601233879,6.57297172934367,110.87976693929));
#36613=CARTESIAN_POINT('Ctrl Pts',(-1.80906628500558,6.52070304311246,110.888963749658));
#36614=CARTESIAN_POINT('Ctrl Pts',(-1.98831342545691,6.4709737491498,110.897713747395));
#36615=CARTESIAN_POINT('Ctrl Pts',(-2.16550875896856,6.41384933989476,110.906463745133));
#36616=CARTESIAN_POINT('Ctrl Pts',(-2.34005036714157,6.34952386240422,110.915213742871));
#36617=CARTESIAN_POINT('Ctrl Pts',(-2.51458843547236,6.28519968948537,110.923963563152));
#36618=CARTESIAN_POINT('Ctrl Pts',(-2.68647261718205,6.21367483971035,110.932713383433));
#36619=CARTESIAN_POINT('Ctrl Pts',(-2.85511905908882,6.13519226743774,110.941463203713));
#36620=CARTESIAN_POINT('Ctrl Pts',(-3.02376230489042,6.05671118252858,110.950212858172));
#36621=CARTESIAN_POINT('Ctrl Pts',(-3.18916767380069,5.97127275992545,110.958962512631));
#36622=CARTESIAN_POINT('Ctrl Pts',(-3.35077334102958,5.87916720437899,110.967712167089));
#36623=CARTESIAN_POINT('Ctrl Pts',(-3.51237616037538,5.7870632719554,110.976461667358));
#36624=CARTESIAN_POINT('Ctrl Pts',(-3.67017916302467,5.6882925836219,110.985211167626));
#36625=CARTESIAN_POINT('Ctrl Pts',(-3.82364636566628,5.58319061740929,110.993960667894));
#36626=CARTESIAN_POINT('Ctrl Pts',(-3.97711106778959,5.47809036367585,111.002710025603));
#36627=CARTESIAN_POINT('Ctrl Pts',(-4.12623987482084,5.36665920043104,111.011459383311));
#36628=CARTESIAN_POINT('Ctrl Pts',(-4.27052628214082,5.2492755951221,111.02020874102));
#36629=CARTESIAN_POINT('Ctrl Pts',(-4.41481053025127,5.13189374642908,111.028957967796));
#36630=CARTESIAN_POINT('Ctrl Pts',(-4.55425230136675,5.00855981477221,111.037707194573));
#36631=CARTESIAN_POINT('Ctrl Pts',(-4.68837800630689,4.87969268191941,111.046456421349));
#36632=CARTESIAN_POINT('Ctrl Pts',(-4.82250188229041,4.75082730631662,111.05520552882));
#36633=CARTESIAN_POINT('Ctrl Pts',(-4.95130963053117,4.61642907903365,111.063954636291));
#36634=CARTESIAN_POINT('Ctrl Pts',(-5.07436379033522,4.47695444731515,111.072703743762));
#36635=CARTESIAN_POINT('Ctrl Pts',(-5.19741643562965,4.33748153220396,111.081452743552));
#36636=CARTESIAN_POINT('Ctrl Pts',(-5.31471544462937,4.19293255254382,111.090201743341));
#36637=CARTESIAN_POINT('Ctrl Pts',(-5.42586245275794,4.0437984177938,111.098950743131));
#36638=CARTESIAN_POINT('Ctrl Pts',(-5.53702160019302,3.8946479948413,111.107700698473));
#36639=CARTESIAN_POINT('Ctrl Pts',(-5.64202723081384,3.7409116444365,111.116450653815));
#36640=CARTESIAN_POINT('Ctrl Pts',(-5.74052265233084,3.58311159163046,111.125200609158));
#36641=CARTESIAN_POINT('Ctrl Pts',(-5.83901427067031,3.4253176319159,111.13395022664));
#36642=CARTESIAN_POINT('Ctrl Pts',(-5.93099603115849,3.26346052695414,111.142699844122));
#36643=CARTESIAN_POINT('Ctrl Pts',(-6.01615550622859,3.09809004466872,111.151449461605));
#36644=CARTESIAN_POINT('Ctrl Pts',(-6.10131214578897,2.93272506863624,111.160198787756));
#36645=CARTESIAN_POINT('Ctrl Pts',(-6.17964682328838,2.76384720416692,111.168948113907));
#36646=CARTESIAN_POINT('Ctrl Pts',(-6.25089348288647,2.59203002791393,111.177697440058));
#36647=CARTESIAN_POINT('Ctrl Pts',(-6.32213814889409,2.42021765936823,111.18644652139));
#36648=CARTESIAN_POINT('Ctrl Pts',(-6.3862950841266,2.24546640831706,111.195195602721));
#36649=CARTESIAN_POINT('Ctrl Pts',(-6.44314639819882,2.06836976659823,111.203944684053));
#36650=CARTESIAN_POINT('Ctrl Pts',(-6.50000285283768,1.89125711158043,111.212694556487));
#36651=CARTESIAN_POINT('Ctrl Pts',(-6.54955227673314,1.71179891440008,111.221444428922));
#36652=CARTESIAN_POINT('Ctrl Pts',(-6.59162635926446,1.53060476278169,111.230194301356));
#36653=CARTESIAN_POINT('Ctrl Pts',(-6.63369752055246,1.34942319164451,111.238943566279));
#36654=CARTESIAN_POINT('Ctrl Pts',(-6.66829431424293,1.16650618642478,111.247692831201));
#36655=CARTESIAN_POINT('Ctrl Pts',(-6.69529923745448,0.982474997616478,
111.256442096124));
#36656=CARTESIAN_POINT('Ctrl Pts',(-6.72230554731469,0.798434359175636,
111.265191810303));
#36657=CARTESIAN_POINT('Ctrl Pts',(-6.74171916496723,0.613279706238205,
111.273941524483));
#36658=CARTESIAN_POINT('Ctrl Pts',(-6.75347414817289,0.427639953653224,
111.282691238663));
#36659=CARTESIAN_POINT('Ctrl Pts',(-6.76248837758739,0.285283364198692,
111.289400897838));
#36660=CARTESIAN_POINT('Ctrl Pts',(-6.76699999999987,0.142641701107519,
111.296110557014));
#36661=CARTESIAN_POINT('Ctrl Pts',(-6.767,6.25035709384319E-12,111.30282021619));
#36662=CARTESIAN_POINT('Ctrl Pts',(-6.767,-6.59981407869779E-10,111.302820216221));
#36663=CARTESIAN_POINT('Ctrl Pts',(-6.76699999998186,-0.186007250075648,
111.311569728027));
#36664=CARTESIAN_POINT('Ctrl Pts',(-6.7593263729181,-0.372014356186741,
111.320319239833));
#36665=CARTESIAN_POINT('Ctrl Pts',(-6.74400518261492,-0.557389537812749,
111.329068751639));
#36666=CARTESIAN_POINT('Ctrl Pts',(-6.72868405702401,-0.74276393646773,
111.33781822649));
#36667=CARTESIAN_POINT('Ctrl Pts',(-6.70571545643943,-0.927506130349254,
111.34656770134));
#36668=CARTESIAN_POINT('Ctrl Pts',(-6.67517739404809,-1.11098863990112,
111.355317176191));
#36669=CARTESIAN_POINT('Ctrl Pts',(-6.64463945810433,-1.29447038971527,
111.364066614813));
#36670=CARTESIAN_POINT('Ctrl Pts',(-6.60653217012702,-1.47669218292891,
111.372816053435));
#36671=CARTESIAN_POINT('Ctrl Pts',(-6.56098496100484,-1.65703510568372,
111.381565492057));
#36672=CARTESIAN_POINT('Ctrl Pts',(-6.51543793669517,-1.83737729667852,
111.390314895177));
#36673=CARTESIAN_POINT('Ctrl Pts',(-6.46245112182883,-2.01584035460391,
111.399064298297));
#36674=CARTESIAN_POINT('Ctrl Pts',(-6.40220448394752,-2.19181813700915,
111.407813701418));
#36675=CARTESIAN_POINT('Ctrl Pts',(-6.34195808551965,-2.36779521998144,
111.416563069763));
#36676=CARTESIAN_POINT('Ctrl Pts',(-6.27445201464304,-2.54128677606384,
111.425312438108));
#36677=CARTESIAN_POINT('Ctrl Pts',(-6.19991555109572,-2.71170355298684,
111.434061806453));
#36678=CARTESIAN_POINT('Ctrl Pts',(-6.1253793776076,-2.88211966673172,111.44281114075));
#36679=CARTESIAN_POINT('Ctrl Pts',(-6.04381298103703,-3.04946076269732,
111.451560475048));
#36680=CARTESIAN_POINT('Ctrl Pts',(-5.95549339394793,-3.21315848265263,
111.460309809345));
#36681=CARTESIAN_POINT('Ctrl Pts',(-5.86717414322048,-3.37685557917168,
111.46905911032));
#36682=CARTESIAN_POINT('Ctrl Pts',(-5.77210188951562,-3.536909075239,111.477808411296));
#36683=CARTESIAN_POINT('Ctrl Pts',(-5.67059953430871,-3.69277536840489,
111.486557712271));
#36684=CARTESIAN_POINT('Ctrl Pts',(-5.56909755724049,-3.8486410809037,111.495306980652));
#36685=CARTESIAN_POINT('Ctrl Pts',(-5.46116568298875,-4.00031938157787,
111.504056249033));
#36686=CARTESIAN_POINT('Ctrl Pts',(-5.34717048645489,-4.14729511715597,
111.512805517413));
#36687=CARTESIAN_POINT('Ctrl Pts',(-5.23317570513439,-4.2942703173932,111.521554753926));
#36688=CARTESIAN_POINT('Ctrl Pts',(-5.11311782135318,-4.4365427603725,111.530303990439));
#36689=CARTESIAN_POINT('Ctrl Pts',(-4.98740459127167,-4.57362924196554,
111.539053226951));
#36690=CARTESIAN_POINT('Ctrl Pts',(-4.8616918086462,-4.71071523562129,111.547802432323));
#36691=CARTESIAN_POINT('Ctrl Pts',(-4.73032391367906,-4.84261509362948,
111.556551637694));
#36692=CARTESIAN_POINT('Ctrl Pts',(-4.59374707188508,-4.96888084376626,
111.565300843065));
#36693=CARTESIAN_POINT('Ctrl Pts',(-4.45717070487386,-5.09514615496477,
111.574050018021));
#36694=CARTESIAN_POINT('Ctrl Pts',(-4.31538563768318,-5.21577720295986,
111.582799192977));
#36695=CARTESIAN_POINT('Ctrl Pts',(-4.16887341238342,-5.33036429069558,
111.591548367933));
#36696=CARTESIAN_POINT('Ctrl Pts',(-4.022361684239,-5.44495098960653,111.600297513201));
#36697=CARTESIAN_POINT('Ctrl Pts',(-3.87112305579928,-5.55349359276757,
111.609046658469));
#36698=CARTESIAN_POINT('Ctrl Pts',(-3.71567117261211,-5.6556234613895,111.617795803737));
#36699=CARTESIAN_POINT('Ctrl Pts',(-3.56021980400825,-5.75775299193688,
111.626544920043));
#36700=CARTESIAN_POINT('Ctrl Pts',(-3.40055544805023,-5.85346967308677,
111.635294036349));
#36701=CARTESIAN_POINT('Ctrl Pts',(-3.23722036265219,-5.94244842835258,
111.644043152656));
#36702=CARTESIAN_POINT('Ctrl Pts',(-3.07388580437007,-6.03142689646564,
111.652792240727));
#36703=CARTESIAN_POINT('Ctrl Pts',(-2.90688079197878,-6.11366734513269,
111.661541328797));
#36704=CARTESIAN_POINT('Ctrl Pts',(-2.73677251034066,-6.18889046814077,
111.670290416868));
#36705=CARTESIAN_POINT('Ctrl Pts',(-2.56666476355359,-6.26411335463382,
111.679039477431));
#36706=CARTESIAN_POINT('Ctrl Pts',(-2.39345402910139,-6.33231884373708,
111.687788537993));
#36707=CARTESIAN_POINT('Ctrl Pts',(-2.21772856411486,-6.39327529642741,
111.696537598555));
#36708=CARTESIAN_POINT('Ctrl Pts',(-2.04200363705142,-6.45423156252053,
111.705286632335));
#36709=CARTESIAN_POINT('Ctrl Pts',(-1.86376426556463,-6.50793874270278,
111.714035666115));
#36710=CARTESIAN_POINT('Ctrl Pts',(-1.68361578130627,-6.55421443812578,
111.722784699895));
#36711=CARTESIAN_POINT('Ctrl Pts',(-1.5034678335538,-6.60048999573368,111.731533707619));
#36712=CARTESIAN_POINT('Ctrl Pts',(-1.32141106192404,-6.639334041584,111.740282715344));
#36713=CARTESIAN_POINT('Ctrl Pts',(-1.13806375893922,-6.6706146553814,111.749031723068));
#36714=CARTESIAN_POINT('Ctrl Pts',(-0.954716986764568,-6.70189517861806,
111.757780705463));
#36715=CARTESIAN_POINT('Ctrl Pts',(-0.770079973152659,-6.72561226543354,
111.766529687858));
#36716=CARTESIAN_POINT('Ctrl Pts',(-0.584779769893354,-6.74168536945499,
111.775278670252));
#36717=CARTESIAN_POINT('Ctrl Pts',(-0.39149064690006,-6.75845143946161,
111.784404850928));
#36718=CARTESIAN_POINT('Ctrl Pts',(-0.197480212456598,-6.76689975925897,
111.793531031604));
#36719=CARTESIAN_POINT('Ctrl Pts',(-0.00346532565696627,-6.7669991127174,
111.80265721228));
#36720=CARTESIAN_POINT('Ctrl Pts',(0.184486595930185,-6.76709536138026,
111.811498199809));
#36721=CARTESIAN_POINT('Ctrl Pts',(0.372442378811916,-6.75935659723298,
111.820339187339));
#36722=CARTESIAN_POINT('Ctrl Pts',(0.55975021834066,-6.74380965723882,111.829180174868));
#36723=CARTESIAN_POINT('Ctrl Pts',(0.745129915074913,-6.72842275710419,
111.837930153466));
#36724=CARTESIAN_POINT('Ctrl Pts',(0.929874656929226,-6.70538772264944,
111.846680132064));
#36725=CARTESIAN_POINT('Ctrl Pts',(1.11335688351,-6.6747828017053,111.855430110662));
#36726=CARTESIAN_POINT('Ctrl Pts',(1.29683723179798,-6.64417819406129,111.864179999687));
#36727=CARTESIAN_POINT('Ctrl Pts',(1.47905480790826,-6.60600390216509,111.872929888712));
#36728=CARTESIAN_POINT('Ctrl Pts',(1.65939064864979,-6.56038959781914,111.881679777737));
#36729=CARTESIAN_POINT('Ctrl Pts',(1.83972470324011,-6.51477574526384,111.890429580098));
#36730=CARTESIAN_POINT('Ctrl Pts',(2.018176781851,-6.46172209801594,111.899179382458));
#36731=CARTESIAN_POINT('Ctrl Pts',(2.19414072406371,-6.40140886703897,111.907929184819));
#36732=CARTESIAN_POINT('Ctrl Pts',(2.3701029819023,-6.34109621339646,111.916678903425));
#36733=CARTESIAN_POINT('Ctrl Pts',(2.54357687984421,-6.27352420802654,111.92542862203));
#36734=CARTESIAN_POINT('Ctrl Pts',(2.71397317846791,-6.1989223730062,111.934178340636));
#36735=CARTESIAN_POINT('Ctrl Pts',(2.88436790263341,-6.12432122730523,111.942927978394));
#36736=CARTESIAN_POINT('Ctrl Pts',(3.05168482181653,-6.04269049689441,111.951677616152));
#36737=CARTESIAN_POINT('Ctrl Pts',(3.21535562051979,-5.95430745205451,111.960427253911));
#36738=CARTESIAN_POINT('Ctrl Pts',(3.37902496129059,-5.86592519450538,111.96917681373));
#36739=CARTESIAN_POINT('Ctrl Pts',(3.5390479943778,-5.77079087907787,111.977926373549));
#36740=CARTESIAN_POINT('Ctrl Pts',(3.69488118866957,-5.66922763713151,111.986675933368));
#36741=CARTESIAN_POINT('Ctrl Pts',(3.85071304661876,-5.56766526613749,111.995425418155));
#36742=CARTESIAN_POINT('Ctrl Pts',(4.00235489756023,-5.4596742354402,112.004174902943));
#36743=CARTESIAN_POINT('Ctrl Pts',(4.14929168656665,-5.34562133898286,112.01292438773));
#36744=CARTESIAN_POINT('Ctrl Pts',(4.29622726433722,-5.23156938269141,112.021673800393));
#36745=CARTESIAN_POINT('Ctrl Pts',(4.43845763138931,-5.11145583636508,112.030423213057));
#36746=CARTESIAN_POINT('Ctrl Pts',(4.57549970706673,-4.98568866162261,112.03917262572));
#36747=CARTESIAN_POINT('Ctrl Pts',(4.71254069859846,-4.85992248182961,112.047921969166));
#36748=CARTESIAN_POINT('Ctrl Pts',(4.84439326974654,-4.728502956896,112.056671312613));
#36749=CARTESIAN_POINT('Ctrl Pts',(4.97060959476779,-4.5918764417613,112.065420656059));
#36750=CARTESIAN_POINT('Ctrl Pts',(5.09682496321357,-4.45525096209941,112.074169933195));
#36751=CARTESIAN_POINT('Ctrl Pts',(5.21740397655394,-4.31341878170482,112.082919210332));
#36752=CARTESIAN_POINT('Ctrl Pts',(5.33193710490156,-4.16686161389768,112.091668487468));
#36753=CARTESIAN_POINT('Ctrl Pts',(5.44646940326257,-4.02030550814558,112.100417701201));
#36754=CARTESIAN_POINT('Ctrl Pts',(5.55495572785148,-3.86902470929188,112.109166914934));
#36755=CARTESIAN_POINT('Ctrl Pts',(5.6570276252551,-3.71353301413905,112.117916128667));
#36756=CARTESIAN_POINT('Ctrl Pts',(5.75909881687784,-3.55804239414078,112.126665281903));
#36757=CARTESIAN_POINT('Ctrl Pts',(5.85475551281949,-3.39834117565858,112.135414435139));
#36758=CARTESIAN_POINT('Ctrl Pts',(5.94367283757764,-3.23497174637457,112.144163588375));
#36759=CARTESIAN_POINT('Ctrl Pts',(6.0325895770449,-3.07160339245624,112.152912684021));
#36760=CARTESIAN_POINT('Ctrl Pts',(6.11476689711938,-2.90456712773393,112.161661779666));
#36761=CARTESIAN_POINT('Ctrl Pts',(6.1899257055036,-2.73443024419088,112.170410875312));
#36762=CARTESIAN_POINT('Ctrl Pts',(6.26508404412242,-2.56429442405506,112.179159916273));
#36763=CARTESIAN_POINT('Ctrl Pts',(6.33322384305276,-2.39105828597825,112.187908957234));
#36764=CARTESIAN_POINT('Ctrl Pts',(6.39411368740385,-2.21531017073336,112.196657998195));
#36765=CARTESIAN_POINT('Ctrl Pts',(6.45500317139635,-2.0395630956019,112.205406987377));
#36766=CARTESIAN_POINT('Ctrl Pts',(6.50864269287186,-1.86130434378794,112.21415597656));
#36767=CARTESIAN_POINT('Ctrl Pts',(6.55485008461795,-1.6811393065966,112.222904965742));
#36768=CARTESIAN_POINT('Ctrl Pts',(6.60199664762854,-1.49731239152371,112.231831779271));
#36769=CARTESIAN_POINT('Ctrl Pts',(6.64140563652433,-1.31150116441116,112.2407585928));
#36770=CARTESIAN_POINT('Ctrl Pts',(6.6729377229187,-1.12436255098105,112.249685406328));
#36771=CARTESIAN_POINT('Ctrl Pts',(6.70384494957986,-0.940932394473189,
112.258435320484));
#36772=CARTESIAN_POINT('Ctrl Pts',(6.72718449355451,-0.75622725992661,112.267185234639));
#36773=CARTESIAN_POINT('Ctrl Pts',(6.74287707378854,-0.570874563960297,
112.275935148795));
#36774=CARTESIAN_POINT('Ctrl Pts',(6.75856934541995,-0.385525513049683,
112.284684890879));
#36775=CARTESIAN_POINT('Ctrl Pts',(6.76661493005824,-0.199529211834698,
112.293434632963));
#36776=CARTESIAN_POINT('Ctrl Pts',(6.76698649909023,-0.0135174380168191,
112.302184375047));
#36777=CARTESIAN_POINT('Ctrl Pts',(6.76735806130902,0.172490925029494,112.310933956693));
#36778=CARTESIAN_POINT('Ctrl Pts',(6.76005588893197,0.358514473484569,112.319683538339));
#36779=CARTESIAN_POINT('Ctrl Pts',(6.74510478449892,0.543921360244159,112.328433119985));
#36780=CARTESIAN_POINT('Ctrl Pts',(6.73015393434395,0.729325093731156,112.337182552824));
#36781=CARTESIAN_POINT('Ctrl Pts',(6.70755443549009,0.914111900835165,112.345931985663));
#36782=CARTESIAN_POINT('Ctrl Pts',(6.67738304672846,1.09765415649164,112.354681418502));
#36783=CARTESIAN_POINT('Ctrl Pts',(6.64721213100804,1.28119353448634,112.363430714163));
#36784=CARTESIAN_POINT('Ctrl Pts',(6.60946960942866,1.46348811729683,112.372180009824));
#36785=CARTESIAN_POINT('Ctrl Pts',(6.56428366976999,1.64391876404857,112.380929305486));
#36786=CARTESIAN_POINT('Ctrl Pts',(6.51909837851975,1.82434682165971,112.389678475596));
#36787=CARTESIAN_POINT('Ctrl Pts',(6.46646995254635,2.00291071876256,112.398427645707));
#36788=CARTESIAN_POINT('Ctrl Pts',(6.4065771326274,2.17900400268007,112.407176815818));
#36789=CARTESIAN_POINT('Ctrl Pts',(6.3466850925873,2.35509499364443,112.415925872004));
#36790=CARTESIAN_POINT('Ctrl Pts',(6.27952894015698,2.52871516452327,112.42467492819));
#36791=CARTESIAN_POINT('Ctrl Pts',(6.20533675038147,2.69927486824982,112.433423984375));
#36792=CARTESIAN_POINT('Ctrl Pts',(6.1283211788406,2.87632521686588,112.442505985657));
#36793=CARTESIAN_POINT('Ctrl Pts',(6.04372366601886,3.05007728967782,112.451587986938));
#36794=CARTESIAN_POINT('Ctrl Pts',(5.95185377983551,3.21989527523145,112.460669988219));
#36795=CARTESIAN_POINT('Ctrl Pts',(5.86334450791821,3.38350129331029,112.469419768526));
#36796=CARTESIAN_POINT('Ctrl Pts',(5.768085620305,3.54345567168515,112.478169548833));
#36797=CARTESIAN_POINT('Ctrl Pts',(5.66640068776555,3.69921508508091,112.48691932914));
#36798=CARTESIAN_POINT('Ctrl Pts',(5.56471941078815,3.85496889894302,112.495668794894));
#36799=CARTESIAN_POINT('Ctrl Pts',(5.45661270784858,4.00652780960844,112.504418260647));
#36800=CARTESIAN_POINT('Ctrl Pts',(5.34244776417745,4.15337704609578,112.513167726401));
#36801=CARTESIAN_POINT('Ctrl Pts',(5.22828631787118,4.30022178395735,112.52191692412));
#36802=CARTESIAN_POINT('Ctrl Pts',(5.1080671781052,4.44235691011256,112.53066612184));
#36803=CARTESIAN_POINT('Ctrl Pts',(4.98219864510137,4.5792996910827,112.539415319559));
#36804=CARTESIAN_POINT('Ctrl Pts',(4.85633329908418,4.71623900466664,112.54816429575));
#36805=CARTESIAN_POINT('Ctrl Pts',(4.72481903997058,4.84798602519277,112.55691327194));
#36806=CARTESIAN_POINT('Ctrl Pts',(4.58810250699667,4.97409332293744,112.56566224813));
#36807=CARTESIAN_POINT('Ctrl Pts',(4.45137708647154,5.10020881855727,112.574411793066));
#36808=CARTESIAN_POINT('Ctrl Pts',(4.30944892596649,5.22068366340458,112.583161338002));
#36809=CARTESIAN_POINT('Ctrl Pts',(4.16280009426389,5.33510865636273,112.591910882939));
#36810=CARTESIAN_POINT('Ctrl Pts',(4.0161598830765,5.4495269230321,112.600659913547));
#36811=CARTESIAN_POINT('Ctrl Pts',(3.86479978190271,5.55789587317804,112.609408944155));
#36812=CARTESIAN_POINT('Ctrl Pts',(3.70923383538335,5.65984746741883,112.618157974763));
#36813=CARTESIAN_POINT('Ctrl Pts',(3.55366577756041,5.76180044532212,112.626907124111));
#36814=CARTESIAN_POINT('Ctrl Pts',(3.39389199982622,5.8573357359668,112.63565627346));
#36815=CARTESIAN_POINT('Ctrl Pts',(3.23045513581156,5.94612887646313,112.644405422808));
#36816=CARTESIAN_POINT('Ctrl Pts',(3.18695122121477,5.96976399222616,112.646734286913));
#36817=CARTESIAN_POINT('Ctrl Pts',(3.14318791247529,5.99292165443131,112.649063151017));
#36818=CARTESIAN_POINT('Ctrl Pts',(3.09917575053259,6.01559628526639,112.651392015122));
#36819=CARTESIAN_POINT('Origin',(0.,0.,-3.69717978381041));
#36820=CARTESIAN_POINT('',(3.09917575053242,6.01559628526648,115.045751582742));
#36821=CARTESIAN_POINT('',(3.09917575053242,6.01559628526647,114.651222310038));
#36822=CARTESIAN_POINT('',(3.09917575053259,6.01559628526639,-3.69717978381041));
#36823=CARTESIAN_POINT('',(-6.767,6.57024998643174E-12,113.69717978381));
#36824=CARTESIAN_POINT('Ctrl Pts',(-6.767,6.95491030238324E-12,113.69717978381));
#36825=CARTESIAN_POINT('Ctrl Pts',(-6.76700000000019,-0.186007249408843,
113.705929295616));
#36826=CARTESIAN_POINT('Ctrl Pts',(-6.75932637295475,-0.372014355520823,
113.714678807422));
#36827=CARTESIAN_POINT('Ctrl Pts',(-6.74400518266982,-0.557389537148472,
113.723428319228));
#36828=CARTESIAN_POINT('Ctrl Pts',(-6.72868405709718,-0.742763935804837,
113.732177794078));
#36829=CARTESIAN_POINT('Ctrl Pts',(-6.70571545653082,-0.927506129688499,
113.740927268929));
#36830=CARTESIAN_POINT('Ctrl Pts',(-6.67517739415758,-1.11098863924325,
113.74967674378));
#36831=CARTESIAN_POINT('Ctrl Pts',(-6.64463945823192,-1.29447038906028,
113.758426182402));
#36832=CARTESIAN_POINT('Ctrl Pts',(-6.6065321702726,-1.47669218227757,113.767175621023));
#36833=CARTESIAN_POINT('Ctrl Pts',(-6.56098496116824,-1.65703510503675,
113.775925059645));
#36834=CARTESIAN_POINT('Ctrl Pts',(-6.51543793687635,-1.83737729603604,
113.784674462766));
#36835=CARTESIAN_POINT('Ctrl Pts',(-6.46245112202761,-2.01584035396665,
113.793423865886));
#36836=CARTESIAN_POINT('Ctrl Pts',(-6.40220448416365,-2.19181813637784,
113.802173269006));
#36837=CARTESIAN_POINT('Ctrl Pts',(-6.34195808575326,-2.36779521935571,
113.810922637351));
#36838=CARTESIAN_POINT('Ctrl Pts',(-6.2744520148939,-2.54128677544442,113.819672005697));
#36839=CARTESIAN_POINT('Ctrl Pts',(-6.19991555136358,-2.71170355237443,
113.828421374042));
#36840=CARTESIAN_POINT('Ctrl Pts',(-6.12537937789223,-2.88211966612679,
113.837170708339));
#36841=CARTESIAN_POINT('Ctrl Pts',(-6.04381298133813,-3.04946076210056,
113.845920042636));
#36842=CARTESIAN_POINT('Ctrl Pts',(-5.95549339426513,-3.21315848206471,
113.854669376933));
#36843=CARTESIAN_POINT('Ctrl Pts',(-5.86717414355384,-3.37685557859248,
113.863418677909));
#36844=CARTESIAN_POINT('Ctrl Pts',(-5.77210188986478,-3.53690907466919,
113.872167978884));
#36845=CARTESIAN_POINT('Ctrl Pts',(-5.67059953467325,-3.6927753678451,113.88091727986));
#36846=CARTESIAN_POINT('Ctrl Pts',(-5.56909755762027,-3.84864108035415,
113.889666548241));
#36847=CARTESIAN_POINT('Ctrl Pts',(-5.46116568338335,-4.00031938103918,
113.898415816621));
#36848=CARTESIAN_POINT('Ctrl Pts',(-5.34717048686382,-4.14729511662873,
113.907165085002));
#36849=CARTESIAN_POINT('Ctrl Pts',(-5.23317570555789,-4.2942703168771,113.915914321515));
#36850=CARTESIAN_POINT('Ctrl Pts',(-5.11311782179079,-4.43654275986814,
113.924663558027));
#36851=CARTESIAN_POINT('Ctrl Pts',(-4.9874045917229,-4.57362924147349,113.93341279454));
#36852=CARTESIAN_POINT('Ctrl Pts',(-4.86169180911112,-4.71071523514146,
113.942161999911));
#36853=CARTESIAN_POINT('Ctrl Pts',(-4.73032391415718,-4.84261509316243,
113.950911205282));
#36854=CARTESIAN_POINT('Ctrl Pts',(-4.59374707237585,-4.96888084331253,
113.959660410653));
#36855=CARTESIAN_POINT('Ctrl Pts',(-4.45717070537701,-5.09514615452463,
113.96840958561));
#36856=CARTESIAN_POINT('Ctrl Pts',(-4.31538563819814,-5.2157772025338,113.977158760566));
#36857=CARTESIAN_POINT('Ctrl Pts',(-4.16887341290959,-5.33036429028407,
113.985907935522));
#36858=CARTESIAN_POINT('Ctrl Pts',(-4.02236168477658,-5.4449509892094,113.99465708079));
#36859=CARTESIAN_POINT('Ctrl Pts',(-3.87112305634767,-5.5534935923853,114.003406226058));
#36860=CARTESIAN_POINT('Ctrl Pts',(-3.71567117317069,-5.65562346102252,
114.012155371326));
#36861=CARTESIAN_POINT('Ctrl Pts',(-3.56021980457638,-5.75775299158561,
114.020904487632));
#36862=CARTESIAN_POINT('Ctrl Pts',(-3.40055544862726,-5.85346967275157,
114.029653603938));
#36863=CARTESIAN_POINT('Ctrl Pts',(-3.23722036323741,-5.94244842803378,
114.038402720244));
#36864=CARTESIAN_POINT('Ctrl Pts',(-3.07388580496405,-6.03142689616292,
114.047151808315));
#36865=CARTESIAN_POINT('Ctrl Pts',(-2.90688079258086,-6.11366734484642,
114.055900896386));
#36866=CARTESIAN_POINT('Ctrl Pts',(-2.73677251095014,-6.18889046787125,
114.064649984457));
#36867=CARTESIAN_POINT('Ctrl Pts',(-2.56666476417083,-6.2641133543809,114.073399045019));
#36868=CARTESIAN_POINT('Ctrl Pts',(-2.3934540297257,-6.33231884350109,114.082148105582));
#36869=CARTESIAN_POINT('Ctrl Pts',(-2.21772856474555,-6.39327529620864,
114.090897166144));
#36870=CARTESIAN_POINT('Ctrl Pts',(-2.042003637688,-6.45423156231914,114.099646199924));
#36871=CARTESIAN_POINT('Ctrl Pts',(-1.86376426620638,-6.507938742519,114.108395233704));
#36872=CARTESIAN_POINT('Ctrl Pts',(-1.68361578195245,-6.5542144379598,114.117144267484));
#36873=CARTESIAN_POINT('Ctrl Pts',(-1.50346783420479,-6.60048999558539,
114.125893275208));
#36874=CARTESIAN_POINT('Ctrl Pts',(-1.32141106257911,-6.63933404145362,
114.134642282932));
#36875=CARTESIAN_POINT('Ctrl Pts',(-1.13806375959763,-6.67061465526907,
114.143391290656));
#36876=CARTESIAN_POINT('Ctrl Pts',(-0.954716987426435,-6.70189517852377,
114.152140273051));
#36877=CARTESIAN_POINT('Ctrl Pts',(-0.770079973817251,-6.72561226535743,
114.160889255446));
#36878=CARTESIAN_POINT('Ctrl Pts',(-0.584779770559915,-6.74168536939717,
114.169638237841));
#36879=CARTESIAN_POINT('Ctrl Pts',(-0.391490647561377,-6.75845143942351,
114.178764418517));
#36880=CARTESIAN_POINT('Ctrl Pts',(-0.1974802131118,-6.76689975924005,114.187890599193));
#36881=CARTESIAN_POINT('Ctrl Pts',(-0.00346532630524953,-6.76699911271707,
114.197016779869));
#36882=CARTESIAN_POINT('Ctrl Pts',(0.184486595288692,-6.76709536139794,
114.205857767399));
#36883=CARTESIAN_POINT('Ctrl Pts',(0.372442378177963,-6.7593565972681,114.214698754929));
#36884=CARTESIAN_POINT('Ctrl Pts',(0.559750217714926,-6.74380965729076,
114.223539742459));
#36885=CARTESIAN_POINT('Ctrl Pts',(0.74512991445061,-6.72842275717332,114.232289721057));
#36886=CARTESIAN_POINT('Ctrl Pts',(0.929874656307067,-6.70538772273572,
114.241039699654));
#36887=CARTESIAN_POINT('Ctrl Pts',(1.11335688289069,-6.67478280180861,114.249789678252));
#36888=CARTESIAN_POINT('Ctrl Pts',(1.29683723118151,-6.64417819418161,114.258539567277));
#36889=CARTESIAN_POINT('Ctrl Pts',(1.47905480729533,-6.60600390230232,114.267289456302));
#36890=CARTESIAN_POINT('Ctrl Pts',(1.6593906480411,-6.56038959797311,114.276039345327));
#36891=CARTESIAN_POINT('Ctrl Pts',(1.83972470263565,-6.51477574543454,114.284789147688));
#36892=CARTESIAN_POINT('Ctrl Pts',(2.01817678125147,-6.46172209820319,114.293538950049));
#36893=CARTESIAN_POINT('Ctrl Pts',(2.19414072346978,-6.40140886724255,114.30228875241));
#36894=CARTESIAN_POINT('Ctrl Pts',(2.37010298131409,-6.34109621361632,114.311038471015));
#36895=CARTESIAN_POINT('Ctrl Pts',(2.54357687926239,-6.27352420826244,114.319788189621));
#36896=CARTESIAN_POINT('Ctrl Pts',(2.71397317789312,-6.19892237325785,114.328537908226));
#36897=CARTESIAN_POINT('Ctrl Pts',(2.88436790206543,-6.12432122757273,114.337287545985));
#36898=CARTESIAN_POINT('Ctrl Pts',(3.051684821256,-6.04269049717748,114.346037183743));
#36899=CARTESIAN_POINT('Ctrl Pts',(3.21535561996735,-5.95430745235282,114.354786821501));
#36900=CARTESIAN_POINT('Ctrl Pts',(3.37902496074636,-5.86592519481888,114.36353638132));
#36901=CARTESIAN_POINT('Ctrl Pts',(3.5390479938424,-5.77079087940621,114.372285941139));
#36902=CARTESIAN_POINT('Ctrl Pts',(3.69488118814359,-5.66922763747432,114.381035500958));
#36903=CARTESIAN_POINT('Ctrl Pts',(3.85071304610221,-5.56766526649475,114.389784985746));
#36904=CARTESIAN_POINT('Ctrl Pts',(4.0023548970537,-5.45967423581152,114.398534470533));
#36905=CARTESIAN_POINT('Ctrl Pts',(4.1492916860707,-5.34562133936781,114.407283955321));
#36906=CARTESIAN_POINT('Ctrl Pts',(4.29622726385176,-5.23156938309007,114.416033367984));
#36907=CARTESIAN_POINT('Ctrl Pts',(4.4384576309149,-5.11145583677703,114.424782780647));
#36908=CARTESIAN_POINT('Ctrl Pts',(4.57549970660391,-4.98568866204736,114.43353219331));
#36909=CARTESIAN_POINT('Ctrl Pts',(4.71254069814741,-4.85992248226699,114.442281536757));
#36910=CARTESIAN_POINT('Ctrl Pts',(4.84439326930777,-4.72850295734552,114.451030880203));
#36911=CARTESIAN_POINT('Ctrl Pts',(4.97060959434179,-4.59187644222243,114.459780223649));
#36912=CARTESIAN_POINT('Ctrl Pts',(5.09682496280016,-4.45525096257235,114.468529500786));
#36913=CARTESIAN_POINT('Ctrl Pts',(5.21740397615361,-4.31341878218905,114.477278777922));
#36914=CARTESIAN_POINT('Ctrl Pts',(5.33193710451476,-4.16686161439263,114.486028055058));
#36915=CARTESIAN_POINT('Ctrl Pts',(5.44646940288938,-4.02030550865117,114.494777268791));
#36916=CARTESIAN_POINT('Ctrl Pts',(5.55495572749233,-3.86902470980753,114.503526482524));
#36917=CARTESIAN_POINT('Ctrl Pts',(5.65702762491039,-3.71353301466417,114.512275696257));
#36918=CARTESIAN_POINT('Ctrl Pts',(5.75909881654756,-3.55804239467538,114.521024849493));
#36919=CARTESIAN_POINT('Ctrl Pts',(5.85475551250403,-3.39834117620206,114.529774002729));
#36920=CARTESIAN_POINT('Ctrl Pts',(5.94367283727735,-3.2349717469263,114.538523155966));
#36921=CARTESIAN_POINT('Ctrl Pts',(6.03258957675978,-3.07160339301621,114.547272251611));
#36922=CARTESIAN_POINT('Ctrl Pts',(6.11476689684977,-2.90456712830153,114.556021347257));
#36923=CARTESIAN_POINT('Ctrl Pts',(6.18992570524978,-2.73443024476546,114.564770442902));
#36924=CARTESIAN_POINT('Ctrl Pts',(6.26508404388429,-2.56429442463684,114.573519483863));
#36925=CARTESIAN_POINT('Ctrl Pts',(6.33322384283063,-2.3910582865666,114.582268524824));
#36926=CARTESIAN_POINT('Ctrl Pts',(6.39411368719797,-2.21531017132761,114.591017565785));
#36927=CARTESIAN_POINT('Ctrl Pts',(6.45500317120672,-2.03956309620204,114.599766554968));
#36928=CARTESIAN_POINT('Ctrl Pts',(6.50864269269873,-1.86130434439332,114.60851554415));
#36929=CARTESIAN_POINT('Ctrl Pts',(6.55485008446152,-1.68113930720651,114.617264533332));
#36930=CARTESIAN_POINT('Ctrl Pts',(6.60199664749247,-1.49731239212534,114.626191346862));
#36931=CARTESIAN_POINT('Ctrl Pts',(6.64140563640773,-1.31150116500351,114.635118160391));
#36932=CARTESIAN_POINT('Ctrl Pts',(6.6729377228206,-1.12436255156325,114.644044973921));
#36933=CARTESIAN_POINT('Ctrl Pts',(6.70384494949778,-0.940932395057959,
114.652794888076));
#36934=CARTESIAN_POINT('Ctrl Pts',(6.72718449348857,-0.756227260513285,
114.661544802232));
#36935=CARTESIAN_POINT('Ctrl Pts',(6.74287707373877,-0.570874564548209,
114.670294716387));
#36936=CARTESIAN_POINT('Ctrl Pts',(6.75856934538633,-0.385525513638959,
114.679044458471));
#36937=CARTESIAN_POINT('Ctrl Pts',(6.76661493004084,-0.199529212424675,
114.687794200555));
#36938=CARTESIAN_POINT('Ctrl Pts',(6.76698649908905,-0.0135174386068253,
114.696543942639));
#36939=CARTESIAN_POINT('Ctrl Pts',(6.76735806132406,0.172490924439331,114.705293524285));
#36940=CARTESIAN_POINT('Ctrl Pts',(6.76005588896323,0.358514472894918,114.714043105931));
#36941=CARTESIAN_POINT('Ctrl Pts',(6.74510478454637,0.543921359655689,114.722792687577));
#36942=CARTESIAN_POINT('Ctrl Pts',(6.73015393440758,0.729325093143993,114.731542120416));
#36943=CARTESIAN_POINT('Ctrl Pts',(6.70755443556984,0.914111900249978,114.740291553255));
#36944=CARTESIAN_POINT('Ctrl Pts',(6.67738304682422,1.09765415590909,114.749040986094));
#36945=CARTESIAN_POINT('Ctrl Pts',(6.6472121311198,1.28119353390655,114.757790281755));
#36946=CARTESIAN_POINT('Ctrl Pts',(6.60946960955629,1.46348811672046,114.766539577417));
#36947=CARTESIAN_POINT('Ctrl Pts',(6.56428366991332,1.64391876347627,114.775288873078));
#36948=CARTESIAN_POINT('Ctrl Pts',(6.51909837867883,1.82434682109123,114.784038043189));
#36949=CARTESIAN_POINT('Ctrl Pts',(6.46646995272104,2.00291071819854,114.7927872133));
#36950=CARTESIAN_POINT('Ctrl Pts',(6.40657713281749,2.17900400212116,114.80153638341));
#36951=CARTESIAN_POINT('Ctrl Pts',(6.34668509279272,2.35509499309088,114.810285439596));
#36952=CARTESIAN_POINT('Ctrl Pts',(6.27952894037749,2.52871516397569,114.819034495782));
#36953=CARTESIAN_POINT('Ctrl Pts',(6.2053367506168,2.69927486770884,114.827783551968));
#36954=CARTESIAN_POINT('Ctrl Pts',(6.12832117908154,2.87632521635419,114.83686555325));
#36955=CARTESIAN_POINT('Ctrl Pts',(6.04372366626319,3.05007728919524,114.845947554532));
#36956=CARTESIAN_POINT('Ctrl Pts',(5.95185378008107,3.21989527477753,114.855029555815));
#36957=CARTESIAN_POINT('Ctrl Pts',(5.86334450817625,3.38350129286312,114.863779336122));
#36958=CARTESIAN_POINT('Ctrl Pts',(5.76808562057524,3.54345567124525,114.872529116429));
#36959=CARTESIAN_POINT('Ctrl Pts',(5.66640068804767,3.69921508464876,114.881278896736));
#36960=CARTESIAN_POINT('Ctrl Pts',(5.56471941108222,3.85496889851852,114.890028362489));
#36961=CARTESIAN_POINT('Ctrl Pts',(5.45661270815428,4.00652780919209,114.898777828243));
#36962=CARTESIAN_POINT('Ctrl Pts',(5.34244776449444,4.15337704568805,114.907527293996));
#36963=CARTESIAN_POINT('Ctrl Pts',(5.22828631819929,4.30022178355844,114.916276491716));
#36964=CARTESIAN_POINT('Ctrl Pts',(5.10806717844407,4.44235690972291,114.925025689436));
#36965=CARTESIAN_POINT('Ctrl Pts',(4.98219864545059,4.57929969070275,114.933774887155));
#36966=CARTESIAN_POINT('Ctrl Pts',(4.85633329944376,4.71623900429639,114.942523863345));
#36967=CARTESIAN_POINT('Ctrl Pts',(4.7248190403401,4.84798602483264,114.951272839536));
#36968=CARTESIAN_POINT('Ctrl Pts',(4.58810250737571,4.97409332258782,114.960021815726));
#36969=CARTESIAN_POINT('Ctrl Pts',(4.45137708686029,5.10020881821798,114.968771360662));
#36970=CARTESIAN_POINT('Ctrl Pts',(4.30944892636451,5.22068366307603,114.977520905598));
#36971=CARTESIAN_POINT('Ctrl Pts',(4.16280009467074,5.33510865604528,114.986270450534));
#36972=CARTESIAN_POINT('Ctrl Pts',(4.01615988349207,5.44952692272583,114.995019481143));
#36973=CARTESIAN_POINT('Ctrl Pts',(3.86479978232654,5.55789587288332,115.003768511751));
#36974=CARTESIAN_POINT('Ctrl Pts',(3.70923383581495,5.65984746713598,115.012517542359));
#36975=CARTESIAN_POINT('Ctrl Pts',(3.55366577799968,5.7618004450512,115.021266691707));
#36976=CARTESIAN_POINT('Ctrl Pts',(3.39389200027266,5.85733573570813,115.030015841055));
#36977=CARTESIAN_POINT('Ctrl Pts',(3.23045513626465,5.94612887621698,115.038764990403));
#36978=CARTESIAN_POINT('Ctrl Pts',(3.18695122151857,5.96976399206541,115.041093854516));
#36979=CARTESIAN_POINT('Ctrl Pts',(3.14318791262796,5.99292165435265,115.043422718629));
#36980=CARTESIAN_POINT('Ctrl Pts',(3.09917575053242,6.01559628526648,115.045751582742));
#36981=CARTESIAN_POINT('Ctrl Pts',(3.09917575053269,6.01559628526634,113.045920956904));
#36982=CARTESIAN_POINT('Ctrl Pts',(2.94401221333304,6.09553500606012,113.054118808949));
#36983=CARTESIAN_POINT('Ctrl Pts',(2.78567091600791,6.16950925910911,113.062316660994));
#36984=CARTESIAN_POINT('Ctrl Pts',(2.62465241465346,6.23726612405257,113.070514513038));
#36985=CARTESIAN_POINT('Ctrl Pts',(2.4636658376091,6.30500955519091,113.078710739737));
#36986=CARTESIAN_POINT('Ctrl Pts',(2.30000344177766,6.36653790893265,113.086906966436));
#36987=CARTESIAN_POINT('Ctrl Pts',(2.1341875282734,6.42164562975584,113.095103193135));
#36988=CARTESIAN_POINT('Ctrl Pts',(1.96838476817524,6.47674897913955,113.103298769665));
#36989=CARTESIAN_POINT('Ctrl Pts',(1.80042917083192,6.52543259589629,113.111494346195));
#36990=CARTESIAN_POINT('Ctrl Pts',(1.63085998250116,6.56754023341131,113.119689922725));
#36991=CARTESIAN_POINT('Ctrl Pts',(1.46127339420084,6.60965219170901,113.127886340227));
#36992=CARTESIAN_POINT('Ctrl Pts',(1.29007323335485,6.64518673986874,113.136082757728));
#36993=CARTESIAN_POINT('Ctrl Pts',(1.11781081896515,6.67403835567376,113.144279175229));
#36994=CARTESIAN_POINT('Ctrl Pts',(0.945499387013171,6.70289818125501,113.152477925035));
#36995=CARTESIAN_POINT('Ctrl Pts',(0.772125453262238,6.72507122739405,113.160676674841));
#36996=CARTESIAN_POINT('Ctrl Pts',(0.598247420093158,6.74050361800599,113.168875424647));
#36997=CARTESIAN_POINT('Ctrl Pts',(0.424188066599475,6.75595210154252,113.177082724123));
#36998=CARTESIAN_POINT('Ctrl Pts',(0.24962392135627,6.76464585412231,113.1852900236));
#36999=CARTESIAN_POINT('Ctrl Pts',(0.0751163829015089,6.76658307634066,
113.193497323077));
#37000=CARTESIAN_POINT('Ctrl Pts',(-0.0994837912842878,6.7685213269157,
113.201708979323));
#37001=CARTESIAN_POINT('Ctrl Pts',(-0.274026940389897,6.76369590689139,
113.20992063557));
#37002=CARTESIAN_POINT('Ctrl Pts',(-0.447954916019131,6.75215709186437,
113.218132291817));
#37003=CARTESIAN_POINT('Ctrl Pts',(-0.622140531443315,6.74060118437177,
113.226356112003));
#37004=CARTESIAN_POINT('Ctrl Pts',(-0.795708795276499,6.72231204483203,
113.23457993219));
#37005=CARTESIAN_POINT('Ctrl Pts',(-0.968108587432515,6.69739163876053,
113.242803752376));
#37006=CARTESIAN_POINT('Ctrl Pts',(-1.13280871767227,6.67358421953876,113.250660283053));
#37007=CARTESIAN_POINT('Ctrl Pts',(-1.29644222447555,6.64372506606673,113.25851681373));
#37008=CARTESIAN_POINT('Ctrl Pts',(-1.45854106774237,6.6079457438533,113.266373344407));
#37009=CARTESIAN_POINT('Ctrl Pts',(-1.62671514307631,6.57082546397929,113.274524326582));
#37010=CARTESIAN_POINT('Ctrl Pts',(-1.79373539429731,6.52722256301833,113.282675308756));
#37011=CARTESIAN_POINT('Ctrl Pts',(-1.95905868094594,6.47721993486483,113.29082629093));
#37012=CARTESIAN_POINT('Ctrl Pts',(-2.1241899292746,6.42727538939828,113.298967804983));
#37013=CARTESIAN_POINT('Ctrl Pts',(-2.2876277903659,6.37094601922237,113.307109319036));
#37014=CARTESIAN_POINT('Ctrl Pts',(-2.44883825663352,6.30836588926547,113.315250833089));
#37015=CARTESIAN_POINT('Ctrl Pts',(-2.60989538659826,6.24584528277491,113.323384603292));
#37016=CARTESIAN_POINT('Ctrl Pts',(-2.76872900099205,6.17708588444185,113.331518373496));
#37017=CARTESIAN_POINT('Ctrl Pts',(-2.92481923568579,6.10227182601385,113.339652143699));
#37018=CARTESIAN_POINT('Ctrl Pts',(-3.08079383320364,6.02751319249087,113.347779888117));
#37019=CARTESIAN_POINT('Ctrl Pts',(-3.23402876944185,5.94670898761275,113.355907632534));
#37020=CARTESIAN_POINT('Ctrl Pts',(-3.38402319921984,5.86009180705746,113.364035376952));
#37021=CARTESIAN_POINT('Ctrl Pts',(-3.53393804301192,5.7735205849669,113.372158808847));
#37022=CARTESIAN_POINT('Ctrl Pts',(-3.68061548855392,5.68114271216995,113.380282240741));
#37023=CARTESIAN_POINT('Ctrl Pts',(-3.82357840007248,5.58323716301746,113.388405672635));
#37024=CARTESIAN_POINT('Ctrl Pts',(-3.96744821206923,5.48471053957093,113.396580636386));
#37025=CARTESIAN_POINT('Ctrl Pts',(-4.10755586438943,5.38058603430221,113.404755600136));
#37026=CARTESIAN_POINT('Ctrl Pts',(-4.24344345309155,5.27119309648342,113.412930563887));
#37027=CARTESIAN_POINT('Ctrl Pts',(-4.3784438277465,5.16251438836008,113.42105215306));
#37028=CARTESIAN_POINT('Ctrl Pts',(-4.50927880893989,5.04863609115681,113.429173742233));
#37029=CARTESIAN_POINT('Ctrl Pts',(-4.63553175135842,4.92992235051911,113.437295331406));
#37030=CARTESIAN_POINT('Ctrl Pts',(-4.76180136175537,4.8111929372323,113.445417992796));
#37031=CARTESIAN_POINT('Ctrl Pts',(-4.88348746182124,4.68762705970827,113.453540654185));
#37032=CARTESIAN_POINT('Ctrl Pts',(-5.00020963035672,4.55962637202741,113.461663315574));
#37033=CARTESIAN_POINT('Ctrl Pts',(-5.11696943596483,4.43158441051454,113.469788596117));
#37034=CARTESIAN_POINT('Ctrl Pts',(-5.22876187624127,4.29910506155716,113.477913876659));
#37035=CARTESIAN_POINT('Ctrl Pts',(-5.33524628096075,4.1626237064494,113.486039157201));
#37036=CARTESIAN_POINT('Ctrl Pts',(-5.44289081117468,4.02465541529691,113.494252960989));
#37037=CARTESIAN_POINT('Ctrl Pts',(-5.54511073204309,3.88259770788784,113.502466764777));
#37038=CARTESIAN_POINT('Ctrl Pts',(-5.6415991215207,3.73693033813274,113.510680568564));
#37039=CARTESIAN_POINT('Ctrl Pts',(-5.73721278734684,3.59258352823217,113.51881990942));
#37040=CARTESIAN_POINT('Ctrl Pts',(-5.82719827915468,3.44469257941896,113.526959250275));
#37041=CARTESIAN_POINT('Ctrl Pts',(-5.91130347514983,3.2937486583954,113.53509859113));
#37042=CARTESIAN_POINT('Ctrl Pts',(-5.99656282840136,3.14073336687334,113.543349626384));
#37043=CARTESIAN_POINT('Ctrl Pts',(-6.07577914989964,2.98458105505613,113.551600661638));
#37044=CARTESIAN_POINT('Ctrl Pts',(-6.1487405934437,2.82582344008568,113.559851696892));
#37045=CARTESIAN_POINT('Ctrl Pts',(-6.2217020369877,2.66706582511535,113.568102732146));
#37046=CARTESIAN_POINT('Ctrl Pts',(-6.28840851789907,2.50570328737299,113.5763537674));
#37047=CARTESIAN_POINT('Ctrl Pts',(-6.34870092747996,2.34228212079911,113.584604802654));
#37048=CARTESIAN_POINT('Ctrl Pts',(-6.41983622137832,2.14947156978188,113.594339690045));
#37049=CARTESIAN_POINT('Ctrl Pts',(-6.48222538237985,1.95330680321043,113.604074577435));
#37050=CARTESIAN_POINT('Ctrl Pts',(-6.53559110260409,1.75451929016532,113.613809464825));
#37051=CARTESIAN_POINT('Ctrl Pts',(-6.58871805857496,1.5566211748822,113.623500797231));
#37052=CARTESIAN_POINT('Ctrl Pts',(-6.63290207036377,1.35612378478015,113.633192129637));
#37053=CARTESIAN_POINT('Ctrl Pts',(-6.66791581979843,1.15377104318053,113.642883462043));
#37054=CARTESIAN_POINT('Ctrl Pts',(-6.70259748840101,0.953337475273793,
113.652482878964));
#37055=CARTESIAN_POINT('Ctrl Pts',(-6.72828196471674,0.751083656522569,
113.662082295886));
#37056=CARTESIAN_POINT('Ctrl Pts',(-6.7447946739725,0.547753417106862,113.671681712808));
#37057=CARTESIAN_POINT('Ctrl Pts',(-6.75941508395749,0.367724118670178,
113.680181069809));
#37058=CARTESIAN_POINT('Ctrl Pts',(-6.76684596472719,0.186851288175511,
113.688680426809));
#37059=CARTESIAN_POINT('Ctrl Pts',(-6.76699762927843,0.0056643923045232,
113.69717978381));
#37060=CARTESIAN_POINT('',(-6.767,6.77926383649621E-12,113.30282021619));
#37061=CARTESIAN_POINT('Ctrl Pts',(3.09917575053259,6.01559628526639,112.651392015122));
#37062=CARTESIAN_POINT('Ctrl Pts',(2.9338238445926,6.10078395293762,112.660141463035));
#37063=CARTESIAN_POINT('Ctrl Pts',(2.76495772122972,6.17915010267055,112.668890910947));
#37064=CARTESIAN_POINT('Ctrl Pts',(2.59315093316693,6.25042856433185,112.67764035886));
#37065=CARTESIAN_POINT('Ctrl Pts',(2.42134553245592,6.32170645041461,112.68638973612));
#37066=CARTESIAN_POINT('Ctrl Pts',(2.24659977927557,6.38589665313469,112.69513911338));
#37067=CARTESIAN_POINT('Ctrl Pts',(2.06950718689877,6.44278115439088,112.70388849064));
#37068=CARTESIAN_POINT('Ctrl Pts',(1.89241596572812,6.49966521519739,112.712637800154));
#37069=CARTESIAN_POINT('Ctrl Pts',(1.7129782145714,6.54924360009561,112.721387109669));
#37070=CARTESIAN_POINT('Ctrl Pts',(1.53180337335779,6.59134792173571,112.730136419184));
#37071=CARTESIAN_POINT('Ctrl Pts',(1.35062987477728,6.63345193135315,112.73888566386));
#37072=CARTESIAN_POINT('Ctrl Pts',(1.16771959102909,6.66808192368245,112.747634908536));
#37073=CARTESIAN_POINT('Ctrl Pts',(0.983693746906529,6.69512028363173,112.756384153212));
#37074=CARTESIAN_POINT('Ctrl Pts',(0.799669205419791,6.72215845218867,112.765133335956));
#37075=CARTESIAN_POINT('Ctrl Pts',(0.614529402873635,6.74160505424577,112.7738825187));
#37076=CARTESIAN_POINT('Ctrl Pts',(0.428903127363647,6.7533940435412,112.782631701445));
#37077=CARTESIAN_POINT('Ctrl Pts',(0.243278104164413,6.76518295330328,112.791380825163));
#37078=CARTESIAN_POINT('Ctrl Pts',(0.0571669005397858,6.76931433552275,
112.800129948882));
#37079=CARTESIAN_POINT('Ctrl Pts',(-0.12879840477671,6.76577415902474,112.8088790726));
#37080=CARTESIAN_POINT('Ctrl Pts',(-0.314762517258404,6.76223400523445,
112.8176281402));
#37081=CARTESIAN_POINT('Ctrl Pts',(-0.500580446818923,6.75102239665094,
112.826377207799));
#37082=CARTESIAN_POINT('Ctrl Pts',(-0.685621118842133,6.73217741012502,
112.835126275398));
#37083=CARTESIAN_POINT('Ctrl Pts',(-0.870660665413852,6.7133325382178,112.843875289784));
#37084=CARTESIAN_POINT('Ctrl Pts',(-1.05492267885408,6.68685441030624,112.85262430417));
#37085=CARTESIAN_POINT('Ctrl Pts',(-1.23778137635158,6.65283295028195,112.861373318555));
#37086=CARTESIAN_POINT('Ctrl Pts',(-1.42999922978739,6.61707018861888,112.870570128923));
#37087=CARTESIAN_POINT('Ctrl Pts',(-1.62066601233575,6.57297172934442,112.87976693929));
#37088=CARTESIAN_POINT('Ctrl Pts',(-1.80906628500253,6.52070304311331,112.888963749657));
#37089=CARTESIAN_POINT('Ctrl Pts',(-1.98831342545397,6.47097374915071,112.897713747395));
#37090=CARTESIAN_POINT('Ctrl Pts',(-2.16550875896574,6.41384933989572,112.906463745133));
#37091=CARTESIAN_POINT('Ctrl Pts',(-2.34005036713886,6.34952386240522,112.915213742871));
#37092=CARTESIAN_POINT('Ctrl Pts',(-2.51458843546966,6.28519968948645,112.923963563152));
#37093=CARTESIAN_POINT('Ctrl Pts',(-2.68647261717933,6.21367483971152,112.932713383432));
#37094=CARTESIAN_POINT('Ctrl Pts',(-2.85511905908611,6.135192267439,112.941463203713));
#37095=CARTESIAN_POINT('Ctrl Pts',(-3.0237623048876,6.05671118252999,112.950212858172));
#37096=CARTESIAN_POINT('Ctrl Pts',(-3.18916767379777,5.97127275992701,112.95896251263));
#37097=CARTESIAN_POINT('Ctrl Pts',(-3.35077334102657,5.87916720438071,112.967712167089));
#37098=CARTESIAN_POINT('Ctrl Pts',(-3.51237616037249,5.78706327195715,112.976461667357));
#37099=CARTESIAN_POINT('Ctrl Pts',(-3.67017916302192,5.68829258362368,112.985211167626));
#37100=CARTESIAN_POINT('Ctrl Pts',(-3.82364636566365,5.58319061741109,112.993960667894));
#37101=CARTESIAN_POINT('Ctrl Pts',(-3.97711106778699,5.47809036367774,113.002710025603));
#37102=CARTESIAN_POINT('Ctrl Pts',(-4.12623987481826,5.36665920043302,113.011459383311));
#37103=CARTESIAN_POINT('Ctrl Pts',(-4.27052628213827,5.24927559512418,113.02020874102));
#37104=CARTESIAN_POINT('Ctrl Pts',(-4.41481053024875,5.13189374643125,113.028957967796));
#37105=CARTESIAN_POINT('Ctrl Pts',(-4.55425230136427,5.00855981477447,113.037707194573));
#37106=CARTESIAN_POINT('Ctrl Pts',(-4.68837800630445,4.87969268192176,113.046456421349));
#37107=CARTESIAN_POINT('Ctrl Pts',(-4.822501882288,4.75082730631905,113.05520552882));
#37108=CARTESIAN_POINT('Ctrl Pts',(-4.95130963052881,4.61642907903617,113.063954636291));
#37109=CARTESIAN_POINT('Ctrl Pts',(-5.07436379033291,4.47695444731776,113.072703743762));
#37110=CARTESIAN_POINT('Ctrl Pts',(-5.19741643562739,4.33748153220666,113.081452743551));
#37111=CARTESIAN_POINT('Ctrl Pts',(-5.31471544462716,4.19293255254661,113.090201743341));
#37112=CARTESIAN_POINT('Ctrl Pts',(-5.4258624527558,4.04379841779667,113.098950743131));
#37113=CARTESIAN_POINT('Ctrl Pts',(-5.53702160019108,3.89464799484406,113.107700698473));
#37114=CARTESIAN_POINT('Ctrl Pts',(-5.6420272308121,3.74091164443912,113.116450653815));
#37115=CARTESIAN_POINT('Ctrl Pts',(-5.74052265232929,3.58311159163293,113.125200609157));
#37116=CARTESIAN_POINT('Ctrl Pts',(-5.83901427066882,3.42531763191845,113.13395022664));
#37117=CARTESIAN_POINT('Ctrl Pts',(-5.93099603115705,3.26346052695676,113.142699844122));
#37118=CARTESIAN_POINT('Ctrl Pts',(-6.01615550622721,3.0980900446714,113.151449461605));
#37119=CARTESIAN_POINT('Ctrl Pts',(-6.10131214578765,2.932725068639,113.160198787756));
#37120=CARTESIAN_POINT('Ctrl Pts',(-6.17964682328711,2.76384720416975,113.168948113907));
#37121=CARTESIAN_POINT('Ctrl Pts',(-6.25089348288527,2.59203002791682,113.177697440058));
#37122=CARTESIAN_POINT('Ctrl Pts',(-6.32213814889296,2.42021765937118,113.18644652139));
#37123=CARTESIAN_POINT('Ctrl Pts',(-6.38629508412554,2.24546640832007,113.195195602721));
#37124=CARTESIAN_POINT('Ctrl Pts',(-6.44314639819783,2.06836976660131,113.203944684053));
#37125=CARTESIAN_POINT('Ctrl Pts',(-6.50000285283673,1.89125711158368,113.212694556487));
#37126=CARTESIAN_POINT('Ctrl Pts',(-6.54955227673224,1.71179891440351,113.221444428922));
#37127=CARTESIAN_POINT('Ctrl Pts',(-6.59162635926362,1.5306047627853,113.230194301356));
#37128=CARTESIAN_POINT('Ctrl Pts',(-6.63369752055177,1.34942319164793,113.238943566278));
#37129=CARTESIAN_POINT('Ctrl Pts',(-6.66829431424237,1.16650618642799,113.247692831201));
#37130=CARTESIAN_POINT('Ctrl Pts',(-6.69529923745404,0.982474997619488,
113.256442096123));
#37131=CARTESIAN_POINT('Ctrl Pts',(-6.72230554731432,0.79843435917869,113.265191810303));
#37132=CARTESIAN_POINT('Ctrl Pts',(-6.74171916496694,0.613279706241307,
113.273941524483));
#37133=CARTESIAN_POINT('Ctrl Pts',(-6.75347414817269,0.427639953656364,
113.282691238662));
#37134=CARTESIAN_POINT('Ctrl Pts',(-6.76248837758731,0.285283364200966,
113.289400897838));
#37135=CARTESIAN_POINT('Ctrl Pts',(-6.76699999999986,0.142641701108919,
113.296110557014));
#37136=CARTESIAN_POINT('Ctrl Pts',(-6.767,6.77926379006094E-12,113.30282021619));
#37137=CARTESIAN_POINT('Ctrl Pts',(-6.76699998064072,-0.000511867680200162,
113.30282021619));
#37138=CARTESIAN_POINT('Ctrl Pts',(-6.76698592553831,-0.186323321307884,
113.3115153707));
#37139=CARTESIAN_POINT('Ctrl Pts',(-6.75931444471214,-0.371956404917808,
113.320210525209));
#37140=CARTESIAN_POINT('Ctrl Pts',(-6.74405514830971,-0.556784659053514,
113.328905679719));
#37141=CARTESIAN_POINT('Ctrl Pts',(-6.72877104404935,-0.741913398411343,
113.337614970409));
#37142=CARTESIAN_POINT('Ctrl Pts',(-6.7058745076392,-0.926234409616834,
113.346324261098));
#37143=CARTESIAN_POINT('Ctrl Pts',(-6.67548653246502,-1.10912963844545,
113.355033551788));
#37144=CARTESIAN_POINT('Ctrl Pts',(-6.64501723535388,-1.29251431726821,
113.363766149604));
#37145=CARTESIAN_POINT('Ctrl Pts',(-6.60701643970961,-1.47446529659286,
113.37249874742));
#37146=CARTESIAN_POINT('Ctrl Pts',(-6.56165615842634,-1.65437524721139,
113.381231345237));
#37147=CARTESIAN_POINT('Ctrl Pts',(-6.51623406590506,-1.83453035629151,
113.38997584273));
#37148=CARTESIAN_POINT('Ctrl Pts',(-6.46343254003278,-2.01263860755329,
113.398720340222));
#37149=CARTESIAN_POINT('Ctrl Pts',(-6.40347279474744,-2.18810995311695,
113.407464837715));
#37150=CARTESIAN_POINT('Ctrl Pts',(-6.34337008561044,-2.36399968036815,
113.416230184981));
#37151=CARTESIAN_POINT('Ctrl Pts',(-6.27607511803839,-2.53723965654339,
113.424995532246));
#37152=CARTESIAN_POINT('Ctrl Pts',(-6.20185744489644,-2.70725935831471,
113.433760879511));
#37153=CARTESIAN_POINT('Ctrl Pts',(-6.13987808394496,-2.84924322844755,
113.441080842521));
#37154=CARTESIAN_POINT('Ctrl Pts',(-6.07307173041068,-2.98898164504308,
113.44840080553));
#37155=CARTESIAN_POINT('Ctrl Pts',(-6.00161913178858,-3.12615687337493,
113.455720768539));
#37156=CARTESIAN_POINT('Ctrl Pts',(-5.92203931340429,-3.27893479843274,
113.463873324752));
#37157=CARTESIAN_POINT('Ctrl Pts',(-5.83649751417518,-3.42891101393908,
113.472025880965));
#37158=CARTESIAN_POINT('Ctrl Pts',(-5.74521528562023,-3.57558251504222,
113.480178437179));
#37159=CARTESIAN_POINT('Ctrl Pts',(-5.65403880972769,-3.72208409367538,
113.488321548459));
#37160=CARTESIAN_POINT('Ctrl Pts',(-5.55713533400066,-3.86528827189059,
113.496464659739));
#37161=CARTESIAN_POINT('Ctrl Pts',(-5.45477343638876,-4.00471419175796,
113.50460777102));
#37162=CARTESIAN_POINT('Ctrl Pts',(-5.35250860718878,-4.14400789589918,
113.512743160297));
#37163=CARTESIAN_POINT('Ctrl Pts',(-5.24479587600462,-4.27953018208464,
113.520878549574));
#37164=CARTESIAN_POINT('Ctrl Pts',(-5.13194847685834,-4.41082688742954,
113.529013938852));
#37165=CARTESIAN_POINT('Ctrl Pts',(-5.01918437742275,-4.542026674479,113.53714332289));
#37166=CARTESIAN_POINT('Ctrl Pts',(-4.90129339429023,-4.66900681542773,
113.545272706929));
#37167=CARTESIAN_POINT('Ctrl Pts',(-4.77863060131114,-4.7913441304307,113.553402090968));
#37168=CARTESIAN_POINT('Ctrl Pts',(-4.65603258834482,-4.91361683731059,
113.56152718176));
#37169=CARTESIAN_POINT('Ctrl Pts',(-4.52866804259884,-5.03125134382306,
113.569652272552));
#37170=CARTESIAN_POINT('Ctrl Pts',(-4.39693064433775,-5.14385943712342,
113.577777363344));
#37171=CARTESIAN_POINT('Ctrl Pts',(-4.26469037586874,-5.2568973799277,113.585933469369));
#37172=CARTESIAN_POINT('Ctrl Pts',(-4.12804405328261,-5.36487018279817,
113.594089575394));
#37173=CARTESIAN_POINT('Ctrl Pts',(-3.98742575639107,-5.46742396721428,
113.602245681419));
#37174=CARTESIAN_POINT('Ctrl Pts',(-3.84737342271321,-5.56956499119532,
113.610368960593));
#37175=CARTESIAN_POINT('Ctrl Pts',(-3.7033813386149,-5.66633033724267,113.618492239766));
#37176=CARTESIAN_POINT('Ctrl Pts',(-3.55590960036512,-5.75741225847439,
113.62661551894));
#37177=CARTESIAN_POINT('Ctrl Pts',(-3.40841822500729,-5.84850630803355,
113.634739879796));
#37178=CARTESIAN_POINT('Ctrl Pts',(-3.25744658387856,-5.93391523312716,
113.642864240653));
#37179=CARTESIAN_POINT('Ctrl Pts',(-3.10348157311169,-6.01337601729313,
113.65098860151));
#37180=CARTESIAN_POINT('Ctrl Pts',(-2.949466767967,-6.09286250015706,113.659115589895));
#37181=CARTESIAN_POINT('Ctrl Pts',(-2.7924569903133,-6.16639684369086,113.667242578281));
#37182=CARTESIAN_POINT('Ctrl Pts',(-2.63296136991059,-6.23376318322717,
113.675369566666));
#37183=CARTESIAN_POINT('Ctrl Pts',(-2.47243462848122,-6.30156503847865,
113.683549095106));
#37184=CARTESIAN_POINT('Ctrl Pts',(-2.3093901376982,-6.36311871612374,113.691728623546));
#37185=CARTESIAN_POINT('Ctrl Pts',(-2.14436396617238,-6.41825460546569,
113.699908151986));
#37186=CARTESIAN_POINT('Ctrl Pts',(-1.98011495608991,-6.47313084212984,
113.70804916039));
#37187=CARTESIAN_POINT('Ctrl Pts',(-1.81390325858461,-6.52164956662919,
113.716190168794));
#37188=CARTESIAN_POINT('Ctrl Pts',(-1.64626880851799,-6.56369469202375,
113.724331177197));
#37189=CARTESIAN_POINT('Ctrl Pts',(-1.47744458843913,-6.6060382288089,113.732529965656));
#37190=CARTESIAN_POINT('Ctrl Pts',(-1.30717771530874,-6.64181585954267,
113.740728754114));
#37191=CARTESIAN_POINT('Ctrl Pts',(-1.13602575965488,-6.67096203507414,
113.748927542572));
#37192=CARTESIAN_POINT('Ctrl Pts',(-0.964873804000891,-6.70010821060564,
113.75712633103));
#37193=CARTESIAN_POINT('Ctrl Pts',(-0.792837142456745,-6.72262294697997,
113.765325119489));
#37194=CARTESIAN_POINT('Ctrl Pts',(-0.620473771617619,-6.73849399337379,
113.773523907947));
#37195=CARTESIAN_POINT('Ctrl Pts',(-0.447390116603392,-6.75443136281237,
113.781756958079));
#37196=CARTESIAN_POINT('Ctrl Pts',(-0.273438990090556,-6.76371906131375,
113.789990008211));
#37197=CARTESIAN_POINT('Ctrl Pts',(-0.0991722470327019,-6.76627326269184,
113.798223058343));
#37198=CARTESIAN_POINT('Ctrl Pts',(0.0748869711218329,-6.76882442240872,
113.806446304178));
#37199=CARTESIAN_POINT('Ctrl Pts',(0.249260702779041,-6.76465804674041,
113.814669550013));
#37200=CARTESIAN_POINT('Ctrl Pts',(0.423390610029359,-6.75374188071612,
113.822892795847));
#37201=CARTESIAN_POINT('Ctrl Pts',(0.597348007803099,-6.74283652927342,
113.831107894961));
#37202=CARTESIAN_POINT('Ctrl Pts',(0.771061707207564,-6.7251947269294,113.839322994074));
#37203=CARTESIAN_POINT('Ctrl Pts',(0.943971899508641,-6.70083622042339,
113.847538093188));
#37204=CARTESIAN_POINT('Ctrl Pts',(1.11674538654388,-6.67649697210028,113.855746697327));
#37205=CARTESIAN_POINT('Ctrl Pts',(1.28871627871096,-6.6454516464543,113.863955301466));
#37206=CARTESIAN_POINT('Ctrl Pts',(1.45932832718849,-6.60777192656233,113.872163905605));
#37207=CARTESIAN_POINT('Ctrl Pts',(1.62983961451151,-6.57011445980026,113.880367661854));
#37208=CARTESIAN_POINT('Ctrl Pts',(1.79899330804695,-6.52583048138147,113.888571418103));
#37209=CARTESIAN_POINT('Ctrl Pts',(1.9662417189917,-6.47504305024272,113.896775174351));
#37210=CARTESIAN_POINT('Ctrl Pts',(2.1334406453472,-6.42427064582474,113.904976503316));
#37211=CARTESIAN_POINT('Ctrl Pts',(2.29873506861704,-6.36699872188743,113.91317783228));
#37212=CARTESIAN_POINT('Ctrl Pts',(2.46159062951145,-6.3034007149079,113.921379161244));
#37213=CARTESIAN_POINT('Ctrl Pts',(2.62442373106923,-6.2398114787007,113.929579359167));
#37214=CARTESIAN_POINT('Ctrl Pts',(2.78481830621493,-6.16989802656108,113.93777955709));
#37215=CARTESIAN_POINT('Ctrl Pts',(2.94225819567853,-6.09388264655322,113.945979755012));
#37216=CARTESIAN_POINT('Ctrl Pts',(3.09970490398974,-6.01786397425843,113.954180308092));
#37217=CARTESIAN_POINT('Ctrl Pts',(3.25419634898187,-5.93574300332145,113.962380861172));
#37218=CARTESIAN_POINT('Ctrl Pts',(3.40523922879428,-5.84778888082329,113.970581414252));
#37219=CARTESIAN_POINT('Ctrl Pts',(3.55631602232321,-5.75981500995182,113.978783808605));
#37220=CARTESIAN_POINT('Ctrl Pts',(3.7039423989177,-5.66600555918314,113.986986202958));
#37221=CARTESIAN_POINT('Ctrl Pts',(3.84765234961335,-5.56667408750637,113.995188597312));
#37222=CARTESIAN_POINT('Ctrl Pts',(3.99149669437555,-5.46724972344219,114.003398662345));
#37223=CARTESIAN_POINT('Ctrl Pts',(4.13141700066247,-5.36229322508902,114.011608727379));
#37224=CARTESIAN_POINT('Ctrl Pts',(4.26697804002371,-5.25216026087889,114.019818792413));
#37225=CARTESIAN_POINT('Ctrl Pts',(4.40260395649353,-5.14197458898586,114.028032786638));
#37226=CARTESIAN_POINT('Ctrl Pts',(4.53386617739443,-5.0266077481711,114.036246780864));
#37227=CARTESIAN_POINT('Ctrl Pts',(4.66036500088654,-4.90645361320291,114.044460775089));
#37228=CARTESIAN_POINT('Ctrl Pts',(4.78703628440682,-4.78613566813017,114.052685967724));
#37229=CARTESIAN_POINT('Ctrl Pts',(4.90893094189138,-4.66101764195539,114.060911160359));
#37230=CARTESIAN_POINT('Ctrl Pts',(5.02568754258432,-4.53152885065435,114.069136352994));
#37231=CARTESIAN_POINT('Ctrl Pts',(5.1306865035162,-4.41507985797864,114.076533251114));
#37232=CARTESIAN_POINT('Ctrl Pts',(5.23153055144813,-4.29509665962651,114.083930149234));
#37233=CARTESIAN_POINT('Ctrl Pts',(5.32798648012009,-4.17191191993042,114.091327047354));
#37234=CARTESIAN_POINT('Ctrl Pts',(5.44073032404227,-4.02792573621825,114.099973013845));
#37235=CARTESIAN_POINT('Ctrl Pts',(5.5477344538295,-3.8792383743941,114.108618980336));
#37236=CARTESIAN_POINT('Ctrl Pts',(5.64861059834346,-3.72632356462532,114.117264946827));
#37237=CARTESIAN_POINT('Ctrl Pts',(5.74935770855487,-3.57360435368641,114.125899853951));
#37238=CARTESIAN_POINT('Ctrl Pts',(5.84399229685624,-3.41666873097097,114.134534761076));
#37239=CARTESIAN_POINT('Ctrl Pts',(5.93216732888985,-3.25602207947855,114.1431696682));
#37240=CARTESIAN_POINT('Ctrl Pts',(6.02326970081915,-3.0900420888177,114.152091247272));
#37241=CARTESIAN_POINT('Ctrl Pts',(6.10747602102705,-2.92010066302637,114.161012826343));
#37242=CARTESIAN_POINT('Ctrl Pts',(6.18445149906859,-2.74678878978131,114.169934405415));
#37243=CARTESIAN_POINT('Ctrl Pts',(6.2587478064584,-2.57950912440569,114.17854546439));
#37244=CARTESIAN_POINT('Ctrl Pts',(6.32630795757735,-2.4090899766247,114.187156523366));
#37245=CARTESIAN_POINT('Ctrl Pts',(6.38687675112069,-2.23608907827796,114.195767582342));
#37246=CARTESIAN_POINT('Ctrl Pts',(6.44738842549554,-2.06325132776503,114.204370520691));
#37247=CARTESIAN_POINT('Ctrl Pts',(6.50092178691575,-1.8878369677393,114.212973459041));
#37248=CARTESIAN_POINT('Ctrl Pts',(6.54726957670759,-1.7104239503466,114.22157639739));
#37249=CARTESIAN_POINT('Ctrl Pts',(6.59356546769672,-1.53320959449155,114.230169702439));
#37250=CARTESIAN_POINT('Ctrl Pts',(6.63269176204127,-1.35400134051198,114.238763007488));
#37251=CARTESIAN_POINT('Ctrl Pts',(6.66449085979511,-1.17339276446867,114.247356312536));
#37252=CARTESIAN_POINT('Ctrl Pts',(6.66803379978303,-1.15327001283657,114.248313747377));
#37253=CARTESIAN_POINT('Ctrl Pts',(6.67148583384404,-1.13312989349662,114.249271182217));
#37254=CARTESIAN_POINT('Ctrl Pts',(6.67484678254197,-1.11297323848738,114.250228617058));
#37255=CARTESIAN_POINT('Ctrl Pts',(6.70502105541736,-0.932008736149903,
114.258824374606));
#37256=CARTESIAN_POINT('Ctrl Pts',(6.727814051586,-0.749922628110056,114.267420132153));
#37257=CARTESIAN_POINT('Ctrl Pts',(6.7431764123795,-0.567327834262293,114.276015889701));
#37258=CARTESIAN_POINT('Ctrl Pts',(6.75855310677793,-0.384562673263889,
114.284619667382));
#37259=CARTESIAN_POINT('Ctrl Pts',(6.7664853016141,-0.201288183326025,114.293223445064));
#37260=CARTESIAN_POINT('Ctrl Pts',(6.76697574324738,-0.0181187831159108,
114.301827222746));
#37261=CARTESIAN_POINT('Ctrl Pts',(6.76748545966571,0.17224933469393,114.310769136414));
#37262=CARTESIAN_POINT('Ctrl Pts',(6.75995667130892,0.362503558851308,114.319711050082));
#37263=CARTESIAN_POINT('Ctrl Pts',(6.74445175682765,0.551959690398153,114.32865296375));
#37264=CARTESIAN_POINT('Ctrl Pts',(6.72949253900064,0.734747898865666,114.33728016608));
#37265=CARTESIAN_POINT('Ctrl Pts',(6.70710915170723,0.916792946695289,114.345907368411));
#37266=CARTESIAN_POINT('Ctrl Pts',(6.67741002177307,1.09749004602529,114.354534570742));
#37267=CARTESIAN_POINT('Ctrl Pts',(6.64768260796348,1.27835923168437,114.363169989162));
#37268=CARTESIAN_POINT('Ctrl Pts',(6.61062560311362,1.45787760733531,114.371805407583));
#37269=CARTESIAN_POINT('Ctrl Pts',(6.56639806318465,1.63545268222744,114.380440826003));
#37270=CARTESIAN_POINT('Ctrl Pts',(6.5221051833651,1.81329009899932,114.389089002024));
#37271=CARTESIAN_POINT('Ctrl Pts',(6.47062068069418,1.98917818406113,114.397737178045));
#37272=CARTESIAN_POINT('Ctrl Pts',(6.41215320994172,2.16254022210782,114.406385354067));
#37273=CARTESIAN_POINT('Ctrl Pts',(6.40596757322697,2.18088126839705,114.407300298298));
#37274=CARTESIAN_POINT('Ctrl Pts',(6.39970382132123,2.19919406032554,114.40821524253));
#37275=CARTESIAN_POINT('Ctrl Pts',(6.39336223237251,2.21747792901593,114.409130186762));
#37276=CARTESIAN_POINT('Ctrl Pts',(6.33633806085052,2.38188821683459,114.417357452393));
#37277=CARTESIAN_POINT('Ctrl Pts',(6.27289305289448,2.54431328152196,114.425584718025));
#37278=CARTESIAN_POINT('Ctrl Pts',(6.20318477630388,2.70421663907161,114.433811983656));
#37279=CARTESIAN_POINT('Ctrl Pts',(6.13355192339866,2.86394698272506,114.442030347465));
#37280=CARTESIAN_POINT('Ctrl Pts',(6.05766944069756,3.02116072729144,114.450248711274));
#37281=CARTESIAN_POINT('Ctrl Pts',(5.97574437115397,3.1753374955462,114.458467075083));
#37282=CARTESIAN_POINT('Ctrl Pts',(5.89390505274607,3.32935288666638,114.466676836714));
#37283=CARTESIAN_POINT('Ctrl Pts',(5.80603592069383,3.48033732246086,114.474886598345));
#37284=CARTESIAN_POINT('Ctrl Pts',(5.71239160679545,3.62779149491986,114.483096359977));
#37285=CARTESIAN_POINT('Ctrl Pts',(5.6188031726874,3.77515767796556,114.491301222648));
#37286=CARTESIAN_POINT('Ctrl Pts',(5.5194466102212,3.91899749110032,114.499506085318));
#37287=CARTESIAN_POINT('Ctrl Pts',(5.41462210654726,4.05883683378498,114.507710947989));
#37288=CARTESIAN_POINT('Ctrl Pts',(5.30984115660537,4.19861807435566,114.515912401606));
#37289=CARTESIAN_POINT('Ctrl Pts',(5.19959700470538,4.33440186885736,114.524113855223));
#37290=CARTESIAN_POINT('Ctrl Pts',(5.08423275478234,4.46574364414242,114.53231530884));
#37291=CARTESIAN_POINT('Ctrl Pts',(4.96889553121661,4.59705465001883,114.540514841105));
#37292=CARTESIAN_POINT('Ctrl Pts',(4.84844083572215,4.72392544117365,114.548714373369));
#37293=CARTESIAN_POINT('Ctrl Pts',(4.72325163232275,4.84594500771114,114.556913905633));
#37294=CARTESIAN_POINT('Ctrl Pts',(4.59803605321582,4.96799028215564,114.56511516543));
#37295=CARTESIAN_POINT('Ctrl Pts',(4.46808422538635,5.0851820351484,114.573316425228));
#37296=CARTESIAN_POINT('Ctrl Pts',(4.33381586545243,5.19714624042395,114.581517685025));
#37297=CARTESIAN_POINT('Ctrl Pts',(4.19953598187009,5.30912005508282,114.589719648699));
#37298=CARTESIAN_POINT('Ctrl Pts',(4.06093910691309,5.41586520299029,114.597921612373));
#37299=CARTESIAN_POINT('Ctrl Pts',(3.918477552277,5.51704836595632,114.606123576048));
#37300=CARTESIAN_POINT('Ctrl Pts',(3.77591697650975,5.61830185857217,114.614331240683));
#37301=CARTESIAN_POINT('Ctrl Pts',(3.62948664892684,5.71398543803148,114.622538905318));
#37302=CARTESIAN_POINT('Ctrl Pts',(3.47966797528055,5.80380907523731,114.630746569953));
#37303=CARTESIAN_POINT('Ctrl Pts',(3.35508327882642,5.87850370644273,114.637571816648));
#37304=CARTESIAN_POINT('Ctrl Pts',(3.22815610505373,5.94914688140496,114.644397063343));
#37305=CARTESIAN_POINT('Ctrl Pts',(3.09917575053242,6.01559628526648,114.651222310038));
#37306=CARTESIAN_POINT('Origin',(0.,0.,-3.69717978381041));
#37307=CARTESIAN_POINT('',(3.09917575053267,6.01559628526635,117.045557306694));
#37308=CARTESIAN_POINT('',(3.09917575053275,6.01559628526631,116.651505798254));
#37309=CARTESIAN_POINT('',(3.09917575053259,6.01559628526639,-3.69717978381041));
#37310=CARTESIAN_POINT('',(-6.76775516591789,-0.00305449199090704,115.695870839299));
#37311=CARTESIAN_POINT('Ctrl Pts',(-6.76699709111062,-0.00627446415628204,
115.69717978381));
#37312=CARTESIAN_POINT('Ctrl Pts',(-6.76680730651523,-0.210956772148241,
115.706766886024));
#37313=CARTESIAN_POINT('Ctrl Pts',(-6.75732645171492,-0.415249572054033,
115.716353988239));
#37314=CARTESIAN_POINT('Ctrl Pts',(-6.73868767582741,-0.618366725860837,
115.725941090453));
#37315=CARTESIAN_POINT('Ctrl Pts',(-6.72065192928063,-0.81491233204604,
115.735218016507));
#37316=CARTESIAN_POINT('Ctrl Pts',(-6.69404169089617,-1.01035708318455,
115.744494942562));
#37317=CARTESIAN_POINT('Ctrl Pts',(-6.65902800631947,-1.20400789492969,
115.753771868617));
#37318=CARTESIAN_POINT('Ctrl Pts',(-6.62225828582773,-1.40737084592869,
115.763514058911));
#37319=CARTESIAN_POINT('Ctrl Pts',(-6.57622078574109,-1.60875504036215,
115.773256249205));
#37320=CARTESIAN_POINT('Ctrl Pts',(-6.52116985770305,-1.80738282800996,
115.782998439499));
#37321=CARTESIAN_POINT('Ctrl Pts',(-6.466118929665,-2.00601061565777,115.792740629794));
#37322=CARTESIAN_POINT('Ctrl Pts',(-6.40205474218278,-2.20188183374535,
115.802482820088));
#37323=CARTESIAN_POINT('Ctrl Pts',(-6.32928672348502,-2.3942469738764,115.812225010382));
#37324=CARTESIAN_POINT('Ctrl Pts',(-6.26780057684206,-2.55678803829943,
115.820456782413));
#37325=CARTESIAN_POINT('Ctrl Pts',(-6.19995887359178,-2.71719767811901,
115.828688554444));
#37326=CARTESIAN_POINT('Ctrl Pts',(-6.12592773741431,-2.87494319178276,
115.836920326475));
#37327=CARTESIAN_POINT('Ctrl Pts',(-6.0519850018116,-3.03250034153918,115.845142268947));
#37328=CARTESIAN_POINT('Ctrl Pts',(-5.9718677008018,-3.18739937853694,115.85336421142));
#37329=CARTESIAN_POINT('Ctrl Pts',(-5.88579116493238,-3.33912434072227,
115.861586153892));
#37330=CARTESIAN_POINT('Ctrl Pts',(-5.79980016685805,-3.49069852757035,
115.869799925882));
#37331=CARTESIAN_POINT('Ctrl Pts',(-5.70786190302352,-3.63910461169729,
115.878013697872));
#37332=CARTESIAN_POINT('Ctrl Pts',(-5.61023910391608,-3.78384806736355,
115.886227469862));
#37333=CARTESIAN_POINT('Ctrl Pts',(-5.51269376411958,-3.92847667559212,
115.894434724592));
#37334=CARTESIAN_POINT('Ctrl Pts',(-5.40947307228732,-4.06944814802103,
115.902641979322));
#37335=CARTESIAN_POINT('Ctrl Pts',(-5.30088489756532,-4.20629389163001,
115.910849234053));
#37336=CARTESIAN_POINT('Ctrl Pts',(-5.19236113966223,-4.34305845542814,
115.919051620065));
#37337=CARTESIAN_POINT('Ctrl Pts',(-5.07847646411138,-4.47570188612679,
115.927254006077));
#37338=CARTESIAN_POINT('Ctrl Pts',(-4.95958118534052,-4.60378577542617,
115.935456392089));
#37339=CARTESIAN_POINT('Ctrl Pts',(-4.84072139392669,-4.73183143479114,
115.943656329887));
#37340=CARTESIAN_POINT('Ctrl Pts',(-4.71685421897549,-4.85531999872025,
115.951856267686));
#37341=CARTESIAN_POINT('Ctrl Pts',(-4.58836943354913,-4.97384709669206,
115.960056205485));
#37342=CARTESIAN_POINT('Ctrl Pts',(-4.45990261361194,-5.09235762151641,
115.96825499672));
#37343=CARTESIAN_POINT('Ctrl Pts',(-4.32681973192093,-5.20590781851671,
115.976453787956));
#37344=CARTESIAN_POINT('Ctrl Pts',(-4.18954651542873,-5.31413106679342,
115.984652579192));
#37345=CARTESIAN_POINT('Ctrl Pts',(-4.05226759120111,-5.42235881492585,
115.992851711328));
#37346=CARTESIAN_POINT('Ctrl Pts',(-3.91079826650141,-5.52525895108938,
116.001050843465));
#37347=CARTESIAN_POINT('Ctrl Pts',(-3.76559639038595,-5.62250592038037,
116.009249975601));
#37348=CARTESIAN_POINT('Ctrl Pts',(-3.62036213658901,-5.71977457418041,
116.017450936012));
#37349=CARTESIAN_POINT('Ctrl Pts',(-3.47139397142424,-5.81138735101325,
116.025651896423));
#37350=CARTESIAN_POINT('Ctrl Pts',(-3.31917772249466,-5.89706267954608,
116.033852856834));
#37351=CARTESIAN_POINT('Ctrl Pts',(-3.16681881029716,-5.98281830648616,
116.042061503519));
#37352=CARTESIAN_POINT('Ctrl Pts',(-3.01120604489765,-6.06262519092112,
116.050270150204));
#37353=CARTESIAN_POINT('Ctrl Pts',(-2.85284963880841,-6.13624787132583,
116.058478796889));
#37354=CARTESIAN_POINT('Ctrl Pts',(-2.69441762892312,-6.20990570126601,
116.066691362613));
#37355=CARTESIAN_POINT('Ctrl Pts',(-2.53323969710407,-6.27737330204125,
116.074903928336));
#37356=CARTESIAN_POINT('Ctrl Pts',(-2.36984484701867,-6.33846388339155,
116.08311649406));
#37357=CARTESIAN_POINT('Ctrl Pts',(-2.2062257956211,-6.39963828983483,116.091340328608));
#37358=CARTESIAN_POINT('Ctrl Pts',(-2.04038408696616,-6.45441807669556,
116.099564163157));
#37359=CARTESIAN_POINT('Ctrl Pts',(-1.8728638419333,-6.5026663784619,116.107787997706));
#37360=CARTESIAN_POINT('Ctrl Pts',(-1.71894424878949,-6.54699749185239,
116.11534415468));
#37361=CARTESIAN_POINT('Ctrl Pts',(-1.5636079609306,-6.58581516289413,116.122900311654));
#37362=CARTESIAN_POINT('Ctrl Pts',(-1.40728280485742,-6.61905160178954,
116.130456468629));
#37363=CARTESIAN_POINT('Ctrl Pts',(-1.22841632173521,-6.65708057349225,
116.139102186681));
#37364=CARTESIAN_POINT('Ctrl Pts',(-1.047847489858,-6.68788907397469,116.147747904733));
#37365=CARTESIAN_POINT('Ctrl Pts',(-0.866172348406481,-6.71133626507091,
116.156393622786));
#37366=CARTESIAN_POINT('Ctrl Pts',(-0.684730440812389,-6.73475335475216,
116.165028241498));
#37367=CARTESIAN_POINT('Ctrl Pts',(-0.502185356772583,-6.75082794082531,
116.17366286021));
#37368=CARTESIAN_POINT('Ctrl Pts',(-0.319143471558151,-6.75947013045859,
116.182297478923));
#37369=CARTESIAN_POINT('Ctrl Pts',(-0.129637258018095,-6.76841752865752,
116.191237038825));
#37370=CARTESIAN_POINT('Ctrl Pts',(0.0604011792848513,-6.76939788746322,
116.200176598727));
#37371=CARTESIAN_POINT('Ctrl Pts',(0.250289741133326,-6.76236970635911,
116.20911615863));
#37372=CARTESIAN_POINT('Ctrl Pts',(0.433191873223424,-6.75560010793705,
116.2177268119));
#37373=CARTESIAN_POINT('Ctrl Pts',(0.615954612343275,-6.74140072917829,
116.226337465171));
#37374=CARTESIAN_POINT('Ctrl Pts',(0.797964871851218,-6.71978727812804,
116.234948118441));
#37375=CARTESIAN_POINT('Ctrl Pts',(0.979802846471547,-6.69819428565522,
116.243550621152));
#37376=CARTESIAN_POINT('Ctrl Pts',(1.16088945969433,-6.66920124857419,116.252153123864));
#37377=CARTESIAN_POINT('Ctrl Pts',(1.34061451440626,-6.63287582604735,116.260755626575));
#37378=CARTESIAN_POINT('Ctrl Pts',(1.52013729218686,-6.59659128705235,116.269348447342));
#37379=CARTESIAN_POINT('Ctrl Pts',(1.69830127025123,-6.55299088630148,116.27794126811));
#37380=CARTESIAN_POINT('Ctrl Pts',(1.87450402870215,-6.50219375644708,116.286534088877));
#37381=CARTESIAN_POINT('Ctrl Pts',(1.89527032414664,-6.4962070839593,116.287546791835));
#37382=CARTESIAN_POINT('Ctrl Pts',(1.91600938847612,-6.49012050984338,116.288559494794));
#37383=CARTESIAN_POINT('Ctrl Pts',(1.93672024385675,-6.48393427611936,116.289572197752));
#37384=CARTESIAN_POINT('Ctrl Pts',(2.11250243048391,-6.43142897534787,116.298167455512));
#37385=CARTESIAN_POINT('Ctrl Pts',(2.28604463769046,-6.37180217845666,116.306762713272));
#37386=CARTESIAN_POINT('Ctrl Pts',(2.45677480068814,-6.30527926254689,116.315357971032));
#37387=CARTESIAN_POINT('Ctrl Pts',(2.62766484524282,-6.23869405074759,116.323961277887));
#37388=CARTESIAN_POINT('Ctrl Pts',(2.79573730478657,-6.16519994052419,116.332564584741));
#37389=CARTESIAN_POINT('Ctrl Pts',(2.96044169954073,-6.08506975667662,116.341167891596));
#37390=CARTESIAN_POINT('Ctrl Pts',(3.13197479561537,-6.00161734762025,116.350127894536));
#37391=CARTESIAN_POINT('Ctrl Pts',(3.29985425666727,-5.91096705046701,116.359087897476));
#37392=CARTESIAN_POINT('Ctrl Pts',(3.4634895674056,-5.81347822017702,116.368047900416));
#37393=CARTESIAN_POINT('Ctrl Pts',(3.6210404273729,-5.71961431647499,116.37667474362));
#37394=CARTESIAN_POINT('Ctrl Pts',(3.77465684366746,-5.61941146417097,116.385301586825));
#37395=CARTESIAN_POINT('Ctrl Pts',(3.92384355705187,-5.51323323828972,116.39392843003));
#37396=CARTESIAN_POINT('Ctrl Pts',(4.07317285522284,-5.40695353286427,116.402563518316));
#37397=CARTESIAN_POINT('Ctrl Pts',(4.21806375686963,-5.29468723858324,116.411198606602));
#37398=CARTESIAN_POINT('Ctrl Pts',(4.35805433583493,-5.17683797369691,116.419833694888));
#37399=CARTESIAN_POINT('Ctrl Pts',(4.49825282890344,-5.05881367900213,116.428481608014));
#37400=CARTESIAN_POINT('Ctrl Pts',(4.63353622735864,-4.93519004623905,116.437129521139));
#37401=CARTESIAN_POINT('Ctrl Pts',(4.76347860229511,-4.80640828534953,116.445777434264));
#37402=CARTESIAN_POINT('Ctrl Pts',(4.77805615862535,-4.79196093224712,116.446747598468));
#37403=CARTESIAN_POINT('Ctrl Pts',(4.79256653711481,-4.77744869677917,116.447717762672));
#37404=CARTESIAN_POINT('Ctrl Pts',(4.80700916793276,-4.76287222791148,116.448687926875));
#37405=CARTESIAN_POINT('Ctrl Pts',(4.92944824517308,-4.63929852308725,116.456912606394));
#37406=CARTESIAN_POINT('Ctrl Pts',(5.04728055501749,-4.51083762810376,116.465137285913));
#37407=CARTESIAN_POINT('Ctrl Pts',(5.16009405546968,-4.3778668708295,116.473361965432));
#37408=CARTESIAN_POINT('Ctrl Pts',(5.27278897617001,-4.24503588086447,116.481577999882));
#37409=CARTESIAN_POINT('Ctrl Pts',(5.38047536257406,-4.1077047394313,116.489794034332));
#37410=CARTESIAN_POINT('Ctrl Pts',(5.48277734926742,-3.96628813103135,116.498010068782));
#37411=CARTESIAN_POINT('Ctrl Pts',(5.58499229626716,-3.82499184148997,116.506219112937));
#37412=CARTESIAN_POINT('Ctrl Pts',(5.68183175847997,-3.67961729653564,116.514428157092));
#37413=CARTESIAN_POINT('Ctrl Pts',(5.77295951792179,-3.5306128935974,116.522637201246));
#37414=CARTESIAN_POINT('Ctrl Pts',(5.8640279927246,-3.38170542788546,116.530840904874));
#37415=CARTESIAN_POINT('Ctrl Pts',(5.94939198004753,-3.22917311268944,116.539044608502));
#37416=CARTESIAN_POINT('Ctrl Pts',(6.02875800466143,-3.07349408999444,116.54724831213));
#37417=CARTESIAN_POINT('Ctrl Pts',(6.10808828585596,-2.9178851791719,116.555448321124));
#37418=CARTESIAN_POINT('Ctrl Pts',(6.18142582352859,-2.75913270287075,116.563648330118));
#37419=CARTESIAN_POINT('Ctrl Pts',(6.24852257478594,-2.59774029348403,116.571848339112));
#37420=CARTESIAN_POINT('Ctrl Pts',(6.3156139608455,-2.43636078937488,116.580047692416));
#37421=CARTESIAN_POINT('Ctrl Pts',(6.37646540892027,-2.27234209999388,116.58824704572));
#37422=CARTESIAN_POINT('Ctrl Pts',(6.43087646788075,-2.10620911945077,116.596446399024));
#37423=CARTESIAN_POINT('Ctrl Pts',(6.48528717209718,-1.9400772220457,116.604645698871));
#37424=CARTESIAN_POINT('Ctrl Pts',(6.53325745821677,-1.77183140130505,116.612844998717));
#37425=CARTESIAN_POINT('Ctrl Pts',(6.57463638418398,-1.60201292621635,116.621044298564));
#37426=CARTESIAN_POINT('Ctrl Pts',(6.61602254691606,-1.432164751556,116.629245032387));
#37427=CARTESIAN_POINT('Ctrl Pts',(6.65081496793062,-1.26074372290376,116.63744576621));
#37428=CARTESIAN_POINT('Ctrl Pts',(6.67891356828393,-1.08830259918501,116.645646500033));
#37429=CARTESIAN_POINT('Ctrl Pts',(6.70702218022163,-0.915800034368081,
116.653850155793));
#37430=CARTESIAN_POINT('Ctrl Pts',(6.7284321627926,-0.742277004077402,116.662053811553));
#37431=CARTESIAN_POINT('Ctrl Pts',(6.74309516001384,-0.568292761697633,
116.670257467313));
#37432=CARTESIAN_POINT('Ctrl Pts',(6.757774954641,-0.394109209183751,116.678470520888));
#37433=CARTESIAN_POINT('Ctrl Pts',(6.76569229223513,-0.219463746644988,
116.686683574463));
#37434=CARTESIAN_POINT('Ctrl Pts',(6.76685091939767,-0.0449180881930758,
116.694896628038));
#37435=CARTESIAN_POINT('Ctrl Pts',(6.76801023214589,0.129730852841009,116.703114541461));
#37436=CARTESIAN_POINT('Ctrl Pts',(6.76240287389372,0.30427951432804,116.711332454884));
#37437=CARTESIAN_POINT('Ctrl Pts',(6.75008462315949,0.478170032714103,116.719550368307));
#37438=CARTESIAN_POINT('Ctrl Pts',(6.73774716010927,0.652331761652603,116.727781098903));
#37439=CARTESIAN_POINT('Ctrl Pts',(6.71867792672728,0.825832939991116,116.736011829499));
#37440=CARTESIAN_POINT('Ctrl Pts',(6.69298430393332,0.99812329263584,116.744242560095));
#37441=CARTESIAN_POINT('Ctrl Pts',(6.66938778429552,1.15635137600839,116.751801501771));
#37442=CARTESIAN_POINT('Ctrl Pts',(6.6402047450701,1.31355813791996,116.759360443447));
#37443=CARTESIAN_POINT('Ctrl Pts',(6.60555540683037,1.46932867912326,116.766919385123));
#37444=CARTESIAN_POINT('Ctrl Pts',(6.56817534673759,1.63737553042465,116.77507404863));
#37445=CARTESIAN_POINT('Ctrl Pts',(6.52431713584427,1.80427031315255,116.783228712137));
#37446=CARTESIAN_POINT('Ctrl Pts',(6.47406192174189,1.96946978485372,116.791383375644));
#37447=CARTESIAN_POINT('Ctrl Pts',(6.42386897374889,2.13446457474109,116.799527935539));
#37448=CARTESIAN_POINT('Ctrl Pts',(6.36729490548146,2.29776788881894,116.807672495434));
#37449=CARTESIAN_POINT('Ctrl Pts',(6.30447207342164,2.45884543545273,116.815817055329));
#37450=CARTESIAN_POINT('Ctrl Pts',(6.24171385401069,2.61975731545512,116.823953238627));
#37451=CARTESIAN_POINT('Ctrl Pts',(6.17271979817483,2.77844764744957,116.832089421924));
#37452=CARTESIAN_POINT('Ctrl Pts',(6.09767238299263,2.93439610647386,116.840225605222));
#37453=CARTESIAN_POINT('Ctrl Pts',(6.0187573433945,3.09838148544117,116.848781092783));
#37454=CARTESIAN_POINT('Ctrl Pts',(5.9331485951568,3.25933451142286,116.857336580344));
#37455=CARTESIAN_POINT('Ctrl Pts',(5.84111685766212,3.41667131213048,116.865892067906));
#37456=CARTESIAN_POINT('Ctrl Pts',(5.7537240793098,3.56607738144107,116.874016306875));
#37457=CARTESIAN_POINT('Ctrl Pts',(5.66054009726045,3.71222244486196,116.882140545844));
#37458=CARTESIAN_POINT('Ctrl Pts',(5.56184473932597,3.85462995573273,116.890264784813));
#37459=CARTESIAN_POINT('Ctrl Pts',(5.46318110551415,3.99699169187367,116.898386412369));
#37460=CARTESIAN_POINT('Ctrl Pts',(5.35900983063957,4.13561796683221,116.906508039925));
#37461=CARTESIAN_POINT('Ctrl Pts',(5.24965458963027,4.27006038476903,116.914629667481));
#37462=CARTESIAN_POINT('Ctrl Pts',(5.14031367721987,4.40448518698425,116.922750230876));
#37463=CARTESIAN_POINT('Ctrl Pts',(5.02579038232472,4.53472694036051,116.930870794271));
#37464=CARTESIAN_POINT('Ctrl Pts',(4.90644923350734,4.66036961184575,116.938991357666));
#37465=CARTESIAN_POINT('Ctrl Pts',(4.78710099840464,4.78601974379058,116.947112403248));
#37466=CARTESIAN_POINT('Ctrl Pts',(4.66293459268715,4.90706998587007,116.955233448829));
#37467=CARTESIAN_POINT('Ctrl Pts',(4.53435199154811,5.02314055315434,116.96335449441));
#37468=CARTESIAN_POINT('Ctrl Pts',(4.40569060790862,5.13928223682169,116.971480515752));
#37469=CARTESIAN_POINT('Ctrl Pts',(4.27260789653572,5.25043790678331,116.979606537094));
#37470=CARTESIAN_POINT('Ctrl Pts',(4.13553997474194,5.35626718128506,116.987732558437));
#37471=CARTESIAN_POINT('Ctrl Pts',(3.99842323160449,5.46213415043714,116.995861474134));
#37472=CARTESIAN_POINT('Ctrl Pts',(3.85731874578134,5.56267072954954,117.003990389832));
#37473=CARTESIAN_POINT('Ctrl Pts',(3.71269209764839,5.65757955207518,117.012119305529));
#37474=CARTESIAN_POINT('Ctrl Pts',(3.56792806304677,5.75257853217648,117.020255943199));
#37475=CARTESIAN_POINT('Ctrl Pts',(3.41963549707585,5.84193889063614,117.02839258087));
#37476=CARTESIAN_POINT('Ctrl Pts',(3.26830560347552,5.92540863420326,117.03652921854));
#37477=CARTESIAN_POINT('Ctrl Pts',(3.2123357350403,5.95628019866832,117.039538581258));
#37478=CARTESIAN_POINT('Ctrl Pts',(3.15595060002474,5.98634644394689,117.042547943976));
#37479=CARTESIAN_POINT('Ctrl Pts',(3.09917575053267,6.01559628526635,117.045557306694));
#37480=CARTESIAN_POINT('Ctrl Pts',(3.09917575053242,6.01559628526648,115.045751582742));
#37481=CARTESIAN_POINT('Ctrl Pts',(2.93382384459253,6.10078395293765,115.054501030655));
#37482=CARTESIAN_POINT('Ctrl Pts',(2.76495772122977,6.17915010267052,115.063250478567));
#37483=CARTESIAN_POINT('Ctrl Pts',(2.5931509331671,6.25042856433178,115.07199992648));
#37484=CARTESIAN_POINT('Ctrl Pts',(2.4213455324562,6.3217064504145,115.08074930374));
#37485=CARTESIAN_POINT('Ctrl Pts',(2.24659977927598,6.38589665313455,115.089498681));
#37486=CARTESIAN_POINT('Ctrl Pts',(2.0695071868993,6.44278115439071,115.09824805826));
#37487=CARTESIAN_POINT('Ctrl Pts',(1.89241596572877,6.49966521519719,115.106997367774));
#37488=CARTESIAN_POINT('Ctrl Pts',(1.71297821457218,6.54924360009541,115.115746677289));
#37489=CARTESIAN_POINT('Ctrl Pts',(1.53180337335869,6.5913479217355,115.124495986804));
#37490=CARTESIAN_POINT('Ctrl Pts',(1.35062987477819,6.63345193135297,115.13324523148));
#37491=CARTESIAN_POINT('Ctrl Pts',(1.16771959102999,6.66808192368229,115.141994476156));
#37492=CARTESIAN_POINT('Ctrl Pts',(0.983693746907436,6.6951202836316,115.150743720832));
#37493=CARTESIAN_POINT('Ctrl Pts',(0.799669205420572,6.72215845218858,115.159492903576));
#37494=CARTESIAN_POINT('Ctrl Pts',(0.614529402874287,6.74160505424571,115.16824208632));
#37495=CARTESIAN_POINT('Ctrl Pts',(0.428903127364168,6.75339404354116,115.176991269065));
#37496=CARTESIAN_POINT('Ctrl Pts',(0.243278104164932,6.76518295330326,115.185740392783));
#37497=CARTESIAN_POINT('Ctrl Pts',(0.0571669005403033,6.76931433552274,
115.194489516502));
#37498=CARTESIAN_POINT('Ctrl Pts',(-0.128798404776197,6.76577415902475,
115.20323864022));
#37499=CARTESIAN_POINT('Ctrl Pts',(-0.314762517257765,6.76223400523448,
115.21198770782));
#37500=CARTESIAN_POINT('Ctrl Pts',(-0.500580446818164,6.75102239665099,
115.220736775419));
#37501=CARTESIAN_POINT('Ctrl Pts',(-0.685621118841252,6.73217741012511,
115.229485843018));
#37502=CARTESIAN_POINT('Ctrl Pts',(-0.870660665413233,6.71333253821788,
115.238234857404));
#37503=CARTESIAN_POINT('Ctrl Pts',(-1.05492267885371,6.6868544103063,115.246983871789));
#37504=CARTESIAN_POINT('Ctrl Pts',(-1.23778137635147,6.65283295028197,115.255732886175));
#37505=CARTESIAN_POINT('Ctrl Pts',(-1.42999922978729,6.6170701886189,115.264929696543));
#37506=CARTESIAN_POINT('Ctrl Pts',(-1.62066601233565,6.57297172934445,115.27412650691));
#37507=CARTESIAN_POINT('Ctrl Pts',(-1.80906628500243,6.52070304311334,115.283323317277));
#37508=CARTESIAN_POINT('Ctrl Pts',(-1.98831342545388,6.47097374915073,115.292073315015));
#37509=CARTESIAN_POINT('Ctrl Pts',(-2.16550875896566,6.41384933989574,115.300823312753));
#37510=CARTESIAN_POINT('Ctrl Pts',(-2.34005036713878,6.34952386240525,115.309573310491));
#37511=CARTESIAN_POINT('Ctrl Pts',(-2.51458843546958,6.28519968948648,115.318323130772));
#37512=CARTESIAN_POINT('Ctrl Pts',(-2.68647261717926,6.21367483971155,115.327072951052));
#37513=CARTESIAN_POINT('Ctrl Pts',(-2.85511905908604,6.13519226743903,115.335822771333));
#37514=CARTESIAN_POINT('Ctrl Pts',(-3.02376230488754,6.05671118253002,115.344572425792));
#37515=CARTESIAN_POINT('Ctrl Pts',(-3.18916767379771,5.97127275992704,115.35332208025));
#37516=CARTESIAN_POINT('Ctrl Pts',(-3.35077334102651,5.87916720438074,115.362071734709));
#37517=CARTESIAN_POINT('Ctrl Pts',(-3.51237616037244,5.78706327195719,115.370821234977));
#37518=CARTESIAN_POINT('Ctrl Pts',(-3.67017916302186,5.68829258362372,115.379570735246));
#37519=CARTESIAN_POINT('Ctrl Pts',(-3.8236463656636,5.58319061741112,115.388320235514));
#37520=CARTESIAN_POINT('Ctrl Pts',(-3.97711106778694,5.47809036367777,115.397069593223));
#37521=CARTESIAN_POINT('Ctrl Pts',(-4.12623987481822,5.36665920043306,115.405818950931));
#37522=CARTESIAN_POINT('Ctrl Pts',(-4.27052628213823,5.24927559512421,115.41456830864));
#37523=CARTESIAN_POINT('Ctrl Pts',(-4.41481053024882,5.13189374643119,115.423317535416));
#37524=CARTESIAN_POINT('Ctrl Pts',(-4.55425230136443,5.00855981477433,115.432066762193));
#37525=CARTESIAN_POINT('Ctrl Pts',(-4.6883780063047,4.87969268192152,115.440815988969));
#37526=CARTESIAN_POINT('Ctrl Pts',(-4.82250188228816,4.75082730631889,115.44956509644));
#37527=CARTESIAN_POINT('Ctrl Pts',(-4.95130963052887,4.6164290790361,115.458314203911));
#37528=CARTESIAN_POINT('Ctrl Pts',(-5.07436379033289,4.47695444731778,115.467063311382));
#37529=CARTESIAN_POINT('Ctrl Pts',(-5.19741643562687,4.33748153220726,115.475812311171));
#37530=CARTESIAN_POINT('Ctrl Pts',(-5.31471544462618,4.19293255254782,115.484561310961));
#37531=CARTESIAN_POINT('Ctrl Pts',(-5.42586245275441,4.04379841779854,115.493310310751));
#37532=CARTESIAN_POINT('Ctrl Pts',(-5.53702160018975,3.89464799484596,115.502060266093));
#37533=CARTESIAN_POINT('Ctrl Pts',(-5.64202723081082,3.74091164444105,115.510810221435));
#37534=CARTESIAN_POINT('Ctrl Pts',(-5.74052265232807,3.5831115916349,115.519560176777));
#37535=CARTESIAN_POINT('Ctrl Pts',(-5.83901427066765,3.42531763192044,115.52830979426));
#37536=CARTESIAN_POINT('Ctrl Pts',(-5.93099603115594,3.26346052695878,115.537059411742));
#37537=CARTESIAN_POINT('Ctrl Pts',(-6.01615550622615,3.09809004467345,115.545809029225));
#37538=CARTESIAN_POINT('Ctrl Pts',(-6.10131214578665,2.93272506864107,115.554558355376));
#37539=CARTESIAN_POINT('Ctrl Pts',(-6.17964682328618,2.76384720417184,115.563307681527));
#37540=CARTESIAN_POINT('Ctrl Pts',(-6.25089348288439,2.59203002791894,115.572057007678));
#37541=CARTESIAN_POINT('Ctrl Pts',(-6.32213814889229,2.42021765937296,115.58080608901));
#37542=CARTESIAN_POINT('Ctrl Pts',(-6.38629508412504,2.24546640832151,115.589555170341));
#37543=CARTESIAN_POINT('Ctrl Pts',(-6.44314639819748,2.06836976660238,115.598304251673));
#37544=CARTESIAN_POINT('Ctrl Pts',(-6.50000285283646,1.89125711158464,115.607054124107));
#37545=CARTESIAN_POINT('Ctrl Pts',(-6.54955227673203,1.71179891440435,115.615803996541));
#37546=CARTESIAN_POINT('Ctrl Pts',(-6.59162635926345,1.53060476278602,115.624553868976));
#37547=CARTESIAN_POINT('Ctrl Pts',(-6.63369752055162,1.34942319164865,115.633303133898));
#37548=CARTESIAN_POINT('Ctrl Pts',(-6.66829431424225,1.16650618642871,115.642052398821));
#37549=CARTESIAN_POINT('Ctrl Pts',(-6.69529923745393,0.982474997620204,
115.650801663743));
#37550=CARTESIAN_POINT('Ctrl Pts',(-6.72230554731424,0.798434359179406,
115.659551377923));
#37551=CARTESIAN_POINT('Ctrl Pts',(-6.74171916496688,0.613279706242019,
115.668301092103));
#37552=CARTESIAN_POINT('Ctrl Pts',(-6.75347414817264,0.427639953657075,
115.677050806282));
#37553=CARTESIAN_POINT('Ctrl Pts',(-6.76248837758729,0.285283364201547,
115.683760465458));
#37554=CARTESIAN_POINT('Ctrl Pts',(-6.76699999999985,0.142641701109372,
115.690470124634));
#37555=CARTESIAN_POINT('Ctrl Pts',(-6.767,7.10081502014786E-12,115.69717978381));
#37556=CARTESIAN_POINT('',(-6.76699755877019,-0.0057480082024489,115.302820216158));
#37557=CARTESIAN_POINT('Ctrl Pts',(3.09917575053242,6.01559628526648,114.651222310038));
#37558=CARTESIAN_POINT('Ctrl Pts',(2.94386794804138,6.09560933011252,114.659440724924));
#37559=CARTESIAN_POINT('Ctrl Pts',(2.78558299399996,6.16954045709756,114.667659139811));
#37560=CARTESIAN_POINT('Ctrl Pts',(2.62484349248842,6.23718571472272,114.675877554697));
#37561=CARTESIAN_POINT('Ctrl Pts',(2.45841482043055,6.30722519034446,114.684386849943));
#37562=CARTESIAN_POINT('Ctrl Pts',(2.2893550773906,6.37052554480549,114.692896145188));
#37563=CARTESIAN_POINT('Ctrl Pts',(2.11826038758146,6.42691698486944,114.701405440433));
#37564=CARTESIAN_POINT('Ctrl Pts',(1.94716569777231,6.48330842493339,114.709914735679));
#37565=CARTESIAN_POINT('Ctrl Pts',(1.77403648248922,6.53279089961688,114.718424030924));
#37566=CARTESIAN_POINT('Ctrl Pts',(1.5994789746382,6.5752533038424,114.72693332617));
#37567=CARTESIAN_POINT('Ctrl Pts',(1.43217998526167,6.61595001978939,114.735088784577));
#37568=CARTESIAN_POINT('Ctrl Pts',(1.26305388888637,6.65032388175451,114.743244242983));
#37569=CARTESIAN_POINT('Ctrl Pts',(1.09262403249341,6.67820797247419,114.75139970139));
#37570=CARTESIAN_POINT('Ctrl Pts',(0.922401611638456,6.70605812459014,114.759545233532));
#37571=CARTESIAN_POINT('Ctrl Pts',(0.750878946201532,6.72743417022452,114.767690765674));
#37572=CARTESIAN_POINT('Ctrl Pts',(0.578593969420025,6.74221907227515,114.775836297816));
#37573=CARTESIAN_POINT('Ctrl Pts',(0.406482458027426,6.75698908812483,114.783973628616));
#37574=CARTESIAN_POINT('Ctrl Pts',(0.233610524755594,6.76518114107602,114.792110959417));
#37575=CARTESIAN_POINT('Ctrl Pts',(0.0605257131714355,6.76672931615009,
114.800248290217));
#37576=CARTESIAN_POINT('Ctrl Pts',(-0.112421202018021,6.76827625779554,
114.808379138019));
#37577=CARTESIAN_POINT('Ctrl Pts',(-0.285580294038634,6.76318985766359,
114.816509985821));
#37578=CARTESIAN_POINT('Ctrl Pts',(-0.458399485989158,6.75145605860283,
114.824640833623));
#37579=CARTESIAN_POINT('Ctrl Pts',(-0.631117296826381,6.73972914295357,
114.832766911617));
#37580=CARTESIAN_POINT('Ctrl Pts',(-0.803495240938185,6.72136261899128,
114.840892989611));
#37581=CARTESIAN_POINT('Ctrl Pts',(-0.974981834225679,6.69639450920642,
114.849019067605));
#37582=CARTESIAN_POINT('Ctrl Pts',(-1.14707648765193,6.67133786706456,114.857173959187));
#37583=CARTESIAN_POINT('Ctrl Pts',(-1.31827308564726,6.63963273996283,114.865328850769));
#37584=CARTESIAN_POINT('Ctrl Pts',(-1.48801942654411,6.60137009917088,114.873483742351));
#37585=CARTESIAN_POINT('Ctrl Pts',(-1.65710381606168,6.56325666929985,114.881606832708));
#37586=CARTESIAN_POINT('Ctrl Pts',(-1.82474888361939,6.51863687565459,114.889729923064));
#37587=CARTESIAN_POINT('Ctrl Pts',(-1.99041941501957,6.46765178038468,114.89785301342));
#37588=CARTESIAN_POINT('Ctrl Pts',(-2.15610295562624,6.41666268153232,114.905976741639));
#37589=CARTESIAN_POINT('Ctrl Pts',(-2.31981130157248,6.35930739300896,114.914100469857));
#37590=CARTESIAN_POINT('Ctrl Pts',(-2.48102495991978,6.2957766914222,114.922224198075));
#37591=CARTESIAN_POINT('Ctrl Pts',(-2.64228194820668,6.23222891447414,114.930350109736));
#37592=CARTESIAN_POINT('Ctrl Pts',(-2.80104257358362,6.16250255358571,114.938476021396));
#37593=CARTESIAN_POINT('Ctrl Pts',(-2.95680790489217,6.086836289368,114.946601933056));
#37594=CARTESIAN_POINT('Ctrl Pts',(-3.11356937168604,6.01068613152521,114.954779810766));
#37595=CARTESIAN_POINT('Ctrl Pts',(-3.26729676315548,5.92851999817133,114.962957688476));
#37596=CARTESIAN_POINT('Ctrl Pts',(-3.41750794396777,5.84062740233592,114.971135566187));
#37597=CARTESIAN_POINT('Ctrl Pts',(-3.56700219939296,5.75315429879762,114.97927441266));
#37598=CARTESIAN_POINT('Ctrl Pts',(-3.71301345948487,5.66000952394965,114.987413259133));
#37599=CARTESIAN_POINT('Ctrl Pts',(-3.85509710640812,5.56152095205653,114.995552105607));
#37600=CARTESIAN_POINT('Ctrl Pts',(-3.99820283314257,5.46232390186104,115.003749498935));
#37601=CARTESIAN_POINT('Ctrl Pts',(-4.13732392511519,5.35770611051118,115.011946892264));
#37602=CARTESIAN_POINT('Ctrl Pts',(-4.27204172903311,5.2480423459991,115.020144285592));
#37603=CARTESIAN_POINT('Ctrl Pts',(-4.40675953295094,5.13837858148711,115.02834167892));
#37604=CARTESIAN_POINT('Ctrl Pts',(-4.53707380978711,5.02366913563118,115.036539072249));
#37605=CARTESIAN_POINT('Ctrl Pts',(-4.66260549184018,4.90432452305736,115.044736465577));
#37606=CARTESIAN_POINT('Ctrl Pts',(-4.78687260473668,4.78618215292621,115.052851280782));
#37607=CARTESIAN_POINT('Ctrl Pts',(-4.9068439986788,4.66312580612143,115.060966095986));
#37608=CARTESIAN_POINT('Ctrl Pts',(-5.02210030006701,4.53550411487707,115.069080911191));
#37609=CARTESIAN_POINT('Ctrl Pts',(-5.13722482978538,4.40802833256057,115.077186448788));
#37610=CARTESIAN_POINT('Ctrl Pts',(-5.24764475170721,4.27599786668457,115.085291986385));
#37611=CARTESIAN_POINT('Ctrl Pts',(-5.35297499051895,4.13980044819538,115.093397523982));
#37612=CARTESIAN_POINT('Ctrl Pts',(-5.45820745226497,4.00372946048322,115.101495537285));
#37613=CARTESIAN_POINT('Ctrl Pts',(-5.55835941220256,3.86349951133587,115.109593550588));
#37614=CARTESIAN_POINT('Ctrl Pts',(-5.65308384297548,3.71953385040243,115.117691563891));
#37615=CARTESIAN_POINT('Ctrl Pts',(-5.74773479793613,3.57567986070092,115.12578329573));
#37616=CARTESIAN_POINT('Ctrl Pts',(-5.83696640731683,3.42809623867887,115.133875027569));
#37617=CARTESIAN_POINT('Ctrl Pts',(-5.92047311482842,3.27723772354003,115.141966759408));
#37618=CARTESIAN_POINT('Ctrl Pts',(-6.0039444365198,3.12644313443126,115.15005506239));
#37619=CARTESIAN_POINT('Ctrl Pts',(-6.08169550585098,2.97237673674744,115.158143365372));
#37620=CARTESIAN_POINT('Ctrl Pts',(-6.15346506327538,2.81552068276001,115.166231668354));
#37621=CARTESIAN_POINT('Ctrl Pts',(-6.22521816066974,2.65870060301363,115.174318116319));
#37622=CARTESIAN_POINT('Ctrl Pts',(-6.29099232365082,2.49909247655245,115.182404564285));
#37623=CARTESIAN_POINT('Ctrl Pts',(-6.35057312732416,2.33720130808373,115.19049101225));
#37624=CARTESIAN_POINT('Ctrl Pts',(-6.41015184862715,2.17531579776913,115.198577177591));
#37625=CARTESIAN_POINT('Ctrl Pts',(-6.46353751519334,2.01114775155845,115.206663342932));
#37626=CARTESIAN_POINT('Ctrl Pts',(-6.51056459216175,1.84522022839815,115.214749508273));
#37627=CARTESIAN_POINT('Ctrl Pts',(-6.55761635707495,1.67920559777138,115.222839918633));
#37628=CARTESIAN_POINT('Ctrl Pts',(-6.59830276205021,1.51143000064262,115.230930328992));
#37629=CARTESIAN_POINT('Ctrl Pts',(-6.63250859599296,1.34243015612713,115.239020739352));
#37630=CARTESIAN_POINT('Ctrl Pts',(-6.66672400141049,1.17338302208344,115.24711341357));
#37631=CARTESIAN_POINT('Ctrl Pts',(-6.69445516007678,1.00311132232287,115.255206087787));
#37632=CARTESIAN_POINT('Ctrl Pts',(-6.71563841851484,0.832159619164219,
115.263298762005));
#37633=CARTESIAN_POINT('Ctrl Pts',(-6.73684188433465,0.661044839756617,
115.271399156081));
#37634=CARTESIAN_POINT('Ctrl Pts',(-6.75148493977132,0.489249129225492,
115.279499550157));
#37635=CARTESIAN_POINT('Ctrl Pts',(-6.75955595540448,0.317320477996312,
115.287599944234));
#37636=CARTESIAN_POINT('Ctrl Pts',(-6.76461097912664,0.209638440197907,
115.292673368208));
#37637=CARTESIAN_POINT('Ctrl Pts',(-6.76708900053199,0.101904270120243,
115.297746792183));
#37638=CARTESIAN_POINT('Ctrl Pts',(-6.76699755877019,-0.0057480082026374,
115.302820216158));
#37639=CARTESIAN_POINT('Ctrl Pts',(-6.76699755876961,-0.00574800888219676,
115.30282021619));
#37640=CARTESIAN_POINT('Ctrl Pts',(-6.76678167727306,-0.259900288408448,
115.314797875077));
#37641=CARTESIAN_POINT('Ctrl Pts',(-6.75224451939847,-0.513469327072015,
115.326775533965));
#37642=CARTESIAN_POINT('Ctrl Pts',(-6.72360183255187,-0.765158413209378,
115.338753192852));
#37643=CARTESIAN_POINT('Ctrl Pts',(-6.70464134507653,-0.931768053951088,
115.346681996897));
#37644=CARTESIAN_POINT('Ctrl Pts',(-6.67950074655919,-1.09755475887882,
115.354610800941));
#37645=CARTESIAN_POINT('Ctrl Pts',(-6.64825307665784,-1.26214897247099,
115.362539604986));
#37646=CARTESIAN_POINT('Ctrl Pts',(-6.61583335578514,-1.43291685624495,
115.370765806004));
#37647=CARTESIAN_POINT('Ctrl Pts',(-6.57678454556754,-1.6026735155636,115.378992007023));
#37648=CARTESIAN_POINT('Ctrl Pts',(-6.53118084059293,-1.77086584118386,
115.387218208042));
#37649=CARTESIAN_POINT('Ctrl Pts',(-6.48562836176938,-1.93886923817469,
115.395435168658));
#37650=CARTESIAN_POINT('Ctrl Pts',(-6.43353574300848,-2.10531145753296,
115.403652129274));
#37651=CARTESIAN_POINT('Ctrl Pts',(-6.37502850393306,-2.26964767619141,
115.411869089889));
#37652=CARTESIAN_POINT('Ctrl Pts',(-6.31657524254206,-2.43383228132836,
115.420078469691));
#37653=CARTESIAN_POINT('Ctrl Pts',(-6.25171926630277,-2.59591441949666,
115.428287849492));
#37654=CARTESIAN_POINT('Ctrl Pts',(-6.18063641974115,-2.75536248921432,
115.436497229294));
#37655=CARTESIAN_POINT('Ctrl Pts',(-6.10960489056996,-2.914695447351,115.444700682434));
#37656=CARTESIAN_POINT('Ctrl Pts',(-6.03235559060419,-3.07139779853106,
115.452904135575));
#37657=CARTESIAN_POINT('Ctrl Pts',(-5.94911320717886,-3.22495597616,115.461107588715));
#37658=CARTESIAN_POINT('Ctrl Pts',(-5.86591422135814,-3.37843409773092,
115.469306765065));
#37659=CARTESIAN_POINT('Ctrl Pts',(-5.77672854701966,-3.52877099675739,
115.477505941416));
#37660=CARTESIAN_POINT('Ctrl Pts',(-5.68182776488053,-3.67547578555929,
115.485705117766));
#37661=CARTESIAN_POINT('Ctrl Pts',(-5.58694483975551,-3.82215296964157,
115.493902751317));
#37662=CARTESIAN_POINT('Ctrl Pts',(-5.48634913824785,-3.96519910063855,
115.502100384868));
#37663=CARTESIAN_POINT('Ctrl Pts',(-5.38035686555694,-4.10415021645825,
115.51029801842));
#37664=CARTESIAN_POINT('Ctrl Pts',(-5.27437222691092,-4.24309132438748,
115.51849506154));
#37665=CARTESIAN_POINT('Ctrl Pts',(-5.16299200800417,-4.3779377188147,115.526692104661));
#37666=CARTESIAN_POINT('Ctrl Pts',(-5.04657416216928,-4.50825667256485,
115.534889147781));
#37667=CARTESIAN_POINT('Ctrl Pts',(-4.93014354252737,-4.63858992540423,
115.543087090313));
#37668=CARTESIAN_POINT('Ctrl Pts',(-4.80867443373095,-4.76439448031514,
115.551285032844));
#37669=CARTESIAN_POINT('Ctrl Pts',(-4.68256330603861,-4.88527275440592,
115.559482975375));
#37670=CARTESIAN_POINT('Ctrl Pts',(-4.55641542038324,-5.00618626122525,
115.567683307383));
#37671=CARTESIAN_POINT('Ctrl Pts',(-4.42562307965035,-5.12217037899755,
115.575883639392));
#37672=CARTESIAN_POINT('Ctrl Pts',(-4.29061766570285,-5.23286623627612,
115.5840839714));
#37673=CARTESIAN_POINT('Ctrl Pts',(-4.15547153962493,-5.34367746855671,
115.592292850371));
#37674=CARTESIAN_POINT('Ctrl Pts',(-4.01610384518723,-5.44918920088608,
115.600501729342));
#37675=CARTESIAN_POINT('Ctrl Pts',(-3.87297773024824,-5.5490839334976,115.608710608313));
#37676=CARTESIAN_POINT('Ctrl Pts',(-3.72977478189105,-5.64903229191858,
115.616923894));
#37677=CARTESIAN_POINT('Ctrl Pts',(-3.5828096924262,-5.74335744589683,115.625137179687));
#37678=CARTESIAN_POINT('Ctrl Pts',(-3.4325722208913,-5.83178677151055,115.633350465375));
#37679=CARTESIAN_POINT('Ctrl Pts',(-3.2821149704518,-5.92034545832902,115.641575766087));
#37680=CARTESIAN_POINT('Ctrl Pts',(-3.12837608715594,-6.0029909107217,115.649801066799));
#37681=CARTESIAN_POINT('Ctrl Pts',(-2.97186856562106,-6.0794972019628,115.658026367511));
#37682=CARTESIAN_POINT('Ctrl Pts',(-2.83032639155331,-6.14868791360352,
115.665465159805));
#37683=CARTESIAN_POINT('Ctrl Pts',(-2.68652018770616,-6.21285794133146,
115.672903952099));
#37684=CARTESIAN_POINT('Ctrl Pts',(-2.5408407664906,-6.27187509436687,115.680342744393));
#37685=CARTESIAN_POINT('Ctrl Pts',(-2.38118317374816,-6.33655503684279,
115.688495300606));
#37686=CARTESIAN_POINT('Ctrl Pts',(-2.21880449344297,-6.39523577316451,
115.69664785682));
#37687=CARTESIAN_POINT('Ctrl Pts',(-2.05419958647906,-6.44767811377935,
115.704800413033));
#37688=CARTESIAN_POINT('Ctrl Pts',(-1.88978537826828,-6.50005969867828,
115.712943524313));
#37689=CARTESIAN_POINT('Ctrl Pts',(-1.72315042216969,-6.5462171647288,115.721086635594));
#37690=CARTESIAN_POINT('Ctrl Pts',(-1.55481101124606,-6.58595867883393,
115.729229746874));
#37691=CARTESIAN_POINT('Ctrl Pts',(-1.38663123432373,-6.62566250659528,
115.737365136151));
#37692=CARTESIAN_POINT('Ctrl Pts',(-1.21675057378088,-6.6589624117825,115.745500525429));
#37693=CARTESIAN_POINT('Ctrl Pts',(-1.04570200091712,-6.68571584239698,
115.753635914706));
#37694=CARTESIAN_POINT('Ctrl Pts',(-0.874779689684171,-6.712449524634,115.761765298744));
#37695=CARTESIAN_POINT('Ctrl Pts',(-0.702691542388614,-6.73264629812668,
115.769894682783));
#37696=CARTESIAN_POINT('Ctrl Pts',(-0.529982283951907,-6.74621432943671,
115.778024066822));
#37697=CARTESIAN_POINT('Ctrl Pts',(-0.357364235797033,-6.75977519527123,
115.786149157614));
#37698=CARTESIAN_POINT('Ctrl Pts',(-0.184126093387903,-6.76671426221848,
115.794274248406));
#37699=CARTESIAN_POINT('Ctrl Pts',(-0.0108192902924455,-6.76699135088538,
115.802399339198));
#37700=CARTESIAN_POINT('Ctrl Pts',(0.163149062441214,-6.76726949725979,
115.810555445223));
#37701=CARTESIAN_POINT('Ctrl Pts',(0.337186232143776,-6.76083465475762,
115.818711551248));
#37702=CARTESIAN_POINT('Ctrl Pts',(0.510732301391071,-6.74769897937925,
115.826867657273));
#37703=CARTESIAN_POINT('Ctrl Pts',(0.683579879095664,-6.73461617271868,
115.834990936447));
#37704=CARTESIAN_POINT('Ctrl Pts',(0.855939936531955,-6.71488642160143,
115.84311421562));
#37705=CARTESIAN_POINT('Ctrl Pts',(1.02726267157644,-6.68857386918808,115.851237494794));
#37706=CARTESIAN_POINT('Ctrl Pts',(1.19860821969072,-6.66225781303605,115.85936185565));
#37707=CARTESIAN_POINT('Ctrl Pts',(1.36891580866499,-6.62935726519153,115.867486216507));
#37708=CARTESIAN_POINT('Ctrl Pts',(1.53764424661283,-6.58998779747417,115.875610577364));
#37709=CARTESIAN_POINT('Ctrl Pts',(1.70642725363144,-6.55060559713571,115.883737565749));
#37710=CARTESIAN_POINT('Ctrl Pts',(1.8736297365495,-6.50475039390041,115.891864554135));
#37711=CARTESIAN_POINT('Ctrl Pts',(2.03872415980008,-6.45258806993345,115.89999154252));
#37712=CARTESIAN_POINT('Ctrl Pts',(2.20488589970089,-6.40008852248075,115.90817107096));
#37713=CARTESIAN_POINT('Ctrl Pts',(2.36891187034279,-6.34120013515826,115.9163505994));
#37714=CARTESIAN_POINT('Ctrl Pts',(2.53028402869268,-6.27614146862089,115.92453012784));
#37715=CARTESIAN_POINT('Ctrl Pts',(2.6908962335249,-6.21138918431819,115.932671136244));
#37716=CARTESIAN_POINT('Ctrl Pts',(2.84887926055234,-6.14052481960731,115.940812144648));
#37717=CARTESIAN_POINT('Ctrl Pts',(3.00374683638185,-6.06381018361608,115.948953153051));
#37718=CARTESIAN_POINT('Ctrl Pts',(3.15971357051451,-5.98655107258757,115.95715194151));
#37719=CARTESIAN_POINT('Ctrl Pts',(3.31252013607327,-5.90335852202639,115.965350729968));
#37720=CARTESIAN_POINT('Ctrl Pts',(3.46169961181315,-5.81454424676369,115.973549518426));
#37721=CARTESIAN_POINT('Ctrl Pts',(3.61087908755314,-5.72572997150092,115.981748306884));
#37722=CARTESIAN_POINT('Ctrl Pts',(3.75643119719572,-5.63129422801327,115.989947095343));
#37723=CARTESIAN_POINT('Ctrl Pts',(3.89792326152257,-5.53158957690113,115.998145883801));
#37724=CARTESIAN_POINT('Ctrl Pts',(4.0400066028375,-5.43146827298173,116.006378933933));
#37725=CARTESIAN_POINT('Ctrl Pts',(4.17843763551627,-5.32572280050154,116.014611984065));
#37726=CARTESIAN_POINT('Ctrl Pts',(4.31274193540481,-5.21464725543356,116.022845034197));
#37727=CARTESIAN_POINT('Ctrl Pts',(4.44688629951697,-5.10370398426562,116.031068280032));
#37728=CARTESIAN_POINT('Ctrl Pts',(4.57691344312677,-4.98744350558531,116.039291525867));
#37729=CARTESIAN_POINT('Ctrl Pts',(4.70237745363485,-4.86620337465941,116.047514771701));
#37730=CARTESIAN_POINT('Ctrl Pts',(4.82771716768466,-4.74508335561908,116.055729870815));
#37731=CARTESIAN_POINT('Ctrl Pts',(4.94850249580004,-4.61899375627437,116.063944969928));
#37732=CARTESIAN_POINT('Ctrl Pts',(5.0643201312491,-4.48831266827804,116.072160069042));
#37733=CARTESIAN_POINT('Ctrl Pts',(5.18004619962243,-4.35773489861517,116.080368673181));
#37734=CARTESIAN_POINT('Ctrl Pts',(5.29081216168008,-4.22257313757797,116.08857727732));
#37735=CARTESIAN_POINT('Ctrl Pts',(5.39624110344065,-4.0832427007879,116.096785881459));
#37736=CARTESIAN_POINT('Ctrl Pts',(5.50160778030266,-3.9439945506581,116.104989637708));
#37737=CARTESIAN_POINT('Ctrl Pts',(5.60164350047405,-3.80058291420172,116.113193393957));
#37738=CARTESIAN_POINT('Ctrl Pts',(5.69601118519311,-3.65345666159529,116.121397150206));
#37739=CARTESIAN_POINT('Ctrl Pts',(5.79035094889282,-3.50637393993865,116.12959847917));
#37740=CARTESIAN_POINT('Ctrl Pts',(5.87902582133705,-3.35557909044896,116.137799808134));
#37741=CARTESIAN_POINT('Ctrl Pts',(5.96174154195762,-3.20155068473025,116.146001137098));
#37742=CARTESIAN_POINT('Ctrl Pts',(6.0444458552907,-3.04754352099909,116.154201335021));
#37743=CARTESIAN_POINT('Ctrl Pts',(6.12119248343146,-2.8903040043522,116.162401532944));
#37744=CARTESIAN_POINT('Ctrl Pts',(6.19173270167273,-2.73033608756075,116.170601730867));
#37745=CARTESIAN_POINT('Ctrl Pts',(6.26227597506725,-2.57036124243092,116.178802283946));
#37746=CARTESIAN_POINT('Ctrl Pts',(6.32661215841506,-2.40765808955534,116.187002837026));
#37747=CARTESIAN_POINT('Ctrl Pts',(6.38454031569593,-2.24275142564961,116.195203390106));
#37748=CARTESIAN_POINT('Ctrl Pts',(6.44248147960843,-2.07780773518664,116.203405784459));
#37749=CARTESIAN_POINT('Ctrl Pts',(6.49401163305737,-1.91065988624609,116.211608178812));
#37750=CARTESIAN_POINT('Ctrl Pts',(6.53897941783983,-1.74184878019509,116.219810573166));
#37751=CARTESIAN_POINT('Ctrl Pts',(6.58398925540597,-1.57287980608452,116.228020638199));
#37752=CARTESIAN_POINT('Ctrl Pts',(6.62242437081179,-1.4022448138883,116.236230703233));
#37753=CARTESIAN_POINT('Ctrl Pts',(6.65418414511383,-1.23049679516678,116.244440768267));
#37754=CARTESIAN_POINT('Ctrl Pts',(6.68595911908042,-1.05866658089045,116.252654762492));
#37755=CARTESIAN_POINT('Ctrl Pts',(6.71105233081618,-0.885722632397782,
116.260868756718));
#37756=CARTESIAN_POINT('Ctrl Pts',(6.72941498191682,-0.712223982433492,
116.269082750943));
#37757=CARTESIAN_POINT('Ctrl Pts',(6.74780266742679,-0.538488796023771,
116.277307943578));
#37758=CARTESIAN_POINT('Ctrl Pts',(6.75944143007326,-0.364197754368599,
116.285533136213));
#37759=CARTESIAN_POINT('Ctrl Pts',(6.7643345877112,-0.189912046732136,116.293758328849));
#37760=CARTESIAN_POINT('Ctrl Pts',(6.76873499389469,-0.0331772831448199,
116.301155226969));
#37761=CARTESIAN_POINT('Ctrl Pts',(6.76768068728745,0.123552989384368,116.308552125088));
#37762=CARTESIAN_POINT('Ctrl Pts',(6.76120990434969,0.279874309867328,116.315949023208));
#37763=CARTESIAN_POINT('Ctrl Pts',(6.75364644037559,0.462592643526132,116.324594989699));
#37764=CARTESIAN_POINT('Ctrl Pts',(6.73866511629857,0.645166944255017,116.33324095619));
#37765=CARTESIAN_POINT('Ctrl Pts',(6.71627762428073,0.826984808558199,116.341886922681));
#37766=CARTESIAN_POINT('Ctrl Pts',(6.69391876890866,1.0085701030955,116.350521829805));
#37767=CARTESIAN_POINT('Ctrl Pts',(6.66417267339425,1.18940058941265,116.35915673693));
#37768=CARTESIAN_POINT('Ctrl Pts',(6.62710294664798,1.36886651450376,116.367791644054));
#37769=CARTESIAN_POINT('Ctrl Pts',(6.58880253489332,1.55429056345799,116.376713223126));
#37770=CARTESIAN_POINT('Ctrl Pts',(6.54268384206054,1.73825756793049,116.385634802197));
#37771=CARTESIAN_POINT('Ctrl Pts',(6.4888753152869,1.9201005553513,116.394556381269));
#37772=CARTESIAN_POINT('Ctrl Pts',(6.43693962164692,2.09561440513564,116.403167440244));
#37773=CARTESIAN_POINT('Ctrl Pts',(6.37784042856936,2.26914925848573,116.41177849922));
#37774=CARTESIAN_POINT('Ctrl Pts',(6.31174519670012,2.44011507350227,116.420389558196));
#37775=CARTESIAN_POINT('Ctrl Pts',(6.24571229568589,2.61091965986242,116.428992496545));
#37776=CARTESIAN_POINT('Ctrl Pts',(6.17269661934349,2.77915975465687,116.437595434895));
#37777=CARTESIAN_POINT('Ctrl Pts',(6.09291523490216,2.94426101769139,116.446198373244));
#37778=CARTESIAN_POINT('Ctrl Pts',(6.01322318715519,3.109177405505,116.454791678293));
#37779=CARTESIAN_POINT('Ctrl Pts',(5.9267806776756,3.27096169942259,116.463384983342));
#37780=CARTESIAN_POINT('Ctrl Pts',(5.83385270556431,3.42905987258608,116.47197828839));
#37781=CARTESIAN_POINT('Ctrl Pts',(5.82349900839469,3.44667459688076,116.472935723231));
#37782=CARTESIAN_POINT('Ctrl Pts',(5.81306485201848,3.46424358452819,116.473893158072));
#37783=CARTESIAN_POINT('Ctrl Pts',(5.80255063946714,3.48176608582764,116.474850592912));
#37784=CARTESIAN_POINT('Ctrl Pts',(5.70815505444422,3.63908141050357,116.48344635046));
#37785=CARTESIAN_POINT('Ctrl Pts',(5.6074136022374,3.79246338865814,116.492042108007));
#37786=CARTESIAN_POINT('Ctrl Pts',(5.5006862180251,3.94141346864659,116.500637865555));
#37787=CARTESIAN_POINT('Ctrl Pts',(5.3938592535346,4.09050252412398,116.509241643236));
#37788=CARTESIAN_POINT('Ctrl Pts',(5.28103538684278,4.23515117942921,116.517845420918));
#37789=CARTESIAN_POINT('Ctrl Pts',(5.16261518628268,4.37489353451755,116.5264491986));
#37790=CARTESIAN_POINT('Ctrl Pts',(5.03954096828901,4.52012788635739,116.535391112268));
#37791=CARTESIAN_POINT('Ctrl Pts',(4.91042189276452,4.66006221666755,116.544333025936));
#37792=CARTESIAN_POINT('Ctrl Pts',(4.77574917437988,4.79421618446748,116.553274939604));
#37793=CARTESIAN_POINT('Ctrl Pts',(4.64581627264668,4.92364859308257,116.561902141934));
#37794=CARTESIAN_POINT('Ctrl Pts',(4.51071423877705,5.04770042059937,116.570529344265));
#37795=CARTESIAN_POINT('Ctrl Pts',(4.37091783660762,5.16598163620675,116.579156546596));
#37796=CARTESIAN_POINT('Ctrl Pts',(4.23098829976288,5.28437549656744,116.587791965016));
#37797=CARTESIAN_POINT('Ctrl Pts',(4.08635570935484,5.39698758560126,116.596427383437));
#37798=CARTESIAN_POINT('Ctrl Pts',(3.93752539171492,5.50347006802075,116.605062801857));
#37799=CARTESIAN_POINT('Ctrl Pts',(3.78847519847974,5.61010986314089,116.613710977878));
#37800=CARTESIAN_POINT('Ctrl Pts',(3.63521513783199,5.71060178466762,116.622359153899));
#37801=CARTESIAN_POINT('Ctrl Pts',(3.47827805848217,5.80464217225158,116.63100732992));
#37802=CARTESIAN_POINT('Ctrl Pts',(3.46167471054514,5.81459128868511,116.631922274152));
#37803=CARTESIAN_POINT('Ctrl Pts',(3.44503022735508,5.82446823737708,116.632837218384));
#37804=CARTESIAN_POINT('Ctrl Pts',(3.42834525442852,5.834272689585,116.633752162616));
#37805=CARTESIAN_POINT('Ctrl Pts',(3.32042649839928,5.8976880928035,116.639670041162));
#37806=CARTESIAN_POINT('Ctrl Pts',(3.21064582768168,5.95816800324278,116.645587919708));
#37807=CARTESIAN_POINT('Ctrl Pts',(3.09917575053275,6.01559628526631,116.651505798254));
#37808=CARTESIAN_POINT('Origin',(0.,0.,-3.69717978381041));
#37809=CARTESIAN_POINT('',(3.09917575053247,6.01559628526645,119.046022396269));
#37810=CARTESIAN_POINT('',(3.09917575053253,6.01559628526642,118.651527161978));
#37811=CARTESIAN_POINT('',(3.09917575053259,6.01559628526639,-3.69717978381041));
#37812=CARTESIAN_POINT('',(-6.76699965976028,-0.00214588076116945,117.697179783767));
#37813=CARTESIAN_POINT('Ctrl Pts',(-6.76699965976,-0.00214588166216128,
117.69717978381));
#37814=CARTESIAN_POINT('Ctrl Pts',(-6.76694504869395,-0.174360907245154,
117.705324442494));
#37815=CARTESIAN_POINT('Ctrl Pts',(-6.76031701235983,-0.346435165966,117.713469101178));
#37816=CARTESIAN_POINT('Ctrl Pts',(-6.74714352014871,-0.518018646879894,
117.721613759863));
#37817=CARTESIAN_POINT('Ctrl Pts',(-6.73395980007567,-0.689735344720907,
117.729764742037));
#37818=CARTESIAN_POINT('Ctrl Pts',(-6.71419573128875,-0.861218168569709,
117.737915724211));
#37819=CARTESIAN_POINT('Ctrl Pts',(-6.68785726649924,-1.03191772100945,
117.746066706386));
#37820=CARTESIAN_POINT('Ctrl Pts',(-6.66154939627771,-1.20241899009811,
117.754208220439));
#37821=CARTESIAN_POINT('Ctrl Pts',(-6.62868238682205,-1.37213844116941,
117.762349734492));
#37822=CARTESIAN_POINT('Ctrl Pts',(-6.5893141368126,-1.54052854773993,117.770491248545));
#37823=CARTESIAN_POINT('Ctrl Pts',(-6.54998333215053,-1.70875848904946,
117.778625018748));
#37824=CARTESIAN_POINT('Ctrl Pts',(-6.50416368043779,-1.87566124947419,
117.786758788951));
#37825=CARTESIAN_POINT('Ctrl Pts',(-6.45196463525836,-2.04069628935213,
117.794892559154));
#37826=CARTESIAN_POINT('Ctrl Pts',(-6.39980426098045,-2.20560906542707,
117.803020303572));
#37827=CARTESIAN_POINT('Ctrl Pts',(-6.34127401341723,-2.36865652885589,
117.81114804799));
#37828=CARTESIAN_POINT('Ctrl Pts',(-6.27653399730527,-2.52931017881777,
117.819275792408));
#37829=CARTESIAN_POINT('Ctrl Pts',(-6.21182833178989,-2.68987858708447,
117.827399224302));
#37830=CARTESIAN_POINT('Ctrl Pts',(-6.14091959589431,-2.84805537294934,
117.835522656196));
#37831=CARTESIAN_POINT('Ctrl Pts',(-6.06401713821602,-3.00332901085153,
117.84364608809));
#37832=CARTESIAN_POINT('Ctrl Pts',(-5.98662684159426,-3.15958764363878,
117.851821051841));
#37833=CARTESIAN_POINT('Ctrl Pts',(-5.90316663576624,-3.31290581242271,
117.859996015592));
#37834=CARTESIAN_POINT('Ctrl Pts',(-5.81389854146031,-3.46278395941845,
117.868170979343));
#37835=CARTESIAN_POINT('Ctrl Pts',(-5.72521328115675,-3.61168354760253,
117.876292568516));
#37836=CARTESIAN_POINT('Ctrl Pts',(-5.63079595855679,-3.75718759590019,
117.884414157689));
#37837=CARTESIAN_POINT('Ctrl Pts',(-5.53094873084053,-3.8988325351076,117.892535746862));
#37838=CARTESIAN_POINT('Ctrl Pts',(-5.43108832124234,-4.04049617435213,
117.900658408251));
#37839=CARTESIAN_POINT('Ctrl Pts',(-5.32579678955697,-4.17829939054383,
117.90878106964));
#37840=CARTESIAN_POINT('Ctrl Pts',(-5.21541850811774,-4.31180922411729,
117.91690373103));
#37841=CARTESIAN_POINT('Ctrl Pts',(-5.10500463519188,-4.44536210794841,
117.925029011572));
#37842=CARTESIAN_POINT('Ctrl Pts',(-4.98950097940368,-4.574618570468,117.933154292114));
#37843=CARTESIAN_POINT('Ctrl Pts',(-4.86929087864139,-4.69918028374947,
117.941279572657));
#37844=CARTESIAN_POINT('Ctrl Pts',(-4.74777111377544,-4.82509907105003,
117.949493376444));
#37845=CARTESIAN_POINT('Ctrl Pts',(-4.62144201836745,-4.94621993675807,
117.957707180232));
#37846=CARTESIAN_POINT('Ctrl Pts',(-4.49073559487885,-5.06217174905081,
117.96592098402));
#37847=CARTESIAN_POINT('Ctrl Pts',(-4.36121410152119,-5.17707239038764,
117.974060324875));
#37848=CARTESIAN_POINT('Ctrl Pts',(-4.2273946426779,-5.28689713218874,117.98219966573));
#37849=CARTESIAN_POINT('Ctrl Pts',(-4.08972820139918,-5.3913275024506,117.990339006586));
#37850=CARTESIAN_POINT('Ctrl Pts',(-3.95017259358062,-5.49719094790064,
117.99859004184));
#37851=CARTESIAN_POINT('Ctrl Pts',(-3.80666397681182,-5.59751067173597,
118.006841077094));
#37852=CARTESIAN_POINT('Ctrl Pts',(-3.65969912910448,-5.69200239673455,
118.015092112348));
#37853=CARTESIAN_POINT('Ctrl Pts',(-3.51273428139714,-5.78649412173314,
118.023343147602));
#37854=CARTESIAN_POINT('Ctrl Pts',(-3.36231356751004,-5.87515771074063,
118.031594182856));
#37855=CARTESIAN_POINT('Ctrl Pts',(-3.20895558971995,-5.95775906051974,
118.03984521811));
#37856=CARTESIAN_POINT('Ctrl Pts',(-3.05595564808691,-6.04016756562088,
118.048076990141));
#37857=CARTESIAN_POINT('Ctrl Pts',(-2.89955458742374,-6.11679952677498,
118.056308762171));
#37858=CARTESIAN_POINT('Ctrl Pts',(-2.74022712140345,-6.18736166092826,
118.064540534202));
#37859=CARTESIAN_POINT('Ctrl Pts',(-2.58108990829981,-6.25783953684181,
118.072762476675));
#37860=CARTESIAN_POINT('Ctrl Pts',(-2.41903357242951,-6.32226187449051,
118.080984419147));
#37861=CARTESIAN_POINT('Ctrl Pts',(-2.25455900449175,-6.38038029393744,
118.089206361619));
#37862=CARTESIAN_POINT('Ctrl Pts',(-2.0902478816989,-6.43844095871987,118.097420133609));
#37863=CARTESIAN_POINT('Ctrl Pts',(-1.92352364810583,-6.49021006239716,
118.105633905599));
#37864=CARTESIAN_POINT('Ctrl Pts',(-1.75490892751252,-6.53548648963005,
118.113847677589));
#37865=CARTESIAN_POINT('Ctrl Pts',(-1.58642799513494,-6.58072699204929,
118.122054932319));
#37866=CARTESIAN_POINT('Ctrl Pts',(-1.41605990795835,-6.61948498648544,
118.13026218705));
#37867=CARTESIAN_POINT('Ctrl Pts',(-1.24434436731198,-6.65160853444781,
118.13846944178));
#37868=CARTESIAN_POINT('Ctrl Pts',(-1.07273069198314,-6.68371302603706,
118.146671827792));
#37869=CARTESIAN_POINT('Ctrl Pts',(-0.899771506820508,-6.70919084581187,
118.154874213804));
#37870=CARTESIAN_POINT('Ctrl Pts',(-0.72601876911571,-6.72794067652887,
118.163076599816));
#37871=CARTESIAN_POINT('Ctrl Pts',(-0.552317892388534,-6.7466849108762,
118.171276537615));
#37872=CARTESIAN_POINT('Ctrl Pts',(-0.377824290307473,-6.75870511405056,
118.179476475413));
#37873=CARTESIAN_POINT('Ctrl Pts',(-0.203097394712037,-6.76395154094566,
118.187676413212));
#37874=CARTESIAN_POINT('Ctrl Pts',(-0.0283949304464053,-6.76919723425487,
118.195875204448));
#37875=CARTESIAN_POINT('Ctrl Pts',(0.146540404253272,-6.76767102608828,
118.204073995684));
#37876=CARTESIAN_POINT('Ctrl Pts',(0.321146783002885,-6.75937524803638,
118.212272786919));
#37877=CARTESIAN_POINT('Ctrl Pts',(0.495760421777843,-6.75107912505116,
118.220471919056));
#37878=CARTESIAN_POINT('Ctrl Pts',(0.670044719306279,-6.73601288834823,
118.228671051192));
#37879=CARTESIAN_POINT('Ctrl Pts',(0.843440522287577,-6.71423093774434,
118.236870183329));
#37880=CARTESIAN_POINT('Ctrl Pts',(1.01687498974217,-6.69244413011605,118.245071143739));
#37881=CARTESIAN_POINT('Ctrl Pts',(1.18942021249064,-6.66393867067187,118.25327210415));
#37882=CARTESIAN_POINT('Ctrl Pts',(1.36052475185444,-6.62882051345422,118.261473064561));
#37883=CARTESIAN_POINT('Ctrl Pts',(1.53178965736135,-6.59366944206931,118.269681711246));
#37884=CARTESIAN_POINT('Ctrl Pts',(1.70161083016143,-6.55189336246376,118.277890357931));
#37885=CARTESIAN_POINT('Ctrl Pts',(1.86944865365989,-6.50364903199191,118.286099004616));
#37886=CARTESIAN_POINT('Ctrl Pts',(2.03736660764926,-6.45538166832167,118.29431157034));
#37887=CARTESIAN_POINT('Ctrl Pts',(2.20329898416183,-6.40064000882376,118.302524136063));
#37888=CARTESIAN_POINT('Ctrl Pts',(2.36672389167267,-6.33962988040988,118.310736701787));
#37889=CARTESIAN_POINT('Ctrl Pts',(2.53037304173894,-6.27853603729601,118.318960536336));
#37890=CARTESIAN_POINT('Ctrl Pts',(2.69150751577272,-6.21115667357201,118.327184370884));
#37891=CARTESIAN_POINT('Ctrl Pts',(2.84962674316229,-6.13774522317881,118.335408205433));
#37892=CARTESIAN_POINT('Ctrl Pts',(2.99490856951235,-6.07029390960862,118.342964362408));
#37893=CARTESIAN_POINT('Ctrl Pts',(3.1376449655099,-5.99775085225321,118.350520519382));
#37894=CARTESIAN_POINT('Ctrl Pts',(3.2774684587162,-5.9203453870632,118.358076676357));
#37895=CARTESIAN_POINT('Ctrl Pts',(3.43745381945471,-5.83177843034095,118.366722394409));
#37896=CARTESIAN_POINT('Ctrl Pts',(3.59399015459903,-5.73664356539932,118.375368112462));
#37897=CARTESIAN_POINT('Ctrl Pts',(3.74653508863061,-5.63522526875897,118.384013830514));
#37898=CARTESIAN_POINT('Ctrl Pts',(3.89888418605455,-5.53393717254313,118.392648449226));
#37899=CARTESIAN_POINT('Ctrl Pts',(4.04725184741961,-5.4263818979817,118.401283067939));
#37900=CARTESIAN_POINT('Ctrl Pts',(4.19112129721432,-5.31288916429061,118.409917686651));
#37901=CARTESIAN_POINT('Ctrl Pts',(4.34007165708638,-5.19538830813057,118.418857246553));
#37902=CARTESIAN_POINT('Ctrl Pts',(4.48419999310274,-5.07152309302713,118.427796806456));
#37903=CARTESIAN_POINT('Ctrl Pts',(4.62296408571115,-4.94170942713398,118.436736366358));
#37904=CARTESIAN_POINT('Ctrl Pts',(4.75662273344032,-4.81667189967356,118.445347019629));
#37905=CARTESIAN_POINT('Ctrl Pts',(4.88530453657023,-4.68611603151257,118.453957672899));
#37906=CARTESIAN_POINT('Ctrl Pts',(5.00855689322294,-4.55045567469336,118.46256832617));
#37907=CARTESIAN_POINT('Ctrl Pts',(5.13169258327398,-4.41492372947812,118.471170828881));
#37908=CARTESIAN_POINT('Ctrl Pts',(5.24940886888443,-4.27429715378923,118.479773331592));
#37909=CARTESIAN_POINT('Ctrl Pts',(5.36128939345573,-4.12902712992045,118.488375834303));
#37910=CARTESIAN_POINT('Ctrl Pts',(5.47304399874879,-3.98392060453924,118.496968655071));
#37911=CARTESIAN_POINT('Ctrl Pts',(5.57897576032858,-3.83418129802877,118.505561475838));
#37912=CARTESIAN_POINT('Ctrl Pts',(5.67870794407446,-3.68029415752405,118.514154296606));
#37913=CARTESIAN_POINT('Ctrl Pts',(5.69046183493653,-3.66215785902308,118.515166999564));
#37914=CARTESIAN_POINT('Ctrl Pts',(5.70212966133994,-3.64396398641442,118.516179702522));
#37915=CARTESIAN_POINT('Ctrl Pts',(5.71371084367568,-3.62571336358281,118.51719240548));
#37916=CARTESIAN_POINT('Ctrl Pts',(5.8120054586408,-3.47081225831558,118.52578766324));
#37917=CARTESIAN_POINT('Ctrl Pts',(5.90393935173546,-3.31200290125589,118.534382921));
#37918=CARTESIAN_POINT('Ctrl Pts',(5.98922837091472,-3.14983055433626,118.54297817876));
#37919=CARTESIAN_POINT('Ctrl Pts',(6.07459725964346,-2.98750633989121,118.551581485614));
#37920=CARTESIAN_POINT('Ctrl Pts',(6.15330871169246,-2.82181311972006,118.560184792469));
#37921=CARTESIAN_POINT('Ctrl Pts',(6.22512598319935,-2.65331782741841,118.568788099323));
#37922=CARTESIAN_POINT('Ctrl Pts',(6.29992082368746,-2.47783666186772,118.577748102263));
#37923=CARTESIAN_POINT('Ctrl Pts',(6.36723749480628,-2.29931647923578,118.586708105203));
#37924=CARTESIAN_POINT('Ctrl Pts',(6.42686576106905,-2.11841579705175,118.595668108143));
#37925=CARTESIAN_POINT('Ctrl Pts',(6.48427686986682,-1.94424154384286,118.604294951348));
#37926=CARTESIAN_POINT('Ctrl Pts',(6.53456098319151,-1.7678609244091,118.612921794553));
#37927=CARTESIAN_POINT('Ctrl Pts',(6.57758255417386,-1.58987318457405,118.621548637758));
#37928=CARTESIAN_POINT('Ctrl Pts',(6.62064524290299,-1.41171533345186,118.630183726044));
#37929=CARTESIAN_POINT('Ctrl Pts',(6.65643147161972,-1.23194759428447,118.63881881433));
#37930=CARTESIAN_POINT('Ctrl Pts',(6.68485711682837,-1.05117759088991,118.647453902616));
#37931=CARTESIAN_POINT('Ctrl Pts',(6.71332497982467,-0.870139107762965,
118.656101815741));
#37932=CARTESIAN_POINT('Ctrl Pts',(6.73441037409266,-0.688095688152995,
118.664749728866));
#37933=CARTESIAN_POINT('Ctrl Pts',(6.74808100361623,-0.505659736021951,
118.673397641991));
#37934=CARTESIAN_POINT('Ctrl Pts',(6.74961464013867,-0.485193199443509,
118.674367806195));
#37935=CARTESIAN_POINT('Ctrl Pts',(6.75105501267373,-0.464721721982968,
118.675337970399));
#37936=CARTESIAN_POINT('Ctrl Pts',(6.75240211649703,-0.444246167261397,
118.676308134604));
#37937=CARTESIAN_POINT('Ctrl Pts',(6.76382234533885,-0.270662278225858,
118.684532814122));
#37938=CARTESIAN_POINT('Ctrl Pts',(6.76855984801392,-0.0964089831302133,
118.692757493641));
#37939=CARTESIAN_POINT('Ctrl Pts',(6.76655092705844,0.077958652659838,118.70098217316));
#37940=CARTESIAN_POINT('Ctrl Pts',(6.76454411770616,0.252143008338005,118.70919820761));
#37941=CARTESIAN_POINT('Ctrl Pts',(6.75580501001684,0.426441109936801,118.71741424206));
#37942=CARTESIAN_POINT('Ctrl Pts',(6.74032171528204,0.600293407008072,118.72563027651));
#37943=CARTESIAN_POINT('Ctrl Pts',(6.72485159391047,0.773997788568004,118.733839320665));
#37944=CARTESIAN_POINT('Ctrl Pts',(6.70264874507641,0.94725676601518,118.74204836482));
#37945=CARTESIAN_POINT('Ctrl Pts',(6.67375332031211,1.11951133072567,118.750257408974));
#37946=CARTESIAN_POINT('Ctrl Pts',(6.64487669393412,1.29165383244077,118.758461112602));
#37947=CARTESIAN_POINT('Ctrl Pts',(6.60931622341778,1.46279287079096,118.76666481623));
#37948=CARTESIAN_POINT('Ctrl Pts',(6.56716383560898,1.63237500479198,118.774868519858));
#37949=CARTESIAN_POINT('Ctrl Pts',(6.52503043162206,1.80188076549141,118.783068528852));
#37950=CARTESIAN_POINT('Ctrl Pts',(6.47631111118444,1.96983067165326,118.791268537846));
#37951=CARTESIAN_POINT('Ctrl Pts',(6.42114881779871,2.13568182547922,118.79946854684));
#37952=CARTESIAN_POINT('Ctrl Pts',(6.36599093530634,2.301519717497,118.807667900144));
#37953=CARTESIAN_POINT('Ctrl Pts',(6.30439121079043,2.46525884885741,118.815867253448));
#37954=CARTESIAN_POINT('Ctrl Pts',(6.23654246216152,2.62637147366025,118.824066606752));
#37955=CARTESIAN_POINT('Ctrl Pts',(6.16869415588639,2.78748304805641,118.832265906599));
#37956=CARTESIAN_POINT('Ctrl Pts',(6.09459704479391,2.94596781916997,118.840465206445));
#37957=CARTESIAN_POINT('Ctrl Pts',(6.01449206460866,3.10131813988174,118.848664506292));
#37958=CARTESIAN_POINT('Ctrl Pts',(5.93437307485473,3.25669562982793,118.856865240115));
#37959=CARTESIAN_POINT('Ctrl Pts',(5.84824428694125,3.40893725855291,118.865065973938));
#37960=CARTESIAN_POINT('Ctrl Pts',(5.75639257376828,3.55756005383822,118.873266707761));
#37961=CARTESIAN_POINT('Ctrl Pts',(5.66450813365637,3.70623580370629,118.881470363521));
#37962=CARTESIAN_POINT('Ctrl Pts',(5.56689689467701,3.8512898468071,118.889674019281));
#37963=CARTESIAN_POINT('Ctrl Pts',(5.46388904065899,3.99226822137073,118.897877675041));
#37964=CARTESIAN_POINT('Ctrl Pts',(5.36076318452232,4.13340809572523,118.906090728616));
#37965=CARTESIAN_POINT('Ctrl Pts',(5.25222857406988,4.27046268395185,118.914303782191));
#37966=CARTESIAN_POINT('Ctrl Pts',(5.13865634582895,4.40301032924883,118.922516835766));
#37967=CARTESIAN_POINT('Ctrl Pts',(5.0250169143524,4.53563640596144,118.930734749189));
#37968=CARTESIAN_POINT('Ctrl Pts',(4.90633416633753,4.6637499611273,118.938952662612));
#37969=CARTESIAN_POINT('Ctrl Pts',(4.78301599943664,4.78696636181342,118.947170576035));
#37970=CARTESIAN_POINT('Ctrl Pts',(4.65950549779279,4.91037493852152,118.955401306631));
#37971=CARTESIAN_POINT('Ctrl Pts',(4.53134539233315,5.02887085370543,118.963632037227));
#37972=CARTESIAN_POINT('Ctrl Pts',(4.3989775666484,5.14210903891819,118.971862767823));
#37973=CARTESIAN_POINT('Ctrl Pts',(4.27741354964925,5.24610476900551,118.979421709499));
#37974=CARTESIAN_POINT('Ctrl Pts',(4.15230118454081,5.34566636734905,118.986980651174));
#37975=CARTESIAN_POINT('Ctrl Pts',(4.02400328533236,5.44055939767543,118.99453959285));
#37976=CARTESIAN_POINT('Ctrl Pts',(3.87836703519418,5.54827639995095,119.003120060086));
#37977=CARTESIAN_POINT('Ctrl Pts',(3.72815140859379,5.65032716849108,119.011700527323));
#37978=CARTESIAN_POINT('Ctrl Pts',(3.57384383489437,5.74629700274773,119.020280994559));
#37979=CARTESIAN_POINT('Ctrl Pts',(3.42736941710198,5.83739509509255,119.028425889283));
#37980=CARTESIAN_POINT('Ctrl Pts',(3.27720854587081,5.92301404249656,119.036570784007));
#37981=CARTESIAN_POINT('Ctrl Pts',(3.12381322269131,6.00283932399818,119.04471567873));
#37982=CARTESIAN_POINT('Ctrl Pts',(3.11560995074811,6.00710821876321,119.045151251243));
#37983=CARTESIAN_POINT('Ctrl Pts',(3.1073974361474,6.01136055409734,119.045586823756));
#37984=CARTESIAN_POINT('Ctrl Pts',(3.09917575053247,6.01559628526645,119.046022396269));
#37985=CARTESIAN_POINT('Ctrl Pts',(3.09917575053267,6.01559628526635,117.045557306694));
#37986=CARTESIAN_POINT('Ctrl Pts',(2.9453982607291,6.09482092814078,117.053708314557));
#37987=CARTESIAN_POINT('Ctrl Pts',(2.78876066226697,6.16805262932651,117.061859322421));
#37988=CARTESIAN_POINT('Ctrl Pts',(2.62978194551124,6.23510512494081,117.070010330285));
#37989=CARTESIAN_POINT('Ctrl Pts',(2.53134751950769,6.27662183895505,117.075057167979));
#37990=CARTESIAN_POINT('Ctrl Pts',(2.43201590677253,6.31577062340739,117.080104005674));
#37991=CARTESIAN_POINT('Ctrl Pts',(2.33191274168623,6.35251697873854,117.085150843369));
#37992=CARTESIAN_POINT('Ctrl Pts',(2.16877389381462,6.41240277822386,117.093375711047));
#37993=CARTESIAN_POINT('Ctrl Pts',(2.00309764348051,6.46608426494995,117.101600578725));
#37994=CARTESIAN_POINT('Ctrl Pts',(1.83539640369543,6.51334085099973,117.109825446402));
#37995=CARTESIAN_POINT('Ctrl Pts',(1.66788409812793,6.56054419721585,117.118041047846));
#37996=CARTESIAN_POINT('Ctrl Pts',(1.4983516880867,6.60133695977287,117.126256649289));
#37997=CARTESIAN_POINT('Ctrl Pts',(1.32733086418371,6.6355468333051,117.134472250733));
#37998=CARTESIAN_POINT('Ctrl Pts',(1.15646835286588,6.66972503903575,117.142680247061));
#37999=CARTESIAN_POINT('Ctrl Pts',(0.984120521212369,6.69733242159352,117.150888243389));
#38000=CARTESIAN_POINT('Ctrl Pts',(0.810833588233664,6.7182466382377,117.159096239717));
#38001=CARTESIAN_POINT('Ctrl Pts',(0.637672259977481,6.73914569549084,117.167298286589));
#38002=CARTESIAN_POINT('Ctrl Pts',(0.463573540954107,6.75336120719183,117.17550033346));
#38003=CARTESIAN_POINT('Ctrl Pts',(0.289093286210853,6.76082199675955,117.183702380331));
#38004=CARTESIAN_POINT('Ctrl Pts',(0.114704463957067,6.76827887666675,117.191900129103));
#38005=CARTESIAN_POINT('Ctrl Pts',(-0.0600651381189869,6.76898807072145,
117.200097877874));
#38006=CARTESIAN_POINT('Ctrl Pts',(-0.234655016416447,6.76293028378015,
117.208295626646));
#38007=CARTESIAN_POINT('Ctrl Pts',(-0.409211595201144,6.75687365224003,
117.216491811862));
#38008=CARTESIAN_POINT('Ctrl Pts',(-0.583588160078158,6.74405261676008,
117.224687997077));
#38009=CARTESIAN_POINT('Ctrl Pts',(-0.757224370010675,6.72450000025741,
117.232884182293));
#38010=CARTESIAN_POINT('Ctrl Pts',(-0.930847734728392,6.70494883021318,
117.241079761173));
#38011=CARTESIAN_POINT('Ctrl Pts',(-1.10373049690652,6.67866711016436,117.249275340054));
#38012=CARTESIAN_POINT('Ctrl Pts',(-1.27531765423223,6.64573952851025,117.257470918934));
#38013=CARTESIAN_POINT('Ctrl Pts',(-1.44692333617855,6.61280839198077,117.265667382612));
#38014=CARTESIAN_POINT('Ctrl Pts',(-1.61723278212875,6.57323003202636,117.273863846291));
#38015=CARTESIAN_POINT('Ctrl Pts',(-1.7857013446595,6.52714023962112,117.282060309969));
#38016=CARTESIAN_POINT('Ctrl Pts',(-1.95421874611441,6.48103708581574,117.290259149797));
#38017=CARTESIAN_POINT('Ctrl Pts',(-2.12089385512129,6.4284188342491,117.298457989625));
#38018=CARTESIAN_POINT('Ctrl Pts',(-2.28519729395325,6.3694711183668,117.306656829453));
#38019=CARTESIAN_POINT('Ctrl Pts',(-2.449672352401,6.31046182991837,117.314864233202));
#38020=CARTESIAN_POINT('Ctrl Pts',(-2.61177045319455,6.2451099899666,117.323071636951));
#38021=CARTESIAN_POINT('Ctrl Pts',(-2.77098138350577,6.17364974486441,117.3312790407));
#38022=CARTESIAN_POINT('Ctrl Pts',(-2.93027759561667,6.1021512218733,117.339490840769));
#38023=CARTESIAN_POINT('Ctrl Pts',(-3.08668323308861,6.02453793029808,117.347702640839));
#38024=CARTESIAN_POINT('Ctrl Pts',(-3.23971291027645,5.94108990497435,117.355914440908));
#38025=CARTESIAN_POINT('Ctrl Pts',(-3.39296786853188,5.85751903249718,117.364138329894));
#38026=CARTESIAN_POINT('Ctrl Pts',(-3.54283662617595,5.76809644417329,117.37236221888));
#38027=CARTESIAN_POINT('Ctrl Pts',(-3.68886190994425,5.67314611211121,117.380586107866));
#38028=CARTESIAN_POINT('Ctrl Pts',(-3.82378674768664,5.58541364677054,117.388184839116));
#38029=CARTESIAN_POINT('Ctrl Pts',(-3.95543040198791,5.4929625013917,117.395783570366));
#38030=CARTESIAN_POINT('Ctrl Pts',(-4.08345817322501,5.39607805239341,117.403382301616));
#38031=CARTESIAN_POINT('Ctrl Pts',(-4.22049288443249,5.29237764145375,117.411515614665));
#38032=CARTESIAN_POINT('Ctrl Pts',(-4.35378887719579,5.18329172566531,117.419648927713));
#38033=CARTESIAN_POINT('Ctrl Pts',(-4.48288915904276,5.06912159922574,117.427782240762));
#38034=CARTESIAN_POINT('Ctrl Pts',(-4.61184316092746,4.95508083580187,117.435906338178));
#38035=CARTESIAN_POINT('Ctrl Pts',(-4.73661064209647,4.83596756979668,117.444030435595));
#38036=CARTESIAN_POINT('Ctrl Pts',(-4.85676435033687,4.71212574591308,117.452154533011));
#38037=CARTESIAN_POINT('Ctrl Pts',(-4.97680748888239,4.58839788565891,117.460271154346));
#38038=CARTESIAN_POINT('Ctrl Pts',(-5.09224505258917,4.4599503924961,117.46838777568));
#38039=CARTESIAN_POINT('Ctrl Pts',(-5.20268363544236,4.32716673927643,117.476504397014));
#38040=CARTESIAN_POINT('Ctrl Pts',(-5.31304407869666,4.19447703566328,117.484615275523));
#38041=CARTESIAN_POINT('Ctrl Pts',(-5.4184123495223,4.05745756245719,117.492726154032));
#38042=CARTESIAN_POINT('Ctrl Pts',(-5.51843265836311,3.91652779833254,117.50083703254));
#38043=CARTESIAN_POINT('Ctrl Pts',(-5.6193170374688,3.77438054927878,117.509017980508));
#38044=CARTESIAN_POINT('Ctrl Pts',(-5.71476035001969,3.6282553980885,117.517198928476));
#38045=CARTESIAN_POINT('Ctrl Pts',(-5.80443930936039,3.47861657903711,117.525379876444));
#38046=CARTESIAN_POINT('Ctrl Pts',(-5.89329220727498,3.33035613075604,117.533485467097));
#38047=CARTESIAN_POINT('Ctrl Pts',(-5.97648632005189,3.17864680254795,117.54159105775));
#38048=CARTESIAN_POINT('Ctrl Pts',(-6.05375118196756,3.02396852279028,117.549696648403));
#38049=CARTESIAN_POINT('Ctrl Pts',(-6.13101408251005,2.86929416955006,117.557802033296));
#38050=CARTESIAN_POINT('Ctrl Pts',(-6.20234786721487,2.71165134378101,117.565907418188));
#38051=CARTESIAN_POINT('Ctrl Pts',(-6.2675286300987,2.55154342916069,117.57401280308));
#38052=CARTESIAN_POINT('Ctrl Pts',(-6.33272028813418,2.39140875204278,117.582119542811));
#38053=CARTESIAN_POINT('Ctrl Pts',(-6.39175673831599,2.22880850653348,117.590226282542));
#38054=CARTESIAN_POINT('Ctrl Pts',(-6.44446273376663,2.06426477785508,117.598333022273));
#38055=CARTESIAN_POINT('Ctrl Pts',(-6.49801711294893,1.89707246581607,117.606570252397));
#38056=CARTESIAN_POINT('Ctrl Pts',(-6.54503536796367,1.72787394132357,117.614807482522));
#38057=CARTESIAN_POINT('Ctrl Pts',(-6.58538694221708,1.55723081824014,117.623044712646));
#38058=CARTESIAN_POINT('Ctrl Pts',(-6.62515362267665,1.38906115760513,117.631162544585));
#38059=CARTESIAN_POINT('Ctrl Pts',(-6.65844556932252,1.21948886721027,117.639280376523));
#38060=CARTESIAN_POINT('Ctrl Pts',(-6.68518986990649,1.04905929446319,117.647398208461));
#38061=CARTESIAN_POINT('Ctrl Pts',(-6.71252420875555,0.874869669397403,
117.655695137679));
#38062=CARTESIAN_POINT('Ctrl Pts',(-6.73301859881323,0.699784906238783,
117.663992066897));
#38063=CARTESIAN_POINT('Ctrl Pts',(-6.74665135838064,0.524389596064545,
117.672288996114));
#38064=CARTESIAN_POINT('Ctrl Pts',(-6.76028411794805,0.34899428589018,117.680585925332));
#38065=CARTESIAN_POINT('Ctrl Pts',(-6.76705529179801,0.173288834536322,
117.68888285455));
#38066=CARTESIAN_POINT('Ctrl Pts',(-6.76699965976028,-0.00214588076117313,
117.697179783767));
#38067=CARTESIAN_POINT('',(-6.76699928917358,0.00310166475318471,117.302820216236));
#38068=CARTESIAN_POINT('Ctrl Pts',(3.09917575053275,6.01559628526631,116.651505798254));
#38069=CARTESIAN_POINT('Ctrl Pts',(2.94434967243014,6.0953611504686,116.659725420501));
#38070=CARTESIAN_POINT('Ctrl Pts',(2.78626342730763,6.16923703737558,116.667945042748));
#38071=CARTESIAN_POINT('Ctrl Pts',(2.62540469763848,6.2369495086635,116.676164664995));
#38072=CARTESIAN_POINT('Ctrl Pts',(2.46469145438008,6.30460073836116,116.684376853121));
#38073=CARTESIAN_POINT('Ctrl Pts',(2.30121104862397,6.36609951607871,116.692589041246));
#38074=CARTESIAN_POINT('Ctrl Pts',(2.13547527859082,6.42121751185299,116.700801229372));
#38075=CARTESIAN_POINT('Ctrl Pts',(1.96985624995048,6.47629668347002,116.709007632975));
#38076=CARTESIAN_POINT('Ctrl Pts',(1.8019853599386,6.52500391289286,116.717214036578));
#38077=CARTESIAN_POINT('Ctrl Pts',(1.63239397125315,6.56715912115858,116.725420440181));
#38078=CARTESIAN_POINT('Ctrl Pts',(1.46288812002016,6.6092930674419,116.733622704689));
#38079=CARTESIAN_POINT('Ctrl Pts',(1.2916638457297,6.64488148983721,116.741824969197));
#38080=CARTESIAN_POINT('Ctrl Pts',(1.11926733503408,6.67379424560914,116.750027233705));
#38081=CARTESIAN_POINT('Ctrl Pts',(0.94277778271374,6.70339344864375,116.758424236552));
#38082=CARTESIAN_POINT('Ctrl Pts',(0.765060007341705,6.72599593777454,116.766821239399));
#38083=CARTESIAN_POINT('Ctrl Pts',(0.586711333395185,6.74151754512778,116.775218242245));
#38084=CARTESIAN_POINT('Ctrl Pts',(0.41253453544973,6.75667607593112,116.783418825046));
#38085=CARTESIAN_POINT('Ctrl Pts',(0.237756399157399,6.76508129044165,116.791619407847));
#38086=CARTESIAN_POINT('Ctrl Pts',(0.0629384146720956,6.76670730532647,
116.799819990648));
#38087=CARTESIAN_POINT('Ctrl Pts',(-0.111902228408066,6.76833353096313,
116.808021636347));
#38088=CARTESIAN_POINT('Ctrl Pts',(-0.28678237158857,6.76317880280661,116.816223282046));
#38089=CARTESIAN_POINT('Ctrl Pts',(-0.461140661102264,6.75126938365506,
116.824424927745));
#38090=CARTESIAN_POINT('Ctrl Pts',(-0.635553147909284,6.73935626259587,
116.832629122833));
#38091=CARTESIAN_POINT('Ctrl Pts',(-0.809443100514926,6.72068429234751,
116.84083331792));
#38092=CARTESIAN_POINT('Ctrl Pts',(-0.982254361380472,6.69533161012575,
116.849037513008));
#38093=CARTESIAN_POINT('Ctrl Pts',(-1.16220527056132,6.668931489016,116.857580662092));
#38094=CARTESIAN_POINT('Ctrl Pts',(-1.34098602962433,6.63528693847101,116.866123811177));
#38095=CARTESIAN_POINT('Ctrl Pts',(-1.51798141790123,6.59454482242001,116.874666960261));
#38096=CARTESIAN_POINT('Ctrl Pts',(-1.68824379914598,6.55535256004908,116.882885123009));
#38097=CARTESIAN_POINT('Ctrl Pts',(-1.85685381083841,6.50959291716969,116.891103285757));
#38098=CARTESIAN_POINT('Ctrl Pts',(-2.02328052428725,6.45744724485148,116.899321448505));
#38099=CARTESIAN_POINT('Ctrl Pts',(-2.18982705907041,6.40526402949761,116.907545528039));
#38100=CARTESIAN_POINT('Ctrl Pts',(-2.35418682673733,6.34668574115767,116.915769607572));
#38101=CARTESIAN_POINT('Ctrl Pts',(-2.51584920345394,6.28194172095541,116.923993687106));
#38102=CARTESIAN_POINT('Ctrl Pts',(-2.67772702715645,6.21711141658307,116.932228726847));
#38103=CARTESIAN_POINT('Ctrl Pts',(-2.83689995803201,6.14609912122177,116.940463766588));
#38104=CARTESIAN_POINT('Ctrl Pts',(-2.9928815796825,6.06918024530473,116.948698806329));
#38105=CARTESIAN_POINT('Ctrl Pts',(-3.01091674181233,6.06028660525067,116.94965097156));
#38106=CARTESIAN_POINT('Ctrl Pts',(-3.02890927166878,6.0513140488267,116.950603136792));
#38107=CARTESIAN_POINT('Ctrl Pts',(-3.0468584428216,6.04226303874688,116.951555302023));
#38108=CARTESIAN_POINT('Ctrl Pts',(-3.20059617020903,5.96473958608241,116.95971076043));
#38109=CARTESIAN_POINT('Ctrl Pts',(-3.35162399650535,5.88121836395444,116.967866218837));
#38110=CARTESIAN_POINT('Ctrl Pts',(-3.49943530889714,5.79191173265305,116.976021677244));
#38111=CARTESIAN_POINT('Ctrl Pts',(-3.64706671549235,5.70271379926106,116.984167209385));
#38112=CARTESIAN_POINT('Ctrl Pts',(-3.79148909161224,5.60774466026573,116.992312741527));
#38113=CARTESIAN_POINT('Ctrl Pts',(-3.93221707123081,5.50726410341115,117.000458273669));
#38114=CARTESIAN_POINT('Ctrl Pts',(-4.0728033586708,5.40688471555682,117.00859560447));
#38115=CARTESIAN_POINT('Ctrl Pts',(-4.20970235965384,5.30100516807636,117.01673293527));
#38116=CARTESIAN_POINT('Ctrl Pts',(-4.3424545479687,5.1899303944105,117.024870266071));
#38117=CARTESIAN_POINT('Ctrl Pts',(-4.47510097282572,5.07894411384063,117.033001113873));
#38118=CARTESIAN_POINT('Ctrl Pts',(-4.60360688419332,4.96277108186089,117.041131961675));
#38119=CARTESIAN_POINT('Ctrl Pts',(-4.72754293730218,4.84175864495168,117.049262809477));
#38120=CARTESIAN_POINT('Ctrl Pts',(-4.85140628566751,4.72081719770179,117.057388887471));
#38121=CARTESIAN_POINT('Ctrl Pts',(-4.97070485371655,4.59504225393221,117.065514965465));
#38122=CARTESIAN_POINT('Ctrl Pts',(-5.08504352387437,4.46482041747519,117.073641043459));
#38123=CARTESIAN_POINT('Ctrl Pts',(-5.1997876180731,4.33413683817055,117.081795935041));
#38124=CARTESIAN_POINT('Ctrl Pts',(-5.30953629481107,4.1989750158833,117.089950826623));
#38125=CARTESIAN_POINT('Ctrl Pts',(-5.41392822995811,4.05976232319858,117.098105718205));
#38126=CARTESIAN_POINT('Ctrl Pts',(-5.51791307305772,3.92109251134091,117.106228808561));
#38127=CARTESIAN_POINT('Ctrl Pts',(-5.61658267113772,3.77840367128628,117.114351898918));
#38128=CARTESIAN_POINT('Ctrl Pts',(-5.70962111670077,3.63215028650036,117.122474989274));
#38129=CARTESIAN_POINT('Ctrl Pts',(-5.80266686806748,3.48588541723072,117.130598717492));
#38130=CARTESIAN_POINT('Ctrl Pts',(-5.89008038974256,3.33605575433806,117.138722445711));
#38131=CARTESIAN_POINT('Ctrl Pts',(-5.9715899829251,3.18314342683905,117.146846173929));
#38132=CARTESIAN_POINT('Ctrl Pts',(-6.05312148371636,3.03019000057718,117.15497208559));
#38133=CARTESIAN_POINT('Ctrl Pts',(-6.12874572435242,2.87415258262508,117.16309799725));
#38134=CARTESIAN_POINT('Ctrl Pts',(-6.19823772506012,2.71553643018125,117.17122390891));
#38135=CARTESIAN_POINT('Ctrl Pts',(-6.2681741343358,2.55590591095495,117.17940178662));
#38136=CARTESIAN_POINT('Ctrl Pts',(-6.33189944809649,2.39366390423532,117.187579664331));
#38137=CARTESIAN_POINT('Ctrl Pts',(-6.38923443824757,2.22934346683306,117.195757542041));
#38138=CARTESIAN_POINT('Ctrl Pts',(-6.44629578092607,2.06580729523899,117.203896388514));
#38139=CARTESIAN_POINT('Ctrl Pts',(-6.49702761724099,1.90021285710961,117.212035234988));
#38140=CARTESIAN_POINT('Ctrl Pts',(-6.54130415551225,1.73309807716651,117.220174081461));
#38141=CARTESIAN_POINT('Ctrl Pts',(-6.5858991974032,1.56478115576442,117.228371474789));
#38142=CARTESIAN_POINT('Ctrl Pts',(-6.6239456360603,1.39492230552711,117.236568868118));
#38143=CARTESIAN_POINT('Ctrl Pts',(-6.65536785607931,1.22407830642747,117.244766261446));
#38144=CARTESIAN_POINT('Ctrl Pts',(-6.68679007609832,1.05323430732783,117.252963654774));
#38145=CARTESIAN_POINT('Ctrl Pts',(-6.71158808479465,0.881405536510773,
117.261161048103));
#38146=CARTESIAN_POINT('Ctrl Pts',(-6.72973958167842,0.70915031043549,117.269358441431));
#38147=CARTESIAN_POINT('Ctrl Pts',(-6.75443772965151,0.474768259743667,
117.280512366351));
#38148=CARTESIAN_POINT('Ctrl Pts',(-6.76689111546283,0.239107568829402,
117.29166629127));
#38149=CARTESIAN_POINT('Ctrl Pts',(-6.76699928917314,0.00310166572580796,
117.30282021619));
#38150=CARTESIAN_POINT('Ctrl Pts',(-6.76699928917358,0.00310166475299538,
117.302820216236));
#38151=CARTESIAN_POINT('Ctrl Pts',(-6.76707794204855,-0.168497779856733,
117.310930213894));
#38152=CARTESIAN_POINT('Ctrl Pts',(-6.76062520672312,-0.340352238830547,
117.319040211552));
#38153=CARTESIAN_POINT('Ctrl Pts',(-6.74760921640779,-0.5119168513037,117.327150209209));
#38154=CARTESIAN_POINT('Ctrl Pts',(-6.73460661988539,-0.68330491932353,
117.335251861468));
#38155=CARTESIAN_POINT('Ctrl Pts',(-6.71505423919447,-0.854403369158645,
117.343353513727));
#38156=CARTESIAN_POINT('Ctrl Pts',(-6.68897219997428,-1.02466575426877,
117.351455165986));
#38157=CARTESIAN_POINT('Ctrl Pts',(-6.6629113960377,-1.19478951639763,117.359550222101));
#38158=CARTESIAN_POINT('Ctrl Pts',(-6.63033157275093,-1.36407820561675,
117.367645278217));
#38159=CARTESIAN_POINT('Ctrl Pts',(-6.59130478648699,-1.53198897242564,
117.375740334332));
#38160=CARTESIAN_POINT('Ctrl Pts',(-6.55230139537651,-1.6997990827743,117.383830537752));
#38161=CARTESIAN_POINT('Ctrl Pts',(-6.50685881998188,-1.86623255659433,
117.391920741173));
#38162=CARTESIAN_POINT('Ctrl Pts',(-6.45510045951788,-2.03075529238065,
117.400010944593));
#38163=CARTESIAN_POINT('Ctrl Pts',(-6.40335638943706,-2.19523260375799,
117.408098914324));
#38164=CARTESIAN_POINT('Ctrl Pts',(-6.34530011202132,-2.35779987388169,
117.416186884055));
#38165=CARTESIAN_POINT('Ctrl Pts',(-6.28110532062709,-2.51793664558703,
117.424274853786));
#38166=CARTESIAN_POINT('Ctrl Pts',(-6.21691802384008,-2.67805472166022,
117.432361879263));
#38167=CARTESIAN_POINT('Ctrl Pts',(-6.14659377637887,-2.83574252080221,
117.44044890474));
#38168=CARTESIAN_POINT('Ctrl Pts',(-6.07035494762533,-2.99049825444535,
117.448535930218));
#38169=CARTESIAN_POINT('Ctrl Pts',(-5.99411020078692,-3.14526600109525,
117.456623583455));
#38170=CARTESIAN_POINT('Ctrl Pts',(-5.91195012196213,-3.29710089746528,
117.464711236693));
#38171=CARTESIAN_POINT('Ctrl Pts',(-5.82414364746011,-3.44552460065954,
117.472798889931));
#38172=CARTESIAN_POINT('Ctrl Pts',(-5.73631328792009,-3.59398867793568,
117.480888743164));
#38173=CARTESIAN_POINT('Ctrl Pts',(-5.64283366346503,-3.73903939694189,
117.488978596398));
#38174=CARTESIAN_POINT('Ctrl Pts',(-5.54401768793729,-3.88022639492059,
117.497068449632));
#38175=CARTESIAN_POINT('Ctrl Pts',(-5.4451020877245,-4.02155573537107,117.505166458926));
#38176=CARTESIAN_POINT('Ctrl Pts',(-5.34083960372453,-4.15901327203359,
117.51326446822));
#38177=CARTESIAN_POINT('Ctrl Pts',(-5.23158467127832,-4.29218019510431,
117.521362477515));
#38178=CARTESIAN_POINT('Ctrl Pts',(-5.1222704713336,-4.4254193572057,117.529464879734));
#38179=CARTESIAN_POINT('Ctrl Pts',(-5.00795867227044,-4.55436299281459,
117.537567281954));
#38180=CARTESIAN_POINT('Ctrl Pts',(-4.88904112237404,-4.67862863494589,
117.545669684173));
#38181=CARTESIAN_POINT('Ctrl Pts',(-4.76995697730049,-4.80306836455782,
117.553783437292));
#38182=CARTESIAN_POINT('Ctrl Pts',(-4.64625445853697,-4.92281675420357,
117.561897190411));
#38183=CARTESIAN_POINT('Ctrl Pts',(-4.51835980497909,-5.03753051333184,
117.57001094353));
#38184=CARTESIAN_POINT('Ctrl Pts',(-4.42824635666586,-5.11835681933018,
117.575727822633));
#38185=CARTESIAN_POINT('Ctrl Pts',(-4.33605242085457,-5.19668454010475,
117.581444701736));
#38186=CARTESIAN_POINT('Ctrl Pts',(-4.24193560225691,-5.27240659910684,
117.587161580839));
#38187=CARTESIAN_POINT('Ctrl Pts',(-4.10650788809726,-5.38136550267915,
117.595387781858));
#38188=CARTESIAN_POINT('Ctrl Pts',(-3.96669008959762,-5.48525542608483,
117.603613982876));
#38189=CARTESIAN_POINT('Ctrl Pts',(-3.82289739792679,-5.58370347394313,
117.611840183895));
#38190=CARTESIAN_POINT('Ctrl Pts',(-3.67926622703936,-5.68204093616854,
117.620057144511));
#38191=CARTESIAN_POINT('Ctrl Pts',(-3.53166934715663,-5.77494849432802,
117.628274105127));
#38192=CARTESIAN_POINT('Ctrl Pts',(-3.38055564291473,-5.86209284685576,
117.636491065743));
#38193=CARTESIAN_POINT('Ctrl Pts',(-3.22958135334985,-5.94915680163384,
117.644700445544));
#38194=CARTESIAN_POINT('Ctrl Pts',(-3.07509700980742,-6.03046796179911,
117.652909825346));
#38195=CARTESIAN_POINT('Ctrl Pts',(-2.917581228281,-6.10573572768936,117.661119205147));
#38196=CARTESIAN_POINT('Ctrl Pts',(-2.760179163344,-6.18094915493782,117.669322658288));
#38197=CARTESIAN_POINT('Ctrl Pts',(-2.59975034183862,-6.25012772416892,
117.677526111428));
#38198=CARTESIAN_POINT('Ctrl Pts',(-2.43679886133955,-6.31302624019371,
117.685729564568));
#38199=CARTESIAN_POINT('Ctrl Pts',(-2.27393233400521,-6.37589196469076,
117.693928740918));
#38200=CARTESIAN_POINT('Ctrl Pts',(-2.10854610149869,-6.4324840296236,117.702127917269));
#38201=CARTESIAN_POINT('Ctrl Pts',(-1.94116524725917,-6.48260491491139,
117.710327093619));
#38202=CARTESIAN_POINT('Ctrl Pts',(-1.77381588825272,-6.53271636919841,
117.71852472717));
#38203=CARTESIAN_POINT('Ctrl Pts',(-1.60447299653246,-6.57635896053857,
117.726722360721));
#38204=CARTESIAN_POINT('Ctrl Pts',(-1.43367816021121,-6.61338460494575,
117.734919994273));
#38205=CARTESIAN_POINT('Ctrl Pts',(-1.26289562530995,-6.65040758259782,
117.743117037393));
#38206=CARTESIAN_POINT('Ctrl Pts',(-1.09066170442501,-6.68081448560249,
117.751314080514));
#38207=CARTESIAN_POINT('Ctrl Pts',(-0.917529506141373,-6.70450808078863,
117.759511123635));
#38208=CARTESIAN_POINT('Ctrl Pts',(-0.744378311137273,-6.72820427572575,
117.767709066166));
#38209=CARTESIAN_POINT('Ctrl Pts',(-0.570328997811365,-6.74518564666166,
117.775907008697));
#38210=CARTESIAN_POINT('Ctrl Pts',(-0.395941200302829,-6.75540669137712,
117.784104951228));
#38211=CARTESIAN_POINT('Ctrl Pts',(-0.221502573495327,-6.76563071524907,
117.792305283237));
#38212=CARTESIAN_POINT('Ctrl Pts',(-0.0467256239640609,-6.76909046701836,
117.800505615245));
#38213=CARTESIAN_POINT('Ctrl Pts',(0.127828546347631,-6.76579255244636,
117.808705947253));
#38214=CARTESIAN_POINT('Ctrl Pts',(0.302564649283056,-6.76249120055602,
117.816914826224));
#38215=CARTESIAN_POINT('Ctrl Pts',(0.477077150016872,-6.75241811763111,
117.825123705195));
#38216=CARTESIAN_POINT('Ctrl Pts',(0.650807598446602,-6.73563200225518,
117.833332584166));
#38217=CARTESIAN_POINT('Ctrl Pts',(0.824631309410862,-6.71883687570316,
117.841545869853));
#38218=CARTESIAN_POINT('Ctrl Pts',(0.99767177606956,-6.69532158082911,117.84975915554));
#38219=CARTESIAN_POINT('Ctrl Pts',(1.1693793964943,-6.66519623319934,117.857972441228));
#38220=CARTESIAN_POINT('Ctrl Pts',(1.34133820400521,-6.63502681589886,117.86619774194));
#38221=CARTESIAN_POINT('Ctrl Pts',(1.51195991815939,-6.5982280972073,117.874423042652));
#38222=CARTESIAN_POINT('Ctrl Pts',(1.68070753585745,-6.55496080681738,117.882648343364));
#38223=CARTESIAN_POINT('Ctrl Pts',(1.83331940040885,-6.51583076189842,117.890087135658));
#38224=CARTESIAN_POINT('Ctrl Pts',(1.98439845459551,-6.47141076516683,117.897525927952));
#38225=CARTESIAN_POINT('Ctrl Pts',(2.13356148950366,-6.42185365533247,117.904964720246));
#38226=CARTESIAN_POINT('Ctrl Pts',(2.29703695419795,-6.36754146220723,117.913117276459));
#38227=CARTESIAN_POINT('Ctrl Pts',(2.45869289501725,-6.30689806659958,117.921269832673));
#38228=CARTESIAN_POINT('Ctrl Pts',(2.61799751028861,-6.24006234232661,117.929422388886));
#38229=CARTESIAN_POINT('Ctrl Pts',(2.77711756732243,-6.17330404885158,117.937565500166));
#38230=CARTESIAN_POINT('Ctrl Pts',(2.93389138767401,-6.10036784715035,117.945708611447));
#38231=CARTESIAN_POINT('Ctrl Pts',(3.08780156878072,-6.02144255738069,117.953851722727));
#38232=CARTESIAN_POINT('Ctrl Pts',(3.24156579893055,-5.94259211140292,117.961987112004));
#38233=CARTESIAN_POINT('Ctrl Pts',(3.39247147310079,-5.85776404991919,117.970122501282));
#38234=CARTESIAN_POINT('Ctrl Pts',(3.54002045463034,-5.76719552129099,117.978257890559));
#38235=CARTESIAN_POINT('Ctrl Pts',(3.68746052104472,-5.67669384694822,117.986387274597));
#38236=CARTESIAN_POINT('Ctrl Pts',(3.83154851828465,-5.58046033329277,117.994516658636));
#38237=CARTESIAN_POINT('Ctrl Pts',(3.97181025635086,-5.47877835722035,118.002646042675));
#38238=CARTESIAN_POINT('Ctrl Pts',(4.11199792014433,-5.37715008088481,118.010771133467));
#38239=CARTESIAN_POINT('Ctrl Pts',(4.24836305376973,-5.27007928670352,118.018896224259));
#38240=CARTESIAN_POINT('Ctrl Pts',(4.38045986071102,-5.15789302028451,118.027021315051));
#38241=CARTESIAN_POINT('Ctrl Pts',(4.51306090980176,-5.04527851456564,118.035177421076));
#38242=CARTESIAN_POINT('Ctrl Pts',(4.64136066852364,-4.92750960717487,118.043333527101));
#38243=CARTESIAN_POINT('Ctrl Pts',(4.76494082448019,-4.80495868236159,118.051489633126));
#38244=CARTESIAN_POINT('Ctrl Pts',(4.88802359265873,-4.68290100285711,118.0596129123));
#38245=CARTESIAN_POINT('Ctrl Pts',(5.00642443226679,-4.55610000262943,118.067736191473));
#38246=CARTESIAN_POINT('Ctrl Pts',(5.11976644642777,-4.42496107712061,118.075859470647));
#38247=CARTESIAN_POINT('Ctrl Pts',(5.23312355303523,-4.29380468935626,118.083983831503));
#38248=CARTESIAN_POINT('Ctrl Pts',(5.34142025322042,-4.15830950258001,118.09210819236));
#38249=CARTESIAN_POINT('Ctrl Pts',(5.4443195577944,-4.0189144744094,118.100232553217));
#38250=CARTESIAN_POINT('Ctrl Pts',(5.54725214140282,-3.87947436399103,118.108359541602));
#38251=CARTESIAN_POINT('Ctrl Pts',(5.64478363622508,-3.73613219477519,118.116486529987));
#38252=CARTESIAN_POINT('Ctrl Pts',(5.73662007644422,-3.58935636271145,118.124613518373));
#38253=CARTESIAN_POINT('Ctrl Pts',(5.82905022879375,-3.44163164160391,118.132793046813));
#38254=CARTESIAN_POINT('Ctrl Pts',(5.91571123614408,-3.29042902584766,118.140972575253));
#38255=CARTESIAN_POINT('Ctrl Pts',(5.99635052252058,-3.13625085270092,118.149152103693));
#38256=CARTESIAN_POINT('Ctrl Pts',(6.07661005250048,-2.98279875427651,118.157293112097));
#38257=CARTESIAN_POINT('Ctrl Pts',(6.15090435722253,-2.82639942147593,118.165434120501));
#38258=CARTESIAN_POINT('Ctrl Pts',(6.21903309158284,-2.66756750726155,118.173575128904));
#38259=CARTESIAN_POINT('Ctrl Pts',(6.28764536333751,-2.50760829821833,118.181773917362));
#38260=CARTESIAN_POINT('Ctrl Pts',(6.35000408858973,-2.34518220323418,118.189972705821));
#38261=CARTESIAN_POINT('Ctrl Pts',(6.40595601871127,-2.18082931160071,118.198171494279));
#38262=CARTESIAN_POINT('Ctrl Pts',(6.46190794883286,-2.01647641996712,118.206370282737));
#38263=CARTESIAN_POINT('Ctrl Pts',(6.5114530398635,-1.85019710608718,118.214569071196));
#38264=CARTESIAN_POINT('Ctrl Pts',(6.55449059770862,-1.68254034262164,118.222767859654));
#38265=CARTESIAN_POINT('Ctrl Pts',(6.59770800392675,-1.51418296328373,118.231000909786));
#38266=CARTESIAN_POINT('Ctrl Pts',(6.63449783408622,-1.34391328261386,118.239233959918));
#38267=CARTESIAN_POINT('Ctrl Pts',(6.66468970190499,-1.17226284480979,118.24746701005));
#38268=CARTESIAN_POINT('Ctrl Pts',(6.69484561585011,-1.00081681629202,118.255690255885));
#38269=CARTESIAN_POINT('Ctrl Pts',(6.71841915156091,-0.827993654093565,
118.26391350172));
#38270=CARTESIAN_POINT('Ctrl Pts',(6.7352898103742,-0.654339491601587,118.272136747554));
#38271=CARTESIAN_POINT('Ctrl Pts',(6.75214375552496,-0.480857367267884,
118.280351846668));
#38272=CARTESIAN_POINT('Ctrl Pts',(6.76230801402065,-0.306546236240227,
118.288566945781));
#38273=CARTESIAN_POINT('Ctrl Pts',(6.76571319567667,-0.13196194090165,118.296782044895));
#38274=CARTESIAN_POINT('Ctrl Pts',(6.76911568514746,0.0424843256004356,
118.304990649034));
#38275=CARTESIAN_POINT('Ctrl Pts',(6.76576973465029,0.217202969746779,118.313199253173));
#38276=CARTESIAN_POINT('Ctrl Pts',(6.75565779671617,0.391633417455661,118.321407857312));
#38277=CARTESIAN_POINT('Ctrl Pts',(6.74555183075505,0.565960848914752,118.329611613561));
#38278=CARTESIAN_POINT('Ctrl Pts',(6.72868785840712,0.740000066384756,118.337815369809));
#38279=CARTESIAN_POINT('Ctrl Pts',(6.70510041546822,0.913190789751989,118.346019126058));
#38280=CARTESIAN_POINT('Ctrl Pts',(6.68151995145901,1.08633027035064,118.354220455023));
#38281=CARTESIAN_POINT('Ctrl Pts',(6.65122002393255,1.25862140194925,118.362421783987));
#38282=CARTESIAN_POINT('Ctrl Pts',(6.61428702359496,1.42950906590458,118.370623112951));
#38283=CARTESIAN_POINT('Ctrl Pts',(6.57735911667073,1.60037316281947,118.378823310874));
#38284=CARTESIAN_POINT('Ctrl Pts',(6.53380003370326,1.76983382733277,118.387023508797));
#38285=CARTESIAN_POINT('Ctrl Pts',(6.48374728705282,1.93734615328164,118.395223706719));
#38286=CARTESIAN_POINT('Ctrl Pts',(6.43369237257765,2.10486573432414,118.403424259799));
#38287=CARTESIAN_POINT('Ctrl Pts',(6.37714333663196,2.27043646536461,118.411624812879));
#38288=CARTESIAN_POINT('Ctrl Pts',(6.31428758543787,2.43352856740683,118.419825365959));
#38289=CARTESIAN_POINT('Ctrl Pts',(6.25141772121773,2.59665728858164,118.428027760312));
#38290=CARTESIAN_POINT('Ctrl Pts',(6.18223845019751,2.757305938066,118.436230154665));
#38291=CARTESIAN_POINT('Ctrl Pts',(6.10698536066305,2.9149646318004,118.444432549019));
#38292=CARTESIAN_POINT('Ctrl Pts',(6.03166189626131,3.07277076412789,118.452642614053));
#38293=CARTESIAN_POINT('Ctrl Pts',(5.95025341953817,3.22758103050455,118.460852679086));
#38294=CARTESIAN_POINT('Ctrl Pts',(5.86304198135088,3.37890925076675,118.46906274412));
#38295=CARTESIAN_POINT('Ctrl Pts',(5.77578880531617,3.53030989403104,118.477276738346));
#38296=CARTESIAN_POINT('Ctrl Pts',(5.68272732123574,3.67822486547193,118.485490732571));
#38297=CARTESIAN_POINT('Ctrl Pts',(5.58418294253159,3.82219699444433,118.493704726796));
#38298=CARTESIAN_POINT('Ctrl Pts',(5.48550421501832,3.96636540537952,118.501929919431));
#38299=CARTESIAN_POINT('Ctrl Pts',(5.38132786770703,4.10657994334918,118.510155112067));
#38300=CARTESIAN_POINT('Ctrl Pts',(5.27202038230147,4.24241559593092,118.518380304702));
#38301=CARTESIAN_POINT('Ctrl Pts',(5.1737203947933,4.36457230736204,118.525777202822));
#38302=CARTESIAN_POINT('Ctrl Pts',(5.07127131958762,4.48318797613906,118.533174100942));
#38303=CARTESIAN_POINT('Ctrl Pts',(4.96496457235056,4.59797953402403,118.540570999062));
#38304=CARTESIAN_POINT('Ctrl Pts',(4.84067184494065,4.73219261253483,118.549219374312));
#38305=CARTESIAN_POINT('Ctrl Pts',(4.71082313055442,4.86148250034786,118.557867749561));
#38306=CARTESIAN_POINT('Ctrl Pts',(4.5758248450852,4.98539025424299,118.566516124811));
#38307=CARTESIAN_POINT('Ctrl Pts',(4.44106290500398,5.1090810792633,118.575149359102));
#38308=CARTESIAN_POINT('Ctrl Pts',(4.30116960500453,5.2274083646177,118.583782593392));
#38309=CARTESIAN_POINT('Ctrl Pts',(4.15658856369466,5.33994948591864,118.592415827682));
#38310=CARTESIAN_POINT('Ctrl Pts',(4.01216266249406,5.45236984697538,118.601039798234));
#38311=CARTESIAN_POINT('Ctrl Pts',(3.86305928735499,5.55901623499744,118.609663768786));
#38312=CARTESIAN_POINT('Ctrl Pts',(3.70975685993916,5.65950466384951,118.618287739338));
#38313=CARTESIAN_POINT('Ctrl Pts',(3.55665871294202,5.75985918863584,118.626900218172));
#38314=CARTESIAN_POINT('Ctrl Pts',(3.39937293016326,5.85407195712336,118.635512697005));
#38315=CARTESIAN_POINT('Ctrl Pts',(3.23840883319496,5.94180084057728,118.644125175839));
#38316=CARTESIAN_POINT('Ctrl Pts',(3.1922953569385,5.96693367367704,118.646592504552));
#38317=CARTESIAN_POINT('Ctrl Pts',(3.14588018611451,5.99153462166168,118.649059833265));
#38318=CARTESIAN_POINT('Ctrl Pts',(3.09917575053251,6.01559628526643,118.651527161978));
#38319=CARTESIAN_POINT('Origin',(0.,0.,-3.69717978381041));
#38320=CARTESIAN_POINT('',(3.09917575053254,6.01559628526642,121.045781922714));
#38321=CARTESIAN_POINT('',(3.09917575053273,6.01559628526632,120.651392015122));
#38322=CARTESIAN_POINT('',(3.09917575053259,6.01559628526639,-3.69717978381041));
#38323=CARTESIAN_POINT('',(-6.76699734236938,0.00599736322975646,119.69717978384));
#38324=CARTESIAN_POINT('Ctrl Pts',(-6.76699734236938,0.00599736322994578,
119.69717978384));
#38325=CARTESIAN_POINT('Ctrl Pts',(-6.76714983230376,-0.166061413446056,
119.705282912405));
#38326=CARTESIAN_POINT('Ctrl Pts',(-6.76073597240442,-0.338315227567415,
119.713386040971));
#38327=CARTESIAN_POINT('Ctrl Pts',(-6.74773798144884,-0.510216751697474,
119.721489169537));
#38328=CARTESIAN_POINT('Ctrl Pts',(-6.73474953927967,-0.681991990854606,
119.729586345257));
#38329=CARTESIAN_POINT('Ctrl Pts',(-6.71518662383408,-0.853415088825623,
119.737683520976));
#38330=CARTESIAN_POINT('Ctrl Pts',(-6.6890835203219,-1.02393879609966,119.745780696695));
#38331=CARTESIAN_POINT('Ctrl Pts',(-6.66175525810802,-1.20246609588577,
119.754257916316));
#38332=CARTESIAN_POINT('Ctrl Pts',(-6.6272580405859,-1.38000712446736,119.762735135937));
#38333=CARTESIAN_POINT('Ctrl Pts',(-6.58569224159668,-1.55593916943217,
119.771212355557));
#38334=CARTESIAN_POINT('Ctrl Pts',(-6.54601773545304,-1.72386609898865,
119.779303851693));
#38335=CARTESIAN_POINT('Ctrl Pts',(-6.4999037588229,-1.89032682745913,119.78739534783));
#38336=CARTESIAN_POINT('Ctrl Pts',(-6.44748993765559,-2.05479013620123,
119.795486843966));
#38337=CARTESIAN_POINT('Ctrl Pts',(-6.39507803907303,-2.21924741228552,
119.803578043299));
#38338=CARTESIAN_POINT('Ctrl Pts',(-6.33636686756971,-2.38170706249172,
119.811669242632));
#38339=CARTESIAN_POINT('Ctrl Pts',(-6.27154580749815,-2.54165343515838,
119.819760441965));
#38340=CARTESIAN_POINT('Ctrl Pts',(-6.20671455163083,-2.70162496601509,
119.827852913974));
#38341=CARTESIAN_POINT('Ctrl Pts',(-6.1357716327652,-2.85908209014954,119.835945385983));
#38342=CARTESIAN_POINT('Ctrl Pts',(-6.05895438609993,-3.01352961610807,
119.844037857993));
#38343=CARTESIAN_POINT('Ctrl Pts',(-5.98211015451093,-3.1680313975221,119.852133172784));
#38344=CARTESIAN_POINT('Ctrl Pts',(-5.89938765153777,-3.31952114582841,
119.860228487576));
#38345=CARTESIAN_POINT('Ctrl Pts',(-5.81106986251145,-3.46752881069663,
119.868323802368));
#38346=CARTESIAN_POINT('Ctrl Pts',(-5.72265967848526,-3.61569131603728,
119.876427586197));
#38347=CARTESIAN_POINT('Ctrl Pts',(-5.62864271045665,-3.76036414767746,
119.884531370026));
#38348=CARTESIAN_POINT('Ctrl Pts',(-5.52934532477899,-3.90110616099393,
119.892635153854));
#38349=CARTESIAN_POINT('Ctrl Pts',(-5.42998710218725,-4.04193440326508,
119.90074390266));
#38350=CARTESIAN_POINT('Ctrl Pts',(-5.32534224098506,-4.17882673761837,
119.908852651465));
#38351=CARTESIAN_POINT('Ctrl Pts',(-5.21577671797108,-4.31137590894959,
119.91696140027));
#38352=CARTESIAN_POINT('Ctrl Pts',(-5.1060677038644,-4.44409867161598,119.925080768596));
#38353=CARTESIAN_POINT('Ctrl Pts',(-4.99142540805335,-4.57246664243129,
119.933200136921));
#38354=CARTESIAN_POINT('Ctrl Pts',(-4.87225238205238,-4.69610963730458,
119.941319505246));
#38355=CARTESIAN_POINT('Ctrl Pts',(-4.83353055095133,-4.73628385562368,
119.943957659361));
#38356=CARTESIAN_POINT('Ctrl Pts',(-4.79433065211497,-4.77595955988454,
119.946595813475));
#38357=CARTESIAN_POINT('Ctrl Pts',(-4.75466721334804,-4.81512499217966,
119.94923396759));
#38358=CARTESIAN_POINT('Ctrl Pts',(-4.63212092974246,-4.93613260833156,
119.957384949765));
#38359=CARTESIAN_POINT('Ctrl Pts',(-4.50475960522731,-5.05264900334892,
119.965535931939));
#38360=CARTESIAN_POINT('Ctrl Pts',(-4.37294796614193,-5.16426326647036,
119.973686914113));
#38361=CARTESIAN_POINT('Ctrl Pts',(-4.24128943849203,-5.27574787928046,
119.981828428166));
#38362=CARTESIAN_POINT('Ctrl Pts',(-4.10519116268699,-5.38234146119476,
119.989969942219));
#38363=CARTESIAN_POINT('Ctrl Pts',(-3.96505585930834,-5.48366857428169,
119.998111456272));
#38364=CARTESIAN_POINT('Ctrl Pts',(-3.82505384646506,-5.5848993094765,120.006245226475));
#38365=CARTESIAN_POINT('Ctrl Pts',(-3.6810227449162,-5.68087333568657,120.014378996678));
#38366=CARTESIAN_POINT('Ctrl Pts',(-3.53339961980484,-5.77125429406494,
120.022512766881));
#38367=CARTESIAN_POINT('Ctrl Pts',(-3.38588585913341,-5.86156829502803,
120.030640511299));
#38368=CARTESIAN_POINT('Ctrl Pts',(-3.2347856841373,-5.94629728845039,120.038768255717));
#38369=CARTESIAN_POINT('Ctrl Pts',(-3.08056650962285,-6.02514721644128,
120.046896000135));
#38370=CARTESIAN_POINT('Ctrl Pts',(-2.92642916271588,-6.1039553072159,120.055019432029));
#38371=CARTESIAN_POINT('Ctrl Pts',(-2.76917643698794,-6.17689037877921,
120.063142863923));
#38372=CARTESIAN_POINT('Ctrl Pts',(-2.60930179761763,-6.24370347862144,
120.071266295817));
#38373=CARTESIAN_POINT('Ctrl Pts',(-2.44841297641819,-6.31094041448966,
120.079441259568));
#38374=CARTESIAN_POINT('Ctrl Pts',(-2.28486918504337,-6.37197724877038,
120.087616223319));
#38375=CARTESIAN_POINT('Ctrl Pts',(-2.11919581083928,-6.42660860137921,
120.09579118707));
#38376=CARTESIAN_POINT('Ctrl Pts',(-1.95460412294866,-6.48088326428647,
120.103912776243));
#38377=CARTESIAN_POINT('Ctrl Pts',(-1.78791093746152,-6.52883574899776,
120.112034365416));
#38378=CARTESIAN_POINT('Ctrl Pts',(-1.61964834893434,-6.57031416492349,
120.120155954589));
#38379=CARTESIAN_POINT('Ctrl Pts',(-1.45136354629416,-6.61179805685092,
120.128278615978));
#38380=CARTESIAN_POINT('Ctrl Pts',(-1.28150928330525,-6.64680608995604,
120.136401277368));
#38381=CARTESIAN_POINT('Ctrl Pts',(-1.11062945811912,-6.67523716483228,
120.144523938757));
#38382=CARTESIAN_POINT('Ctrl Pts',(-0.93969453271823,-6.70367740731112,
120.152649219299));
#38383=CARTESIAN_POINT('Ctrl Pts',(-0.767733747445996,-6.72553640847876,
120.160774499841));
#38384=CARTESIAN_POINT('Ctrl Pts',(-0.595297713324265,-6.74076476614567,
120.168899780384));
#38385=CARTESIAN_POINT('Ctrl Pts',(-0.420983024390873,-6.75615903360951,
120.177113584172));
#38386=CARTESIAN_POINT('Ctrl Pts',(-0.246183053081737,-6.76477729835143,
120.185327387959));
#38387=CARTESIAN_POINT('Ctrl Pts',(-0.071467321751315,-6.76662260081953,
120.193541191747));
#38388=CARTESIAN_POINT('Ctrl Pts',(0.101664509346737,-6.76845117454211,
120.201680532602));
#38389=CARTESIAN_POINT('Ctrl Pts',(0.274713258622926,-6.76362915725161,
120.209819873457));
#38390=CARTESIAN_POINT('Ctrl Pts',(0.447129601000251,-6.75221179465732,
120.217959214313));
#38391=CARTESIAN_POINT('Ctrl Pts',(0.621911975230568,-6.74063775408689,
120.226210249567));
#38392=CARTESIAN_POINT('Ctrl Pts',(0.79604406955542,-6.7222860837576,120.234461284821));
#38393=CARTESIAN_POINT('Ctrl Pts',(0.968964403150727,-6.69726787469538,
120.242712320075));
#38394=CARTESIAN_POINT('Ctrl Pts',(1.14188473674603,-6.67224966563316,120.250963355329));
#38395=CARTESIAN_POINT('Ctrl Pts',(1.3135929442763,-6.64056505344879,120.259214390583));
#38396=CARTESIAN_POINT('Ctrl Pts',(1.48354396519664,-6.60237732209608,120.267465425837));
#38397=CARTESIAN_POINT('Ctrl Pts',(1.65309821112369,-6.56427874547025,120.275697197868));
#38398=CARTESIAN_POINT('Ctrl Pts',(1.82143282316018,-6.51958861638674,120.283928969899));
#38399=CARTESIAN_POINT('Ctrl Pts',(1.98799707482147,-6.46839675889639,120.29216074193));
#38400=CARTESIAN_POINT('Ctrl Pts',(2.15436243212074,-6.41726602959972,120.300382684402));
#38401=CARTESIAN_POINT('Ctrl Pts',(2.31896129935446,-6.35964913546916,120.308604626875));
#38402=CARTESIAN_POINT('Ctrl Pts',(2.48125262780259,-6.29568696783939,120.316826569347));
#38403=CARTESIAN_POINT('Ctrl Pts',(2.64338268068096,-6.231788362047,120.325040341337));
#38404=CARTESIAN_POINT('Ctrl Pts',(2.80320943040884,-6.16155717072647,120.333254113327));
#38405=CARTESIAN_POINT('Ctrl Pts',(2.96020640973506,-6.08518422167838,120.341467885317));
#38406=CARTESIAN_POINT('Ctrl Pts',(3.11707881900236,-6.00887187113863,120.349675140047));
#38407=CARTESIAN_POINT('Ctrl Pts',(3.27112560925306,-5.9264276252834,120.357882394778));
#38408=CARTESIAN_POINT('Ctrl Pts',(3.42183966365579,-5.83809063960402,120.366089649508));
#38409=CARTESIAN_POINT('Ctrl Pts',(3.57246431127022,-5.74980605730671,120.37429203552));
#38410=CARTESIAN_POINT('Ctrl Pts',(3.71975985325519,-5.65563587973298,120.382494421532));
#38411=CARTESIAN_POINT('Ctrl Pts',(3.86324311071821,-5.55586551920475,120.390696807544));
#38412=CARTESIAN_POINT('Ctrl Pts',(4.00668354190892,-5.45612493770931,120.398896745343));
#38413=CARTESIAN_POINT('Ctrl Pts',(4.14631365914936,-5.35078770397324,120.407096683141));
#38414=CARTESIAN_POINT('Ctrl Pts',(4.28167845510226,-5.24018306999986,120.41529662094));
#38415=CARTESIAN_POINT('Ctrl Pts',(4.41702432356284,-5.12959390140908,120.423495412176));
#38416=CARTESIAN_POINT('Ctrl Pts',(4.54810578057691,-5.01373902552941,120.431694203412));
#38417=CARTESIAN_POINT('Ctrl Pts',(4.67450015677126,-4.89298858412172,120.439892994648));
#38418=CARTESIAN_POINT('Ctrl Pts',(4.80089978836559,-4.77223312198537,120.448092126784));
#38419=CARTESIAN_POINT('Ctrl Pts',(4.92261169164524,-4.64658193634217,120.45629125892));
#38420=CARTESIAN_POINT('Ctrl Pts',(5.03924935587985,-4.51644272954552,120.464490391057));
#38421=CARTESIAN_POINT('Ctrl Pts',(5.15591302843692,-4.38627450379964,120.472691351468));
#38422=CARTESIAN_POINT('Ctrl Pts',(5.26749996920537,-4.25161653054213,120.480892311879));
#38423=CARTESIAN_POINT('Ctrl Pts',(5.37366329560932,-4.11291037896782,120.48909327229));
#38424=CARTESIAN_POINT('Ctrl Pts',(5.47992612260608,-3.97407422633969,120.497301918975));
#38425=CARTESIAN_POINT('Ctrl Pts',(5.58075496111583,-3.83118259998144,120.50551056566));
#38426=CARTESIAN_POINT('Ctrl Pts',(5.67584516562826,-3.68470767576131,120.513719212345));
#38427=CARTESIAN_POINT('Ctrl Pts',(5.77098076887493,-3.53816282029861,120.521931778069));
#38428=CARTESIAN_POINT('Ctrl Pts',(5.86037209218311,-3.388031563803,120.530144343792));
#38429=CARTESIAN_POINT('Ctrl Pts',(5.94376004726729,-3.23481150927055,120.538356909516));
#38430=CARTESIAN_POINT('Ctrl Pts',(6.0272624226589,-3.08138121471329,120.546580744064));
#38431=CARTESIAN_POINT('Ctrl Pts',(6.10474480772534,-2.92485397305057,120.554804578613));
#38432=CARTESIAN_POINT('Ctrl Pts',(6.17599542743257,-2.7657493524056,120.563028413162));
#38433=CARTESIAN_POINT('Ctrl Pts',(6.24146134407012,-2.6195621350229,120.570584570136));
#38434=CARTESIAN_POINT('Ctrl Pts',(6.30166679179529,-2.47119947808256,120.57814072711));
#38435=CARTESIAN_POINT('Ctrl Pts',(6.35648468855408,-2.32107548437736,120.585696884084));
#38436=CARTESIAN_POINT('Ctrl Pts',(6.41920705936011,-2.1493043410682,120.594342602137));
#38437=CARTESIAN_POINT('Ctrl Pts',(6.47501881650106,-1.97483567765751,120.602988320189));
#38438=CARTESIAN_POINT('Ctrl Pts',(6.52369697497116,-1.79823991134447,120.611634038242));
#38439=CARTESIAN_POINT('Ctrl Pts',(6.57231264060621,-1.62187085800584,120.620268656954));
#38440=CARTESIAN_POINT('Ctrl Pts',(6.6138128886129,-1.44338043966331,120.628903275666));
#38441=CARTESIAN_POINT('Ctrl Pts',(6.64802372784018,-1.26335644775096,120.637537894379));
#38442=CARTESIAN_POINT('Ctrl Pts',(6.68344276101051,-1.07697470778149,120.646477454281));
#38443=CARTESIAN_POINT('Ctrl Pts',(6.71104798408059,-0.888949389233346,
120.655417014183));
#38444=CARTESIAN_POINT('Ctrl Pts',(6.73070270760108,-0.69995004242549,120.664356574086));
#38445=CARTESIAN_POINT('Ctrl Pts',(6.74963428938018,-0.517904409142569,
120.672967227356));
#38446=CARTESIAN_POINT('Ctrl Pts',(6.76118988786407,-0.334955483724732,
120.681577880627));
#38447=CARTESIAN_POINT('Ctrl Pts',(6.76529912985488,-0.151712503060123,
120.690188533897));
#38448=CARTESIAN_POINT('Ctrl Pts',(6.76940448217319,0.0313570258617701,
120.698791036608));
#38449=CARTESIAN_POINT('Ctrl Pts',(6.76607752394736,0.214719751179746,120.707393539319));
#38450=CARTESIAN_POINT('Ctrl Pts',(6.75529972530593,0.397762015885989,120.71599604203));
#38451=CARTESIAN_POINT('Ctrl Pts',(6.7445340568598,0.580598270209753,120.724588862798));
#38452=CARTESIAN_POINT('Ctrl Pts',(6.72633429525022,0.763114479634569,120.733181683565));
#38453=CARTESIAN_POINT('Ctrl Pts',(6.70073396604544,0.944697473419382,120.741774504333));
#38454=CARTESIAN_POINT('Ctrl Pts',(6.69771685096488,0.966097854037087,120.742787207291));
#38455=CARTESIAN_POINT('Ctrl Pts',(6.69459700377117,0.987485273873215,120.74379991025));
#38456=CARTESIAN_POINT('Ctrl Pts',(6.69137452704879,1.00885873082541,120.744812613208));
#38457=CARTESIAN_POINT('Ctrl Pts',(6.66402394233424,1.19026470994503,120.753407870968));
#38458=CARTESIAN_POINT('Ctrl Pts',(6.6293082112977,1.37045092087214,120.762003128728));
#38459=CARTESIAN_POINT('Ctrl Pts',(6.58737030967475,1.54881935783862,120.770598386488));
#38460=CARTESIAN_POINT('Ctrl Pts',(6.54539313498565,1.72735482928111,120.779201693343));
#38461=CARTESIAN_POINT('Ctrl Pts',(6.49618035987755,1.90406883172741,120.787805000197));
#38462=CARTESIAN_POINT('Ctrl Pts',(6.43992496467969,2.07837808141235,120.796408307052));
#38463=CARTESIAN_POINT('Ctrl Pts',(6.38133720128924,2.25991425303447,120.805368309992));
#38464=CARTESIAN_POINT('Ctrl Pts',(6.31511052490924,2.43884166052911,120.814328312932));
#38465=CARTESIAN_POINT('Ctrl Pts',(6.24151798084411,2.61452525227807,120.823288315872));
#38466=CARTESIAN_POINT('Ctrl Pts',(6.17066182790065,2.7836764020957,120.831915159076));
#38467=CARTESIAN_POINT('Ctrl Pts',(6.0929778672566,2.94982036745001,120.840542002281));
#38468=CARTESIAN_POINT('Ctrl Pts',(6.00875667309165,3.11241582112297,120.849168845486));
#38469=CARTESIAN_POINT('Ctrl Pts',(5.92445498475476,3.27516667494829,120.857803933772));
#38470=CARTESIAN_POINT('Ctrl Pts',(5.83360373987583,3.43436198114582,120.866439022058));
#38471=CARTESIAN_POINT('Ctrl Pts',(5.73653783237106,3.5894878043776,120.875074110344));
#38472=CARTESIAN_POINT('Ctrl Pts',(5.63932776251445,3.74484402058756,120.883722023469));
#38473=CARTESIAN_POINT('Ctrl Pts',(5.53588475378216,3.89611842165814,120.892369936595));
#38474=CARTESIAN_POINT('Ctrl Pts',(5.426585965883,4.04282744559815,120.90101784972));
#38475=CARTESIAN_POINT('Ctrl Pts',(5.41432430575596,4.05928596470618,120.901988013924));
#38476=CARTESIAN_POINT('Ctrl Pts',(5.4019889884601,4.07568706251909,120.902958178127));
#38477=CARTESIAN_POINT('Ctrl Pts',(5.38958057669206,4.09203008387569,120.903928342331));
#38478=CARTESIAN_POINT('Ctrl Pts',(5.28437976957529,4.23058923790611,120.912153573666));
#38479=CARTESIAN_POINT('Ctrl Pts',(5.17369361909269,4.36527153031135,120.920378805));
#38480=CARTESIAN_POINT('Ctrl Pts',(5.05783804477281,4.4956160103871,120.928604036335));
#38481=CARTESIAN_POINT('Ctrl Pts',(4.94210130662626,4.62582679262985,120.936820830829));
#38482=CARTESIAN_POINT('Ctrl Pts',(4.82120593882783,4.75170835624018,120.945037625322));
#38483=CARTESIAN_POINT('Ctrl Pts',(4.69550995806903,4.87283031037143,120.953254419816));
#38484=CARTESIAN_POINT('Ctrl Pts',(4.56994151436316,4.99382936847227,120.961462877164));
#38485=CARTESIAN_POINT('Ctrl Pts',(4.43958242156076,5.11007819399288,120.969671334512));
#38486=CARTESIAN_POINT('Ctrl Pts',(4.30482944885586,5.22118113229788,120.977879791859));
#38487=CARTESIAN_POINT('Ctrl Pts',(4.17015618308229,5.33221835276307,120.986083393871));
#38488=CARTESIAN_POINT('Ctrl Pts',(4.0310944877603,5.43811551941107,120.994286995883));
#38489=CARTESIAN_POINT('Ctrl Pts',(3.88807664071038,5.53851505694101,121.002490597895));
#38490=CARTESIAN_POINT('Ctrl Pts',(3.74511689813727,5.63887380471834,121.010690866994));
#38491=CARTESIAN_POINT('Ctrl Pts',(3.59820449732004,5.73373916572205,121.018891136093));
#38492=CARTESIAN_POINT('Ctrl Pts',(3.4478033825354,5.82279493330973,121.027091405192));
#38493=CARTESIAN_POINT('Ctrl Pts',(3.33353580435362,5.89045524885949,121.033321577699));
#38494=CARTESIAN_POINT('Ctrl Pts',(3.21725514951042,5.95476294596038,121.039551750207));
#38495=CARTESIAN_POINT('Ctrl Pts',(3.09917575053254,6.01559628526642,121.045781922714));
#38496=CARTESIAN_POINT('Ctrl Pts',(3.09917575053247,6.01559628526645,119.046022396269));
#38497=CARTESIAN_POINT('Ctrl Pts',(2.94562386889167,6.09470469704523,119.054157343536));
#38498=CARTESIAN_POINT('Ctrl Pts',(2.78887073773776,6.16801775510825,119.062292290804));
#38499=CARTESIAN_POINT('Ctrl Pts',(2.62939800615144,6.23526704522323,119.070427238072));
#38500=CARTESIAN_POINT('Ctrl Pts',(2.47004920856827,6.30246407264947,119.078555863277));
#38501=CARTESIAN_POINT('Ctrl Pts',(2.30798535432348,6.36360657381629,119.086684488482));
#38502=CARTESIAN_POINT('Ctrl Pts',(2.14371192052861,6.41847241964812,119.094813113687));
#38503=CARTESIAN_POINT('Ctrl Pts',(1.97953161228569,6.47330716238519,119.102937130827));
#38504=CARTESIAN_POINT('Ctrl Pts',(1.81314456505499,6.52187222037921,119.111061147967));
#38505=CARTESIAN_POINT('Ctrl Pts',(1.64507542085962,6.56399389546361,119.119185165107));
#38506=CARTESIAN_POINT('Ctrl Pts',(1.47704468740609,6.60610594400535,119.127307325573));
#38507=CARTESIAN_POINT('Ctrl Pts',(1.30733297539201,6.64177744705332,119.13542948604));
#38508=CARTESIAN_POINT('Ctrl Pts',(1.13647944425169,6.67088475936988,119.143551646506));
#38509=CARTESIAN_POINT('Ctrl Pts',(0.965641992742876,6.6999893322941,119.151673042567));
#38510=CARTESIAN_POINT('Ctrl Pts',(0.793663296563194,6.72253088196121,119.159794438628));
#38511=CARTESIAN_POINT('Ctrl Pts',(0.621091916664614,6.73843704660464,119.167915834689));
#38512=CARTESIAN_POINT('Ctrl Pts',(0.448503918134599,6.75434474301242,119.176038012841));
#38513=CARTESIAN_POINT('Ctrl Pts',(0.275323486650185,6.76361574810797,119.184160190993));
#38514=CARTESIAN_POINT('Ctrl Pts',(0.102103459539556,6.76622966529736,119.192282369145));
#38515=CARTESIAN_POINT('Ctrl Pts',(-0.0711662339817113,6.76884433196063,
119.200406876123));
#38516=CARTESIAN_POINT('Ctrl Pts',(-0.244475179974578,6.76479810455379,
119.208531383102));
#38517=CARTESIAN_POINT('Ctrl Pts',(-0.417271432542778,6.75412270776773,
119.216655890081));
#38518=CARTESIAN_POINT('Ctrl Pts',(-0.590252249292328,6.74343590855923,
119.224789074869));
#38519=CARTESIAN_POINT('Ctrl Pts',(-0.762718913032112,6.72610581803722,
119.232922259657));
#38520=CARTESIAN_POINT('Ctrl Pts',(-0.934124560177369,6.70221607426032,
119.241055444445));
#38521=CARTESIAN_POINT('Ctrl Pts',(-1.1056239568358,6.67831326410034,119.249193077641));
#38522=CARTESIAN_POINT('Ctrl Pts',(-1.27606082085335,6.64784371569736,119.257330710836));
#38523=CARTESIAN_POINT('Ctrl Pts',(-1.44489964802669,6.61094199090662,119.265468344032));
#38524=CARTESIAN_POINT('Ctrl Pts',(-1.61399553029689,6.57398408368083,119.273618366676));
#38525=CARTESIAN_POINT('Ctrl Pts',(-1.78148816028607,6.53057452402652,119.281768389321));
#38526=CARTESIAN_POINT('Ctrl Pts',(-1.94685714723015,6.48089779646917,119.289918411966));
#38527=CARTESIAN_POINT('Ctrl Pts',(-2.10142186223526,6.43446666461561,119.297535958343));
#38528=CARTESIAN_POINT('Ctrl Pts',(-2.25413131420236,6.38256110597155,119.30515350472));
#38529=CARTESIAN_POINT('Ctrl Pts',(-2.40457833917693,6.32536892289779,119.312771051097));
#38530=CARTESIAN_POINT('Ctrl Pts',(-2.56701999842782,6.26361699981222,119.320995918775));
#38531=CARTESIAN_POINT('Ctrl Pts',(-2.72730940645269,6.19551687046572,119.329220786452));
#38532=CARTESIAN_POINT('Ctrl Pts',(-2.88491503761136,6.12123796513123,119.33744565413));
#38533=CARTESIAN_POINT('Ctrl Pts',(-3.04234310838568,6.04704274329765,119.345661255573));
#38534=CARTESIAN_POINT('Ctrl Pts',(-3.19709310142715,5.96668275832247,119.353876857017));
#38535=CARTESIAN_POINT('Ctrl Pts',(-3.34865059400865,5.88037653549886,119.36209245846));
#38536=CARTESIAN_POINT('Ctrl Pts',(-3.50006779105231,5.79415020564354,119.370300454789));
#38537=CARTESIAN_POINT('Ctrl Pts',(-3.64829806332022,5.70198877645099,119.378508451117));
#38538=CARTESIAN_POINT('Ctrl Pts',(-3.79284877840813,5.60415802276559,119.386716447445));
#38539=CARTESIAN_POINT('Ctrl Pts',(-3.93729471783775,5.50639818039747,119.394918494316));
#38540=CARTESIAN_POINT('Ctrl Pts',(-4.07806611648757,5.40297739882671,119.403120541188));
#38541=CARTESIAN_POINT('Ctrl Pts',(-4.21469661531684,5.29420640330889,119.411322588059));
#38542=CARTESIAN_POINT('Ctrl Pts',(-4.351255515978,5.1854924068073,119.419520336831));
#38543=CARTESIAN_POINT('Ctrl Pts',(-4.48367755967624,5.0714340046226,119.427718085602));
#38544=CARTESIAN_POINT('Ctrl Pts',(-4.61152689545234,4.95238414226116,119.435915834374));
#38545=CARTESIAN_POINT('Ctrl Pts',(-4.7393518465354,4.83335698626992,119.444112019589));
#38546=CARTESIAN_POINT('Ctrl Pts',(-4.86260556037688,4.70934050610102,119.452308204805));
#38547=CARTESIAN_POINT('Ctrl Pts',(-4.9808864818079,4.58072689159082,119.460504390021));
#38548=CARTESIAN_POINT('Ctrl Pts',(-5.0991586530833,4.45212279162556,119.468699968901));
#38549=CARTESIAN_POINT('Ctrl Pts',(-5.21245852102895,4.3189224981175,119.476895547781));
#38550=CARTESIAN_POINT('Ctrl Pts',(-5.32042256883231,4.18155386059534,119.485091126662));
#38551=CARTESIAN_POINT('Ctrl Pts',(-5.42839827247901,4.04417039269816,119.49328759034));
#38552=CARTESIAN_POINT('Ctrl Pts',(-5.53103678652313,3.90261796639809,119.501484054019));
#38553=CARTESIAN_POINT('Ctrl Pts',(-5.6280159196581,3.7573562258688,119.509680517697));
#38554=CARTESIAN_POINT('Ctrl Pts',(-5.72502316697936,3.6120523740574,119.517879357525));
#38555=CARTESIAN_POINT('Ctrl Pts',(-5.81636756623627,3.46303736446124,119.526078197353));
#38556=CARTESIAN_POINT('Ctrl Pts',(-5.90177113624453,3.31079846191081,119.534277037181));
#38557=CARTESIAN_POINT('Ctrl Pts',(-5.98726391271099,3.15840054149617,119.54248444093));
#38558=CARTESIAN_POINT('Ctrl Pts',(-6.0668032866236,3.00277231377503,119.550691844679));
#38559=CARTESIAN_POINT('Ctrl Pts',(-6.14015755615572,2.84442510634114,119.558899248428));
#38560=CARTESIAN_POINT('Ctrl Pts',(-6.21355111811655,2.68599307976314,119.567111048497));
#38561=CARTESIAN_POINT('Ctrl Pts',(-6.28075283303179,2.52483950091763,119.575322848566));
#38562=CARTESIAN_POINT('Ctrl Pts',(-6.34157983285418,2.36149406595426,119.583534648635));
#38563=CARTESIAN_POINT('Ctrl Pts',(-6.40249637851955,2.19790816368667,119.591758537622));
#38564=CARTESIAN_POINT('Ctrl Pts',(-6.45701934238125,2.03212429766803,119.599982426608));
#38565=CARTESIAN_POINT('Ctrl Pts',(-6.50501589122862,1.86468690531767,119.608206315594));
#38566=CARTESIAN_POINT('Ctrl Pts',(-6.54936387260667,1.70997764941767,119.615805046844));
#38567=CARTESIAN_POINT('Ctrl Pts',(-6.58814047872425,1.55385705238916,119.623403778094));
#38568=CARTESIAN_POINT('Ctrl Pts',(-6.6212801170397,1.39676004084263,119.631002509344));
#38569=CARTESIAN_POINT('Ctrl Pts',(-6.67106662401678,1.16074927370662,119.642418273233));
#38570=CARTESIAN_POINT('Ctrl Pts',(-6.7082475624925,0.921995435047206,119.653834037122));
#38571=CARTESIAN_POINT('Ctrl Pts',(-6.73258355588105,0.681621348756109,
119.665249801012));
#38572=CARTESIAN_POINT('Ctrl Pts',(-6.75527287852273,0.457511935530984,
119.675893128611));
#38573=CARTESIAN_POINT('Ctrl Pts',(-6.76679704929885,0.231993769023563,
119.686536456211));
#38574=CARTESIAN_POINT('Ctrl Pts',(-6.76699734236883,0.00599736385734007,
119.69717978381));
#38575=CARTESIAN_POINT('',(-6.76734675747272,0.000426170603140981,119.303420271511));
#38576=CARTESIAN_POINT('Ctrl Pts',(3.09917575053251,6.01559628526643,118.651527161978));
#38577=CARTESIAN_POINT('Ctrl Pts',(2.9364285471412,6.09944203592837,118.660124864592));
#38578=CARTESIAN_POINT('Ctrl Pts',(2.77016691089095,6.17673605197334,118.668722567206));
#38579=CARTESIAN_POINT('Ctrl Pts',(2.60093428501794,6.24719375760175,118.677320269819));
#38580=CARTESIAN_POINT('Ctrl Pts',(2.45558957732084,6.30770605289198,118.684704369468));
#38581=CARTESIAN_POINT('Ctrl Pts',(2.30805396901044,6.36317642841517,118.692088469117));
#38582=CARTESIAN_POINT('Ctrl Pts',(2.15868605499137,6.41345176297334,118.699472568766));
#38583=CARTESIAN_POINT('Ctrl Pts',(1.98480833998704,6.4719767839021,118.708068326314));
#38584=CARTESIAN_POINT('Ctrl Pts',(1.80865124904983,6.52339225558145,118.716664083861));
#38585=CARTESIAN_POINT('Ctrl Pts',(1.63081208939963,6.56755212610209,118.725259841409));
#38586=CARTESIAN_POINT('Ctrl Pts',(1.4528069997693,6.61175319928277,118.73386361909));
#38587=CARTESIAN_POINT('Ctrl Pts',(1.27311700509798,6.6486850851154,118.742467396772));
#38588=CARTESIAN_POINT('Ctrl Pts',(1.09234916559985,6.67825293773853,118.751071174453));
#38589=CARTESIAN_POINT('Ctrl Pts',(0.90447699193578,6.70898283282556,118.760013088121));
#38590=CARTESIAN_POINT('Ctrl Pts',(0.715440913483375,6.73175811563873,118.768955001789));
#38591=CARTESIAN_POINT('Ctrl Pts',(0.525926353928126,6.74653173639937,118.777896915457));
#38592=CARTESIAN_POINT('Ctrl Pts',(0.343081773831211,6.76078539844428,118.786524117788));
#38593=CARTESIAN_POINT('Ctrl Pts',(0.159792117190445,6.76759107506568,118.795151320119));
#38594=CARTESIAN_POINT('Ctrl Pts',(-0.0233282844672006,6.76695978938429,
118.80377852245));
#38595=CARTESIAN_POINT('Ctrl Pts',(-0.206623080280642,6.7663279024999,118.81241394087));
#38596=CARTESIAN_POINT('Ctrl Pts',(-0.389747994752091,6.75824492624368,
118.82104935929));
#38597=CARTESIAN_POINT('Ctrl Pts',(-0.572092798571519,6.74277382312521,
118.829684777711));
#38598=CARTESIAN_POINT('Ctrl Pts',(-0.754706990862874,6.72727986365581,
118.838332953732));
#38599=CARTESIAN_POINT('Ctrl Pts',(-0.936538466375629,6.70437599947752,
118.846981129753));
#38600=CARTESIAN_POINT('Ctrl Pts',(-1.11698469582036,6.6741766675226,118.855629305774));
#38601=CARTESIAN_POINT('Ctrl Pts',(-1.13607522269945,6.67098169270828,118.856544250006));
#38602=CARTESIAN_POINT('Ctrl Pts',(-1.15515025678087,6.66770510744618,118.857459194238));
#38603=CARTESIAN_POINT('Ctrl Pts',(-1.17420909350834,6.66434708015139,118.85837413847));
#38604=CARTESIAN_POINT('Ctrl Pts',(-1.34556144845317,6.63415605154042,118.866600131011));
#38605=CARTESIAN_POINT('Ctrl Pts',(-1.51597355623133,6.59731248824598,118.874826123552));
#38606=CARTESIAN_POINT('Ctrl Pts',(-1.68489097720878,6.55388673955543,118.883052116094));
#38607=CARTESIAN_POINT('Ctrl Pts',(-1.85363131010308,6.51050651714955,118.891269484745));
#38608=CARTESIAN_POINT('Ctrl Pts',(-2.02087973248993,6.46055793941455,118.899486853396));
#38609=CARTESIAN_POINT('Ctrl Pts',(-2.18608979098266,6.40416274197973,118.907704222048));
#38610=CARTESIAN_POINT('Ctrl Pts',(-2.3511597059005,6.3478153831853,118.91591462011));
#38611=CARTESIAN_POINT('Ctrl Pts',(-2.5141943634725,6.28503241105296,118.924125018173));
#38612=CARTESIAN_POINT('Ctrl Pts',(-2.67466023208142,6.21598597512271,118.932335416235));
#38613=CARTESIAN_POINT('Ctrl Pts',(-2.8350220809772,6.14698429756083,118.940540492024));
#38614=CARTESIAN_POINT('Ctrl Pts',(-2.99281812989276,6.07172738493515,118.948745567813));
#38615=CARTESIAN_POINT('Ctrl Pts',(-3.14753258526244,5.99043634677067,118.956950643601));
#38616=CARTESIAN_POINT('Ctrl Pts',(-3.30217769187314,5.90918174626549,118.965152041571));
#38617=CARTESIAN_POINT('Ctrl Pts',(-3.45374364035245,5.82189857511661,118.97335343954));
#38618=CARTESIAN_POINT('Ctrl Pts',(-3.60173702516266,5.72885498171951,118.98155483751));
#38619=CARTESIAN_POINT('Ctrl Pts',(-3.74971881790022,5.63581867627042,118.989755593077));
#38620=CARTESIAN_POINT('Ctrl Pts',(-3.89412829664089,5.53702303048263,118.997956348645));
#38621=CARTESIAN_POINT('Ctrl Pts',(-4.03449864668078,5.43278102539859,119.006157104213));
#38622=CARTESIAN_POINT('Ctrl Pts',(-4.17486828370632,5.32853954981417,119.014357818125));
#38623=CARTESIAN_POINT('Ctrl Pts',(-4.31119854454766,5.21885198284553,119.022558532036));
#38624=CARTESIAN_POINT('Ctrl Pts',(-4.44305359015752,5.10407325525295,119.030759245948));
#38625=CARTESIAN_POINT('Ctrl Pts',(-4.57493186142344,4.98927430991869,119.038961404378));
#38626=CARTESIAN_POINT('Ctrl Pts',(-4.7023330766182,4.86938265257377,119.047163562807));
#38627=CARTESIAN_POINT('Ctrl Pts',(-4.82485629627255,4.7447919575382,119.055365721237));
#38628=CARTESIAN_POINT('Ctrl Pts',(-4.94742330231965,4.62015673725164,119.06357081089));
#38629=CARTESIAN_POINT('Ctrl Pts',(-5.06510858903167,4.49081938935732,119.071775900543));
#38630=CARTESIAN_POINT('Ctrl Pts',(-5.17754970096221,4.35720875034306,119.079980990196));
#38631=CARTESIAN_POINT('Ctrl Pts',(-5.29011926356815,4.22344547697179,119.088195453194));
#38632=CARTESIAN_POINT('Ctrl Pts',(-5.397432451742,4.08539943411786,119.096409916192));
#38633=CARTESIAN_POINT('Ctrl Pts',(-5.49916793506262,3.9435315419024,119.104624379189));
#38634=CARTESIAN_POINT('Ctrl Pts',(-5.60096369344182,3.80157959744446,119.112843708997));
#38635=CARTESIAN_POINT('Ctrl Pts',(-5.6971749625305,3.65580158855592,119.121063038804));
#38636=CARTESIAN_POINT('Ctrl Pts',(-5.78752511743648,3.50668533162613,119.129282368612));
#38637=CARTESIAN_POINT('Ctrl Pts',(-5.87801526442972,3.3573380280969,119.137514433772));
#38638=CARTESIAN_POINT('Ctrl Pts',(-5.96262597540469,3.20464245327407,119.145746498933));
#38639=CARTESIAN_POINT('Ctrl Pts',(-6.04112714443894,3.0491100053496,119.153978564094));
#38640=CARTESIAN_POINT('Ctrl Pts',(-6.11168963186089,2.90930627331108,119.161378135355));
#38641=CARTESIAN_POINT('Ctrl Pts',(-6.17731636364992,2.76721088265161,119.168777706616));
#38642=CARTESIAN_POINT('Ctrl Pts',(-6.23787435940597,2.62320652566006,119.176177277877));
#38643=CARTESIAN_POINT('Ctrl Pts',(-6.31224016700351,2.44636777511126,119.185264023333));
#38644=CARTESIAN_POINT('Ctrl Pts',(-6.3791586711013,2.26618310769137,119.194350768788));
#38645=CARTESIAN_POINT('Ctrl Pts',(-6.4383458134576,2.08326479025903,119.203437514243));
#38646=CARTESIAN_POINT('Ctrl Pts',(-6.49727338773895,1.9011486699533,119.212484409337));
#38647=CARTESIAN_POINT('Ctrl Pts',(-6.54853714765832,1.71632302445248,119.22153130443));
#38648=CARTESIAN_POINT('Ctrl Pts',(-6.59190212197188,1.52941669088011,119.230578199524));
#38649=CARTESIAN_POINT('Ctrl Pts',(-6.63514767601595,1.34302506774115,119.239600180902));
#38650=CARTESIAN_POINT('Ctrl Pts',(-6.67053776868456,1.15456440198809,119.24862216228));
#38651=CARTESIAN_POINT('Ctrl Pts',(-6.69788636448025,0.964679868406895,
119.257644143657));
#38652=CARTESIAN_POINT('Ctrl Pts',(-6.7251110861169,0.775655407755472,119.266625260401));
#38653=CARTESIAN_POINT('Ctrl Pts',(-6.74436689747264,0.585220162905082,
119.275606377145));
#38654=CARTESIAN_POINT('Ctrl Pts',(-6.75551850612324,0.394028823090993,
119.284587493889));
#38655=CARTESIAN_POINT('Ctrl Pts',(-6.76306486476055,0.264648527943292,
119.290665067989));
#38656=CARTESIAN_POINT('Ctrl Pts',(-6.76690105714519,0.134922369537897,
119.29674264209));
#38657=CARTESIAN_POINT('Ctrl Pts',(-6.76699811026943,0.00505723343474368,
119.30282021619));
#38658=CARTESIAN_POINT('Ctrl Pts',(-6.767,6.83169908337797E-12,119.30282021619));
#38659=CARTESIAN_POINT('Ctrl Pts',(-6.76700000000019,-0.186007249408865,
119.311569727996));
#38660=CARTESIAN_POINT('Ctrl Pts',(-6.75932637295476,-0.372014355520747,
119.320319239802));
#38661=CARTESIAN_POINT('Ctrl Pts',(-6.74400518266984,-0.557389537148295,
119.329068751608));
#38662=CARTESIAN_POINT('Ctrl Pts',(-6.72868405709716,-0.74276393580507,
119.337818226458));
#38663=CARTESIAN_POINT('Ctrl Pts',(-6.70571545653074,-0.927506129689138,
119.346567701309));
#38664=CARTESIAN_POINT('Ctrl Pts',(-6.67517739415741,-1.11098863924429,
119.35531717616));
#38665=CARTESIAN_POINT('Ctrl Pts',(-6.64463945823172,-1.29447038906135,
119.364066614782));
#38666=CARTESIAN_POINT('Ctrl Pts',(-6.60653217027236,-1.47669218227865,
119.372816053404));
#38667=CARTESIAN_POINT('Ctrl Pts',(-6.56098496116797,-1.65703510503784,
119.381565492026));
#38668=CARTESIAN_POINT('Ctrl Pts',(-6.51543793687607,-1.83737729603703,
119.390314895146));
#38669=CARTESIAN_POINT('Ctrl Pts',(-6.46245112202733,-2.01584035396754,
119.399064298266));
#38670=CARTESIAN_POINT('Ctrl Pts',(-6.40220448416338,-2.19181813637863,
119.407813701386));
#38671=CARTESIAN_POINT('Ctrl Pts',(-6.34195808575291,-2.36779521935663,
119.416563069732));
#38672=CARTESIAN_POINT('Ctrl Pts',(-6.27445201489348,-2.54128677544547,
119.425312438077));
#38673=CARTESIAN_POINT('Ctrl Pts',(-6.19991555136306,-2.71170355237562,
119.434061806422));
#38674=CARTESIAN_POINT('Ctrl Pts',(-6.12537937789167,-2.88211966612799,
119.442811140719));
#38675=CARTESIAN_POINT('Ctrl Pts',(-6.04381298133752,-3.04946076210177,
119.451560475016));
#38676=CARTESIAN_POINT('Ctrl Pts',(-5.95549339426448,-3.21315848206592,
119.460309809313));
#38677=CARTESIAN_POINT('Ctrl Pts',(-5.8671741435532,-3.37685557859358,119.469059110289));
#38678=CARTESIAN_POINT('Ctrl Pts',(-5.77210188986416,-3.53690907467019,
119.477808411264));
#38679=CARTESIAN_POINT('Ctrl Pts',(-5.67059953467267,-3.692775367846,119.48655771224));
#38680=CARTESIAN_POINT('Ctrl Pts',(-5.56909755761972,-3.84864108035495,
119.495306980621));
#38681=CARTESIAN_POINT('Ctrl Pts',(-5.46116568338284,-4.00031938103988,
119.504056249001));
#38682=CARTESIAN_POINT('Ctrl Pts',(-5.34717048686335,-4.14729511662934,
119.512805517382));
#38683=CARTESIAN_POINT('Ctrl Pts',(-5.23317570555738,-4.29427031687772,
119.521554753895));
#38684=CARTESIAN_POINT('Ctrl Pts',(-5.11311782179025,-4.43654275986877,
119.530303990407));
#38685=CARTESIAN_POINT('Ctrl Pts',(-4.98740459172232,-4.57362924147412,
119.53905322692));
#38686=CARTESIAN_POINT('Ctrl Pts',(-4.86169180911051,-4.71071523514209,
119.547802432291));
#38687=CARTESIAN_POINT('Ctrl Pts',(-4.73032391415654,-4.84261509316307,
119.556551637662));
#38688=CARTESIAN_POINT('Ctrl Pts',(-4.59374707237517,-4.96888084331317,
119.565300843033));
#38689=CARTESIAN_POINT('Ctrl Pts',(-4.45717070537638,-5.09514615452517,
119.57405001799));
#38690=CARTESIAN_POINT('Ctrl Pts',(-4.31538563819758,-5.21577720253427,
119.582799192946));
#38691=CARTESIAN_POINT('Ctrl Pts',(-4.16887341290909,-5.33036429028446,
119.591548367902));
#38692=CARTESIAN_POINT('Ctrl Pts',(-4.02236168477605,-5.44495098920979,
119.60029751317));
#38693=CARTESIAN_POINT('Ctrl Pts',(-3.87112305634711,-5.55349359238569,
119.609046658438));
#38694=CARTESIAN_POINT('Ctrl Pts',(-3.7156711731701,-5.65562346102291,119.617795803706));
#38695=CARTESIAN_POINT('Ctrl Pts',(-3.56021980457576,-5.75775299158599,
119.626544920012));
#38696=CARTESIAN_POINT('Ctrl Pts',(-3.4005554486266,-5.85346967275195,119.635294036318));
#38697=CARTESIAN_POINT('Ctrl Pts',(-3.23722036323671,-5.94244842803415,
119.644043152624));
#38698=CARTESIAN_POINT('Ctrl Pts',(-3.07388580496343,-6.03142689616323,
119.652792240695));
#38699=CARTESIAN_POINT('Ctrl Pts',(-2.90688079258032,-6.11366734484667,
119.661541328766));
#38700=CARTESIAN_POINT('Ctrl Pts',(-2.7367725109497,-6.18889046787145,119.670290416837));
#38701=CARTESIAN_POINT('Ctrl Pts',(-2.56666476417012,-6.2641133543812,119.679039477399));
#38702=CARTESIAN_POINT('Ctrl Pts',(-2.39345402972472,-6.33231884350147,
119.687788537962));
#38703=CARTESIAN_POINT('Ctrl Pts',(-2.21772856474429,-6.39327529620908,
119.696537598524));
#38704=CARTESIAN_POINT('Ctrl Pts',(-2.04200363768658,-6.45423156231959,
119.705286632304));
#38705=CARTESIAN_POINT('Ctrl Pts',(-1.86376426620479,-6.50793874251945,
119.714035666084));
#38706=CARTESIAN_POINT('Ctrl Pts',(-1.68361578195071,-6.55421443796024,
119.722784699864));
#38707=CARTESIAN_POINT('Ctrl Pts',(-1.50346783420238,-6.60048999558596,
119.731533707588));
#38708=CARTESIAN_POINT('Ctrl Pts',(-1.32141106257604,-6.63933404145425,
119.740282715312));
#38709=CARTESIAN_POINT('Ctrl Pts',(-1.13806375959388,-6.67061465526971,
119.749031723037));
#38710=CARTESIAN_POINT('Ctrl Pts',(-0.954716987422261,-6.70189517852437,
119.757780705431));
#38711=CARTESIAN_POINT('Ctrl Pts',(-0.770079973812654,-6.72561226535797,
119.766529687826));
#38712=CARTESIAN_POINT('Ctrl Pts',(-0.584779770554896,-6.74168536939761,
119.775278670221));
#38713=CARTESIAN_POINT('Ctrl Pts',(-0.391490647556318,-6.7584514394238,
119.784404850897));
#38714=CARTESIAN_POINT('Ctrl Pts',(-0.197480213106707,-6.7668997592402,
119.793531031573));
#38715=CARTESIAN_POINT('Ctrl Pts',(-0.00346532630012875,-6.76699911271707,
119.802657212249));
#38716=CARTESIAN_POINT('Ctrl Pts',(0.184486595293712,-6.7670953613978,119.811498199779));
#38717=CARTESIAN_POINT('Ctrl Pts',(0.372442378182879,-6.75935659726783,
119.820339187309));
#38718=CARTESIAN_POINT('Ctrl Pts',(0.55975021771973,-6.74380965729036,119.829180174839));
#38719=CARTESIAN_POINT('Ctrl Pts',(0.745129914455429,-6.72842275717279,
119.837930153437));
#38720=CARTESIAN_POINT('Ctrl Pts',(0.929874656311892,-6.70538772273505,
119.846680132035));
#38721=CARTESIAN_POINT('Ctrl Pts',(1.11335688289552,-6.6747828018078,119.855430110633));
#38722=CARTESIAN_POINT('Ctrl Pts',(1.29683723118622,-6.64417819418069,119.864179999657));
#38723=CARTESIAN_POINT('Ctrl Pts',(1.47905480729991,-6.60600390230129,119.872929888682));
#38724=CARTESIAN_POINT('Ctrl Pts',(1.65939064804556,-6.56038959797198,119.881679777707));
#38725=CARTESIAN_POINT('Ctrl Pts',(1.8397247026401,-6.51477574543328,119.890429580068));
#38726=CARTESIAN_POINT('Ctrl Pts',(2.0181767812559,-6.4617220982018,119.899179382429));
#38727=CARTESIAN_POINT('Ctrl Pts',(2.1941407234742,-6.40140886724103,119.90792918479));
#38728=CARTESIAN_POINT('Ctrl Pts',(2.37010298131849,-6.34109621361467,119.916678903396));
#38729=CARTESIAN_POINT('Ctrl Pts',(2.54357687926678,-6.27352420826067,119.925428622001));
#38730=CARTESIAN_POINT('Ctrl Pts',(2.71397317789748,-6.19892237325594,119.934178340607));
#38731=CARTESIAN_POINT('Ctrl Pts',(2.88436790206976,-6.12432122757069,119.942927978365));
#38732=CARTESIAN_POINT('Ctrl Pts',(3.0516848212603,-6.04269049717531,119.951677616123));
#38733=CARTESIAN_POINT('Ctrl Pts',(3.21535561997161,-5.95430745235052,119.960427253881));
#38734=CARTESIAN_POINT('Ctrl Pts',(3.37902496075058,-5.86592519481645,119.9691768137));
#38735=CARTESIAN_POINT('Ctrl Pts',(3.53904799384657,-5.77079087940366,119.977926373519));
#38736=CARTESIAN_POINT('Ctrl Pts',(3.69488118814771,-5.66922763747163,119.986675933338));
#38737=CARTESIAN_POINT('Ctrl Pts',(3.85071304610618,-5.56766526649201,119.995425418126));
#38738=CARTESIAN_POINT('Ctrl Pts',(4.0023548970575,-5.45967423580873,120.004174902913));
#38739=CARTESIAN_POINT('Ctrl Pts',(4.14929168607435,-5.34562133936498,120.012924387701));
#38740=CARTESIAN_POINT('Ctrl Pts',(4.29622726385545,-5.23156938308705,120.021673800364));
#38741=CARTESIAN_POINT('Ctrl Pts',(4.43845763091862,-5.1114558367738,120.030423213027));
#38742=CARTESIAN_POINT('Ctrl Pts',(4.57549970660765,-4.98568866204393,120.039172625691));
#38743=CARTESIAN_POINT('Ctrl Pts',(4.71254069815098,-4.85992248226352,120.047921969137));
#38744=CARTESIAN_POINT('Ctrl Pts',(4.84439326931117,-4.72850295734203,120.056671312583));
#38745=CARTESIAN_POINT('Ctrl Pts',(4.97060959434503,-4.59187644221893,120.06542065603));
#38746=CARTESIAN_POINT('Ctrl Pts',(5.09682496280324,-4.45525096256883,120.074169933166));
#38747=CARTESIAN_POINT('Ctrl Pts',(5.21740397615652,-4.31341878218552,120.082919210302));
#38748=CARTESIAN_POINT('Ctrl Pts',(5.33193710451751,-4.16686161438911,120.091668487439));
#38749=CARTESIAN_POINT('Ctrl Pts',(5.44646940289213,-4.02030550864745,120.100417701171));
#38750=CARTESIAN_POINT('Ctrl Pts',(5.55495572749507,-3.86902470980361,120.109166914904));
#38751=CARTESIAN_POINT('Ctrl Pts',(5.65702762491309,-3.71353301466005,120.117916128637));
#38752=CARTESIAN_POINT('Ctrl Pts',(5.75909881655017,-3.55804239467115,120.126665281874));
#38753=CARTESIAN_POINT('Ctrl Pts',(5.85475551250654,-3.39834117619774,120.13541443511));
#38754=CARTESIAN_POINT('Ctrl Pts',(5.94367283727975,-3.23497174692189,120.144163588346));
#38755=CARTESIAN_POINT('Ctrl Pts',(6.03258957676195,-3.07160339301194,120.152912683991));
#38756=CARTESIAN_POINT('Ctrl Pts',(6.11476689685172,-2.90456712829741,120.161661779637));
#38757=CARTESIAN_POINT('Ctrl Pts',(6.18992570525153,-2.7344302447615,120.170410875282));
#38758=CARTESIAN_POINT('Ctrl Pts',(6.26508404388595,-2.56429442463281,120.179159916243));
#38759=CARTESIAN_POINT('Ctrl Pts',(6.33322384283218,-2.3910582865625,120.187908957204));
#38760=CARTESIAN_POINT('Ctrl Pts',(6.39411368719942,-2.21531017132344,120.196657998165));
#38761=CARTESIAN_POINT('Ctrl Pts',(6.45500317120806,-2.03956309619781,120.205406987348));
#38762=CARTESIAN_POINT('Ctrl Pts',(6.50864269269996,-1.86130434438902,120.21415597653));
#38763=CARTESIAN_POINT('Ctrl Pts',(6.55485008446264,-1.68113930720216,120.222904965713));
#38764=CARTESIAN_POINT('Ctrl Pts',(6.60199664749344,-1.49731239212105,120.231831779242));
#38765=CARTESIAN_POINT('Ctrl Pts',(6.64140563640856,-1.3115011649993,120.240758592771));
#38766=CARTESIAN_POINT('Ctrl Pts',(6.6729377228213,-1.12436255155912,120.249685406301));
#38767=CARTESIAN_POINT('Ctrl Pts',(6.70384494949835,-0.940932395053909,
120.258435320456));
#38768=CARTESIAN_POINT('Ctrl Pts',(6.72718449348901,-0.756227260509322,
120.267185234612));
#38769=CARTESIAN_POINT('Ctrl Pts',(6.7428770737391,-0.570874564544338,120.275935148767));
#38770=CARTESIAN_POINT('Ctrl Pts',(6.75856934538655,-0.385525513635181,
120.284684890851));
#38771=CARTESIAN_POINT('Ctrl Pts',(6.76661493004095,-0.199529212420992,
120.293434632935));
#38772=CARTESIAN_POINT('Ctrl Pts',(6.76698649908906,-0.013517438603244,
120.302184375019));
#38773=CARTESIAN_POINT('Ctrl Pts',(6.76735806132397,0.172490924442939,120.310933956665));
#38774=CARTESIAN_POINT('Ctrl Pts',(6.76005588896304,0.358514472898549,120.319683538311));
#38775=CARTESIAN_POINT('Ctrl Pts',(6.74510478454608,0.543921359659338,120.328433119957));
#38776=CARTESIAN_POINT('Ctrl Pts',(6.73015393440718,0.729325093147661,120.337182552796));
#38777=CARTESIAN_POINT('Ctrl Pts',(6.70755443556934,0.91411190025366,120.345931985635));
#38778=CARTESIAN_POINT('Ctrl Pts',(6.67738304682361,1.09765415591278,120.354681418474));
#38779=CARTESIAN_POINT('Ctrl Pts',(6.64721213111908,1.28119353391025,120.363430714135));
#38780=CARTESIAN_POINT('Ctrl Pts',(6.60946960955547,1.46348811672417,120.372180009797));
#38781=CARTESIAN_POINT('Ctrl Pts',(6.56428366991239,1.64391876347998,120.380929305458));
#38782=CARTESIAN_POINT('Ctrl Pts',(6.5190983786778,1.82434682109494,120.389678475569));
#38783=CARTESIAN_POINT('Ctrl Pts',(6.46646995271989,2.00291071820225,120.39842764568));
#38784=CARTESIAN_POINT('Ctrl Pts',(6.40657713281623,2.17900400212486,120.407176815791));
#38785=CARTESIAN_POINT('Ctrl Pts',(6.34668509279139,2.35509499309444,120.415925871976));
#38786=CARTESIAN_POINT('Ctrl Pts',(6.2795289403761,2.52871516397912,120.424674928162));
#38787=CARTESIAN_POINT('Ctrl Pts',(6.20533675061536,2.69927486771214,120.433423984348));
#38788=CARTESIAN_POINT('Ctrl Pts',(6.1283211790801,2.87632521635724,120.44250598563));
#38789=CARTESIAN_POINT('Ctrl Pts',(6.04372366626177,3.05007728919804,120.451587986912));
#38790=CARTESIAN_POINT('Ctrl Pts',(5.95185378007969,3.21989527478009,120.460669988195));
#38791=CARTESIAN_POINT('Ctrl Pts',(5.86334450817478,3.38350129286567,120.469419768502));
#38792=CARTESIAN_POINT('Ctrl Pts',(5.76808562057368,3.54345567124778,120.478169548809));
#38793=CARTESIAN_POINT('Ctrl Pts',(5.66640068804603,3.69921508465127,120.486919329116));
#38794=CARTESIAN_POINT('Ctrl Pts',(5.56471941108049,3.85496889852101,120.49566879487));
#38795=CARTESIAN_POINT('Ctrl Pts',(5.45661270815247,4.00652780919455,120.504418260623));
#38796=CARTESIAN_POINT('Ctrl Pts',(5.34244776449255,4.15337704569048,120.513167726377));
#38797=CARTESIAN_POINT('Ctrl Pts',(5.2282863181974,4.30022178356074,120.521916924096));
#38798=CARTESIAN_POINT('Ctrl Pts',(5.10806717844218,4.44235690972508,120.530666121816));
#38799=CARTESIAN_POINT('Ctrl Pts',(4.98219864544872,4.57929969070479,120.539415319535));
#38800=CARTESIAN_POINT('Ctrl Pts',(4.85633329944181,4.7162390042984,120.548164295726));
#38801=CARTESIAN_POINT('Ctrl Pts',(4.72481904033808,4.84798602483461,120.556913271916));
#38802=CARTESIAN_POINT('Ctrl Pts',(4.58810250737362,4.97409332258975,120.565662248106));
#38803=CARTESIAN_POINT('Ctrl Pts',(4.45137708685812,5.10020881821987,120.574411793042));
#38804=CARTESIAN_POINT('Ctrl Pts',(4.30944892636227,5.22068366307788,120.583161337978));
#38805=CARTESIAN_POINT('Ctrl Pts',(4.16280009466842,5.33510865604709,120.591910882915));
#38806=CARTESIAN_POINT('Ctrl Pts',(4.01615988348969,5.44952692272759,120.600659913523));
#38807=CARTESIAN_POINT('Ctrl Pts',(3.86479978232409,5.55789587288503,120.609408944131));
#38808=CARTESIAN_POINT('Ctrl Pts',(3.70923383581243,5.65984746713763,120.618157974739));
#38809=CARTESIAN_POINT('Ctrl Pts',(3.55366577799719,5.76180044505272,120.626907124087));
#38810=CARTESIAN_POINT('Ctrl Pts',(3.39389200027023,5.85733573570953,120.635656273435));
#38811=CARTESIAN_POINT('Ctrl Pts',(3.23045513626227,5.94612887621827,120.644405422784));
#38812=CARTESIAN_POINT('Ctrl Pts',(3.18695122151708,5.9697639920662,120.646734286897));
#38813=CARTESIAN_POINT('Ctrl Pts',(3.14318791262736,5.99292165435295,120.649063151009));
#38814=CARTESIAN_POINT('Ctrl Pts',(3.09917575053273,6.01559628526632,120.651392015122));
#38815=CARTESIAN_POINT('Origin',(0.,0.,-3.69717978381041));
#38816=CARTESIAN_POINT('',(3.09917575053267,6.01559628526635,123.045751582742));
#38817=CARTESIAN_POINT('',(3.0991757505325,6.01559628526643,122.651206263353));
#38818=CARTESIAN_POINT('',(3.09917575053259,6.01559628526639,-3.69717978381041));
#38819=CARTESIAN_POINT('',(-6.767,6.76859095031027E-12,121.69717978381));
#38820=CARTESIAN_POINT('Ctrl Pts',(-6.767,6.7685908980338E-12,121.69717978381));
#38821=CARTESIAN_POINT('Ctrl Pts',(-6.76700000000019,-0.186007249408928,
121.705929295616));
#38822=CARTESIAN_POINT('Ctrl Pts',(-6.75932637295475,-0.372014355520807,
121.714678807422));
#38823=CARTESIAN_POINT('Ctrl Pts',(-6.74400518266983,-0.557389537148355,
121.723428319228));
#38824=CARTESIAN_POINT('Ctrl Pts',(-6.72868405709718,-0.742763935804875,
121.732177794078));
#38825=CARTESIAN_POINT('Ctrl Pts',(-6.70571545653079,-0.927506129688694,
121.740927268929));
#38826=CARTESIAN_POINT('Ctrl Pts',(-6.67517739415753,-1.1109886392436,121.74967674378));
#38827=CARTESIAN_POINT('Ctrl Pts',(-6.64463945823183,-1.29447038906078,
121.758426182402));
#38828=CARTESIAN_POINT('Ctrl Pts',(-6.60653217027247,-1.47669218227821,
121.767175621024));
#38829=CARTESIAN_POINT('Ctrl Pts',(-6.56098496116805,-1.65703510503753,
121.775925059646));
#38830=CARTESIAN_POINT('Ctrl Pts',(-6.51543793687619,-1.83737729603659,
121.784674462766));
#38831=CARTESIAN_POINT('Ctrl Pts',(-6.4624511220275,-2.01584035396699,121.793423865886));
#38832=CARTESIAN_POINT('Ctrl Pts',(-6.40220448416361,-2.19181813637796,
121.802173269006));
#38833=CARTESIAN_POINT('Ctrl Pts',(-6.34195808575316,-2.36779521935597,
121.810922637351));
#38834=CARTESIAN_POINT('Ctrl Pts',(-6.27445201489374,-2.54128677544482,
121.819672005697));
#38835=CARTESIAN_POINT('Ctrl Pts',(-6.19991555136334,-2.71170355237498,
121.828421374042));
#38836=CARTESIAN_POINT('Ctrl Pts',(-6.12537937789192,-2.88211966612747,
121.837170708339));
#38837=CARTESIAN_POINT('Ctrl Pts',(-6.04381298133772,-3.04946076210137,
121.845920042636));
#38838=CARTESIAN_POINT('Ctrl Pts',(-5.95549339426463,-3.21315848206564,
121.854669376933));
#38839=CARTESIAN_POINT('Ctrl Pts',(-5.8671741435533,-3.37685557859342,121.863418677909));
#38840=CARTESIAN_POINT('Ctrl Pts',(-5.7721018898642,-3.53690907467014,121.872167978884));
#38841=CARTESIAN_POINT('Ctrl Pts',(-5.67059953467263,-3.69277536784605,
121.88091727986));
#38842=CARTESIAN_POINT('Ctrl Pts',(-5.56909755761975,-3.84864108035489,
121.889666548241));
#38843=CARTESIAN_POINT('Ctrl Pts',(-5.46116568338295,-4.00031938103972,
121.898415816621));
#38844=CARTESIAN_POINT('Ctrl Pts',(-5.34717048686355,-4.14729511662908,
121.907165085002));
#38845=CARTESIAN_POINT('Ctrl Pts',(-5.23317570555759,-4.29427031687747,
121.915914321515));
#38846=CARTESIAN_POINT('Ctrl Pts',(-5.11311782179046,-4.43654275986852,
121.924663558027));
#38847=CARTESIAN_POINT('Ctrl Pts',(-4.98740459172254,-4.57362924147388,
121.93341279454));
#38848=CARTESIAN_POINT('Ctrl Pts',(-4.8616918091109,-4.71071523514167,121.942161999911));
#38849=CARTESIAN_POINT('Ctrl Pts',(-4.73032391415713,-4.84261509316248,
121.950911205282));
#38850=CARTESIAN_POINT('Ctrl Pts',(-4.59374707237597,-4.96888084331243,
121.959660410653));
#38851=CARTESIAN_POINT('Ctrl Pts',(-4.4571707053772,-5.09514615452446,121.96840958561));
#38852=CARTESIAN_POINT('Ctrl Pts',(-4.31538563819842,-5.21577720253357,
121.977158760566));
#38853=CARTESIAN_POINT('Ctrl Pts',(-4.16887341290995,-5.33036429028378,
121.985907935522));
#38854=CARTESIAN_POINT('Ctrl Pts',(-4.02236168477693,-5.44495098920914,
121.99465708079));
#38855=CARTESIAN_POINT('Ctrl Pts',(-3.87112305634801,-5.55349359238507,
122.003406226058));
#38856=CARTESIAN_POINT('Ctrl Pts',(-3.71567117317101,-5.65562346102231,
122.012155371326));
#38857=CARTESIAN_POINT('Ctrl Pts',(-3.56021980457712,-5.75775299158514,
122.020904487632));
#38858=CARTESIAN_POINT('Ctrl Pts',(-3.40055544862842,-5.85346967275088,
122.029653603938));
#38859=CARTESIAN_POINT('Ctrl Pts',(-3.23722036323902,-5.9424484280329,122.038402720244));
#38860=CARTESIAN_POINT('Ctrl Pts',(-3.07388580496566,-6.0314268961621,122.047151808315));
#38861=CARTESIAN_POINT('Ctrl Pts',(-2.90688079258247,-6.11366734484565,
122.055900896386));
#38862=CARTESIAN_POINT('Ctrl Pts',(-2.73677251095175,-6.18889046787054,
122.064649984457));
#38863=CARTESIAN_POINT('Ctrl Pts',(-2.56666476417232,-6.26411335438029,
122.073399045019));
#38864=CARTESIAN_POINT('Ctrl Pts',(-2.39345402972706,-6.33231884350058,
122.082148105581));
#38865=CARTESIAN_POINT('Ctrl Pts',(-2.21772856474678,-6.39327529620821,
122.090897166144));
#38866=CARTESIAN_POINT('Ctrl Pts',(-2.04200363768909,-6.45423156231879,
122.099646199924));
#38867=CARTESIAN_POINT('Ctrl Pts',(-1.86376426620732,-6.50793874251873,
122.108395233704));
#38868=CARTESIAN_POINT('Ctrl Pts',(-1.68361578195325,-6.55421443795959,
122.117144267484));
#38869=CARTESIAN_POINT('Ctrl Pts',(-1.50346783420507,-6.60048999558534,
122.125893275208));
#38870=CARTESIAN_POINT('Ctrl Pts',(-1.32141106257887,-6.63933404145368,
122.134642282932));
#38871=CARTESIAN_POINT('Ctrl Pts',(-1.13806375959685,-6.67061465526921,
122.143391290656));
#38872=CARTESIAN_POINT('Ctrl Pts',(-0.954716987425374,-6.70189517852392,
122.152140273051));
#38873=CARTESIAN_POINT('Ctrl Pts',(-0.770079973815904,-6.72561226535759,
122.160889255446));
#38874=CARTESIAN_POINT('Ctrl Pts',(-0.584779770558282,-6.74168536939732,
122.169638237841));
#38875=CARTESIAN_POINT('Ctrl Pts',(-0.391490647559712,-6.7584514394236,
122.178764418517));
#38876=CARTESIAN_POINT('Ctrl Pts',(-0.197480213110103,-6.7668997592401,
122.187890599193));
#38877=CARTESIAN_POINT('Ctrl Pts',(-0.00346532630352457,-6.76699911271707,
122.197016779869));
#38878=CARTESIAN_POINT('Ctrl Pts',(0.184486595290316,-6.76709536139789,
122.205857767399));
#38879=CARTESIAN_POINT('Ctrl Pts',(0.372442378179485,-6.75935659726802,
122.214698754929));
#38880=CARTESIAN_POINT('Ctrl Pts',(0.559750217716344,-6.74380965729064,
122.223539742459));
#38881=CARTESIAN_POINT('Ctrl Pts',(0.745129914452052,-6.72842275717317,
122.232289721057));
#38882=CARTESIAN_POINT('Ctrl Pts',(0.929874656308528,-6.70538772273551,
122.241039699655));
#38883=CARTESIAN_POINT('Ctrl Pts',(1.11335688289217,-6.67478280180836,122.249789678252));
#38884=CARTESIAN_POINT('Ctrl Pts',(1.29683723118301,-6.64417819418132,122.258539567277));
#38885=CARTESIAN_POINT('Ctrl Pts',(1.47905480729685,-6.60600390230198,122.267289456302));
#38886=CARTESIAN_POINT('Ctrl Pts',(1.65939064804263,-6.56038959797272,122.276039345327));
#38887=CARTESIAN_POINT('Ctrl Pts',(1.83972470263732,-6.51477574543407,122.284789147688));
#38888=CARTESIAN_POINT('Ctrl Pts',(2.01817678125327,-6.46172209820263,122.293538950049));
#38889=CARTESIAN_POINT('Ctrl Pts',(2.19414072347171,-6.40140886724189,122.30228875241));
#38890=CARTESIAN_POINT('Ctrl Pts',(2.37010298131591,-6.34109621361563,122.311038471016));
#38891=CARTESIAN_POINT('Ctrl Pts',(2.5435768792641,-6.27352420826175,122.319788189621));
#38892=CARTESIAN_POINT('Ctrl Pts',(2.71397317789472,-6.19892237325715,122.328537908226));
#38893=CARTESIAN_POINT('Ctrl Pts',(2.88436790206703,-6.12432122757198,122.337287545985));
#38894=CARTESIAN_POINT('Ctrl Pts',(3.05168482125761,-6.04269049717667,122.346037183743));
#38895=CARTESIAN_POINT('Ctrl Pts',(3.21535561996896,-5.95430745235196,122.354786821501));
#38896=CARTESIAN_POINT('Ctrl Pts',(3.37902496074785,-5.86592519481802,122.36353638132));
#38897=CARTESIAN_POINT('Ctrl Pts',(3.53904799384378,-5.77079087940536,122.372285941139));
#38898=CARTESIAN_POINT('Ctrl Pts',(3.69488118814487,-5.66922763747348,122.381035500958));
#38899=CARTESIAN_POINT('Ctrl Pts',(3.85071304610349,-5.56766526649387,122.389784985746));
#38900=CARTESIAN_POINT('Ctrl Pts',(4.00235489705497,-5.45967423581059,122.398534470533));
#38901=CARTESIAN_POINT('Ctrl Pts',(4.14929168607197,-5.34562133936683,122.407283955321));
#38902=CARTESIAN_POINT('Ctrl Pts',(4.29622726385302,-5.23156938308904,122.416033367984));
#38903=CARTESIAN_POINT('Ctrl Pts',(4.43845763091615,-5.11145583677594,122.424782780647));
#38904=CARTESIAN_POINT('Ctrl Pts',(4.57549970660514,-4.98568866204622,122.43353219331));
#38905=CARTESIAN_POINT('Ctrl Pts',(4.71254069814863,-4.8599224822658,122.442281536757));
#38906=CARTESIAN_POINT('Ctrl Pts',(4.84439326930898,-4.72850295734428,122.451030880203));
#38907=CARTESIAN_POINT('Ctrl Pts',(4.97060959434299,-4.59187644222114,122.459780223649));
#38908=CARTESIAN_POINT('Ctrl Pts',(5.09682496280126,-4.4552509625711,122.468529500786));
#38909=CARTESIAN_POINT('Ctrl Pts',(5.2174039761546,-4.31341878218784,122.477278777922));
#38910=CARTESIAN_POINT('Ctrl Pts',(5.33193710451566,-4.16686161439148,122.486028055058));
#38911=CARTESIAN_POINT('Ctrl Pts',(5.44646940289026,-4.02030550864997,122.494777268791));
#38912=CARTESIAN_POINT('Ctrl Pts',(5.5549557274932,-3.86902470980629,122.503526482524));
#38913=CARTESIAN_POINT('Ctrl Pts',(5.65702762491123,-3.71353301466289,122.512275696257));
#38914=CARTESIAN_POINT('Ctrl Pts',(5.75909881654838,-3.55804239467404,122.521024849493));
#38915=CARTESIAN_POINT('Ctrl Pts',(5.85475551250483,-3.39834117620068,122.529774002729));
#38916=CARTESIAN_POINT('Ctrl Pts',(5.94367283727813,-3.23497174692487,122.538523155966));
#38917=CARTESIAN_POINT('Ctrl Pts',(6.03258957676047,-3.07160339301485,122.547272251611));
#38918=CARTESIAN_POINT('Ctrl Pts',(6.11476689685037,-2.90456712830024,122.556021347257));
#38919=CARTESIAN_POINT('Ctrl Pts',(6.18992570525031,-2.73443024476425,122.564770442902));
#38920=CARTESIAN_POINT('Ctrl Pts',(6.26508404388496,-2.56429442463524,122.573519483863));
#38921=CARTESIAN_POINT('Ctrl Pts',(6.3332238428314,-2.3910582865646,122.582268524824));
#38922=CARTESIAN_POINT('Ctrl Pts',(6.39411368719881,-2.2153101713252,122.591017565785));
#38923=CARTESIAN_POINT('Ctrl Pts',(6.4550031712075,-2.03956309619958,122.599766554968));
#38924=CARTESIAN_POINT('Ctrl Pts',(6.50864269269945,-1.86130434439081,122.60851554415));
#38925=CARTESIAN_POINT('Ctrl Pts',(6.55485008446218,-1.68113930720396,122.617264533333));
#38926=CARTESIAN_POINT('Ctrl Pts',(6.60199664749303,-1.49731239212287,122.626191346862));
#38927=CARTESIAN_POINT('Ctrl Pts',(6.6414056364082,-1.31150116500113,122.635118160391));
#38928=CARTESIAN_POINT('Ctrl Pts',(6.67293772282099,-1.12436255156095,122.644044973921));
#38929=CARTESIAN_POINT('Ctrl Pts',(6.70384494949809,-0.94093239505575,122.652794888076));
#38930=CARTESIAN_POINT('Ctrl Pts',(6.7271844934888,-0.75622726051117,122.661544802232));
#38931=CARTESIAN_POINT('Ctrl Pts',(6.74287707373894,-0.57087456454619,122.670294716387));
#38932=CARTESIAN_POINT('Ctrl Pts',(6.75856934538644,-0.385525513637037,
122.679044458471));
#38933=CARTESIAN_POINT('Ctrl Pts',(6.76661493004089,-0.19952921242285,122.687794200555));
#38934=CARTESIAN_POINT('Ctrl Pts',(6.76698649908906,-0.0135174386051019,
122.696543942639));
#38935=CARTESIAN_POINT('Ctrl Pts',(6.76735806132401,0.172490924441081,122.705293524285));
#38936=CARTESIAN_POINT('Ctrl Pts',(6.76005588896314,0.358514472896692,122.714043105931));
#38937=CARTESIAN_POINT('Ctrl Pts',(6.74510478454622,0.543921359657485,122.722792687577));
#38938=CARTESIAN_POINT('Ctrl Pts',(6.73015393440739,0.729325093145684,122.731542120416));
#38939=CARTESIAN_POINT('Ctrl Pts',(6.70755443556962,0.914111900251564,122.740291553255));
#38940=CARTESIAN_POINT('Ctrl Pts',(6.67738304682398,1.09765415591057,122.749040986094));
#38941=CARTESIAN_POINT('Ctrl Pts',(6.64721213111951,1.28119353390805,122.757790281755));
#38942=CARTESIAN_POINT('Ctrl Pts',(6.60946960955595,1.46348811672198,122.766539577417));
#38943=CARTESIAN_POINT('Ctrl Pts',(6.56428366991293,1.6439187634778,122.775288873078));
#38944=CARTESIAN_POINT('Ctrl Pts',(6.5190983786784,1.82434682109278,122.784038043189));
#38945=CARTESIAN_POINT('Ctrl Pts',(6.46646995272056,2.0029107182001,122.7927872133));
#38946=CARTESIAN_POINT('Ctrl Pts',(6.40657713281696,2.17900400212273,122.80153638341));
#38947=CARTESIAN_POINT('Ctrl Pts',(6.34668509279217,2.35509499309234,122.810285439596));
#38948=CARTESIAN_POINT('Ctrl Pts',(6.27952894037694,2.52871516397704,122.819034495782));
#38949=CARTESIAN_POINT('Ctrl Pts',(6.20533675061626,2.69927486771008,122.827783551968));
#38950=CARTESIAN_POINT('Ctrl Pts',(6.12832117908101,2.87632521635532,122.83686555325));
#38951=CARTESIAN_POINT('Ctrl Pts',(6.04372366626267,3.05007728919627,122.845947554532));
#38952=CARTESIAN_POINT('Ctrl Pts',(5.95185378008057,3.21989527477846,122.855029555815));
#38953=CARTESIAN_POINT('Ctrl Pts',(5.86334450817571,3.38350129286406,122.863779336122));
#38954=CARTESIAN_POINT('Ctrl Pts',(5.76808562057466,3.54345567124619,122.872529116429));
#38955=CARTESIAN_POINT('Ctrl Pts',(5.66640068804705,3.69921508464971,122.881278896736));
#38956=CARTESIAN_POINT('Ctrl Pts',(5.56471941108155,3.85496889851948,122.890028362489));
#38957=CARTESIAN_POINT('Ctrl Pts',(5.45661270815357,4.00652780919305,122.898777828243));
#38958=CARTESIAN_POINT('Ctrl Pts',(5.34244776449369,4.15337704568901,122.907527293996));
#38959=CARTESIAN_POINT('Ctrl Pts',(5.22828631819858,4.3002217835593,122.916276491716));
#38960=CARTESIAN_POINT('Ctrl Pts',(5.1080671784434,4.44235690972368,122.925025689436));
#38961=CARTESIAN_POINT('Ctrl Pts',(4.98219864544997,4.57929969070342,122.933774887155));
#38962=CARTESIAN_POINT('Ctrl Pts',(4.85633329944311,4.71623900429707,122.942523863345));
#38963=CARTESIAN_POINT('Ctrl Pts',(4.72481904033941,4.84798602483331,122.951272839536));
#38964=CARTESIAN_POINT('Ctrl Pts',(4.58810250737498,4.97409332258849,122.960021815726));
#38965=CARTESIAN_POINT('Ctrl Pts',(4.45137708685942,5.10020881821873,122.968771360662));
#38966=CARTESIAN_POINT('Ctrl Pts',(4.30944892636351,5.22068366307686,122.977520905598));
#38967=CARTESIAN_POINT('Ctrl Pts',(4.16280009466959,5.33510865604618,122.986270450534));
#38968=CARTESIAN_POINT('Ctrl Pts',(4.01615988349087,5.44952692272672,122.995019481143));
#38969=CARTESIAN_POINT('Ctrl Pts',(3.8647997823253,5.55789587288419,123.003768511751));
#38970=CARTESIAN_POINT('Ctrl Pts',(3.70923383581366,5.65984746713682,123.012517542359));
#38971=CARTESIAN_POINT('Ctrl Pts',(3.55366577799845,5.76180044505195,123.021266691707));
#38972=CARTESIAN_POINT('Ctrl Pts',(3.3938920002715,5.85733573570879,123.030015841055));
#38973=CARTESIAN_POINT('Ctrl Pts',(3.23045513626356,5.94612887621757,123.038764990403));
#38974=CARTESIAN_POINT('Ctrl Pts',(3.18695122151793,5.96976399206575,123.041093854516));
#38975=CARTESIAN_POINT('Ctrl Pts',(3.14318791262776,5.99292165435275,123.043422718629));
#38976=CARTESIAN_POINT('Ctrl Pts',(3.09917575053267,6.01559628526635,123.045751582742));
#38977=CARTESIAN_POINT('Ctrl Pts',(3.09917575053254,6.01559628526642,121.045781922714));
#38978=CARTESIAN_POINT('Ctrl Pts',(2.94377814450788,6.0956555960054,121.053981099718));
#38979=CARTESIAN_POINT('Ctrl Pts',(2.78526454007982,6.16969567928123,121.062180276722));
#38980=CARTESIAN_POINT('Ctrl Pts',(2.62414456692463,6.23747980292361,121.070379453726));
#38981=CARTESIAN_POINT('Ctrl Pts',(2.46300343222845,6.30527282935118,121.078579707612));
#38982=CARTESIAN_POINT('Ctrl Pts',(2.29925557718677,6.36680811987964,121.086779961498));
#38983=CARTESIAN_POINT('Ctrl Pts',(2.13343027031341,6.42189724938904,121.094980215385));
#38984=CARTESIAN_POINT('Ctrl Pts',(1.96755310133998,6.47700360810187,121.103183033912));
#38985=CARTESIAN_POINT('Ctrl Pts',(1.79959752632693,6.52565967670675,121.111385852439));
#38986=CARTESIAN_POINT('Ctrl Pts',(1.63010766546976,6.56772700399284,121.119588670966));
#38987=CARTESIAN_POINT('Ctrl Pts',(1.45349391549002,6.61156247819789,121.1281362651));
#38988=CARTESIAN_POINT('Ctrl Pts',(1.27521453189092,6.64824324314782,121.136683859235));
#38989=CARTESIAN_POINT('Ctrl Pts',(1.09589560549116,6.67767188635869,121.145231453369));
#38990=CARTESIAN_POINT('Ctrl Pts',(0.923515546466782,6.70596176827772,121.153448292556));
#38991=CARTESIAN_POINT('Ctrl Pts',(0.750175246529651,6.72755026350163,121.161665131743));
#38992=CARTESIAN_POINT('Ctrl Pts',(0.576434595129533,6.74240403398802,121.16988197093));
#38993=CARTESIAN_POINT('Ctrl Pts',(0.402568471726121,6.75726853156864,121.178104744153));
#38994=CARTESIAN_POINT('Ctrl Pts',(0.228301777134898,6.76538859449395,121.186327517375));
#38995=CARTESIAN_POINT('Ctrl Pts',(0.0541937887683528,6.76678298996347,
121.194550290598));
#38996=CARTESIAN_POINT('Ctrl Pts',(-0.120146997815844,6.76817924986657,
121.202784058417));
#38997=CARTESIAN_POINT('Ctrl Pts',(-0.294328298351081,6.76283190029155,
121.211017826235));
#38998=CARTESIAN_POINT('Ctrl Pts',(-0.467795785605221,6.75081151440107,
121.219251594054));
#38999=CARTESIAN_POINT('Ctrl Pts',(-0.488218970115628,6.74939629496823,
121.220220996229));
#39000=CARTESIAN_POINT('Ctrl Pts',(-0.508632271863779,6.74788863533063,
121.221190398403));
#39001=CARTESIAN_POINT('Ctrl Pts',(-0.529034796293258,6.74628869707715,
121.222159800578));
#39002=CARTESIAN_POINT('Ctrl Pts',(-0.700645700907447,6.73283120303253,
121.230313692745));
#39003=CARTESIAN_POINT('Ctrl Pts',(-0.872023887206462,6.7127992772155,121.238467584911));
#39004=CARTESIAN_POINT('Ctrl Pts',(-1.04262025750242,6.68619712532061,121.246621477078));
#39005=CARTESIAN_POINT('Ctrl Pts',(-1.21300845256476,6.65962743548324,121.254765419218));
#39006=CARTESIAN_POINT('Ctrl Pts',(-1.38261637336091,6.62650353435076,121.262909361359));
#39007=CARTESIAN_POINT('Ctrl Pts',(-1.55089657585776,6.58688156952838,121.271053303499));
#39008=CARTESIAN_POINT('Ctrl Pts',(-1.71900684911815,6.54729961493971,121.279189021892));
#39009=CARTESIAN_POINT('Ctrl Pts',(-1.88579171996496,6.50123274296745,121.287324740285));
#39010=CARTESIAN_POINT('Ctrl Pts',(-2.05071051547285,6.4487886755366,121.295460458677));
#39011=CARTESIAN_POINT('Ctrl Pts',(-2.2154974667992,6.39638653446791,121.303589672978));
#39012=CARTESIAN_POINT('Ctrl Pts',(-2.37842096635326,6.33761745936685,121.311718887278));
#39013=CARTESIAN_POINT('Ctrl Pts',(-2.53895216831899,6.27263986587691,121.319848101578));
#39014=CARTESIAN_POINT('Ctrl Pts',(-2.69938878743832,6.20770055631975,121.327972526253));
#39015=CARTESIAN_POINT('Ctrl Pts',(-2.85743557786453,6.13656014993194,121.336096950929));
#39016=CARTESIAN_POINT('Ctrl Pts',(-3.01258046364437,6.05942637137117,121.344221375604));
#39017=CARTESIAN_POINT('Ctrl Pts',(-3.16866717820063,5.98182434139548,121.352395120738));
#39018=CARTESIAN_POINT('Ctrl Pts',(-3.32181628228949,5.89815604766954,121.360568865872));
#39019=CARTESIAN_POINT('Ctrl Pts',(-3.47152777146921,5.80868177230583,121.368742611006));
#39020=CARTESIAN_POINT('Ctrl Pts',(-3.620280552081,5.71978046401948,121.376864013869));
#39021=CARTESIAN_POINT('Ctrl Pts',(-3.76563931006539,5.62514752606199,121.384985416731));
#39022=CARTESIAN_POINT('Ctrl Pts',(-3.90713957320407,5.52508365144843,121.393106819593));
#39023=CARTESIAN_POINT('Ctrl Pts',(-4.04865077639776,5.42501204042317,121.401228850359));
#39024=CARTESIAN_POINT('Ctrl Pts',(-4.18630259167283,5.31950886763514,121.409350881125));
#39025=CARTESIAN_POINT('Ctrl Pts',(-4.31966097371313,5.20891716887299,121.417472911892));
#39026=CARTESIAN_POINT('Ctrl Pts',(-4.45305506083704,5.09829586052956,121.425597117233));
#39027=CARTESIAN_POINT('Ctrl Pts',(-4.58215314423595,4.98258354697544,121.433721322574));
#39028=CARTESIAN_POINT('Ctrl Pts',(-4.70655564283561,4.86216237705944,121.441845527915));
#39029=CARTESIAN_POINT('Ctrl Pts',(-4.83230471240292,4.74043773130393,121.450057672157));
#39030=CARTESIAN_POINT('Ctrl Pts',(-4.95325567413202,4.6139019596473,121.4582698164));
#39031=CARTESIAN_POINT('Ctrl Pts',(-5.06903596436854,4.4829859906025,121.466481960642));
#39032=CARTESIAN_POINT('Ctrl Pts',(-5.18375930816161,4.353265140067,121.474619137059));
#39033=CARTESIAN_POINT('Ctrl Pts',(-5.2934058099648,4.21924405500319,121.482756313475));
#39034=CARTESIAN_POINT('Ctrl Pts',(-5.39765548183425,4.08137284494135,121.490893489892));
#39035=CARTESIAN_POINT('Ctrl Pts',(-5.50334583242183,3.94159632319252,121.499143118047));
#39036=CARTESIAN_POINT('Ctrl Pts',(-5.60348887338751,3.79786280554131,121.507392746203));
#39037=CARTESIAN_POINT('Ctrl Pts',(-5.69779850792845,3.65066859123754,121.515642374358));
#39038=CARTESIAN_POINT('Ctrl Pts',(-5.79210814246933,3.50347437693388,121.523892002513));
#39039=CARTESIAN_POINT('Ctrl Pts',(-5.8805842302813,3.35281982980438,121.532141630669));
#39040=CARTESIAN_POINT('Ctrl Pts',(-5.96299075072147,3.1992233912014,121.540391258824));
#39041=CARTESIAN_POINT('Ctrl Pts',(-6.05007866566296,3.03690136244782,121.54910953635));
#39042=CARTESIAN_POINT('Ctrl Pts',(-6.13062359919724,2.87085576499492,121.557827813875));
#39043=CARTESIAN_POINT('Ctrl Pts',(-6.2043141710099,2.70162444973497,121.566546091401));
#39044=CARTESIAN_POINT('Ctrl Pts',(-6.2778836205095,2.53267129337434,121.575250039034));
#39045=CARTESIAN_POINT('Ctrl Pts',(-6.34462105769029,2.36054312842015,121.583953986667));
#39046=CARTESIAN_POINT('Ctrl Pts',(-6.40426083818913,2.18580239647528,121.592657934301));
#39047=CARTESIAN_POINT('Ctrl Pts',(-6.46394314581031,2.01093706278939,121.601368088426));
#39048=CARTESIAN_POINT('Ctrl Pts',(-6.51651750873807,1.83345568667579,121.610078242552));
#39049=CARTESIAN_POINT('Ctrl Pts',(-6.56176449452805,1.65394550041742,121.618788396678));
#39050=CARTESIAN_POINT('Ctrl Pts',(-6.60680989005414,1.47523509131964,121.627459744191));
#39051=CARTESIAN_POINT('Ctrl Pts',(-6.6445929576778,1.29451418989422,121.636131091703));
#39052=CARTESIAN_POINT('Ctrl Pts',(-6.6749454105017,1.1123815742911,121.644802439216));
#39053=CARTESIAN_POINT('Ctrl Pts',(-6.70550161641409,0.929026320005028,
121.653531996648));
#39054=CARTESIAN_POINT('Ctrl Pts',(-6.72852694174223,0.744240600378212,
121.662261554081));
#39055=CARTESIAN_POINT('Ctrl Pts',(-6.74390080922855,0.558650942258707,
121.670991111513));
#39056=CARTESIAN_POINT('Ctrl Pts',(-6.75927467671487,0.373061284139074,
121.679720668945));
#39057=CARTESIAN_POINT('Ctrl Pts',(-6.7669969978568,0.186667984783223,121.688450226378));
#39058=CARTESIAN_POINT('Ctrl Pts',(-6.76699999912433,0.000108864028085915,
121.69717978381));
#39059=CARTESIAN_POINT('',(-6.76699876671586,-0.00266907362020019,121.30282021619));
#39060=CARTESIAN_POINT('Ctrl Pts',(3.09917575053273,6.01559628526632,120.651392015122));
#39061=CARTESIAN_POINT('Ctrl Pts',(2.9338238445927,6.10078395293757,120.660141463035));
#39062=CARTESIAN_POINT('Ctrl Pts',(2.76495772122981,6.17915010267051,120.668890910947));
#39063=CARTESIAN_POINT('Ctrl Pts',(2.59315093316699,6.25042856433183,120.67764035886));
#39064=CARTESIAN_POINT('Ctrl Pts',(2.42134553245594,6.3217064504146,120.68638973612));
#39065=CARTESIAN_POINT('Ctrl Pts',(2.24659977927557,6.38589665313469,120.69513911338));
#39066=CARTESIAN_POINT('Ctrl Pts',(2.06950718689874,6.44278115439089,120.70388849064));
#39067=CARTESIAN_POINT('Ctrl Pts',(1.89241596572818,6.49966521519736,120.712637800154));
#39068=CARTESIAN_POINT('Ctrl Pts',(1.71297821457156,6.54924360009557,120.721387109669));
#39069=CARTESIAN_POINT('Ctrl Pts',(1.53180337335804,6.59134792173565,120.730136419184));
#39070=CARTESIAN_POINT('Ctrl Pts',(1.35062987477738,6.63345193135314,120.73888566386));
#39071=CARTESIAN_POINT('Ctrl Pts',(1.16771959102903,6.66808192368246,120.747634908536));
#39072=CARTESIAN_POINT('Ctrl Pts',(0.983693746906317,6.69512028363176,120.756384153212));
#39073=CARTESIAN_POINT('Ctrl Pts',(0.799669205419294,6.72215845218874,120.765133335956));
#39074=CARTESIAN_POINT('Ctrl Pts',(0.614529402872849,6.74160505424585,120.7738825187));
#39075=CARTESIAN_POINT('Ctrl Pts',(0.428903127362573,6.75339404354126,120.782631701445));
#39076=CARTESIAN_POINT('Ctrl Pts',(0.243278104163051,6.76518295330334,120.791380825163));
#39077=CARTESIAN_POINT('Ctrl Pts',(0.0571669005381381,6.76931433552277,
120.800129948882));
#39078=CARTESIAN_POINT('Ctrl Pts',(-0.128798404778644,6.76577415902471,
120.8088790726));
#39079=CARTESIAN_POINT('Ctrl Pts',(-0.31476251726011,6.76223400523436,120.8176281402));
#39080=CARTESIAN_POINT('Ctrl Pts',(-0.500580446820403,6.75102239665082,
120.826377207799));
#39081=CARTESIAN_POINT('Ctrl Pts',(-0.685621118843384,6.7321774101249,120.835126275398));
#39082=CARTESIAN_POINT('Ctrl Pts',(-0.87066066541513,6.71333253821763,120.843875289784));
#39083=CARTESIAN_POINT('Ctrl Pts',(-1.05492267885538,6.68685441030604,120.85262430417));
#39084=CARTESIAN_POINT('Ctrl Pts',(-1.2377813763529,6.6528329502817,120.861373318555));
#39085=CARTESIAN_POINT('Ctrl Pts',(-1.42999922978874,6.61707018861859,120.870570128923));
#39086=CARTESIAN_POINT('Ctrl Pts',(-1.62066601233712,6.57297172934408,120.87976693929));
#39087=CARTESIAN_POINT('Ctrl Pts',(-1.80906628500392,6.52070304311292,120.888963749658));
#39088=CARTESIAN_POINT('Ctrl Pts',(-1.98831342545526,6.47097374915031,120.897713747395));
#39089=CARTESIAN_POINT('Ctrl Pts',(-2.16550875896692,6.41384933989531,120.906463745133));
#39090=CARTESIAN_POINT('Ctrl Pts',(-2.34005036713994,6.34952386240482,120.915213742871));
#39091=CARTESIAN_POINT('Ctrl Pts',(-2.51458843547075,6.28519968948602,120.923963563152));
#39092=CARTESIAN_POINT('Ctrl Pts',(-2.68647261718045,6.21367483971104,120.932713383433));
#39093=CARTESIAN_POINT('Ctrl Pts',(-2.85511905908723,6.13519226743847,120.941463203713));
#39094=CARTESIAN_POINT('Ctrl Pts',(-3.02376230488874,6.05671118252942,120.950212858172));
#39095=CARTESIAN_POINT('Ctrl Pts',(-3.18916767379892,5.97127275992639,120.95896251263));
#39096=CARTESIAN_POINT('Ctrl Pts',(-3.35077334102773,5.87916720438005,120.967712167089));
#39097=CARTESIAN_POINT('Ctrl Pts',(-3.51237616037354,5.78706327195651,120.976461667357));
#39098=CARTESIAN_POINT('Ctrl Pts',(-3.67017916302287,5.68829258362307,120.985211167626));
#39099=CARTESIAN_POINT('Ctrl Pts',(-3.8236463656645,5.5831906174105,120.993960667894));
#39100=CARTESIAN_POINT('Ctrl Pts',(-3.97711106778785,5.47809036367711,121.002710025603));
#39101=CARTESIAN_POINT('Ctrl Pts',(-4.12623987481913,5.36665920043236,121.011459383311));
#39102=CARTESIAN_POINT('Ctrl Pts',(-4.27052628213915,5.24927559512347,121.02020874102));
#39103=CARTESIAN_POINT('Ctrl Pts',(-4.41481053024973,5.13189374643041,121.028957967796));
#39104=CARTESIAN_POINT('Ctrl Pts',(-4.55425230136534,5.0085598147735,121.037707194573));
#39105=CARTESIAN_POINT('Ctrl Pts',(-4.6883780063056,4.87969268192065,121.046456421349));
#39106=CARTESIAN_POINT('Ctrl Pts',(-4.82250188228906,4.75082730631798,121.05520552882));
#39107=CARTESIAN_POINT('Ctrl Pts',(-4.95130963052977,4.61642907903514,121.063954636291));
#39108=CARTESIAN_POINT('Ctrl Pts',(-5.07436379033377,4.47695444731678,121.072703743762));
#39109=CARTESIAN_POINT('Ctrl Pts',(-5.19741643562825,4.33748153220563,121.081452743552));
#39110=CARTESIAN_POINT('Ctrl Pts',(-5.31471544462801,4.19293255254554,121.090201743341));
#39111=CARTESIAN_POINT('Ctrl Pts',(-5.42586245275663,4.04379841779555,121.098950743131));
#39112=CARTESIAN_POINT('Ctrl Pts',(-5.53702160019175,3.8946479948431,121.107700698473));
#39113=CARTESIAN_POINT('Ctrl Pts',(-5.64202723081262,3.74091164443833,121.116450653815));
#39114=CARTESIAN_POINT('Ctrl Pts',(-5.74052265232967,3.58311159163232,121.125200609157));
#39115=CARTESIAN_POINT('Ctrl Pts',(-5.8390142706692,3.4253176319178,121.13395022664));
#39116=CARTESIAN_POINT('Ctrl Pts',(-5.93099603115743,3.26346052695607,121.142699844122));
#39117=CARTESIAN_POINT('Ctrl Pts',(-6.01615550622758,3.09809004467068,121.151449461605));
#39118=CARTESIAN_POINT('Ctrl Pts',(-6.10131214578807,2.93272506863812,121.160198787756));
#39119=CARTESIAN_POINT('Ctrl Pts',(-6.17964682328758,2.76384720416872,121.168948113907));
#39120=CARTESIAN_POINT('Ctrl Pts',(-6.25089348288576,2.59203002791563,121.177697440058));
#39121=CARTESIAN_POINT('Ctrl Pts',(-6.32213814889348,2.42021765936983,121.18644652139));
#39122=CARTESIAN_POINT('Ctrl Pts',(-6.38629508412607,2.24546640831856,121.195195602721));
#39123=CARTESIAN_POINT('Ctrl Pts',(-6.44314639819837,2.06836976659963,121.203944684053));
#39124=CARTESIAN_POINT('Ctrl Pts',(-6.50000285283727,1.89125711158184,121.212694556487));
#39125=CARTESIAN_POINT('Ctrl Pts',(-6.54955227673277,1.71179891440149,121.221444428922));
#39126=CARTESIAN_POINT('Ctrl Pts',(-6.59162635926413,1.53060476278312,121.230194301356));
#39127=CARTESIAN_POINT('Ctrl Pts',(-6.63369752055219,1.34942319164583,121.238943566279));
#39128=CARTESIAN_POINT('Ctrl Pts',(-6.66829431424272,1.16650618642598,121.247692831201));
#39129=CARTESIAN_POINT('Ctrl Pts',(-6.69529923745432,0.982474997617564,
121.256442096124));
#39130=CARTESIAN_POINT('Ctrl Pts',(-6.72230554731455,0.798434359176729,
121.265191810303));
#39131=CARTESIAN_POINT('Ctrl Pts',(-6.74171916496712,0.613279706239307,
121.273941524483));
#39132=CARTESIAN_POINT('Ctrl Pts',(-6.75347414817282,0.427639953654331,
121.282691238663));
#39133=CARTESIAN_POINT('Ctrl Pts',(-6.76248837758734,0.285283364199802,
121.289400897838));
#39134=CARTESIAN_POINT('Ctrl Pts',(-6.76699999999985,0.142641701108631,
121.296110557014));
#39135=CARTESIAN_POINT('Ctrl Pts',(-6.767,7.36526836825673E-12,121.30282021619));
#39136=CARTESIAN_POINT('Ctrl Pts',(-6.76699711044301,-0.00625357945092592,
121.30282021619));
#39137=CARTESIAN_POINT('Ctrl Pts',(-6.7667990677175,-0.220555574302487,
121.312887263886));
#39138=CARTESIAN_POINT('Ctrl Pts',(-6.75641746286505,-0.434393464847247,
121.322954311582));
#39139=CARTESIAN_POINT('Ctrl Pts',(-6.73600616481901,-0.64692344795989,
121.333021359278));
#39140=CARTESIAN_POINT('Ctrl Pts',(-6.71538293818884,-0.861660109859227,
121.343192932182));
#39141=CARTESIAN_POINT('Ctrl Pts',(-6.68452074611038,-1.07506164536285,
121.353364505086));
#39142=CARTESIAN_POINT('Ctrl Pts',(-6.64362620636337,-1.28628139616565,
121.363536077989));
#39143=CARTESIAN_POINT('Ctrl Pts',(-6.60229775646945,-1.49974228707341,
121.373815576027));
#39144=CARTESIAN_POINT('Ctrl Pts',(-6.55072295034635,-1.71097494008967,
121.384095074065));
#39145=CARTESIAN_POINT('Ctrl Pts',(-6.48916295838299,-1.91912821342145,
121.394374572103));
#39146=CARTESIAN_POINT('Ctrl Pts',(-6.47633796933195,-1.96249344733842,
121.396516132646));
#39147=CARTESIAN_POINT('Ctrl Pts',(-6.46307976012568,-2.00572510299209,
121.398657693188));
#39148=CARTESIAN_POINT('Ctrl Pts',(-6.44939095057919,-2.04881560092343,
121.400799253731));
#39149=CARTESIAN_POINT('Ctrl Pts',(-6.39726143349232,-2.21291218219047,
121.408954712138));
#39150=CARTESIAN_POINT('Ctrl Pts',(-6.33877995666408,-2.37528556587604,
121.417110170545));
#39151=CARTESIAN_POINT('Ctrl Pts',(-6.2740757464106,-2.5354018474992,121.425265628951));
#39152=CARTESIAN_POINT('Ctrl Pts',(-6.20945028968617,-2.69532324656078,
121.433411161093));
#39153=CARTESIAN_POINT('Ctrl Pts',(-6.13861731113867,-2.85299267681184,
121.441556693235));
#39154=CARTESIAN_POINT('Ctrl Pts',(-6.06175623643756,-3.00788968049202,
121.449702225377));
#39155=CARTESIAN_POINT('Ctrl Pts',(-5.98497254942552,-3.16263072589024,
121.457839556178));
#39156=CARTESIAN_POINT('Ctrl Pts',(-5.90217301060363,-3.3146045769819,121.465976886978));
#39157=CARTESIAN_POINT('Ctrl Pts',(-5.81358572146447,-3.46330911978478,
121.474114217779));
#39158=CARTESIAN_POINT('Ctrl Pts',(-5.72506900967825,-3.61189518991396,
121.482245065581));
#39159=CARTESIAN_POINT('Ctrl Pts',(-5.63077391502269,-3.75721682539706,
121.490375913383));
#39160=CARTESIAN_POINT('Ctrl Pts',(-5.53097520618648,-3.89879497647035,
121.498506761185));
#39161=CARTESIAN_POINT('Ctrl Pts',(-5.43123504237683,-4.04029007339683,
121.506632839179));
#39162=CARTESIAN_POINT('Ctrl Pts',(-5.32599790411775,-4.1780457613,121.514758917172));
#39163=CARTESIAN_POINT('Ctrl Pts',(-5.21558275402377,-4.31161055012275,
121.522884995166));
#39164=CARTESIAN_POINT('Ctrl Pts',(-5.10477609197409,-4.44564893529203,
121.531039886748));
#39165=CARTESIAN_POINT('Ctrl Pts',(-4.98875482570804,-4.57546633021193,
121.539194778331));
#39166=CARTESIAN_POINT('Ctrl Pts',(-4.86788353512265,-4.70063813630467,
121.547349669913));
#39167=CARTESIAN_POINT('Ctrl Pts',(-4.74748360030912,-4.8253218161187,121.555472760269));
#39168=CARTESIAN_POINT('Ctrl Pts',(-4.6222716682509,-4.94539582134728,121.563595850625));
#39169=CARTESIAN_POINT('Ctrl Pts',(-4.49264629704856,-5.0604760892248,121.571718940982));
#39170=CARTESIAN_POINT('Ctrl Pts',(-4.36301074707036,-5.17556539373026,
121.5798426692));
#39171=CARTESIAN_POINT('Ctrl Pts',(-4.22896134117997,-5.28565993689408,
121.587966397419));
#39172=CARTESIAN_POINT('Ctrl Pts',(-4.09093095177298,-5.39041491425529,
121.596090125637));
#39173=CARTESIAN_POINT('Ctrl Pts',(-3.9528634634716,-5.4951980469659,121.604216037297));
#39174=CARTESIAN_POINT('Ctrl Pts',(-3.8108131524038,-5.59463853519105,121.612341948958));
#39175=CARTESIAN_POINT('Ctrl Pts',(-3.66524314378872,-5.68843402852752,
121.620467860618));
#39176=CARTESIAN_POINT('Ctrl Pts',(-3.51874219983684,-5.78282935379372,
121.628645738328));
#39177=CARTESIAN_POINT('Ctrl Pts',(-3.36867670015287,-5.8715070294679,121.636823616038));
#39178=CARTESIAN_POINT('Ctrl Pts',(-3.21554448135241,-5.95420546239749,
121.645001493748));
#39179=CARTESIAN_POINT('Ctrl Pts',(-3.06314312941981,-6.03650919364296,
121.653140340222));
#39180=CARTESIAN_POINT('Ctrl Pts',(-2.90770462327633,-6.11289052619905,
121.661279186695));
#39181=CARTESIAN_POINT('Ctrl Pts',(-2.74974009032668,-6.18313985250619,
121.669418033168));
#39182=CARTESIAN_POINT('Ctrl Pts',(-2.59063923828957,-6.25389451788453,
121.677615426497));
#39183=CARTESIAN_POINT('Ctrl Pts',(-2.42897623128213,-6.31842848308074,
121.685812819825));
#39184=CARTESIAN_POINT('Ctrl Pts',(-2.26528877975034,-6.37657868643815,
121.694010213154));
#39185=CARTESIAN_POINT('Ctrl Pts',(-2.10160132821855,-6.43472888979555,
121.702207606482));
#39186=CARTESIAN_POINT('Ctrl Pts',(-1.93588980568439,-6.48649527865371,
121.71040499981));
#39187=CARTESIAN_POINT('Ctrl Pts',(-1.768701904929,-6.53176718595363,121.718602393139));
#39188=CARTESIAN_POINT('Ctrl Pts',(-1.60092629442354,-6.57719823599775,
121.726828602476));
#39189=CARTESIAN_POINT('Ctrl Pts',(-1.4311646085969,-6.61622438915903,121.735054811813));
#39190=CARTESIAN_POINT('Ctrl Pts',(-1.25994680357312,-6.64867077333251,
121.74328102115));
#39191=CARTESIAN_POINT('Ctrl Pts',(-1.0889213544183,-6.68108070538337,121.751497988693));
#39192=CARTESIAN_POINT('Ctrl Pts',(-0.916443392727803,-6.70692552193531,
121.759714956236));
#39193=CARTESIAN_POINT('Ctrl Pts',(-0.743057841187611,-6.72608013962439,
121.767931923779));
#39194=CARTESIAN_POINT('Ctrl Pts',(-0.569832281017914,-6.74521708240625,
121.776141309123));
#39195=CARTESIAN_POINT('Ctrl Pts',(-0.395701153094108,-6.75767608169907,
121.784350694466));
#39196=CARTESIAN_POINT('Ctrl Pts',(-0.221219470160394,-6.76338309916139,
121.792560079809));
#39197=CARTESIAN_POINT('Ctrl Pts',(-0.0468637814196446,-6.76908599555469,
121.80076353711));
#39198=CARTESIAN_POINT('Ctrl Pts',(0.127841601131879,-6.76804660988572,
121.808966994411));
#39199=CARTESIAN_POINT('Ctrl Pts',(0.302336551891229,-6.76024271823065,
121.817170451711));
#39200=CARTESIAN_POINT('Ctrl Pts',(0.476740502135301,-6.75244289636763,
121.825369630843));
#39201=CARTESIAN_POINT('Ctrl Pts',(0.650933881786635,-6.73788561239784,
121.833568809975));
#39202=CARTESIAN_POINT('Ctrl Pts',(0.824356481458405,-6.716600731879,121.841767989107));
#39203=CARTESIAN_POINT('Ctrl Pts',(0.997746404574913,-6.69531986189037,
121.849965623337));
#39204=CARTESIAN_POINT('Ctrl Pts',(1.17036548064243,-6.66731395780021,121.858163257566));
#39205=CARTESIAN_POINT('Ctrl Pts',(1.34165822783221,-6.63266478873237,121.866360891796));
#39206=CARTESIAN_POINT('Ctrl Pts',(1.51293861092379,-6.59801812067951,121.874557934312));
#39207=CARTESIAN_POINT('Ctrl Pts',(1.68289250406754,-6.55672921288288,121.882754976827));
#39208=CARTESIAN_POINT('Ctrl Pts',(1.8509742857312,-6.50893103309306,121.890952019343));
#39209=CARTESIAN_POINT('Ctrl Pts',(2.01907448365012,-6.46112761618907,121.899149959986));
#39210=CARTESIAN_POINT('Ctrl Pts',(2.18530181635332,-6.40681360451515,121.907347900629));
#39211=CARTESIAN_POINT('Ctrl Pts',(2.34912545074222,-6.34617196557698,121.915545841271));
#39212=CARTESIAN_POINT('Ctrl Pts',(2.51299680961457,-6.28551266074521,121.923746170107));
#39213=CARTESIAN_POINT('Ctrl Pts',(2.67446273909679,-6.21852218142059,121.931946498943));
#39214=CARTESIAN_POINT('Ctrl Pts',(2.83301197825863,-6.14543180997423,121.940146827779));
#39215=CARTESIAN_POINT('Ctrl Pts',(2.99172642984156,-6.07226527646434,121.948355701571));
#39216=CARTESIAN_POINT('Ctrl Pts',(3.14751779294393,-5.99298630237409,121.956564575362));
#39217=CARTESIAN_POINT('Ctrl Pts',(3.29989814603073,-5.90787281733646,121.964773449153));
#39218=CARTESIAN_POINT('Ctrl Pts',(3.45236027997206,-5.82271365283032,121.972986728557));
#39219=CARTESIAN_POINT('Ctrl Pts',(3.60140744859456,-5.73171392171152,121.98120000796));
#39220=CARTESIAN_POINT('Ctrl Pts',(3.74658047352514,-5.63519509470614,121.989413287364));
#39221=CARTESIAN_POINT('Ctrl Pts',(3.89196583682183,-5.5385350937462,121.997638579979));
#39222=CARTESIAN_POINT('Ctrl Pts',(4.03346544145236,-5.43634007443489,122.005863872595));
#39223=CARTESIAN_POINT('Ctrl Pts',(4.17065196527354,-5.32897280763938,122.01408916521));
#39224=CARTESIAN_POINT('Ctrl Pts',(4.2947206966164,-5.23187201225489,122.021527954322));
#39225=CARTESIAN_POINT('Ctrl Pts',(4.41526204542133,-5.13054146037317,122.028966743434));
#39226=CARTESIAN_POINT('Ctrl Pts',(4.53198638129172,-5.0252749616102,122.036405532546));
#39227=CARTESIAN_POINT('Ctrl Pts',(4.66106624041878,-4.908865776415,122.044631733565));
#39228=CARTESIAN_POINT('Ctrl Pts',(4.78583848198063,-4.78731734698028,122.052857934584));
#39229=CARTESIAN_POINT('Ctrl Pts',(4.90586901710682,-4.66098038903742,122.061084135603));
#39230=CARTESIAN_POINT('Ctrl Pts',(5.02576472322457,-4.53478534403988,122.069301096219));
#39231=CARTESIAN_POINT('Ctrl Pts',(5.1409290842546,-4.40381273903107,122.077518056834));
#39232=CARTESIAN_POINT('Ctrl Pts',(5.2509617530061,-4.26845284247901,122.08573501745));
#39233=CARTESIAN_POINT('Ctrl Pts',(5.36089290767535,-4.13321782643586,122.093944397252));
#39234=CARTESIAN_POINT('Ctrl Pts',(5.46570157400974,-3.9936038564033,122.102153777053));
#39235=CARTESIAN_POINT('Ctrl Pts',(5.56502484426122,-3.85003733524175,122.110363156855));
#39236=CARTESIAN_POINT('Ctrl Pts',(5.66427640929441,-3.70657446017152,122.118566609995));
#39237=CARTESIAN_POINT('Ctrl Pts',(5.75805026289624,-3.55916501138617,122.126770063136));
#39238=CARTESIAN_POINT('Ctrl Pts',(5.8460242798256,-3.40826775938887,122.134973516276));
#39239=CARTESIAN_POINT('Ctrl Pts',(5.93395243235963,-3.25744917620151,122.143172692626));
#39240=CARTESIAN_POINT('Ctrl Pts',(6.01608659174577,-3.10314672133383,122.151371868976));
#39241=CARTESIAN_POINT('Ctrl Pts',(6.09214837090922,-2.94584745477903,122.159571045326));
#39242=CARTESIAN_POINT('Ctrl Pts',(6.16819583790101,-2.78857778645518,122.167768678878));
#39243=CARTESIAN_POINT('Ctrl Pts',(6.23817303906425,-2.62831274949341,122.175966312429));
#39244=CARTESIAN_POINT('Ctrl Pts',(6.30184777566054,-2.46556354864407,122.184163945981));
#39245=CARTESIAN_POINT('Ctrl Pts',(6.36551792611308,-2.3028260697314,122.192360989101));
#39246=CARTESIAN_POINT('Ctrl Pts',(6.42288638452119,-2.13760511696331,122.200558032222));
#39247=CARTESIAN_POINT('Ctrl Pts',(6.4737693286473,-1.97043134350466,122.208755075342));
#39248=CARTESIAN_POINT('Ctrl Pts',(6.52465785584281,-1.80323922710623,122.216953017873));
#39249=CARTESIAN_POINT('Ctrl Pts',(6.56905934654972,-1.63409420633661,122.225150960405));
#39250=CARTESIAN_POINT('Ctrl Pts',(6.60684001709581,-1.46354159097082,122.233348902936));
#39251=CARTESIAN_POINT('Ctrl Pts',(6.6446316996796,-1.29293926415734,122.241549234944));
#39252=CARTESIAN_POINT('Ctrl Pts',(6.67579864064143,-1.1209288756312,122.249749566953));
#39253=CARTESIAN_POINT('Ctrl Pts',(6.70025827018953,-0.948065458054879,
122.257949898961));
#39254=CARTESIAN_POINT('Ctrl Pts',(6.72474339328254,-0.775021870076149,
122.266158777932));
#39255=CARTESIAN_POINT('Ctrl Pts',(6.74250718802028,-0.601123832397273,
122.274367656903));
#39256=CARTESIAN_POINT('Ctrl Pts',(6.75351893764249,-0.426932030778096,
122.282576535873));
#39257=CARTESIAN_POINT('Ctrl Pts',(6.7645365986273,-0.252646718959552,122.290789821561));
#39258=CARTESIAN_POINT('Ctrl Pts',(6.76879497988533,-0.0780676870470245,
122.299003107248));
#39259=CARTESIAN_POINT('Ctrl Pts',(6.76631553427568,0.0962449511384691,
122.307216392936));
#39260=CARTESIAN_POINT('Ctrl Pts',(6.76383246154269,0.270812587230064,122.315441693648));
#39261=CARTESIAN_POINT('Ctrl Pts',(6.75459188313694,0.445112692648713,122.32366699436));
#39262=CARTESIAN_POINT('Ctrl Pts',(6.7386672243945,0.618589556063905,122.331892295072));
#39263=CARTESIAN_POINT('Ctrl Pts',(6.72426529151869,0.775478452888617,122.339331087366));
#39264=CARTESIAN_POINT('Ctrl Pts',(6.70439713560802,0.931693923007618,122.34676987966));
#39265=CARTESIAN_POINT('Ctrl Pts',(6.67915281055769,1.08683335117182,122.354208671954));
#39266=CARTESIAN_POINT('Ctrl Pts',(6.65148500222167,1.2568663370111,122.362361596583));
#39267=CARTESIAN_POINT('Ctrl Pts',(6.61727681365689,1.42610807811444,122.370514521212));
#39268=CARTESIAN_POINT('Ctrl Pts',(6.57658092578735,1.59401139474282,122.378667445841));
#39269=CARTESIAN_POINT('Ctrl Pts',(6.53593258489289,1.76171854180155,122.386810845014));
#39270=CARTESIAN_POINT('Ctrl Pts',(6.48881171897181,1.92809002555886,122.394954244186));
#39271=CARTESIAN_POINT('Ctrl Pts',(6.43532261394787,2.0925849694603,122.403097643359));
#39272=CARTESIAN_POINT('Ctrl Pts',(6.3818847567147,2.25692231112737,122.411233240359));
#39273=CARTESIAN_POINT('Ctrl Pts',(6.32209092029141,2.41938634719022,122.419368837359));
#39274=CARTESIAN_POINT('Ctrl Pts',(6.25609616704935,2.57944756655963,122.427504434359));
#39275=CARTESIAN_POINT('Ctrl Pts',(6.19015077552044,2.73938906586634,122.435633946224));
#39276=CARTESIAN_POINT('Ctrl Pts',(6.11801384166961,2.8969309906905,122.443763458089));
#39277=CARTESIAN_POINT('Ctrl Pts',(6.03988987083367,3.05156014985792,122.451892969954));
#39278=CARTESIAN_POINT('Ctrl Pts',(5.96008215820792,3.20952190431493,122.460197690512));
#39279=CARTESIAN_POINT('Ctrl Pts',(5.87402652457492,3.364443543617,122.46850241107));
#39280=CARTESIAN_POINT('Ctrl Pts',(5.78199273309133,3.51579991388576,122.476807131629));
#39281=CARTESIAN_POINT('Ctrl Pts',(5.69196934586634,3.66385002580691,122.484930442236));
#39282=CARTESIAN_POINT('Ctrl Pts',(5.5962264751229,3.80848869102389,122.493053752844));
#39283=CARTESIAN_POINT('Ctrl Pts',(5.49506263634738,3.94925000761144,122.501177063452));
#39284=CARTESIAN_POINT('Ctrl Pts',(5.39390564159697,4.09000180129046,122.509299824494));
#39285=CARTESIAN_POINT('Ctrl Pts',(5.28732862221035,4.22687647149645,122.517422585536));
#39286=CARTESIAN_POINT('Ctrl Pts',(5.17567266775499,4.3594382019079,122.525545346578));
#39287=CARTESIAN_POINT('Ctrl Pts',(5.06400302596988,4.49201618238076,122.533669103348));
#39288=CARTESIAN_POINT('Ctrl Pts',(4.9472534453284,4.62027989086817,122.541792860118));
#39289=CARTESIAN_POINT('Ctrl Pts',(4.8258044005045,4.7438276621386,122.549916616888));
#39290=CARTESIAN_POINT('Ctrl Pts',(4.69961554516717,4.87219715124163,122.55835742076));
#39291=CARTESIAN_POINT('Ctrl Pts',(4.56835331246919,4.99547486805166,122.566798224632));
#39292=CARTESIAN_POINT('Ctrl Pts',(4.4324849164597,5.11325399969112,122.575239028504));
#39293=CARTESIAN_POINT('Ctrl Pts',(4.30155297331786,5.2267539085738,122.583373155977));
#39294=CARTESIAN_POINT('Ctrl Pts',(4.16634401070505,5.33514757407355,122.59150728345));
#39295=CARTESIAN_POINT('Ctrl Pts',(4.02730790080774,5.43811365016322,122.599641410922));
#39296=CARTESIAN_POINT('Ctrl Pts',(3.88819094874203,5.54113959559813,122.607780267961));
#39297=CARTESIAN_POINT('Ctrl Pts',(3.74524271662562,5.63873145810819,122.615919125));
#39298=CARTESIAN_POINT('Ctrl Pts',(3.59894037176235,5.73061228844694,122.624057982039));
#39299=CARTESIAN_POINT('Ctrl Pts',(3.4524688313739,5.82259937699609,122.632206251492));
#39300=CARTESIAN_POINT('Ctrl Pts',(3.30263575147417,5.90886206933069,122.640354520945));
#39301=CARTESIAN_POINT('Ctrl Pts',(3.14994160343767,5.98916996711001,122.648502790398));
#39302=CARTESIAN_POINT('Ctrl Pts',(3.13305439803827,5.99805161701233,122.649403948049));
#39303=CARTESIAN_POINT('Ctrl Pts',(3.11613221692979,6.00686048136917,122.650305105701));
#39304=CARTESIAN_POINT('Ctrl Pts',(3.0991757505325,6.01559628526643,122.651206263353));
#39305=CARTESIAN_POINT('Origin',(0.,0.,-3.69717978381041));
#39306=CARTESIAN_POINT('',(3.09917575053273,6.01559628526632,125.045751582742));
#39307=CARTESIAN_POINT('',(3.09917575053274,6.01559628526631,124.651594452187));
#39308=CARTESIAN_POINT('',(3.09917575053259,6.01559628526639,-3.69717978381041));
#39309=CARTESIAN_POINT('',(-6.767,9.5990736862783E-10,123.697179783765));
#39310=CARTESIAN_POINT('Ctrl Pts',(-6.767,7.29749759425155E-12,123.69717978381));
#39311=CARTESIAN_POINT('Ctrl Pts',(-6.7670000000002,-0.186007249408372,
123.705929295616));
#39312=CARTESIAN_POINT('Ctrl Pts',(-6.75932637295478,-0.372014355520227,
123.714678807422));
#39313=CARTESIAN_POINT('Ctrl Pts',(-6.74400518266988,-0.55738953714775,
123.723428319228));
#39314=CARTESIAN_POINT('Ctrl Pts',(-6.72868405709725,-0.742763935804244,
123.732177794078));
#39315=CARTESIAN_POINT('Ctrl Pts',(-6.70571545653088,-0.927506129688036,
123.740927268929));
#39316=CARTESIAN_POINT('Ctrl Pts',(-6.67517739415764,-1.11098863924292,
123.74967674378));
#39317=CARTESIAN_POINT('Ctrl Pts',(-6.64463945823195,-1.2944703890602,123.758426182402));
#39318=CARTESIAN_POINT('Ctrl Pts',(-6.60653217027257,-1.47669218227774,
123.767175621024));
#39319=CARTESIAN_POINT('Ctrl Pts',(-6.56098496116814,-1.65703510503716,
123.775925059646));
#39320=CARTESIAN_POINT('Ctrl Pts',(-6.51543793687627,-1.83737729603632,
123.784674462766));
#39321=CARTESIAN_POINT('Ctrl Pts',(-6.46245112202755,-2.01584035396681,
123.793423865886));
#39322=CARTESIAN_POINT('Ctrl Pts',(-6.40220448416364,-2.19181813637788,
123.802173269006));
#39323=CARTESIAN_POINT('Ctrl Pts',(-6.3419580857532,-2.36779521935587,123.810922637351));
#39324=CARTESIAN_POINT('Ctrl Pts',(-6.27445201489379,-2.54128677544469,
123.819672005697));
#39325=CARTESIAN_POINT('Ctrl Pts',(-6.1999155513634,-2.71170355237482,123.828421374042));
#39326=CARTESIAN_POINT('Ctrl Pts',(-6.1253793778921,-2.88211966612706,123.837170708339));
#39327=CARTESIAN_POINT('Ctrl Pts',(-6.04381298133805,-3.04946076210072,
123.845920042636));
#39328=CARTESIAN_POINT('Ctrl Pts',(-5.95549339426511,-3.21315848206475,
123.854669376933));
#39329=CARTESIAN_POINT('Ctrl Pts',(-5.86717414355369,-3.37685557859274,
123.863418677909));
#39330=CARTESIAN_POINT('Ctrl Pts',(-5.7721018898645,-3.53690907466967,123.872167978884));
#39331=CARTESIAN_POINT('Ctrl Pts',(-5.67059953467281,-3.69277536784578,
123.88091727986));
#39332=CARTESIAN_POINT('Ctrl Pts',(-5.56909755761995,-3.8486410803546,123.889666548241));
#39333=CARTESIAN_POINT('Ctrl Pts',(-5.46116568338317,-4.00031938103941,
123.898415816621));
#39334=CARTESIAN_POINT('Ctrl Pts',(-5.3471704868638,-4.14729511662876,123.907165085002));
#39335=CARTESIAN_POINT('Ctrl Pts',(-5.23317570555786,-4.29427031687713,
123.915914321515));
#39336=CARTESIAN_POINT('Ctrl Pts',(-5.11311782179076,-4.43654275986818,
123.924663558027));
#39337=CARTESIAN_POINT('Ctrl Pts',(-4.98740459172287,-4.57362924147352,
123.93341279454));
#39338=CARTESIAN_POINT('Ctrl Pts',(-4.86169180911126,-4.7107152351413,123.942161999911));
#39339=CARTESIAN_POINT('Ctrl Pts',(-4.73032391415752,-4.8426150931621,123.950911205282));
#39340=CARTESIAN_POINT('Ctrl Pts',(-4.59374707237639,-4.96888084331204,
123.959660410653));
#39341=CARTESIAN_POINT('Ctrl Pts',(-4.45717070537756,-5.09514615452415,
123.96840958561));
#39342=CARTESIAN_POINT('Ctrl Pts',(-4.3153856381987,-5.21577720253334,123.977158760566));
#39343=CARTESIAN_POINT('Ctrl Pts',(-4.16887341291016,-5.33036429028362,
123.985907935522));
#39344=CARTESIAN_POINT('Ctrl Pts',(-4.02236168477707,-5.44495098920905,
123.99465708079));
#39345=CARTESIAN_POINT('Ctrl Pts',(-3.87112305634806,-5.55349359238503,
124.003406226058));
#39346=CARTESIAN_POINT('Ctrl Pts',(-3.71567117317098,-5.65562346102233,
124.012155371326));
#39347=CARTESIAN_POINT('Ctrl Pts',(-3.56021980457667,-5.75775299158543,
124.020904487632));
#39348=CARTESIAN_POINT('Ctrl Pts',(-3.40055544862755,-5.8534696727514,124.029653603938));
#39349=CARTESIAN_POINT('Ctrl Pts',(-3.23722036323771,-5.94244842803361,
124.038402720244));
#39350=CARTESIAN_POINT('Ctrl Pts',(-3.07388580496435,-6.03142689616277,
124.047151808315));
#39351=CARTESIAN_POINT('Ctrl Pts',(-2.90688079258117,-6.11366734484627,
124.055900896386));
#39352=CARTESIAN_POINT('Ctrl Pts',(-2.73677251095046,-6.18889046787111,
124.064649984457));
#39353=CARTESIAN_POINT('Ctrl Pts',(-2.56666476417127,-6.26411335438071,
124.073399045019));
#39354=CARTESIAN_POINT('Ctrl Pts',(-2.39345402972626,-6.33231884350088,
124.082148105582));
#39355=CARTESIAN_POINT('Ctrl Pts',(-2.21772856474624,-6.3932752962084,124.090897166144));
#39356=CARTESIAN_POINT('Ctrl Pts',(-2.0420036376887,-6.45423156231892,124.099646199924));
#39357=CARTESIAN_POINT('Ctrl Pts',(-1.86376426620707,-6.5079387425188,124.108395233704));
#39358=CARTESIAN_POINT('Ctrl Pts',(-1.68361578195316,-6.55421443795962,
124.117144267484));
#39359=CARTESIAN_POINT('Ctrl Pts',(-1.50346783420525,-6.60048999558529,
124.125893275208));
#39360=CARTESIAN_POINT('Ctrl Pts',(-1.32141106257932,-6.63933404145358,
124.134642282932));
#39361=CARTESIAN_POINT('Ctrl Pts',(-1.13806375959759,-6.67061465526908,
124.143391290656));
#39362=CARTESIAN_POINT('Ctrl Pts',(-0.954716987426143,-6.70189517852381,
124.152140273051));
#39363=CARTESIAN_POINT('Ctrl Pts',(-0.770079973816703,-6.7256122653575,
124.160889255446));
#39364=CARTESIAN_POINT('Ctrl Pts',(-0.58477977055911,-6.74168536939724,
124.169638237841));
#39365=CARTESIAN_POINT('Ctrl Pts',(-0.39149064756057,-6.75845143942355,
124.178764418517));
#39366=CARTESIAN_POINT('Ctrl Pts',(-0.19748021311099,-6.76689975924007,
124.187890599193));
#39367=CARTESIAN_POINT('Ctrl Pts',(-0.00346532630443964,-6.76699911271707,
124.197016779869));
#39368=CARTESIAN_POINT('Ctrl Pts',(0.184486595289502,-6.76709536139791,
124.205857767399));
#39369=CARTESIAN_POINT('Ctrl Pts',(0.372442378178774,-6.75935659726806,
124.214698754929));
#39370=CARTESIAN_POINT('Ctrl Pts',(0.559750217715735,-6.74380965729069,
124.223539742459));
#39371=CARTESIAN_POINT('Ctrl Pts',(0.745129914451417,-6.72842275717324,
124.232289721057));
#39372=CARTESIAN_POINT('Ctrl Pts',(0.929874656307869,-6.7053877227356,124.241039699655));
#39373=CARTESIAN_POINT('Ctrl Pts',(1.11335688289149,-6.67478280180847,124.249789678252));
#39374=CARTESIAN_POINT('Ctrl Pts',(1.2968372311823,-6.64417819418146,124.258539567277));
#39375=CARTESIAN_POINT('Ctrl Pts',(1.47905480729612,-6.60600390230215,124.267289456302));
#39376=CARTESIAN_POINT('Ctrl Pts',(1.65939064804189,-6.56038959797291,124.276039345327));
#39377=CARTESIAN_POINT('Ctrl Pts',(1.83972470263655,-6.51477574543428,124.284789147688));
#39378=CARTESIAN_POINT('Ctrl Pts',(2.01817678125248,-6.46172209820287,124.293538950049));
#39379=CARTESIAN_POINT('Ctrl Pts',(2.1941407234709,-6.40140886724216,124.30228875241));
#39380=CARTESIAN_POINT('Ctrl Pts',(2.37010298131508,-6.34109621361594,124.311038471015));
#39381=CARTESIAN_POINT('Ctrl Pts',(2.54357687926326,-6.27352420826209,124.319788189621));
#39382=CARTESIAN_POINT('Ctrl Pts',(2.71397317789386,-6.19892237325752,124.328537908226));
#39383=CARTESIAN_POINT('Ctrl Pts',(2.88436790206616,-6.12432122757239,124.337287545985));
#39384=CARTESIAN_POINT('Ctrl Pts',(3.05168482125673,-6.04269049717712,124.346037183743));
#39385=CARTESIAN_POINT('Ctrl Pts',(3.21535561996807,-5.95430745235244,124.354786821501));
#39386=CARTESIAN_POINT('Ctrl Pts',(3.37902496074706,-5.86592519481847,124.36353638132));
#39387=CARTESIAN_POINT('Ctrl Pts',(3.53904799384309,-5.77079087940579,124.372285941139));
#39388=CARTESIAN_POINT('Ctrl Pts',(3.69488118814427,-5.66922763747387,124.381035500958));
#39389=CARTESIAN_POINT('Ctrl Pts',(3.85071304610288,-5.56766526649429,124.389784985746));
#39390=CARTESIAN_POINT('Ctrl Pts',(4.00235489705435,-5.45967423581104,124.398534470533));
#39391=CARTESIAN_POINT('Ctrl Pts',(4.14929168607134,-5.34562133936732,124.407283955321));
#39392=CARTESIAN_POINT('Ctrl Pts',(4.29622726385239,-5.23156938308956,124.416033367984));
#39393=CARTESIAN_POINT('Ctrl Pts',(4.43845763091551,-5.11145583677649,124.424782780647));
#39394=CARTESIAN_POINT('Ctrl Pts',(4.5754997066045,-4.98568866204681,124.43353219331));
#39395=CARTESIAN_POINT('Ctrl Pts',(4.71254069814799,-4.85992248226643,124.442281536757));
#39396=CARTESIAN_POINT('Ctrl Pts',(4.84439326930833,-4.72850295734495,124.451030880203));
#39397=CARTESIAN_POINT('Ctrl Pts',(4.97060959434234,-4.59187644222184,124.459780223649));
#39398=CARTESIAN_POINT('Ctrl Pts',(5.09682496280061,-4.45525096257183,124.468529500786));
#39399=CARTESIAN_POINT('Ctrl Pts',(5.21740397615396,-4.31341878218862,124.477278777922));
#39400=CARTESIAN_POINT('Ctrl Pts',(5.33193710451502,-4.1668616143923,124.486028055058));
#39401=CARTESIAN_POINT('Ctrl Pts',(5.44646940288971,-4.02030550865072,124.494777268791));
#39402=CARTESIAN_POINT('Ctrl Pts',(5.55495572749272,-3.86902470980697,124.503526482524));
#39403=CARTESIAN_POINT('Ctrl Pts',(5.65702762491083,-3.7135330146635,124.512275696257));
#39404=CARTESIAN_POINT('Ctrl Pts',(5.75909881654798,-3.55804239467469,124.521024849493));
#39405=CARTESIAN_POINT('Ctrl Pts',(5.85475551250444,-3.39834117620136,124.529774002729));
#39406=CARTESIAN_POINT('Ctrl Pts',(5.94367283727774,-3.23497174692558,124.538523155966));
#39407=CARTESIAN_POINT('Ctrl Pts',(6.03258957676015,-3.07160339301549,124.547272251611));
#39408=CARTESIAN_POINT('Ctrl Pts',(6.11476689685011,-2.9045671283008,124.556021347257));
#39409=CARTESIAN_POINT('Ctrl Pts',(6.1899257052501,-2.73443024476471,124.564770442902));
#39410=CARTESIAN_POINT('Ctrl Pts',(6.2650840438847,-2.56429442463586,124.573519483863));
#39411=CARTESIAN_POINT('Ctrl Pts',(6.3332238428311,-2.39105828656536,124.582268524824));
#39412=CARTESIAN_POINT('Ctrl Pts',(6.39411368719849,-2.21531017132612,124.591017565785));
#39413=CARTESIAN_POINT('Ctrl Pts',(6.45500317120724,-2.03956309620041,124.599766554968));
#39414=CARTESIAN_POINT('Ctrl Pts',(6.50864269269924,-1.86130434439155,124.60851554415));
#39415=CARTESIAN_POINT('Ctrl Pts',(6.55485008446201,-1.68113930720461,124.617264533333));
#39416=CARTESIAN_POINT('Ctrl Pts',(6.60199664749287,-1.49731239212355,124.626191346862));
#39417=CARTESIAN_POINT('Ctrl Pts',(6.64140563640805,-1.31150116500184,124.635118160391));
#39418=CARTESIAN_POINT('Ctrl Pts',(6.67293772282086,-1.1243625515617,124.644044973921));
#39419=CARTESIAN_POINT('Ctrl Pts',(6.703844949498,-0.940932395056396,124.652794888076));
#39420=CARTESIAN_POINT('Ctrl Pts',(6.72718449348874,-0.756227260511717,
124.661544802232));
#39421=CARTESIAN_POINT('Ctrl Pts',(6.7428770737389,-0.570874564546637,124.670294716387));
#39422=CARTESIAN_POINT('Ctrl Pts',(6.75856934538642,-0.385525513637384,
124.679044458471));
#39423=CARTESIAN_POINT('Ctrl Pts',(6.76661493004089,-0.199529212423096,
124.687794200555));
#39424=CARTESIAN_POINT('Ctrl Pts',(6.76698649908906,-0.0135174386052461,
124.696543942639));
#39425=CARTESIAN_POINT('Ctrl Pts',(6.76735806132402,0.17249092444091,124.705293524285));
#39426=CARTESIAN_POINT('Ctrl Pts',(6.76005588896315,0.358514472896495,124.714043105931));
#39427=CARTESIAN_POINT('Ctrl Pts',(6.74510478454624,0.543921359657261,124.722792687577));
#39428=CARTESIAN_POINT('Ctrl Pts',(6.73015393440741,0.729325093145562,124.731542120416));
#39429=CARTESIAN_POINT('Ctrl Pts',(6.70755443556963,0.914111900251542,124.740291553255));
#39430=CARTESIAN_POINT('Ctrl Pts',(6.67738304682396,1.09765415591065,124.749040986094));
#39431=CARTESIAN_POINT('Ctrl Pts',(6.64721213111952,1.28119353390797,124.757790281755));
#39432=CARTESIAN_POINT('Ctrl Pts',(6.609469609556,1.46348811672175,124.766539577417));
#39433=CARTESIAN_POINT('Ctrl Pts',(6.56428366991303,1.64391876347743,124.775288873078));
#39434=CARTESIAN_POINT('Ctrl Pts',(6.51909837867848,1.8243468210925,124.784038043189));
#39435=CARTESIAN_POINT('Ctrl Pts',(6.46646995272061,2.00291071819993,124.7927872133));
#39436=CARTESIAN_POINT('Ctrl Pts',(6.40657713281698,2.17900400212265,124.80153638341));
#39437=CARTESIAN_POINT('Ctrl Pts',(6.34668509279221,2.35509499309223,124.810285439596));
#39438=CARTESIAN_POINT('Ctrl Pts',(6.27952894037699,2.52871516397691,124.819034495782));
#39439=CARTESIAN_POINT('Ctrl Pts',(6.20533675061632,2.69927486770993,124.827783551968));
#39440=CARTESIAN_POINT('Ctrl Pts',(6.12832117908109,2.87632521635515,124.83686555325));
#39441=CARTESIAN_POINT('Ctrl Pts',(6.04372366626276,3.05007728919607,124.845947554532));
#39442=CARTESIAN_POINT('Ctrl Pts',(5.95185378008069,3.21989527477824,124.855029555815));
#39443=CARTESIAN_POINT('Ctrl Pts',(5.86334450817578,3.38350129286393,124.863779336122));
#39444=CARTESIAN_POINT('Ctrl Pts',(5.76808562057468,3.54345567124616,124.872529116429));
#39445=CARTESIAN_POINT('Ctrl Pts',(5.66640068804701,3.69921508464976,124.881278896736));
#39446=CARTESIAN_POINT('Ctrl Pts',(5.56471941108154,3.8549688985195,124.890028362489));
#39447=CARTESIAN_POINT('Ctrl Pts',(5.45661270815357,4.00652780919305,124.898777828243));
#39448=CARTESIAN_POINT('Ctrl Pts',(5.34244776449371,4.15337704568899,124.907527293996));
#39449=CARTESIAN_POINT('Ctrl Pts',(5.22828631819854,4.30022178355936,124.916276491716));
#39450=CARTESIAN_POINT('Ctrl Pts',(5.10806717844328,4.44235690972381,124.925025689436));
#39451=CARTESIAN_POINT('Ctrl Pts',(4.98219864544978,4.57929969070363,124.933774887155));
#39452=CARTESIAN_POINT('Ctrl Pts',(4.85633329944293,4.71623900429725,124.942523863345));
#39453=CARTESIAN_POINT('Ctrl Pts',(4.72481904033925,4.84798602483347,124.951272839536));
#39454=CARTESIAN_POINT('Ctrl Pts',(4.58810250737484,4.97409332258863,124.960021815726));
#39455=CARTESIAN_POINT('Ctrl Pts',(4.45137708685929,5.10020881821885,124.968771360662));
#39456=CARTESIAN_POINT('Ctrl Pts',(4.30944892636339,5.22068366307696,124.977520905598));
#39457=CARTESIAN_POINT('Ctrl Pts',(4.16280009466949,5.33510865604625,124.986270450534));
#39458=CARTESIAN_POINT('Ctrl Pts',(4.0161598834906,5.44952692272693,124.995019481143));
#39459=CARTESIAN_POINT('Ctrl Pts',(3.86479978232483,5.55789587288452,125.003768511751));
#39460=CARTESIAN_POINT('Ctrl Pts',(3.70923383581298,5.65984746713726,125.012517542359));
#39461=CARTESIAN_POINT('Ctrl Pts',(3.55366577799778,5.76180044505236,125.021266691707));
#39462=CARTESIAN_POINT('Ctrl Pts',(3.39389200027085,5.85733573570917,125.030015841055));
#39463=CARTESIAN_POINT('Ctrl Pts',(3.23045513626293,5.94612887621791,125.038764990403));
#39464=CARTESIAN_POINT('Ctrl Pts',(3.18695122151752,5.96976399206596,125.041093854516));
#39465=CARTESIAN_POINT('Ctrl Pts',(3.14318791262759,5.99292165435284,125.043422718629));
#39466=CARTESIAN_POINT('Ctrl Pts',(3.09917575053273,6.01559628526632,125.045751582742));
#39467=CARTESIAN_POINT('Ctrl Pts',(3.09917575053267,6.01559628526635,123.045751582742));
#39468=CARTESIAN_POINT('Ctrl Pts',(2.93382384459276,6.10078395293754,123.054501030655));
#39469=CARTESIAN_POINT('Ctrl Pts',(2.76495772122998,6.17915010267043,123.063250478567));
#39470=CARTESIAN_POINT('Ctrl Pts',(2.59315093316728,6.2504285643317,123.07199992648));
#39471=CARTESIAN_POINT('Ctrl Pts',(2.42134553245636,6.32170645041444,123.08074930374));
#39472=CARTESIAN_POINT('Ctrl Pts',(2.24659977927612,6.3858966531345,123.089498681));
#39473=CARTESIAN_POINT('Ctrl Pts',(2.06950718689942,6.44278115439068,123.09824805826));
#39474=CARTESIAN_POINT('Ctrl Pts',(1.89241596572886,6.49966521519717,123.106997367774));
#39475=CARTESIAN_POINT('Ctrl Pts',(1.71297821457224,6.54924360009539,123.115746677289));
#39476=CARTESIAN_POINT('Ctrl Pts',(1.53180337335873,6.59134792173549,123.124495986804));
#39477=CARTESIAN_POINT('Ctrl Pts',(1.3506298747782,6.63345193135297,123.13324523148));
#39478=CARTESIAN_POINT('Ctrl Pts',(1.16771959102998,6.6680819236823,123.141994476156));
#39479=CARTESIAN_POINT('Ctrl Pts',(0.983693746907394,6.6951202836316,123.150743720832));
#39480=CARTESIAN_POINT('Ctrl Pts',(0.799669205420503,6.72215845218859,123.159492903576));
#39481=CARTESIAN_POINT('Ctrl Pts',(0.614529402874191,6.74160505424572,123.16824208632));
#39482=CARTESIAN_POINT('Ctrl Pts',(0.428903127364045,6.75339404354117,123.176991269065));
#39483=CARTESIAN_POINT('Ctrl Pts',(0.243278104164782,6.76518295330327,123.185740392783));
#39484=CARTESIAN_POINT('Ctrl Pts',(0.0571669005401258,6.76931433552275,
123.194489516502));
#39485=CARTESIAN_POINT('Ctrl Pts',(-0.128798404776401,6.76577415902475,
123.20323864022));
#39486=CARTESIAN_POINT('Ctrl Pts',(-0.314762517257868,6.76223400523447,
123.21198770782));
#39487=CARTESIAN_POINT('Ctrl Pts',(-0.500580446818165,6.75102239665099,
123.220736775419));
#39488=CARTESIAN_POINT('Ctrl Pts',(-0.685621118841152,6.73217741012512,
123.229485843018));
#39489=CARTESIAN_POINT('Ctrl Pts',(-0.87066066541316,6.71333253821789,123.238234857404));
#39490=CARTESIAN_POINT('Ctrl Pts',(-1.05492267885367,6.68685441030631,123.24698387179));
#39491=CARTESIAN_POINT('Ctrl Pts',(-1.23778137635145,6.65283295028197,123.255732886175));
#39492=CARTESIAN_POINT('Ctrl Pts',(-1.42999922976776,6.61707018862254,123.264929696542));
#39493=CARTESIAN_POINT('Ctrl Pts',(-1.62066601229693,6.5729717293534,123.274126506908));
#39494=CARTESIAN_POINT('Ctrl Pts',(-1.80906628494505,6.52070304312926,123.283323317275));
#39495=CARTESIAN_POINT('Ctrl Pts',(-1.98831342539696,6.47097374916823,123.292073315012));
#39496=CARTESIAN_POINT('Ctrl Pts',(-2.16550875890926,6.41384933991479,123.30082331275));
#39497=CARTESIAN_POINT('Ctrl Pts',(-2.34005036708298,6.34952386242581,123.309573310488));
#39498=CARTESIAN_POINT('Ctrl Pts',(-2.51458843541424,6.28519968950862,123.318323130769));
#39499=CARTESIAN_POINT('Ctrl Pts',(-2.68647261712446,6.21367483973524,123.32707295105));
#39500=CARTESIAN_POINT('Ctrl Pts',(-2.85511905903184,6.13519226746425,123.335822771331));
#39501=CARTESIAN_POINT('Ctrl Pts',(-3.02376230483394,6.05671118255677,123.344572425789));
#39502=CARTESIAN_POINT('Ctrl Pts',(-3.18916767374478,5.97127275995531,123.353322080248));
#39503=CARTESIAN_POINT('Ctrl Pts',(-3.35077334097431,5.87916720441049,123.362071734706));
#39504=CARTESIAN_POINT('Ctrl Pts',(-3.51237616032097,5.78706327198842,123.370821234975));
#39505=CARTESIAN_POINT('Ctrl Pts',(-3.67017916297119,5.68829258365641,123.379570735243));
#39506=CARTESIAN_POINT('Ctrl Pts',(-3.82364636561378,5.58319061744524,123.388320235511));
#39507=CARTESIAN_POINT('Ctrl Pts',(-3.97711106773808,5.47809036371325,123.39706959322));
#39508=CARTESIAN_POINT('Ctrl Pts',(-4.12623987477037,5.36665920046984,123.405818950928));
#39509=CARTESIAN_POINT('Ctrl Pts',(-4.27052628209146,5.24927559516227,123.414568308637));
#39510=CARTESIAN_POINT('Ctrl Pts',(-4.41481053020291,5.13189374647068,123.423317535413));
#39511=CARTESIAN_POINT('Ctrl Pts',(-4.55425230131945,5.00855981481522,123.43206676219));
#39512=CARTESIAN_POINT('Ctrl Pts',(-4.68837800626071,4.87969268196378,123.440815988966));
#39513=CARTESIAN_POINT('Ctrl Pts',(-4.82250188224545,4.75082730636225,123.449565096437));
#39514=CARTESIAN_POINT('Ctrl Pts',(-4.95130963048748,4.6164290790805,123.458314203908));
#39515=CARTESIAN_POINT('Ctrl Pts',(-5.07436379029284,4.47695444736317,123.467063311379));
#39516=CARTESIAN_POINT('Ctrl Pts',(-5.19741643558843,4.33748153225334,123.475812311169));
#39517=CARTESIAN_POINT('Ctrl Pts',(-5.31471544458936,4.19293255259452,123.484561310958));
#39518=CARTESIAN_POINT('Ctrl Pts',(-5.4258624527192,4.04379841784577,123.493310310748));
#39519=CARTESIAN_POINT('Ctrl Pts',(-5.53702160015578,3.89464799489424,123.50206026609));
#39520=CARTESIAN_POINT('Ctrl Pts',(-5.64202723077814,3.74091164449034,123.510810221432));
#39521=CARTESIAN_POINT('Ctrl Pts',(-5.74052265229671,3.58311159168513,123.519560176775));
#39522=CARTESIAN_POINT('Ctrl Pts',(-5.83901427063769,3.42531763197151,123.528309794257));
#39523=CARTESIAN_POINT('Ctrl Pts',(-5.93099603112741,3.26346052701063,123.537059411739));
#39524=CARTESIAN_POINT('Ctrl Pts',(-6.01615550619908,3.09809004472602,123.545809029222));
#39525=CARTESIAN_POINT('Ctrl Pts',(-6.10131214576109,2.93272506869425,123.554558355373));
#39526=CARTESIAN_POINT('Ctrl Pts',(-6.17964682326215,2.76384720422556,123.563307681524));
#39527=CARTESIAN_POINT('Ctrl Pts',(-6.25089348286192,2.59203002797313,123.572057007675));
#39528=CARTESIAN_POINT('Ctrl Pts',(-6.32213814887107,2.42021765942834,123.580806089007));
#39529=CARTESIAN_POINT('Ctrl Pts',(-6.38629508410515,2.24546640837803,123.589555170338));
#39530=CARTESIAN_POINT('Ctrl Pts',(-6.44314639817899,2.06836976666,123.59830425167));
#39531=CARTESIAN_POINT('Ctrl Pts',(-6.50000285281951,1.89125711164286,123.607054124104));
#39532=CARTESIAN_POINT('Ctrl Pts',(-6.54955227671666,1.71179891446311,123.615803996539));
#39533=CARTESIAN_POINT('Ctrl Pts',(-6.5916263592497,1.53060476284526,123.624553868973));
#39534=CARTESIAN_POINT('Ctrl Pts',(-6.63369752053947,1.34942319170836,123.633303133896));
#39535=CARTESIAN_POINT('Ctrl Pts',(-6.66829431423173,1.16650618648884,123.642052398818));
#39536=CARTESIAN_POINT('Ctrl Pts',(-6.69529923744506,0.982474997680675,
123.65080166374));
#39537=CARTESIAN_POINT('Ctrl Pts',(-6.72230554730701,0.798434359240222,
123.65955137792));
#39538=CARTESIAN_POINT('Ctrl Pts',(-6.74171916496132,0.613279706303111,
123.6683010921));
#39539=CARTESIAN_POINT('Ctrl Pts',(-6.75347414816876,0.427639953718374,
123.67705080628));
#39540=CARTESIAN_POINT('Ctrl Pts',(-6.76248837756593,0.285283364559399,
123.683760465441));
#39541=CARTESIAN_POINT('Ctrl Pts',(-6.76699999997977,0.142641701764922,
123.690470124603));
#39542=CARTESIAN_POINT('Ctrl Pts',(-6.767,9.59715867638603E-10,123.697179783765));
#39543=CARTESIAN_POINT('',(-6.766999991942,0.000330237817373678,123.302820216223));
#39544=CARTESIAN_POINT('Ctrl Pts',(3.0991757505325,6.01559628526643,122.651206263353));
#39545=CARTESIAN_POINT('Ctrl Pts',(2.96868116764643,6.08282580461548,122.658141446023));
#39546=CARTESIAN_POINT('Ctrl Pts',(2.83615539198715,6.14572607912599,122.665076628692));
#39547=CARTESIAN_POINT('Ctrl Pts',(2.70191747454246,6.20418656721106,122.672011811362));
#39548=CARTESIAN_POINT('Ctrl Pts',(2.54255793686262,6.27358749752281,122.680244861494));
#39549=CARTESIAN_POINT('Ctrl Pts',(2.38028978695587,6.33694602721171,122.688477911626));
#39550=CARTESIAN_POINT('Ctrl Pts',(2.21561077191667,6.39400953294307,122.696710961758));
#39551=CARTESIAN_POINT('Ctrl Pts',(2.05112786427039,6.45100508481075,122.704934207593));
#39552=CARTESIAN_POINT('Ctrl Pts',(1.88424014342203,6.50172042379528,122.713157453427));
#39553=CARTESIAN_POINT('Ctrl Pts',(1.71546768173177,6.54594986483504,122.721380699262));
#39554=CARTESIAN_POINT('Ctrl Pts',(1.54686242192798,6.59013548802735,122.729595798376));
#39555=CARTESIAN_POINT('Ctrl Pts',(1.37637648393742,6.62784791964217,122.737810897489));
#39556=CARTESIAN_POINT('Ctrl Pts',(1.20454764095067,6.65893039313974,122.746025996603));
#39557=CARTESIAN_POINT('Ctrl Pts',(1.03285464829981,6.68998829239011,122.754234600742));
#39558=CARTESIAN_POINT('Ctrl Pts',(0.859821216261961,6.71442661054856,122.762443204881));
#39559=CARTESIAN_POINT('Ctrl Pts',(0.685998021285147,6.7321390148149,122.77065180902));
#39560=CARTESIAN_POINT('Ctrl Pts',(0.512277483922408,6.74984095837625,122.778855565268));
#39561=CARTESIAN_POINT('Ctrl Pts',(0.3377684681806,6.76082486506108,122.787059321517));
#39562=CARTESIAN_POINT('Ctrl Pts',(0.163029630048409,6.76503587128156,122.795263077766));
#39563=CARTESIAN_POINT('Ctrl Pts',(-0.01165750726604,6.76924563157145,122.803464406731));
#39564=CARTESIAN_POINT('Ctrl Pts',(-0.186573973989754,6.76668647067645,
122.811665735695));
#39565=CARTESIAN_POINT('Ctrl Pts',(-0.361157976604668,6.75735554162535,
122.819867064659));
#39566=CARTESIAN_POINT('Ctrl Pts',(-0.535717902419002,6.74802589939844,
122.828067262582));
#39567=CARTESIAN_POINT('Ctrl Pts',(-0.709945097750385,6.73192636731659,
122.836267460505));
#39568=CARTESIAN_POINT('Ctrl Pts',(-0.883279734910622,6.70910619307045,
122.844467658427));
#39569=CARTESIAN_POINT('Ctrl Pts',(-1.05662187933245,6.68628503046433,122.852668211507));
#39570=CARTESIAN_POINT('Ctrl Pts',(-1.22907103332113,6.6567426925079,122.860868764587));
#39571=CARTESIAN_POINT('Ctrl Pts',(-1.40007438230559,6.6205800896909,122.869069317667));
#39572=CARTESIAN_POINT('Ctrl Pts',(-1.57111612673847,6.58440936727064,122.87727171202));
#39573=CARTESIAN_POINT('Ctrl Pts',(-1.74071106914144,6.5416154935125,122.885474106373));
#39574=CARTESIAN_POINT('Ctrl Pts',(-1.90831838714597,6.49235010864946,122.893676500726));
#39575=CARTESIAN_POINT('Ctrl Pts',(-2.07608244745648,6.44303865199121,122.90188656576));
#39576=CARTESIAN_POINT('Ctrl Pts',(-2.24185482549696,6.38724369400404,122.910096630794));
#39577=CARTESIAN_POINT('Ctrl Pts',(-2.40511072476101,6.32516651177181,122.918306695828));
#39578=CARTESIAN_POINT('Ctrl Pts',(-2.56844475540239,6.26305962050138,122.926520690053));
#39579=CARTESIAN_POINT('Ctrl Pts',(-2.72925957648426,6.19466465054113,122.934734684279));
#39580=CARTESIAN_POINT('Ctrl Pts',(-2.88705214789691,6.12023029757246,122.942948678504));
#39581=CARTESIAN_POINT('Ctrl Pts',(-3.04505984313874,6.04569446578961,122.951173871139));
#39582=CARTESIAN_POINT('Ctrl Pts',(-3.20003673621005,5.96510296120563,122.959399063774));
#39583=CARTESIAN_POINT('Ctrl Pts',(-3.35150501644361,5.87875013287292,122.967624256409));
#39584=CARTESIAN_POINT('Ctrl Pts',(-3.48772011644028,5.80109321930529,122.975021154529));
#39585=CARTESIAN_POINT('Ctrl Pts',(-3.62109788751653,5.71877760673496,122.982418052649));
#39586=CARTESIAN_POINT('Ctrl Pts',(-3.75131258146814,5.63204606835907,122.989814950769));
#39587=CARTESIAN_POINT('Ctrl Pts',(-3.90351582426913,5.53066871229175,122.99846091726));
#39588=CARTESIAN_POINT('Ctrl Pts',(-4.0517427285922,5.42302764116862,123.007106883751));
#39589=CARTESIAN_POINT('Ctrl Pts',(-4.19547607149495,5.30945096347196,123.015752850242));
#39590=CARTESIAN_POINT('Ctrl Pts',(-4.33902555991244,5.19601956578614,123.024387757366));
#39591=CARTESIAN_POINT('Ctrl Pts',(-4.47809271039161,5.07666788947707,123.033022664491));
#39592=CARTESIAN_POINT('Ctrl Pts',(-4.61218953336684,4.95176702887983,123.041657571615));
#39593=CARTESIAN_POINT('Ctrl Pts',(-4.75073826263271,4.82271956052067,123.050579150687));
#39594=CARTESIAN_POINT('Ctrl Pts',(-4.88398068823489,4.68774827252662,123.059500729758));
#39595=CARTESIAN_POINT('Ctrl Pts',(-5.01141360740328,4.54730938638809,123.06842230883));
#39596=CARTESIAN_POINT('Ctrl Pts',(-5.13441115902607,4.41175854708852,123.077033367805));
#39597=CARTESIAN_POINT('Ctrl Pts',(-5.25199653218815,4.2711145284883,123.085644426781));
#39598=CARTESIAN_POINT('Ctrl Pts',(-5.36375252695179,4.1258269267649,123.094255485757));
#39599=CARTESIAN_POINT('Ctrl Pts',(-5.47540313065247,3.98067633795801,123.102858424106));
#39600=CARTESIAN_POINT('Ctrl Pts',(-5.58123513095635,3.83089113775599,123.111461362456));
#39601=CARTESIAN_POINT('Ctrl Pts',(-5.68087051348509,3.67695515461035,123.120064300805));
#39602=CARTESIAN_POINT('Ctrl Pts',(-5.78039432743483,3.52319154415464,123.128657605854));
#39603=CARTESIAN_POINT('Ctrl Pts',(-5.87373520092814,3.36528667868517,123.137250910903));
#39604=CARTESIAN_POINT('Ctrl Pts',(-5.96055737582634,3.20375479234636,123.145844215951));
#39605=CARTESIAN_POINT('Ctrl Pts',(-5.97023078724505,3.18575749619905,123.146801650792));
#39606=CARTESIAN_POINT('Ctrl Pts',(-5.97982332173152,3.1677152062004,123.147759085632));
#39607=CARTESIAN_POINT('Ctrl Pts',(-5.98933454802696,3.14962865617691,123.148716520473));
#39608=CARTESIAN_POINT('Ctrl Pts',(-6.0740841776925,2.98846874169211,123.157247728295));
#39609=CARTESIAN_POINT('Ctrl Pts',(-6.15228050461095,2.82397133033367,123.165778936117));
#39610=CARTESIAN_POINT('Ctrl Pts',(-6.2236859368796,2.65669387756421,123.174310143939));
#39611=CARTESIAN_POINT('Ctrl Pts',(-6.29514980765615,2.4892795242196,123.182848333738));
#39612=CARTESIAN_POINT('Ctrl Pts',(-6.35981156980806,2.3190808789042,123.191386523536));
#39613=CARTESIAN_POINT('Ctrl Pts',(-6.41748259220156,2.14667328179906,123.199924713335));
#39614=CARTESIAN_POINT('Ctrl Pts',(-6.47539971699918,1.97352996123396,123.208499338573));
#39615=CARTESIAN_POINT('Ctrl Pts',(-6.526266216052,1.7981591019537,123.21707396381));
#39616=CARTESIAN_POINT('Ctrl Pts',(-6.56994244704369,1.62115552694169,123.225648589048));
#39617=CARTESIAN_POINT('Ctrl Pts',(-6.61354175832605,1.44446367900022,123.23420811322));
#39618=CARTESIAN_POINT('Ctrl Pts',(-6.64997609272299,1.26614518054161,123.242767637391));
#39619=CARTESIAN_POINT('Ctrl Pts',(-6.67915839676466,1.08679902048545,123.251327161562));
#39620=CARTESIAN_POINT('Ctrl Pts',(-6.70841792774907,0.906978245552623,
123.259909337333));
#39621=CARTESIAN_POINT('Ctrl Pts',(-6.73038697429634,0.726124680428343,
123.268491513104));
#39622=CARTESIAN_POINT('Ctrl Pts',(-6.74503026730746,0.544844650433756,
123.277073688876));
#39623=CARTESIAN_POINT('Ctrl Pts',(-6.75967356031858,0.363564620439041,
123.285655864647));
#39624=CARTESIAN_POINT('Ctrl Pts',(-6.76699113312658,0.181858442082662,
123.294238040419));
#39625=CARTESIAN_POINT('Ctrl Pts',(-6.76699999194196,0.000330238511045327,
123.30282021619));
#39626=CARTESIAN_POINT('Ctrl Pts',(-6.766999991942,0.00033023781756751,
123.302820216223));
#39627=CARTESIAN_POINT('Ctrl Pts',(-6.76700164278173,-0.033497603479895,
123.304419507541));
#39628=CARTESIAN_POINT('Ctrl Pts',(-6.76674963937631,-0.0673246409772959,
123.306018798859));
#39629=CARTESIAN_POINT('Ctrl Pts',(-6.76624401275958,-0.101148207078348,
123.307618090177));
#39630=CARTESIAN_POINT('Ctrl Pts',(-6.76364331035425,-0.275120515509138,
123.315844082718));
#39631=CARTESIAN_POINT('Ctrl Pts',(-6.75432517494951,-0.449220794044856,
123.32407007526));
#39632=CARTESIAN_POINT('Ctrl Pts',(-6.73827102947005,-0.62289046661881,
123.332296067801));
#39633=CARTESIAN_POINT('Ctrl Pts',(-6.72223371468706,-0.79637806898869,
123.340513436452));
#39634=CARTESIAN_POINT('Ctrl Pts',(-6.69947448526771,-0.969435610532295,
123.348730805104));
#39635=CARTESIAN_POINT('Ctrl Pts',(-6.67002676664729,-1.1415042409946,123.356948173755));
#39636=CARTESIAN_POINT('Ctrl Pts',(-6.64060402779263,-1.31342690992635,
123.365158571818));
#39637=CARTESIAN_POINT('Ctrl Pts',(-6.60450415972966,-1.48436198732553,
123.37336896988));
#39638=CARTESIAN_POINT('Ctrl Pts',(-6.56181241397131,-1.65375537606142,
123.381579367942));
#39639=CARTESIAN_POINT('Ctrl Pts',(-6.51914834252906,-1.82303895794583,
123.389784443731));
#39640=CARTESIAN_POINT('Ctrl Pts',(-6.46990099232645,-1.99078249567337,
123.39798951952));
#39641=CARTESIAN_POINT('Ctrl Pts',(-6.41420677020203,-2.15644163127465,
123.406194595309));
#39642=CARTESIAN_POINT('Ctrl Pts',(-6.35853751229379,-2.32202651230668,
123.414395993278));
#39643=CARTESIAN_POINT('Ctrl Pts',(-6.29642725358434,-2.48552851372514,
123.422597391248));
#39644=CARTESIAN_POINT('Ctrl Pts',(-6.22806239781778,-2.64641791274323,
123.430798789217));
#39645=CARTESIAN_POINT('Ctrl Pts',(-6.15970289695587,-2.80729470956417,
123.438999544785));
#39646=CARTESIAN_POINT('Ctrl Pts',(-6.08508990686431,-2.96555897870409,
123.447200300352));
#39647=CARTESIAN_POINT('Ctrl Pts',(-6.00445831727879,-3.12070013235197,
123.45540105592));
#39648=CARTESIAN_POINT('Ctrl Pts',(-5.92382713726337,-3.27584049795663,
123.463601769832));
#39649=CARTESIAN_POINT('Ctrl Pts',(-5.83717758297189,-3.42785746118635,
123.471802483744));
#39650=CARTESIAN_POINT('Ctrl Pts',(-5.74479087999741,-3.57626435615414,
123.480003197656));
#39651=CARTESIAN_POINT('Ctrl Pts',(-5.65238790353241,-3.72469739231022,
123.488205356085));
#39652=CARTESIAN_POINT('Ctrl Pts',(-5.55424595439009,-3.8695187890467,123.496407514515));
#39653=CARTESIAN_POINT('Ctrl Pts',(-5.45069005157621,-4.01027018561694,
123.504609672944));
#39654=CARTESIAN_POINT('Ctrl Pts',(-5.34709714076258,-4.151071882822,123.512814762597));
#39655=CARTESIAN_POINT('Ctrl Pts',(-5.23808663429509,-4.28780039392327,
123.52101985225));
#39656=CARTESIAN_POINT('Ctrl Pts',(-5.12402437777205,-4.42002977094021,
123.529224941903));
#39657=CARTESIAN_POINT('Ctrl Pts',(-5.00983181860643,-4.552410204387,123.537439404901));
#39658=CARTESIAN_POINT('Ctrl Pts',(-4.89057621420478,-4.68028096383782,
123.545653867899));
#39659=CARTESIAN_POINT('Ctrl Pts',(-4.76666161661593,-4.80325161038649,
123.553868330897));
#39660=CARTESIAN_POINT('Ctrl Pts',(-4.64267360354444,-4.92629511315664,
123.562087660704));
#39661=CARTESIAN_POINT('Ctrl Pts',(-4.51402135845631,-5.04443247392336,
123.570306990512));
#39662=CARTESIAN_POINT('Ctrl Pts',(-4.38114258680509,-5.15731312158597,
123.578526320319));
#39663=CARTESIAN_POINT('Ctrl Pts',(-4.24805792755352,-5.27036867096828,
123.58675838548));
#39664=CARTESIAN_POINT('Ctrl Pts',(-4.11073393650097,-5.37815100933363,
123.59499045064));
#39665=CARTESIAN_POINT('Ctrl Pts',(-3.96963898802552,-5.48035175009303,
123.603222515801));
#39666=CARTESIAN_POINT('Ctrl Pts',(-3.8428127171619,-5.57221711430392,123.610622087062));
#39667=CARTESIAN_POINT('Ctrl Pts',(-3.71294016052135,-5.65957320741325,
123.618021658324));
#39668=CARTESIAN_POINT('Ctrl Pts',(-3.5803780409309,-5.74222797213937,123.625421229585));
#39669=CARTESIAN_POINT('Ctrl Pts',(-3.43427432566459,-5.83332615500079,
123.633576687991));
#39670=CARTESIAN_POINT('Ctrl Pts',(-3.28445321693816,-5.91899315122175,
123.641732146398));
#39671=CARTESIAN_POINT('Ctrl Pts',(-3.13135933964687,-5.99890637416574,
123.649887604805));
#39672=CARTESIAN_POINT('Ctrl Pts',(-2.97845179772811,-6.07872233221298,
123.658033136947));
#39673=CARTESIAN_POINT('Ctrl Pts',(-2.82227973681938,-6.15279828969649,
123.666178669089));
#39674=CARTESIAN_POINT('Ctrl Pts',(-2.66331727159753,-6.22085445182656,
123.674324201231));
#39675=CARTESIAN_POINT('Ctrl Pts',(-2.50451485797348,-6.28884209150717,
123.682461532031));
#39676=CARTESIAN_POINT('Ctrl Pts',(-2.34292796678921,-6.35082185951427,
123.690598862832));
#39677=CARTESIAN_POINT('Ctrl Pts',(-2.17905586686755,-6.40655949235392,
123.698736193632));
#39678=CARTESIAN_POINT('Ctrl Pts',(-2.01531432358844,-6.46225271910974,
123.706867041434));
#39679=CARTESIAN_POINT('Ctrl Pts',(-1.84929154108083,-6.51171359560858,
123.714997889236));
#39680=CARTESIAN_POINT('Ctrl Pts',(-1.68150735197763,-6.55475568005743,
123.723128737038));
#39681=CARTESIAN_POINT('Ctrl Pts',(-1.51382159029733,-6.59777251468107,
123.731254815032));
#39682=CARTESIAN_POINT('Ctrl Pts',(-1.34437683296057,-6.63437796550534,
123.739380893026));
#39683=CARTESIAN_POINT('Ctrl Pts',(-1.17370867829032,-6.66443523027316,
123.74750697102));
#39684=CARTESIAN_POINT('Ctrl Pts',(-1.00243536551594,-6.69459907261191,
123.755661862602));
#39685=CARTESIAN_POINT('Ctrl Pts',(-0.829930317602609,-6.71816809240825,
123.763816754184));
#39686=CARTESIAN_POINT('Ctrl Pts',(-0.656746415364533,-6.7350555414121,
123.771971645766));
#39687=CARTESIAN_POINT('Ctrl Pts',(-0.484237869793059,-6.75187713526937,
123.780094736123));
#39688=CARTESIAN_POINT('Ctrl Pts',(-0.311056123235351,-6.76206915767,123.788217826479));
#39689=CARTESIAN_POINT('Ctrl Pts',(-0.137753630643398,-6.76559775165835,
123.796340916835));
#39690=CARTESIAN_POINT('Ctrl Pts',(0.0355624704512306,-6.76912662272801,
123.804464645054));
#39691=CARTESIAN_POINT('Ctrl Pts',(0.20899897071073,-6.76599101565496,123.812588373272));
#39692=CARTESIAN_POINT('Ctrl Pts',(0.382002756699721,-6.75620921033932,
123.820712101491));
#39693=CARTESIAN_POINT('Ctrl Pts',(0.555053041500488,-6.74642477593483,
123.828838013151));
#39694=CARTESIAN_POINT('Ctrl Pts',(0.727670015361962,-6.72999060703069,
123.836963924811));
#39695=CARTESIAN_POINT('Ctrl Pts',(0.899305070451042,-6.70697691887046,
123.845089836471));
#39696=CARTESIAN_POINT('Ctrl Pts',(1.07203774955942,-6.6838160557821,123.853267714182));
#39697=CARTESIAN_POINT('Ctrl Pts',(1.24377553509034,-6.65399127783878,123.861445591892));
#39698=CARTESIAN_POINT('Ctrl Pts',(1.4139698305962,-6.61762633564058,123.869623469602));
#39699=CARTESIAN_POINT('Ctrl Pts',(1.58335182564263,-6.58143495542439,123.877762316075));
#39700=CARTESIAN_POINT('Ctrl Pts',(1.75120469244766,-6.53876585348229,123.885901162548));
#39701=CARTESIAN_POINT('Ctrl Pts',(1.91700343289675,-6.48979097030576,123.894040009022));
#39702=CARTESIAN_POINT('Ctrl Pts',(2.08399484786531,-6.44046378592898,123.90223740235));
#39703=CARTESIAN_POINT('Ctrl Pts',(2.24890211442958,-6.38473987783791,123.910434795679));
#39704=CARTESIAN_POINT('Ctrl Pts',(2.41121018717397,-6.32284385646748,123.918632189007));
#39705=CARTESIAN_POINT('Ctrl Pts',(2.57351825991824,-6.26094783509708,123.926829582335));
#39706=CARTESIAN_POINT('Ctrl Pts',(2.73322682037374,-6.19287990260906,123.935026975664));
#39707=CARTESIAN_POINT('Ctrl Pts',(2.88984720503379,-6.11891102497482,123.943224368992));
#39708=CARTESIAN_POINT('Ctrl Pts',(3.04701815182596,-6.04468212714545,123.951450578329));
#39709=CARTESIAN_POINT('Ctrl Pts',(3.20154699203705,-5.96428991267037,123.959676787666));
#39710=CARTESIAN_POINT('Ctrl Pts',(3.35291692305904,-5.8779449731232,123.967902997003));
#39711=CARTESIAN_POINT('Ctrl Pts',(3.50411679644857,-5.79169703841639,123.976119964546));
#39712=CARTESIAN_POINT('Ctrl Pts',(3.65216451878241,-5.69950987161253,123.984336932089));
#39713=CARTESIAN_POINT('Ctrl Pts',(3.79656418546999,-5.60164166879734,123.992553899633));
#39714=CARTESIAN_POINT('Ctrl Pts',(3.94083060748751,-5.50386377378335,124.000763284976));
#39715=CARTESIAN_POINT('Ctrl Pts',(4.08145538284242,-5.40041548268226,124.008972670319));
#39716=CARTESIAN_POINT('Ctrl Pts',(4.21796803159714,-5.29160038971431,124.017182055663));
#39717=CARTESIAN_POINT('Ctrl Pts',(4.35438210380969,-5.18286387272958,124.025385512963));
#39718=CARTESIAN_POINT('Ctrl Pts',(4.48668968462899,-5.06876849564165,124.033588970264));
#39719=CARTESIAN_POINT('Ctrl Pts',(4.61445000628577,-4.94966060851542,124.041792427565));
#39720=CARTESIAN_POINT('Ctrl Pts',(4.74214369991099,-4.83061483710681,124.049991606696));
#39721=CARTESIAN_POINT('Ctrl Pts',(4.86529459699136,-4.70656200731514,124.058190785828));
#39722=CARTESIAN_POINT('Ctrl Pts',(4.98349564833184,-4.5778881728432,124.06638996496));
#39723=CARTESIAN_POINT('Ctrl Pts',(5.10167442804651,-4.44923858329514,124.07458759919));
#39724=CARTESIAN_POINT('Ctrl Pts',(5.21490497283096,-4.31596998303971,124.08278523342));
#39725=CARTESIAN_POINT('Ctrl Pts',(5.32281749377134,-4.17850486753358,124.09098286765));
#39726=CARTESIAN_POINT('Ctrl Pts',(5.43072222546795,-4.04104967440982,124.099179910165));
#39727=CARTESIAN_POINT('Ctrl Pts',(5.53330947562752,-3.89939885088064,124.107376952681));
#39728=CARTESIAN_POINT('Ctrl Pts',(5.63025016535381,-3.75400746876367,124.115573995196));
#39729=CARTESIAN_POINT('Ctrl Pts',(5.72720147660268,-3.6086001565161,124.123771935839));
#39730=CARTESIAN_POINT('Ctrl Pts',(5.81850479581267,-3.45945176764502,124.131969876482));
#39731=CARTESIAN_POINT('Ctrl Pts',(5.90387472776674,-3.30704584165947,124.140167817125));
#39732=CARTESIAN_POINT('Ctrl Pts',(5.9892695293673,-3.15459551735456,124.148368145961));
#39733=CARTESIAN_POINT('Ctrl Pts',(6.06872732552163,-2.99888607854712,124.156568474797));
#39734=CARTESIAN_POINT('Ctrl Pts',(6.14200895323333,-2.84042514747382,124.164768803633));
#39735=CARTESIAN_POINT('Ctrl Pts',(6.21536694230291,-2.68179909599794,124.172977677424));
#39736=CARTESIAN_POINT('Ctrl Pts',(6.28253575456501,-2.52041615015348,124.181186551216));
#39737=CARTESIAN_POINT('Ctrl Pts',(6.34332424525404,-2.35680430234931,124.189395425007));
#39738=CARTESIAN_POINT('Ctrl Pts',(6.40414536045541,-2.19310464587141,124.19760870441));
#39739=CARTESIAN_POINT('Ctrl Pts',(6.45857921603039,-2.02717404319272,124.205821983814));
#39740=CARTESIAN_POINT('Ctrl Pts',(6.50648478417683,-1.85955498796765,124.214035263217));
#39741=CARTESIAN_POINT('Ctrl Pts',(6.55446042174608,-1.69169076352939,124.222260555833));
#39742=CARTESIAN_POINT('Ctrl Pts',(6.59588860441139,-1.52213349956341,124.230485848448));
#39743=CARTESIAN_POINT('Ctrl Pts',(6.63067933757173,-1.35143646624593,124.238711141064));
#39744=CARTESIAN_POINT('Ctrl Pts',(6.66214337649842,-1.19706150449338,124.246149930176));
#39745=CARTESIAN_POINT('Ctrl Pts',(6.68817926852513,-1.04175461526081,124.253588719288));
#39746=CARTESIAN_POINT('Ctrl Pts',(6.70875710235929,-0.885927277796426,
124.2610275084));
#39747=CARTESIAN_POINT('Ctrl Pts',(6.73151314438449,-0.713605279835282,
124.269253709419));
#39748=CARTESIAN_POINT('Ctrl Pts',(6.74765729947289,-0.540165090666825,
124.277479910438));
#39749=CARTESIAN_POINT('Ctrl Pts',(6.75708660405581,-0.366155192902602,
124.285706111457));
#39750=CARTESIAN_POINT('Ctrl Pts',(6.76650531680238,-0.192340758583608,
124.293923072072));
#39751=CARTESIAN_POINT('Ctrl Pts',(6.76922417941891,-0.0179582448376579,
124.302140032688));
#39752=CARTESIAN_POINT('Ctrl Pts',(6.76519156342863,0.156435642083491,124.310356993304));
#39753=CARTESIAN_POINT('Ctrl Pts',(6.76116266785444,0.330668636466773,124.318566373105));
#39754=CARTESIAN_POINT('Ctrl Pts',(6.75039470677595,0.504912626840805,124.326775752907));
#39755=CARTESIAN_POINT('Ctrl Pts',(6.73288798451109,0.678607683441808,124.334985132709));
#39756=CARTESIAN_POINT('Ctrl Pts',(6.71539390100989,0.852177343024529,124.343188585849));
#39757=CARTESIAN_POINT('Ctrl Pts',(6.69117078231921,1.02519850280473,124.35139203899));
#39758=CARTESIAN_POINT('Ctrl Pts',(6.66027096730924,1.19711304479471,124.35959549213));
#39759=CARTESIAN_POINT('Ctrl Pts',(6.62938726161657,1.36893796081429,124.36779466848));
#39760=CARTESIAN_POINT('Ctrl Pts',(6.59183385733291,1.53965705623929,124.37599384483));
#39761=CARTESIAN_POINT('Ctrl Pts',(6.54771473279626,1.70871904592966,124.38419302118));
#39762=CARTESIAN_POINT('Ctrl Pts',(6.50360390993851,1.87774922405607,124.392390654732));
#39763=CARTESIAN_POINT('Ctrl Pts',(6.45292991213696,2.04512256931115,124.400588288283));
#39764=CARTESIAN_POINT('Ctrl Pts',(6.39584753416592,2.21029937332111,124.408785921835));
#39765=CARTESIAN_POINT('Ctrl Pts',(6.3387692675271,2.37546428054717,124.416982964955));
#39766=CARTESIAN_POINT('Ctrl Pts',(6.27528365626154,2.53843262230696,124.425180008076));
#39767=CARTESIAN_POINT('Ctrl Pts',(6.20559493137233,2.69868126086168,124.433377051196));
#39768=CARTESIAN_POINT('Ctrl Pts',(6.13589855997216,2.85894748250427,124.441574993728));
#39769=CARTESIAN_POINT('Ctrl Pts',(6.05999786200951,3.01649307741875,124.449772936259));
#39770=CARTESIAN_POINT('Ctrl Pts',(5.97814466214256,3.17081620383404,124.45797087879));
#39771=CARTESIAN_POINT('Ctrl Pts',(5.89626760429474,3.32518431124216,124.466171210798));
#39772=CARTESIAN_POINT('Ctrl Pts',(5.8084347566719,3.4763277624671,124.474371542807));
#39773=CARTESIAN_POINT('Ctrl Pts',(5.71494323247086,3.62377052938448,124.482571874815));
#39774=CARTESIAN_POINT('Ctrl Pts',(5.6213542648325,3.77136697151617,124.490780753786));
#39775=CARTESIAN_POINT('Ctrl Pts',(5.52209502989166,3.91525472009512,124.498989632757));
#39776=CARTESIAN_POINT('Ctrl Pts',(5.41750577645059,4.05498707299104,124.507198511727));
#39777=CARTESIAN_POINT('Ctrl Pts',(5.31286037707233,4.1947944374551,124.515411797415));
#39778=CARTESIAN_POINT('Ctrl Pts',(5.20287948081253,4.33044168089375,124.523625083102));
#39779=CARTESIAN_POINT('Ctrl Pts',(5.08794267584501,4.46151637084469,124.53183836879));
#39780=CARTESIAN_POINT('Ctrl Pts',(4.97283773249764,4.59278280691223,124.540063669502));
#39781=CARTESIAN_POINT('Ctrl Pts',(4.85276263875451,4.71946306149385,124.548288970214));
#39782=CARTESIAN_POINT('Ctrl Pts',(4.72813368781738,4.84118175966638,124.556514270926));
#39783=CARTESIAN_POINT('Ctrl Pts',(4.61542183541384,4.95126163950179,124.56395306322));
#39784=CARTESIAN_POINT('Ctrl Pts',(4.49898596854104,5.05728383354036,124.571391855514));
#39785=CARTESIAN_POINT('Ctrl Pts',(4.37915574804594,5.15900028439195,124.578830647808));
#39786=CARTESIAN_POINT('Ctrl Pts',(4.24781994086785,5.27048311502257,124.586983681211));
#39787=CARTESIAN_POINT('Ctrl Pts',(4.11201878678538,5.37712181140436,124.595136714613));
#39788=CARTESIAN_POINT('Ctrl Pts',(3.97214727178368,5.47853402392113,124.603289748016));
#39789=CARTESIAN_POINT('Ctrl Pts',(3.83246405080114,5.57980971605285,124.611431805864));
#39790=CARTESIAN_POINT('Ctrl Pts',(3.68872167560797,5.67587272549816,124.619573863713));
#39791=CARTESIAN_POINT('Ctrl Pts',(3.54135009387041,5.76637915096155,124.627715921561));
#39792=CARTESIAN_POINT('Ctrl Pts',(3.39728263191387,5.85485639232339,124.63567543177));
#39793=CARTESIAN_POINT('Ctrl Pts',(3.24974724590813,5.93802333903456,124.643634941979));
#39794=CARTESIAN_POINT('Ctrl Pts',(3.09917575053274,6.01559628526631,124.651594452187));
#39795=CARTESIAN_POINT('Origin',(0.,0.,-3.69717978381041));
#39796=CARTESIAN_POINT('',(3.09917575053273,6.01559628526631,127.045911902629));
#39797=CARTESIAN_POINT('',(3.09917575053261,6.01559628526638,126.651394038606));
#39798=CARTESIAN_POINT('',(3.09917575053259,6.01559628526639,-3.69717978381041));
#39799=CARTESIAN_POINT('',(-6.76699999483142,0.000264483490106234,125.697369247924));
#39800=CARTESIAN_POINT('Ctrl Pts',(-6.76699999483143,0.000264483490106234,
125.697369247924));
#39801=CARTESIAN_POINT('Ctrl Pts',(-6.76700666497119,-0.170395831555567,
125.705445979297));
#39802=CARTESIAN_POINT('Ctrl Pts',(-6.76055310740299,-0.341346504411689,
125.713522710671));
#39803=CARTESIAN_POINT('Ctrl Pts',(-6.74759927607116,-0.512047858665496,
125.721599442044));
#39804=CARTESIAN_POINT('Ctrl Pts',(-6.73466049174337,-0.682550928419518,
125.729666791591));
#39805=CARTESIAN_POINT('Ctrl Pts',(-6.71523648697607,-0.852804888403578,
125.737734141137));
#39806=CARTESIAN_POINT('Ctrl Pts',(-6.68933914014784,-1.02226751297604,
125.745801490683));
#39807=CARTESIAN_POINT('Ctrl Pts',(-6.6634662145074,-1.19157033436069,125.753861232721));
#39808=CARTESIAN_POINT('Ctrl Pts',(-6.63113215195376,-1.36008293983411,
125.76192097476));
#39809=CARTESIAN_POINT('Ctrl Pts',(-6.59240079476521,-1.52726577948277,
125.769980716799));
#39810=CARTESIAN_POINT('Ctrl Pts',(-6.55369750536983,-1.694327465273,125.778034618113));
#39811=CARTESIAN_POINT('Ctrl Pts',(-6.50860623349195,-1.86006094202274,
125.786088519428));
#39812=CARTESIAN_POINT('Ctrl Pts',(-6.45724228911631,-2.02393453936831,
125.794142420743));
#39813=CARTESIAN_POINT('Ctrl Pts',(-6.40370052093684,-2.19475635351177,
125.802537806307));
#39814=CARTESIAN_POINT('Ctrl Pts',(-6.34334257886107,-2.36355670945537,
125.810933191871));
#39815=CARTESIAN_POINT('Ctrl Pts',(-6.27635770124143,-2.52974761706922,
125.819328577435));
#39816=CARTESIAN_POINT('Ctrl Pts',(-6.21213961181366,-2.68907406426871,
125.827377194378));
#39817=CARTESIAN_POINT('Ctrl Pts',(-6.14183121813148,-2.84600193101904,
125.835425811321));
#39818=CARTESIAN_POINT('Ctrl Pts',(-6.06564932049882,-3.00003121995958,
125.843474428264));
#39819=CARTESIAN_POINT('Ctrl Pts',(-5.98946870220167,-3.15405792226021,
125.851522910045));
#39820=CARTESIAN_POINT('Ctrl Pts',(-5.90741494106427,-3.30518580913329,
125.859571391826));
#39821=CARTESIAN_POINT('Ctrl Pts',(-5.81975164502797,-3.45293784916472,
125.867619873607));
#39822=CARTESIAN_POINT('Ctrl Pts',(-5.73207250866444,-3.60071658726442,
125.87566980971));
#39823=CARTESIAN_POINT('Ctrl Pts',(-5.63878201021364,-3.74511794376387,
125.883719745812));
#39824=CARTESIAN_POINT('Ctrl Pts',(-5.54018800530699,-3.88569245641656,
125.891769681914));
#39825=CARTESIAN_POINT('Ctrl Pts',(-5.4415567090948,-4.02632013870272,125.899822662752));
#39826=CARTESIAN_POINT('Ctrl Pts',(-5.33761812784836,-4.1631177913874,125.907875643589));
#39827=CARTESIAN_POINT('Ctrl Pts',(-5.22872134141143,-4.29566783327909,
125.915928624427));
#39828=CARTESIAN_POINT('Ctrl Pts',(-5.11970598587234,-4.42836219843294,
125.923990373518));
#39829=CARTESIAN_POINT('Ctrl Pts',(-5.00572188434,-4.55679943201993,125.93205212261));
#39830=CARTESIAN_POINT('Ctrl Pts',(-4.88715649169459,-4.68059722959447,
125.940113871702));
#39831=CARTESIAN_POINT('Ctrl Pts',(-4.76851500700475,-4.80447447722863,
125.948180794605));
#39832=CARTESIAN_POINT('Ctrl Pts',(-4.64528664285792,-4.92370610134431,
125.956247717508));
#39833=CARTESIAN_POINT('Ctrl Pts',(-4.51789267863167,-5.03794945829812,
125.964314640411));
#39834=CARTESIAN_POINT('Ctrl Pts',(-4.39032760122543,-5.15234626478324,
125.972392398653));
#39835=CARTESIAN_POINT('Ctrl Pts',(-4.25858604145576,-5.26174119461539,
125.980470156895));
#39836=CARTESIAN_POINT('Ctrl Pts',(-4.12311955990129,-5.36583396078926,
125.988547915138));
#39837=CARTESIAN_POINT('Ctrl Pts',(-4.08352062257188,-5.3962618782849,125.990909168185));
#39838=CARTESIAN_POINT('Ctrl Pts',(-4.04360356575319,-5.4262370299317,125.993270421233));
#39839=CARTESIAN_POINT('Ctrl Pts',(-4.00338006729888,-5.45575265538624,
125.99563167428));
#39840=CARTESIAN_POINT('Ctrl Pts',(-3.86327100415885,-5.55856337025048,
126.003856541958));
#39841=CARTESIAN_POINT('Ctrl Pts',(-3.71900227672201,-5.65611774598859,
126.012081409635));
#39842=CARTESIAN_POINT('Ctrl Pts',(-3.57100494534304,-5.74806164548846,
126.020306277313));
#39843=CARTESIAN_POINT('Ctrl Pts',(-3.42317434952305,-5.83990195989437,
126.028521878756));
#39844=CARTESIAN_POINT('Ctrl Pts',(-3.27162381637479,-5.92614419684376,
126.0367374802));
#39845=CARTESIAN_POINT('Ctrl Pts',(-3.11681632686272,-6.00647525463995,
126.044953081644));
#39846=CARTESIAN_POINT('Ctrl Pts',(-2.9621521413842,-6.08673195062949,126.053161077972));
#39847=CARTESIAN_POINT('Ctrl Pts',(-2.80423732029464,-6.16108820072119,
126.0613690743));
#39848=CARTESIAN_POINT('Ctrl Pts',(-2.64356266883131,-6.22927487079849,
126.069577070628));
#39849=CARTESIAN_POINT('Ctrl Pts',(-2.48300448024666,-6.29741211667718,
126.077779117499));
#39850=CARTESIAN_POINT('Ctrl Pts',(-2.3196907746823,-6.35938855020906,126.085981164371));
#39851=CARTESIAN_POINT('Ctrl Pts',(-2.154135815517,-6.41498151893729,126.094183211242));
#39852=CARTESIAN_POINT('Ctrl Pts',(-1.98866761173854,-6.47054535540918,
126.102380960014));
#39853=CARTESIAN_POINT('Ctrl Pts',(-1.82096083341129,-6.51973227713905,
126.110578708785));
#39854=CARTESIAN_POINT('Ctrl Pts',(-1.65154860902888,-6.56236818473444,
126.118776457557));
#39855=CARTESIAN_POINT('Ctrl Pts',(-1.48216869662586,-6.60499596038674,
126.126972642773));
#39856=CARTESIAN_POINT('Ctrl Pts',(-1.31108433213543,-6.64107511719608,
126.135168827988));
#39857=CARTESIAN_POINT('Ctrl Pts',(-1.1388429527302,-6.67048167143999,126.143365013204));
#39858=CARTESIAN_POINT('Ctrl Pts',(-0.966614315353741,-6.69988605025333,
126.151560592084));
#39859=CARTESIAN_POINT('Ctrl Pts',(-0.793229187079543,-6.72261874829726,
126.159756170965));
#39860=CARTESIAN_POINT('Ctrl Pts',(-0.619244270849144,-6.73860709145596,
126.167951749845));
#39861=CARTESIAN_POINT('Ctrl Pts',(-0.445240571134841,-6.75459716072283,
126.176148213523));
#39862=CARTESIAN_POINT('Ctrl Pts',(-0.27063731185326,-6.76384139161749,
126.184344677202));
#39863=CARTESIAN_POINT('Ctrl Pts',(-0.0959954308768129,-6.76631907888261,
126.19254114088));
#39864=CARTESIAN_POINT('Ctrl Pts',(0.07869707866419,-6.76879748442761,126.200739980708));
#39865=CARTESIAN_POINT('Ctrl Pts',(0.25342787349751,-6.7645054339659,126.208938820536));
#39866=CARTESIAN_POINT('Ctrl Pts',(0.427636852273128,-6.75347434455614,
126.217137660364));
#39867=CARTESIAN_POINT('Ctrl Pts',(0.602027797283428,-6.74243173285965,
126.225345064113));
#39868=CARTESIAN_POINT('Ctrl Pts',(0.77589547870112,-6.72463604168225,126.233552467862));
#39869=CARTESIAN_POINT('Ctrl Pts',(0.948684742881594,-6.70017061414287,
126.241759871611));
#39870=CARTESIAN_POINT('Ctrl Pts',(1.1215665621358,-6.67569208162582,126.24997167168));
#39871=CARTESIAN_POINT('Ctrl Pts',(1.29336845984038,-6.64453675451651,126.258183471749));
#39872=CARTESIAN_POINT('Ctrl Pts',(1.46354639827537,-6.60683895218396,126.266395271818));
#39873=CARTESIAN_POINT('Ctrl Pts',(1.6339748624145,-6.5690856534189,126.274619160804));
#39874=CARTESIAN_POINT('Ctrl Pts',(1.8027742424728,-6.52477072238826,126.282843049791));
#39875=CARTESIAN_POINT('Ctrl Pts',(1.96941531432961,-6.47407849193104,126.291066938777));
#39876=CARTESIAN_POINT('Ctrl Pts',(2.12338878386462,-6.42723974734667,126.298665670027));
#39877=CARTESIAN_POINT('Ctrl Pts',(2.27551959781055,-6.37495704037652,126.306264401277));
#39878=CARTESIAN_POINT('Ctrl Pts',(2.42540700211847,-6.31741164355108,126.313863132527));
#39879=CARTESIAN_POINT('Ctrl Pts',(2.58764476592958,-6.25512464524265,126.322087980849));
#39880=CARTESIAN_POINT('Ctrl Pts',(2.74770929359056,-6.18649655697364,126.330312829171));
#39881=CARTESIAN_POINT('Ctrl Pts',(2.90506962383229,-6.11169857573874,126.338537677493));
#39882=CARTESIAN_POINT('Ctrl Pts',(3.0622527314522,-6.03698483361494,126.346753262812));
#39883=CARTESIAN_POINT('Ctrl Pts',(3.21673738499637,-5.9561151877116,126.354968848131));
#39884=CARTESIAN_POINT('Ctrl Pts',(3.36800988956307,-5.86930987287308,126.363184433451));
#39885=CARTESIAN_POINT('Ctrl Pts',(3.51914242140731,-5.78258487914959,126.371392416874));
#39886=CARTESIAN_POINT('Ctrl Pts',(3.66706841426848,-5.68993533192966,126.379600400297));
#39887=CARTESIAN_POINT('Ctrl Pts',(3.81129612084373,-5.59162864282326,126.38780838372));
#39888=CARTESIAN_POINT('Ctrl Pts',(3.9554193421296,-5.49339317167563,126.396010420897));
#39889=CARTESIAN_POINT('Ctrl Pts',(4.09584931835875,-5.3895089229256,126.404212458073));
#39890=CARTESIAN_POINT('Ctrl Pts',(4.23212072517856,-5.280288170878,126.41241449525));
#39891=CARTESIAN_POINT('Ctrl Pts',(4.36832077513082,-5.17112461095103,126.420612237529));
#39892=CARTESIAN_POINT('Ctrl Pts',(4.5003663144841,-5.05663033845595,126.428809979809));
#39893=CARTESIAN_POINT('Ctrl Pts',(4.62782266742955,-4.9371597461319,126.437007722088));
#39894=CARTESIAN_POINT('Ctrl Pts',(4.755254786659,-4.81771186916364,126.445203905702));
#39895=CARTESIAN_POINT('Ctrl Pts',(4.87809919175065,-4.69328979756881,126.453400089317));
#39896=CARTESIAN_POINT('Ctrl Pts',(4.99595563296128,-4.56428705423777,126.461596272931));
#39897=CARTESIAN_POINT('Ctrl Pts',(5.11380339829346,-4.43529380730853,126.469791853192));
#39898=CARTESIAN_POINT('Ctrl Pts',(5.22666368831546,-4.30172082449852,126.477987433453));
#39899=CARTESIAN_POINT('Ctrl Pts',(5.33417441025133,-4.16399716150478,126.486183013714));
#39900=CARTESIAN_POINT('Ctrl Pts',(5.4416967782023,-4.02625857970267,126.494379481754));
#39901=CARTESIAN_POINT('Ctrl Pts',(5.54386820270352,-3.88436870484852,126.502575949795));
#39902=CARTESIAN_POINT('Ctrl Pts',(5.64036802219003,-3.73878824945411,126.510772417836));
#39903=CARTESIAN_POINT('Ctrl Pts',(5.73689585201883,-3.59316553741706,126.518971265009));
#39904=CARTESIAN_POINT('Ctrl Pts',(5.82774859949183,-3.44385041008105,126.527170112183));
#39905=CARTESIAN_POINT('Ctrl Pts',(5.91264990493643,-3.2913310531843,126.535368959356));
#39906=CARTESIAN_POINT('Ctrl Pts',(5.99763994050094,-3.13865229872875,126.543576375122));
#39907=CARTESIAN_POINT('Ctrl Pts',(6.07666593285695,-2.98276293833167,126.551783790888));
#39908=CARTESIAN_POINT('Ctrl Pts',(6.14949788143819,-2.8241750664906,126.559991206654));
#39909=CARTESIAN_POINT('Ctrl Pts',(6.22236886538212,-2.66550219712831,126.568203021306));
#39910=CARTESIAN_POINT('Ctrl Pts',(6.28903905058444,-2.50412826439997,126.576414835958));
#39911=CARTESIAN_POINT('Ctrl Pts',(6.34932733121625,-2.34058356848678,126.58462665061));
#39912=CARTESIAN_POINT('Ctrl Pts',(6.40970439550668,-2.17679802814581,126.592850558408));
#39913=CARTESIAN_POINT('Ctrl Pts',(6.46368066195745,-2.01083567718833,126.601074466205));
#39914=CARTESIAN_POINT('Ctrl Pts',(6.51112510832687,-1.8432413905171,126.609298374003));
#39915=CARTESIAN_POINT('Ctrl Pts',(6.55496290055401,-1.68838736481421,126.616897112926));
#39916=CARTESIAN_POINT('Ctrl Pts',(6.5932247183944,-1.53214043268882,126.62449585185));
#39917=CARTESIAN_POINT('Ctrl Pts',(6.62584641610265,-1.37493573312345,126.632094590773));
#39918=CARTESIAN_POINT('Ctrl Pts',(6.66083891672611,-1.20630608065252,126.640245572948));
#39919=CARTESIAN_POINT('Ctrl Pts',(6.68944467460571,-1.03607480295576,126.648396555122));
#39920=CARTESIAN_POINT('Ctrl Pts',(6.71151692872969,-0.864771365954496,
126.656547537296));
#39921=CARTESIAN_POINT('Ctrl Pts',(6.73356354388478,-0.693666913772199,
126.664689051349));
#39922=CARTESIAN_POINT('Ctrl Pts',(6.74909171605032,-0.521493140358055,
126.672830565402));
#39923=CARTESIAN_POINT('Ctrl Pts',(6.75800510869489,-0.348792131295672,
126.680972079455));
#39924=CARTESIAN_POINT('Ctrl Pts',(6.76691002331251,-0.176255387835315,
126.689105849658));
#39925=CARTESIAN_POINT('Ctrl Pts',(6.76921266551185,-0.00319276980574204,
126.697239619861));
#39926=CARTESIAN_POINT('Ctrl Pts',(6.76486816740433,0.169846040988923,126.705373390065));
#39927=CARTESIAN_POINT('Ctrl Pts',(6.76052688785489,0.342756658503348,126.713501134483));
#39928=CARTESIAN_POINT('Ctrl Pts',(6.74954828245963,0.515643139853826,126.721628878901));
#39929=CARTESIAN_POINT('Ctrl Pts',(6.73193948586503,0.687953311389146,126.729756623319));
#39930=CARTESIAN_POINT('Ctrl Pts',(6.71434003237387,0.860172056361169,126.737880055213));
#39931=CARTESIAN_POINT('Ctrl Pts',(6.69011743081647,1.03181473749403,126.746003487107));
#39932=CARTESIAN_POINT('Ctrl Pts',(6.65933083642415,1.20233182235624,126.754126919001));
#39933=CARTESIAN_POINT('Ctrl Pts',(6.62834894398616,1.37393060053607,126.762301882752));
#39934=CARTESIAN_POINT('Ctrl Pts',(6.59071950768561,1.54438907747378,126.770476846502));
#39935=CARTESIAN_POINT('Ctrl Pts',(6.54655560714764,1.71315459971475,126.778651810253));
#39936=CARTESIAN_POINT('Ctrl Pts',(6.50268005401,1.88081824691726,126.786773399426));
#39937=CARTESIAN_POINT('Ctrl Pts',(6.45235522942674,2.04681062899697,126.794894988599));
#39938=CARTESIAN_POINT('Ctrl Pts',(6.39574276095292,2.21060252775536,126.803016577772));
#39939=CARTESIAN_POINT('Ctrl Pts',(6.33912281847213,2.37441605040376,126.811139239162));
#39940=CARTESIAN_POINT('Ctrl Pts',(6.27621369826234,2.53602816514689,126.819261900551));
#39941=CARTESIAN_POINT('Ctrl Pts',(6.20722607997339,2.6949273444934,126.82738456194));
#39942=CARTESIAN_POINT('Ctrl Pts',(6.1382162166206,2.85387776089482,126.835509842483));
#39943=CARTESIAN_POINT('Ctrl Pts',(6.06312409787922,3.01011316439387,126.843635123025));
#39944=CARTESIAN_POINT('Ctrl Pts',(5.98220744982599,3.16314448409276,126.851760403567));
#39945=CARTESIAN_POINT('Ctrl Pts',(5.90040923168254,3.31784304826555,126.859974207355));
#39946=CARTESIAN_POINT('Ctrl Pts',(5.81265900614377,3.46926696439047,126.868188011143));
#39947=CARTESIAN_POINT('Ctrl Pts',(5.71926880003638,3.61693978287314,126.876401814931));
#39948=CARTESIAN_POINT('Ctrl Pts',(5.62672523073721,3.76327386093632,126.884541155786));
#39949=CARTESIAN_POINT('Ctrl Pts',(5.52864377957336,3.90592430928612,126.892680496641));
#39950=CARTESIAN_POINT('Ctrl Pts',(5.42536932350576,4.0444600014789,126.900819837496));
#39951=CARTESIAN_POINT('Ctrl Pts',(5.32067765460782,4.18489678875281,126.90907087275));
#39952=CARTESIAN_POINT('Ctrl Pts',(5.21064966899737,4.32110476377659,126.917321908004));
#39953=CARTESIAN_POINT('Ctrl Pts',(5.09568372992345,4.45267294157042,126.925572943258));
#39954=CARTESIAN_POINT('Ctrl Pts',(4.98071779084954,4.58424111936425,126.933823978513));
#39955=CARTESIAN_POINT('Ctrl Pts',(4.86081421067522,4.71116926692677,126.942075013767));
#39956=CARTESIAN_POINT('Ctrl Pts',(4.73640624482451,4.83308854501833,126.950326049021));
#39957=CARTESIAN_POINT('Ctrl Pts',(4.612305237309,4.95470700524524,126.95855672606));
#39958=CARTESIAN_POINT('Ctrl Pts',(4.48333480053266,5.07172103184382,126.9667874031));
#39959=CARTESIAN_POINT('Ctrl Pts',(4.34986944856124,5.18371727435762,126.97501808014));
#39960=CARTESIAN_POINT('Ctrl Pts',(4.21654329177819,5.29559671248853,126.983240173149));
#39961=CARTESIAN_POINT('Ctrl Pts',(4.07873182077674,5.40246855319842,126.991462266158));
#39962=CARTESIAN_POINT('Ctrl Pts',(3.93684733088864,5.50395513183701,126.999684359167));
#39963=CARTESIAN_POINT('Ctrl Pts',(3.79512205608919,5.6053278277346,127.007897225789));
#39964=CARTESIAN_POINT('Ctrl Pts',(3.6493331580027,5.70132709457614,127.016110092411));
#39965=CARTESIAN_POINT('Ctrl Pts',(3.49992675786233,5.79161477392957,127.024322959033));
#39966=CARTESIAN_POINT('Ctrl Pts',(3.3690132171906,5.87072704604166,127.031519273565));
#39967=CARTESIAN_POINT('Ctrl Pts',(3.23532291245085,5.94545461306768,127.038715588097));
#39968=CARTESIAN_POINT('Ctrl Pts',(3.09917575053273,6.01559628526631,127.045911902629));
#39969=CARTESIAN_POINT('Ctrl Pts',(3.09917575053273,6.01559628526632,125.045751582742));
#39970=CARTESIAN_POINT('Ctrl Pts',(2.93382384521587,6.10078395261652,125.054501030622));
#39971=CARTESIAN_POINT('Ctrl Pts',(2.76495772250264,6.17915010207986,125.063250478501));
#39972=CARTESIAN_POINT('Ctrl Pts',(2.59315093510946,6.25042856352594,125.071999926381));
#39973=CARTESIAN_POINT('Ctrl Pts',(2.42134553504201,6.32170644940429,125.080749303609));
#39974=CARTESIAN_POINT('Ctrl Pts',(2.24659978252431,6.38589665197217,125.089498680837));
#39975=CARTESIAN_POINT('Ctrl Pts',(2.06950719082269,6.44278115313047,125.098248058066));
#39976=CARTESIAN_POINT('Ctrl Pts',(1.89241597030047,6.49966521384767,125.10699736755));
#39977=CARTESIAN_POINT('Ctrl Pts',(1.71297821980402,6.54924359870869,125.115746677035));
#39978=CARTESIAN_POINT('Ctrl Pts',(1.53180337925603,6.59134792036498,125.124495986519));
#39979=CARTESIAN_POINT('Ctrl Pts',(1.3506298813133,6.63345193000509,125.133245231166));
#39980=CARTESIAN_POINT('Ctrl Pts',(1.16771959820771,6.66808192240814,125.141994475813));
#39981=CARTESIAN_POINT('Ctrl Pts',(0.983693754726281,6.6951202824828,125.15074372046));
#39982=CARTESIAN_POINT('Ctrl Pts',(0.799669213852509,6.72215845116926,125.159492903177));
#39983=CARTESIAN_POINT('Ctrl Pts',(0.614529411917502,6.74160505340517,125.168242085893));
#39984=CARTESIAN_POINT('Ctrl Pts',(0.428903137010801,6.75339404292851,125.17699126861));
#39985=CARTESIAN_POINT('Ctrl Pts',(0.24327811438683,6.76518295292029,125.185740392302));
#39986=CARTESIAN_POINT('Ctrl Pts',(0.0571669113294544,6.76931433541626,
125.194489515994));
#39987=CARTESIAN_POINT('Ctrl Pts',(-0.128798393433531,6.76577415924068,
125.203238639687));
#39988=CARTESIAN_POINT('Ctrl Pts',(-0.314762505389531,6.76223400577229,
125.211987707261));
#39989=CARTESIAN_POINT('Ctrl Pts',(-0.500580434438059,6.75102239755431,
125.220736774835));
#39990=CARTESIAN_POINT('Ctrl Pts',(-0.685621105968318,6.73217741143612,
125.229485842409));
#39991=CARTESIAN_POINT('Ctrl Pts',(-0.870660652075532,6.71333253993372,
125.238234856771));
#39992=CARTESIAN_POINT('Ctrl Pts',(-1.05492266507006,6.68685441246682,125.246983871133));
#39993=CARTESIAN_POINT('Ctrl Pts',(-1.23778136214556,6.65283295292502,125.255732885496));
#39994=CARTESIAN_POINT('Ctrl Pts',(-1.42999398956116,6.61707116400479,125.264929445816));
#39995=CARTESIAN_POINT('Ctrl Pts',(-1.62065563051565,6.57297413101274,125.274126006137));
#39996=CARTESIAN_POINT('Ctrl Pts',(-1.80905090416564,6.52070731026455,125.283322566458));
#39997=CARTESIAN_POINT('Ctrl Pts',(-1.98829816030723,6.47097843955113,125.292072564117));
#39998=CARTESIAN_POINT('Ctrl Pts',(-2.16549362698938,6.41385444883848,125.300822561776));
#39999=CARTESIAN_POINT('Ctrl Pts',(-2.34003538537155,6.34952938375822,125.309572559436));
#40000=CARTESIAN_POINT('Ctrl Pts',(-2.51457360400769,6.28520562320472,125.318322379643));
#40001=CARTESIAN_POINT('Ctrl Pts',(-2.68645795305744,6.21368117965436,125.32707219985));
#40002=CARTESIAN_POINT('Ctrl Pts',(-2.85510457878042,6.1351990060818,125.335822020057));
#40003=CARTESIAN_POINT('Ctrl Pts',(-3.02374800849086,6.05671831982041,125.344571674447));
#40004=CARTESIAN_POINT('Ctrl Pts',(-3.1891535777815,5.97128028833215,125.353321328837));
#40005=CARTESIAN_POINT('Ctrl Pts',(-3.35075946119047,5.87917511503464,125.362070983227));
#40006=CARTESIAN_POINT('Ctrl Pts',(-3.51236249680474,5.78707156480072,125.370820483432));
#40007=CARTESIAN_POINT('Ctrl Pts',(-3.67016573151701,5.68830124978307,125.379569983637));
#40008=CARTESIAN_POINT('Ctrl Pts',(-3.82363318123566,5.58319964673965,125.388319483842));
#40009=CARTESIAN_POINT('Ctrl Pts',(-3.97709813051924,5.47809975610972,125.397068841492));
#40010=CARTESIAN_POINT('Ctrl Pts',(-4.12622719971903,5.36666894581433,125.405818199142));
#40011=CARTESIAN_POINT('Ctrl Pts',(-4.27051388333216,5.24928568209688,125.414567556791));
#40012=CARTESIAN_POINT('Ctrl Pts',(-4.41479840781406,5.13190417492316,125.423316783514));
#40013=CARTESIAN_POINT('Ctrl Pts',(-4.55424046941923,5.00857057342068,125.432066010237));
#40014=CARTESIAN_POINT('Ctrl Pts',(-4.68836647798648,4.87970375823089,125.44081523696));
#40015=CARTESIAN_POINT('Ctrl Pts',(-4.82249065766897,4.75083870021376,125.449564344382));
#40016=CARTESIAN_POINT('Ctrl Pts',(-4.95129872273929,4.61644077801867,125.458313451804));
#40017=CARTESIAN_POINT('Ctrl Pts',(-5.07435321143231,4.47696643784903,125.467062559227));
#40018=CARTESIAN_POINT('Ctrl Pts',(-5.19740618568199,4.33749381420342,125.475811558973));
#40019=CARTESIAN_POINT('Ctrl Pts',(-5.31470553568899,4.19294511246392,125.484560558719));
#40020=CARTESIAN_POINT('Ctrl Pts',(-5.42585289572275,4.04381124114084,125.493309558465));
#40021=CARTESIAN_POINT('Ctrl Pts',(-5.53701239368999,3.89466108353792,125.502059513652));
#40022=CARTESIAN_POINT('Ctrl Pts',(-5.64201838589909,3.74092498410192,125.51080946884));
#40023=CARTESIAN_POINT('Ctrl Pts',(-5.7405141788448,3.58312516701298,125.519559424027));
#40024=CARTESIAN_POINT('Ctrl Pts',(-5.83900616882317,3.42533144264672,125.528309041375));
#40025=CARTESIAN_POINT('Ctrl Pts',(-5.93098831075965,3.2634745577638,125.537058658722));
#40026=CARTESIAN_POINT('Ctrl Pts',(-6.01614817580147,3.09810427952332,125.54580827607));
#40027=CARTESIAN_POINT('Ctrl Pts',(-6.10130520551454,2.93273950715233,125.554557602106));
#40028=CARTESIAN_POINT('Ctrl Pts',(-6.17964028165778,2.76386183029532,125.563306928142));
#40029=CARTESIAN_POINT('Ctrl Pts',(-6.25088734704388,2.59204482495321,125.572056254179));
#40030=CARTESIAN_POINT('Ctrl Pts',(-6.32213241899031,2.42023262692257,125.580805335415));
#40031=CARTESIAN_POINT('Ctrl Pts',(-6.38628976727249,2.24548152967231,125.589554416652));
#40032=CARTESIAN_POINT('Ctrl Pts',(-6.44314150010717,2.06838502450504,125.598303497888));
#40033=CARTESIAN_POINT('Ctrl Pts',(-6.49999837221279,1.89127251020532,125.607053370022));
#40034=CARTESIAN_POINT('Ctrl Pts',(-6.54954821963115,1.71181443660043,125.615803242157));
#40035=CARTESIAN_POINT('Ctrl Pts',(-6.59162273031443,1.53062039095333,125.624553114291));
#40036=CARTESIAN_POINT('Ctrl Pts',(-6.63369432010818,1.34943892412851,125.633302378993));
#40037=CARTESIAN_POINT('Ctrl Pts',(-6.66829154679582,1.16652200558753,125.642051643695));
#40038=CARTESIAN_POINT('Ctrl Pts',(-6.69529690603127,0.982490885498748,
125.650800908397));
#40039=CARTESIAN_POINT('Ctrl Pts',(-6.72230365088011,0.798450322988453,
125.659550622014));
#40040=CARTESIAN_POINT('Ctrl Pts',(-6.7417177071427,0.61329572810763,125.66830033563));
#40041=CARTESIAN_POINT('Ctrl Pts',(-6.75347313109847,0.427656015427243,
125.677050049247));
#40042=CARTESIAN_POINT('Ctrl Pts',(-6.76248266272047,0.285378980759063,
125.683755959796));
#40043=CARTESIAN_POINT('Ctrl Pts',(-6.76699461942155,0.142817180247322,
125.690461870345));
#40044=CARTESIAN_POINT('Ctrl Pts',(-6.76699999518896,0.00025517189615077,
125.697167780894));
#40045=CARTESIAN_POINT('',(-6.76699862817337,0.00430886293122851,125.302820216149));
#40046=CARTESIAN_POINT('Ctrl Pts',(3.09917575053274,6.01559628526631,124.651594452187));
#40047=CARTESIAN_POINT('Ctrl Pts',(2.94538860019882,6.0948259051505,124.659723948344));
#40048=CARTESIAN_POINT('Ctrl Pts',(2.78843446991074,6.16821968728965,124.667853444502));
#40049=CARTESIAN_POINT('Ctrl Pts',(2.62880128532791,6.23551864741485,124.675982940659));
#40050=CARTESIAN_POINT('Ctrl Pts',(2.469253132826,6.30278175928809,124.684108106464));
#40051=CARTESIAN_POINT('Ctrl Pts',(2.30702910414561,6.36395637304771,124.692233272268));
#40052=CARTESIAN_POINT('Ctrl Pts',(2.14263979064315,6.41883040183745,124.700358438073));
#40053=CARTESIAN_POINT('Ctrl Pts',(1.97717870612209,6.47406219350409,124.708536577621));
#40054=CARTESIAN_POINT('Ctrl Pts',(1.80952433868321,6.52291078568762,124.716714717168));
#40055=CARTESIAN_POINT('Ctrl Pts',(1.64021620764073,6.56520980564922,124.724892856716));
#40056=CARTESIAN_POINT('Ctrl Pts',(1.47204394050188,6.60722504756875,124.733016130301));
#40057=CARTESIAN_POINT('Ctrl Pts',(1.30224039707465,6.64277826479993,124.741139403887));
#40058=CARTESIAN_POINT('Ctrl Pts',(1.13134756793747,6.67175701599826,124.749262677472));
#40059=CARTESIAN_POINT('Ctrl Pts',(0.960432600274631,6.70073952128522,124.757387003397));
#40060=CARTESIAN_POINT('Ctrl Pts',(0.788428426541787,6.72314580292431,124.765511329322));
#40061=CARTESIAN_POINT('Ctrl Pts',(0.61588508276254,6.73891493972365,124.773635655247));
#40062=CARTESIAN_POINT('Ctrl Pts',(0.443286559430474,6.75468911951044,124.781762579341));
#40063=CARTESIAN_POINT('Ctrl Pts',(0.27014888681954,6.76382189447387,124.789889503434));
#40064=CARTESIAN_POINT('Ctrl Pts',(0.0970250051294995,6.76630439371298,
124.798016427528));
#40065=CARTESIAN_POINT('Ctrl Pts',(-0.0780414356972559,6.7688147481592,
124.806234540835));
#40066=CARTESIAN_POINT('Ctrl Pts',(-0.25309338976398,6.7645246807498,124.814452654142));
#40067=CARTESIAN_POINT('Ctrl Pts',(-0.427562340379117,6.75347906231222,
124.82267076745));
#40068=CARTESIAN_POINT('Ctrl Pts',(-0.600392740664454,6.74253718039435,
124.83081169916));
#40069=CARTESIAN_POINT('Ctrl Pts',(-0.772650685166828,6.72496619823817,
124.83895263087));
#40070=CARTESIAN_POINT('Ctrl Pts',(-0.943792187809526,6.70086153462596,
124.84709356258));
#40071=CARTESIAN_POINT('Ctrl Pts',(-1.11736749809088,6.67641407798271,124.855350266686));
#40072=CARTESIAN_POINT('Ctrl Pts',(-1.28979398685506,6.64524578252713,124.863606970792));
#40073=CARTESIAN_POINT('Ctrl Pts',(-1.4605188123745,6.60750889509051,124.871863674898));
#40074=CARTESIAN_POINT('Ctrl Pts',(-1.63124363789394,6.56977200765389,124.880120379004));
#40075=CARTESIAN_POINT('Ctrl Pts',(-1.8002664449856,6.52546669049656,124.888377083109));
#40076=CARTESIAN_POINT('Ctrl Pts',(-1.96705462613735,6.47479614333854,124.896633787215));
#40077=CARTESIAN_POINT('Ctrl Pts',(-2.13336498911482,6.4242707581948,124.904866837347));
#40078=CARTESIAN_POINT('Ctrl Pts',(-2.2979705540881,6.36725967384907,124.913099887479));
#40079=CARTESIAN_POINT('Ctrl Pts',(-2.46032861007741,6.30389341045949,124.921332937611));
#40080=CARTESIAN_POINT('Ctrl Pts',(-2.62249332257937,6.24060260654907,124.929556183446));
#40081=CARTESIAN_POINT('Ctrl Pts',(-2.78241552515022,6.17097182238606,124.937779429281));
#40082=CARTESIAN_POINT('Ctrl Pts',(-2.93956595489824,6.09518178537796,124.946002675116));
#40083=CARTESIAN_POINT('Ctrl Pts',(-3.09656069663765,6.01946683311479,124.954217774229));
#40084=CARTESIAN_POINT('Ctrl Pts',(-3.25078881380083,5.93760493461024,124.962432873343));
#40085=CARTESIAN_POINT('Ctrl Pts',(-3.40173929587612,5.84982553268832,124.970647972456));
#40086=CARTESIAN_POINT('Ctrl Pts',(-3.55257043434711,5.76211553041366,124.978856576595));
#40087=CARTESIAN_POINT('Ctrl Pts',(-3.70012879092889,5.66849752252889,124.987065180734));
#40088=CARTESIAN_POINT('Ctrl Pts',(-3.84392624197688,5.56924770918313,124.995273784873));
#40089=CARTESIAN_POINT('Ctrl Pts',(-3.9876387682076,5.47005651142618,125.003477541122));
#40090=CARTESIAN_POINT('Ctrl Pts',(-4.12759451972279,5.36524033710329,125.011681297371));
#40091=CARTESIAN_POINT('Ctrl Pts',(-4.26333267911365,5.25511973861696,125.01988505362));
#40092=CARTESIAN_POINT('Ctrl Pts',(-4.39903067700317,5.14503172204116,125.028086382585));
#40093=CARTESIAN_POINT('Ctrl Pts',(-4.53051328826264,5.02964262995709,125.036287711549));
#40094=CARTESIAN_POINT('Ctrl Pts',(-4.65735104236138,4.90931464343195,125.044489040513));
#40095=CARTESIAN_POINT('Ctrl Pts',(-4.784171304323,4.78900325128484,125.052689238436));
#40096=CARTESIAN_POINT('Ctrl Pts',(-4.90634772452803,4.66375456717125,125.060889436359));
#40097=CARTESIAN_POINT('Ctrl Pts',(-5.0234861144979,4.53396915047366,125.069089634281));
#40098=CARTESIAN_POINT('Ctrl Pts',(-5.14062957782509,4.4041781126659,125.077290187361));
#40099=CARTESIAN_POINT('Ctrl Pts',(-5.25273433609446,4.26985021676648,125.085490740441));
#40100=CARTESIAN_POINT('Ctrl Pts',(-5.35944504467483,4.13142079835865,125.093691293521));
#40101=CARTESIAN_POINT('Ctrl Pts',(-5.4661797130524,3.99296029833928,125.101893687874));
#40102=CARTESIAN_POINT('Ctrl Pts',(-5.56751770081911,3.85039672530774,125.110096082227));
#40103=CARTESIAN_POINT('Ctrl Pts',(-5.66314569202678,3.70419625166898,125.118298476581));
#40104=CARTESIAN_POINT('Ctrl Pts',(-5.75886311221631,3.55785905488736,125.126508541614));
#40105=CARTESIAN_POINT('Ctrl Pts',(-5.84885967089522,3.40787846252971,125.134718606648));
#40106=CARTESIAN_POINT('Ctrl Pts',(-5.93286644233673,3.25474803593069,125.142928671682));
#40107=CARTESIAN_POINT('Ctrl Pts',(-6.01691341792889,3.10154432382583,125.151142665907));
#40108=CARTESIAN_POINT('Ctrl Pts',(-6.094964730807,2.94518809224704,125.159356660133));
#40109=CARTESIAN_POINT('Ctrl Pts',(-6.16679876877899,2.78619488646899,125.167570654358));
#40110=CARTESIAN_POINT('Ctrl Pts',(-6.23873074046976,2.62698491999723,125.175795846993));
#40111=CARTESIAN_POINT('Ctrl Pts',(-6.30442836263358,2.46513112659334,125.184021039628));
#40112=CARTESIAN_POINT('Ctrl Pts',(-6.36371883538669,2.30116743939781,125.192246232263));
#40113=CARTESIAN_POINT('Ctrl Pts',(-6.41703863054339,2.1537152466854,125.199643130383));
#40114=CARTESIAN_POINT('Ctrl Pts',(-6.4651773432269,2.00455709494514,125.207040028503));
#40115=CARTESIAN_POINT('Ctrl Pts',(-6.5080444707201,1.85408903969836,125.214436926623));
#40116=CARTESIAN_POINT('Ctrl Pts',(-6.56532637959985,1.65302360951934,125.224321154209));
#40117=CARTESIAN_POINT('Ctrl Pts',(-6.61330786675181,1.44922672452033,125.234205381795));
#40118=CARTESIAN_POINT('Ctrl Pts',(-6.6517697274498,1.24348240557814,125.24408960938));
#40119=CARTESIAN_POINT('Ctrl Pts',(-6.68992873370557,1.03935814816764,125.25389600708));
#40120=CARTESIAN_POINT('Ctrl Pts',(-6.71871742499295,0.833317035117996,
125.26370240478));
#40121=CARTESIAN_POINT('Ctrl Pts',(-6.73796965843727,0.626142062138283,
125.27350880248));
#40122=CARTESIAN_POINT('Ctrl Pts',(-6.75715135987306,0.419726090289727,
125.283279273703));
#40123=CARTESIAN_POINT('Ctrl Pts',(-6.76686626403555,0.212184572460418,
125.293049744926));
#40124=CARTESIAN_POINT('Ctrl Pts',(-6.76699862817337,0.00430886293105204,
125.302820216149));
#40125=CARTESIAN_POINT('Ctrl Pts',(-6.76699862817393,0.0043088620540932,
125.30282021619));
#40126=CARTESIAN_POINT('Ctrl Pts',(-6.76710572847117,-0.163890434048294,
125.310725836264));
#40127=CARTESIAN_POINT('Ctrl Pts',(-6.76093751050823,-0.332268221061752,
125.318631456339));
#40128=CARTESIAN_POINT('Ctrl Pts',(-6.74848063473331,-0.5002980338053,125.326537076413));
#40129=CARTESIAN_POINT('Ctrl Pts',(-6.73602882106901,-0.668259564138937,
125.334439483874));
#40130=CARTESIAN_POINT('Ctrl Pts',(-6.71729345518341,-0.835873016889208,
125.342341891336));
#40131=CARTESIAN_POINT('Ctrl Pts',(-6.69231329044887,-1.00261249866605,
125.350244298797));
#40132=CARTESIAN_POINT('Ctrl Pts',(-6.66797906649877,-1.165040406328,125.35794236464));
#40133=CARTESIAN_POINT('Ctrl Pts',(-6.63771907011902,-1.32663862890468,
125.365640430484));
#40134=CARTESIAN_POINT('Ctrl Pts',(-6.60161642942235,-1.48692619816216,
125.373338496327));
#40135=CARTESIAN_POINT('Ctrl Pts',(-6.56130376484322,-1.66590532243092,
125.381934253874));
#40136=CARTESIAN_POINT('Ctrl Pts',(-6.51373197784661,-1.8431390565141,125.390530011422));
#40137=CARTESIAN_POINT('Ctrl Pts',(-6.45908654331555,-2.01804113584437,
125.39912576897));
#40138=CARTESIAN_POINT('Ctrl Pts',(-6.40439012273616,-2.19310640476121,
125.407729546651));
#40139=CARTESIAN_POINT('Ctrl Pts',(-6.34260697192179,-2.36583538510928,
125.416333324333));
#40140=CARTESIAN_POINT('Ctrl Pts',(-6.27397138739989,-2.53566007778794,
125.424937102014));
#40141=CARTESIAN_POINT('Ctrl Pts',(-6.20263836438787,-2.71215902939211,
125.433879015682));
#40142=CARTESIAN_POINT('Ctrl Pts',(-6.12390355555075,-2.88552045053691,
125.44282092935));
#40143=CARTESIAN_POINT('Ctrl Pts',(-6.03808280548288,-3.05513420885761,
125.451762843018));
#40144=CARTESIAN_POINT('Ctrl Pts',(-5.95528252329576,-3.2187783979455,125.460390045349));
#40145=CARTESIAN_POINT('Ctrl Pts',(-5.86588676675858,-3.37893399160023,
125.46901724768));
#40146=CARTESIAN_POINT('Ctrl Pts',(-5.77022407419043,-3.53508177184535,
125.47764445001));
#40147=CARTESIAN_POINT('Ctrl Pts',(-5.67447027755016,-3.69137825895048,
125.486279868431));
#40148=CARTESIAN_POINT('Ctrl Pts',(-5.57243779871761,-3.84365905901317,
125.494915286851));
#40149=CARTESIAN_POINT('Ctrl Pts',(-5.46449742710046,-3.99143543968989,
125.503550705272));
#40150=CARTESIAN_POINT('Ctrl Pts',(-5.35639758895895,-4.13943013892024,
125.512198881293));
#40151=CARTESIAN_POINT('Ctrl Pts',(-5.2423726027151,-4.28290687917374,125.520847057314));
#40152=CARTESIAN_POINT('Ctrl Pts',(-5.12283324264721,-4.42141024651962,
125.529495233335));
#40153=CARTESIAN_POINT('Ctrl Pts',(-5.11018643160661,-4.43606337762485,
125.530410177567));
#40154=CARTESIAN_POINT('Ctrl Pts',(-5.09747793258958,-4.45066087703468,
125.531325121799));
#40155=CARTESIAN_POINT('Ctrl Pts',(-5.08470825549322,-4.46520223019283,
125.532240066031));
#40156=CARTESIAN_POINT('Ctrl Pts',(-4.96989987167918,-4.59593922862748,
125.540466058572));
#40157=CARTESIAN_POINT('Ctrl Pts',(-4.84989533998742,-4.72241708047132,
125.548692051113));
#40158=CARTESIAN_POINT('Ctrl Pts',(-4.72504278143572,-4.84419856256968,
125.556918043655));
#40159=CARTESIAN_POINT('Ctrl Pts',(-4.60032111465371,-4.96585237252506,
125.565135412306));
#40160=CARTESIAN_POINT('Ctrl Pts',(-4.47076179658654,-5.0828193691989,125.573352780958));
#40161=CARTESIAN_POINT('Ctrl Pts',(-4.3367527091754,-5.19469584667474,125.581570149609));
#40162=CARTESIAN_POINT('Ctrl Pts',(-4.20285729833344,-5.30647742212285,
125.589780547671));
#40163=CARTESIAN_POINT('Ctrl Pts',(-4.06451990932337,-5.41317685024397,
125.597990945734));
#40164=CARTESIAN_POINT('Ctrl Pts',(-3.92216479027695,-5.51442765460857,
125.606201343796));
#40165=CARTESIAN_POINT('Ctrl Pts',(-3.77990195090861,-5.61561282458156,
125.614406419585));
#40166=CARTESIAN_POINT('Ctrl Pts',(-3.63362686027734,-5.71135619935031,
125.622611495374));
#40167=CARTESIAN_POINT('Ctrl Pts',(-3.48379638847768,-5.80133189221492,
125.630816571162));
#40168=CARTESIAN_POINT('Ctrl Pts',(-3.33403307625314,-5.89126725463651,
125.639017969132));
#40169=CARTESIAN_POINT('Ctrl Pts',(-3.18071786440322,-5.97543990173833,
125.647219367101));
#40170=CARTESIAN_POINT('Ctrl Pts',(-3.02433618793491,-6.05356751200045,
125.655420765071));
#40171=CARTESIAN_POINT('Ctrl Pts',(-2.86796676058128,-6.13168900265778,
125.663621520639));
#40172=CARTESIAN_POINT('Ctrl Pts',(-2.70853166340291,-6.20376623182548,
125.671822276206));
#40173=CARTESIAN_POINT('Ctrl Pts',(-2.54654082793056,-6.2695628884064,125.680023031774));
#40174=CARTESIAN_POINT('Ctrl Pts',(-2.38455081529468,-6.33535921077156,
125.688223745686));
#40175=CARTESIAN_POINT('Ctrl Pts',(-2.22000542185178,-6.39487488824521,
125.696424459597));
#40176=CARTESIAN_POINT('Ctrl Pts',(-2.0534343344751,-6.44792186940869,125.704625173509));
#40177=CARTESIAN_POINT('Ctrl Pts',(-1.8868339063714,-6.50097819455268,125.712827331939));
#40178=CARTESIAN_POINT('Ctrl Pts',(-1.71820741491762,-6.5475634445163,125.721029490369));
#40179=CARTESIAN_POINT('Ctrl Pts',(-1.5480995243689,-6.58753951507304,125.729231648798));
#40180=CARTESIAN_POINT('Ctrl Pts',(-1.37793084199032,-6.62752987196578,
125.737436738451));
#40181=CARTESIAN_POINT('Ctrl Pts',(-1.20628005454706,-6.66090626240241,
125.745641828104));
#40182=CARTESIAN_POINT('Ctrl Pts',(-1.03370188142339,-6.68758173186256,
125.753846917757));
#40183=CARTESIAN_POINT('Ctrl Pts',(-0.860926558141236,-6.71428767489266,
125.762061380755));
#40184=CARTESIAN_POINT('Ctrl Pts',(-0.687222087152422,-6.73427734878347,
125.770275843753));
#40185=CARTESIAN_POINT('Ctrl Pts',(-0.513149240485588,-6.74751560627977,
125.77849030675));
#40186=CARTESIAN_POINT('Ctrl Pts',(-0.338973261159087,-6.76076170702521,
125.786709636558));
#40187=CARTESIAN_POINT('Ctrl Pts',(-0.164428828620265,-6.76724840455046,
125.794928966365));
#40188=CARTESIAN_POINT('Ctrl Pts',(0.00992352496164936,-6.76699272377711,
125.803148296173));
#40189=CARTESIAN_POINT('Ctrl Pts',(0.184546026944872,-6.7667366468419,125.811380361333));
#40190=CARTESIAN_POINT('Ctrl Pts',(0.35897549738885,-6.75971732901395,125.819612426494));
#40191=CARTESIAN_POINT('Ctrl Pts',(0.532655418187711,-6.74600379524614,
125.827844491655));
#40192=CARTESIAN_POINT('Ctrl Pts',(0.688771401904405,-6.73367708640986,
125.835244062916));
#40193=CARTESIAN_POINT('Ctrl Pts',(0.844281684288117,-6.71594237343187,
125.842643634177));
#40194=CARTESIAN_POINT('Ctrl Pts',(0.998790178529936,-6.69288481742157,
125.850043205438));
#40195=CARTESIAN_POINT('Ctrl Pts',(1.1690821527284,-6.66747186681032,125.858198663845));
#40196=CARTESIAN_POINT('Ctrl Pts',(1.33868135385016,-6.63551392819872,125.866354122252));
#40197=CARTESIAN_POINT('Ctrl Pts',(1.50704013197942,-6.59705381519686,125.874509580658));
#40198=CARTESIAN_POINT('Ctrl Pts',(1.67519399534527,-6.55864051320803,125.8826551128));
#40199=CARTESIAN_POINT('Ctrl Pts',(1.8421100885522,-6.51374087051423,125.890800644942));
#40200=CARTESIAN_POINT('Ctrl Pts',(2.00724606716769,-6.46244939831949,125.898946177084));
#40201=CARTESIAN_POINT('Ctrl Pts',(2.17221577837386,-6.41120956902094,125.907083507885));
#40202=CARTESIAN_POINT('Ctrl Pts',(2.33540859671976,-6.35359083001216,125.915220838685));
#40203=CARTESIAN_POINT('Ctrl Pts',(2.49629256009574,-6.28973866344307,125.923358169486));
#40204=CARTESIAN_POINT('Ctrl Pts',(2.65704834747318,-6.22593736779386,125.931489017288));
#40205=CARTESIAN_POINT('Ctrl Pts',(2.81549860433318,-6.15591266703359,125.93961986509));
#40206=CARTESIAN_POINT('Ctrl Pts',(2.9711267303755,-6.07985978062391,125.947750712892));
#40207=CARTESIAN_POINT('Ctrl Pts',(3.12666356011906,-6.00385150920263,125.955876790886));
#40208=CARTESIAN_POINT('Ctrl Pts',(3.27938122847468,-5.92182225472123,125.964002868879));
#40209=CARTESIAN_POINT('Ctrl Pts',(3.42878332811567,-5.83401524585221,125.972128946873));
#40210=CARTESIAN_POINT('Ctrl Pts',(3.57871518031466,-5.74589688936713,125.980283838455));
#40211=CARTESIAN_POINT('Ctrl Pts',(3.72530756450427,-5.65195987244917,125.988438730038));
#40212=CARTESIAN_POINT('Ctrl Pts',(3.86808338058065,-5.55249673218056,125.99659362162));
#40213=CARTESIAN_POINT('Ctrl Pts',(4.01030242089413,-5.45342146338294,126.004716711976));
#40214=CARTESIAN_POINT('Ctrl Pts',(4.14873431378981,-5.34886331835999,126.012839802332));
#40215=CARTESIAN_POINT('Ctrl Pts',(4.28293658568011,-5.23915481762496,126.020962892689));
#40216=CARTESIAN_POINT('Ctrl Pts',(4.4171493957457,-5.12943770207741,126.029086620907));
#40217=CARTESIAN_POINT('Ctrl Pts',(4.54713163998007,-5.01456965674763,126.037210349126));
#40218=CARTESIAN_POINT('Ctrl Pts',(4.67247415664623,-4.89492331456511,126.045334077344));
#40219=CARTESIAN_POINT('Ctrl Pts',(4.79785036204331,-4.7752448146317,126.053459989004));
#40220=CARTESIAN_POINT('Ctrl Pts',(4.91858409228166,-4.65078571309535,126.061585900665));
#40221=CARTESIAN_POINT('Ctrl Pts',(5.03430329756695,-4.52195525277579,126.069711812325));
#40222=CARTESIAN_POINT('Ctrl Pts',(5.1507625392001,-4.39230090826939,126.077889690035));
#40223=CARTESIAN_POINT('Ctrl Pts',(5.26214264545633,-4.25821937975416,126.086067567745));
#40224=CARTESIAN_POINT('Ctrl Pts',(5.36810629527053,-4.12016065253249,126.094245445455));
#40225=CARTESIAN_POINT('Ctrl Pts',(5.47356420356573,-3.98276084967344,126.102384291929));
#40226=CARTESIAN_POINT('Ctrl Pts',(5.5736570840351,-3.84142206365063,126.110523138402));
#40227=CARTESIAN_POINT('Ctrl Pts',(5.66809683140575,-3.69661565621964,126.118661984875));
#40228=CARTESIAN_POINT('Ctrl Pts',(5.76321593182907,-3.55076758277752,126.126859378204));
#40229=CARTESIAN_POINT('Ctrl Pts',(5.85260006682131,-3.40140213526468,126.135056771532));
#40230=CARTESIAN_POINT('Ctrl Pts',(5.93600286567616,-3.24902431180261,126.143254164861));
#40231=CARTESIAN_POINT('Ctrl Pts',(6.01940566453096,-3.09664648834064,126.151451558189));
#40232=CARTESIAN_POINT('Ctrl Pts',(6.09682701594818,-2.9412566493515,126.159648951518));
#40233=CARTESIAN_POINT('Ctrl Pts',(6.16807069414603,-2.78337796786872,126.167846344846));
#40234=CARTESIAN_POINT('Ctrl Pts',(6.23956481274092,-2.62494430100793,126.176072554183));
#40235=CARTESIAN_POINT('Ctrl Pts',(6.30505063601268,-2.46353278482734,126.18429876352));
#40236=CARTESIAN_POINT('Ctrl Pts',(6.36427136386523,-2.2996388862352,126.192524972857));
#40237=CARTESIAN_POINT('Ctrl Pts',(6.42342555976696,-2.13592911541713,126.2007419404));
#40238=CARTESIAN_POINT('Ctrl Pts',(6.47632855517849,-1.96974284977542,126.208958907943));
#40239=CARTESIAN_POINT('Ctrl Pts',(6.52277033073405,-1.80159823836937,126.217175875487));
#40240=CARTESIAN_POINT('Ctrl Pts',(6.56916925218075,-1.63360878226038,126.22538526083));
#40241=CARTESIAN_POINT('Ctrl Pts',(6.60911873260524,-1.46366492273824,126.233594646173));
#40242=CARTESIAN_POINT('Ctrl Pts',(6.64245754800751,-1.2923028758453,126.241804031517));
#40243=CARTESIAN_POINT('Ctrl Pts',(6.67577228926573,-1.12106457043968,126.250007488817));
#40244=CARTESIAN_POINT('Ctrl Pts',(6.70248580547753,-0.948410468066173,
126.258210946118));
#40245=CARTESIAN_POINT('Ctrl Pts',(6.72248721792287,-0.774890059856023,
126.266414403419));
#40246=CARTESIAN_POINT('Ctrl Pts',(6.74247819947153,-0.601460143927614,
126.27461358255));
#40247=CARTESIAN_POINT('Ctrl Pts',(6.75576400973546,-0.42716517762927,126.282812761682));
#40248=CARTESIAN_POINT('Ctrl Pts',(6.76228518536541,-0.252563005579774,
126.291011940814));
#40249=CARTESIAN_POINT('Ctrl Pts',(6.76880513226528,-0.0779937323438108,
126.299209575044));
#40250=CARTESIAN_POINT('Ctrl Pts',(6.76856296382229,0.0968822735593504,
126.307407209274));
#40251=CARTESIAN_POINT('Ctrl Pts',(6.76155121244582,0.271503593848233,126.315604843504));
#40252=CARTESIAN_POINT('Ctrl Pts',(6.75453996718524,0.446112309778875,126.323801886019));
#40253=CARTESIAN_POINT('Ctrl Pts',(6.74076012564427,0.620466018281871,126.331998928535));
#40254=CARTESIAN_POINT('Ctrl Pts',(6.7202563349705,0.794004906967783,126.34019597105));
#40255=CARTESIAN_POINT('Ctrl Pts',(6.69975029775319,0.967562809828921,126.348393911693));
#40256=CARTESIAN_POINT('Ctrl Pts',(6.67251888572896,1.14030535872973,126.356591852336));
#40257=CARTESIAN_POINT('Ctrl Pts',(6.63865845961037,1.31167940314837,126.364789792979));
#40258=CARTESIAN_POINT('Ctrl Pts',(6.60478816939993,1.48310337160845,126.372990121815));
#40259=CARTESIAN_POINT('Ctrl Pts',(6.56428508800642,1.65315768969983,126.381190450651));
#40260=CARTESIAN_POINT('Ctrl Pts',(6.51729638575349,1.82130085934328,126.389390779487));
#40261=CARTESIAN_POINT('Ctrl Pts',(6.47025872005376,1.98961923853169,126.397599653278));
#40262=CARTESIAN_POINT('Ctrl Pts',(6.41672202832614,2.15602214472305,126.40580852707));
#40263=CARTESIAN_POINT('Ctrl Pts',(6.35688324221719,2.31998371649852,126.414017400861));
#40264=CARTESIAN_POINT('Ctrl Pts',(6.29701234129188,2.48403328464072,126.422230680265));
#40265=CARTESIAN_POINT('Ctrl Pts',(6.23083273911924,2.64563857475918,126.430443959668));
#40266=CARTESIAN_POINT('Ctrl Pts',(6.15858891991479,2.80429519050737,126.438657239071));
#40267=CARTESIAN_POINT('Ctrl Pts',(6.08623943277005,2.96318386649247,126.446882531687));
#40268=CARTESIAN_POINT('Ctrl Pts',(6.00780816389592,3.11911492864928,126.455107824302));
#40269=CARTESIAN_POINT('Ctrl Pts',(5.92358543184648,3.27160887509741,126.463333116918));
#40270=CARTESIAN_POINT('Ctrl Pts',(5.84741608791609,3.40952133141019,126.47077190603));
#40271=CARTESIAN_POINT('Ctrl Pts',(5.76651056850129,3.54462275421643,126.478210695142));
#40272=CARTESIAN_POINT('Ctrl Pts',(5.68111296843999,3.67658053628953,126.485649484254));
#40273=CARTESIAN_POINT('Ctrl Pts',(5.58667845118299,3.82250231207049,126.4938754585));
#40274=CARTESIAN_POINT('Ctrl Pts',(5.48648624044273,3.96498731542591,126.502101432746));
#40275=CARTESIAN_POINT('Ctrl Pts',(5.38081365457187,4.10355131742896,126.510327406992));
#40276=CARTESIAN_POINT('Ctrl Pts',(5.27525496088637,4.24196597741609,126.518544515417));
#40277=CARTESIAN_POINT('Ctrl Pts',(5.16422786736725,4.37646776719986,126.526761623842));
#40278=CARTESIAN_POINT('Ctrl Pts',(5.04805414095819,4.50659942639179,126.534978732268));
#40279=CARTESIAN_POINT('Ctrl Pts',(4.93198449783409,4.63661449699711,126.543188478756));
#40280=CARTESIAN_POINT('Ctrl Pts',(4.8107776411001,4.76226696770519,126.551398225245));
#40281=CARTESIAN_POINT('Ctrl Pts',(4.68479699099187,4.88313077371409,126.559607971733));
#40282=CARTESIAN_POINT('Ctrl Pts',(4.55891905785163,5.00389603471879,126.567811024493));
#40283=CARTESIAN_POINT('Ctrl Pts',(4.42827534534742,5.11988016414388,126.576014077253));
#40284=CARTESIAN_POINT('Ctrl Pts',(4.29326759855843,5.23069233726935,126.584217130013));
#40285=CARTESIAN_POINT('Ctrl Pts',(4.1583245922381,5.34145137246614,126.592416249151));
#40286=CARTESIAN_POINT('Ctrl Pts',(4.01902199568574,5.44704316348565,126.600615368289));
#40287=CARTESIAN_POINT('Ctrl Pts',(3.87579647803769,5.54711552618391,126.608814487427));
#40288=CARTESIAN_POINT('Ctrl Pts',(3.7326042956021,5.64716459740782,126.61701169825));
#40289=CARTESIAN_POINT('Ctrl Pts',(3.58549130240188,5.74169659109429,126.625208909073));
#40290=CARTESIAN_POINT('Ctrl Pts',(3.43492527580759,5.83040113110737,126.633406119896));
#40291=CARTESIAN_POINT('Ctrl Pts',(3.3247914955315,5.89528539843029,126.639402092799));
#40292=CARTESIAN_POINT('Ctrl Pts',(3.21281087344299,5.95705259306496,126.645398065703));
#40293=CARTESIAN_POINT('Ctrl Pts',(3.09917575053261,6.01559628526638,126.651394038606));
#40294=CARTESIAN_POINT('Origin',(0.,0.,-3.69717978381041));
#40295=CARTESIAN_POINT('',(3.09917575053253,6.01559628526642,129.045751582742));
#40296=CARTESIAN_POINT('',(3.09917575053256,6.01559628526641,128.651204297413));
#40297=CARTESIAN_POINT('',(3.09917575053259,6.01559628526639,-3.69717978381041));
#40298=CARTESIAN_POINT('',(-6.767,7.58899778956212E-12,127.69717978381));
#40299=CARTESIAN_POINT('Ctrl Pts',(-6.767,7.58899730750792E-12,127.69717978381));
#40300=CARTESIAN_POINT('Ctrl Pts',(-6.76700000000021,-0.186007249408207,
127.705929295616));
#40301=CARTESIAN_POINT('Ctrl Pts',(-6.75932637295479,-0.372014355520188,
127.714678807422));
#40302=CARTESIAN_POINT('Ctrl Pts',(-6.74400518266988,-0.557389537147837,
127.723428319228));
#40303=CARTESIAN_POINT('Ctrl Pts',(-6.72868405709723,-0.742763935804457,
127.732177794078));
#40304=CARTESIAN_POINT('Ctrl Pts',(-6.70571545653084,-0.927506129688376,
127.740927268929));
#40305=CARTESIAN_POINT('Ctrl Pts',(-6.67517739415756,-1.11098863924338,
127.74967674378));
#40306=CARTESIAN_POINT('Ctrl Pts',(-6.64463945823188,-1.29447038906054,
127.758426182402));
#40307=CARTESIAN_POINT('Ctrl Pts',(-6.60653217027252,-1.47669218227794,
127.767175621024));
#40308=CARTESIAN_POINT('Ctrl Pts',(-6.56098496116812,-1.65703510503724,
127.775925059646));
#40309=CARTESIAN_POINT('Ctrl Pts',(-6.51543793687625,-1.8373772960364,127.784674462766));
#40310=CARTESIAN_POINT('Ctrl Pts',(-6.46245112202753,-2.01584035396688,
127.793423865886));
#40311=CARTESIAN_POINT('Ctrl Pts',(-6.40220448416362,-2.19181813637795,
127.802173269006));
#40312=CARTESIAN_POINT('Ctrl Pts',(-6.34195808575317,-2.36779521935593,
127.810922637352));
#40313=CARTESIAN_POINT('Ctrl Pts',(-6.27445201489377,-2.54128677544476,
127.819672005697));
#40314=CARTESIAN_POINT('Ctrl Pts',(-6.19991555136338,-2.71170355237489,
127.828421374042));
#40315=CARTESIAN_POINT('Ctrl Pts',(-6.12537937789207,-2.88211966612712,
127.837170708339));
#40316=CARTESIAN_POINT('Ctrl Pts',(-6.04381298133802,-3.04946076210077,
127.845920042636));
#40317=CARTESIAN_POINT('Ctrl Pts',(-5.95549339426508,-3.21315848206481,
127.854669376933));
#40318=CARTESIAN_POINT('Ctrl Pts',(-5.86717414355366,-3.3768555785928,127.863418677909));
#40319=CARTESIAN_POINT('Ctrl Pts',(-5.77210188986446,-3.53690907466972,
127.872167978884));
#40320=CARTESIAN_POINT('Ctrl Pts',(-5.67059953467278,-3.69277536784583,
127.88091727986));
#40321=CARTESIAN_POINT('Ctrl Pts',(-5.56909755761985,-3.84864108035475,
127.889666548241));
#40322=CARTESIAN_POINT('Ctrl Pts',(-5.46116568338299,-4.00031938103966,
127.898415816621));
#40323=CARTESIAN_POINT('Ctrl Pts',(-5.34717048686353,-4.14729511662911,
127.907165085002));
#40324=CARTESIAN_POINT('Ctrl Pts',(-5.23317570555759,-4.29427031687747,
127.915914321515));
#40325=CARTESIAN_POINT('Ctrl Pts',(-5.11311782179048,-4.4365427598685,127.924663558027));
#40326=CARTESIAN_POINT('Ctrl Pts',(-4.98740459172257,-4.57362924147384,
127.93341279454));
#40327=CARTESIAN_POINT('Ctrl Pts',(-4.86169180911079,-4.7107152351418,127.942161999911));
#40328=CARTESIAN_POINT('Ctrl Pts',(-4.73032391415684,-4.84261509316276,
127.950911205282));
#40329=CARTESIAN_POINT('Ctrl Pts',(-4.59374707237551,-4.96888084331285,
127.959660410653));
#40330=CARTESIAN_POINT('Ctrl Pts',(-4.45717070537675,-5.09514615452485,
127.96840958561));
#40331=CARTESIAN_POINT('Ctrl Pts',(-4.31538563819798,-5.21577720253393,
127.977158760566));
#40332=CARTESIAN_POINT('Ctrl Pts',(-4.16887341290952,-5.33036429028412,
127.985907935522));
#40333=CARTESIAN_POINT('Ctrl Pts',(-4.02236168477642,-5.44495098920953,
127.99465708079));
#40334=CARTESIAN_POINT('Ctrl Pts',(-3.8711230563474,-5.55349359238549,128.003406226058));
#40335=CARTESIAN_POINT('Ctrl Pts',(-3.71567117317031,-5.65562346102277,
128.012155371326));
#40336=CARTESIAN_POINT('Ctrl Pts',(-3.56021980457621,-5.75775299158571,
128.020904487632));
#40337=CARTESIAN_POINT('Ctrl Pts',(-3.4005554486273,-5.85346967275154,128.029653603938));
#40338=CARTESIAN_POINT('Ctrl Pts',(-3.23722036323768,-5.94244842803363,
128.038402720244));
#40339=CARTESIAN_POINT('Ctrl Pts',(-3.0738858049641,-6.0314268961629,128.047151808315));
#40340=CARTESIAN_POINT('Ctrl Pts',(-2.90688079258068,-6.11366734484651,
128.055900896386));
#40341=CARTESIAN_POINT('Ctrl Pts',(-2.73677251094973,-6.18889046787144,
128.064649984457));
#40342=CARTESIAN_POINT('Ctrl Pts',(-2.56666476416983,-6.26411335438133,
128.073399045019));
#40343=CARTESIAN_POINT('Ctrl Pts',(-2.39345402972409,-6.33231884350172,
128.082148105582));
#40344=CARTESIAN_POINT('Ctrl Pts',(-2.21772856474332,-6.39327529620941,
128.090897166144));
#40345=CARTESIAN_POINT('Ctrl Pts',(-2.04200363768575,-6.45423156231985,
128.099646199924));
#40346=CARTESIAN_POINT('Ctrl Pts',(-1.8637642662041,-6.50793874251965,128.108395233704));
#40347=CARTESIAN_POINT('Ctrl Pts',(-1.68361578195017,-6.55421443796038,
128.117144267484));
#40348=CARTESIAN_POINT('Ctrl Pts',(-1.50346783420211,-6.60048999558601,
128.125893275208));
#40349=CARTESIAN_POINT('Ctrl Pts',(-1.32141106257604,-6.63933404145424,
128.134642282932));
#40350=CARTESIAN_POINT('Ctrl Pts',(-1.13806375959417,-6.67061465526966,
128.143391290657));
#40351=CARTESIAN_POINT('Ctrl Pts',(-0.954716987422707,-6.7018951785243,
128.152140273051));
#40352=CARTESIAN_POINT('Ctrl Pts',(-0.770079973813257,-6.7256122653579,
128.160889255446));
#40353=CARTESIAN_POINT('Ctrl Pts',(-0.584779770555658,-6.74168536939754,
128.169638237841));
#40354=CARTESIAN_POINT('Ctrl Pts',(-0.391490647557111,-6.75845143942375,
128.178764418517));
#40355=CARTESIAN_POINT('Ctrl Pts',(-0.197480213107528,-6.76689975924017,
128.187890599193));
#40356=CARTESIAN_POINT('Ctrl Pts',(-0.00346532630097921,-6.76699911271707,
128.197016779869));
#40357=CARTESIAN_POINT('Ctrl Pts',(0.184486595292832,-6.76709536139782,
128.205857767399));
#40358=CARTESIAN_POINT('Ctrl Pts',(0.372442378181968,-6.75935659726788,
128.214698754929));
#40359=CARTESIAN_POINT('Ctrl Pts',(0.559750217718792,-6.74380965729044,
128.223539742459));
#40360=CARTESIAN_POINT('Ctrl Pts',(0.745129914454466,-6.7284227571729,128.232289721057));
#40361=CARTESIAN_POINT('Ctrl Pts',(0.929874656310905,-6.70538772273518,
128.241039699655));
#40362=CARTESIAN_POINT('Ctrl Pts',(1.11335688289451,-6.67478280180797,128.249789678252));
#40363=CARTESIAN_POINT('Ctrl Pts',(1.29683723118518,-6.64417819418089,128.258539567277));
#40364=CARTESIAN_POINT('Ctrl Pts',(1.47905480729886,-6.60600390230153,128.267289456302));
#40365=CARTESIAN_POINT('Ctrl Pts',(1.65939064804448,-6.56038959797225,128.276039345327));
#40366=CARTESIAN_POINT('Ctrl Pts',(1.83972470263913,-6.51477574543356,128.284789147688));
#40367=CARTESIAN_POINT('Ctrl Pts',(2.01817678125503,-6.46172209820208,128.293538950049));
#40368=CARTESIAN_POINT('Ctrl Pts',(2.19414072347343,-6.4014088672413,128.30228875241));
#40369=CARTESIAN_POINT('Ctrl Pts',(2.37010298131771,-6.34109621361496,128.311038471016));
#40370=CARTESIAN_POINT('Ctrl Pts',(2.54357687926597,-6.27352420826099,128.319788189621));
#40371=CARTESIAN_POINT('Ctrl Pts',(2.71397317789666,-6.1989223732563,128.328537908227));
#40372=CARTESIAN_POINT('Ctrl Pts',(2.88436790206904,-6.12432122757104,128.337287545985));
#40373=CARTESIAN_POINT('Ctrl Pts',(3.05168482125968,-6.04269049717563,128.346037183743));
#40374=CARTESIAN_POINT('Ctrl Pts',(3.21535561997108,-5.95430745235081,128.354786821501));
#40375=CARTESIAN_POINT('Ctrl Pts',(3.37902496075003,-5.86592519481676,128.36353638132));
#40376=CARTESIAN_POINT('Ctrl Pts',(3.53904799384601,-5.770790879404,128.372285941139));
#40377=CARTESIAN_POINT('Ctrl Pts',(3.69488118814714,-5.669227637472,128.381035500958));
#40378=CARTESIAN_POINT('Ctrl Pts',(3.85071304610559,-5.56766526649241,128.389784985746));
#40379=CARTESIAN_POINT('Ctrl Pts',(4.0023548970569,-5.45967423580917,128.398534470533));
#40380=CARTESIAN_POINT('Ctrl Pts',(4.14929168607374,-5.34562133936546,128.407283955321));
#40381=CARTESIAN_POINT('Ctrl Pts',(4.29622726385473,-5.23156938308763,128.416033367984));
#40382=CARTESIAN_POINT('Ctrl Pts',(4.4384576309178,-5.11145583677451,128.424782780647));
#40383=CARTESIAN_POINT('Ctrl Pts',(4.57549970660673,-4.98568866204476,128.433532193311));
#40384=CARTESIAN_POINT('Ctrl Pts',(4.71254069815016,-4.85992248226432,128.442281536757));
#40385=CARTESIAN_POINT('Ctrl Pts',(4.84439326931045,-4.72850295734278,128.451030880203));
#40386=CARTESIAN_POINT('Ctrl Pts',(4.97060959434439,-4.59187644221962,128.45978022365));
#40387=CARTESIAN_POINT('Ctrl Pts',(5.09682496280269,-4.45525096256946,128.468529500786));
#40388=CARTESIAN_POINT('Ctrl Pts',(5.21740397615605,-4.3134187821861,128.477278777922));
#40389=CARTESIAN_POINT('Ctrl Pts',(5.33193710451712,-4.16686161438962,128.486028055058));
#40390=CARTESIAN_POINT('Ctrl Pts',(5.44646940289165,-4.02030550864809,128.494777268791));
#40391=CARTESIAN_POINT('Ctrl Pts',(5.55495572749452,-3.86902470980439,128.503526482524));
#40392=CARTESIAN_POINT('Ctrl Pts',(5.65702762491248,-3.71353301466098,128.512275696257));
#40393=CARTESIAN_POINT('Ctrl Pts',(5.75909881654957,-3.55804239467212,128.521024849494));
#40394=CARTESIAN_POINT('Ctrl Pts',(5.85475551250595,-3.39834117619875,128.52977400273));
#40395=CARTESIAN_POINT('Ctrl Pts',(5.94367283727918,-3.23497174692294,128.538523155966));
#40396=CARTESIAN_POINT('Ctrl Pts',(6.03258957676146,-3.07160339301292,128.547272251611));
#40397=CARTESIAN_POINT('Ctrl Pts',(6.11476689685129,-2.90456712829831,128.556021347257));
#40398=CARTESIAN_POINT('Ctrl Pts',(6.18992570525116,-2.73443024476232,128.564770442902));
#40399=CARTESIAN_POINT('Ctrl Pts',(6.2650840438857,-2.56429442463343,128.573519483863));
#40400=CARTESIAN_POINT('Ctrl Pts',(6.33322384283203,-2.39105828656292,128.582268524824));
#40401=CARTESIAN_POINT('Ctrl Pts',(6.39411368719935,-2.21531017132365,128.591017565785));
#40402=CARTESIAN_POINT('Ctrl Pts',(6.45500317120798,-2.03956309619804,128.599766554968));
#40403=CARTESIAN_POINT('Ctrl Pts',(6.50864269269989,-1.86130434438929,128.60851554415));
#40404=CARTESIAN_POINT('Ctrl Pts',(6.55485008446256,-1.68113930720245,128.617264533333));
#40405=CARTESIAN_POINT('Ctrl Pts',(6.60199664749336,-1.49731239212138,128.626191346862));
#40406=CARTESIAN_POINT('Ctrl Pts',(6.64140563640849,-1.31150116499966,128.635118160391));
#40407=CARTESIAN_POINT('Ctrl Pts',(6.67293772282123,-1.12436255155951,128.644044973921));
#40408=CARTESIAN_POINT('Ctrl Pts',(6.70384494949829,-0.940932395054325,
128.652794888076));
#40409=CARTESIAN_POINT('Ctrl Pts',(6.72718449348896,-0.756227260509767,
128.661544802232));
#40410=CARTESIAN_POINT('Ctrl Pts',(6.74287707373906,-0.570874564544813,
128.670294716387));
#40411=CARTESIAN_POINT('Ctrl Pts',(6.75856934538653,-0.385525513635557,
128.679044458471));
#40412=CARTESIAN_POINT('Ctrl Pts',(6.76661493004094,-0.199529212421269,
128.687794200555));
#40413=CARTESIAN_POINT('Ctrl Pts',(6.76698649908906,-0.0135174386034205,
128.696543942639));
#40414=CARTESIAN_POINT('Ctrl Pts',(6.76735806132397,0.172490924442862,128.705293524285));
#40415=CARTESIAN_POINT('Ctrl Pts',(6.76005588896304,0.35851447289857,128.714043105931));
#40416=CARTESIAN_POINT('Ctrl Pts',(6.74510478454607,0.543921359659458,128.722792687577));
#40417=CARTESIAN_POINT('Ctrl Pts',(6.73015393440717,0.729325093147752,128.731542120416));
#40418=CARTESIAN_POINT('Ctrl Pts',(6.70755443556933,0.914111900253724,128.740291553255));
#40419=CARTESIAN_POINT('Ctrl Pts',(6.67738304682361,1.09765415591282,128.749040986094));
#40420=CARTESIAN_POINT('Ctrl Pts',(6.6472121311191,1.28119353391013,128.757790281755));
#40421=CARTESIAN_POINT('Ctrl Pts',(6.60946960955552,1.4634881167239,128.766539577417));
#40422=CARTESIAN_POINT('Ctrl Pts',(6.5642836699125,1.64391876347956,128.775288873078));
#40423=CARTESIAN_POINT('Ctrl Pts',(6.51909837867792,1.82434682109449,128.784038043189));
#40424=CARTESIAN_POINT('Ctrl Pts',(6.46646995272004,2.00291071820178,128.7927872133));
#40425=CARTESIAN_POINT('Ctrl Pts',(6.4065771328164,2.17900400212436,128.801536383411));
#40426=CARTESIAN_POINT('Ctrl Pts',(6.34668509279158,2.35509499309393,128.810285439596));
#40427=CARTESIAN_POINT('Ctrl Pts',(6.27952894037632,2.52871516397859,128.819034495782));
#40428=CARTESIAN_POINT('Ctrl Pts',(6.20533675061561,2.69927486771158,128.827783551968));
#40429=CARTESIAN_POINT('Ctrl Pts',(6.12832117908032,2.87632521635678,128.83686555325));
#40430=CARTESIAN_POINT('Ctrl Pts',(6.04372366626195,3.05007728919768,128.845947554532));
#40431=CARTESIAN_POINT('Ctrl Pts',(5.95185378007983,3.21989527477982,128.855029555815));
#40432=CARTESIAN_POINT('Ctrl Pts',(5.86334450817489,3.38350129286548,128.863779336122));
#40433=CARTESIAN_POINT('Ctrl Pts',(5.76808562057375,3.54345567124769,128.872529116429));
#40434=CARTESIAN_POINT('Ctrl Pts',(5.66640068804604,3.69921508465126,128.881278896736));
#40435=CARTESIAN_POINT('Ctrl Pts',(5.56471941108052,3.85496889852097,128.89002836249));
#40436=CARTESIAN_POINT('Ctrl Pts',(5.45661270815251,4.00652780919449,128.898777828243));
#40437=CARTESIAN_POINT('Ctrl Pts',(5.34244776449261,4.1533770456904,128.907527293997));
#40438=CARTESIAN_POINT('Ctrl Pts',(5.2282863181974,4.30022178356074,128.916276491716));
#40439=CARTESIAN_POINT('Ctrl Pts',(5.10806717844212,4.44235690972516,128.925025689436));
#40440=CARTESIAN_POINT('Ctrl Pts',(4.98219864544858,4.57929969070494,128.933774887155));
#40441=CARTESIAN_POINT('Ctrl Pts',(4.85633329944169,4.71623900429852,128.942523863346));
#40442=CARTESIAN_POINT('Ctrl Pts',(4.72481904033798,4.84798602483471,128.951272839536));
#40443=CARTESIAN_POINT('Ctrl Pts',(4.58810250737353,4.97409332258983,128.960021815726));
#40444=CARTESIAN_POINT('Ctrl Pts',(4.45137708685805,5.10020881821993,128.968771360662));
#40445=CARTESIAN_POINT('Ctrl Pts',(4.30944892636222,5.22068366307792,128.977520905598));
#40446=CARTESIAN_POINT('Ctrl Pts',(4.1628000946684,5.33510865604711,128.986270450535));
#40447=CARTESIAN_POINT('Ctrl Pts',(4.01615988348958,5.44952692272767,128.995019481143));
#40448=CARTESIAN_POINT('Ctrl Pts',(3.8647997823239,5.55789587288516,129.003768511751));
#40449=CARTESIAN_POINT('Ctrl Pts',(3.70923383581215,5.65984746713781,129.012517542359));
#40450=CARTESIAN_POINT('Ctrl Pts',(3.55366577799683,5.76180044505295,129.021266691707));
#40451=CARTESIAN_POINT('Ctrl Pts',(3.39389200026977,5.8573357357098,129.030015841055));
#40452=CARTESIAN_POINT('Ctrl Pts',(3.23045513626172,5.94612887621857,129.038764990404));
#40453=CARTESIAN_POINT('Ctrl Pts',(3.18695122151664,5.96976399206643,129.041093854517));
#40454=CARTESIAN_POINT('Ctrl Pts',(3.14318791262705,5.99292165435312,129.043422718629));
#40455=CARTESIAN_POINT('Ctrl Pts',(3.09917575053253,6.01559628526642,129.045751582742));
#40456=CARTESIAN_POINT('Ctrl Pts',(3.09917575053273,6.01559628526631,127.045911902629));
#40457=CARTESIAN_POINT('Ctrl Pts',(2.94398502489705,6.09554901327362,127.05411480057));
#40458=CARTESIAN_POINT('Ctrl Pts',(2.78560179809225,6.16954220727552,127.062317698511));
#40459=CARTESIAN_POINT('Ctrl Pts',(2.62452527368248,6.23731962366864,127.070520596452));
#40460=CARTESIAN_POINT('Ctrl Pts',(2.46249362782818,6.30549893390749,127.078772134402));
#40461=CARTESIAN_POINT('Ctrl Pts',(2.29773695407367,6.3673883226108,127.087023672353));
#40462=CARTESIAN_POINT('Ctrl Pts',(2.13078641942083,6.42277496373739,127.095275210304));
#40463=CARTESIAN_POINT('Ctrl Pts',(1.96490192961397,6.47780793936998,127.103474058938));
#40464=CARTESIAN_POINT('Ctrl Pts',(1.79685186523018,6.52642087548502,127.111672907573));
#40465=CARTESIAN_POINT('Ctrl Pts',(1.62717491405476,6.56845421686647,127.119871756207));
#40466=CARTESIAN_POINT('Ctrl Pts',(1.45749451425469,6.61048841256087,127.12807077148));
#40467=CARTESIAN_POINT('Ctrl Pts',(1.28618750966292,6.6459426607097,127.136269786754));
#40468=CARTESIAN_POINT('Ctrl Pts',(1.11380504865354,6.67470803208604,127.144468802027));
#40469=CARTESIAN_POINT('Ctrl Pts',(0.941387813069357,6.70347920627754,127.152669471281));
#40470=CARTESIAN_POINT('Ctrl Pts',(0.767895042453905,6.72555875720563,127.160870140535));
#40471=CARTESIAN_POINT('Ctrl Pts',(0.593885370547981,6.74088934537937,127.169070809789));
#40472=CARTESIAN_POINT('Ctrl Pts',(0.417968350331196,6.75638797462311,127.177361367912));
#40473=CARTESIAN_POINT('Ctrl Pts',(0.241523403679143,6.76498877367479,127.185651926035));
#40474=CARTESIAN_POINT('Ctrl Pts',(0.0651295830442705,6.76668657005868,
127.193942484159));
#40475=CARTESIAN_POINT('Ctrl Pts',(-0.109594544721961,6.76836829559323,
127.202154566257));
#40476=CARTESIAN_POINT('Ctrl Pts',(-0.284268152398203,6.76327720213396,
127.210366648356));
#40477=CARTESIAN_POINT('Ctrl Pts',(-0.458332117798099,6.75146063232207,
127.218578730455));
#40478=CARTESIAN_POINT('Ctrl Pts',(-0.634891159568652,6.73947468084608,
127.22690852659));
#40479=CARTESIAN_POINT('Ctrl Pts',(-0.810822565445924,6.72056901307334,
127.235238322726));
#40480=CARTESIAN_POINT('Ctrl Pts',(-0.985552264639139,6.69484695371483,
127.243568118861));
#40481=CARTESIAN_POINT('Ctrl Pts',(-1.16028196383248,6.6691248943563,127.251897914997));
#40482=CARTESIAN_POINT('Ctrl Pts',(-1.3338095928365,6.63658656471674,127.260227711132));
#40483=CARTESIAN_POINT('Ctrl Pts',(-1.50557612075279,6.59738808503934,127.268557507268));
#40484=CARTESIAN_POINT('Ctrl Pts',(-1.68385719114858,6.55670293526335,127.27720322532));
#40485=CARTESIAN_POINT('Ctrl Pts',(-1.86064759279046,6.50875066070558,127.285848943373));
#40486=CARTESIAN_POINT('Ctrl Pts',(-2.0353473042416,6.45365403094375,127.294494661425));
#40487=CARTESIAN_POINT('Ctrl Pts',(-2.20982273686541,6.39862813402635,127.303129280137));
#40488=CARTESIAN_POINT('Ctrl Pts',(-2.38221254190671,6.33647626243224,127.31176389885));
#40489=CARTESIAN_POINT('Ctrl Pts',(-2.55192873554816,6.26737175606199,127.320398517562));
#40490=CARTESIAN_POINT('Ctrl Pts',(-2.72763864585318,6.19582674697676,127.329338077464));
#40491=CARTESIAN_POINT('Ctrl Pts',(-2.90048233561038,6.11682910355213,127.338277637367));
#40492=CARTESIAN_POINT('Ctrl Pts',(-3.06982345566104,6.0306279068662,127.347217197269));
#40493=CARTESIAN_POINT('Ctrl Pts',(-3.23293413282105,5.94759824721095,127.35582785054));
#40494=CARTESIAN_POINT('Ctrl Pts',(-3.392795046907,5.85788576583019,127.36443850381));
#40495=CARTESIAN_POINT('Ctrl Pts',(-3.54885651637059,5.7617624409736,127.373049157081));
#40496=CARTESIAN_POINT('Ctrl Pts',(-3.7047702632137,5.66573010327409,127.381651659792));
#40497=CARTESIAN_POINT('Ctrl Pts',(-3.85689147691732,5.56329918006359,127.390254162503));
#40498=CARTESIAN_POINT('Ctrl Pts',(-4.00469493663627,5.45478757280976,127.398856665214));
#40499=CARTESIAN_POINT('Ctrl Pts',(-4.1523320465364,5.3463980931857,127.407449485982));
#40500=CARTESIAN_POINT('Ctrl Pts',(-4.29566085177274,5.2319417625806,127.416042306749));
#40501=CARTESIAN_POINT('Ctrl Pts',(-4.43418482626982,5.11177991764889,127.424635127517));
#40502=CARTESIAN_POINT('Ctrl Pts',(-4.45051050587183,5.09761829842114,127.425647830475));
#40503=CARTESIAN_POINT('Ctrl Pts',(-4.46676948127015,5.08337748059413,127.426660533433));
#40504=CARTESIAN_POINT('Ctrl Pts',(-4.48296096696515,5.06905809482067,127.427673236391));
#40505=CARTESIAN_POINT('Ctrl Pts',(-4.62038526494443,4.94752313660364,127.436268494151));
#40506=CARTESIAN_POINT('Ctrl Pts',(-4.75278342515784,4.82046811009498,127.444863751911));
#40507=CARTESIAN_POINT('Ctrl Pts',(-4.87973112664818,4.68833799246821,127.453459009671));
#40508=CARTESIAN_POINT('Ctrl Pts',(-5.0067977092774,4.55608414058963,127.462062316525));
#40509=CARTESIAN_POINT('Ctrl Pts',(-5.12840343360427,4.41874593139391,127.47066562338));
#40510=CARTESIAN_POINT('Ctrl Pts',(-5.24416350962005,4.27680232000142,127.479268930234));
#40511=CARTESIAN_POINT('Ctrl Pts',(-5.36472303853082,4.12897367725727,127.488228933174));
#40512=CARTESIAN_POINT('Ctrl Pts',(-5.47894163461994,3.97614991560686,127.497188936114));
#40513=CARTESIAN_POINT('Ctrl Pts',(-5.58643455662435,3.81890533327985,127.506148939054));
#40514=CARTESIAN_POINT('Ctrl Pts',(-5.68993056995751,3.66750757531013,127.514775782259));
#40515=CARTESIAN_POINT('Ctrl Pts',(-5.78719193407782,3.51201210266221,127.523402625464));
#40516=CARTESIAN_POINT('Ctrl Pts',(-5.87792211240528,3.35295699950015,127.532029468668));
#40517=CARTESIAN_POINT('Ctrl Pts',(-5.96873900584857,3.1937498798652,127.540664556954));
#40518=CARTESIAN_POINT('Ctrl Pts',(-6.05301211073054,3.03097660808893,127.549299645241));
#40519=CARTESIAN_POINT('Ctrl Pts',(-6.13049196839731,2.86519758924513,127.557934733527));
#40520=CARTESIAN_POINT('Ctrl Pts',(-6.20808689920134,2.69917235528989,127.566582646652));
#40521=CARTESIAN_POINT('Ctrl Pts',(-6.27886829901054,2.53013273296519,127.575230559777));
#40522=CARTESIAN_POINT('Ctrl Pts',(-6.34263517387559,2.35865810390489,127.583878472902));
#40523=CARTESIAN_POINT('Ctrl Pts',(-6.34978884650288,2.33942126090797,127.584848637106));
#40524=CARTESIAN_POINT('Ctrl Pts',(-6.35685429040264,2.32015378663128,127.58581880131));
#40525=CARTESIAN_POINT('Ctrl Pts',(-6.36383126134657,2.30085650945647,127.586788965515));
#40526=CARTESIAN_POINT('Ctrl Pts',(-6.43074697946329,2.11577745864367,127.596093753357));
#40527=CARTESIAN_POINT('Ctrl Pts',(-6.48963299559788,1.92764419908136,127.605398541199));
#40528=CARTESIAN_POINT('Ctrl Pts',(-6.54023679096125,1.73712167626706,127.614703329041));
#40529=CARTESIAN_POINT('Ctrl Pts',(-6.59070015032034,1.54712789288107,127.623982294171));
#40530=CARTESIAN_POINT('Ctrl Pts',(-6.63292709922294,1.35475824550878,127.633261259301));
#40531=CARTESIAN_POINT('Ctrl Pts',(-6.66671434958378,1.1606932329663,127.642540224431));
#40532=CARTESIAN_POINT('Ctrl Pts',(-6.70031803070446,0.967682593493919,
127.65176877609));
#40533=CARTESIAN_POINT('Ctrl Pts',(-6.72557339603793,0.772995129116876,
127.660997327749));
#40534=CARTESIAN_POINT('Ctrl Pts',(-6.74232838574441,0.577318749726029,
127.670225879408));
#40535=CARTESIAN_POINT('Ctrl Pts',(-6.75864052974762,0.386814229307502,
127.679210514209));
#40536=CARTESIAN_POINT('Ctrl Pts',(-6.76689579452237,0.195372590733599,
127.688195149009));
#40537=CARTESIAN_POINT('Ctrl Pts',(-6.76699901925401,0.00364326986908226,
127.69717978381));
#40538=CARTESIAN_POINT('',(-6.76699990560448,-0.00113028709160019,127.302820216231));
#40539=CARTESIAN_POINT('Ctrl Pts',(3.09917575053261,6.01559628526638,126.651394038606));
#40540=CARTESIAN_POINT('Ctrl Pts',(2.94381645487386,6.0956358588835,126.659591593228));
#40541=CARTESIAN_POINT('Ctrl Pts',(2.78536392356738,6.16964823799883,126.667789147851));
#40542=CARTESIAN_POINT('Ctrl Pts',(2.62432973771906,6.23740189724243,126.675986702473));
#40543=CARTESIAN_POINT('Ctrl Pts',(2.46325647582193,6.30517199737578,126.684186246288));
#40544=CARTESIAN_POINT('Ctrl Pts',(2.29960064213102,6.36668021339887,126.692385790104));
#40545=CARTESIAN_POINT('Ctrl Pts',(2.13389282594102,6.42174356443773,126.700585333919));
#40546=CARTESIAN_POINT('Ctrl Pts',(1.96065235544694,6.47930995484877,126.709157608064));
#40547=CARTESIAN_POINT('Ctrl Pts',(1.78516939970454,6.52983170258234,126.717729882209));
#40548=CARTESIAN_POINT('Ctrl Pts',(1.60806593701526,6.57315852100124,126.726302156354));
#40549=CARTESIAN_POINT('Ctrl Pts',(1.43840199385435,6.61466532581434,126.734514338156));
#40550=CARTESIAN_POINT('Ctrl Pts',(1.26725127013855,6.64956931183984,126.742726519958));
#40551=CARTESIAN_POINT('Ctrl Pts',(1.09516889223115,6.67779110915348,126.75093870176));
#40552=CARTESIAN_POINT('Ctrl Pts',(0.92297235080651,6.70603162947457,126.759156331717));
#40553=CARTESIAN_POINT('Ctrl Pts',(0.749843277962059,6.72758108136217,126.767373961674));
#40554=CARTESIAN_POINT('Ctrl Pts',(0.576340570410812,6.74241207187002,126.775591591632));
#40555=CARTESIAN_POINT('Ctrl Pts',(0.402618889735319,6.75726178017411,126.78381959284));
#40556=CARTESIAN_POINT('Ctrl Pts',(0.228522989437664,6.76537608254519,126.792047594048));
#40557=CARTESIAN_POINT('Ctrl Pts',(0.0546111582759515,6.76677963446363,
126.800275595256));
#40558=CARTESIAN_POINT('Ctrl Pts',(0.032227316660986,6.76696028280498,126.801334604725));
#40559=CARTESIAN_POINT('Ctrl Pts',(0.00984651627423833,6.76702983287537,
126.802393614193));
#40560=CARTESIAN_POINT('Ctrl Pts',(-0.0125300605691292,6.76698839939763,
126.803452623661));
#40561=CARTESIAN_POINT('Ctrl Pts',(-0.184791316048411,6.76666943269672,
126.811605179874));
#40562=CARTESIAN_POINT('Ctrl Pts',(-0.35730982263907,6.75976801858847,126.819757736088));
#40563=CARTESIAN_POINT('Ctrl Pts',(-0.529537051957871,6.7462492920588,126.827910292301));
#40564=CARTESIAN_POINT('Ctrl Pts',(-0.701564751879324,6.73274622729973,
126.836053403581));
#40565=CARTESIAN_POINT('Ctrl Pts',(-0.873301485542799,6.71264113896775,
126.844196514862));
#40566=CARTESIAN_POINT('Ctrl Pts',(-1.04419673789595,6.68595110456003,126.852339626142));
#40567=CARTESIAN_POINT('Ctrl Pts',(-1.21492993257824,6.6592863799532,126.860475015419));
#40568=CARTESIAN_POINT('Ctrl Pts',(-1.38482287589788,6.62604919712483,126.868610404697));
#40569=CARTESIAN_POINT('Ctrl Pts',(-1.55332819486716,6.58630856542804,126.876745793974));
#40570=CARTESIAN_POINT('Ctrl Pts',(-1.72170912953962,6.54659726877278,126.884875178013));
#40571=CARTESIAN_POINT('Ctrl Pts',(-1.88870412510679,6.50039216564878,126.893004562051));
#40572=CARTESIAN_POINT('Ctrl Pts',(-2.05377405370416,6.4478136710308,126.90113394609));
#40573=CARTESIAN_POINT('Ctrl Pts',(-2.21875680646001,6.39526294388417,126.909259036882));
#40574=CARTESIAN_POINT('Ctrl Pts',(-2.3818161694176,6.336345639237,126.917384127674));
#40575=CARTESIAN_POINT('Ctrl Pts',(-2.54242628502315,6.27123254115357,126.925509218466));
#40576=CARTESIAN_POINT('Ctrl Pts',(-2.70364948425946,6.20587089225854,126.933665324491));
#40577=CARTESIAN_POINT('Ctrl Pts',(-2.86240434015847,6.13426614824959,126.941821430516));
#40578=CARTESIAN_POINT('Ctrl Pts',(-3.01817687839044,6.05664076289401,126.949977536541));
#40579=CARTESIAN_POINT('Ctrl Pts',(-3.17332246032779,5.97932780567579,126.958100815715));
#40580=CARTESIAN_POINT('Ctrl Pts',(-3.32550936654906,5.89604276468142,126.966224094888));
#40581=CARTESIAN_POINT('Ctrl Pts',(-3.47425259993951,5.80705242544043,126.974347374062));
#40582=CARTESIAN_POINT('Ctrl Pts',(-3.62301563974854,5.71805023638369,126.982471734918));
#40583=CARTESIAN_POINT('Ctrl Pts',(-3.76833377940971,5.62334142371958,126.990596095775));
#40584=CARTESIAN_POINT('Ctrl Pts',(-3.9097493944689,5.52323715518808,126.998720456632));
#40585=CARTESIAN_POINT('Ctrl Pts',(-4.05121074525977,5.42310051157576,127.006847445017));
#40586=CARTESIAN_POINT('Ctrl Pts',(-4.18876675971709,5.31756514857308,127.014974433403));
#40587=CARTESIAN_POINT('Ctrl Pts',(-4.32199143758641,5.20698367708502,127.023101421788));
#40588=CARTESIAN_POINT('Ctrl Pts',(-4.45607739783106,5.09568730897304,127.031280950228));
#40589=CARTESIAN_POINT('Ctrl Pts',(-4.58577553494708,4.97927960117355,127.039460478668));
#40590=CARTESIAN_POINT('Ctrl Pts',(-4.71068850989165,4.85815837152051,127.047640007108));
#40591=CARTESIAN_POINT('Ctrl Pts',(-4.83501322936692,4.73760754078578,127.055781015512));
#40592=CARTESIAN_POINT('Ctrl Pts',(-4.95459755359684,4.61238779628413,127.063922023916));
#40593=CARTESIAN_POINT('Ctrl Pts',(-5.06908987945627,4.48292502658633,127.072063032319));
#40594=CARTESIAN_POINT('Ctrl Pts',(-5.18439480401483,4.35254340684812,127.080261820778));
#40595=CARTESIAN_POINT('Ctrl Pts',(-5.2945349455551,4.21785860381408,127.088460609236));
#40596=CARTESIAN_POINT('Ctrl Pts',(-5.39919544763404,4.07933542605261,127.096659397694));
#40597=CARTESIAN_POINT('Ctrl Pts',(-5.50385594971299,3.94081224829114,127.104858186152));
#40598=CARTESIAN_POINT('Ctrl Pts',(-5.60303665319985,3.79845103754411,127.113056974611));
#40599=CARTESIAN_POINT('Ctrl Pts',(-5.69646982105714,3.65274151532589,127.121255763069));
#40600=CARTESIAN_POINT('Ctrl Pts',(-5.79352559600295,3.50138251808548,127.129772436384));
#40601=CARTESIAN_POINT('Ctrl Pts',(-5.88466267022944,3.34596973003752,127.138289109699));
#40602=CARTESIAN_POINT('Ctrl Pts',(-5.96953903341556,3.18698803394805,127.146805783014));
#40603=CARTESIAN_POINT('Ctrl Pts',(-6.05429517479537,3.02823152501265,127.15531039302));
#40604=CARTESIAN_POINT('Ctrl Pts',(-6.1328081275134,2.86591646572114,127.163815003025));
#40605=CARTESIAN_POINT('Ctrl Pts',(-6.20477906986329,2.70055655267325,127.172319613031));
#40606=CARTESIAN_POINT('Ctrl Pts',(-6.27665674318821,2.53541093385795,127.18081320169));
#40607=CARTESIAN_POINT('Ctrl Pts',(-6.34200917572603,2.36722862078917,127.189306790349));
#40608=CARTESIAN_POINT('Ctrl Pts',(-6.40058318452126,2.19654817794276,127.197800379008));
#40609=CARTESIAN_POINT('Ctrl Pts',(-6.46093687318422,2.02068187614292,127.206552032106));
#40610=CARTESIAN_POINT('Ctrl Pts',(-6.51409354487708,1.84216352814561,127.215303685205));
#40611=CARTESIAN_POINT('Ctrl Pts',(-6.55982847582034,1.66160746502193,127.224055338303));
#40612=CARTESIAN_POINT('Ctrl Pts',(-6.60410049396021,1.48682680750238,127.232527054271));
#40613=CARTESIAN_POINT('Ctrl Pts',(-6.64141811180504,1.31013712320766,127.240998770238));
#40614=CARTESIAN_POINT('Ctrl Pts',(-6.67162700840373,1.13211397868671,127.249470486205));
#40615=CARTESIAN_POINT('Ctrl Pts',(-6.70333322713052,0.945267009941253,
127.258362107869));
#40616=CARTESIAN_POINT('Ctrl Pts',(-6.72720797912353,0.756951360983467,
127.267253729533));
#40617=CARTESIAN_POINT('Ctrl Pts',(-6.74313260258851,0.567848310649833,
127.276145351197));
#40618=CARTESIAN_POINT('Ctrl Pts',(-6.75905722605351,0.37874526031607,127.285036972862));
#40619=CARTESIAN_POINT('Ctrl Pts',(-6.76703163872077,0.188855216149285,
127.293928594526));
#40620=CARTESIAN_POINT('Ctrl Pts',(-6.76699990560463,-0.00113028621264427,
127.30282021619));
#40621=CARTESIAN_POINT('Ctrl Pts',(-6.76699990560448,-0.00113028709141402,
127.302820216231));
#40622=CARTESIAN_POINT('Ctrl Pts',(-6.76696867316269,-0.188118117230485,
127.311571542099));
#40623=CARTESIAN_POINT('Ctrl Pts',(-6.75918283403797,-0.374911890116693,
127.320322867967));
#40624=CARTESIAN_POINT('Ctrl Pts',(-6.74371597829373,-0.560877708690457,
127.329074193836));
#40625=CARTESIAN_POINT('Ctrl Pts',(-6.72751731262625,-0.755642447592097,
127.338239586222));
#40626=CARTESIAN_POINT('Ctrl Pts',(-6.70289324644896,-0.949498613544085,
127.347404978609));
#40627=CARTESIAN_POINT('Ctrl Pts',(-6.66998776417228,-1.14173211647567,
127.356570370996));
#40628=CARTESIAN_POINT('Ctrl Pts',(-6.63842328888005,-1.32613146982976,
127.365362243399));
#40629=CARTESIAN_POINT('Ctrl Pts',(-6.59923911678114,-1.50903756531875,
127.374154115802));
#40630=CARTESIAN_POINT('Ctrl Pts',(-6.55261329048496,-1.68983669783796,
127.382945988205));
#40631=CARTESIAN_POINT('Ctrl Pts',(-6.50591798061802,-1.87090526406621,
127.391750962589));
#40632=CARTESIAN_POINT('Ctrl Pts',(-6.45175894277092,-2.04986033104845,
127.400555936973));
#40633=CARTESIAN_POINT('Ctrl Pts',(-6.39036327152211,-2.22610562597134,
127.409360911357));
#40634=CARTESIAN_POINT('Ctrl Pts',(-6.32883926742469,-2.40271931919156,
127.418184290417));
#40635=CARTESIAN_POINT('Ctrl Pts',(-6.26004848239057,-2.57661165666901,
127.427007669477));
#40636=CARTESIAN_POINT('Ctrl Pts',(-6.18426591542891,-2.74720659712084,
127.435831048537));
#40637=CARTESIAN_POINT('Ctrl Pts',(-6.17502474468359,-2.76800949462363,
127.43690699985));
#40638=CARTESIAN_POINT('Ctrl Pts',(-6.1656796601793,-2.78876339116494,127.437982951164));
#40639=CARTESIAN_POINT('Ctrl Pts',(-6.15623120611983,-2.80946726921607,
127.439058902477));
#40640=CARTESIAN_POINT('Ctrl Pts',(-6.08030675100585,-2.97583635455899,
127.447704868968));
#40641=CARTESIAN_POINT('Ctrl Pts',(-5.99756667944973,-3.13927409780236,
127.456350835459));
#40642=CARTESIAN_POINT('Ctrl Pts',(-5.90825281290134,-3.29921774044143,
127.464996801949));
#40643=CARTESIAN_POINT('Ctrl Pts',(-5.81905319093026,-3.45895679341762,
127.473631709074));
#40644=CARTESIAN_POINT('Ctrl Pts',(-5.72329668953091,-3.6152103931188,127.482266616198));
#40645=CARTESIAN_POINT('Ctrl Pts',(-5.62127221236195,-3.76743781826952,
127.490901523322));
#40646=CARTESIAN_POINT('Ctrl Pts',(-5.5158606048961,-3.92471907107075,127.499823102394));
#40647=CARTESIAN_POINT('Ctrl Pts',(-5.40375779265452,-4.07770191994871,
127.508744681466));
#40648=CARTESIAN_POINT('Ctrl Pts',(-5.28533431097518,-4.22581710693074,
127.517666260537));
#40649=CARTESIAN_POINT('Ctrl Pts',(-5.17103261878915,-4.36877706951941,
127.526277319513));
#40650=CARTESIAN_POINT('Ctrl Pts',(-5.05084301385447,-4.50720220746502,
127.534888378489));
#40651=CARTESIAN_POINT('Ctrl Pts',(-4.92514314577255,-4.64060922656172,
127.543499437464));
#40652=CARTESIAN_POINT('Ctrl Pts',(-4.79956181846957,-4.77389043668023,
127.552102375814));
#40653=CARTESIAN_POINT('Ctrl Pts',(-4.66848079678642,-4.90216274172892,
127.560705314163));
#40654=CARTESIAN_POINT('Ctrl Pts',(-4.53231775020979,-5.02497610055344,
127.569308252513));
#40655=CARTESIAN_POINT('Ctrl Pts',(-4.39630717474531,-5.14765193682778,
127.577901557562));
#40656=CARTESIAN_POINT('Ctrl Pts',(-4.2552261531301,-5.26488081784157,127.58649486261));
#40657=CARTESIAN_POINT('Ctrl Pts',(-4.10952908426155,-5.37624959480198,
127.595088167659));
#40658=CARTESIAN_POINT('Ctrl Pts',(-4.09329604597001,-5.3886578994777,127.5960456025));
#40659=CARTESIAN_POINT('Ctrl Pts',(-4.0770057429822,-5.40099349734913,127.59700303734));
#40660=CARTESIAN_POINT('Ctrl Pts',(-4.06065883134004,-5.41325584611149,
127.597960472181));
#40661=CARTESIAN_POINT('Ctrl Pts',(-3.91389783709851,-5.52334602922951,
127.606556229728));
#40662=CARTESIAN_POINT('Ctrl Pts',(-3.76274333118558,-5.62739979781851,
127.615151987276));
#40663=CARTESIAN_POINT('Ctrl Pts',(-3.60771671144361,-5.72509118966419,
127.623747744824));
#40664=CARTESIAN_POINT('Ctrl Pts',(-3.45254544659429,-5.82287373090011,
127.632351522505));
#40665=CARTESIAN_POINT('Ctrl Pts',(-3.29349511490486,-5.91428188352603,
127.640955300187));
#40666=CARTESIAN_POINT('Ctrl Pts',(-3.13111243014787,-5.99903525158617,
127.649559077868));
#40667=CARTESIAN_POINT('Ctrl Pts',(-2.96234796388609,-6.08711950112276,
127.658500991536));
#40668=CARTESIAN_POINT('Ctrl Pts',(-2.78998425885458,-6.16801514780056,
127.667442905204));
#40669=CARTESIAN_POINT('Ctrl Pts',(-2.61465742661348,-6.24146261235738,
127.676384818872));
#40670=CARTESIAN_POINT('Ctrl Pts',(-2.44550123567848,-6.31232508776661,
127.685012021203));
#40671=CARTESIAN_POINT('Ctrl Pts',(-2.27358723276122,-6.37625466673425,
127.693639223534));
#40672=CARTESIAN_POINT('Ctrl Pts',(-2.0995022295599,-6.43306920435907,127.702266425864));
#40673=CARTESIAN_POINT('Ctrl Pts',(-1.92525143703901,-6.48993784913477,
127.710901844285));
#40674=CARTESIAN_POINT('Ctrl Pts',(-1.74882580973115,-6.53967784143297,
127.719537262705));
#40675=CARTESIAN_POINT('Ctrl Pts',(-1.57082454858861,-6.58215764301885,
127.728172681126));
#40676=CARTESIAN_POINT('Ctrl Pts',(-1.39256031593683,-6.62470020246084,
127.736820857147));
#40677=CARTESIAN_POINT('Ctrl Pts',(-1.21271609613202,-6.65996107432725,
127.745469033168));
#40678=CARTESIAN_POINT('Ctrl Pts',(-1.03189991720437,-6.68786001355244,
127.754117209189));
#40679=CARTESIAN_POINT('Ctrl Pts',(-1.01277025107528,-6.69081161553794,
127.755032153421));
#40680=CARTESIAN_POINT('Ctrl Pts',(-0.993629709127076,-6.69368086457255,
127.755947097652));
#40681=CARTESIAN_POINT('Ctrl Pts',(-0.97447901319423,-6.69646769967899,
127.756862041884));
#40682=CARTESIAN_POINT('Ctrl Pts',(-0.802300779324919,-6.72152330854014,
127.765088034425));
#40683=CARTESIAN_POINT('Ctrl Pts',(-0.628929604938511,-6.73996702089787,
127.773314026967));
#40684=CARTESIAN_POINT('Ctrl Pts',(-0.454914030333935,-6.75169180465203,
127.781540019508));
#40685=CARTESIAN_POINT('Ctrl Pts',(-0.28108088856713,-6.76340429648589,
127.789757388159));
#40686=CARTESIAN_POINT('Ctrl Pts',(-0.106605046435611,-6.76841186289632,
127.797974756811));
#40687=CARTESIAN_POINT('Ctrl Pts',(0.0679564280944051,-6.7666587710539,
127.806192125462));
#40688=CARTESIAN_POINT('Ctrl Pts',(0.242369826476127,-6.7649071663156,127.814402523525));
#40689=CARTESIAN_POINT('Ctrl Pts',(0.416868356325892,-6.7564063287222,127.822612921587));
#40690=CARTESIAN_POINT('Ctrl Pts',(0.590891413560338,-6.74115244875687,
127.830823319649));
#40691=CARTESIAN_POINT('Ctrl Pts',(0.764801662826502,-6.72590845690196,
127.839028395438));
#40692=CARTESIAN_POINT('Ctrl Pts',(0.938236697782867,-6.70392017363867,
127.847233471227));
#40693=CARTESIAN_POINT('Ctrl Pts',(1.11063740751498,-6.67523584220276,127.855438547016));
#40694=CARTESIAN_POINT('Ctrl Pts',(1.28296084085476,-6.64656436814809,127.863639944985));
#40695=CARTESIAN_POINT('Ctrl Pts',(1.45425051995198,-6.61120288430478,127.871841342955));
#40696=CARTESIAN_POINT('Ctrl Pts',(1.62395384490536,-6.56925132032693,127.880042740924));
#40697=CARTESIAN_POINT('Ctrl Pts',(1.79364387728128,-6.52730304234488,127.888243496492));
#40698=CARTESIAN_POINT('Ctrl Pts',(1.96174745338401,-6.47876578986581,127.89644425206));
#40699=CARTESIAN_POINT('Ctrl Pts',(2.12772316693707,-6.4237904016927,127.904645007627));
#40700=CARTESIAN_POINT('Ctrl Pts',(2.29369803741249,-6.3688152927684,127.912845721539));
#40701=CARTESIAN_POINT('Ctrl Pts',(2.45754472633466,-6.30740222495959,127.921046435451));
#40702=CARTESIAN_POINT('Ctrl Pts',(2.61873808867114,-6.23975158343207,127.929247149363));
#40703=CARTESIAN_POINT('Ctrl Pts',(2.77995984447301,-6.17208902555688,127.937449307792));
#40704=CARTESIAN_POINT('Ctrl Pts',(2.93852701207702,-6.09818684363949,127.945651466222));
#40705=CARTESIAN_POINT('Ctrl Pts',(3.09393543899492,-6.01829315498434,127.953853624651));
#40706=CARTESIAN_POINT('Ctrl Pts',(3.24939940456278,-5.93837091454666,127.962058714304));
#40707=CARTESIAN_POINT('Ctrl Pts',(3.40170206219766,-5.85245306572805,127.970263803957));
#40708=CARTESIAN_POINT('Ctrl Pts',(3.55036477854347,-5.76083318099717,127.97846889361));
#40709=CARTESIAN_POINT('Ctrl Pts',(3.6991973244663,-5.66910863138022,127.986683356608));
#40710=CARTESIAN_POINT('Ctrl Pts',(3.8443813163463,-5.57166922043436,127.994897819606));
#40711=CARTESIAN_POINT('Ctrl Pts',(3.98546711301411,-5.46885188052145,128.003112282604));
#40712=CARTESIAN_POINT('Ctrl Pts',(4.12663649855741,-5.3659736245842,128.011331612411));
#40713=CARTESIAN_POINT('Ctrl Pts',(4.26370256809365,-5.2577113100097,128.019550942219));
#40714=CARTESIAN_POINT('Ctrl Pts',(4.39624969900895,-5.14444142584632,128.027770272026));
#40715=CARTESIAN_POINT('Ctrl Pts',(4.5290022036674,-5.03099603686487,128.036002337187));
#40716=CARTESIAN_POINT('Ctrl Pts',(4.65722151430005,-4.91252781596581,128.044234402348));
#40717=CARTESIAN_POINT('Ctrl Pts',(4.78052878804062,-4.78945023011148,128.052466467508));
#40718=CARTESIAN_POINT('Ctrl Pts',(4.89136621962794,-4.67881925848881,128.059866038769));
#40719=CARTESIAN_POINT('Ctrl Pts',(4.99823527393971,-4.56446466434207,128.067265610031));
#40720=CARTESIAN_POINT('Ctrl Pts',(5.10088968969296,-4.44670815025948,128.074665181292));
#40721=CARTESIAN_POINT('Ctrl Pts',(5.21403054453363,-4.31692247500527,128.082820639699));
#40722=CARTESIAN_POINT('Ctrl Pts',(5.32239936044838,-4.18260420149505,128.090976098106));
#40723=CARTESIAN_POINT('Ctrl Pts',(5.42560704560762,-4.04414109381127,128.099131556512));
#40724=CARTESIAN_POINT('Ctrl Pts',(5.52868911344757,-3.90584651393023,128.107277088654));
#40725=CARTESIAN_POINT('Ctrl Pts',(5.6266223386572,-3.76341743162741,128.115422620796));
#40726=CARTESIAN_POINT('Ctrl Pts',(5.7190551960092,-3.61727752114767,128.123568152938));
#40727=CARTESIAN_POINT('Ctrl Pts',(5.81139498719925,-3.47128475185737,128.131705483739));
#40728=CARTESIAN_POINT('Ctrl Pts',(5.89824524189807,-3.3215888991978,128.139842814539));
#40729=CARTESIAN_POINT('Ctrl Pts',(5.97929539458907,-3.16864570191209,128.14798014534));
#40730=CARTESIAN_POINT('Ctrl Pts',(6.06028097475199,-3.01582435422904,128.156110993142));
#40731=CARTESIAN_POINT('Ctrl Pts',(6.13547548340759,-2.85976113471935,128.164241840944));
#40732=CARTESIAN_POINT('Ctrl Pts',(6.20461230495252,-2.70093967819198,128.172372688746));
#40733=CARTESIAN_POINT('Ctrl Pts',(6.27370856868759,-2.54221139127081,128.18049876674));
#40734=CARTESIAN_POINT('Ctrl Pts',(6.3367540767727,-2.3807284239678,128.188624844733));
#40735=CARTESIAN_POINT('Ctrl Pts',(6.39352872013706,-2.21699785854262,128.196750922727));
#40736=CARTESIAN_POINT('Ctrl Pts',(6.45050467601728,-2.05268673443676,128.204905814309));
#40737=CARTESIAN_POINT('Ctrl Pts',(6.50116504619806,-1.88611237523665,128.213060705892));
#40738=CARTESIAN_POINT('Ctrl Pts',(6.54533639651662,-1.71780687402132,128.221215597474));
#40739=CARTESIAN_POINT('Ctrl Pts',(6.58933549401299,-1.55015770541441,128.22933868783));
#40740=CARTESIAN_POINT('Ctrl Pts',(6.62689601368207,-1.38079123286572,128.237461778186));
#40741=CARTESIAN_POINT('Ctrl Pts',(6.65789680929449,-1.210247527073,128.245584868543));
#40742=CARTESIAN_POINT('Ctrl Pts',(6.68890003923093,-1.03969042940975,128.253708596761));
#40743=CARTESIAN_POINT('Ctrl Pts',(6.71334245362125,-0.867956274295264,
128.26183232498));
#40744=CARTESIAN_POINT('Ctrl Pts',(6.7311542771293,-0.69559406084577,128.269956053198));
#40745=CARTESIAN_POINT('Ctrl Pts',(6.74897088798132,-0.523185521021988,
128.278081964858));
#40746=CARTESIAN_POINT('Ctrl Pts',(6.76015332181594,-0.350148950475839,
128.286207876519));
#40747=CARTESIAN_POINT('Ctrl Pts',(6.76468379518772,-0.177037146171877,
128.294333788179));
#40748=CARTESIAN_POINT('Ctrl Pts',(6.76924324140766,-0.00281827388451997,
128.302511665889));
#40749=CARTESIAN_POINT('Ctrl Pts',(6.76706534206994,0.171476422285105,128.310689543599));
#40750=CARTESIAN_POINT('Ctrl Pts',(6.75818517174349,0.34528565627094,128.318867421309));
#40751=CARTESIAN_POINT('Ctrl Pts',(6.74934738454401,0.518265336480143,128.327006267783));
#40752=CARTESIAN_POINT('Ctrl Pts',(6.73387125710201,0.690763819472348,128.335145114256));
#40753=CARTESIAN_POINT('Ctrl Pts',(6.71184318948325,0.86223546655618,128.34328396073));
#40754=CARTESIAN_POINT('Ctrl Pts',(6.68965666279002,1.03494059625703,128.351481354058));
#40755=CARTESIAN_POINT('Ctrl Pts',(6.66082364023708,1.20660368870575,128.359678747386));
#40756=CARTESIAN_POINT('Ctrl Pts',(6.6254841039516,1.37668056871761,128.367876140715));
#40757=CARTESIAN_POINT('Ctrl Pts',(6.59014456766612,1.54675744872948,128.376073534043));
#40758=CARTESIAN_POINT('Ctrl Pts',(6.54829866667873,1.71524776977647,128.384270927372));
#40759=CARTESIAN_POINT('Ctrl Pts',(6.50013633950522,1.88162604357074,128.3924683207));
#40760=CARTESIAN_POINT('Ctrl Pts',(6.45179842136804,2.04861090187087,128.400695600213));
#40761=CARTESIAN_POINT('Ctrl Pts',(6.39695416720556,2.21396535831026,128.408922879726));
#40762=CARTESIAN_POINT('Ctrl Pts',(6.3357294915854,2.37714551709715,128.417150159238));
#40763=CARTESIAN_POINT('Ctrl Pts',(6.27457521065064,2.54013805519308,128.42536797922));
#40764=CARTESIAN_POINT('Ctrl Pts',(6.20705524254268,2.70096094122537,128.433585799201));
#40765=CARTESIAN_POINT('Ctrl Pts',(6.13334583212878,2.85908340268496,128.441803619182));
#40766=CARTESIAN_POINT('Ctrl Pts',(6.05970637539851,3.01705579852086,128.450013640067));
#40767=CARTESIAN_POINT('Ctrl Pts',(5.97988932671191,3.17233255114162,128.458223660952));
#40768=CARTESIAN_POINT('Ctrl Pts',(5.89411979160669,3.32440083055434,128.466433681837));
#40769=CARTESIAN_POINT('Ctrl Pts',(5.8084230412695,3.47634006351216,128.474636735628));
#40770=CARTESIAN_POINT('Ctrl Pts',(5.71678404734098,3.62507593853215,128.482839789418));
#40771=CARTESIAN_POINT('Ctrl Pts',(5.61947475416967,3.77011836515111,128.491042843209));
#40772=CARTESIAN_POINT('Ctrl Pts',(5.52221150991263,3.91509215447913,128.499242015132));
#40773=CARTESIAN_POINT('Ctrl Pts',(5.41928350913567,4.0563756788621,128.507441187056));
#40774=CARTESIAN_POINT('Ctrl Pts',(5.31100728740936,4.19350576404572,128.51564035898));
#40775=CARTESIAN_POINT('Ctrl Pts',(5.2027626251986,4.33059587961286,128.523837141072));
#40776=CARTESIAN_POINT('Ctrl Pts',(5.08917306910854,4.46353468625805,128.532033923165));
#40777=CARTESIAN_POINT('Ctrl Pts',(4.97059693649293,4.5918901440395,128.540230705257));
#40778=CARTESIAN_POINT('Ctrl Pts',(4.85203381518062,4.72023151743691,128.54842658792));
#40779=CARTESIAN_POINT('Ctrl Pts',(4.72848545144471,4.84399028133397,128.556622470584));
#40780=CARTESIAN_POINT('Ctrl Pts',(4.60034872764433,4.96276944699844,128.564818353247));
#40781=CARTESIAN_POINT('Ctrl Pts',(4.47216607729763,5.08159118528918,128.573017173465));
#40782=CARTESIAN_POINT('Ctrl Pts',(4.33939204282602,5.19542951388512,128.581215993682));
#40783=CARTESIAN_POINT('Ctrl Pts',(4.20245885588674,5.303925769143,128.5894148139));
#40784=CARTESIAN_POINT('Ctrl Pts',(4.06549886044986,5.41244326557449,128.597615239266));
#40785=CARTESIAN_POINT('Ctrl Pts',(3.92437837564445,5.51561638776814,128.605815664632));
#40786=CARTESIAN_POINT('Ctrl Pts',(3.77956062976668,5.61312840098262,128.614016089998));
#40787=CARTESIAN_POINT('Ctrl Pts',(3.63463457808358,5.71071334115129,128.62222264827));
#40788=CARTESIAN_POINT('Ctrl Pts',(3.48600604426765,5.80262852217369,128.630429206542));
#40789=CARTESIAN_POINT('Ctrl Pts',(3.33416555725262,5.88860161981012,128.638635764814));
#40790=CARTESIAN_POINT('Ctrl Pts',(3.25664982541948,5.9324915447719,128.64282527568));
#40791=CARTESIAN_POINT('Ctrl Pts',(3.17829739323455,5.97483359695155,128.647014786547));
#40792=CARTESIAN_POINT('Ctrl Pts',(3.09917575053256,6.01559628526641,128.651204297413));
#40793=CARTESIAN_POINT('Origin',(0.,0.,-3.69717978381041));
#40794=CARTESIAN_POINT('',(3.09917575053245,6.01559628526646,131.045629062141));
#40795=CARTESIAN_POINT('',(3.09917575053269,6.01559628526634,130.651392015122));
#40796=CARTESIAN_POINT('',(3.09917575053259,6.01559628526639,-3.69717978381041));
#40797=CARTESIAN_POINT('',(-6.767,7.73790753694215E-12,129.69717978381));
#40798=CARTESIAN_POINT('Ctrl Pts',(-6.76699924398711,-0.0031987306766745,
129.69717978381));
#40799=CARTESIAN_POINT('Ctrl Pts',(-6.76690738963476,-0.19751903948158,
129.70629472893));
#40800=CARTESIAN_POINT('Ctrl Pts',(-6.75844129896495,-0.391590285911398,
129.71540967405));
#40801=CARTESIAN_POINT('Ctrl Pts',(-6.74168986956949,-0.584727887606004,
129.72452461917));
#40802=CARTESIAN_POINT('Ctrl Pts',(-6.72486379031202,-0.778726173781559,
129.733680183475));
#40803=CARTESIAN_POINT('Ctrl Pts',(-6.6996784308952,-0.971782271623306,
129.742835747779));
#40804=CARTESIAN_POINT('Ctrl Pts',(-6.66627455968819,-1.16321644368282,
129.751991312083));
#40805=CARTESIAN_POINT('Ctrl Pts',(-6.63279655757565,-1.35507545238578,
129.761167194699));
#40806=CARTESIAN_POINT('Ctrl Pts',(-6.5910636168629,-1.54530513563145,129.770343077315));
#40807=CARTESIAN_POINT('Ctrl Pts',(-6.5412670110954,-1.73323826681593,129.779518959932));
#40808=CARTESIAN_POINT('Ctrl Pts',(-6.49133564545543,-1.92167998376446,
129.788719674376));
#40809=CARTESIAN_POINT('Ctrl Pts',(-6.43329700355376,-2.10781251261126,
129.797920388821));
#40810=CARTESIAN_POINT('Ctrl Pts',(-6.36739232471245,-2.2909831913816,129.807121103265));
#40811=CARTESIAN_POINT('Ctrl Pts',(-6.34999085318926,-2.33934757774299,
129.809550459924));
#40812=CARTESIAN_POINT('Ctrl Pts',(-6.33204124098797,-2.38750558883375,
129.811979816583));
#40813=CARTESIAN_POINT('Ctrl Pts',(-6.31354847724027,-2.43544546757612,
129.814409173242));
#40814=CARTESIAN_POINT('Ctrl Pts',(-6.25094052106384,-2.59774775339746,
129.822633852761));
#40815=CARTESIAN_POINT('Ctrl Pts',(-6.18198758564383,-2.75784818275406,
129.83085853228));
#40816=CARTESIAN_POINT('Ctrl Pts',(-6.10686520993706,-2.91521633976974,
129.839083211799));
#40817=CARTESIAN_POINT('Ctrl Pts',(-6.03182179634599,-3.0724190850488,129.847299246249));
#40818=CARTESIAN_POINT('Ctrl Pts',(-5.95062200909514,-3.22689495622112,
129.855515280699));
#40819=CARTESIAN_POINT('Ctrl Pts',(-5.86349028128006,-3.37813124690772,
129.863731315149));
#40820=CARTESIAN_POINT('Ctrl Pts',(-5.77643268612984,-3.5292388640384,129.871940359304));
#40821=CARTESIAN_POINT('Ctrl Pts',(-5.68345337995602,-3.67711208130814,
129.880149403458));
#40822=CARTESIAN_POINT('Ctrl Pts',(-5.58482378685168,-3.82126056031457,
129.888358447613));
#40823=CARTESIAN_POINT('Ctrl Pts',(-5.48625835882553,-3.96531526119484,
129.896562151241));
#40824=CARTESIAN_POINT('Ctrl Pts',(-5.38205016757828,-4.10564975584145,
129.904765854869));
#40825=CARTESIAN_POINT('Ctrl Pts',(-5.27251527509775,-4.24180052263905,
129.912969558497));
#40826=CARTESIAN_POINT('Ctrl Pts',(-5.16302971293989,-4.37788997234302,
129.921169567491));
#40827=CARTESIAN_POINT('Ctrl Pts',(-5.04822245310552,-4.50979916934204,
129.929369576485));
#40828=CARTESIAN_POINT('Ctrl Pts',(-4.92845141551991,-4.63709560445542,
129.937569585479));
#40829=CARTESIAN_POINT('Ctrl Pts',(-4.80868995507916,-4.76438186067728,
129.945768938783));
#40830=CARTESIAN_POINT('Ctrl Pts',(-4.68396574653091,-4.88705582287398,
129.953968292087));
#40831=CARTESIAN_POINT('Ctrl Pts',(-4.55467559393565,-5.0047196958478,129.962167645391));
#40832=CARTESIAN_POINT('Ctrl Pts',(-4.42538628427397,-5.12238280168796,
129.970366945237));
#40833=CARTESIAN_POINT('Ctrl Pts',(-4.29153135427883,-5.2350356412576,129.978566245084));
#40834=CARTESIAN_POINT('Ctrl Pts',(-4.15354281875892,-5.34231888347525,
129.98676554493));
#40835=CARTESIAN_POINT('Ctrl Pts',(-4.01553015040907,-5.44962088847076,
129.994966278753));
#40836=CARTESIAN_POINT('Ctrl Pts',(-3.87338271926515,-5.55155120507676,
130.003167012576));
#40837=CARTESIAN_POINT('Ctrl Pts',(-3.72756384859864,-5.64779220179182,
130.011367746399));
#40838=CARTESIAN_POINT('Ctrl Pts',(-3.58169302239312,-5.74406748935576,
130.019571402159));
#40839=CARTESIAN_POINT('Ctrl Pts',(-3.43214844981436,-5.83464922154886,
130.027775057919));
#40840=CARTESIAN_POINT('Ctrl Pts',(-3.27942055711838,-5.91926429630823,
130.035978713679));
#40841=CARTESIAN_POINT('Ctrl Pts',(-3.12651770480307,-6.00397630307529,
130.044191767254));
#40842=CARTESIAN_POINT('Ctrl Pts',(-2.97042456076769,-6.08270782284415,
130.052404820829));
#40843=CARTESIAN_POINT('Ctrl Pts',(-2.81165512958056,-6.15523228093818,
130.060617874404));
#40844=CARTESIAN_POINT('Ctrl Pts',(-2.65279175095887,-6.2277996533812,130.068835787827));
#40845=CARTESIAN_POINT('Ctrl Pts',(-2.49124925952316,-6.29415250678049,
130.07705370125));
#40846=CARTESIAN_POINT('Ctrl Pts',(-2.32755945122351,-6.35411331351748,
130.085271614674));
#40847=CARTESIAN_POINT('Ctrl Pts',(-2.1636143420384,-6.41416763888714,130.09350234527));
#40848=CARTESIAN_POINT('Ctrl Pts',(-1.99751556403329,-6.46780988428938,
130.101733075865));
#40849=CARTESIAN_POINT('Ctrl Pts',(-1.82980911846274,-6.51491270777979,
130.109963806461));
#40850=CARTESIAN_POINT('Ctrl Pts',(-1.67579080551377,-6.5581710177657,130.117522748137));
#40851=CARTESIAN_POINT('Ctrl Pts',(-1.52041688788452,-6.59591438128047,
130.125081689813));
#40852=CARTESIAN_POINT('Ctrl Pts',(-1.36411511610003,-6.6280825998193,130.132640631489));
#40853=CARTESIAN_POINT('Ctrl Pts',(-1.19551111738506,-6.66278272007554,
130.140794523656));
#40854=CARTESIAN_POINT('Ctrl Pts',(-1.02530602535819,-6.69110210282341,
130.148948415823));
#40855=CARTESIAN_POINT('Ctrl Pts',(-0.854028533119562,-6.71289239185447,
130.157102307989));
#40856=CARTESIAN_POINT('Ctrl Pts',(-0.682960047273748,-6.73465609064505,
130.165246250129));
#40857=CARTESIAN_POINT('Ctrl Pts',(-0.510822124793817,-6.74990650923921,
130.17339019227));
#40858=CARTESIAN_POINT('Ctrl Pts',(-0.338156286058496,-6.75854565170637,
130.18153413441));
#40859=CARTESIAN_POINT('Ctrl Pts',(-0.16566480517129,-6.76717607037327,
130.189669852803));
#40860=CARTESIAN_POINT('Ctrl Pts',(0.00735316824682647,-6.76920848550534,
130.197805571196));
#40861=CARTESIAN_POINT('Ctrl Pts',(0.180348304968705,-6.76459632859899,
130.205941289589));
#40862=CARTESIAN_POINT('Ctrl Pts',(0.353205140885511,-6.75998785887729,
130.214070503889));
#40863=CARTESIAN_POINT('Ctrl Pts',(0.526038812645128,-6.74874540355847,
130.222199718189));
#40864=CARTESIAN_POINT('Ctrl Pts',(0.698297283945808,-6.73087437880354,
130.230328932489));
#40865=CARTESIAN_POINT('Ctrl Pts',(0.870454262849295,-6.71301388341839,
130.238453357165));
#40866=CARTESIAN_POINT('Ctrl Pts',(1.04203635341537,-6.68853263380989,130.24657778184));
#40867=CARTESIAN_POINT('Ctrl Pts',(1.21249394515143,-6.65748807231159,130.254702206516));
#40868=CARTESIAN_POINT('Ctrl Pts',(1.3839863235906,-6.62625505045131,130.26287595165));
#40869=CARTESIAN_POINT('Ctrl Pts',(1.55434013045905,-6.58837877894014,130.271049696784));
#40870=CARTESIAN_POINT('Ctrl Pts',(1.72300276572845,-6.54397054312534,130.279223441918));
#40871=CARTESIAN_POINT('Ctrl Pts',(1.89058533483587,-6.4998466846579,130.28734484478));
#40872=CARTESIAN_POINT('Ctrl Pts',(2.05649797640161,-6.44927439147436,130.295466247642));
#40873=CARTESIAN_POINT('Ctrl Pts',(2.22021101105309,-6.39241363386309,130.303587650505));
#40874=CARTESIAN_POINT('Ctrl Pts',(2.38393670313444,-6.3355484800774,130.311709681271));
#40875=CARTESIAN_POINT('Ctrl Pts',(2.54546210380607,-6.27239401345154,130.319831712037));
#40876=CARTESIAN_POINT('Ctrl Pts',(2.70427501342557,-6.20315932825864,130.327953742803));
#40877=CARTESIAN_POINT('Ctrl Pts',(2.86313044326826,-6.13390610632162,130.336077948144));
#40878=CARTESIAN_POINT('Ctrl Pts',(3.0192716006406,-6.05856957056588,130.344202153486));
#40879=CARTESIAN_POINT('Ctrl Pts',(3.17220854073453,-5.97740595694244,130.352326358827));
#40880=CARTESIAN_POINT('Ctrl Pts',(3.32680091738079,-5.89536380336239,130.360538503069));
#40881=CARTESIAN_POINT('Ctrl Pts',(3.47811896533468,-5.80736786586981,130.368750647312));
#40882=CARTESIAN_POINT('Ctrl Pts',(3.62568515748499,-5.71372874214317,130.376962791554));
#40883=CARTESIAN_POINT('Ctrl Pts',(3.77190423294008,-5.62094444041242,130.38509996797));
#40884=CARTESIAN_POINT('Ctrl Pts',(3.91443940300342,-5.52261981534696,130.393237144387));
#40885=CARTESIAN_POINT('Ctrl Pts',(4.05285832728311,-5.41909848397055,130.401374320803));
#40886=CARTESIAN_POINT('Ctrl Pts',(4.19319013238832,-5.31414653918017,130.409623948959));
#40887=CARTESIAN_POINT('Ctrl Pts',(4.32929078473411,-5.20385345154031,130.417873577114));
#40888=CARTESIAN_POINT('Ctrl Pts',(4.46074768411949,-5.08861661933994,130.42612320527));
#40889=CARTESIAN_POINT('Ctrl Pts',(4.59220458350477,-4.97337978713966,130.434372833425));
#40890=CARTESIAN_POINT('Ctrl Pts',(4.71901749416093,-4.85319952097227,130.44262246158));
#40891=CARTESIAN_POINT('Ctrl Pts',(4.84081577943282,-4.72850838950237,130.450872089736));
#40892=CARTESIAN_POINT('Ctrl Pts',(4.96224849868354,-4.60419150665758,130.459096957413));
#40893=CARTESIAN_POINT('Ctrl Pts',(5.07905975120422,-4.47501932224297,130.467321825091));
#40894=CARTESIAN_POINT('Ctrl Pts',(5.19083848069689,-4.34136900842539,130.475546692768));
#40895=CARTESIAN_POINT('Ctrl Pts',(5.30249127893944,-4.20786926664575,130.483762294212));
#40896=CARTESIAN_POINT('Ctrl Pts',(5.40912261590147,-4.06990171426767,130.491977895656));
#40897=CARTESIAN_POINT('Ctrl Pts',(5.51035759188929,-3.92788088025949,130.500193497099));
#40898=CARTESIAN_POINT('Ctrl Pts',(5.6114988554834,-3.78599151378199,130.508401493427));
#40899=CARTESIAN_POINT('Ctrl Pts',(5.70725349954401,-3.64005662834271,130.516609489755));
#40900=CARTESIAN_POINT('Ctrl Pts',(5.79728625832106,-3.49052446475911,130.524817486083));
#40901=CARTESIAN_POINT('Ctrl Pts',(5.88725375805353,-3.34110068757021,130.533019532955));
#40902=CARTESIAN_POINT('Ctrl Pts',(5.97150744909434,-3.18808513187573,130.541221579826));
#40903=CARTESIAN_POINT('Ctrl Pts',(6.04975480083046,-3.03195577966251,130.549423626698));
#40904=CARTESIAN_POINT('Ctrl Pts',(6.12796114878569,-2.87590824355686,130.557621375469));
#40905=CARTESIAN_POINT('Ctrl Pts',(6.20016726736905,-2.7167504815555,130.565819124241));
#40906=CARTESIAN_POINT('Ctrl Pts',(6.26612605579254,-2.55498595943653,130.574016873012));
#40907=CARTESIAN_POINT('Ctrl Pts',(6.33207226390178,-2.39325229065147,130.582213058228));
#40908=CARTESIAN_POINT('Ctrl Pts',(6.39177337419266,-2.22891318161422,130.590409243444));
#40909=CARTESIAN_POINT('Ctrl Pts',(6.44502990148471,-2.06249328943587,130.598605428659));
#40910=CARTESIAN_POINT('Ctrl Pts',(6.4982824889791,-1.89608570862543,130.60680100754));
#40911=CARTESIAN_POINT('Ctrl Pts',(6.54509133272955,-1.72759799271165,130.61499658642));
#40912=CARTESIAN_POINT('Ctrl Pts',(6.58530645209658,-1.55757116433732,130.6231921653));
#40913=CARTESIAN_POINT('Ctrl Pts',(6.6255259131046,-1.38752597979602,130.631388628979));
#40914=CARTESIAN_POINT('Ctrl Pts',(6.65915014887506,-1.21594170101305,130.639585092657));
#40915=CARTESIAN_POINT('Ctrl Pts',(6.68608004114364,-1.0433708273767,130.647781556336));
#40916=CARTESIAN_POINT('Ctrl Pts',(6.71301774037002,-0.870749925559182,
130.655980396163));
#40917=CARTESIAN_POINT('Ctrl Pts',(6.73325717518532,-0.697142213637369,
130.664179235991));
#40918=CARTESIAN_POINT('Ctrl Pts',(6.7467509524248,-0.523106667855641,130.672378075819));
#40919=CARTESIAN_POINT('Ctrl Pts',(6.76025882429848,-0.348889336995441,
130.680585479568));
#40920=CARTESIAN_POINT('Ctrl Pts',(6.76700693376946,-0.174243637693806,
130.688792883317));
#40921=CARTESIAN_POINT('Ctrl Pts',(6.76699999465041,0.000269075059461636,
130.697000287067));
#40922=CARTESIAN_POINT('Ctrl Pts',(6.7669930518144,0.174875266056849,130.705212087136));
#40923=CARTESIAN_POINT('Ctrl Pts',(6.76022386098969,0.349347970276594,130.713423887205));
#40924=CARTESIAN_POINT('Ctrl Pts',(6.74674916702813,0.523129694440314,130.721635687274));
#40925=CARTESIAN_POINT('Ctrl Pts',(6.73325463643426,0.69716724958432,130.72985957626));
#40926=CARTESIAN_POINT('Ctrl Pts',(6.7130349164852,0.870511435369368,130.738083465246));
#40927=CARTESIAN_POINT('Ctrl Pts',(6.68619834803656,1.04261241634332,130.746307354232));
#40928=CARTESIAN_POINT('Ctrl Pts',(6.66140182273576,1.20163074751253,130.753906085482));
#40929=CARTESIAN_POINT('Ctrl Pts',(6.63095681354871,1.35958760053109,130.761504816732));
#40930=CARTESIAN_POINT('Ctrl Pts',(6.59498663675077,1.51606077090555,130.769103547982));
#40931=CARTESIAN_POINT('Ctrl Pts',(6.55604909223164,1.68544223021088,130.777329138254));
#40932=CARTESIAN_POINT('Ctrl Pts',(6.51052727055085,1.85356040123578,130.785554728526));
#40933=CARTESIAN_POINT('Ctrl Pts',(6.45851629097573,2.01986542106178,130.793780318797));
#40934=CARTESIAN_POINT('Ctrl Pts',(6.40656485515067,2.18598004984698,130.801996492163));
#40935=CARTESIAN_POINT('Ctrl Pts',(6.34813916151968,2.35028532159709,130.810212665529));
#40936=CARTESIAN_POINT('Ctrl Pts',(6.28338531284172,2.51224163056919,130.818428838895));
#40937=CARTESIAN_POINT('Ctrl Pts',(6.21869258501756,2.67404506974153,130.826637257054));
#40938=CARTESIAN_POINT('Ctrl Pts',(6.14768373105114,2.83350363088453,130.834845675212));
#40939=CARTESIAN_POINT('Ctrl Pts',(6.07055464352359,2.99009286143327,130.84305409337));
#40940=CARTESIAN_POINT('Ctrl Pts',(5.99124367379952,3.15111179892206,130.851494717069));
#40941=CARTESIAN_POINT('Ctrl Pts',(5.90546119169844,3.3090963010754,130.859935340768));
#40942=CARTESIAN_POINT('Ctrl Pts',(5.81347385054582,3.46349690183491,130.868375964467));
#40943=CARTESIAN_POINT('Ctrl Pts',(5.72413345520992,3.61345460839659,130.876573708294));
#40944=CARTESIAN_POINT('Ctrl Pts',(5.62894054988741,3.76003148253646,130.884771452121));
#40945=CARTESIAN_POINT('Ctrl Pts',(5.52818643102089,3.90274823475413,130.892969195949));
#40946=CARTESIAN_POINT('Ctrl Pts',(5.42746020013165,4.04542548405532,130.901164670703));
#40947=CARTESIAN_POINT('Ctrl Pts',(5.32117602798296,4.18424444651526,130.909360145457));
#40948=CARTESIAN_POINT('Ctrl Pts',(5.20966860603309,4.31875468339118,130.917555620211));
#40949=CARTESIAN_POINT('Ctrl Pts',(5.09817176159913,4.45325216072028,130.925750317548));
#40950=CARTESIAN_POINT('Ctrl Pts',(4.98145288366333,4.58344145087146,130.933945014885));
#40951=CARTESIAN_POINT('Ctrl Pts',(4.85988705663106,4.70890505285358,130.942139712222));
#40952=CARTESIAN_POINT('Ctrl Pts',(4.73195098717559,4.84094314685721,130.950763824715));
#40953=CARTESIAN_POINT('Ctrl Pts',(4.59864662326234,4.9677466415458,130.959387937208));
#40954=CARTESIAN_POINT('Ctrl Pts',(4.46045520800506,5.08887299285221,130.968012049701));
#40955=CARTESIAN_POINT('Ctrl Pts',(4.32905181572083,5.20404956461711,130.976212542004));
#40956=CARTESIAN_POINT('Ctrl Pts',(4.19323028367595,5.31409314157282,130.984413034306));
#40957=CARTESIAN_POINT('Ctrl Pts',(4.05343801734618,5.41866489455961,130.992613526608));
#40958=CARTESIAN_POINT('Ctrl Pts',(3.91359325594592,5.52327591653951,131.000817098376));
#40959=CARTESIAN_POINT('Ctrl Pts',(3.76977508164834,5.62241081314886,131.009020670143));
#40960=CARTESIAN_POINT('Ctrl Pts',(3.6224597627499,5.71577416167381,131.017224241911));
#40961=CARTESIAN_POINT('Ctrl Pts',(3.47501555347743,5.80921919645517,131.025434991217));
#40962=CARTESIAN_POINT('Ctrl Pts',(3.32406839923682,5.89688241953781,131.033645740524));
#40963=CARTESIAN_POINT('Ctrl Pts',(3.17011952322347,5.97851413049074,131.04185648983));
#40964=CARTESIAN_POINT('Ctrl Pts',(3.14654135573895,5.99101650272455,131.043114013934));
#40965=CARTESIAN_POINT('Ctrl Pts',(3.12289281746731,6.00337748679119,131.044371538037));
#40966=CARTESIAN_POINT('Ctrl Pts',(3.09917575053245,6.01559628526646,131.045629062141));
#40967=CARTESIAN_POINT('Ctrl Pts',(3.09917575053253,6.01559628526642,129.045751582742));
#40968=CARTESIAN_POINT('Ctrl Pts',(2.93382384459265,6.10078395293759,129.054501030655));
#40969=CARTESIAN_POINT('Ctrl Pts',(2.76495772122989,6.17915010267047,129.063250478567));
#40970=CARTESIAN_POINT('Ctrl Pts',(2.59315093316722,6.25042856433173,129.07199992648));
#40971=CARTESIAN_POINT('Ctrl Pts',(2.42134553245632,6.32170645041445,129.08074930374));
#40972=CARTESIAN_POINT('Ctrl Pts',(2.2465997792761,6.3858966531345,129.089498681));
#40973=CARTESIAN_POINT('Ctrl Pts',(2.06950718689943,6.44278115439067,129.09824805826));
#40974=CARTESIAN_POINT('Ctrl Pts',(1.8924159657289,6.49966521519715,129.106997367774));
#40975=CARTESIAN_POINT('Ctrl Pts',(1.71297821457231,6.54924360009537,129.115746677289));
#40976=CARTESIAN_POINT('Ctrl Pts',(1.53180337335883,6.59134792173547,129.124495986804));
#40977=CARTESIAN_POINT('Ctrl Pts',(1.35062987477833,6.63345193135294,129.13324523148));
#40978=CARTESIAN_POINT('Ctrl Pts',(1.16771959103014,6.66808192368227,129.141994476156));
#40979=CARTESIAN_POINT('Ctrl Pts',(0.983693746907582,6.69512028363157,129.150743720832));
#40980=CARTESIAN_POINT('Ctrl Pts',(0.79966920542072,6.72215845218857,129.159492903576));
#40981=CARTESIAN_POINT('Ctrl Pts',(0.614529402874435,6.7416050542457,129.16824208632));
#40982=CARTESIAN_POINT('Ctrl Pts',(0.428903127364318,6.75339404354115,129.176991269065));
#40983=CARTESIAN_POINT('Ctrl Pts',(0.243278104164956,6.76518295330326,129.185740392783));
#40984=CARTESIAN_POINT('Ctrl Pts',(0.0571669005402013,6.76931433552275,
129.194489516502));
#40985=CARTESIAN_POINT('Ctrl Pts',(-0.128798404776425,6.76577415902475,
129.20323864022));
#40986=CARTESIAN_POINT('Ctrl Pts',(-0.314762517257864,6.76223400523447,
129.21198770782));
#40987=CARTESIAN_POINT('Ctrl Pts',(-0.500580446818132,6.75102239665099,
129.220736775419));
#40988=CARTESIAN_POINT('Ctrl Pts',(-0.685621118841091,6.73217741012513,
129.229485843018));
#40989=CARTESIAN_POINT('Ctrl Pts',(-0.870660665412942,6.71333253821792,
129.238234857404));
#40990=CARTESIAN_POINT('Ctrl Pts',(-1.0549226788533,6.68685441030637,129.24698387179));
#40991=CARTESIAN_POINT('Ctrl Pts',(-1.23778137635093,6.65283295028207,129.255732886175));
#40992=CARTESIAN_POINT('Ctrl Pts',(-1.42999922978675,6.61707018861902,129.264929696543));
#40993=CARTESIAN_POINT('Ctrl Pts',(-1.62066601233511,6.57297172934458,129.27412650691));
#40994=CARTESIAN_POINT('Ctrl Pts',(-1.8090662850019,6.52070304311349,129.283323317277));
#40995=CARTESIAN_POINT('Ctrl Pts',(-1.98831342545335,6.4709737491509,129.292073315015));
#40996=CARTESIAN_POINT('Ctrl Pts',(-2.16550875896513,6.41384933989592,129.300823312753));
#40997=CARTESIAN_POINT('Ctrl Pts',(-2.34005036713826,6.34952386240544,129.309573310491));
#40998=CARTESIAN_POINT('Ctrl Pts',(-2.51458843546905,6.28519968948669,129.318323130772));
#40999=CARTESIAN_POINT('Ctrl Pts',(-2.68647261717874,6.21367483971177,129.327072951052));
#41000=CARTESIAN_POINT('Ctrl Pts',(-2.85511905908553,6.13519226743927,129.335822771333));
#41001=CARTESIAN_POINT('Ctrl Pts',(-3.02376230488714,6.05671118253022,129.344572425792));
#41002=CARTESIAN_POINT('Ctrl Pts',(-3.18916767379743,5.97127275992719,129.35332208025));
#41003=CARTESIAN_POINT('Ctrl Pts',(-3.35077334102635,5.87916720438083,129.362071734709));
#41004=CARTESIAN_POINT('Ctrl Pts',(-3.51237616037228,5.78706327195729,129.370821234977));
#41005=CARTESIAN_POINT('Ctrl Pts',(-3.67017916302171,5.68829258362382,129.379570735246));
#41006=CARTESIAN_POINT('Ctrl Pts',(-3.82364636566344,5.58319061741123,129.388320235514));
#41007=CARTESIAN_POINT('Ctrl Pts',(-3.977111067787,5.47809036367774,129.397069593223));
#41008=CARTESIAN_POINT('Ctrl Pts',(-4.12623987481848,5.36665920043287,129.405818950931));
#41009=CARTESIAN_POINT('Ctrl Pts',(-4.27052628213868,5.24927559512385,129.41456830864));
#41010=CARTESIAN_POINT('Ctrl Pts',(-4.41481053024925,5.13189374643082,129.423317535416));
#41011=CARTESIAN_POINT('Ctrl Pts',(-4.55425230136485,5.00855981477394,129.432066762193));
#41012=CARTESIAN_POINT('Ctrl Pts',(-4.6883780063051,4.87969268192113,129.440815988969));
#41013=CARTESIAN_POINT('Ctrl Pts',(-4.82250188228874,4.75082730631831,129.44956509644));
#41014=CARTESIAN_POINT('Ctrl Pts',(-4.95130963052961,4.61642907903532,129.458314203911));
#41015=CARTESIAN_POINT('Ctrl Pts',(-5.07436379033377,4.47695444731678,129.467063311382));
#41016=CARTESIAN_POINT('Ctrl Pts',(-5.19741643562798,4.33748153220595,129.475812311171));
#41017=CARTESIAN_POINT('Ctrl Pts',(-5.31471544462749,4.19293255254619,129.484561310961));
#41018=CARTESIAN_POINT('Ctrl Pts',(-5.42586245275589,4.04379841779655,129.493310310751));
#41019=CARTESIAN_POINT('Ctrl Pts',(-5.5370216001911,3.89464799484404,129.502060266093));
#41020=CARTESIAN_POINT('Ctrl Pts',(-5.64202723081205,3.7409116444392,129.510810221435));
#41021=CARTESIAN_POINT('Ctrl Pts',(-5.74052265232917,3.58311159163312,129.519560176777));
#41022=CARTESIAN_POINT('Ctrl Pts',(-5.83901427066877,3.42531763191853,129.52830979426));
#41023=CARTESIAN_POINT('Ctrl Pts',(-5.93099603115707,3.26346052695673,129.537059411742));
#41024=CARTESIAN_POINT('Ctrl Pts',(-6.01615550622728,3.09809004467126,129.545809029225));
#41025=CARTESIAN_POINT('Ctrl Pts',(-6.10131214578772,2.93272506863885,129.554558355376));
#41026=CARTESIAN_POINT('Ctrl Pts',(-6.17964682328718,2.76384720416959,129.563307681527));
#41027=CARTESIAN_POINT('Ctrl Pts',(-6.25089348288533,2.59203002791667,129.572057007678));
#41028=CARTESIAN_POINT('Ctrl Pts',(-6.32213814889297,2.42021765937114,129.58080608901));
#41029=CARTESIAN_POINT('Ctrl Pts',(-6.38629508412551,2.24546640832015,129.589555170341));
#41030=CARTESIAN_POINT('Ctrl Pts',(-6.44314639819777,2.06836976660151,129.598304251673));
#41031=CARTESIAN_POINT('Ctrl Pts',(-6.50000285283667,1.89125711158388,129.607054124107));
#41032=CARTESIAN_POINT('Ctrl Pts',(-6.54955227673219,1.71179891440371,129.615803996542));
#41033=CARTESIAN_POINT('Ctrl Pts',(-6.59162635926357,1.5306047627855,129.624553868976));
#41034=CARTESIAN_POINT('Ctrl Pts',(-6.63369752055173,1.34942319164813,129.633303133898));
#41035=CARTESIAN_POINT('Ctrl Pts',(-6.66829431424234,1.16650618642819,129.642052398821));
#41036=CARTESIAN_POINT('Ctrl Pts',(-6.69529923745401,0.982474997619684,
129.650801663743));
#41037=CARTESIAN_POINT('Ctrl Pts',(-6.7223055473143,0.798434359178886,129.659551377923));
#41038=CARTESIAN_POINT('Ctrl Pts',(-6.74171916496692,0.6132797062415,129.668301092103));
#41039=CARTESIAN_POINT('Ctrl Pts',(-6.75347414817267,0.427639953656556,
129.677050806283));
#41040=CARTESIAN_POINT('Ctrl Pts',(-6.76248837758729,0.285283364201413,
129.683760465458));
#41041=CARTESIAN_POINT('Ctrl Pts',(-6.76699999999984,0.142641701109623,
129.690470124634));
#41042=CARTESIAN_POINT('Ctrl Pts',(-6.767,7.7379071769556E-12,129.69717978381));
#41043=CARTESIAN_POINT('',(-6.76699999999221,-7.25967800658328E-6,129.302661224348));
#41044=CARTESIAN_POINT('Ctrl Pts',(3.09917575053256,6.01559628526641,128.651204297413));
#41045=CARTESIAN_POINT('Ctrl Pts',(2.9440104223218,6.09553592877141,128.659420340539));
#41046=CARTESIAN_POINT('Ctrl Pts',(2.78588580690729,6.16939841906691,128.667636383664));
#41047=CARTESIAN_POINT('Ctrl Pts',(2.62532466559796,6.2369831970435,128.67585242679));
#41048=CARTESIAN_POINT('Ctrl Pts',(2.46455027994386,6.30465773566566,128.684079381801));
#41049=CARTESIAN_POINT('Ctrl Pts',(2.30133324025139,6.36603778476158,128.692306336812));
#41050=CARTESIAN_POINT('Ctrl Pts',(2.13621222485776,6.42097238199701,128.700533291823));
#41051=CARTESIAN_POINT('Ctrl Pts',(2.07106150047759,6.44264756849515,128.703779347918));
#41052=CARTESIAN_POINT('Ctrl Pts',(2.00561448731159,6.46331988343004,128.707025404012));
#41053=CARTESIAN_POINT('Ctrl Pts',(1.93990468080482,6.48298224811634,128.710271460107));
#41054=CARTESIAN_POINT('Ctrl Pts',(1.77338196479372,6.53281088930136,128.718497661126));
#41055=CARTESIAN_POINT('Ctrl Pts',(1.60470540771669,6.57628906836901,128.726723862145));
#41056=CARTESIAN_POINT('Ctrl Pts',(1.4344001855779,6.61322803989202,128.734950063164));
#41057=CARTESIAN_POINT('Ctrl Pts',(1.26428626546245,6.65012551826583,128.743167023779));
#41058=CARTESIAN_POINT('Ctrl Pts',(1.09254767054565,6.6804983404962,128.751383984395));
#41059=CARTESIAN_POINT('Ctrl Pts',(0.919725847131263,6.70420713926104,128.759600945011));
#41060=CARTESIAN_POINT('Ctrl Pts',(0.747063465898483,6.72789406473162,128.767810324813));
#41061=CARTESIAN_POINT('Ctrl Pts',(0.573320199519717,6.74492916247715,128.776019704614));
#41062=CARTESIAN_POINT('Ctrl Pts',(0.399048922805098,6.7552238273212,128.784229084416));
#41063=CARTESIAN_POINT('Ctrl Pts',(0.224903459104328,6.76551106005805,128.792432537556));
#41064=CARTESIAN_POINT('Ctrl Pts',(0.0502311008960856,6.76906753141212,
128.800635990696));
#41065=CARTESIAN_POINT('Ctrl Pts',(-0.124408803756455,6.76585629832233,
128.808839443837));
#41066=CARTESIAN_POINT('Ctrl Pts',(-0.298957661599014,6.76264673937757,
128.817038620187));
#41067=CARTESIAN_POINT('Ctrl Pts',(-0.473473741869148,6.75267651152258,
128.825237796537));
#41068=CARTESIAN_POINT('Ctrl Pts',(-0.647396243356407,6.73596074098477,
128.833436972887));
#41069=CARTESIAN_POINT('Ctrl Pts',(-0.821286018700192,6.71924811577145,
128.841634606439));
#41070=CARTESIAN_POINT('Ctrl Pts',(-0.994582080518735,6.69579250422001,
128.84983223999));
#41071=CARTESIAN_POINT('Ctrl Pts',(-1.1667269888724,6.66566104249509,128.858029873541));
#41072=CARTESIAN_POINT('Ctrl Pts',(-1.33885949856776,6.63553175097493,128.866226916662));
#41073=CARTESIAN_POINT('Ctrl Pts',(-1.50984066646091,6.59872762784131,128.874423959783));
#41074=CARTESIAN_POINT('Ctrl Pts',(-1.67912156354888,6.55536724942434,128.882621002903));
#41075=CARTESIAN_POINT('Ctrl Pts',(-1.84842103477821,6.51200211334236,128.890818945434));
#41076=CARTESIAN_POINT('Ctrl Pts',(-2.01601951598553,6.46207937778859,128.899016887966));
#41077=CARTESIAN_POINT('Ctrl Pts',(-2.18138154705541,6.40576799034793,128.907214830497));
#41078=CARTESIAN_POINT('Ctrl Pts',(-2.34679177665886,6.34944018966972,128.915415162505));
#41079=CARTESIAN_POINT('Ctrl Pts',(-2.50996391824188,6.28672014358343,128.923615494514));
#41080=CARTESIAN_POINT('Ctrl Pts',(-2.6703808069506,6.21782561237205,128.931815826522));
#41081=CARTESIAN_POINT('Ctrl Pts',(-2.83096489341449,6.14885927443848,128.940024705493));
#41082=CARTESIAN_POINT('Ctrl Pts',(-2.98878765973918,6.07370573598786,128.948233584464));
#41083=CARTESIAN_POINT('Ctrl Pts',(-3.14335404596476,5.99263000207063,128.956442463434));
#41084=CARTESIAN_POINT('Ctrl Pts',(-3.29800340701176,5.91151074481881,128.964655749122));
#41085=CARTESIAN_POINT('Ctrl Pts',(-3.44939259242023,5.82446313292807,128.972869034809));
#41086=CARTESIAN_POINT('Ctrl Pts',(-3.59705413084859,5.73179645309785,128.981082320497));
#41087=CARTESIAN_POINT('Ctrl Pts',(-3.74493167990867,5.63899421333603,128.989307621209));
#41088=CARTESIAN_POINT('Ctrl Pts',(-3.88907038817019,5.54055668076361,128.997532921921));
#41089=CARTESIAN_POINT('Ctrl Pts',(-4.02903354369501,5.43683526546284,129.005758222633));
#41090=CARTESIAN_POINT('Ctrl Pts',(-4.15561333441668,5.34303175701167,129.013197014927));
#41091=CARTESIAN_POINT('Ctrl Pts',(-4.2787782140976,5.24490719771872,129.020635807221));
#41092=CARTESIAN_POINT('Ctrl Pts',(-4.39823092866461,5.14274767980484,129.028074599515));
#41093=CARTESIAN_POINT('Ctrl Pts',(-4.52725775511892,5.03240009635888,129.036109609567));
#41094=CARTESIAN_POINT('Ctrl Pts',(-4.65235748891922,4.9169981106864,129.04414461962));
#41095=CARTESIAN_POINT('Ctrl Pts',(-4.77309623590166,4.7968574424118,129.052179629672));
#41096=CARTESIAN_POINT('Ctrl Pts',(-4.89369434429776,4.67685671607107,129.060205280406));
#41097=CARTESIAN_POINT('Ctrl Pts',(-5.00994130901634,4.55212855192056,129.068230931139));
#41098=CARTESIAN_POINT('Ctrl Pts',(-5.12143488514761,4.42302992497147,129.076256581873));
#41099=CARTESIAN_POINT('Ctrl Pts',(-5.23282341484566,4.29405293149011,129.084274671041));
#41100=CARTESIAN_POINT('Ctrl Pts',(-5.3394672239266,4.16071395224508,129.092292760209));
#41101=CARTESIAN_POINT('Ctrl Pts',(-5.44099976391248,4.02340783032299,129.100310849377));
#41102=CARTESIAN_POINT('Ctrl Pts',(-5.54768044892983,3.87913968588614,129.108735490827));
#41103=CARTESIAN_POINT('Ctrl Pts',(-5.64871771618113,3.73049188693583,129.117160132278));
#41104=CARTESIAN_POINT('Ctrl Pts',(-5.74373245937411,3.57796400696434,129.125584773729));
#41105=CARTESIAN_POINT('Ctrl Pts',(-5.83405496340395,3.43296861371881,129.13359336993));
#41106=CARTESIAN_POINT('Ctrl Pts',(-5.91893522435928,3.28446750234395,129.141601966131));
#41107=CARTESIAN_POINT('Ctrl Pts',(-5.99809093790158,3.13292101730365,129.149610562332));
#41108=CARTESIAN_POINT('Ctrl Pts',(-6.07723035421531,2.98140573389866,129.157617509658));
#41109=CARTESIAN_POINT('Ctrl Pts',(-6.15064739374005,2.8268466578194,129.165624456983));
#41110=CARTESIAN_POINT('Ctrl Pts',(-6.21810531290707,2.66972944651643,129.173631404309));
#41111=CARTESIAN_POINT('Ctrl Pts',(-6.28556289144914,2.51261302856794,129.181638311204));
#41112=CARTESIAN_POINT('Ctrl Pts',(-6.34706126145097,2.35293884734312,129.189645218099));
#41113=CARTESIAN_POINT('Ctrl Pts',(-6.40241158852347,2.19121310034885,129.197652124993));
#41114=CARTESIAN_POINT('Ctrl Pts',(-6.45777275425353,2.02945568434587,129.205660599795));
#41115=CARTESIAN_POINT('Ctrl Pts',(-6.50698336058093,1.86564625967157,129.213669074596));
#41116=CARTESIAN_POINT('Ctrl Pts',(-6.54990431716319,1.70030657118269,129.221677549397));
#41117=CARTESIAN_POINT('Ctrl Pts',(-6.59286143806111,1.53482757087132,129.229692771974));
#41118=CARTESIAN_POINT('Ctrl Pts',(-6.62951823469096,1.36781609729384,129.237707994551));
#41119=CARTESIAN_POINT('Ctrl Pts',(-6.65978655532315,1.19980499979664,129.245723217129));
#41120=CARTESIAN_POINT('Ctrl Pts',(-6.69006970683263,1.0317115801911,129.253742367006));
#41121=CARTESIAN_POINT('Ctrl Pts',(-6.71395809635258,0.86261793319884,129.261761516884));
#41122=CARTESIAN_POINT('Ctrl Pts',(-6.73141547101049,0.69306187071619,129.269780666762));
#41123=CARTESIAN_POINT('Ctrl Pts',(-6.74889317667775,0.523308341778371,
129.27780915581));
#41124=CARTESIAN_POINT('Ctrl Pts',(-6.75992489399972,0.353091696664028,
129.285837644859));
#41125=CARTESIAN_POINT('Ctrl Pts',(-6.76452646095415,0.182950154553431,
129.293866133908));
#41126=CARTESIAN_POINT('Ctrl Pts',(-6.76617640361321,0.12194402529639,129.296744837337));
#41127=CARTESIAN_POINT('Ctrl Pts',(-6.76700013301525,0.0609475105471824,
129.299623540766));
#41128=CARTESIAN_POINT('Ctrl Pts',(-6.76699999998389,-1.47668897061706E-5,
129.302502244194));
#41129=CARTESIAN_POINT('Ctrl Pts',(-6.767,7.17729152692933E-12,129.30282021619));
#41130=CARTESIAN_POINT('Ctrl Pts',(-6.7670000000002,-0.186007249408519,
129.311569727996));
#41131=CARTESIAN_POINT('Ctrl Pts',(-6.75932637295478,-0.372014355520398,
129.320319239802));
#41132=CARTESIAN_POINT('Ctrl Pts',(-6.74400518266987,-0.557389537147947,
129.329068751608));
#41133=CARTESIAN_POINT('Ctrl Pts',(-6.72868405709722,-0.742763935804469,
129.337818226458));
#41134=CARTESIAN_POINT('Ctrl Pts',(-6.70571545653085,-0.927506129688286,
129.346567701309));
#41135=CARTESIAN_POINT('Ctrl Pts',(-6.67517739415759,-1.11098863924319,
129.35531717616));
#41136=CARTESIAN_POINT('Ctrl Pts',(-6.64463945823193,-1.29447038906025,
129.364066614782));
#41137=CARTESIAN_POINT('Ctrl Pts',(-6.60653217027261,-1.47669218227756,
129.372816053404));
#41138=CARTESIAN_POINT('Ctrl Pts',(-6.56098496116824,-1.65703510503676,
129.381565492025));
#41139=CARTESIAN_POINT('Ctrl Pts',(-6.51543793687637,-1.83737729603595,
129.390314895146));
#41140=CARTESIAN_POINT('Ctrl Pts',(-6.46245112202766,-2.01584035396648,
129.399064298266));
#41141=CARTESIAN_POINT('Ctrl Pts',(-6.40220448416374,-2.19181813637757,
129.407813701386));
#41142=CARTESIAN_POINT('Ctrl Pts',(-6.34195808575326,-2.36779521935571,
129.416563069731));
#41143=CARTESIAN_POINT('Ctrl Pts',(-6.2744520148938,-2.54128677544468,129.425312438077));
#41144=CARTESIAN_POINT('Ctrl Pts',(-6.19991555136335,-2.71170355237495,
129.434061806422));
#41145=CARTESIAN_POINT('Ctrl Pts',(-6.12537937789198,-2.88211966612733,
129.442811140719));
#41146=CARTESIAN_POINT('Ctrl Pts',(-6.04381298133785,-3.04946076210112,
129.451560475016));
#41147=CARTESIAN_POINT('Ctrl Pts',(-5.95549339426482,-3.21315848206528,
129.460309809313));
#41148=CARTESIAN_POINT('Ctrl Pts',(-5.86717414355344,-3.37685557859318,
129.469059110289));
#41149=CARTESIAN_POINT('Ctrl Pts',(-5.77210188986428,-3.53690907467001,
129.477808411264));
#41150=CARTESIAN_POINT('Ctrl Pts',(-5.67059953467265,-3.69277536784603,
129.48655771224));
#41151=CARTESIAN_POINT('Ctrl Pts',(-5.56909755761984,-3.84864108035476,
129.495306980621));
#41152=CARTESIAN_POINT('Ctrl Pts',(-5.46116568338311,-4.00031938103949,
129.504056249001));
#41153=CARTESIAN_POINT('Ctrl Pts',(-5.3471704868638,-4.14729511662876,129.512805517382));
#41154=CARTESIAN_POINT('Ctrl Pts',(-5.23317570555785,-4.29427031687715,
129.521554753895));
#41155=CARTESIAN_POINT('Ctrl Pts',(-5.11311782179073,-4.43654275986821,
129.530303990407));
#41156=CARTESIAN_POINT('Ctrl Pts',(-4.98740459172281,-4.57362924147358,
129.53905322692));
#41157=CARTESIAN_POINT('Ctrl Pts',(-4.86169180911101,-4.71071523514156,
129.547802432291));
#41158=CARTESIAN_POINT('Ctrl Pts',(-4.73032391415706,-4.84261509316256,
129.556551637662));
#41159=CARTESIAN_POINT('Ctrl Pts',(-4.59374707237571,-4.96888084331267,
129.565300843033));
#41160=CARTESIAN_POINT('Ctrl Pts',(-4.45717070537693,-5.09514615452469,
129.57405001799));
#41161=CARTESIAN_POINT('Ctrl Pts',(-4.31538563819814,-5.2157772025338,129.582799192946));
#41162=CARTESIAN_POINT('Ctrl Pts',(-4.16887341290967,-5.33036429028401,
129.591548367902));
#41163=CARTESIAN_POINT('Ctrl Pts',(-4.02236168477664,-5.44495098920936,
129.60029751317));
#41164=CARTESIAN_POINT('Ctrl Pts',(-3.87112305634771,-5.55349359238527,
129.609046658438));
#41165=CARTESIAN_POINT('Ctrl Pts',(-3.71567117317071,-5.65562346102251,
129.617795803706));
#41166=CARTESIAN_POINT('Ctrl Pts',(-3.56021980457659,-5.75775299158547,
129.626544920012));
#41167=CARTESIAN_POINT('Ctrl Pts',(-3.40055544862767,-5.85346967275132,
129.635294036318));
#41168=CARTESIAN_POINT('Ctrl Pts',(-3.23722036323803,-5.94244842803344,
129.644043152624));
#41169=CARTESIAN_POINT('Ctrl Pts',(-3.07388580496466,-6.03142689616261,
129.652792240695));
#41170=CARTESIAN_POINT('Ctrl Pts',(-2.90688079258145,-6.11366734484614,
129.661541328766));
#41171=CARTESIAN_POINT('Ctrl Pts',(-2.73677251095072,-6.188890467871,129.670290416837));
#41172=CARTESIAN_POINT('Ctrl Pts',(-2.56666476417092,-6.26411335438088,
129.679039477399));
#41173=CARTESIAN_POINT('Ctrl Pts',(-2.39345402972529,-6.33231884350126,
129.687788537962));
#41174=CARTESIAN_POINT('Ctrl Pts',(-2.21772856474462,-6.39327529620896,
129.696537598524));
#41175=CARTESIAN_POINT('Ctrl Pts',(-2.04200363768691,-6.45423156231948,
129.705286632304));
#41176=CARTESIAN_POINT('Ctrl Pts',(-1.86376426620512,-6.50793874251936,
129.714035666084));
#41177=CARTESIAN_POINT('Ctrl Pts',(-1.68361578195104,-6.55421443796016,
129.722784699864));
#41178=CARTESIAN_POINT('Ctrl Pts',(-1.50346783420284,-6.60048999558585,
129.731533707588));
#41179=CARTESIAN_POINT('Ctrl Pts',(-1.32141106257663,-6.63933404145413,
129.740282715312));
#41180=CARTESIAN_POINT('Ctrl Pts',(-1.1380637595946,-6.67061465526959,129.749031723037));
#41181=CARTESIAN_POINT('Ctrl Pts',(-0.954716987423112,-6.70189517852425,
129.757780705431));
#41182=CARTESIAN_POINT('Ctrl Pts',(-0.770079973813634,-6.72561226535785,
129.766529687826));
#41183=CARTESIAN_POINT('Ctrl Pts',(-0.584779770556007,-6.74168536939751,
129.775278670221));
#41184=CARTESIAN_POINT('Ctrl Pts',(-0.391490647557431,-6.75845143942374,
129.784404850897));
#41185=CARTESIAN_POINT('Ctrl Pts',(-0.197480213107819,-6.76689975924016,
129.793531031573));
#41186=CARTESIAN_POINT('Ctrl Pts',(-0.00346532630124065,-6.76699911271707,
129.802657212249));
#41187=CARTESIAN_POINT('Ctrl Pts',(0.1844865952926,-6.76709536139783,129.811498199779));
#41188=CARTESIAN_POINT('Ctrl Pts',(0.372442378181765,-6.75935659726789,
129.820339187309));
#41189=CARTESIAN_POINT('Ctrl Pts',(0.559750217718619,-6.74380965729045,
129.829180174839));
#41190=CARTESIAN_POINT('Ctrl Pts',(0.745129914454193,-6.72842275717292,
129.837930153437));
#41191=CARTESIAN_POINT('Ctrl Pts',(0.929874656310534,-6.70538772273523,
129.846680132035));
#41192=CARTESIAN_POINT('Ctrl Pts',(1.11335688289404,-6.67478280180805,129.855430110632));
#41193=CARTESIAN_POINT('Ctrl Pts',(1.29683723118487,-6.64417819418096,129.864179999657));
#41194=CARTESIAN_POINT('Ctrl Pts',(1.4790548072987,-6.60600390230157,129.872929888682));
#41195=CARTESIAN_POINT('Ctrl Pts',(1.65939064804448,-6.56038959797225,129.881679777707));
#41196=CARTESIAN_POINT('Ctrl Pts',(1.83972470263903,-6.51477574543358,129.890429580068));
#41197=CARTESIAN_POINT('Ctrl Pts',(2.01817678125484,-6.46172209820213,129.899179382429));
#41198=CARTESIAN_POINT('Ctrl Pts',(2.19414072347314,-6.40140886724139,129.90792918479));
#41199=CARTESIAN_POINT('Ctrl Pts',(2.37010298131733,-6.3410962136151,129.916678903396));
#41200=CARTESIAN_POINT('Ctrl Pts',(2.5435768792655,-6.27352420826118,129.925428622001));
#41201=CARTESIAN_POINT('Ctrl Pts',(2.71397317789611,-6.19892237325654,129.934178340607));
#41202=CARTESIAN_POINT('Ctrl Pts',(2.8843679020684,-6.12432122757133,129.942927978365));
#41203=CARTESIAN_POINT('Ctrl Pts',(3.05168482125896,-6.04269049717599,129.951677616123));
#41204=CARTESIAN_POINT('Ctrl Pts',(3.21535561997029,-5.95430745235124,129.960427253881));
#41205=CARTESIAN_POINT('Ctrl Pts',(3.37902496074928,-5.8659251948172,129.9691768137));
#41206=CARTESIAN_POINT('Ctrl Pts',(3.53904799384529,-5.77079087940444,129.977926373519));
#41207=CARTESIAN_POINT('Ctrl Pts',(3.69488118814646,-5.66922763747245,129.986675933338));
#41208=CARTESIAN_POINT('Ctrl Pts',(3.85071304610505,-5.56766526649279,129.995425418126));
#41209=CARTESIAN_POINT('Ctrl Pts',(4.0023548970565,-5.45967423580947,130.004174902913));
#41210=CARTESIAN_POINT('Ctrl Pts',(4.14929168607347,-5.34562133936567,130.012924387701));
#41211=CARTESIAN_POINT('Ctrl Pts',(4.29622726385449,-5.23156938308783,130.021673800364));
#41212=CARTESIAN_POINT('Ctrl Pts',(4.43845763091759,-5.11145583677469,130.030423213027));
#41213=CARTESIAN_POINT('Ctrl Pts',(4.57549970660654,-4.98568866204494,130.039172625691));
#41214=CARTESIAN_POINT('Ctrl Pts',(4.7125406981499,-4.85992248226457,130.047921969137));
#41215=CARTESIAN_POINT('Ctrl Pts',(4.84439326931013,-4.7285029573431,130.056671312583));
#41216=CARTESIAN_POINT('Ctrl Pts',(4.97060959434401,-4.59187644222003,130.06542065603));
#41217=CARTESIAN_POINT('Ctrl Pts',(5.09682496280234,-4.45525096256986,130.074169933166));
#41218=CARTESIAN_POINT('Ctrl Pts',(5.21740397615573,-4.31341878218648,130.082919210302));
#41219=CARTESIAN_POINT('Ctrl Pts',(5.33193710451683,-4.16686161438999,130.091668487438));
#41220=CARTESIAN_POINT('Ctrl Pts',(5.44646940289147,-4.02030550864834,130.100417701171));
#41221=CARTESIAN_POINT('Ctrl Pts',(5.55495572749443,-3.86902470980452,130.109166914904));
#41222=CARTESIAN_POINT('Ctrl Pts',(5.65702762491248,-3.71353301466098,130.117916128637));
#41223=CARTESIAN_POINT('Ctrl Pts',(5.75909881654965,-3.55804239467199,130.126665281873));
#41224=CARTESIAN_POINT('Ctrl Pts',(5.85475551250611,-3.39834117619848,130.13541443511));
#41225=CARTESIAN_POINT('Ctrl Pts',(5.94367283727941,-3.23497174692253,130.144163588346));
#41226=CARTESIAN_POINT('Ctrl Pts',(6.03258957676174,-3.07160339301236,130.152912683991));
#41227=CARTESIAN_POINT('Ctrl Pts',(6.11476689685163,-2.9045671282976,130.161661779637));
#41228=CARTESIAN_POINT('Ctrl Pts',(6.18992570525154,-2.73443024476146,130.170410875282));
#41229=CARTESIAN_POINT('Ctrl Pts',(6.26508404388601,-2.56429442463265,130.179159916243));
#41230=CARTESIAN_POINT('Ctrl Pts',(6.33322384283229,-2.39105828656222,130.187908957204));
#41231=CARTESIAN_POINT('Ctrl Pts',(6.39411368719956,-2.21531017132304,130.196657998165));
#41232=CARTESIAN_POINT('Ctrl Pts',(6.45500317120823,-2.03956309619728,130.205406987348));
#41233=CARTESIAN_POINT('Ctrl Pts',(6.50864269270015,-1.86130434438837,130.21415597653));
#41234=CARTESIAN_POINT('Ctrl Pts',(6.55485008446284,-1.68113930720138,130.222904965713));
#41235=CARTESIAN_POINT('Ctrl Pts',(6.60199664749362,-1.49731239212026,130.231831779242));
#41236=CARTESIAN_POINT('Ctrl Pts',(6.64140563640871,-1.31150116499851,130.240758592771));
#41237=CARTESIAN_POINT('Ctrl Pts',(6.67293772282143,-1.12436255155832,130.249685406301));
#41238=CARTESIAN_POINT('Ctrl Pts',(6.70384494949846,-0.940932395053107,
130.258435320456));
#41239=CARTESIAN_POINT('Ctrl Pts',(6.7271844934891,-0.756227260508516,130.267185234612));
#41240=CARTESIAN_POINT('Ctrl Pts',(6.74287707373917,-0.57087456454353,130.275935148767));
#41241=CARTESIAN_POINT('Ctrl Pts',(6.7585693453866,-0.385525513634243,130.284684890851));
#41242=CARTESIAN_POINT('Ctrl Pts',(6.76661493004098,-0.199529212419925,
130.293434632935));
#41243=CARTESIAN_POINT('Ctrl Pts',(6.76698649908906,-0.0135174386020487,
130.302184375019));
#41244=CARTESIAN_POINT('Ctrl Pts',(6.76735806132393,0.172490924444134,130.310933956665));
#41245=CARTESIAN_POINT('Ctrl Pts',(6.76005588896298,0.358514472899743,130.319683538311));
#41246=CARTESIAN_POINT('Ctrl Pts',(6.74510478454598,0.543921359660529,130.328433119957));
#41247=CARTESIAN_POINT('Ctrl Pts',(6.73015393440706,0.729325093148722,130.337182552796));
#41248=CARTESIAN_POINT('Ctrl Pts',(6.70755443556921,0.914111900254591,130.345931985635));
#41249=CARTESIAN_POINT('Ctrl Pts',(6.67738304682348,1.09765415591358,130.354681418474));
#41250=CARTESIAN_POINT('Ctrl Pts',(6.64721213111895,1.28119353391092,130.363430714135));
#41251=CARTESIAN_POINT('Ctrl Pts',(6.60946960955534,1.46348811672471,130.372180009797));
#41252=CARTESIAN_POINT('Ctrl Pts',(6.56428366991229,1.64391876348039,130.380929305458));
#41253=CARTESIAN_POINT('Ctrl Pts',(6.51909837867768,1.82434682109535,130.389678475569));
#41254=CARTESIAN_POINT('Ctrl Pts',(6.46646995271977,2.00291071820265,130.39842764568));
#41255=CARTESIAN_POINT('Ctrl Pts',(6.4065771328161,2.17900400212526,130.407176815791));
#41256=CARTESIAN_POINT('Ctrl Pts',(6.34668509279124,2.35509499309484,130.415925871976));
#41257=CARTESIAN_POINT('Ctrl Pts',(6.27952894037595,2.52871516397952,130.424674928162));
#41258=CARTESIAN_POINT('Ctrl Pts',(6.20533675061519,2.69927486771253,130.433423984348));
#41259=CARTESIAN_POINT('Ctrl Pts',(6.12832117907992,2.87632521635762,130.44250598563));
#41260=CARTESIAN_POINT('Ctrl Pts',(6.04372366626158,3.05007728919842,130.451587986912));
#41261=CARTESIAN_POINT('Ctrl Pts',(5.95185378007948,3.21989527478047,130.460669988195));
#41262=CARTESIAN_POINT('Ctrl Pts',(5.8633445081745,3.38350129286615,130.469419768502));
#41263=CARTESIAN_POINT('Ctrl Pts',(5.76808562057333,3.54345567124836,130.478169548809));
#41264=CARTESIAN_POINT('Ctrl Pts',(5.66640068804559,3.69921508465195,130.486919329116));
#41265=CARTESIAN_POINT('Ctrl Pts',(5.56471941107996,3.85496889852178,130.49566879487));
#41266=CARTESIAN_POINT('Ctrl Pts',(5.45661270815184,4.00652780919541,130.504418260623));
#41267=CARTESIAN_POINT('Ctrl Pts',(5.34244776449182,4.15337704569142,130.513167726377));
#41268=CARTESIAN_POINT('Ctrl Pts',(5.22828631819664,4.30022178356166,130.521916924096));
#41269=CARTESIAN_POINT('Ctrl Pts',(5.10806717844139,4.44235690972598,130.530666121816));
#41270=CARTESIAN_POINT('Ctrl Pts',(4.98219864544791,4.57929969070567,130.539415319535));
#41271=CARTESIAN_POINT('Ctrl Pts',(4.85633329944115,4.71623900429907,130.548164295726));
#41272=CARTESIAN_POINT('Ctrl Pts',(4.72481904033759,4.84798602483508,130.556913271916));
#41273=CARTESIAN_POINT('Ctrl Pts',(4.5881025073733,4.97409332259004,130.565662248106));
#41274=CARTESIAN_POINT('Ctrl Pts',(4.45137708685779,5.10020881822015,130.574411793042));
#41275=CARTESIAN_POINT('Ctrl Pts',(4.30944892636194,5.22068366307815,130.583161337978));
#41276=CARTESIAN_POINT('Ctrl Pts',(4.16280009466809,5.33510865604735,130.591910882915));
#41277=CARTESIAN_POINT('Ctrl Pts',(4.01615988348944,5.44952692272776,130.600659913523));
#41278=CARTESIAN_POINT('Ctrl Pts',(3.86479978232394,5.55789587288512,130.609408944131));
#41279=CARTESIAN_POINT('Ctrl Pts',(3.70923383581239,5.65984746713765,130.618157974739));
#41280=CARTESIAN_POINT('Ctrl Pts',(3.55366577799716,5.76180044505275,130.626907124087));
#41281=CARTESIAN_POINT('Ctrl Pts',(3.39389200027019,5.85733573570955,130.635656273435));
#41282=CARTESIAN_POINT('Ctrl Pts',(3.23045513626223,5.94612887621829,130.644405422783));
#41283=CARTESIAN_POINT('Ctrl Pts',(3.18695122151704,5.96976399206622,130.646734286896));
#41284=CARTESIAN_POINT('Ctrl Pts',(3.14318791262733,5.99292165435297,130.649063151009));
#41285=CARTESIAN_POINT('Ctrl Pts',(3.09917575053269,6.01559628526634,130.651392015122));
#41286=CARTESIAN_POINT('Origin',(0.,0.,-3.69717978381041));
#41287=CARTESIAN_POINT('',(3.09917575053245,6.01559628526646,133.045751582742));
#41288=CARTESIAN_POINT('',(3.09917575053271,6.01559628526633,132.65155107452));
#41289=CARTESIAN_POINT('',(3.09917575053259,6.01559628526639,-3.69717978381041));
#41290=CARTESIAN_POINT('',(-6.767,7.88350220065452E-12,131.69717978381));
#41291=CARTESIAN_POINT('Ctrl Pts',(-6.767,7.88350217244735E-12,131.69717978381));
#41292=CARTESIAN_POINT('Ctrl Pts',(-6.76700000000022,-0.186007249407913,
131.705929295616));
#41293=CARTESIAN_POINT('Ctrl Pts',(-6.75932637295481,-0.372014355519894,
131.714678807422));
#41294=CARTESIAN_POINT('Ctrl Pts',(-6.7440051826699,-0.557389537147543,
131.723428319228));
#41295=CARTESIAN_POINT('Ctrl Pts',(-6.72868405709726,-0.742763935804164,
131.732177794078));
#41296=CARTESIAN_POINT('Ctrl Pts',(-6.70571545653088,-0.927506129688081,
131.740927268929));
#41297=CARTESIAN_POINT('Ctrl Pts',(-6.67517739415761,-1.11098863924309,
131.74967674378));
#41298=CARTESIAN_POINT('Ctrl Pts',(-6.64463945823194,-1.29447038906024,
131.758426182402));
#41299=CARTESIAN_POINT('Ctrl Pts',(-6.60653217027259,-1.47669218227765,
131.767175621024));
#41300=CARTESIAN_POINT('Ctrl Pts',(-6.56098496116819,-1.65703510503695,
131.775925059646));
#41301=CARTESIAN_POINT('Ctrl Pts',(-6.51543793687633,-1.83737729603611,
131.784674462766));
#41302=CARTESIAN_POINT('Ctrl Pts',(-6.46245112202762,-2.0158403539666,131.793423865886));
#41303=CARTESIAN_POINT('Ctrl Pts',(-6.40220448416371,-2.19181813637767,
131.802173269006));
#41304=CARTESIAN_POINT('Ctrl Pts',(-6.34195808575328,-2.36779521935566,
131.810922637351));
#41305=CARTESIAN_POINT('Ctrl Pts',(-6.27445201489388,-2.54128677544449,
131.819672005697));
#41306=CARTESIAN_POINT('Ctrl Pts',(-6.19991555136349,-2.71170355237462,
131.828421374042));
#41307=CARTESIAN_POINT('Ctrl Pts',(-6.12537937789215,-2.88211966612697,
131.837170708339));
#41308=CARTESIAN_POINT('Ctrl Pts',(-6.04381298133804,-3.04946076210074,
131.845920042636));
#41309=CARTESIAN_POINT('Ctrl Pts',(-5.95549339426504,-3.21315848206488,
131.854669376933));
#41310=CARTESIAN_POINT('Ctrl Pts',(-5.86717414355368,-3.37685557859276,
131.863418677909));
#41311=CARTESIAN_POINT('Ctrl Pts',(-5.77210188986455,-3.53690907466958,
131.872167978884));
#41312=CARTESIAN_POINT('Ctrl Pts',(-5.67059953467294,-3.69277536784558,
131.88091727986));
#41313=CARTESIAN_POINT('Ctrl Pts',(-5.56909755762016,-3.8486410803543,131.889666548241));
#41314=CARTESIAN_POINT('Ctrl Pts',(-5.46116568338346,-4.00031938103901,
131.898415816621));
#41315=CARTESIAN_POINT('Ctrl Pts',(-5.34717048686418,-4.14729511662827,
131.907165085002));
#41316=CARTESIAN_POINT('Ctrl Pts',(-5.23317570555834,-4.29427031687655,
131.915914321515));
#41317=CARTESIAN_POINT('Ctrl Pts',(-5.11311782179134,-4.4365427598675,131.924663558027));
#41318=CARTESIAN_POINT('Ctrl Pts',(-4.98740459172355,-4.57362924147277,
131.93341279454));
#41319=CARTESIAN_POINT('Ctrl Pts',(-4.86169180911188,-4.71071523514066,
131.942161999911));
#41320=CARTESIAN_POINT('Ctrl Pts',(-4.73032391415806,-4.84261509316157,
131.950911205282));
#41321=CARTESIAN_POINT('Ctrl Pts',(-4.59374707237685,-4.96888084331161,
131.959660410653));
#41322=CARTESIAN_POINT('Ctrl Pts',(-4.45717070537813,-5.09514615452364,
131.96840958561));
#41323=CARTESIAN_POINT('Ctrl Pts',(-4.31538563819939,-5.21577720253277,
131.977158760566));
#41324=CARTESIAN_POINT('Ctrl Pts',(-4.16887341291097,-5.33036429028299,
131.985907935522));
#41325=CARTESIAN_POINT('Ctrl Pts',(-4.02236168477799,-5.44495098920836,
131.99465708079));
#41326=CARTESIAN_POINT('Ctrl Pts',(-3.87112305634911,-5.5534935923843,132.003406226058));
#41327=CARTESIAN_POINT('Ctrl Pts',(-3.71567117317216,-5.65562346102156,
132.012155371326));
#41328=CARTESIAN_POINT('Ctrl Pts',(-3.56021980457788,-5.75775299158468,
132.020904487632));
#41329=CARTESIAN_POINT('Ctrl Pts',(-3.40055544862878,-5.85346967275069,
132.029653603938));
#41330=CARTESIAN_POINT('Ctrl Pts',(-3.23722036323895,-5.94244842803293,
132.038402720244));
#41331=CARTESIAN_POINT('Ctrl Pts',(-3.07388580496573,-6.03142689616206,
132.047151808315));
#41332=CARTESIAN_POINT('Ctrl Pts',(-2.90688079258268,-6.11366734484555,
132.055900896386));
#41333=CARTESIAN_POINT('Ctrl Pts',(-2.73677251095211,-6.18889046787039,
132.064649984457));
#41334=CARTESIAN_POINT('Ctrl Pts',(-2.56666476417235,-6.26411335438029,
132.073399045019));
#41335=CARTESIAN_POINT('Ctrl Pts',(-2.39345402972676,-6.3323188435007,132.082148105582));
#41336=CARTESIAN_POINT('Ctrl Pts',(-2.21772856474614,-6.39327529620844,
132.090897166144));
#41337=CARTESIAN_POINT('Ctrl Pts',(-2.04200363768847,-6.45423156231899,
132.099646199924));
#41338=CARTESIAN_POINT('Ctrl Pts',(-1.86376426620672,-6.5079387425189,132.108395233704));
#41339=CARTESIAN_POINT('Ctrl Pts',(-1.68361578195268,-6.55421443795974,
132.117144267484));
#41340=CARTESIAN_POINT('Ctrl Pts',(-1.50346783420465,-6.60048999558543,
132.125893275208));
#41341=CARTESIAN_POINT('Ctrl Pts',(-1.3214110625786,-6.63933404145373,132.134642282932));
#41342=CARTESIAN_POINT('Ctrl Pts',(-1.13806375959673,-6.67061465526923,
132.143391290656));
#41343=CARTESIAN_POINT('Ctrl Pts',(-0.954716987425285,-6.70189517852394,
132.152140273051));
#41344=CARTESIAN_POINT('Ctrl Pts',(-0.770079973815841,-6.7256122653576,
132.160889255446));
#41345=CARTESIAN_POINT('Ctrl Pts',(-0.584779770558248,-6.74168536939732,
132.169638237841));
#41346=CARTESIAN_POINT('Ctrl Pts',(-0.391490647559707,-6.7584514394236,
132.178764418517));
#41347=CARTESIAN_POINT('Ctrl Pts',(-0.19748021311013,-6.7668997592401,132.187890599193));
#41348=CARTESIAN_POINT('Ctrl Pts',(-0.00346532630358167,-6.76699911271707,
132.197016779869));
#41349=CARTESIAN_POINT('Ctrl Pts',(0.184486595290358,-6.76709536139789,
132.205857767399));
#41350=CARTESIAN_POINT('Ctrl Pts',(0.372442378179628,-6.75935659726801,
132.214698754929));
#41351=CARTESIAN_POINT('Ctrl Pts',(0.559750217716585,-6.74380965729062,
132.223539742459));
#41352=CARTESIAN_POINT('Ctrl Pts',(0.745129914452264,-6.72842275717314,
132.232289721057));
#41353=CARTESIAN_POINT('Ctrl Pts',(0.929874656308712,-6.70538772273549,
132.241039699655));
#41354=CARTESIAN_POINT('Ctrl Pts',(1.11335688289232,-6.67478280180833,132.249789678252));
#41355=CARTESIAN_POINT('Ctrl Pts',(1.29683723118313,-6.64417819418129,132.258539567277));
#41356=CARTESIAN_POINT('Ctrl Pts',(1.47905480729694,-6.60600390230196,132.267289456302));
#41357=CARTESIAN_POINT('Ctrl Pts',(1.6593906480427,-6.5603895979727,132.276039345327));
#41358=CARTESIAN_POINT('Ctrl Pts',(1.83972470263724,-6.51477574543409,132.284789147688));
#41359=CARTESIAN_POINT('Ctrl Pts',(2.01817678125304,-6.4617220982027,132.293538950049));
#41360=CARTESIAN_POINT('Ctrl Pts',(2.19414072347133,-6.40140886724202,132.30228875241));
#41361=CARTESIAN_POINT('Ctrl Pts',(2.37010298131551,-6.34109621361578,132.311038471016));
#41362=CARTESIAN_POINT('Ctrl Pts',(2.54357687926368,-6.27352420826192,132.319788189621));
#41363=CARTESIAN_POINT('Ctrl Pts',(2.71397317789427,-6.19892237325734,132.328537908226));
#41364=CARTESIAN_POINT('Ctrl Pts',(2.88436790206668,-6.12432122757214,132.337287545985));
#41365=CARTESIAN_POINT('Ctrl Pts',(3.05168482125735,-6.0426904971768,132.346037183743));
#41366=CARTESIAN_POINT('Ctrl Pts',(3.2153556199688,-5.95430745235204,132.354786821501));
#41367=CARTESIAN_POINT('Ctrl Pts',(3.37902496074778,-5.86592519481806,132.36353638132));
#41368=CARTESIAN_POINT('Ctrl Pts',(3.53904799384379,-5.77079087940536,132.372285941139));
#41369=CARTESIAN_POINT('Ctrl Pts',(3.69488118814496,-5.66922763747342,132.381035500958));
#41370=CARTESIAN_POINT('Ctrl Pts',(3.85071304610356,-5.56766526649382,132.389784985746));
#41371=CARTESIAN_POINT('Ctrl Pts',(4.00235489705502,-5.45967423581056,132.398534470533));
#41372=CARTESIAN_POINT('Ctrl Pts',(4.14929168607199,-5.34562133936682,132.407283955321));
#41373=CARTESIAN_POINT('Ctrl Pts',(4.29622726385312,-5.23156938308896,132.416033367984));
#41374=CARTESIAN_POINT('Ctrl Pts',(4.43845763091632,-5.11145583677579,132.424782780647));
#41375=CARTESIAN_POINT('Ctrl Pts',(4.57549970660538,-4.985688662046,132.433532193311));
#41376=CARTESIAN_POINT('Ctrl Pts',(4.71254069814875,-4.85992248226568,132.442281536757));
#41377=CARTESIAN_POINT('Ctrl Pts',(4.84439326930899,-4.72850295734427,132.451030880203));
#41378=CARTESIAN_POINT('Ctrl Pts',(4.97060959434289,-4.59187644222125,132.45978022365));
#41379=CARTESIAN_POINT('Ctrl Pts',(5.09682496280114,-4.45525096257122,132.468529500786));
#41380=CARTESIAN_POINT('Ctrl Pts',(5.21740397615447,-4.313418782188,132.477278777922));
#41381=CARTESIAN_POINT('Ctrl Pts',(5.33193710451552,-4.16686161439166,132.486028055058));
#41382=CARTESIAN_POINT('Ctrl Pts',(5.44646940289019,-4.02030550865008,132.494777268791));
#41383=CARTESIAN_POINT('Ctrl Pts',(5.55495572749318,-3.86902470980632,132.503526482524));
#41384=CARTESIAN_POINT('Ctrl Pts',(5.65702762491127,-3.71353301466283,132.512275696257));
#41385=CARTESIAN_POINT('Ctrl Pts',(5.75909881654833,-3.55804239467412,132.521024849493));
#41386=CARTESIAN_POINT('Ctrl Pts',(5.85475551250471,-3.39834117620089,132.52977400273));
#41387=CARTESIAN_POINT('Ctrl Pts',(5.94367283727794,-3.23497174692523,132.538523155966));
#41388=CARTESIAN_POINT('Ctrl Pts',(6.03258957676021,-3.07160339301535,132.547272251611));
#41389=CARTESIAN_POINT('Ctrl Pts',(6.11476689685006,-2.90456712830089,132.556021347257));
#41390=CARTESIAN_POINT('Ctrl Pts',(6.18992570524996,-2.73443024476505,132.564770442902));
#41391=CARTESIAN_POINT('Ctrl Pts',(6.26508404388457,-2.5642944246362,132.573519483863));
#41392=CARTESIAN_POINT('Ctrl Pts',(6.33322384283097,-2.39105828656571,132.582268524824));
#41393=CARTESIAN_POINT('Ctrl Pts',(6.39411368719837,-2.21531017132647,132.591017565785));
#41394=CARTESIAN_POINT('Ctrl Pts',(6.45500317120708,-2.03956309620089,132.599766554968));
#41395=CARTESIAN_POINT('Ctrl Pts',(6.50864269269907,-1.86130434439216,132.60851554415));
#41396=CARTESIAN_POINT('Ctrl Pts',(6.55485008446182,-1.68113930720535,132.617264533333));
#41397=CARTESIAN_POINT('Ctrl Pts',(6.60199664749274,-1.49731239212417,132.626191346862));
#41398=CARTESIAN_POINT('Ctrl Pts',(6.64140563640796,-1.31150116500233,132.635118160391));
#41399=CARTESIAN_POINT('Ctrl Pts',(6.6729377228208,-1.12436255156207,132.644044973921));
#41400=CARTESIAN_POINT('Ctrl Pts',(6.70384494949795,-0.940932395056772,
132.652794888076));
#41401=CARTESIAN_POINT('Ctrl Pts',(6.7271844934887,-0.756227260512096,132.661544802232));
#41402=CARTESIAN_POINT('Ctrl Pts',(6.74287707373887,-0.570874564547019,
132.670294716387));
#41403=CARTESIAN_POINT('Ctrl Pts',(6.7585693453864,-0.385525513637769,132.679044458471));
#41404=CARTESIAN_POINT('Ctrl Pts',(6.76661493004088,-0.199529212423483,
132.687794200555));
#41405=CARTESIAN_POINT('Ctrl Pts',(6.76698649908906,-0.0135174386056353,
132.696543942639));
#41406=CARTESIAN_POINT('Ctrl Pts',(6.76735806132403,0.172490924440647,132.705293524285));
#41407=CARTESIAN_POINT('Ctrl Pts',(6.76005588896316,0.358514472896359,132.714043105931));
#41408=CARTESIAN_POINT('Ctrl Pts',(6.74510478454624,0.543921359657251,132.722792687577));
#41409=CARTESIAN_POINT('Ctrl Pts',(6.73015393440741,0.729325093145551,132.731542120416));
#41410=CARTESIAN_POINT('Ctrl Pts',(6.70755443556963,0.91411190025153,132.740291553255));
#41411=CARTESIAN_POINT('Ctrl Pts',(6.67738304682397,1.09765415591064,132.749040986094));
#41412=CARTESIAN_POINT('Ctrl Pts',(6.6472121311195,1.28119353390808,132.757790281755));
#41413=CARTESIAN_POINT('Ctrl Pts',(6.60946960955595,1.46348811672199,132.766539577417));
#41414=CARTESIAN_POINT('Ctrl Pts',(6.56428366991294,1.64391876347778,132.775288873078));
#41415=CARTESIAN_POINT('Ctrl Pts',(6.51909837867838,1.82434682109285,132.784038043189));
#41416=CARTESIAN_POINT('Ctrl Pts',(6.46646995272051,2.00291071820027,132.7927872133));
#41417=CARTESIAN_POINT('Ctrl Pts',(6.40657713281687,2.179004002123,132.801536383411));
#41418=CARTESIAN_POINT('Ctrl Pts',(6.34668509279213,2.35509499309245,132.810285439596));
#41419=CARTESIAN_POINT('Ctrl Pts',(6.27952894037695,2.52871516397701,132.819034495782));
#41420=CARTESIAN_POINT('Ctrl Pts',(6.20533675061634,2.6992748677099,132.827783551968));
#41421=CARTESIAN_POINT('Ctrl Pts',(6.1283211790811,2.87632521635512,132.83686555325));
#41422=CARTESIAN_POINT('Ctrl Pts',(6.04372366626278,3.05007728919604,132.845947554532));
#41423=CARTESIAN_POINT('Ctrl Pts',(5.9518537800807,3.21989527477821,132.855029555815));
#41424=CARTESIAN_POINT('Ctrl Pts',(5.86334450817586,3.38350129286379,132.863779336122));
#41425=CARTESIAN_POINT('Ctrl Pts',(5.76808562057483,3.54345567124591,132.872529116429));
#41426=CARTESIAN_POINT('Ctrl Pts',(5.66640068804725,3.69921508464941,132.881278896736));
#41427=CARTESIAN_POINT('Ctrl Pts',(5.56471941108171,3.85496889851926,132.890028362489));
#41428=CARTESIAN_POINT('Ctrl Pts',(5.45661270815367,4.00652780919292,132.898777828243));
#41429=CARTESIAN_POINT('Ctrl Pts',(5.34244776449373,4.15337704568896,132.907527293996));
#41430=CARTESIAN_POINT('Ctrl Pts',(5.22828631819872,4.30022178355912,132.916276491716));
#41431=CARTESIAN_POINT('Ctrl Pts',(5.10806717844365,4.44235690972338,132.925025689436));
#41432=CARTESIAN_POINT('Ctrl Pts',(4.98219864545034,4.57929969070303,132.933774887155));
#41433=CARTESIAN_POINT('Ctrl Pts',(4.8563332994435,4.71623900429666,132.942523863345));
#41434=CARTESIAN_POINT('Ctrl Pts',(4.72481904033984,4.84798602483289,132.951272839536));
#41435=CARTESIAN_POINT('Ctrl Pts',(4.58810250737544,4.97409332258807,132.960021815726));
#41436=CARTESIAN_POINT('Ctrl Pts',(4.45137708686001,5.10020881821822,132.968771360662));
#41437=CARTESIAN_POINT('Ctrl Pts',(4.30944892636423,5.22068366307626,132.977520905598));
#41438=CARTESIAN_POINT('Ctrl Pts',(4.16280009467045,5.33510865604551,132.986270450534));
#41439=CARTESIAN_POINT('Ctrl Pts',(4.01615988349198,5.44952692272589,132.995019481143));
#41440=CARTESIAN_POINT('Ctrl Pts',(3.86479978232666,5.55789587288323,133.003768511751));
#41441=CARTESIAN_POINT('Ctrl Pts',(3.70923383581529,5.65984746713575,133.012517542359));
#41442=CARTESIAN_POINT('Ctrl Pts',(3.55366577800013,5.76180044505091,133.021266691707));
#41443=CARTESIAN_POINT('Ctrl Pts',(3.39389200027324,5.85733573570779,133.030015841055));
#41444=CARTESIAN_POINT('Ctrl Pts',(3.23045513626535,5.94612887621659,133.038764990403));
#41445=CARTESIAN_POINT('Ctrl Pts',(3.18695122151905,5.96976399206515,133.041093854516));
#41446=CARTESIAN_POINT('Ctrl Pts',(3.14318791262822,5.99292165435252,133.043422718629));
#41447=CARTESIAN_POINT('Ctrl Pts',(3.09917575053245,6.01559628526646,133.045751582742));
#41448=CARTESIAN_POINT('Ctrl Pts',(3.09917575053245,6.01559628526646,131.045629062141));
#41449=CARTESIAN_POINT('Ctrl Pts',(2.94405850634437,6.09551115635822,131.053853674147));
#41450=CARTESIAN_POINT('Ctrl Pts',(2.78600859645521,6.1693398725509,131.062078286153));
#41451=CARTESIAN_POINT('Ctrl Pts',(2.62555104399233,6.23688790306438,131.070302898159));
#41452=CARTESIAN_POINT('Ctrl Pts',(2.514788762354,6.28351564893866,131.075980267516));
#41453=CARTESIAN_POINT('Ctrl Pts',(2.4028796157962,6.32715167023281,131.081657636872));
#41454=CARTESIAN_POINT('Ctrl Pts',(2.29000000142994,6.36774599002276,131.087335006229));
#41455=CARTESIAN_POINT('Ctrl Pts',(2.12793907730266,6.42602713331344,131.095485988403));
#41456=CARTESIAN_POINT('Ctrl Pts',(1.96339721235476,6.47820904559648,131.103636970578));
#41457=CARTESIAN_POINT('Ctrl Pts',(1.79687807751048,6.52407220795128,131.111787952752));
#41458=CARTESIAN_POINT('Ctrl Pts',(1.63055237007467,6.56988209599231,131.119929466805));
#41459=CARTESIAN_POINT('Ctrl Pts',(1.46225431362094,6.60938774845269,131.128070980858));
#41460=CARTESIAN_POINT('Ctrl Pts',(1.29250714134153,6.6424178045032,131.136212494911));
#41461=CARTESIAN_POINT('Ctrl Pts',(1.1229214251043,6.67541644381757,131.144346265114));
#41462=CARTESIAN_POINT('Ctrl Pts',(0.951889693599731,6.70195167961719,131.152480035317));
#41463=CARTESIAN_POINT('Ctrl Pts',(0.77994991477165,6.72190204707326,131.16061380552));
#41464=CARTESIAN_POINT('Ctrl Pts',(0.608137515021744,6.74183763459049,131.168741549938));
#41465=CARTESIAN_POINT('Ctrl Pts',(0.435418769161226,6.75519802525391,131.176869294356));
#41466=CARTESIAN_POINT('Ctrl Pts',(0.262341400720126,6.76191289425324,131.184997038774));
#41467=CARTESIAN_POINT('Ctrl Pts',(0.0893558659115955,6.76862420039038,
131.193120470668));
#41468=CARTESIAN_POINT('Ctrl Pts',(-0.0839875479063557,6.76869699295374,
131.201243902562));
#41469=CARTESIAN_POINT('Ctrl Pts',(-0.257136441490172,6.76211282444014,
131.209367334456));
#41470=CARTESIAN_POINT('Ctrl Pts',(-0.431383723550725,6.75548688855122,
131.217542298207));
#41471=CARTESIAN_POINT('Ctrl Pts',(-0.605433635510642,6.74211920427105,
131.225717261958));
#41472=CARTESIAN_POINT('Ctrl Pts',(-0.778723130219089,6.72204427882336,
131.233892225709));
#41473=CARTESIAN_POINT('Ctrl Pts',(-0.950881212740323,6.70210042315198,
131.242013814882));
#41474=CARTESIAN_POINT('Ctrl Pts',(-1.12228841344074,6.67553671810307,131.250135404055));
#41475=CARTESIAN_POINT('Ctrl Pts',(-1.29239808495552,6.64243902418406,131.258256993228));
#41476=CARTESIAN_POINT('Ctrl Pts',(-1.46253021443577,6.60933696069065,131.266379654617));
#41477=CARTESIAN_POINT('Ctrl Pts',(-1.63136411424499,6.56969926004439,131.274502316007));
#41478=CARTESIAN_POINT('Ctrl Pts',(-1.79836377829489,6.52366283010679,131.282624977396));
#41479=CARTESIAN_POINT('Ctrl Pts',(-1.96541729140136,6.47761155571825,131.290750257938));
#41480=CARTESIAN_POINT('Ctrl Pts',(-2.130635038348,6.42515754064479,131.29887553848));
#41481=CARTESIAN_POINT('Ctrl Pts',(-2.29349665427035,6.36648742218586,131.307000819023));
#41482=CARTESIAN_POINT('Ctrl Pts',(-2.45813261370486,6.30717810496019,131.31521462281));
#41483=CARTESIAN_POINT('Ctrl Pts',(-2.6203604408427,6.24151657467816,131.323428426598));
#41484=CARTESIAN_POINT('Ctrl Pts',(-2.77966465711112,6.16974500234875,131.331642230386));
#41485=CARTESIAN_POINT('Ctrl Pts',(-2.93752468753957,6.09862408127577,131.339781571241));
#41486=CARTESIAN_POINT('Ctrl Pts',(-3.09251359962079,6.02150366498666,131.347920912096));
#41487=CARTESIAN_POINT('Ctrl Pts',(-3.24415618652469,5.93866480258262,131.356060252952));
#41488=CARTESIAN_POINT('Ctrl Pts',(-3.39787973156745,5.85468916054131,131.364311288206));
#41489=CARTESIAN_POINT('Ctrl Pts',(-3.54816410673956,5.76483718973923,131.37256232346));
#41490=CARTESIAN_POINT('Ctrl Pts',(-3.69454655158716,5.66944572054054,131.380813358714));
#41491=CARTESIAN_POINT('Ctrl Pts',(-3.84092899643477,5.57405425134184,131.389064393968));
#41492=CARTESIAN_POINT('Ctrl Pts',(-3.98340923647753,5.47312356037056,131.397315429222));
#41493=CARTESIAN_POINT('Ctrl Pts',(-4.12156135075643,5.36703093264338,131.405566464476));
#41494=CARTESIAN_POINT('Ctrl Pts',(-4.25809289771122,5.26218280447902,131.413720712517));
#41495=CARTESIAN_POINT('Ctrl Pts',(-4.39083963367724,5.15195354324774,131.421874960558));
#41496=CARTESIAN_POINT('Ctrl Pts',(-4.51934434987102,5.03664726254369,131.430029208599));
#41497=CARTESIAN_POINT('Ctrl Pts',(-4.64769529331749,4.92147896092782,131.438173699013));
#41498=CARTESIAN_POINT('Ctrl Pts',(-4.77181405209426,4.80124597537327,131.446318189427));
#41499=CARTESIAN_POINT('Ctrl Pts',(-4.89127328872895,4.67629496663403,131.454462679841));
#41500=CARTESIAN_POINT('Ctrl Pts',(-5.01061475687302,4.55146714043063,131.462599141036));
#41501=CARTESIAN_POINT('Ctrl Pts',(-5.12530559718819,4.42193081397343,131.470735602231));
#41502=CARTESIAN_POINT('Ctrl Pts',(-5.23495242298611,4.28807207601176,131.478872063426));
#41503=CARTESIAN_POINT('Ctrl Pts',(-5.34451425144837,4.15431710426494,131.487002217301));
#41504=CARTESIAN_POINT('Ctrl Pts',(-5.44903962045856,4.01624667499518,131.495132371177));
#41505=CARTESIAN_POINT('Ctrl Pts',(-5.54817283983348,3.87428279031541,131.503262525053));
#41506=CARTESIAN_POINT('Ctrl Pts',(-5.64725193114259,3.73239641981848,131.511388239756));
#41507=CARTESIAN_POINT('Ctrl Pts',(-5.74094452676531,3.58662112671041,131.519513954459));
#41508=CARTESIAN_POINT('Ctrl Pts',(-5.82893598936872,3.43741097802432,131.527639669162));
#41509=CARTESIAN_POINT('Ctrl Pts',(-5.91690213338752,3.28824376293273,131.535763045779));
#41510=CARTESIAN_POINT('Ctrl Pts',(-5.99917022374606,3.13564397445797,131.543886422396));
#41511=CARTESIAN_POINT('Ctrl Pts',(-6.07546961088446,2.98009362390167,131.552009799013));
#41512=CARTESIAN_POINT('Ctrl Pts',(-6.15176159262743,2.82455837060762,131.560132387199));
#41513=CARTESIAN_POINT('Ctrl Pts',(-6.22208586332717,2.6660734540278,131.568254975385));
#41514=CARTESIAN_POINT('Ctrl Pts',(-6.28621832596571,2.50514433881421,131.576377563571));
#41515=CARTESIAN_POINT('Ctrl Pts',(-6.35035679321795,2.34420015608053,131.584500912261));
#41516=CARTESIAN_POINT('Ctrl Pts',(-6.40830216323169,2.18081165940008,131.592624260951));
#41517=CARTESIAN_POINT('Ctrl Pts',(-6.45987898538334,2.01550303750769,131.600747609641));
#41518=CARTESIAN_POINT('Ctrl Pts',(-6.51149544134953,1.85006738546904,131.608877200656));
#41519=CARTESIAN_POINT('Ctrl Pts',(-6.5567334623823,1.68270901015757,131.617006791671));
#41520=CARTESIAN_POINT('Ctrl Pts',(-6.59546767552983,1.51396669086249,131.625136382686));
#41521=CARTESIAN_POINT('Ctrl Pts',(-6.63421667542437,1.34515995435631,131.633269077165));
#41522=CARTESIAN_POINT('Ctrl Pts',(-6.66645684959307,1.17496858031579,131.641401771643));
#41523=CARTESIAN_POINT('Ctrl Pts',(-6.69211428126259,1.00393996161192,131.649534466122));
#41524=CARTESIAN_POINT('Ctrl Pts',(-6.71780393099843,0.832696582075747,
131.657677372834));
#41525=CARTESIAN_POINT('Ctrl Pts',(-6.73689427888086,0.660614220954811,
131.665820279546));
#41526=CARTESIAN_POINT('Ctrl Pts',(-6.74936337392912,0.488244863428358,
131.673963186258));
#41527=CARTESIAN_POINT('Ctrl Pts',(-6.76112933129812,0.325595488752011,
131.681646910928));
#41528=CARTESIAN_POINT('Ctrl Pts',(-6.76700018369326,0.162690847753514,
131.689330635598));
#41529=CARTESIAN_POINT('Ctrl Pts',(-6.76699999999569,-7.64039950798852E-6,
131.697014360268));
#41530=CARTESIAN_POINT('',(-6.76699999999398,6.3820334706712E-6,131.30295982093));
#41531=CARTESIAN_POINT('Ctrl Pts',(3.09917575053269,6.01559628526634,130.651392015122));
#41532=CARTESIAN_POINT('Ctrl Pts',(2.93382384459278,6.10078395293753,130.660141463035));
#41533=CARTESIAN_POINT('Ctrl Pts',(2.76495772123,6.17915010267042,130.668890910947));
#41534=CARTESIAN_POINT('Ctrl Pts',(2.5931509331673,6.25042856433169,130.67764035886));
#41535=CARTESIAN_POINT('Ctrl Pts',(2.42134553245638,6.32170645041443,130.68638973612));
#41536=CARTESIAN_POINT('Ctrl Pts',(2.24659977927614,6.38589665313449,130.69513911338));
#41537=CARTESIAN_POINT('Ctrl Pts',(2.06950718689944,6.44278115439067,130.70388849064));
#41538=CARTESIAN_POINT('Ctrl Pts',(1.89241596572888,6.49966521519716,130.712637800154));
#41539=CARTESIAN_POINT('Ctrl Pts',(1.71297821457226,6.54924360009538,130.721387109669));
#41540=CARTESIAN_POINT('Ctrl Pts',(1.53180337335875,6.59134792173549,130.730136419184));
#41541=CARTESIAN_POINT('Ctrl Pts',(1.3506298747781,6.63345193135299,130.73888566386));
#41542=CARTESIAN_POINT('Ctrl Pts',(1.16771959102975,6.66808192368234,130.747634908536));
#41543=CARTESIAN_POINT('Ctrl Pts',(0.983693746907036,6.69512028363166,130.756384153212));
#41544=CARTESIAN_POINT('Ctrl Pts',(0.799669205420017,6.72215845218865,130.765133335956));
#41545=CARTESIAN_POINT('Ctrl Pts',(0.614529402873574,6.74160505424578,130.7738825187));
#41546=CARTESIAN_POINT('Ctrl Pts',(0.428903127363299,6.75339404354122,130.782631701445));
#41547=CARTESIAN_POINT('Ctrl Pts',(0.243278104163778,6.76518295330331,130.791380825163));
#41548=CARTESIAN_POINT('Ctrl Pts',(0.0571669005388655,6.76931433552276,
130.800129948882));
#41549=CARTESIAN_POINT('Ctrl Pts',(-0.128798404777917,6.76577415902472,
130.8088790726));
#41550=CARTESIAN_POINT('Ctrl Pts',(-0.314762517259383,6.7622340052344,130.8176281402));
#41551=CARTESIAN_POINT('Ctrl Pts',(-0.500580446819676,6.75102239665087,
130.826377207799));
#41552=CARTESIAN_POINT('Ctrl Pts',(-0.685621118842659,6.73217741012497,
130.835126275398));
#41553=CARTESIAN_POINT('Ctrl Pts',(-0.87066066541428,6.71333253821774,130.843875289784));
#41554=CARTESIAN_POINT('Ctrl Pts',(-1.0549226788544,6.68685441030619,130.85262430417));
#41555=CARTESIAN_POINT('Ctrl Pts',(-1.23778137635181,6.6528329502819,130.861373318555));
#41556=CARTESIAN_POINT('Ctrl Pts',(-1.42999922978765,6.61707018861883,130.870570128923));
#41557=CARTESIAN_POINT('Ctrl Pts',(-1.62066601233604,6.57297172934435,130.87976693929));
#41558=CARTESIAN_POINT('Ctrl Pts',(-1.80906628500285,6.52070304311322,130.888963749658));
#41559=CARTESIAN_POINT('Ctrl Pts',(-1.9883134254542,6.47097374915064,130.897713747395));
#41560=CARTESIAN_POINT('Ctrl Pts',(-2.16550875896587,6.41384933989567,130.906463745133));
#41561=CARTESIAN_POINT('Ctrl Pts',(-2.3400503671389,6.34952386240521,130.915213742871));
#41562=CARTESIAN_POINT('Ctrl Pts',(-2.51458843546972,6.28519968948643,130.923963563152));
#41563=CARTESIAN_POINT('Ctrl Pts',(-2.68647261717942,6.21367483971148,130.932713383433));
#41564=CARTESIAN_POINT('Ctrl Pts',(-2.85511905908623,6.13519226743894,130.941463203713));
#41565=CARTESIAN_POINT('Ctrl Pts',(-3.02376230488774,6.05671118252992,130.950212858172));
#41566=CARTESIAN_POINT('Ctrl Pts',(-3.18916767379794,5.97127275992692,130.95896251263));
#41567=CARTESIAN_POINT('Ctrl Pts',(-3.35077334102676,5.8791672043806,130.967712167089));
#41568=CARTESIAN_POINT('Ctrl Pts',(-3.51237616037259,5.78706327195709,130.976461667357));
#41569=CARTESIAN_POINT('Ctrl Pts',(-3.67017916302193,5.68829258362367,130.985211167626));
#41570=CARTESIAN_POINT('Ctrl Pts',(-3.82364636566359,5.58319061741113,130.993960667894));
#41571=CARTESIAN_POINT('Ctrl Pts',(-3.97711106778695,5.47809036367777,131.002710025603));
#41572=CARTESIAN_POINT('Ctrl Pts',(-4.12623987481825,5.36665920043303,131.011459383311));
#41573=CARTESIAN_POINT('Ctrl Pts',(-4.27052628213828,5.24927559512417,131.02020874102));
#41574=CARTESIAN_POINT('Ctrl Pts',(-4.41481053024869,5.1318937464313,131.028957967796));
#41575=CARTESIAN_POINT('Ctrl Pts',(-4.55425230136413,5.00855981477459,131.037707194573));
#41576=CARTESIAN_POINT('Ctrl Pts',(-4.68837800630424,4.87969268192195,131.046456421349));
#41577=CARTESIAN_POINT('Ctrl Pts',(-4.82250188228764,4.75082730631941,131.05520552882));
#41578=CARTESIAN_POINT('Ctrl Pts',(-4.95130963052831,4.6164290790367,131.063954636291));
#41579=CARTESIAN_POINT('Ctrl Pts',(-5.07436379033227,4.47695444731848,131.072703743762));
#41580=CARTESIAN_POINT('Ctrl Pts',(-5.19741643562654,4.33748153220766,131.081452743551));
#41581=CARTESIAN_POINT('Ctrl Pts',(-5.31471544462612,4.19293255254792,131.090201743341));
#41582=CARTESIAN_POINT('Ctrl Pts',(-5.42586245275459,4.04379841779829,131.098950743131));
#41583=CARTESIAN_POINT('Ctrl Pts',(-5.53702160018986,3.89464799484579,131.107700698473));
#41584=CARTESIAN_POINT('Ctrl Pts',(-5.64202723081088,3.74091164444097,131.116450653815));
#41585=CARTESIAN_POINT('Ctrl Pts',(-5.74052265232807,3.58311159163489,131.125200609157));
#41586=CARTESIAN_POINT('Ctrl Pts',(-5.83901427066773,3.42531763192031,131.13395022664));
#41587=CARTESIAN_POINT('Ctrl Pts',(-5.93099603115609,3.26346052695851,131.142699844122));
#41588=CARTESIAN_POINT('Ctrl Pts',(-6.01615550622637,3.09809004467304,131.151449461605));
#41589=CARTESIAN_POINT('Ctrl Pts',(-6.10131214578692,2.93272506864051,131.160198787756));
#41590=CARTESIAN_POINT('Ctrl Pts',(-6.1796468232865,2.76384720417114,131.168948113907));
#41591=CARTESIAN_POINT('Ctrl Pts',(-6.25089348288475,2.59203002791808,131.177697440058));
#41592=CARTESIAN_POINT('Ctrl Pts',(-6.32213814889253,2.42021765937231,131.18644652139));
#41593=CARTESIAN_POINT('Ctrl Pts',(-6.38629508412519,2.24546640832106,131.195195602721));
#41594=CARTESIAN_POINT('Ctrl Pts',(-6.44314639819756,2.06836976660215,131.203944684053));
#41595=CARTESIAN_POINT('Ctrl Pts',(-6.50000285283649,1.8912571115845,131.212694556487));
#41596=CARTESIAN_POINT('Ctrl Pts',(-6.54955227673203,1.71179891440431,131.221444428922));
#41597=CARTESIAN_POINT('Ctrl Pts',(-6.59162635926344,1.53060476278608,131.230194301356));
#41598=CARTESIAN_POINT('Ctrl Pts',(-6.63369752055156,1.34942319164893,131.238943566278));
#41599=CARTESIAN_POINT('Ctrl Pts',(-6.66829431424215,1.16650618642922,131.247692831201));
#41600=CARTESIAN_POINT('Ctrl Pts',(-6.69529923745382,0.982474997620944,
131.256442096123));
#41601=CARTESIAN_POINT('Ctrl Pts',(-6.72230554731415,0.798434359180123,
131.265191810303));
#41602=CARTESIAN_POINT('Ctrl Pts',(-6.74171916496681,0.613279706242714,
131.273941524483));
#41603=CARTESIAN_POINT('Ctrl Pts',(-6.7534741481726,0.427639953657744,131.282691238662));
#41604=CARTESIAN_POINT('Ctrl Pts',(-6.76248837758727,0.285283364202196,
131.289400897838));
#41605=CARTESIAN_POINT('Ctrl Pts',(-6.76699999999984,0.142641701109999,
131.296110557014));
#41606=CARTESIAN_POINT('Ctrl Pts',(-6.767,7.70785566012505E-12,131.30282021619));
#41607=CARTESIAN_POINT('Ctrl Pts',(-6.76699999998758,1.29644361483994E-5,
131.303099416223));
#41608=CARTESIAN_POINT('Ctrl Pts',(-6.76700032597589,-0.170141975692278,
131.311122812505));
#41609=CARTESIAN_POINT('Ctrl Pts',(-6.76057857050752,-0.340538674351975,
131.319146208787));
#41610=CARTESIAN_POINT('Ctrl Pts',(-6.74770595799441,-0.510640092870492,
131.327169605069));
#41611=CARTESIAN_POINT('Ctrl Pts',(-6.73484484324927,-0.680589577456409,
131.335185834884));
#41612=CARTESIAN_POINT('Ctrl Pts',(-6.71554436537688,-0.850243933885984,
131.3432020647));
#41613=CARTESIAN_POINT('Ctrl Pts',(-6.68982777624885,-1.01906492635622,
131.351218294515));
#41614=CARTESIAN_POINT('Ctrl Pts',(-6.66412844176742,-1.18777264771769,
131.35922914581));
#41615=CARTESIAN_POINT('Ctrl Pts',(-6.63202162055116,-1.35564774722754,
131.367239997104));
#41616=CARTESIAN_POINT('Ctrl Pts',(-6.59358247779592,-1.52215607232066,
131.375250848398));
#41617=CARTESIAN_POINT('Ctrl Pts',(-6.55454584916757,-1.69125255013695,
131.383386217831));
#41618=CARTESIAN_POINT('Ctrl Pts',(-6.50897843464434,-1.85893901713537,
131.391521587263));
#41619=CARTESIAN_POINT('Ctrl Pts',(-6.45701324385285,-2.02466514977389,
131.399656956696));
#41620=CARTESIAN_POINT('Ctrl Pts',(-6.40586949160468,-2.18777157043,131.407663726465));
#41621=CARTESIAN_POINT('Ctrl Pts',(-6.34852886718192,-2.34897880902788,
131.415670496235));
#41622=CARTESIAN_POINT('Ctrl Pts',(-6.28516872439752,-2.50777652629879,
131.423677266004));
#41623=CARTESIAN_POINT('Ctrl Pts',(-6.22180617553912,-2.66658027384431,
131.431684339828));
#41624=CARTESIAN_POINT('Ctrl Pts',(-6.15242379264544,-2.82297396783599,
131.439691413651));
#41625=CARTESIAN_POINT('Ctrl Pts',(-6.07724728556253,-2.97646676953109,
131.447698487474));
#41626=CARTESIAN_POINT('Ctrl Pts',(-6.0020528154004,-3.12999624762236,131.45570747455));
#41627=CARTESIAN_POINT('Ctrl Pts',(-5.92106163175092,-3.28062311585741,
131.463716461627));
#41628=CARTESIAN_POINT('Ctrl Pts',(-5.83454555268109,-3.42788086048646,
131.471725448703));
#41629=CARTESIAN_POINT('Ctrl Pts',(-5.74562916691742,-3.57922413180548,
131.479956637543));
#41630=CARTESIAN_POINT('Ctrl Pts',(-5.65087709593312,-3.72700825724675,
131.488187826382));
#41631=CARTESIAN_POINT('Ctrl Pts',(-5.5506316478381,-3.87075926789798,131.496419015222));
#41632=CARTESIAN_POINT('Ctrl Pts',(-5.45293581359008,-4.01085415675773,
131.504440854376));
#41633=CARTESIAN_POINT('Ctrl Pts',(-5.35002292236622,-4.14711833637079,
131.512462693529));
#41634=CARTESIAN_POINT('Ctrl Pts',(-5.24224991833763,-4.2791476714048,131.520484532683));
#41635=CARTESIAN_POINT('Ctrl Pts',(-5.13025801062407,-4.41634545333438,
131.528820396365));
#41636=CARTESIAN_POINT('Ctrl Pts',(-5.01301810471143,-4.54896979008951,
131.537156260048));
#41637=CARTESIAN_POINT('Ctrl Pts',(-4.89097127108512,-4.67661084819124,
131.54549212373));
#41638=CARTESIAN_POINT('Ctrl Pts',(-4.7689244374589,-4.80425190629289,131.553827987412));
#41639=CARTESIAN_POINT('Ctrl Pts',(-4.64207105328817,-4.92690943361687,
131.562163851094));
#41640=CARTESIAN_POINT('Ctrl Pts',(-4.51088814299665,-5.04422215622709,
131.570499714777));
#41641=CARTESIAN_POINT('Ctrl Pts',(-4.38132322710275,-5.16008795768324,
131.578732764909));
#41642=CARTESIAN_POINT('Ctrl Pts',(-4.24710187528017,-5.27112797062188,
131.586965815041));
#41643=CARTESIAN_POINT('Ctrl Pts',(-4.10861753179622,-5.37694625018855,
131.595198865173));
#41644=CARTESIAN_POINT('Ctrl Pts',(-3.97029810187795,-5.48263851645035,
131.603422111007));
#41645=CARTESIAN_POINT('Ctrl Pts',(-3.82772607081388,-5.58312121613811,
131.611645356842));
#41646=CARTESIAN_POINT('Ctrl Pts',(-3.68133079907053,-5.67803597626986,
131.619868602677));
#41647=CARTESIAN_POINT('Ctrl Pts',(-3.53508056026301,-5.77285670490625,
131.628083701791));
#41648=CARTESIAN_POINT('Ctrl Pts',(-3.38501492242836,-5.86212028590153,
131.636298800904));
#41649=CARTESIAN_POINT('Ctrl Pts',(-3.23159539184113,-5.94550924845225,
131.644513900018));
#41650=CARTESIAN_POINT('Ctrl Pts',(-3.07829715692509,-6.02883228249866,
131.652722504157));
#41651=CARTESIAN_POINT('Ctrl Pts',(-2.92165062406743,-6.10628977884796,
131.660931108295));
#41652=CARTESIAN_POINT('Ctrl Pts',(-2.76214536475003,-6.17760811188197,
131.669139712434));
#41653=CARTESIAN_POINT('Ctrl Pts',(-2.60273430706811,-6.24888432527905,
131.677343468683));
#41654=CARTESIAN_POINT('Ctrl Pts',(-2.44046821240763,-6.3140284524504,131.685547224932));
#41655=CARTESIAN_POINT('Ctrl Pts',(-2.27586036665872,-6.37281323996491,
131.693750981181));
#41656=CARTESIAN_POINT('Ctrl Pts',(-2.11130122422227,-6.43158063454252,
131.701952310145));
#41657=CARTESIAN_POINT('Ctrl Pts',(-1.94440204645033,-6.48399231353383,
131.71015363911));
#41658=CARTESIAN_POINT('Ctrl Pts',(-1.77569540740306,-6.52986943362022,
131.718354968074));
#41659=CARTESIAN_POINT('Ctrl Pts',(-1.60701203461207,-6.57574022681373,
131.726555165997));
#41660=CARTESIAN_POINT('Ctrl Pts',(-1.4365220423951,-6.61507816117883,131.734755363919));
#41661=CARTESIAN_POINT('Ctrl Pts',(-1.26477247141517,-6.6477544776827,131.742955561842));
#41662=CARTESIAN_POINT('Ctrl Pts',(-1.0930154618235,-6.68043220942406,131.751156114922));
#41663=CARTESIAN_POINT('Ctrl Pts',(-0.919999116764714,-6.7064476814748,
131.759356668002));
#41664=CARTESIAN_POINT('Ctrl Pts',(-0.746280015309969,-6.72572339148355,
131.767557221082));
#41665=CARTESIAN_POINT('Ctrl Pts',(-0.57252190863849,-6.74500342947489,
131.775759615435));
#41666=CARTESIAN_POINT('Ctrl Pts',(-0.398061087323339,-6.75754065189055,
131.783962009788));
#41667=CARTESIAN_POINT('Ctrl Pts',(-0.22345864827241,-6.76330948815092,
131.792164404141));
#41668=CARTESIAN_POINT('Ctrl Pts',(-0.0486929252473757,-6.76908371928731,
131.800374469175));
#41669=CARTESIAN_POINT('Ctrl Pts',(0.126214321559992,-6.7680769063473,131.808584534209));
#41670=CARTESIAN_POINT('Ctrl Pts',(0.300701650334965,-6.7603156374156,131.816794599243));
#41671=CARTESIAN_POINT('Ctrl Pts',(0.475272485650197,-6.75255065407826,
131.825008593468));
#41672=CARTESIAN_POINT('Ctrl Pts',(0.649422645394069,-6.73802479931206,
131.833222587694));
#41673=CARTESIAN_POINT('Ctrl Pts',(0.822596479925594,-6.71681651016417,
131.841436581919));
#41674=CARTESIAN_POINT('Ctrl Pts',(0.996006408070551,-6.69557930705459,
131.849661774554));
#41675=CARTESIAN_POINT('Ctrl Pts',(1.16843699709867,-6.66764151965963,131.857886967189));
#41676=CARTESIAN_POINT('Ctrl Pts',(1.33934224092393,-6.63313284667787,131.866112159824));
#41677=CARTESIAN_POINT('Ctrl Pts',(1.49303696064819,-6.60209927097665,131.873509057944));
#41678=CARTESIAN_POINT('Ctrl Pts',(1.64549806404139,-6.56575230628646,131.880905956064));
#41679=CARTESIAN_POINT('Ctrl Pts',(1.79634011081175,-6.52422035237076,131.888302854184));
#41680=CARTESIAN_POINT('Ctrl Pts',(1.97265391974131,-6.47567515463612,131.896948820675));
#41681=CARTESIAN_POINT('Ctrl Pts',(2.14715575700586,-6.4199353649967,131.905594787166));
#41682=CARTESIAN_POINT('Ctrl Pts',(2.31925160685557,-6.35715038237243,131.914240753657));
#41683=CARTESIAN_POINT('Ctrl Pts',(2.49112732271792,-6.29444571027618,131.922875660781));
#41684=CARTESIAN_POINT('Ctrl Pts',(2.66060290294181,-6.2247139191908,131.931510567906));
#41685=CARTESIAN_POINT('Ctrl Pts',(2.82709861373037,-6.14815439203049,131.94014547503));
#41686=CARTESIAN_POINT('Ctrl Pts',(2.99912184773473,-6.06905315036136,131.949067054102));
#41687=CARTESIAN_POINT('Ctrl Pts',(3.16796363672579,-5.98266308812476,131.957988633173));
#41688=CARTESIAN_POINT('Ctrl Pts',(3.33300311075027,-5.88925965327808,131.966910212245));
#41689=CARTESIAN_POINT('Ctrl Pts',(3.49229830196621,-5.79910717247266,131.97552127122));
#41690=CARTESIAN_POINT('Ctrl Pts',(3.64805107999634,-5.70242143368215,131.984132330196));
#41691=CARTESIAN_POINT('Ctrl Pts',(3.79972431851457,-5.59949855820046,131.992743389172));
#41692=CARTESIAN_POINT('Ctrl Pts',(3.95125452216798,-5.49667274374104,132.001346327521));
#41693=CARTESIAN_POINT('Ctrl Pts',(4.09871260509386,-5.38762169024554,132.009949265871));
#41694=CARTESIAN_POINT('Ctrl Pts',(4.24158791781282,-5.27268631111925,132.01855220422));
#41695=CARTESIAN_POINT('Ctrl Pts',(4.38430324323248,-5.15787963302991,132.027145509269));
#41696=CARTESIAN_POINT('Ctrl Pts',(4.52244579881903,-5.03720196508959,132.035738814318));
#41697=CARTESIAN_POINT('Ctrl Pts',(4.6555355275429,-4.91103634193292,132.044332119367));
#41698=CARTESIAN_POINT('Ctrl Pts',(4.6703639017783,-4.89697942639369,132.045289554207));
#41699=CARTESIAN_POINT('Ctrl Pts',(4.68512958405555,-4.88285442823404,132.046246989047));
#41700=CARTESIAN_POINT('Ctrl Pts',(4.6998319347832,-4.86866190906619,132.047204423888));
#41701=CARTESIAN_POINT('Ctrl Pts',(4.83182821996074,-4.74124284240334,132.055800181436));
#41702=CARTESIAN_POINT('Ctrl Pts',(4.95856227028189,-4.60852753844506,132.064395938983));
#41703=CARTESIAN_POINT('Ctrl Pts',(5.0796294711552,-4.47097902430459,132.072991696531));
#41704=CARTESIAN_POINT('Ctrl Pts',(5.20080963184321,-4.33330217272376,132.081595474212));
#41705=CARTESIAN_POINT('Ctrl Pts',(5.31631218759829,-4.19078333891176,132.090199251894));
#41706=CARTESIAN_POINT('Ctrl Pts',(5.42577349237088,-4.04391777976327,132.098803029576));
#41707=CARTESIAN_POINT('Ctrl Pts',(5.53953672213847,-3.891280275715,132.107744943244));
#41708=CARTESIAN_POINT('Ctrl Pts',(5.6467740307585,-3.73394778668705,132.116686856912));
#41709=CARTESIAN_POINT('Ctrl Pts',(5.74712813021583,-3.57250713853478,132.12562877058));
#41710=CARTESIAN_POINT('Ctrl Pts',(5.84395025944658,-3.41674840637513,132.13425597291));
#41711=CARTESIAN_POINT('Ctrl Pts',(5.93436532832941,-3.25716604273515,132.142883175241));
#41712=CARTESIAN_POINT('Ctrl Pts',(6.01810032870807,-3.09431049405257,132.151510377572));
#41713=CARTESIAN_POINT('Ctrl Pts',(6.10191507385792,-2.93129985038691,132.160145795992));
#41714=CARTESIAN_POINT('Ctrl Pts',(6.17903692088215,-2.76501007464464,132.168781214413));
#41715=CARTESIAN_POINT('Ctrl Pts',(6.24924085912893,-2.59601188067265,132.177416632833));
#41716=CARTESIAN_POINT('Ctrl Pts',(6.31954851369482,-2.42676401594067,132.186064808854));
#41717=CARTESIAN_POINT('Ctrl Pts',(6.38291772654913,-2.25480002161542,132.194712984876));
#41718=CARTESIAN_POINT('Ctrl Pts',(6.43917272794045,-2.08070747096941,132.203361160897));
#41719=CARTESIAN_POINT('Ctrl Pts',(6.44512429378552,-2.06228913921792,132.204276105128));
#41720=CARTESIAN_POINT('Ctrl Pts',(6.45099627827213,-2.04384699361859,132.20519104936));
#41721=CARTESIAN_POINT('Ctrl Pts',(6.45678850658372,-2.0253817371667,132.206105993592));
#41722=CARTESIAN_POINT('Ctrl Pts',(6.50886471542337,-1.85936608661941,132.214331986133));
#41723=CARTESIAN_POINT('Ctrl Pts',(6.55460232139394,-1.69112279244775,132.222557978675));
#41724=CARTESIAN_POINT('Ctrl Pts',(6.59380855299048,-1.52117644161011,132.230783971216));
#41725=CARTESIAN_POINT('Ctrl Pts',(6.63297368192087,-1.35140825755458,132.239001339867));
#41726=CARTESIAN_POINT('Ctrl Pts',(6.66562099211021,-1.17994091854675,132.247218708519));
#41727=CARTESIAN_POINT('Ctrl Pts',(6.69160700651859,-1.00731557632714,132.25543607717));
#41728=CARTESIAN_POINT('Ctrl Pts',(6.71757097763852,-0.834836667883547,
132.263646475233));
#41729=CARTESIAN_POINT('Ctrl Pts',(6.73688485389486,-0.661202064928187,
132.271856873295));
#41730=CARTESIAN_POINT('Ctrl Pts',(6.74945586139615,-0.486964654841808,
132.280067271357));
#41731=CARTESIAN_POINT('Ctrl Pts',(6.76201871992094,-0.312840191673998,
132.288272347146));
#41732=CARTESIAN_POINT('Ctrl Pts',(6.76784739065311,-0.138114055824268,
132.296477422935));
#41733=CARTESIAN_POINT('Ctrl Pts',(6.76690072919752,0.0366540746184688,
132.304682498724));
#41734=CARTESIAN_POINT('Ctrl Pts',(6.7659544920707,0.211343867503229,132.312883896693));
#41735=CARTESIAN_POINT('Ctrl Pts',(6.75823897519756,0.386075259944744,132.321085294663));
#41736=CARTESIAN_POINT('Ctrl Pts',(6.74376509872549,0.560286795500323,132.329286692632));
#41737=CARTESIAN_POINT('Ctrl Pts',(6.729292355968,0.734484685357088,132.3374874482));
#41738=CARTESIAN_POINT('Ctrl Pts',(6.70806232900693,0.908162441941088,132.345688203768));
#41739=CARTESIAN_POINT('Ctrl Pts',(6.68013797862818,1.08076157707862,132.353888959336));
#41740=CARTESIAN_POINT('Ctrl Pts',(6.65221377009181,1.25335983549483,132.362089673247));
#41741=CARTESIAN_POINT('Ctrl Pts',(6.61759536205288,1.42487912943406,132.370290387159));
#41742=CARTESIAN_POINT('Ctrl Pts',(6.57639721507449,1.5947691587062,132.378491101071));
#41743=CARTESIAN_POINT('Ctrl Pts',(6.53519181123308,1.76468911332114,132.386693259501));
#41744=CARTESIAN_POINT('Ctrl Pts',(6.4874044438204,1.93297888321195,132.39489541793));
#41745=CARTESIAN_POINT('Ctrl Pts',(6.43320003320356,2.09910131551333,132.40309757636));
#41746=CARTESIAN_POINT('Ctrl Pts',(6.37897625143767,2.26528311535249,132.411302666013));
#41747=CARTESIAN_POINT('Ctrl Pts',(6.31833096923049,2.42929569418225,132.419507755666));
#41748=CARTESIAN_POINT('Ctrl Pts',(6.25147803739596,2.59061987716377,132.427712845319));
#41749=CARTESIAN_POINT('Ctrl Pts',(6.18454873399093,2.75212835395074,132.435927308317));
#41750=CARTESIAN_POINT('Ctrl Pts',(6.11139775071242,2.91094196781649,132.444141771314));
#41751=CARTESIAN_POINT('Ctrl Pts',(6.03228635158229,3.06656328363105,132.452356234312));
#41752=CARTESIAN_POINT('Ctrl Pts',(5.95312808144862,3.22227680015656,132.46057556412));
#41753=CARTESIAN_POINT('Ctrl Pts',(5.86800253047451,3.37479393606735,132.468794893927));
#41754=CARTESIAN_POINT('Ctrl Pts',(5.77721541901727,3.52364456241959,132.477014223735));
#41755=CARTESIAN_POINT('Ctrl Pts',(5.68628763843497,3.672725823793,132.485246288895));
#41756=CARTESIAN_POINT('Ctrl Pts',(5.58968096518597,3.81812892439933,132.493478354056));
#41757=CARTESIAN_POINT('Ctrl Pts',(5.48774346832688,3.95941417710192,132.501710419217));
#41758=CARTESIAN_POINT('Ctrl Pts',(5.3961147266374,4.08641150706691,132.509109990478));
#41759=CARTESIAN_POINT('Ctrl Pts',(5.30017950148412,4.21008203931098,132.516509561739));
#41760=CARTESIAN_POINT('Ctrl Pts',(5.20021631297347,4.33013155669485,132.523909133));
#41761=CARTESIAN_POINT('Ctrl Pts',(5.09002475574849,4.46246470314334,132.532065838405));
#41762=CARTESIAN_POINT('Ctrl Pts',(4.97459879515334,4.59080481309166,132.54022254381));
#41763=CARTESIAN_POINT('Ctrl Pts',(4.85425964675934,4.71470595921357,132.548379249216));
#41764=CARTESIAN_POINT('Ctrl Pts',(4.73406400826925,4.83845934758739,132.556526227379));
#41765=CARTESIAN_POINT('Ctrl Pts',(4.60896709600273,4.95778404897345,132.564673205542));
#41766=CARTESIAN_POINT('Ctrl Pts',(4.47933159729462,5.07226551370076,132.572820183705));
#41767=CARTESIAN_POINT('Ctrl Pts',(4.34985683951493,5.18660502767299,132.580957060061));
#41768=CARTESIAN_POINT('Ctrl Pts',(4.21585497965262,5.29611302958615,132.589093936417));
#41769=CARTESIAN_POINT('Ctrl Pts',(4.07772660760713,5.40041060601996,132.597230812773));
#41770=CARTESIAN_POINT('Ctrl Pts',(3.93969708384112,5.50463354437739,132.605361866168));
#41771=CARTESIAN_POINT('Ctrl Pts',(3.79754721515286,5.60365325874456,132.613492919562));
#41772=CARTESIAN_POINT('Ctrl Pts',(3.65171221038628,5.69712970999571,132.621623972956));
#41773=CARTESIAN_POINT('Ctrl Pts',(3.50596741225155,5.79054834113817,132.629749996865));
#41774=CARTESIAN_POINT('Ctrl Pts',(3.35654232549878,5.87843034232569,132.637876020775));
#41775=CARTESIAN_POINT('Ctrl Pts',(3.20390264998644,5.96047790109232,132.646002044684));
#41776=CARTESIAN_POINT('Ctrl Pts',(3.16915822380653,5.97915387992443,132.647851721296));
#41777=CARTESIAN_POINT('Ctrl Pts',(3.1342473592408,5.99752773909303,132.649701397908));
#41778=CARTESIAN_POINT('Ctrl Pts',(3.09917575053271,6.01559628526633,132.65155107452));
#41779=CARTESIAN_POINT('Origin',(0.,0.,-3.69717978381041));
#41780=CARTESIAN_POINT('',(3.09917575053244,6.01559628526647,135.045784814338));
#41781=CARTESIAN_POINT('',(3.09917575053266,6.01559628526635,134.651234928213));
#41782=CARTESIAN_POINT('',(3.09917575053259,6.01559628526639,-3.69717978381041));
#41783=CARTESIAN_POINT('',(-6.76699999998776,1.28714121708955E-5,133.697456813947));
#41784=CARTESIAN_POINT('Ctrl Pts',(-6.76699999998776,1.28714121708955E-5,
133.697456813947));
#41785=CARTESIAN_POINT('Ctrl Pts',(-6.76700032527401,-0.171002714082819,
133.705521296298));
#41786=CARTESIAN_POINT('Ctrl Pts',(-6.76051347811588,-0.342244911284379,
133.713585778649));
#41787=CARTESIAN_POINT('Ctrl Pts',(-6.7475138736617,-0.513172022564486,
133.721650260999));
#41788=CARTESIAN_POINT('Ctrl Pts',(-6.73452560713797,-0.683950055485557,
133.72970770971));
#41789=CARTESIAN_POINT('Ctrl Pts',(-6.71503591741793,-0.854413179796611,
133.73776515842));
#41790=CARTESIAN_POINT('Ctrl Pts',(-6.68907126218211,-1.02401887162759,
133.745822607131));
#41791=CARTESIAN_POINT('Ctrl Pts',(-6.66312357564471,-1.19351372093789,
133.753874790051));
#41792=CARTESIAN_POINT('Ctrl Pts',(-6.63070940404323,-1.36215188586963,
133.761926972972));
#41793=CARTESIAN_POINT('Ctrl Pts',(-6.59190709710128,-1.52939524753605,
133.769979155893));
#41794=CARTESIAN_POINT('Ctrl Pts',(-6.55311856901176,-1.69657922042424,
133.778028479451));
#41795=CARTESIAN_POINT('Ctrl Pts',(-6.50794650233443,-1.86236901246893,
133.78607780301));
#41796=CARTESIAN_POINT('Ctrl Pts',(-6.45652048573947,-2.02623597274024,
133.794127126569));
#41797=CARTESIAN_POINT('Ctrl Pts',(-6.40510272581285,-2.19007662346568,
133.802175157774));
#41798=CARTESIAN_POINT('Ctrl Pts',(-6.34743312544498,-2.35199470073605,
133.810223188979));
#41799=CARTESIAN_POINT('Ctrl Pts',(-6.28369131190787,-2.51147615888616,
133.818271220184));
#41800=CARTESIAN_POINT('Ctrl Pts',(-6.21994712371109,-2.67096355841392,
133.826319551213));
#41801=CARTESIAN_POINT('Ctrl Pts',(-6.1501304108429,-2.82801381168899,133.834367882243));
#41802=CARTESIAN_POINT('Ctrl Pts',(-6.074469112433,-2.9821324588451,133.842416213272));
#41803=CARTESIAN_POINT('Ctrl Pts',(-5.99879002679068,-3.13628733779016,
133.850466436385));
#41804=CARTESIAN_POINT('Ctrl Pts',(-5.91726378593629,-3.28750890436765,
133.858516659499));
#41805=CARTESIAN_POINT('Ctrl Pts',(-5.83016440604902,-3.4353270584384,133.866566882612));
#41806=CARTESIAN_POINT('Ctrl Pts',(-5.74298475381357,-3.58328144436692,
133.874624524955));
#41807=CARTESIAN_POINT('Ctrl Pts',(-5.65022189619028,-3.72782583301491,
133.882682167298));
#41808=CARTESIAN_POINT('Ctrl Pts',(-5.55219368370658,-3.86851835960601,
133.890739809641));
#41809=CARTESIAN_POINT('Ctrl Pts',(-5.45411471478756,-4.0092837330944,133.89880162402));
#41810=CARTESIAN_POINT('Ctrl Pts',(-5.3507651851877,-4.14619297502003,133.906863438399));
#41811=CARTESIAN_POINT('Ctrl Pts',(-5.24250308656071,-4.27883750420618,
133.914925252778));
#41812=CARTESIAN_POINT('Ctrl Pts',(-5.13410347514908,-4.41165051634998,
133.922997307144));
#41813=CARTESIAN_POINT('Ctrl Pts',(-5.02077908181994,-4.54018772098142,
133.93106936151));
#41814=CARTESIAN_POINT('Ctrl Pts',(-4.90292507915519,-4.66407704355225,
133.939141415877));
#41815=CARTESIAN_POINT('Ctrl Pts',(-4.84317738311493,-4.72688442743595,
133.943233654068));
#41816=CARTESIAN_POINT('Ctrl Pts',(-4.78226606659154,-4.78849787873628,
133.947325892259));
#41817=CARTESIAN_POINT('Ctrl Pts',(-4.72024576960563,-4.84887294889443,
133.951418130451));
#41818=CARTESIAN_POINT('Ctrl Pts',(-4.58921478455554,-4.97642804456073,
133.960063848503));
#41819=CARTESIAN_POINT('Ctrl Pts',(-4.45289322364292,-5.0987828514879,133.968709566555));
#41820=CARTESIAN_POINT('Ctrl Pts',(-4.31171019670708,-5.21550037672439,
133.977355284608));
#41821=CARTESIAN_POINT('Ctrl Pts',(-4.17070842000576,-5.33206806044465,
133.98598990332));
#41822=CARTESIAN_POINT('Ctrl Pts',(-4.02485785635243,-5.4430127002739,133.994624522033));
#41823=CARTESIAN_POINT('Ctrl Pts',(-3.8746235271258,-5.5479348881402,134.003259140745));
#41824=CARTESIAN_POINT('Ctrl Pts',(-3.7190835050056,-5.65656252009112,134.012198700647));
#41825=CARTESIAN_POINT('Ctrl Pts',(-3.55884464090013,-5.75873431260608,
134.02113826055));
#41826=CARTESIAN_POINT('Ctrl Pts',(-3.3944618206614,-5.85405141317294,134.030077820452));
#41827=CARTESIAN_POINT('Ctrl Pts',(-3.23612701624646,-5.94586158198338,
134.038688473723));
#41828=CARTESIAN_POINT('Ctrl Pts',(-3.07394802526566,-6.03131224641852,
134.047299126993));
#41829=CARTESIAN_POINT('Ctrl Pts',(-2.90845186068453,-6.11008975172057,
134.055909780264));
#41830=CARTESIAN_POINT('Ctrl Pts',(-2.74311234929429,-6.18879268884391,
134.064512282975));
#41831=CARTESIAN_POINT('Ctrl Pts',(-2.57446219895012,-6.260834929767,134.073114785686));
#41832=CARTESIAN_POINT('Ctrl Pts',(-2.40305368239629,-6.32594830831881,
134.081717288397));
#41833=CARTESIAN_POINT('Ctrl Pts',(-2.23183808267917,-6.39098840307312,
134.090310109165));
#41834=CARTESIAN_POINT('Ctrl Pts',(-2.05787059461596,-6.44911508474629,
134.098902929932));
#41835=CARTESIAN_POINT('Ctrl Pts',(-1.8817243613191,-6.50010787818312,134.1074957507));
#41836=CARTESIAN_POINT('Ctrl Pts',(-1.8609647276262,-6.50611761051127,134.108508453658));
#41837=CARTESIAN_POINT('Ctrl Pts',(-1.84017485500911,-6.51202831013581,
134.109521156616));
#41838=CARTESIAN_POINT('Ctrl Pts',(-1.81935569972229,-6.517839660339,134.110533859574));
#41839=CARTESIAN_POINT('Ctrl Pts',(-1.64265432386261,-6.56716315893246,
134.119129117334));
#41840=CARTESIAN_POINT('Ctrl Pts',(-1.46405013740167,-6.60926775687536,
134.127724375094));
#41841=CARTESIAN_POINT('Ctrl Pts',(-1.28414726211396,-6.64403904332336,
134.136319632854));
#41842=CARTESIAN_POINT('Ctrl Pts',(-1.10407591541294,-6.67884289160653,
134.144922939708));
#41843=CARTESIAN_POINT('Ctrl Pts',(-0.922703752168723,-6.70629966298467,
134.153526246563));
#41844=CARTESIAN_POINT('Ctrl Pts',(-0.740641937071527,-6.7263465953704,
134.162129553417));
#41845=CARTESIAN_POINT('Ctrl Pts',(-0.551031775985763,-6.74722468052463,
134.171089556357));
#41846=CARTESIAN_POINT('Ctrl Pts',(-0.36067393837606,-6.76006537669041,
134.180049559297));
#41847=CARTESIAN_POINT('Ctrl Pts',(-0.170259600931682,-6.76485777147536,
134.189009562237));
#41848=CARTESIAN_POINT('Ctrl Pts',(0.0130745613519903,-6.76947197067393,
134.197636405442));
#41849=CARTESIAN_POINT('Ctrl Pts',(0.196460802399278,-6.76662564682148,
134.206263248647));
#41850=CARTESIAN_POINT('Ctrl Pts',(0.379286276252665,-6.75636225498947,
134.214890091852));
#41851=CARTESIAN_POINT('Ctrl Pts',(0.562286485044416,-6.74608905394925,
134.223525180138));
#41852=CARTESIAN_POINT('Ctrl Pts',(0.744724553152227,-6.72838466137047,
134.232160268424));
#41853=CARTESIAN_POINT('Ctrl Pts',(0.925994478508959,-6.70334418225492,
134.24079535671));
#41854=CARTESIAN_POINT('Ctrl Pts',(1.10753362608138,-6.67826651300287,134.249443269835));
#41855=CARTESIAN_POINT('Ctrl Pts',(1.28790086302661,-6.64583103379531,134.25809118296));
#41856=CARTESIAN_POINT('Ctrl Pts',(1.46650059224313,-6.60618384643892,134.266739096085));
#41857=CARTESIAN_POINT('Ctrl Pts',(1.48653676300824,-6.60173603557317,134.267709260289));
#41858=CARTESIAN_POINT('Ctrl Pts',(1.50655070520403,-6.59719751376894,134.268679424493));
#41859=CARTESIAN_POINT('Ctrl Pts',(1.52654159070996,-6.59256852613856,134.269649588698));
#41860=CARTESIAN_POINT('Ctrl Pts',(1.6960166402935,-6.55332574682559,134.277874268216));
#41861=CARTESIAN_POINT('Ctrl Pts',(1.86420083684811,-6.50749201675033,134.286098947735));
#41862=CARTESIAN_POINT('Ctrl Pts',(2.03054439742182,-6.45516680265498,134.294323627254));
#41863=CARTESIAN_POINT('Ctrl Pts',(2.19671311209436,-6.40289658827937,134.302539661704));
#41864=CARTESIAN_POINT('Ctrl Pts',(2.3610447044058,-6.34414858412145,134.310755696154));
#41865=CARTESIAN_POINT('Ctrl Pts',(2.52300007342333,-6.27907315051401,134.318971730604));
#41866=CARTESIAN_POINT('Ctrl Pts',(2.68481764897097,-6.21405308382559,134.327180774759));
#41867=CARTESIAN_POINT('Ctrl Pts',(2.84426269701035,-6.14271644234302,134.335389818914));
#41868=CARTESIAN_POINT('Ctrl Pts',(3.00081167785889,-6.0652632485347,134.343598863068));
#41869=CARTESIAN_POINT('Ctrl Pts',(3.15725881323326,-5.98786044315566,134.351802566696));
#41870=CARTESIAN_POINT('Ctrl Pts',(3.31081331424066,-5.90434917007936,134.360006270324));
#41871=CARTESIAN_POINT('Ctrl Pts',(3.46097193714386,-5.81497740754878,134.368209973952));
#41872=CARTESIAN_POINT('Ctrl Pts',(3.61106293435191,-5.72564589463857,134.376409982946));
#41873=CARTESIAN_POINT('Ctrl Pts',(3.75776079303372,-5.63045933349806,134.38460999194));
#41874=CARTESIAN_POINT('Ctrl Pts',(3.90058710925378,-5.5297114936607,134.392810000934));
#41875=CARTESIAN_POINT('Ctrl Pts',(4.04340200478046,-5.42897170983302,134.401009354238));
#41876=CARTESIAN_POINT('Ctrl Pts',(4.18234567677989,-5.32267173236167,134.409208707542));
#41877=CARTESIAN_POINT('Ctrl Pts',(4.31696864292013,-5.21114869640508,134.417408060846));
#41878=CARTESIAN_POINT('Ctrl Pts',(4.45159073135833,-5.09962638754579,134.425607360692));
#41879=CARTESIAN_POINT('Ctrl Pts',(4.58189189326765,-4.98288131590588,134.433806660539));
#41880=CARTESIAN_POINT('Ctrl Pts',(4.70745579587629,-4.86129087073287,134.442005960386));
#41881=CARTESIAN_POINT('Ctrl Pts',(4.83304165836984,-4.73967916059336,134.450206694209));
#41882=CARTESIAN_POINT('Ctrl Pts',(4.9538883533594,-4.61322063800784,134.458407428032));
#41883=CARTESIAN_POINT('Ctrl Pts',(5.06961644808113,-4.48232953600528,134.466608161855));
#41884=CARTESIAN_POINT('Ctrl Pts',(5.18538577694114,-4.35139179725636,134.474811817615));
#41885=CARTESIAN_POINT('Ctrl Pts',(5.29603263517155,-4.21601860139181,134.483015473375));
#41886=CARTESIAN_POINT('Ctrl Pts',(5.40121788135593,-4.07665725786715,134.491219129135));
#41887=CARTESIAN_POINT('Ctrl Pts',(5.50652362400182,-3.93713626696442,134.49943218271));
#41888=CARTESIAN_POINT('Ctrl Pts',(5.60635503863194,-3.79361828734885,134.507645236285));
#41889=CARTESIAN_POINT('Ctrl Pts',(5.70041574739976,-3.64658049503873,134.51585828986));
#41890=CARTESIAN_POINT('Ctrl Pts',(5.79453211399928,-3.49945569716798,134.524076203283));
#41891=CARTESIAN_POINT('Ctrl Pts',(5.88287078699965,-3.34880724365436,134.532294116706));
#41892=CARTESIAN_POINT('Ctrl Pts',(5.9651814579846,-3.19513680040727,134.540512030129));
#41893=CARTESIAN_POINT('Ctrl Pts',(6.04762050585149,-3.04122668310437,134.548742760725));
#41894=CARTESIAN_POINT('Ctrl Pts',(6.12401260637912,-2.8842854790704,134.556973491321));
#41895=CARTESIAN_POINT('Ctrl Pts',(6.19415515056027,-2.72483595300481,134.565204221917));
#41896=CARTESIAN_POINT('Ctrl Pts',(6.25857268850193,-2.57840063311418,134.572763163592));
#41897=CARTESIAN_POINT('Ctrl Pts',(6.31771970627631,-2.42985014992169,134.580322105268));
#41898=CARTESIAN_POINT('Ctrl Pts',(6.37147664884281,-2.27959959494004,134.587881046944));
#41899=CARTESIAN_POINT('Ctrl Pts',(6.42946470215801,-2.11752309324662,134.596034939111));
#41900=CARTESIAN_POINT('Ctrl Pts',(6.48135939587856,-1.95296701905082,134.604188831277));
#41901=CARTESIAN_POINT('Ctrl Pts',(6.52693973994569,-1.7864340545113,134.612342723444));
#41902=CARTESIAN_POINT('Ctrl Pts',(6.57246446325864,-1.62010430671513,134.620486665584));
#41903=CARTESIAN_POINT('Ctrl Pts',(6.61169007900027,-1.45180281922105,134.628630607725));
#41904=CARTESIAN_POINT('Ctrl Pts',(6.64444366253621,-1.28205203302455,134.636774549865));
#41905=CARTESIAN_POINT('Ctrl Pts',(6.67716417152547,-1.11247266105808,134.644910268258));
#41906=CARTESIAN_POINT('Ctrl Pts',(6.70342559035815,-0.941447260260673,
134.653045986651));
#41907=CARTESIAN_POINT('Ctrl Pts',(6.72310481979071,-0.76951321113216,134.661181705044));
#41908=CARTESIAN_POINT('Ctrl Pts',(6.74276831668116,-0.597716614523205,
134.669310919344));
#41909=CARTESIAN_POINT('Ctrl Pts',(6.75586006022769,-0.42501317753814,134.677440133644));
#41910=CARTESIAN_POINT('Ctrl Pts',(6.76230804334633,-0.251950246861532,
134.685569347944));
#41911=CARTESIAN_POINT('Ctrl Pts',(6.76875222739921,-0.0789892825583523,
134.69369377262));
#41912=CARTESIAN_POINT('Ctrl Pts',(6.76856043284408,0.0943303891482489,
134.701818197295));
#41913=CARTESIAN_POINT('Ctrl Pts',(6.7617125052461,0.267456531792584,134.709942621971));
#41914=CARTESIAN_POINT('Ctrl Pts',(6.75482300634381,0.441633660951844,134.718116367105));
#41915=CARTESIAN_POINT('Ctrl Pts',(6.74119625329659,0.615614530761113,134.726290112239));
#41916=CARTESIAN_POINT('Ctrl Pts',(6.72086498424807,0.788836398442758,134.734463857373));
#41917=CARTESIAN_POINT('Ctrl Pts',(6.70066391069721,0.960949003971931,134.742585260235));
#41918=CARTESIAN_POINT('Ctrl Pts',(6.67384400370626,1.13231193478869,134.750706663097));
#41919=CARTESIAN_POINT('Ctrl Pts',(6.64048941823838,1.30237831917767,134.75882806596));
#41920=CARTESIAN_POINT('Ctrl Pts',(6.6071322539696,1.47245785220396,134.766950096726));
#41921=CARTESIAN_POINT('Ctrl Pts',(6.56723947525108,1.64124027997104,134.775072127492));
#41922=CARTESIAN_POINT('Ctrl Pts',(6.52094632601134,1.80818915306979,134.783194158258));
#41923=CARTESIAN_POINT('Ctrl Pts',(6.47464078234438,1.97518272469717,134.791318363599));
#41924=CARTESIAN_POINT('Ctrl Pts',(6.42193155378337,2.14034141163114,134.799442568941));
#41925=CARTESIAN_POINT('Ctrl Pts',(6.36300367972833,2.30314419256888,134.807566774282));
#41926=CARTESIAN_POINT('Ctrl Pts',(6.30343795221144,2.46770920095981,134.815778918524));
#41927=CARTESIAN_POINT('Ctrl Pts',(6.23751829741433,2.62986664224246,134.823991062767));
#41928=CARTESIAN_POINT('Ctrl Pts',(6.16548532028607,2.7891001712626,134.832203207009));
#41929=CARTESIAN_POINT('Ctrl Pts',(6.09410992484852,2.9468800736605,134.840340383426));
#41930=CARTESIAN_POINT('Ctrl Pts',(6.01673257818537,3.10178892693418,134.848477559842));
#41931=CARTESIAN_POINT('Ctrl Pts',(5.9336329117574,3.25335049887181,134.856614736258));
#41932=CARTESIAN_POINT('Ctrl Pts',(5.84938484918781,3.40700657650256,134.864864364414));
#41933=CARTESIAN_POINT('Ctrl Pts',(5.75925535132503,3.55722184325435,134.873113992569));
#41934=CARTESIAN_POINT('Ctrl Pts',(5.66358006671869,3.70353207463723,134.881363620725));
#41935=CARTESIAN_POINT('Ctrl Pts',(5.56790478211242,3.84984230602,134.88961324888));
#41936=CARTESIAN_POINT('Ctrl Pts',(5.46668398524656,3.99224722506152,134.897862877036));
#41937=CARTESIAN_POINT('Ctrl Pts',(5.36029402924288,4.13031922737978,134.906112505191));
#41938=CARTESIAN_POINT('Ctrl Pts',(5.2542144966466,4.26798836477511,134.914338062675));
#41939=CARTESIAN_POINT('Ctrl Pts',(5.14267895516024,4.40176148366843,134.922563620159));
#41940=CARTESIAN_POINT('Ctrl Pts',(5.0260033245659,4.53117860842546,134.930789177643));
#41941=CARTESIAN_POINT('Ctrl Pts',(4.90945576977456,4.66045367093616,134.939005705865));
#41942=CARTESIAN_POINT('Ctrl Pts',(4.78777959814272,4.7853819955667,134.947222234086));
#41943=CARTESIAN_POINT('Ctrl Pts',(4.66133283063708,4.90553414441536,134.955438762308));
#41944=CARTESIAN_POINT('Ctrl Pts',(4.53502820507165,5.02555122726039,134.963646054127));
#41945=CARTESIAN_POINT('Ctrl Pts',(4.40396392947557,5.14080258849623,134.971853345946));
#41946=CARTESIAN_POINT('Ctrl Pts',(4.26853673551919,5.25089355610292,134.980060637764));
#41947=CARTESIAN_POINT('Ctrl Pts',(4.1331977895448,5.3609127854904,134.988262581492));
#41948=CARTESIAN_POINT('Ctrl Pts',(3.99350186251409,5.46577809063417,134.99646452522));
#41949=CARTESIAN_POINT('Ctrl Pts',(3.84988120676472,5.56513285499995,135.004666468948));
#41950=CARTESIAN_POINT('Ctrl Pts',(3.70633385705389,5.66443690727178,135.012864226287));
#41951=CARTESIAN_POINT('Ctrl Pts',(3.55886606330543,5.75823581780362,135.021061983626));
#41952=CARTESIAN_POINT('Ctrl Pts',(3.40794169440871,5.8462143655113,135.029259740964));
#41953=CARTESIAN_POINT('Ctrl Pts',(3.3065303706811,5.90533020643143,135.034768098755));
#41954=CARTESIAN_POINT('Ctrl Pts',(3.20355908066341,5.96181902526415,135.040276456547));
#41955=CARTESIAN_POINT('Ctrl Pts',(3.09917575053244,6.01559628526647,135.045784814338));
#41956=CARTESIAN_POINT('Ctrl Pts',(3.09917575053245,6.01559628526646,133.045751582742));
#41957=CARTESIAN_POINT('Ctrl Pts',(2.93382384459245,6.10078395293769,133.054501030655));
#41958=CARTESIAN_POINT('Ctrl Pts',(2.76495772122957,6.17915010267061,133.063250478567));
#41959=CARTESIAN_POINT('Ctrl Pts',(2.59315093316678,6.25042856433191,133.07199992648));
#41960=CARTESIAN_POINT('Ctrl Pts',(2.42134553245588,6.32170645041462,133.08074930374));
#41961=CARTESIAN_POINT('Ctrl Pts',(2.24659977927565,6.38589665313466,133.089498681));
#41962=CARTESIAN_POINT('Ctrl Pts',(2.06950718689898,6.44278115439082,133.09824805826));
#41963=CARTESIAN_POINT('Ctrl Pts',(1.89241596572832,6.49966521519733,133.106997367774));
#41964=CARTESIAN_POINT('Ctrl Pts',(1.7129782145716,6.54924360009556,133.115746677289));
#41965=CARTESIAN_POINT('Ctrl Pts',(1.53180337335799,6.59134792173567,133.124495986804));
#41966=CARTESIAN_POINT('Ctrl Pts',(1.35062987477748,6.63345193135311,133.13324523148));
#41967=CARTESIAN_POINT('Ctrl Pts',(1.16771959102929,6.66808192368242,133.141994476156));
#41968=CARTESIAN_POINT('Ctrl Pts',(0.983693746906729,6.6951202836317,133.150743720832));
#41969=CARTESIAN_POINT('Ctrl Pts',(0.799669205419863,6.72215845218867,133.159492903576));
#41970=CARTESIAN_POINT('Ctrl Pts',(0.614529402873576,6.74160505424578,133.16824208632));
#41971=CARTESIAN_POINT('Ctrl Pts',(0.428903127363458,6.75339404354121,133.176991269065));
#41972=CARTESIAN_POINT('Ctrl Pts',(0.243278104164094,6.76518295330329,133.185740392783));
#41973=CARTESIAN_POINT('Ctrl Pts',(0.0571669005393355,6.76931433552276,
133.194489516502));
#41974=CARTESIAN_POINT('Ctrl Pts',(-0.12879840477729,6.76577415902473,133.20323864022));
#41975=CARTESIAN_POINT('Ctrl Pts',(-0.314762517258985,6.76223400523442,
133.21198770782));
#41976=CARTESIAN_POINT('Ctrl Pts',(-0.500580446819504,6.75102239665089,
133.220736775419));
#41977=CARTESIAN_POINT('Ctrl Pts',(-0.685621118842714,6.73217741012497,
133.229485843018));
#41978=CARTESIAN_POINT('Ctrl Pts',(-0.870660665414561,6.71333253821771,
133.238234857404));
#41979=CARTESIAN_POINT('Ctrl Pts',(-1.05492267885491,6.68685441030611,133.24698387179));
#41980=CARTESIAN_POINT('Ctrl Pts',(-1.23778137635253,6.65283295028177,133.255732886175));
#41981=CARTESIAN_POINT('Ctrl Pts',(-1.42999922978835,6.61707018861868,133.264929696543));
#41982=CARTESIAN_POINT('Ctrl Pts',(-1.6206660123367,6.57297172934419,133.27412650691));
#41983=CARTESIAN_POINT('Ctrl Pts',(-1.80906628500347,6.52070304311305,133.283323317278));
#41984=CARTESIAN_POINT('Ctrl Pts',(-1.98831342545479,6.47097374915045,133.292073315015));
#41985=CARTESIAN_POINT('Ctrl Pts',(-2.16550875896643,6.41384933989548,133.300823312753));
#41986=CARTESIAN_POINT('Ctrl Pts',(-2.34005036713943,6.34952386240501,133.309573310491));
#41987=CARTESIAN_POINT('Ctrl Pts',(-2.51458843547021,6.28519968948623,133.318323130772));
#41988=CARTESIAN_POINT('Ctrl Pts',(-2.68647261717989,6.21367483971128,133.327072951053));
#41989=CARTESIAN_POINT('Ctrl Pts',(-2.85511905908666,6.13519226743874,133.335822771333));
#41990=CARTESIAN_POINT('Ctrl Pts',(-3.02376230488826,6.05671118252966,133.344572425792));
#41991=CARTESIAN_POINT('Ctrl Pts',(-3.18916767379853,5.9712727599266,133.35332208025));
#41992=CARTESIAN_POINT('Ctrl Pts',(-3.35077334102743,5.87916720438021,133.362071734709));
#41993=CARTESIAN_POINT('Ctrl Pts',(-3.51237616037334,5.78706327195664,133.370821234977));
#41994=CARTESIAN_POINT('Ctrl Pts',(-3.67017916302276,5.68829258362314,133.379570735246));
#41995=CARTESIAN_POINT('Ctrl Pts',(-3.82364636566447,5.58319061741052,133.388320235514));
#41996=CARTESIAN_POINT('Ctrl Pts',(-3.9771110677879,5.47809036367708,133.397069593223));
#41997=CARTESIAN_POINT('Ctrl Pts',(-4.12623987481926,5.36665920043226,133.405818950931));
#41998=CARTESIAN_POINT('Ctrl Pts',(-4.27052628213935,5.2492755951233,133.41456830864));
#41999=CARTESIAN_POINT('Ctrl Pts',(-4.41481053024981,5.13189374643034,133.423317535416));
#42000=CARTESIAN_POINT('Ctrl Pts',(-4.5542523013653,5.00855981477353,133.432066762193));
#42001=CARTESIAN_POINT('Ctrl Pts',(-4.68837800630545,4.87969268192079,133.440815988969));
#42002=CARTESIAN_POINT('Ctrl Pts',(-4.8225018822888,4.75082730631824,133.44956509644));
#42003=CARTESIAN_POINT('Ctrl Pts',(-4.95130963052941,4.61642907903552,133.458314203911));
#42004=CARTESIAN_POINT('Ctrl Pts',(-5.07436379033332,4.47695444731729,133.467063311382));
#42005=CARTESIAN_POINT('Ctrl Pts',(-5.19741643562746,4.33748153220656,133.475812311171));
#42006=CARTESIAN_POINT('Ctrl Pts',(-5.31471544462691,4.19293255254692,133.484561310961));
#42007=CARTESIAN_POINT('Ctrl Pts',(-5.42586245275525,4.0437984177974,133.493310310751));
#42008=CARTESIAN_POINT('Ctrl Pts',(-5.53702160019049,3.89464799484491,133.502060266093));
#42009=CARTESIAN_POINT('Ctrl Pts',(-5.64202723081146,3.74091164444008,133.510810221435));
#42010=CARTESIAN_POINT('Ctrl Pts',(-5.74052265232861,3.58311159163402,133.519560176777));
#42011=CARTESIAN_POINT('Ctrl Pts',(-5.83901427066824,3.42531763191944,133.52830979426));
#42012=CARTESIAN_POINT('Ctrl Pts',(-5.93099603115656,3.26346052695765,133.537059411742));
#42013=CARTESIAN_POINT('Ctrl Pts',(-6.0161555062268,3.0980900446722,133.545809029225));
#42014=CARTESIAN_POINT('Ctrl Pts',(-6.10131214578732,2.93272506863969,133.554558355376));
#42015=CARTESIAN_POINT('Ctrl Pts',(-6.17964682328686,2.76384720417033,133.563307681527));
#42016=CARTESIAN_POINT('Ctrl Pts',(-6.25089348288508,2.59203002791729,133.572057007678));
#42017=CARTESIAN_POINT('Ctrl Pts',(-6.32213814889278,2.42021765937165,133.58080608901));
#42018=CARTESIAN_POINT('Ctrl Pts',(-6.38629508412537,2.24546640832054,133.589555170341));
#42019=CARTESIAN_POINT('Ctrl Pts',(-6.44314639819768,2.06836976660178,133.598304251673));
#42020=CARTESIAN_POINT('Ctrl Pts',(-6.50000285283659,1.89125711158416,133.607054124107));
#42021=CARTESIAN_POINT('Ctrl Pts',(-6.54955227673212,1.71179891440399,133.615803996542));
#42022=CARTESIAN_POINT('Ctrl Pts',(-6.59162635926351,1.53060476278579,133.624553868976));
#42023=CARTESIAN_POINT('Ctrl Pts',(-6.63369752055164,1.34942319164854,133.633303133898));
#42024=CARTESIAN_POINT('Ctrl Pts',(-6.66829431424224,1.16650618642873,133.642052398821));
#42025=CARTESIAN_POINT('Ctrl Pts',(-6.69529923745391,0.982474997620353,
133.650801663743));
#42026=CARTESIAN_POINT('Ctrl Pts',(-6.72230554731422,0.798434359179557,
133.659551377923));
#42027=CARTESIAN_POINT('Ctrl Pts',(-6.74171916496686,0.61327970624217,133.668301092103));
#42028=CARTESIAN_POINT('Ctrl Pts',(-6.75347414817263,0.427639953657228,
133.677050806282));
#42029=CARTESIAN_POINT('Ctrl Pts',(-6.76248837758727,0.285283364201958,
133.683760465458));
#42030=CARTESIAN_POINT('Ctrl Pts',(-6.76699999999983,0.142641701110043,
133.690470124634));
#42031=CARTESIAN_POINT('Ctrl Pts',(-6.767,8.02940689021197E-12,133.69717978381));
#42032=CARTESIAN_POINT('',(-6.76699974091591,0.00187255015161877,133.302820216163));
#42033=CARTESIAN_POINT('Ctrl Pts',(3.09917575053271,6.01559628526633,132.65155107452));
#42034=CARTESIAN_POINT('Ctrl Pts',(2.94514351274779,6.09495217178293,132.659674734604));
#42035=CARTESIAN_POINT('Ctrl Pts',(2.78800879566836,6.16841517401018,132.667798394687));
#42036=CARTESIAN_POINT('Ctrl Pts',(2.62826910112264,6.23574298156074,132.67592205477));
#42037=CARTESIAN_POINT('Ctrl Pts',(2.46854044018786,6.30306613861515,132.684045153733));
#42038=CARTESIAN_POINT('Ctrl Pts',(2.3062074966978,6.36425480178092,132.692168252695));
#42039=CARTESIAN_POINT('Ctrl Pts',(2.14178848258467,6.4191145102629,132.700291351658));
#42040=CARTESIAN_POINT('Ctrl Pts',(1.97734954609699,6.47398086600319,132.708415434882));
#42041=CARTESIAN_POINT('Ctrl Pts',(1.81082438261073,6.52251662403311,132.716539518107));
#42042=CARTESIAN_POINT('Ctrl Pts',(1.64274707558439,6.56457698908764,132.724663601331));
#42043=CARTESIAN_POINT('Ctrl Pts',(1.47461742592983,6.60665045257937,132.732790214558));
#42044=CARTESIAN_POINT('Ctrl Pts',(1.30493502492591,6.64224441901035,132.740916827784));
#42045=CARTESIAN_POINT('Ctrl Pts',(1.13424482946422,6.67126507244568,132.74904344101));
#42046=CARTESIAN_POINT('Ctrl Pts',(0.963371144075798,6.70031692273774,132.757178790249));
#42047=CARTESIAN_POINT('Ctrl Pts',(0.791487861200154,6.72278128436248,132.765314139487));
#42048=CARTESIAN_POINT('Ctrl Pts',(0.619146654162468,6.73861606122796,132.773449488726));
#42049=CARTESIAN_POINT('Ctrl Pts',(0.446707403851209,6.7544598463474,132.781589466087));
#42050=CARTESIAN_POINT('Ctrl Pts',(0.273810074801987,6.76366651217163,132.789729443449));
#42051=CARTESIAN_POINT('Ctrl Pts',(0.101006745760999,6.76624612597789,132.79786942081));
#42052=CARTESIAN_POINT('Ctrl Pts',(-0.072052076187581,6.76882955379071,
132.806021433278));
#42053=CARTESIAN_POINT('Ctrl Pts',(-0.245016255431909,6.76476636325331,
132.814173445746));
#42054=CARTESIAN_POINT('Ctrl Pts',(-0.417337295311639,6.75411863842663,
132.822325458214));
#42055=CARTESIAN_POINT('Ctrl Pts',(-0.553939800715431,6.7456779634563,132.828787729612));
#42056=CARTESIAN_POINT('Ctrl Pts',(-0.690138208722745,6.73310055831335,
132.83525000101));
#42057=CARTESIAN_POINT('Ctrl Pts',(-0.825664237599166,6.7164400962675,132.841712272407));
#42058=CARTESIAN_POINT('Ctrl Pts',(-0.998183374532949,6.6952320039409,132.849938481744));
#42059=CARTESIAN_POINT('Ctrl Pts',(-1.17012601879114,6.66734297938474,132.858164691081));
#42060=CARTESIAN_POINT('Ctrl Pts',(-1.34093539900288,6.63281096185479,132.866390900418));
#42061=CARTESIAN_POINT('Ctrl Pts',(-1.51155288219382,6.59831773956709,132.874607867961));
#42062=CARTESIAN_POINT('Ctrl Pts',(-1.68103928824092,6.55719645582258,132.882824835504));
#42063=CARTESIAN_POINT('Ctrl Pts',(-1.84884276455914,6.50953680625107,132.891041803048));
#42064=CARTESIAN_POINT('Ctrl Pts',(-2.01649140036118,6.46192113458098,132.899251188391));
#42065=CARTESIAN_POINT('Ctrl Pts',(-2.18245985631306,6.40777920993767,132.907460573734));
#42066=CARTESIAN_POINT('Ctrl Pts',(-2.34620618877694,6.34725180844,132.915669959078));
#42067=CARTESIAN_POINT('Ctrl Pts',(-2.50983427910421,6.2867681141153,132.923873416378));
#42068=CARTESIAN_POINT('Ctrl Pts',(-2.67124310701897,6.21990825107323,132.932076873679));
#42069=CARTESIAN_POINT('Ctrl Pts',(-2.82990553760095,6.14686291113243,132.940280330979));
#42070=CARTESIAN_POINT('Ctrl Pts',(-2.98848522445533,6.07385566492112,132.948479510111));
#42071=CARTESIAN_POINT('Ctrl Pts',(-3.14432104231472,5.99466951775266,132.956678689243));
#42072=CARTESIAN_POINT('Ctrl Pts',(-3.29690542633323,5.90954343497148,132.964877868375));
#42073=CARTESIAN_POINT('Ctrl Pts',(-3.44946106016427,5.82443339177951,132.973075502605));
#42074=CARTESIAN_POINT('Ctrl Pts',(-3.59876616457057,5.73338581144675,132.981273136835));
#42075=CARTESIAN_POINT('Ctrl Pts',(-3.74433713061009,5.63668594586701,132.989470771064));
#42076=CARTESIAN_POINT('Ctrl Pts',(-3.88989758917809,5.53999306018931,132.99766781358));
#42077=CARTESIAN_POINT('Ctrl Pts',(-4.0317241469153,5.43764889952437,133.005864856096));
#42078=CARTESIAN_POINT('Ctrl Pts',(-4.16936163849881,5.32998241342451,133.014061898611));
#42079=CARTESIAN_POINT('Ctrl Pts',(-4.30701421064042,5.22230413060646,133.022259839254));
#42080=CARTESIAN_POINT('Ctrl Pts',(-4.44047651962785,5.10930258158499,133.030457779897));
#42081=CARTESIAN_POINT('Ctrl Pts',(-4.56932595567727,4.99134744440557,133.03865572054));
#42082=CARTESIAN_POINT('Ctrl Pts',(-4.69821292765836,4.87335794498053,133.046856049375));
#42083=CARTESIAN_POINT('Ctrl Pts',(-4.82248408550876,4.75041222512862,133.055056378211));
#42084=CARTESIAN_POINT('Ctrl Pts',(-4.94175316984594,4.62291732657178,133.063256707047));
#42085=CARTESIAN_POINT('Ctrl Pts',(-5.06114653566438,4.49528957502179,133.071465580839));
#42086=CARTESIAN_POINT('Ctrl Pts',(-5.17552716924335,4.36310343651924,133.07967445463));
#42087=CARTESIAN_POINT('Ctrl Pts',(-5.28454802155997,4.2268003510725,133.087883328422));
#42088=CARTESIAN_POINT('Ctrl Pts',(-5.39362738416555,4.0904241132632,133.096096607825));
#42089=CARTESIAN_POINT('Ctrl Pts',(-5.49734101822078,3.94992681204619,133.104309887229));
#42090=CARTESIAN_POINT('Ctrl Pts',(-5.59538491806513,3.80577937073201,133.112523166632));
#42091=CARTESIAN_POINT('Ctrl Pts',(-5.69357222252262,3.66142109112916,133.120748459247));
#42092=CARTESIAN_POINT('Ctrl Pts',(-5.78607302992193,3.51340230612826,133.128973751863));
#42093=CARTESIAN_POINT('Ctrl Pts',(-5.87262841582157,3.36222017269617,133.137199044478));
#42094=CARTESIAN_POINT('Ctrl Pts',(-5.95090736495183,3.22549409367369,133.144637833591));
#42095=CARTESIAN_POINT('Ctrl Pts',(-6.02432405458796,3.08618118257169,133.152076622703));
#42096=CARTESIAN_POINT('Ctrl Pts',(-6.09272106997221,2.94466279283667,133.159515411815));
#42097=CARTESIAN_POINT('Ctrl Pts',(-6.17384614171449,2.77680913057368,133.168338491258));
#42098=CARTESIAN_POINT('Ctrl Pts',(-6.24811056664241,2.60543610680238,133.177161570701));
#42099=CARTESIAN_POINT('Ctrl Pts',(-6.3152199428182,2.43110799304172,133.185984650144));
#42100=CARTESIAN_POINT('Ctrl Pts',(-6.3822040503645,2.25710528602949,133.194791260129));
#42101=CARTESIAN_POINT('Ctrl Pts',(-6.44205964745616,2.08015874708851,133.203597870113));
#42102=CARTESIAN_POINT('Ctrl Pts',(-6.49453917221377,1.90085505512149,133.212404480098));
#42103=CARTESIAN_POINT('Ctrl Pts',(-6.5468758864848,1.7220392953073,133.221187124998));
#42104=CARTESIAN_POINT('Ctrl Pts',(-6.59187649572117,1.54087944384467,133.229969769898));
#42105=CARTESIAN_POINT('Ctrl Pts',(-6.62934246164935,1.35797920682642,133.238752414798));
#42106=CARTESIAN_POINT('Ctrl Pts',(-6.66674524472862,1.1753874139589,133.247520248589));
#42107=CARTESIAN_POINT('Ctrl Pts',(-6.69663866505402,0.991061356626386,
133.256288082379));
#42108=CARTESIAN_POINT('Ctrl Pts',(-6.71887386000849,0.805619670374654,
133.265055916169));
#42109=CARTESIAN_POINT('Ctrl Pts',(-6.74105530833422,0.620626231394264,
133.273802556464));
#42110=CARTESIAN_POINT('Ctrl Pts',(-6.75561542493228,0.434522816148734,
133.282549196759));
#42111=CARTESIAN_POINT('Ctrl Pts',(-6.76245635510104,0.24793758358425,133.291295837054));
#42112=CARTESIAN_POINT('Ctrl Pts',(-6.76546084101675,0.165990729941485,
133.295137296757));
#42113=CARTESIAN_POINT('Ctrl Pts',(-6.76697702831058,0.0839510964780675,
133.29897875646));
#42114=CARTESIAN_POINT('Ctrl Pts',(-6.76699974091591,0.0018725501516181,
133.302820216163));
#42115=CARTESIAN_POINT('Ctrl Pts',(-6.76699974091606,0.00187254958292456,
133.30282021619));
#42116=CARTESIAN_POINT('Ctrl Pts',(-6.76704976530886,-0.178905068379914,
133.311281013386));
#42117=CARTESIAN_POINT('Ctrl Pts',(-6.75985133561909,-0.35959956883799,
133.319741810583));
#42118=CARTESIAN_POINT('Ctrl Pts',(-6.74545066451291,-0.539614985542796,
133.328202607779));
#42119=CARTESIAN_POINT('Ctrl Pts',(-6.73103955054426,-0.719760943124762,
133.336669540449));
#42120=CARTESIAN_POINT('Ctrl Pts',(-6.70941580134513,-0.899226511591429,
133.345136473119));
#42121=CARTESIAN_POINT('Ctrl Pts',(-6.68067734035097,-1.07742251420748,
133.353603405789));
#42122=CARTESIAN_POINT('Ctrl Pts',(-6.6519146210961,-1.25576893284921,133.362077485434));
#42123=CARTESIAN_POINT('Ctrl Pts',(-6.61602526000546,-1.43284332815699,
133.370551565079));
#42124=CARTESIAN_POINT('Ctrl Pts',(-6.57315804405913,-1.60806788657095,
133.379025644724));
#42125=CARTESIAN_POINT('Ctrl Pts',(-6.53021695282447,-1.78359441852084,
133.387514328189));
#42126=CARTESIAN_POINT('Ctrl Pts',(-6.48027404540615,-1.95726442568419,
133.396003011653));
#42127=CARTESIAN_POINT('Ctrl Pts',(-6.42352818474407,-2.12851466046127,
133.404491695118));
#42128=CARTESIAN_POINT('Ctrl Pts',(-6.36673137777479,-2.29991864331735,
133.412987999703));
#42129=CARTESIAN_POINT('Ctrl Pts',(-6.30311954325868,-2.46889821573112,
133.421484304289));
#42130=CARTESIAN_POINT('Ctrl Pts',(-6.23293949359794,-2.6349106757435,133.429980608874));
#42131=CARTESIAN_POINT('Ctrl Pts',(-6.16262828771194,-2.80123338870822,
133.438492791808));
#42132=CARTESIAN_POINT('Ctrl Pts',(-6.08572446155392,-2.9645776087454,133.447004974741));
#42133=CARTESIAN_POINT('Ctrl Pts',(-6.0025214309379,-3.12442402230095,133.455517157674));
#42134=CARTESIAN_POINT('Ctrl Pts',(-5.93148826083242,-3.26089017504536,
133.462784288857));
#42135=CARTESIAN_POINT('Ctrl Pts',(-5.85586467189241,-3.39480726791467,
133.47005142004));
#42136=CARTESIAN_POINT('Ctrl Pts',(-5.77585773945136,-3.52586959112499,
133.477318551222));
#42137=CARTESIAN_POINT('Ctrl Pts',(-5.68610278694159,-3.67290050752998,
133.485471107435));
#42138=CARTESIAN_POINT('Ctrl Pts',(-5.59058952644183,-3.81673194255564,
133.493623663649));
#42139=CARTESIAN_POINT('Ctrl Pts',(-5.48957310309481,-3.95687706983399,
133.501776219862));
#42140=CARTESIAN_POINT('Ctrl Pts',(-5.38867370970947,-4.09685983560386,
133.509919331142));
#42141=CARTESIAN_POINT('Ctrl Pts',(-5.28228405618291,-4.23316450129326,
133.518062442423));
#42142=CARTESIAN_POINT('Ctrl Pts',(-5.17070470433181,-4.36532952485845,
133.526205553703));
#42143=CARTESIAN_POINT('Ctrl Pts',(-5.05923116168047,-4.49736921810807,
133.53434094298));
#42144=CARTESIAN_POINT('Ctrl Pts',(-4.94257795262434,-4.62527680712845,
133.542476332258));
#42145=CARTESIAN_POINT('Ctrl Pts',(-4.82108838239013,-4.74862041114921,
133.550611721535));
#42146=CARTESIAN_POINT('Ctrl Pts',(-4.69968849119311,-4.8718729675547,133.558741105574));
#42147=CARTESIAN_POINT('Ctrl Pts',(-4.57345960279974,-4.99056798781283,
133.566870489612));
#42148=CARTESIAN_POINT('Ctrl Pts',(-4.44278466535951,-5.10430733961489,
133.574999873651));
#42149=CARTESIAN_POINT('Ctrl Pts',(-4.31217873926266,-5.21798662400374,
133.583124964443));
#42150=CARTESIAN_POINT('Ctrl Pts',(-4.17713171543183,-5.32671521265316,
133.591250055235));
#42151=CARTESIAN_POINT('Ctrl Pts',(-4.03806268885521,-5.43013247728593,
133.599375146027));
#42152=CARTESIAN_POINT('Ctrl Pts',(-3.89846280565517,-5.53394450803778,
133.607531252052));
#42153=CARTESIAN_POINT('Ctrl Pts',(-3.75481042015292,-5.63240432611419,
133.615687358077));
#42154=CARTESIAN_POINT('Ctrl Pts',(-3.60756260607739,-5.72518829762237,
133.623843464102));
#42155=CARTESIAN_POINT('Ctrl Pts',(-3.46090743782367,-5.81759883042525,
133.631966743276));
#42156=CARTESIAN_POINT('Ctrl Pts',(-3.31068605227303,-5.9043789422125,133.640090022449));
#42157=CARTESIAN_POINT('Ctrl Pts',(-3.15737835205038,-5.98525278847967,
133.648213301623));
#42158=CARTESIAN_POINT('Ctrl Pts',(-3.00405023761226,-6.06613740378271,
133.656337662479));
#42159=CARTESIAN_POINT('Ctrl Pts',(-2.84763531352529,-6.14111401635927,
133.664462023336));
#42160=CARTESIAN_POINT('Ctrl Pts',(-2.68863718791606,-6.20995322621313,
133.672586384193));
#42161=CARTESIAN_POINT('Ctrl Pts',(-2.52958764015158,-6.27881469960325,
133.680713372578));
#42162=CARTESIAN_POINT('Ctrl Pts',(-2.36795356277147,-6.34153467239499,
133.688840360963));
#42163=CARTESIAN_POINT('Ctrl Pts',(-2.20425754950671,-6.39793229531563,
133.696967349349));
#42164=CARTESIAN_POINT('Ctrl Pts',(-2.03950326015197,-6.45469452244793,
133.705146877789));
#42165=CARTESIAN_POINT('Ctrl Pts',(-1.87266063744718,-6.50505224733347,
133.713326406229));
#42166=CARTESIAN_POINT('Ctrl Pts',(-1.70427601599646,-6.54887259467607,
133.721505934669));
#42167=CARTESIAN_POINT('Ctrl Pts',(-1.53668437201362,-6.5924865778758,133.729646943073));
#42168=CARTESIAN_POINT('Ctrl Pts',(-1.36756559221563,-6.62962460870949,
133.737787951476));
#42169=CARTESIAN_POINT('Ctrl Pts',(-1.19746623968315,-6.66020747460761,
133.74592895988));
#42170=CARTESIAN_POINT('Ctrl Pts',(-1.02615962271941,-6.69100739956948,
133.754127748338));
#42171=CARTESIAN_POINT('Ctrl Pts',(-0.853858836676677,-6.71515871580873,
133.762326536797));
#42172=CARTESIAN_POINT('Ctrl Pts',(-0.681124613291064,-6.7326338279435,
133.770525325255));
#42173=CARTESIAN_POINT('Ctrl Pts',(-0.508390389905324,-6.75010894007828,
133.778724113713));
#42174=CARTESIAN_POINT('Ctrl Pts',(-0.335223103855506,-6.7609078896523,
133.786922902172));
#42175=CARTESIAN_POINT('Ctrl Pts',(-0.16218029837062,-6.76505628585753,
133.79512169063));
#42176=CARTESIAN_POINT('Ctrl Pts',(0.0115856305573594,-6.76922201767252,
133.803354740762));
#42177=CARTESIAN_POINT('Ctrl Pts',(0.185766191311162,-6.76669456557975,
133.811587790894));
#42178=CARTESIAN_POINT('Ctrl Pts',(0.359805115405753,-6.75742771170568,
133.819820841026));
#42179=CARTESIAN_POINT('Ctrl Pts',(0.533636785894009,-6.74817189323013,
133.828044086861));
#42180=CARTESIAN_POINT('Ctrl Pts',(0.707326801414873,-6.73219267276864,
133.836267332696));
#42181=CARTESIAN_POINT('Ctrl Pts',(0.880315921941427,-6.70949572453671,
133.844490578531));
#42182=CARTESIAN_POINT('Ctrl Pts',(1.05313366316287,-6.68682126203801,133.852705677644));
#42183=CARTESIAN_POINT('Ctrl Pts',(1.22525153954443,-6.65744237198378,133.860920776758));
#42184=CARTESIAN_POINT('Ctrl Pts',(1.39611236930303,-6.62141671036336,133.869135875871));
#42185=CARTESIAN_POINT('Ctrl Pts',(1.56683811405107,-6.58541953114518,133.87734448001));
#42186=CARTESIAN_POINT('Ctrl Pts',(1.73630844280544,-6.54278612089831,133.885553084149));
#42187=CARTESIAN_POINT('Ctrl Pts',(1.90397324675609,-6.49362571108292,133.893761688288));
#42188=CARTESIAN_POINT('Ctrl Pts',(2.07153903015424,-6.44449433473683,133.901965444537));
#42189=CARTESIAN_POINT('Ctrl Pts',(2.23730107020929,-6.38884373853091,133.910169200786));
#42190=CARTESIAN_POINT('Ctrl Pts',(2.40072128168432,-6.32683383120404,133.918372957035));
#42191=CARTESIAN_POINT('Ctrl Pts',(2.56409314123769,-6.26484227104583,133.926574285999));
#42192=CARTESIAN_POINT('Ctrl Pts',(2.72512421659101,-6.19649527106696,133.934775614963));
#42193=CARTESIAN_POINT('Ctrl Pts',(2.88329313691535,-6.12200209789386,133.942976943928));
#42194=CARTESIAN_POINT('Ctrl Pts',(3.04144024423566,-6.04751919804047,133.95117714185));
#42195=CARTESIAN_POINT('Ctrl Pts',(3.19672565830619,-5.96689196502827,133.959377339773));
#42196=CARTESIAN_POINT('Ctrl Pts',(3.34864947854664,-5.88037717071187,133.967577537696));
#42197=CARTESIAN_POINT('Ctrl Pts',(3.50057987872931,-5.7938586293705,133.975778090776));
#42198=CARTESIAN_POINT('Ctrl Pts',(3.64914808363584,-5.70145219596756,133.983978643855));
#42199=CARTESIAN_POINT('Ctrl Pts',(3.79388017451233,-5.60345984383241,133.992179196935));
#42200=CARTESIAN_POINT('Ctrl Pts',(3.93864476214154,-5.50544548943627,134.000381591288));
#42201=CARTESIAN_POINT('Ctrl Pts',(4.07957122360723,-5.40184291910736,134.008583985642));
#42202=CARTESIAN_POINT('Ctrl Pts',(4.21621588135013,-5.29299656544862,134.016786379995));
#42203=CARTESIAN_POINT('Ctrl Pts',(4.35298832586857,-5.1840484213153,134.024996445029));
#42204=CARTESIAN_POINT('Ctrl Pts',(4.48547068592351,-5.06984691987039,134.033206510063));
#42205=CARTESIAN_POINT('Ctrl Pts',(4.61325284863728,-4.95077641936495,134.041416575096));
#42206=CARTESIAN_POINT('Ctrl Pts',(4.74109616562688,-4.83164893383064,134.049630569322));
#42207=CARTESIAN_POINT('Ctrl Pts',(4.86423454795761,-4.70764805725219,134.057844563547));
#42208=CARTESIAN_POINT('Ctrl Pts',(4.98229591798076,-4.57919385762082,134.066058557772));
#42209=CARTESIAN_POINT('Ctrl Pts',(5.10051824497317,-4.45056453213196,134.074283750407));
#42210=CARTESIAN_POINT('Ctrl Pts',(5.21364949452321,-4.31747002295741,134.082508943043));
#42211=CARTESIAN_POINT('Ctrl Pts',(5.32135817489546,-4.18036316298875,134.090734135678));
#42212=CARTESIAN_POINT('Ctrl Pts',(5.41822036046025,-4.05706325747888,134.098131033798));
#42213=CARTESIAN_POINT('Ctrl Pts',(5.51069757661604,-3.93051897913587,134.105527931918));
#42214=CARTESIAN_POINT('Ctrl Pts',(5.59857970815348,-3.80107803806395,134.112924830037));
#42215=CARTESIAN_POINT('Ctrl Pts',(5.70130195092437,-3.64977920699706,134.121570796528));
#42216=CARTESIAN_POINT('Ctrl Pts',(5.79797894980601,-3.49417916443688,134.130216763019));
#42217=CARTESIAN_POINT('Ctrl Pts',(5.88825544569583,-3.33477687502978,134.13886272951));
#42218=CARTESIAN_POINT('Ctrl Pts',(5.97841646567461,-3.17557848282107,134.147497636634));
#42219=CARTESIAN_POINT('Ctrl Pts',(6.06219315868862,-3.01258780613254,134.156132543759));
#42220=CARTESIAN_POINT('Ctrl Pts',(6.13927355357156,-2.84633259378043,134.164767450883));
#42221=CARTESIAN_POINT('Ctrl Pts',(6.21891295535231,-2.67455784256438,134.173689029955));
#42222=CARTESIAN_POINT('Ctrl Pts',(6.29140359053872,-2.49929831964581,134.182610609026));
#42223=CARTESIAN_POINT('Ctrl Pts',(6.35645150764813,-2.32116635140997,134.191532188098));
#42224=CARTESIAN_POINT('Ctrl Pts',(6.41923539892832,-2.14923435690143,134.200143247074));
#42225=CARTESIAN_POINT('Ctrl Pts',(6.47508577903036,-1.97462681126812,134.208754306049));
#42226=CARTESIAN_POINT('Ctrl Pts',(6.52378584774984,-1.7979174654858,134.217365365025));
#42227=CARTESIAN_POINT('Ctrl Pts',(6.57243999005592,-1.62137476477566,134.225968303375));
#42228=CARTESIAN_POINT('Ctrl Pts',(6.61395718414473,-1.44273450872252,134.234571241724));
#42229=CARTESIAN_POINT('Ctrl Pts',(6.64816983304999,-1.2625873716001,134.243174180074));
#42230=CARTESIAN_POINT('Ctrl Pts',(6.68234417170306,-1.08264195759693,134.251767485122));
#42231=CARTESIAN_POINT('Ctrl Pts',(6.70923022607123,-0.901193327721689,
134.260360790171));
#42232=CARTESIAN_POINT('Ctrl Pts',(6.72871100294165,-0.718844377380814,
134.26895409522));
#42233=CARTESIAN_POINT('Ctrl Pts',(6.7308814803534,-0.698527719559418,134.269911530061));
#42234=CARTESIAN_POINT('Ctrl Pts',(6.73296008349514,-0.67819989735964,134.270868964901));
#42235=CARTESIAN_POINT('Ctrl Pts',(6.73494668975532,-0.657861753071142,
134.271826399742));
#42236=CARTESIAN_POINT('Ctrl Pts',(6.7527822489269,-0.475267857557712,134.28042215729));
#42237=CARTESIAN_POINT('Ctrl Pts',(6.76317747172217,-0.292055383205121,
134.289017914837));
#42238=CARTESIAN_POINT('Ctrl Pts',(6.76612466864008,-0.108839186050769,
134.297613672385));
#42239=CARTESIAN_POINT('Ctrl Pts',(6.76907461539293,0.0745479580457943,
134.306217450066));
#42240=CARTESIAN_POINT('Ctrl Pts',(6.76456266037914,0.257938526612442,134.314821227748));
#42241=CARTESIAN_POINT('Ctrl Pts',(6.75263320084626,0.440719700976544,134.32342500543));
#42242=CARTESIAN_POINT('Ctrl Pts',(6.74023490312219,0.63068433532344,134.332366919098));
#42243=CARTESIAN_POINT('Ctrl Pts',(6.7198243193483,0.819990332411676,134.341308832766));
#42244=CARTESIAN_POINT('Ctrl Pts',(6.6915100729088,1.00795929687667,134.350250746434));
#42245=CARTESIAN_POINT('Ctrl Pts',(6.66419234854404,1.18931267922269,134.358877948764));
#42246=CARTESIAN_POINT('Ctrl Pts',(6.6295179237513,1.36942125684008,134.367505151095));
#42247=CARTESIAN_POINT('Ctrl Pts',(6.58763598010825,1.54768898477156,134.376132353426));
#42248=CARTESIAN_POINT('Ctrl Pts',(6.54571415032432,1.72612648542832,134.384767771846));
#42249=CARTESIAN_POINT('Ctrl Pts',(6.49657117916455,1.90271934256209,134.393403190267));
#42250=CARTESIAN_POINT('Ctrl Pts',(6.44040592710666,2.0768872126549,134.402038608687));
#42251=CARTESIAN_POINT('Ctrl Pts',(6.38415769888914,2.25131239096695,134.410686784708));
#42252=CARTESIAN_POINT('Ctrl Pts',(6.32086655941959,2.4233051354262,134.41933496073));
#42253=CARTESIAN_POINT('Ctrl Pts',(6.25077978429076,2.59230420442933,134.427983136751));
#42254=CARTESIAN_POINT('Ctrl Pts',(6.24336486923098,2.6101836651341,134.428898080982));
#42255=CARTESIAN_POINT('Ctrl Pts',(6.23587393435357,2.62802964033025,134.429813025214));
#42256=CARTESIAN_POINT('Ctrl Pts',(6.22830730251598,2.64584148153779,134.430727969446));
#42257=CARTESIAN_POINT('Ctrl Pts',(6.16026405941084,2.80601518463973,134.438955642487));
#42258=CARTESIAN_POINT('Ctrl Pts',(6.08594872974335,2.96377266448755,134.447183315528));
#42259=CARTESIAN_POINT('Ctrl Pts',(6.00555492202109,3.11858927699501,134.455410988569));
#42260=CARTESIAN_POINT('Ctrl Pts',(5.92527093089928,3.27319441259199,134.463627422746));
#42261=CARTESIAN_POINT('Ctrl Pts',(5.83892517462812,3.42486637195514,134.471843856923));
#42262=CARTESIAN_POINT('Ctrl Pts',(5.74675932745894,3.57310036694517,134.480060291099));
#42263=CARTESIAN_POINT('Ctrl Pts',(5.65466644834513,3.72121700451175,134.488270220294));
#42264=CARTESIAN_POINT('Ctrl Pts',(5.55676284076521,3.86590079466694,134.496480149488));
#42265=CARTESIAN_POINT('Ctrl Pts',(5.45333641300495,4.00667080836377,134.504690078683));
#42266=CARTESIAN_POINT('Ctrl Pts',(5.34997312202254,4.14735488884917,134.512894996117));
#42267=CARTESIAN_POINT('Ctrl Pts',(5.24109393611688,4.2841296630918,134.52109991355));
#42268=CARTESIAN_POINT('Ctrl Pts',(5.12703049513253,4.41654246011302,134.529304830984));
#42269=CARTESIAN_POINT('Ctrl Pts',(5.01301601183697,4.54889842363479,134.537506226748));
#42270=CARTESIAN_POINT('Ctrl Pts',(4.89382193916935,4.67689586840449,134.545707622512));
#42271=CARTESIAN_POINT('Ctrl Pts',(4.76982071906617,4.80011450988069,134.553909018276));
#42272=CARTESIAN_POINT('Ctrl Pts',(4.64582916844672,4.92332354289779,134.562109774504));
#42273=CARTESIAN_POINT('Ctrl Pts',(4.51703146484481,5.04175425634369,134.570310530732));
#42274=CARTESIAN_POINT('Ctrl Pts',(4.38383773760777,5.15502237534679,134.57851128696));
#42275=CARTESIAN_POINT('Ctrl Pts',(4.25065495043721,5.2682811909031,134.586711369606));
#42276=CARTESIAN_POINT('Ctrl Pts',(4.11307713424406,5.3763780274387,134.594911452253));
#42277=CARTESIAN_POINT('Ctrl Pts',(3.97154820464094,5.47896832060684,134.603111534899));
#42278=CARTESIAN_POINT('Ctrl Pts',(3.82995342251291,5.58160634839613,134.611315432993));
#42279=CARTESIAN_POINT('Ctrl Pts',(3.6844041436477,5.67873250239356,134.619519331086));
#42280=CARTESIAN_POINT('Ctrl Pts',(3.53537457188812,5.77004468236138,134.62772322918));
#42281=CARTESIAN_POINT('Ctrl Pts',(3.39300572892145,5.85727575507597,134.635560462191));
#42282=CARTESIAN_POINT('Ctrl Pts',(3.24746117470512,5.93920110032378,134.643397695202));
#42283=CARTESIAN_POINT('Ctrl Pts',(3.09917575053266,6.01559628526635,134.651234928213));
#42284=CARTESIAN_POINT('Origin',(0.,0.,-3.69717978381041));
#42285=CARTESIAN_POINT('',(3.09917575053248,6.01559628526645,137.045751582742));
#42286=CARTESIAN_POINT('',(3.0991757505325,6.01559628526643,136.651412426306));
#42287=CARTESIAN_POINT('',(3.09917575053259,6.01559628526639,-3.69717978381041));
#42288=CARTESIAN_POINT('',(-6.76699999982859,-4.81653644018645E-5,135.697182049439));
#42289=CARTESIAN_POINT('Ctrl Pts',(-6.76699999982859,-4.81653644018645E-5,
135.697182049439));
#42290=CARTESIAN_POINT('Ctrl Pts',(-6.76699867588785,-0.186055414706891,
135.705931561242));
#42291=CARTESIAN_POINT('Ctrl Pts',(-6.75932372490837,-0.372062466127105,
135.714681073045));
#42292=CARTESIAN_POINT('Ctrl Pts',(-6.74400121519305,-0.55743753863076,
135.723430584848));
#42293=CARTESIAN_POINT('Ctrl Pts',(-6.72867877019546,-0.742811828165125,
135.732180059695));
#42294=CARTESIAN_POINT('Ctrl Pts',(-6.70570885470968,-0.927553858495178,
135.740929534542));
#42295=CARTESIAN_POINT('Ctrl Pts',(-6.67516948638864,-1.11103615062068,
135.74967900939));
#42296=CARTESIAN_POINT('Ctrl Pts',(-6.64463024452037,-1.29451768301062,
135.758428448009));
#42297=CARTESIAN_POINT('Ctrl Pts',(-6.60652165959189,-1.47673920492593,
135.767177886628));
#42298=CARTESIAN_POINT('Ctrl Pts',(-6.56097316689686,-1.65708180343017,
135.775927325246));
#42299=CARTESIAN_POINT('Ctrl Pts',(-6.51542485901923,-1.83742367017695,
135.784676728364));
#42300=CARTESIAN_POINT('Ctrl Pts',(-6.46243677396501,-2.01588635090299,
135.793426131481));
#42301=CARTESIAN_POINT('Ctrl Pts',(-6.40218888358992,-2.19186370443913,
135.802175534598));
#42302=CARTESIAN_POINT('Ctrl Pts',(-6.34194123267288,-2.3678403585451,135.81092490294));
#42303=CARTESIAN_POINT('Ctrl Pts',(-6.27443392700289,-2.54133143409247,
135.819674271283));
#42304=CARTESIAN_POINT('Ctrl Pts',(-6.19989625055173,-2.71174768044421,
135.828423639625));
#42305=CARTESIAN_POINT('Ctrl Pts',(-6.12535886416388,-2.8821632636213,135.837172973919));
#42306=CARTESIAN_POINT('Ctrl Pts',(-6.04379127658468,-3.04950377898405,
135.845922308213));
#42307=CARTESIAN_POINT('Ctrl Pts',(-5.95547052442305,-3.21320087027379,
135.854671642507));
#42308=CARTESIAN_POINT('Ctrl Pts',(-5.86715010862682,-3.3768973381309,135.86342094348));
#42309=CARTESIAN_POINT('Ctrl Pts',(-5.77207671579077,-3.53695015747485,
135.872170244453));
#42310=CARTESIAN_POINT('Ctrl Pts',(-5.67057325125895,-3.69281572815468,
135.880919545426));
#42311=CARTESIAN_POINT('Ctrl Pts',(-5.56907016486904,-3.84868071817152,
135.889668813803));
#42312=CARTESIAN_POINT('Ctrl Pts',(-5.46113721110327,-4.00035825060242,
135.898418082181));
#42313=CARTESIAN_POINT('Ctrl Pts',(-5.34714096852922,-4.1473331747855,135.907167350559));
#42314=CARTESIAN_POINT('Ctrl Pts',(-5.2331451411717,-4.29430756363148,135.915916587069));
#42315=CARTESIAN_POINT('Ctrl Pts',(-5.11308624482862,-4.4365791520693,135.924665823579));
#42316=CARTESIAN_POINT('Ctrl Pts',(-4.98737203909913,-4.57366473887322,
135.933415060089));
#42317=CARTESIAN_POINT('Ctrl Pts',(-4.86165828082827,-4.71074983774398,
135.942164265458));
#42318=CARTESIAN_POINT('Ctrl Pts',(-4.7302894471308,-4.84264876072114,135.950913470826));
#42319=CARTESIAN_POINT('Ctrl Pts',(-4.59371170670946,-4.96891353875679,
135.959662676195));
#42320=CARTESIAN_POINT('Ctrl Pts',(-4.45713444107297,-5.09517787785851,
135.968411851148));
#42321=CARTESIAN_POINT('Ctrl Pts',(-4.31534851536104,-5.21580791668835,
135.977161026102));
#42322=CARTESIAN_POINT('Ctrl Pts',(-4.16883547455953,-5.33039396161804,
135.985910201056));
#42323=CARTESIAN_POINT('Ctrl Pts',(-4.02232293091532,-5.44497961772713,
135.994659346321));
#42324=CARTESIAN_POINT('Ctrl Pts',(-3.87108352999623,-5.55352114444728,
136.003408491586));
#42325=CARTESIAN_POINT('Ctrl Pts',(-3.71563091997335,-5.65564990664539,
136.012157636852));
#42326=CARTESIAN_POINT('Ctrl Pts',(-3.56017882453426,-5.75777833077388,
136.020906753155));
#42327=CARTESIAN_POINT('Ctrl Pts',(-3.40051378738538,-5.85349387552368,
136.029655869459));
#42328=CARTESIAN_POINT('Ctrl Pts',(-3.23717806875404,-5.94247146826789,
136.038404985763));
#42329=CARTESIAN_POINT('Ctrl Pts',(-3.07384287723976,-6.03144877386358,
136.047154073831));
#42330=CARTESIAN_POINT('Ctrl Pts',(-2.9068372795745,-6.11368803389362,136.0559031619));
#42331=CARTESIAN_POINT('Ctrl Pts',(-2.73672846260799,-6.18890994618207,
136.064652249968));
#42332=CARTESIAN_POINT('Ctrl Pts',(-2.56662018049375,-6.26413162195949,
136.073401310528));
#42333=CARTESIAN_POINT('Ctrl Pts',(-2.39340896066045,-6.33233587826648,
136.082150371088));
#42334=CARTESIAN_POINT('Ctrl Pts',(-2.21768306188705,-6.39329108026682,
136.090899431648));
#42335=CARTESIAN_POINT('Ctrl Pts',(-2.04195770103624,-6.4542460956744,136.099648465426));
#42336=CARTESIAN_POINT('Ctrl Pts',(-1.86371794735658,-6.50795200727928,
136.108397499203));
#42337=CARTESIAN_POINT('Ctrl Pts',(-1.68356913379756,-6.55422642054149,
136.117146532981));
#42338=CARTESIAN_POINT('Ctrl Pts',(-1.50342085674391,-6.6005006959928,136.125895540703));
#42339=CARTESIAN_POINT('Ctrl Pts',(-1.32136380870533,-6.63934344610502,
136.134644548425));
#42340=CARTESIAN_POINT('Ctrl Pts',(-1.13801628314245,-6.67062275498343,
136.143393556147));
#42341=CARTESIAN_POINT('Ctrl Pts',(-0.95466928838962,-6.701901973305,136.15214253854));
#42342=CARTESIAN_POINT('Ctrl Pts',(-0.770032106030325,-6.72561774602647,
136.160891520933));
#42343=CARTESIAN_POINT('Ctrl Pts',(-0.584731788427198,-6.7416895312379,
136.169640503325));
#42344=CARTESIAN_POINT('Ctrl Pts',(-0.391443045919639,-6.75845418223015,
136.178766660403));
#42345=CARTESIAN_POINT('Ctrl Pts',(-0.197433054891392,-6.76690112092229,
136.18789281748));
#42346=CARTESIAN_POINT('Ctrl Pts',(-0.00341866909486969,-6.76699913644901,
136.197018974557));
#42347=CARTESIAN_POINT('Ctrl Pts',(0.1845327671456,-6.76709408899052,136.205859939226));
#42348=CARTESIAN_POINT('Ctrl Pts',(0.372488010641898,-6.75935406923834,
136.214700903894));
#42349=CARTESIAN_POINT('Ctrl Pts',(0.559795261984329,-6.74380591837131,
136.223541868563));
#42350=CARTESIAN_POINT('Ctrl Pts',(0.745174855785072,-6.72841778005085,
136.232291847153));
#42351=CARTESIAN_POINT('Ctrl Pts',(0.929919443623088,-6.70538151166438,
136.241041825744));
#42352=CARTESIAN_POINT('Ctrl Pts',(1.11340146562901,-6.67477536523404,136.249791804334));
#42353=CARTESIAN_POINT('Ctrl Pts',(1.29688160934916,-6.64416953211554,136.258541693352));
#42354=CARTESIAN_POINT('Ctrl Pts',(1.47909893033434,-6.60599402319168,136.26729158237));
#42355=CARTESIAN_POINT('Ctrl Pts',(1.65943446626114,-6.56037851439874,136.276041471387));
#42356=CARTESIAN_POINT('Ctrl Pts',(1.8397682160447,-6.51476345740711,136.284791273742));
#42357=CARTESIAN_POINT('Ctrl Pts',(2.01821994016055,-6.46170861830474,136.293541076096));
#42358=CARTESIAN_POINT('Ctrl Pts',(2.19418347939502,-6.40139421210333,136.30229087845));
#42359=CARTESIAN_POINT('Ctrl Pts',(2.37014533426395,-6.34108038324599,136.311040597048));
#42360=CARTESIAN_POINT('Ctrl Pts',(2.54361878075444,-6.27350721929238,136.319790315647));
#42361=CARTESIAN_POINT('Ctrl Pts',(2.71401458097926,-6.19890424625449,136.328540034246));
#42362=CARTESIAN_POINT('Ctrl Pts',(2.88440880675507,-6.12430196254449,136.337289671998));
#42363=CARTESIAN_POINT('Ctrl Pts',(3.05172518060253,-6.04267011469176,136.34603930975));
#42364=CARTESIAN_POINT('Ctrl Pts',(3.21539538887731,-5.95428597677224,136.354788947502));
#42365=CARTESIAN_POINT('Ctrl Pts',(3.37906413922919,-5.86590262615091,136.363538507314));
#42366=CARTESIAN_POINT('Ctrl Pts',(3.53908653680616,-5.77076724201437,136.372288067127));
#42367=CARTESIAN_POINT('Ctrl Pts',(3.69491905265573,-5.66920295935167,136.38103762694));
#42368=CARTESIAN_POINT('Ctrl Pts',(3.85075023217284,-5.56763954764742,136.389787111722));
#42369=CARTESIAN_POINT('Ctrl Pts',(4.00239136175179,-5.45964750423334,136.398536596503));
#42370=CARTESIAN_POINT('Ctrl Pts',(4.14932738891612,-5.34559362649188,136.407286081285));
#42371=CARTESIAN_POINT('Ctrl Pts',(4.29626220485472,-5.2315406889214,136.416035493942));
#42372=CARTESIAN_POINT('Ctrl Pts',(4.43849176959685,-5.11142619274938,136.4247849066));
#42373=CARTESIAN_POINT('Ctrl Pts',(4.57553300521195,-4.98565810282014,136.433534319257));
#42374=CARTESIAN_POINT('Ctrl Pts',(4.71257315669189,-4.85989100784405,136.442283662698));
#42375=CARTESIAN_POINT('Ctrl Pts',(4.84442485003742,-4.72847060238681,136.451033006139));
#42376=CARTESIAN_POINT('Ctrl Pts',(4.97064026248733,-4.591843244378,136.45978234958));
#42377=CARTESIAN_POINT('Ctrl Pts',(5.0968547183719,-4.45521692184491,136.468531626711));
#42378=CARTESIAN_POINT('Ctrl Pts',(5.21743278438389,-4.31338393622911,136.477280903842));
#42379=CARTESIAN_POINT('Ctrl Pts',(5.33196493385394,-4.16682600358497,136.486030180973));
#42380=CARTESIAN_POINT('Ctrl Pts',(5.44649625334771,-4.02026913299729,136.494779394701));
#42381=CARTESIAN_POINT('Ctrl Pts',(5.55498156752181,-3.86898760969255,136.503528608429));
#42382=CARTESIAN_POINT('Ctrl Pts',(5.65705242639514,-3.71349523293311,136.512277822157));
#42383=CARTESIAN_POINT('Ctrl Pts',(5.75912257949751,-3.55800393132876,136.521026975388));
#42384=CARTESIAN_POINT('Ctrl Pts',(5.85477820880497,-3.39830207408514,136.529776128619));
#42385=CARTESIAN_POINT('Ctrl Pts',(5.94369444243805,-3.23493205105318,136.538525281851));
#42386=CARTESIAN_POINT('Ctrl Pts',(6.03261009078973,-3.07156310338652,136.547274377492));
#42387=CARTESIAN_POINT('Ctrl Pts',(6.11478629525939,-2.90452628992948,136.556023473133));
#42388=CARTESIAN_POINT('Ctrl Pts',(6.18994396733866,-2.73438890452834,136.564772568774));
#42389=CARTESIAN_POINT('Ctrl Pts',(6.26510116966157,-2.56425258253322,136.57352160973));
#42390=CARTESIAN_POINT('Ctrl Pts',(6.33323981159752,-2.39101598947377,136.582270650687));
#42391=CARTESIAN_POINT('Ctrl Pts',(6.39412848218535,-2.21526746766753,136.591019691644));
#42392=CARTESIAN_POINT('Ctrl Pts',(6.4550167924232,-2.03951998597227,136.599768680822));
#42393=CARTESIAN_POINT('Ctrl Pts',(6.5086551233768,-1.86126087601571,136.608517670001));
#42394=CARTESIAN_POINT('Ctrl Pts',(6.55486131187705,-1.68109553031869,136.617266659179));
#42395=CARTESIAN_POINT('Ctrl Pts',(6.60200641330949,-1.49726921239052,136.62619342842));
#42396=CARTESIAN_POINT('Ctrl Pts',(6.64141400419643,-1.31145865379569,136.635120197661));
#42397=CARTESIAN_POINT('Ctrl Pts',(6.67294476247483,-1.12432077138144,136.644046966902));
#42398=CARTESIAN_POINT('Ctrl Pts',(6.70385084062283,-0.94089042164866,136.652796881044));
#42399=CARTESIAN_POINT('Ctrl Pts',(6.72718922812515,-0.756185141262743,
136.661546795186));
#42400=CARTESIAN_POINT('Ctrl Pts',(6.74288064785628,-0.570832347336133,
136.670296709328));
#42401=CARTESIAN_POINT('Ctrl Pts',(6.75857175900919,-0.385483198448501,
136.679046451399));
#42402=CARTESIAN_POINT('Ctrl Pts',(6.76661617913882,-0.199486847133674,
136.68779619347));
#42403=CARTESIAN_POINT('Ctrl Pts',(6.76698658358759,-0.0134750712614812,
136.696545935542));
#42404=CARTESIAN_POINT('Ctrl Pts',(6.76735698124455,0.172533293857823,136.705295517176));
#42405=CARTESIAN_POINT('Ctrl Pts',(6.76005364423136,0.358556796342125,136.71404509881));
#42406=CARTESIAN_POINT('Ctrl Pts',(6.74510137904359,0.543963589245015,136.722794680444));
#42407=CARTESIAN_POINT('Ctrl Pts',(6.73014936815213,0.729367228895691,136.731544113272));
#42408=CARTESIAN_POINT('Ctrl Pts',(6.7075487124433,0.914153894279106,136.740293546101));
#42409=CARTESIAN_POINT('Ctrl Pts',(6.67737617463727,1.09769596081362,136.749042978929));
#42410=CARTESIAN_POINT('Ctrl Pts',(6.64720410988742,1.28123514970791,136.75779227458));
#42411=CARTESIAN_POINT('Ctrl Pts',(6.60946044708916,1.46352949601816,136.766541570231));
#42412=CARTESIAN_POINT('Ctrl Pts',(6.5642733778979,1.64395985967447,136.775290865883));
#42413=CARTESIAN_POINT('Ctrl Pts',(6.51908695712672,1.8243876342124,136.784040035985));
#42414=CARTESIAN_POINT('Ctrl Pts',(6.46645741331857,2.00295120164824,136.792789206086));
#42415=CARTESIAN_POINT('Ctrl Pts',(6.40656349104716,2.17904411042586,136.801538376188));
#42416=CARTESIAN_POINT('Ctrl Pts',(6.34667034866294,2.35513472627295,136.810287432366));
#42417=CARTESIAN_POINT('Ctrl Pts',(6.27951310937061,2.52875447656288,136.819036488543));
#42418=CARTESIAN_POINT('Ctrl Pts',(6.20531985190598,2.69931371565841,136.827785544721));
#42419=CARTESIAN_POINT('Ctrl Pts',(6.12830387608104,2.87636196348825,136.836867462972));
#42420=CARTESIAN_POINT('Ctrl Pts',(6.04370611833773,3.05011194839779,136.845949381223));
#42421=CARTESIAN_POINT('Ctrl Pts',(5.95183614183747,3.21992787818567,136.855031299473));
#42422=CARTESIAN_POINT('Ctrl Pts',(5.86332597394906,3.38353341100748,136.863781079758));
#42423=CARTESIAN_POINT('Ctrl Pts',(5.76806621040237,3.54348726717114,136.872530860043));
#42424=CARTESIAN_POINT('Ctrl Pts',(5.66638042494076,3.6992461231781,136.881280640328));
#42425=CARTESIAN_POINT('Ctrl Pts',(5.56469829503605,3.8549993797263,136.890030106062));
#42426=CARTESIAN_POINT('Ctrl Pts',(5.45659076217561,4.00655769790067,136.898779571796));
#42427=CARTESIAN_POINT('Ctrl Pts',(5.34242501440727,4.1534063087345,136.90752903753));
#42428=CARTESIAN_POINT('Ctrl Pts',(5.22826276398812,4.30025042101353,136.916278235233));
#42429=CARTESIAN_POINT('Ctrl Pts',(5.10804284592829,4.4423848884234,136.925027432937));
#42430=CARTESIAN_POINT('Ctrl Pts',(4.98217356309145,4.5793269797245,136.93377663064));
#42431=CARTESIAN_POINT('Ctrl Pts',(4.85630746721564,4.71626560370538,136.942525606817));
#42432=CARTESIAN_POINT('Ctrl Pts',(4.72479248669995,4.84801190370368,136.951274582994));
#42433=CARTESIAN_POINT('Ctrl Pts',(4.58807526322912,4.97411845244411,136.960023559171));
#42434=CARTESIAN_POINT('Ctrl Pts',(4.45134915258695,5.10023319861921,136.968773104067));
#42435=CARTESIAN_POINT('Ctrl Pts',(4.30942033290745,5.22070726557791,136.977522648963));
#42436=CARTESIAN_POINT('Ctrl Pts',(4.16277087520749,5.33513145484947,136.986272193859));
#42437=CARTESIAN_POINT('Ctrl Pts',(4.01613003785245,5.44954891804108,136.995021224439));
#42438=CARTESIAN_POINT('Ctrl Pts',(3.8647693436718,5.55791703889848,137.003770255019));
#42439=CARTESIAN_POINT('Ctrl Pts',(3.70920283931706,5.65986778085869,137.0125192856));
#42440=CARTESIAN_POINT('Ctrl Pts',(3.55363422426545,5.76181990606726,137.021268434885));
#42441=CARTESIAN_POINT('Ctrl Pts',(3.39385992450911,5.8573543210766,137.030017584171));
#42442=CARTESIAN_POINT('Ctrl Pts',(3.23042257544398,5.94614656597547,137.038766733456));
#42443=CARTESIAN_POINT('Ctrl Pts',(3.18692938489662,5.96977554704133,137.041095016552));
#42444=CARTESIAN_POINT('Ctrl Pts',(3.14317693223697,5.99292731134156,137.043423299647));
#42445=CARTESIAN_POINT('Ctrl Pts',(3.09917575053248,6.01559628526645,137.045751582743));
#42446=CARTESIAN_POINT('Ctrl Pts',(3.09917575053244,6.01559628526647,135.045784814338));
#42447=CARTESIAN_POINT('Ctrl Pts',(2.94386895177856,6.09560881299704,135.053980427697));
#42448=CARTESIAN_POINT('Ctrl Pts',(2.78543539305422,6.16961655946919,135.062176041057));
#42449=CARTESIAN_POINT('Ctrl Pts',(2.62438265169782,6.23737963390618,135.070371654417));
#42450=CARTESIAN_POINT('Ctrl Pts',(2.46332212967719,6.30514598206408,135.078567663717));
#42451=CARTESIAN_POINT('Ctrl Pts',(2.29964250359656,6.36666691759768,135.086763673017));
#42452=CARTESIAN_POINT('Ctrl Pts',(2.13387138950178,6.42175068755131,135.094959682317));
#42453=CARTESIAN_POINT('Ctrl Pts',(1.96806210663525,6.47684714053392,135.103157578748));
#42454=CARTESIAN_POINT('Ctrl Pts',(1.80016071703524,6.52550336246885,135.111355475178));
#42455=CARTESIAN_POINT('Ctrl Pts',(1.63071009932585,6.56757745077717,135.119553371608));
#42456=CARTESIAN_POINT('Ctrl Pts',(1.46118963574362,6.60966888160958,135.12775464713));
#42457=CARTESIAN_POINT('Ctrl Pts',(1.29011902001511,6.64517268827312,135.135955922652));
#42458=CARTESIAN_POINT('Ctrl Pts',(1.11805147058748,6.67399804533364,135.144157198174));
#42459=CARTESIAN_POINT('Ctrl Pts',(0.945796492507914,6.70285480109678,135.152367407129));
#42460=CARTESIAN_POINT('Ctrl Pts',(0.772542766060607,6.72501852076012,135.160577616085));
#42461=CARTESIAN_POINT('Ctrl Pts',(0.598849659984146,6.74045013962249,135.168787825041));
#42462=CARTESIAN_POINT('Ctrl Pts',(0.42504445880697,6.75589171748041,135.177003332561));
#42463=CARTESIAN_POINT('Ctrl Pts',(0.250799670077478,6.7645925172971,135.185218840082));
#42464=CARTESIAN_POINT('Ctrl Pts',(0.0766746961772759,6.76656559792086,
135.193434347602));
#42465=CARTESIAN_POINT('Ctrl Pts',(-0.0976759411793136,6.76854123562867,
135.201660502302));
#42466=CARTESIAN_POINT('Ctrl Pts',(-0.271906096475163,6.76377175418914,
135.209886657002));
#42467=CARTESIAN_POINT('Ctrl Pts',(-0.445460622895264,6.75232210676074,
135.218112811702));
#42468=CARTESIAN_POINT('Ctrl Pts',(-0.489282012439895,6.74943114522572,
135.22018986228));
#42469=CARTESIAN_POINT('Ctrl Pts',(-0.533060375600027,6.74611455845737,
135.222266912859));
#42470=CARTESIAN_POINT('Ctrl Pts',(-0.576786882283782,6.74237390630521,
135.224343963438));
#42471=CARTESIAN_POINT('Ctrl Pts',(-0.749938123180659,6.72756141358553,
135.23256881176));
#42472=CARTESIAN_POINT('Ctrl Pts',(-0.922761412954599,6.70605378641513,
135.240793660082));
#42473=CARTESIAN_POINT('Ctrl Pts',(-1.09469913561974,6.67786813305515,135.249018508404));
#42474=CARTESIAN_POINT('Ctrl Pts',(-1.26644321828709,6.64971422299018,135.257234093723));
#42475=CARTESIAN_POINT('Ctrl Pts',(-1.43730336899484,6.61489732035186,135.265449679043));
#42476=CARTESIAN_POINT('Ctrl Pts',(-1.60672494982419,6.57348643686229,135.273665264362));
#42477=CARTESIAN_POINT('Ctrl Pts',(-1.77598976455819,6.53211387093815,135.281873247785));
#42478=CARTESIAN_POINT('Ctrl Pts',(-1.94381831403307,6.4841595599196,135.290081231208));
#42479=CARTESIAN_POINT('Ctrl Pts',(-2.10966395224759,6.42974393025003,135.298289214632));
#42480=CARTESIAN_POINT('Ctrl Pts',(-2.2753894441314,6.37536772180557,135.306491251808));
#42481=CARTESIAN_POINT('Ctrl Pts',(-2.43913454650945,6.31453962953897,135.314693288985));
#42482=CARTESIAN_POINT('Ctrl Pts',(-2.60036554707839,6.24743051354457,135.322895326161));
#42483=CARTESIAN_POINT('Ctrl Pts',(-2.76151212099262,6.18035653842347,135.33109306844));
#42484=CARTESIAN_POINT('Ctrl Pts',(-2.92014688529361,6.10700822929251,135.33929081072));
#42485=CARTESIAN_POINT('Ctrl Pts',(-3.07575388260547,6.0276054162194,135.347488552999));
#42486=CARTESIAN_POINT('Ctrl Pts',(-3.23133129382267,5.94821770027678,135.355684736613));
#42487=CARTESIAN_POINT('Ctrl Pts',(-3.38388176265211,5.86277793071786,135.363880920228));
#42488=CARTESIAN_POINT('Ctrl Pts',(-3.53291154513242,5.77155308511237,135.372077103842));
#42489=CARTESIAN_POINT('Ctrl Pts',(-3.68193035694097,5.68033495492859,135.380272684103));
#42490=CARTESIAN_POINT('Ctrl Pts',(-3.82742869203973,5.58333278338579,135.388468264364));
#42491=CARTESIAN_POINT('Ctrl Pts',(-3.96893960261898,5.48085827501156,135.396663844625));
#42492=CARTESIAN_POINT('Ctrl Pts',(-4.11046584225693,5.37837266616636,135.404860312666));
#42493=CARTESIAN_POINT('Ctrl Pts',(-4.24800350613985,5.27041374997989,135.413056780706));
#42494=CARTESIAN_POINT('Ctrl Pts',(-4.38111666396505,5.157335142952,135.421253248747));
#42495=CARTESIAN_POINT('Ctrl Pts',(-4.51426845963583,5.04422371337052,135.42945209592));
#42496=CARTESIAN_POINT('Ctrl Pts',(-4.64299291773781,4.92598986516729,135.437650943094));
#42497=CARTESIAN_POINT('Ctrl Pts',(-4.76688904449317,4.80302590431189,135.445849790267));
#42498=CARTESIAN_POINT('Ctrl Pts',(-4.89091465474872,4.67993343416031,135.454057206033));
#42499=CARTESIAN_POINT('Ctrl Pts',(-5.01010159722915,4.55210122814411,135.462264621799));
#42500=CARTESIAN_POINT('Ctrl Pts',(-5.12408678035863,4.41995742822869,135.470472037565));
#42501=CARTESIAN_POINT('Ctrl Pts',(-5.2381330555376,4.28774280388379,135.478683852217));
#42502=CARTESIAN_POINT('Ctrl Pts',(-5.34697179003514,4.15121225919749,135.486895666869));
#42503=CARTESIAN_POINT('Ctrl Pts',(-5.45028181332655,4.01082499684564,135.495107481522));
#42504=CARTESIAN_POINT('Ctrl Pts',(-5.55374397633277,3.87023099290788,135.503331389319));
#42505=CARTESIAN_POINT('Ctrl Pts',(-5.65166095550955,3.72576921781061,135.511555297117));
#42506=CARTESIAN_POINT('Ctrl Pts',(-5.74375565126593,3.57792677657757,135.519779204914));
#42507=CARTESIAN_POINT('Ctrl Pts',(-5.82884944931349,3.44132309127496,135.527377943838));
#42508=CARTESIAN_POINT('Ctrl Pts',(-5.90897291807125,3.30183366422781,135.534976682761));
#42509=CARTESIAN_POINT('Ctrl Pts',(-5.98394366326475,3.15985873653771,135.542575421685));
#42510=CARTESIAN_POINT('Ctrl Pts',(-6.06893960768602,2.99889871097019,135.551190275246));
#42511=CARTESIAN_POINT('Ctrl Pts',(-6.14754099250621,2.83431097684033,135.559805128807));
#42512=CARTESIAN_POINT('Ctrl Pts',(-6.21943977118642,2.66661919527041,135.568419982368));
#42513=CARTESIAN_POINT('Ctrl Pts',(-6.29121675126856,2.49921148839938,135.57702024212));
#42514=CARTESIAN_POINT('Ctrl Pts',(-6.35631363926335,2.32871049720225,135.585620501872));
#42515=CARTESIAN_POINT('Ctrl Pts',(-6.41446782623058,2.15566498005899,135.594220761623));
#42516=CARTESIAN_POINT('Ctrl Pts',(-6.472486908962,1.98302148353667,135.602801041188));
#42517=CARTESIAN_POINT('Ctrl Pts',(-6.52359536620775,1.80784554277667,135.611381320753));
#42518=CARTESIAN_POINT('Ctrl Pts',(-6.56757851987453,1.63070579360064,135.619961600317));
#42519=CARTESIAN_POINT('Ctrl Pts',(-6.6115023361629,1.45380502247536,135.628530304284));
#42520=CARTESIAN_POINT('Ctrl Pts',(-6.6483199339772,1.27494601980787,135.637099008251));
#42521=CARTESIAN_POINT('Ctrl Pts',(-6.67786559221037,1.09471463513233,135.645667712218));
#42522=CARTESIAN_POINT('Ctrl Pts',(-6.70745774600986,0.914199622986577,
135.654249900628));
#42523=CARTESIAN_POINT('Ctrl Pts',(-6.72975492875082,0.732308194204803,
135.662832089038));
#42524=CARTESIAN_POINT('Ctrl Pts',(-6.74464084693375,0.549644290312154,
135.671414277448));
#42525=CARTESIAN_POINT('Ctrl Pts',(-6.75952676511669,0.366980386419505,
135.679996465858));
#42526=CARTESIAN_POINT('Ctrl Pts',(-6.76700133295404,0.183544311678704,
135.688578654268));
#42527=CARTESIAN_POINT('Ctrl Pts',(-6.7669999998216,-4.91374134034539E-5,
135.697160842678));
#42528=CARTESIAN_POINT('',(-6.76699727515127,-0.00607273375871645,135.302820216236));
#42529=CARTESIAN_POINT('Ctrl Pts',(3.09917575053266,6.01559628526635,134.651234928213));
#42530=CARTESIAN_POINT('Ctrl Pts',(2.94375641574756,6.09566679044796,134.659449205158));
#42531=CARTESIAN_POINT('Ctrl Pts',(2.78532630390312,6.16966174797828,134.667663482103));
#42532=CARTESIAN_POINT('Ctrl Pts',(2.62440605859029,6.23736978538507,134.675877759049));
#42533=CARTESIAN_POINT('Ctrl Pts',(2.46339164215883,6.30511744578405,134.684096843019));
#42534=CARTESIAN_POINT('Ctrl Pts',(2.29988452233624,6.36657072615371,134.692315926989));
#42535=CARTESIAN_POINT('Ctrl Pts',(2.13442169041754,6.42156780291816,134.70053501096));
#42536=CARTESIAN_POINT('Ctrl Pts',(1.96870032426658,6.47665081213555,134.708766937177));
#42537=CARTESIAN_POINT('Ctrl Pts',(1.80101748311864,6.52525735769499,134.716998863395));
#42538=CARTESIAN_POINT('Ctrl Pts',(1.631922906266,6.56727619550178,134.725230789612));
#42539=CARTESIAN_POINT('Ctrl Pts',(1.47238318581289,6.60692071729683,134.732997562692));
#42540=CARTESIAN_POINT('Ctrl Pts',(1.31158709881734,6.64070139695056,134.740764335773));
#42541=CARTESIAN_POINT('Ctrl Pts',(1.15000040363666,6.66856716781315,134.748531108853));
#42542=CARTESIAN_POINT('Ctrl Pts',(0.980327161221296,6.69782747101679,134.75668656726));
#42543=CARTESIAN_POINT('Ctrl Pts',(0.809259701637315,6.72065559255727,134.764842025667));
#42544=CARTESIAN_POINT('Ctrl Pts',(0.637331484518815,6.73692048185527,134.772997484073));
#42545=CARTESIAN_POINT('Ctrl Pts',(0.465612526639907,6.75316557464503,134.781143016215));
#42546=CARTESIAN_POINT('Ctrl Pts',(0.293035256511699,6.76286330225553,134.789288548357));
#42547=CARTESIAN_POINT('Ctrl Pts',(0.120144304616915,6.76593336843248,134.797434080499));
#42548=CARTESIAN_POINT('Ctrl Pts',(-0.0525725717618749,6.76900034350867,
134.8055714113));
#42549=CARTESIAN_POINT('Ctrl Pts',(-0.225602138431937,6.76545293561209,
134.8137087421));
#42550=CARTESIAN_POINT('Ctrl Pts',(-0.398393642743159,6.75526250455316,
134.821846072901));
#42551=CARTESIAN_POINT('Ctrl Pts',(-0.571047484336989,6.74508019219449,
134.829976920703));
#42552=CARTESIAN_POINT('Ctrl Pts',(-0.743463278046017,6.72826541608935,
134.838107768505));
#42553=CARTESIAN_POINT('Ctrl Pts',(-0.915089264245877,6.70484158190646,
134.846238616307));
#42554=CARTESIAN_POINT('Ctrl Pts',(-1.08661456930557,6.68143148887306,134.854364694301));
#42555=CARTESIAN_POINT('Ctrl Pts',(-1.25735062832298,6.65142010819043,134.862490772295));
#42556=CARTESIAN_POINT('Ctrl Pts',(-1.42674980407973,6.61488276514093,134.870616850288));
#42557=CARTESIAN_POINT('Ctrl Pts',(-1.59674963837203,6.57821586734671,134.878771741871));
#42558=CARTESIAN_POINT('Ctrl Pts',(-1.76540272049193,6.53497667053279,134.886926633453));
#42559=CARTESIAN_POINT('Ctrl Pts',(-1.93216428719813,6.48529337557494,134.895081525035));
#42560=CARTESIAN_POINT('Ctrl Pts',(-2.09827554210092,6.43580382809608,134.903204615391));
#42561=CARTESIAN_POINT('Ctrl Pts',(-2.26250965949945,6.37992047329634,134.911327705747));
#42562=CARTESIAN_POINT('Ctrl Pts',(-2.42434222066462,6.31782033593097,134.919450796104));
#42563=CARTESIAN_POINT('Ctrl Pts',(-2.5861874896611,6.2557153221794,134.927574524322));
#42564=CARTESIAN_POINT('Ctrl Pts',(-2.74563048522756,6.18739268450539,134.935698252541));
#42565=CARTESIAN_POINT('Ctrl Pts',(-2.90216584432869,6.11307798183631,134.943821980759));
#42566=CARTESIAN_POINT('Ctrl Pts',(-3.05874327596736,6.03874330535343,134.951947892419));
#42567=CARTESIAN_POINT('Ctrl Pts',(-3.2124111847011,5.95841351387982,134.96007380408));
#42568=CARTESIAN_POINT('Ctrl Pts',(-3.36268796982347,5.87236056604195,134.96819971574));
#42569=CARTESIAN_POINT('Ctrl Pts',(-3.51392579060767,5.78575730065763,134.97637759345));
#42570=CARTESIAN_POINT('Ctrl Pts',(-3.66172863811399,5.69335761111662,134.98455547116));
#42571=CARTESIAN_POINT('Ctrl Pts',(-3.80563511522079,5.59548303275048,134.99273334887));
#42572=CARTESIAN_POINT('Ctrl Pts',(-3.94885475792429,5.49807558851882,135.000872195343));
#42573=CARTESIAN_POINT('Ctrl Pts',(-4.08821488393055,5.39524566857946,135.009011041817));
#42574=CARTESIAN_POINT('Ctrl Pts',(-4.22329412815464,5.28735053756554,135.01714988829));
#42575=CARTESIAN_POINT('Ctrl Pts',(-4.35934506596433,5.17867926209414,135.025347281619));
#42576=CARTESIAN_POINT('Ctrl Pts',(-4.49105301484361,5.06486987451833,135.033544674947));
#42577=CARTESIAN_POINT('Ctrl Pts',(-4.6180256938709,4.94632466491518,135.041742068275));
#42578=CARTESIAN_POINT('Ctrl Pts',(-4.74499837289828,4.82777945531193,135.049939461604));
#42579=CARTESIAN_POINT('Ctrl Pts',(-4.8672355633818,4.70449873103403,135.058136854932));
#42580=CARTESIAN_POINT('Ctrl Pts',(-4.98438690250362,4.57691776265975,135.06633424826));
#42581=CARTESIAN_POINT('Ctrl Pts',(-5.10086689039312,4.45006791388668,135.074484665343));
#42582=CARTESIAN_POINT('Ctrl Pts',(-5.21268078880439,4.31857319100973,135.082635082425));
#42583=CARTESIAN_POINT('Ctrl Pts',(-5.3194320149186,4.18281389003373,135.090785499508));
#42584=CARTESIAN_POINT('Ctrl Pts',(-5.42605861687286,4.0472130779993,135.098926401581));
#42585=CARTESIAN_POINT('Ctrl Pts',(-5.52763408874244,3.90735788464401,135.107067303655));
#42586=CARTESIAN_POINT('Ctrl Pts',(-5.62379884921759,3.76366516889308,135.115208205728));
#42587=CARTESIAN_POINT('Ctrl Pts',(-5.71985329518928,3.62013728889394,135.123339769042));
#42588=CARTESIAN_POINT('Ctrl Pts',(-5.81050919468711,3.47278096033235,135.131471332356));
#42589=CARTESIAN_POINT('Ctrl Pts',(-5.89544760215918,3.32204554005445,135.13960289567));
#42590=CARTESIAN_POINT('Ctrl Pts',(-5.98033041312994,3.17140878376426,135.147729136463));
#42591=CARTESIAN_POINT('Ctrl Pts',(-6.05950300213959,3.01739765578338,135.155855377256));
#42592=CARTESIAN_POINT('Ctrl Pts',(-6.13268982894256,2.8604902485386,135.163981618048));
#42593=CARTESIAN_POINT('Ctrl Pts',(-6.20584271886969,2.70365559956784,135.172104090687));
#42594=CARTESIAN_POINT('Ctrl Pts',(-6.27301521813021,2.5439276762172,135.180226563326));
#42595=CARTESIAN_POINT('Ctrl Pts',(-6.33397785597443,2.38180887562909,135.188349035965));
#42596=CARTESIAN_POINT('Ctrl Pts',(-6.39492385896012,2.21973431235435,135.196469292227));
#42597=CARTESIAN_POINT('Ctrl Pts',(-6.4496632467032,2.05527051365083,135.204589548489));
#42598=CARTESIAN_POINT('Ctrl Pts',(-6.49801481700214,1.88893950088949,135.212709804751));
#42599=CARTESIAN_POINT('Ctrl Pts',(-6.54637421784645,1.72258155079119,135.22083137609));
#42600=CARTESIAN_POINT('Ctrl Pts',(-6.58834362541911,1.55435613228336,135.228952947429));
#42601=CARTESIAN_POINT('Ctrl Pts',(-6.62379172668878,1.38480040491377,135.237074518768));
#42602=CARTESIAN_POINT('Ctrl Pts',(-6.65924229645898,1.21523287018671,135.245196655669));
#42603=CARTESIAN_POINT('Ctrl Pts',(-6.68817058647215,1.04433520189303,135.25331879257));
#42604=CARTESIAN_POINT('Ctrl Pts',(-6.71049652523991,0.872654218315073,
135.261440929471));
#42605=CARTESIAN_POINT('Ctrl Pts',(-6.73283687678045,0.700862404055715,
135.269568309714));
#42606=CARTESIAN_POINT('Ctrl Pts',(-6.748566321262,0.528286628481025,135.277695689956));
#42607=CARTESIAN_POINT('Ctrl Pts',(-6.75765667739668,0.355478874809866,
135.285823070198));
#42608=CARTESIAN_POINT('Ctrl Pts',(-6.76399369727002,0.235012068773062,
135.291488785529));
#42609=CARTESIAN_POINT('Ctrl Pts',(-6.76710541717883,0.11443261880474,135.297154500859));
#42610=CARTESIAN_POINT('Ctrl Pts',(-6.76699727515214,-0.00607273278968599,
135.30282021619));
#42611=CARTESIAN_POINT('Ctrl Pts',(-6.76699727515127,-0.0060727337587121,
135.302820216236));
#42612=CARTESIAN_POINT('Ctrl Pts',(-6.76679986671651,-0.226049830262332,
135.31316272461));
#42613=CARTESIAN_POINT('Ctrl Pts',(-6.75587263188703,-0.445562092144057,
135.323505232985));
#42614=CARTESIAN_POINT('Ctrl Pts',(-6.73437268671693,-0.663711922750399,
135.333847741359));
#42615=CARTESIAN_POINT('Ctrl Pts',(-6.71248172404542,-0.88582922401878,
135.344378347971));
#42616=CARTESIAN_POINT('Ctrl Pts',(-6.67962999568742,-1.10653425722591,
135.354908954583));
#42617=CARTESIAN_POINT('Ctrl Pts',(-6.63603191500124,-1.32490355237086,
135.365439561194));
#42618=CARTESIAN_POINT('Ctrl Pts',(-6.61022810402908,-1.45414685678616,
135.371672170019));
#42619=CARTESIAN_POINT('Ctrl Pts',(-6.58066082080314,-1.5825724067862,135.377904778844));
#42620=CARTESIAN_POINT('Ctrl Pts',(-6.54738235195893,-1.70999220385846,
135.384137387669));
#42621=CARTESIAN_POINT('Ctrl Pts',(-6.5034592722332,-1.87816910922156,135.392363588688));
#42622=CARTESIAN_POINT('Ctrl Pts',(-6.45299091726314,-2.04488766880344,
135.400589789706));
#42623=CARTESIAN_POINT('Ctrl Pts',(-6.3960888113794,-2.20960107642698,135.408815990725));
#42624=CARTESIAN_POINT('Ctrl Pts',(-6.3392506230189,-2.37412946325213,135.417032951341));
#42625=CARTESIAN_POINT('Ctrl Pts',(-6.27599319063386,-2.53665684729028,
135.425249911957));
#42626=CARTESIAN_POINT('Ctrl Pts',(-6.20647868369198,-2.69664816927923,
135.433466872572));
#42627=CARTESIAN_POINT('Ctrl Pts',(-6.13702830953398,-2.85649188626708,
135.441676252374));
#42628=CARTESIAN_POINT('Ctrl Pts',(-6.06133249930582,-3.01380387398899,
135.449885632176));
#42629=CARTESIAN_POINT('Ctrl Pts',(-5.97960273516409,-3.16806567634228,
135.458095011977));
#42630=CARTESIAN_POINT('Ctrl Pts',(-5.89793197482443,-3.32221611127702,
135.466298465118));
#42631=CARTESIAN_POINT('Ctrl Pts',(-5.81023610447354,-3.47332043131457,
135.474501918258));
#42632=CARTESIAN_POINT('Ctrl Pts',(-5.71677411393429,-3.62088148525339,
135.482705371398));
#42633=CARTESIAN_POINT('Ctrl Pts',(-5.62336084889186,-3.76836560967657,
135.490904547749));
#42634=CARTESIAN_POINT('Ctrl Pts',(-5.52418764381147,-3.91230984579046,
135.499103724099));
#42635=CARTESIAN_POINT('Ctrl Pts',(-5.41955873637874,-4.05224284846564,
135.507302900449));
#42636=CARTESIAN_POINT('Ctrl Pts',(-5.31494951645399,-4.19214952063451,
135.515500534));
#42637=CARTESIAN_POINT('Ctrl Pts',(-5.20488684855691,-4.32804617214016,
135.523698167552));
#42638=CARTESIAN_POINT('Ctrl Pts',(-5.08971766663502,-4.45949134699726,
135.531895801103));
#42639=CARTESIAN_POINT('Ctrl Pts',(-4.97455677972071,-4.59092705457584,
135.540092844224));
#42640=CARTESIAN_POINT('Ctrl Pts',(-4.85429034697056,-4.71791165367092,
135.548289887344));
#42641=CARTESIAN_POINT('Ctrl Pts',(-4.72930483669364,-4.84003768183949,
135.556486930465));
#42642=CARTESIAN_POINT('Ctrl Pts',(-4.60430561253319,-4.96217711013838,
135.564684872996));
#42643=CARTESIAN_POINT('Ctrl Pts',(-4.47458653584447,-5.07945665469392,
135.572882815527));
#42644=CARTESIAN_POINT('Ctrl Pts',(-4.3405701204733,-5.19150652790252,135.581080758058));
#42645=CARTESIAN_POINT('Ctrl Pts',(-4.2065146429628,-5.30358906060097,135.589281090067));
#42646=CARTESIAN_POINT('Ctrl Pts',(-4.06815960692982,-5.41043865570606,
135.597481422075));
#42647=CARTESIAN_POINT('Ctrl Pts',(-3.92595973287986,-5.51172651496842,
135.605681754084));
#42648=CARTESIAN_POINT('Ctrl Pts',(-3.78361164812745,-5.61311994355615,
135.613890633054));
#42649=CARTESIAN_POINT('Ctrl Pts',(-3.63741101178872,-5.70893984674031,
135.622099512025));
#42650=CARTESIAN_POINT('Ctrl Pts',(-3.48784143229593,-5.79890085646926,
135.630308390996));
#42651=CARTESIAN_POINT('Ctrl Pts',(-3.3381915603836,-5.88891015935487,135.638521676683));
#42652=CARTESIAN_POINT('Ctrl Pts',(-3.18516945394858,-5.9730541260828,135.646734962371));
#42653=CARTESIAN_POINT('Ctrl Pts',(-3.02928222881453,-6.05109396540729,
135.654948248058));
#42654=CARTESIAN_POINT('Ctrl Pts',(-2.87316695988291,-6.12924796739845,
135.66317354877));
#42655=CARTESIAN_POINT('Ctrl Pts',(-2.71417852287252,-6.20127984877912,
135.671398849482));
#42656=CARTESIAN_POINT('Ctrl Pts',(-2.55284404967992,-6.26699898340616,
135.679624150194));
#42657=CARTESIAN_POINT('Ctrl Pts',(-2.40693648010347,-6.32643401312018,
135.687062942488));
#42658=CARTESIAN_POINT('Ctrl Pts',(-2.25911048961878,-6.38070641181775,
135.694501734782));
#42659=CARTESIAN_POINT('Ctrl Pts',(-2.10976495382097,-6.42971078973455,
135.701940527076));
#42660=CARTESIAN_POINT('Ctrl Pts',(-1.94608947698599,-6.48341721543843,
135.710093083289));
#42661=CARTESIAN_POINT('Ctrl Pts',(-1.78010591636705,-6.53095375125263,
135.718245639503));
#42662=CARTESIAN_POINT('Ctrl Pts',(-1.61232421108503,-6.5721153092706,135.726398195716));
#42663=CARTESIAN_POINT('Ctrl Pts',(-1.44473688495347,-6.61322918063129,
135.734541306996));
#42664=CARTESIAN_POINT('Ctrl Pts',(-1.27535591236074,-6.64798268966008,
135.742684418277));
#42665=CARTESIAN_POINT('Ctrl Pts',(-1.104709404532,-6.67621944902492,135.750827529557));
#42666=CARTESIAN_POINT('Ctrl Pts',(-0.934224718493542,-6.70442943185028,
135.758962918834));
#42667=CARTESIAN_POINT('Ctrl Pts',(-0.762477244622202,-6.72613490882853,
135.767098308112));
#42668=CARTESIAN_POINT('Ctrl Pts',(-0.590008392774742,-6.74122979110306,
135.775233697389));
#42669=CARTESIAN_POINT('Ctrl Pts',(-0.41766685095481,-6.75631353090254,
135.783363081428));
#42670=CARTESIAN_POINT('Ctrl Pts',(-0.244605354082271,-6.76479636058453,
135.791492465466));
#42671=CARTESIAN_POINT('Ctrl Pts',(-0.0713735999031859,-6.76662359003638,
135.799621849505));
#42672=CARTESIAN_POINT('Ctrl Pts',(0.101766668056435,-6.76844985450167,
135.807746940297));
#42673=CARTESIAN_POINT('Ctrl Pts',(0.27507664952675,-6.76362751499981,135.815872031089));
#42674=CARTESIAN_POINT('Ctrl Pts',(0.448003455664473,-6.75215387144818,
135.823997121881));
#42675=CARTESIAN_POINT('Ctrl Pts',(0.621590360909375,-6.7406364305118,135.832153227906));
#42676=CARTESIAN_POINT('Ctrl Pts',(0.794790788257611,-6.72241678171025,
135.840309333931));
#42677=CARTESIAN_POINT('Ctrl Pts',(0.967046932838719,-6.69754501512959,
135.848465439957));
#42678=CARTESIAN_POINT('Ctrl Pts',(1.13860977759075,-6.67277335291131,135.85658871913));
#42679=CARTESIAN_POINT('Ctrl Pts',(1.3092355651262,-6.64140309460029,135.864711998303));
#42680=CARTESIAN_POINT('Ctrl Pts',(1.47838010729718,-6.60353551200779,135.872835277477));
#42681=CARTESIAN_POINT('Ctrl Pts',(1.64754717249343,-6.56566288702664,135.880959638333));
#42682=CARTESIAN_POINT('Ctrl Pts',(1.81523224243433,-6.5212912944284,135.88908399919));
#42683=CARTESIAN_POINT('Ctrl Pts',(1.98090320622816,-6.47057273257592,135.897208360047));
#42684=CARTESIAN_POINT('Ctrl Pts',(2.14662775026381,-6.41983776765107,135.905335348432));
#42685=CARTESIAN_POINT('Ctrl Pts',(2.31033654141122,-6.36275185293676,135.913462336818));
#42686=CARTESIAN_POINT('Ctrl Pts',(2.4715145046851,-6.29951625548591,135.921589325203));
#42687=CARTESIAN_POINT('Ctrl Pts',(2.63373446514111,-6.23587184709703,135.929768853643));
#42688=CARTESIAN_POINT('Ctrl Pts',(2.79339041138535,-6.16599810356462,135.937948382083));
#42689=CARTESIAN_POINT('Ctrl Pts',(2.94998031069297,-6.09014820562881,135.946127910523));
#42690=CARTESIAN_POINT('Ctrl Pts',(3.10583277768259,-6.01465550931522,135.954268918927));
#42691=CARTESIAN_POINT('Ctrl Pts',(3.25864772138151,-5.93324305328491,135.962409927331));
#42692=CARTESIAN_POINT('Ctrl Pts',(3.40795773782195,-5.8462050132731,135.970550935734));
#42693=CARTESIAN_POINT('Ctrl Pts',(3.55832746830142,-5.75854922881836,135.978749724193));
#42694=CARTESIAN_POINT('Ctrl Pts',(3.70514201828591,-5.66518791531266,135.986948512651));
#42695=CARTESIAN_POINT('Ctrl Pts',(3.847956675002,-5.56646372729649,135.995147301109));
#42696=CARTESIAN_POINT('Ctrl Pts',(3.99077133171809,-5.46773953928033,136.003346089567));
#42697=CARTESIAN_POINT('Ctrl Pts',(4.12958583691194,-5.36365275137169,136.011544878026));
#42698=CARTESIAN_POINT('Ctrl Pts',(4.26399241036301,-5.2545844483048,136.019743666484));
#42699=CARTESIAN_POINT('Ctrl Pts',(4.39896065145484,-5.14506036294325,136.027976716616));
#42700=CARTESIAN_POINT('Ctrl Pts',(4.52990367279796,-5.03017267465564,136.036209766748));
#42701=CARTESIAN_POINT('Ctrl Pts',(4.65636808142651,-4.91024696835835,136.04444281688));
#42702=CARTESIAN_POINT('Ctrl Pts',(4.78268189038405,-4.79046407514272,136.052666062715));
#42703=CARTESIAN_POINT('Ctrl Pts',(4.90452744927105,-4.6656553544627,136.06088930855));
#42704=CARTESIAN_POINT('Ctrl Pts',(5.02148275758391,-4.53618781746165,136.069112554384));
#42705=CARTESIAN_POINT('Ctrl Pts',(5.1383221989597,-4.40684854318915,136.077327653498));
#42706=CARTESIAN_POINT('Ctrl Pts',(5.25028079967261,-4.27285990830849,136.085542752611));
#42707=CARTESIAN_POINT('Ctrl Pts',(5.35697183840158,-4.13462715641598,136.093757851725));
#42708=CARTESIAN_POINT('Ctrl Pts',(5.46357852567245,-3.9965036933102,136.101966455864));
#42709=CARTESIAN_POINT('Ctrl Pts',(5.56492572816444,-3.85414307886854,136.110175060003));
#42710=CARTESIAN_POINT('Ctrl Pts',(5.66066555732851,-3.70798522759661,136.118383664142));
#42711=CARTESIAN_POINT('Ctrl Pts',(5.75634884385217,-3.56191369516294,136.126587420391));
#42712=CARTESIAN_POINT('Ctrl Pts',(5.84643115854175,-3.41204969227551,136.13479117664));
#42713=CARTESIAN_POINT('Ctrl Pts',(5.93060663138424,-3.25886390998172,136.142994932889));
#42714=CARTESIAN_POINT('Ctrl Pts',(6.01475719882597,-3.10572345149982,136.151196261853));
#42715=CARTESIAN_POINT('Ctrl Pts',(6.09300423008896,-2.94926348302826,136.159397590817));
#42716=CARTESIAN_POINT('Ctrl Pts',(6.16508658856647,-2.78998142565105,136.167598919781));
#42717=CARTESIAN_POINT('Ctrl Pts',(6.23715900619858,-2.6307213347902,136.175799117704));
#42718=CARTESIAN_POINT('Ctrl Pts',(6.30306829588569,-2.46864025613144,136.183999315627));
#42719=CARTESIAN_POINT('Ctrl Pts',(6.36260047293043,-2.30425784621979,136.192199513549));
#42720=CARTESIAN_POINT('Ctrl Pts',(6.42213522836136,-2.13986831677454,136.200400066629));
#42721=CARTESIAN_POINT('Ctrl Pts',(6.47529219883229,-1.97317759437616,136.208600619709));
#42722=CARTESIAN_POINT('Ctrl Pts',(6.52190649157642,-1.80472289150809,136.216801172789));
#42723=CARTESIAN_POINT('Ctrl Pts',(6.56853125064582,-1.63623036544012,136.225003567142));
#42724=CARTESIAN_POINT('Ctrl Pts',(6.60861031056241,-1.46597341528508,136.233205961495));
#42725=CARTESIAN_POINT('Ctrl Pts',(6.6420293341823,-1.29450195977522,136.241408355848));
#42726=CARTESIAN_POINT('Ctrl Pts',(6.67547961046399,-1.12287014831153,136.249618420882));
#42727=CARTESIAN_POINT('Ctrl Pts',(6.70225733818844,-0.950021914430184,
136.257828485916));
#42728=CARTESIAN_POINT('Ctrl Pts',(6.72229962242656,-0.776515799146235,
136.26603855095));
#42729=CARTESIAN_POINT('Ctrl Pts',(6.74235149854637,-0.602926646913526,
136.274252545175));
#42730=CARTESIAN_POINT('Ctrl Pts',(6.75566147684693,-0.428679342564065,
136.282466539401));
#42731=CARTESIAN_POINT('Ctrl Pts',(6.76221877328653,-0.254334940995662,
136.290680533626));
#42732=CARTESIAN_POINT('Ctrl Pts',(6.76878500950514,-0.0797528499407057,
136.298905726261));
#42733=CARTESIAN_POINT('Ctrl Pts',(6.76858016566121,0.0949262445043662,
136.307130918896));
#42734=CARTESIAN_POINT('Ctrl Pts',(6.76164560026206,0.269142669334809,136.315356111531));
#42735=CARTESIAN_POINT('Ctrl Pts',(6.75540936045118,0.425815127045349,136.322753009651));
#42736=CARTESIAN_POINT('Ctrl Pts',(6.74373126377443,0.582113277860358,136.330149907771));
#42737=CARTESIAN_POINT('Ctrl Pts',(6.72667688091511,0.737636183875304,136.337546805891));
#42738=CARTESIAN_POINT('Ctrl Pts',(6.7067426300531,0.919421279757408,136.346192772382));
#42739=CARTESIAN_POINT('Ctrl Pts',(6.67941735311857,1.1005597477816,136.354838738873));
#42740=CARTESIAN_POINT('Ctrl Pts',(6.64475423594991,1.28044138632964,136.363484705364));
#42741=CARTESIAN_POINT('Ctrl Pts',(6.6101354576204,1.46009293180789,136.372119612488));
#42742=CARTESIAN_POINT('Ctrl Pts',(6.56819761291054,1.63849055556209,136.380754519613));
#42743=CARTESIAN_POINT('Ctrl Pts',(6.51904550524376,1.81503022028866,136.389389426737));
#42744=CARTESIAN_POINT('Ctrl Pts',(6.46826158727407,1.99743085939558,136.398311005809));
#42745=CARTESIAN_POINT('Ctrl Pts',(6.40977616501106,2.17784773207027,136.40723258488));
#42746=CARTESIAN_POINT('Ctrl Pts',(6.34376261036176,2.35562410910064,136.416154163952));
#42747=CARTESIAN_POINT('Ctrl Pts',(6.28004669104689,2.52721288893735,136.424765222927));
#42748=CARTESIAN_POINT('Ctrl Pts',(6.20931793043112,2.69634154520653,136.433376281903));
#42749=CARTESIAN_POINT('Ctrl Pts',(6.1317834083069,2.86243274743919,136.441987340879));
#42750=CARTESIAN_POINT('Ctrl Pts',(6.05432200481651,3.02836731800034,136.450590279228));
#42751=CARTESIAN_POINT('Ctrl Pts',(5.97006776449354,3.19126987008528,136.459193217578));
#42752=CARTESIAN_POINT('Ctrl Pts',(5.8792761950018,3.35058210209587,136.467796155927));
#42753=CARTESIAN_POINT('Ctrl Pts',(5.78858629106469,3.50971594126098,136.476389460976));
#42754=CARTESIAN_POINT('Ctrl Pts',(5.69137381241983,3.66526721640593,136.484982766025));
#42755=CARTESIAN_POINT('Ctrl Pts',(5.58794071107854,3.81670114227865,136.493576071074));
#42756=CARTESIAN_POINT('Ctrl Pts',(5.57641657056191,3.83357336034144,136.494533505914));
#42757=CARTESIAN_POINT('Ctrl Pts',(5.56481525689396,3.85039449191347,136.495490940755));
#42758=CARTESIAN_POINT('Ctrl Pts',(5.55313722300797,3.86716381634439,136.496448375595));
#42759=CARTESIAN_POINT('Ctrl Pts',(5.4482957167536,4.01771323668101,136.505043907326));
#42760=CARTESIAN_POINT('Ctrl Pts',(5.33738994259946,4.16390834428211,136.513639439056));
#42761=CARTESIAN_POINT('Ctrl Pts',(5.22081277752856,4.3052761748806,136.522234970787));
#42762=CARTESIAN_POINT('Ctrl Pts',(5.10412689175144,4.44677584613904,136.530838518772));
#42763=CARTESIAN_POINT('Ctrl Pts',(4.98175925188976,4.58343901883024,136.539442066758));
#42764=CARTESIAN_POINT('Ctrl Pts',(4.85414105635593,4.71482805677999,136.548045614743));
#42765=CARTESIAN_POINT('Ctrl Pts',(4.72629659892285,4.84645004218008,136.556664416472));
#42766=CARTESIAN_POINT('Ctrl Pts',(4.59318318588712,4.9727789761998,136.5652832182));
#42767=CARTESIAN_POINT('Ctrl Pts',(4.45526823835273,5.09341476068122,136.573902019928));
#42768=CARTESIAN_POINT('Ctrl Pts',(4.31723216976737,5.21415649113343,136.582528390947));
#42769=CARTESIAN_POINT('Ctrl Pts',(4.17438638564857,5.32919489817194,136.591154761965));
#42770=CARTESIAN_POINT('Ctrl Pts',(4.02722979680182,5.43817149083693,136.599781132984));
#42771=CARTESIAN_POINT('Ctrl Pts',(3.87980799723326,5.54734448490691,136.608423050749));
#42772=CARTESIAN_POINT('Ctrl Pts',(3.72806010805104,5.65043364266486,136.617064968514));
#42773=CARTESIAN_POINT('Ctrl Pts',(3.57251416560888,5.74712376206776,136.625706886278));
#42774=CARTESIAN_POINT('Ctrl Pts',(3.41828942990522,5.84299259590516,136.634275399621));
#42775=CARTESIAN_POINT('Ctrl Pts',(3.26033119644323,5.93257059232623,136.642843912964));
#42776=CARTESIAN_POINT('Ctrl Pts',(3.0991757505325,6.01559628526643,136.651412426306));
#42777=CARTESIAN_POINT('Origin',(0.,0.,-3.69717978381041));
#42778=CARTESIAN_POINT('',(3.09917575053254,6.01559628526642,139.045839590042));
#42779=CARTESIAN_POINT('',(3.09917575053274,6.01559628526631,138.651549674451));
#42780=CARTESIAN_POINT('',(3.09917575053259,6.01559628526639,-3.69717978381041));
#42781=CARTESIAN_POINT('',(-6.7669998232546,-0.000434751987798659,137.69717978381));
#42782=CARTESIAN_POINT('Ctrl Pts',(-6.76699776313827,-0.00550215245942883,
137.69717978381));
#42783=CARTESIAN_POINT('Ctrl Pts',(-6.76680634472756,-0.24092419258413,
137.708261686933));
#42784=CARTESIAN_POINT('Ctrl Pts',(-6.75432628838775,-0.475813744433624,
137.719343590055));
#42785=CARTESIAN_POINT('Ctrl Pts',(-6.72974340733669,-0.709114004521386,
137.730425493178));
#42786=CARTESIAN_POINT('Ctrl Pts',(-6.70434842898574,-0.950121356015059,
137.741873487793));
#42787=CARTESIAN_POINT('Ctrl Pts',(-6.66603767317495,-1.18943322621959,
137.753321482407));
#42788=CARTESIAN_POINT('Ctrl Pts',(-6.61506338143551,-1.42591215002575,
137.764769477022));
#42789=CARTESIAN_POINT('Ctrl Pts',(-6.60700973581777,-1.46327446313319,
137.766578194485));
#42790=CARTESIAN_POINT('Ctrl Pts',(-6.59864007656568,-1.50056610371897,
137.768386911949));
#42791=CARTESIAN_POINT('Ctrl Pts',(-6.58995550656827,-1.5377826314049,137.770195629413));
#42792=CARTESIAN_POINT('Ctrl Pts',(-6.55081850664034,-1.70549885014642,
137.778346611587));
#42793=CARTESIAN_POINT('Ctrl Pts',(-6.50521320785507,-1.87198348611265,
137.786497593761));
#42794=CARTESIAN_POINT('Ctrl Pts',(-6.45322902003838,-2.03669443337349,
137.794648575935));
#42795=CARTESIAN_POINT('Ctrl Pts',(-6.4013052166738,-2.20121405360344,137.802790089988));
#42796=CARTESIAN_POINT('Ctrl Pts',(-6.34301738273073,-2.36396374115074,
137.810931604041));
#42797=CARTESIAN_POINT('Ctrl Pts',(-6.2785059857144,-2.5244111367502,137.819073118094));
#42798=CARTESIAN_POINT('Ctrl Pts',(-6.21405594910061,-2.68470592184615,
137.827206888297));
#42799=CARTESIAN_POINT('Ctrl Pts',(-6.14339426990799,-2.84270243767562,
137.8353406585));
#42800=CARTESIAN_POINT('Ctrl Pts',(-6.06671130901988,-2.99788306860195,
137.843474428703));
#42801=CARTESIAN_POINT('Ctrl Pts',(-5.9900851575855,-3.15294873622001,137.851602173121));
#42802=CARTESIAN_POINT('Ctrl Pts',(-5.90744676789015,-3.30520234622276,
137.859729917539));
#42803=CARTESIAN_POINT('Ctrl Pts',(-5.81903473287829,-3.45414588249484,
137.867857661957));
#42804=CARTESIAN_POINT('Ctrl Pts',(-5.73066960866939,-3.60301039037583,
137.875981093851));
#42805=CARTESIAN_POINT('Ctrl Pts',(-5.63653712633621,-3.74856800846109,
137.884104525745));
#42806=CARTESIAN_POINT('Ctrl Pts',(-5.53692196945519,-3.89034498523774,
137.89222795764));
#42807=CARTESIAN_POINT('Ctrl Pts',(-5.43667489320057,-4.03302133938991,
137.90040292139));
#42808=CARTESIAN_POINT('Ctrl Pts',(-5.330875513871,-4.17186858700254,137.908577885141));
#42809=CARTESIAN_POINT('Ctrl Pts',(-5.21985875539365,-4.30643281309952,
137.916752848892));
#42810=CARTESIAN_POINT('Ctrl Pts',(-5.10956682858407,-4.44011846542296,
137.924874438065));
#42811=CARTESIAN_POINT('Ctrl Pts',(-4.99412570466661,-4.56957658910254,
137.932996027238));
#42812=CARTESIAN_POINT('Ctrl Pts',(-4.87390450601608,-4.69439494144199,
137.941117616411));
#42813=CARTESIAN_POINT('Ctrl Pts',(-4.75366743570169,-4.81922977236388,
137.9492402778));
#42814=CARTESIAN_POINT('Ctrl Pts',(-4.62864928759518,-4.93942334823802,
137.95736293919));
#42815=CARTESIAN_POINT('Ctrl Pts',(-4.49925625483112,-5.05460009826327,
137.965485600579));
#42816=CARTESIAN_POINT('Ctrl Pts',(-4.36982149927201,-5.16981398704192,
137.973610881121));
#42817=CARTESIAN_POINT('Ctrl Pts',(-4.23600932318569,-5.28000758547039,
137.981736161664));
#42818=CARTESIAN_POINT('Ctrl Pts',(-4.09825916716812,-5.38484547584445,
137.989861442206));
#42819=CARTESIAN_POINT('Ctrl Pts',(-3.95900825178452,-5.49082555327981,
137.998075245994));
#42820=CARTESIAN_POINT('Ctrl Pts',(-3.81573335245716,-5.59133230767598,
138.006289049781));
#42821=CARTESIAN_POINT('Ctrl Pts',(-3.66891787395882,-5.68606459989205,
138.014502853569));
#42822=CARTESIAN_POINT('Ctrl Pts',(-3.52343336359155,-5.77993808850503,
138.022642194424));
#42823=CARTESIAN_POINT('Ctrl Pts',(-3.37447255167075,-5.86814125164929,
138.03078153528));
#42824=CARTESIAN_POINT('Ctrl Pts',(-3.22252959690908,-5.95042788352611,
138.038920876135));
#42825=CARTESIAN_POINT('Ctrl Pts',(-3.06850156212743,-6.03384371690035,
138.047171911389));
#42826=CARTESIAN_POINT('Ctrl Pts',(-2.91140929657605,-6.11117928556882,
138.055422946643));
#42827=CARTESIAN_POINT('Ctrl Pts',(-2.7517870228635,-6.18222914334304,138.063673981897));
#42828=CARTESIAN_POINT('Ctrl Pts',(-2.59216474915094,-6.25327900111727,
138.071925017151));
#42829=CARTESIAN_POINT('Ctrl Pts',(-2.43001284864779,-6.31804306789245,
138.080176052405));
#42830=CARTESIAN_POINT('Ctrl Pts',(-2.26587948645026,-6.37636880621596,
138.088427087659));
#42831=CARTESIAN_POINT('Ctrl Pts',(-2.10212931708763,-6.43455837475218,
138.09665885969));
#42832=CARTESIAN_POINT('Ctrl Pts',(-1.93589578800268,-6.4865214679517,138.104890631721));
#42833=CARTESIAN_POINT('Ctrl Pts',(-1.76769268313256,-6.53204038398414,
138.113122403752));
#42834=CARTESIAN_POINT('Ctrl Pts',(-1.59969042957885,-6.57750494588195,
138.121344346224));
#42835=CARTESIAN_POINT('Ctrl Pts',(-1.42972362582028,-6.61654056044007,
138.129566288696));
#42836=CARTESIAN_POINT('Ctrl Pts',(-1.25832510178768,-6.64897788672898,
138.137788231169));
#42837=CARTESIAN_POINT('Ctrl Pts',(-1.08709690351991,-6.68138297871226,
138.146002003159));
#42838=CARTESIAN_POINT('Ctrl Pts',(-0.914440168031664,-6.70720277447715,
138.154215775149));
#42839=CARTESIAN_POINT('Ctrl Pts',(-0.740902019958573,-6.72631795240318,
138.162429547139));
#42840=CARTESIAN_POINT('Ctrl Pts',(-0.567501566619891,-6.74541796329316,
138.170636801869));
#42841=CARTESIAN_POINT('Ctrl Pts',(-0.393221448224845,-6.75782391320529,
138.178844056599));
#42842=CARTESIAN_POINT('Ctrl Pts',(-0.218618191936567,-6.76346768205145,
138.18705131133));
#42843=CARTESIAN_POINT('Ctrl Pts',(-0.0441185140205303,-6.76910810289367,
138.195253697342));
#42844=CARTESIAN_POINT('Ctrl Pts',(0.130703562748177,-6.76799432244862,
138.203456083354));
#42845=CARTESIAN_POINT('Ctrl Pts',(0.305287093792983,-6.76011011673356,
138.211658469366));
#42846=CARTESIAN_POINT('Ctrl Pts',(0.479818515888508,-6.75222826426267,
138.219858407164));
#42847=CARTESIAN_POINT('Ctrl Pts',(0.654111176415007,-6.73758002415768,
138.228058344963));
#42848=CARTESIAN_POINT('Ctrl Pts',(0.827604583781613,-6.71620128144651,
138.236258282762));
#42849=CARTESIAN_POINT('Ctrl Pts',(1.00107373229203,-6.69482552803535,138.244457073997));
#42850=CARTESIAN_POINT('Ctrl Pts',(1.17374349451156,-6.66672118934978,138.252655865233));
#42851=CARTESIAN_POINT('Ctrl Pts',(1.34505892949523,-6.63197598579678,138.260854656469));
#42852=CARTESIAN_POINT('Ctrl Pts',(1.51638148766872,-6.5972293375597,138.269053788605));
#42853=CARTESIAN_POINT('Ctrl Pts',(1.68634925510853,-6.55584134552222,138.277252920742));
#42854=CARTESIAN_POINT('Ctrl Pts',(1.85441784894717,-6.50795078665367,138.285452052878));
#42855=CARTESIAN_POINT('Ctrl Pts',(2.02252391937709,-6.46004954896132,138.293653013289));
#42856=CARTESIAN_POINT('Ctrl Pts',(2.18872962810827,-6.40564295472346,138.3018539737));
#42857=CARTESIAN_POINT('Ctrl Pts',(2.35250605513895,-6.34491956296804,138.310054934111));
#42858=CARTESIAN_POINT('Ctrl Pts',(2.51643598010764,-6.28413925877662,138.318263580796));
#42859=CARTESIAN_POINT('Ctrl Pts',(2.6779317379114,-6.21703045331984,138.326472227481));
#42860=CARTESIAN_POINT('Ctrl Pts',(2.83648381696526,-6.14383012103152,138.334680874166));
#42861=CARTESIAN_POINT('Ctrl Pts',(2.99511159323484,-6.07059484084863,138.34289343989));
#42862=CARTESIAN_POINT('Ctrl Pts',(3.15079256944966,-5.99126239789787,138.351106005613));
#42863=CARTESIAN_POINT('Ctrl Pts',(3.3030422132211,-5.90611557097213,138.359318571337));
#42864=CARTESIAN_POINT('Ctrl Pts',(3.4555007654734,-5.82085191031318,138.367542405885));
#42865=CARTESIAN_POINT('Ctrl Pts',(3.60451826961661,-5.72975810790641,138.375766240434));
#42866=CARTESIAN_POINT('Ctrl Pts',(3.74963850414986,-5.63316075469153,138.383990074983));
#42867=CARTESIAN_POINT('Ctrl Pts',(3.88297670128961,-5.54440595790133,138.391546231957));
#42868=CARTESIAN_POINT('Ctrl Pts',(4.0130249464866,-5.45100559476595,138.399102388932));
#42869=CARTESIAN_POINT('Ctrl Pts',(4.13945490553084,-5.3532422031024,138.406658545906));
#42870=CARTESIAN_POINT('Ctrl Pts',(4.28411544963616,-5.24138180594225,138.415304263959));
#42871=CARTESIAN_POINT('Ctrl Pts',(4.42436852531527,-5.12355421362863,138.423949982011));
#42872=CARTESIAN_POINT('Ctrl Pts',(4.55972131160622,-5.00012305453416,138.432595700064));
#42873=CARTESIAN_POINT('Ctrl Pts',(4.69490033250359,-4.87685035589351,138.441230318776));
#42874=CARTESIAN_POINT('Ctrl Pts',(4.82519138426705,-4.74798863987478,138.449864937488));
#42875=CARTESIAN_POINT('Ctrl Pts',(4.95013382671809,-4.61394235958592,138.458499556201));
#42876=CARTESIAN_POINT('Ctrl Pts',(5.07948875087282,-4.47516208540662,138.467439116103));
#42877=CARTESIAN_POINT('Ctrl Pts',(5.20311011490759,-4.33082453966867,138.476378676005));
#42878=CARTESIAN_POINT('Ctrl Pts',(5.32052523390524,-4.18142323083632,138.485318235908));
#42879=CARTESIAN_POINT('Ctrl Pts',(5.43362038505844,-4.03751873413159,138.493928889178));
#42880=CARTESIAN_POINT('Ctrl Pts',(5.54095757740913,-3.88891668735461,138.502539542449));
#42881=CARTESIAN_POINT('Ctrl Pts',(5.64215238935616,-3.73609494195244,138.511150195719));
#42882=CARTESIAN_POINT('Ctrl Pts',(5.74325141364355,-3.58341785255637,138.51975269843));
#42883=CARTESIAN_POINT('Ctrl Pts',(5.83821948159534,-3.42652928140618,138.528355201141));
#42884=CARTESIAN_POINT('Ctrl Pts',(5.92671367097066,-3.26593846579043,138.536957703852));
#42885=CARTESIAN_POINT('Ctrl Pts',(6.01510826191704,-3.10552839190528,138.54555052462));
#42886=CARTESIAN_POINT('Ctrl Pts',(6.09704336319448,-2.94142465275138,138.554143345387));
#42887=CARTESIAN_POINT('Ctrl Pts',(6.172220347804,-2.77416383405058,138.562736166155));
#42888=CARTESIAN_POINT('Ctrl Pts',(6.18108029691207,-2.75445138682809,138.563748869113));
#42889=CARTESIAN_POINT('Ctrl Pts',(6.18984642887871,-2.73469511937173,138.564761572071));
#42890=CARTESIAN_POINT('Ctrl Pts',(6.19851829608991,-2.71489593410845,138.565774275029));
#42891=CARTESIAN_POINT('Ctrl Pts',(6.27212026727549,-2.5468514948022,138.574369532789));
#42892=CARTESIAN_POINT('Ctrl Pts',(6.33884127528107,-2.3759112722682,138.582964790549));
#42893=CARTESIAN_POINT('Ctrl Pts',(6.39848336877615,-2.20265739040257,138.591560048309));
#42894=CARTESIAN_POINT('Ctrl Pts',(6.45818131456241,-2.02924126362413,138.600163355164));
#42895=CARTESIAN_POINT('Ctrl Pts',(6.51078701450223,-1.85350744152906,138.608766662018));
#42896=CARTESIAN_POINT('Ctrl Pts',(6.55615266914944,-1.67605226016515,138.617369968872));
#42897=CARTESIAN_POINT('Ctrl Pts',(6.6033991995701,-1.49123972544446,138.626329971812));
#42898=CARTESIAN_POINT('Ctrl Pts',(6.64279246110562,-1.30456042620896,138.635289974752));
#42899=CARTESIAN_POINT('Ctrl Pts',(6.67422477828092,-1.11669718768384,138.644249977692));
#42900=CARTESIAN_POINT('Ctrl Pts',(6.70448834779617,-0.935819266824322,
138.652876820897));
#42901=CARTESIAN_POINT('Ctrl Pts',(6.72737233016089,-0.753844163263907,
138.661503664102));
#42902=CARTESIAN_POINT('Ctrl Pts',(6.74283385906733,-0.571384764423357,
138.670130507306));
#42903=CARTESIAN_POINT('Ctrl Pts',(6.75831016528702,-0.388750980520001,
138.678765595593));
#42904=CARTESIAN_POINT('Ctrl Pts',(6.76634984139253,-0.205632281804545,
138.687400683879));
#42905=CARTESIAN_POINT('Ctrl Pts',(6.76696212040592,-0.0226420182733682,
138.696035772165));
#42906=CARTESIAN_POINT('Ctrl Pts',(6.76757530877651,0.160620022521937,138.70468368529));
#42907=CARTESIAN_POINT('Ctrl Pts',(6.76073906296994,0.343752942058419,138.713331598415));
#42908=CARTESIAN_POINT('Ctrl Pts',(6.74651456775601,0.526146545228584,138.72197951154));
#42909=CARTESIAN_POINT('Ctrl Pts',(6.74491879593467,0.546608330898569,138.722949675744));
#42910=CARTESIAN_POINT('Ctrl Pts',(6.74323009309983,0.567060820849754,138.723919839948));
#42911=CARTESIAN_POINT('Ctrl Pts',(6.74144858588057,0.587503160781988,138.724890004153));
#42912=CARTESIAN_POINT('Ctrl Pts',(6.72634565188616,0.760805467587939,138.733114683671));
#42913=CARTESIAN_POINT('Ctrl Pts',(6.70453590366463,0.933753406765605,138.74133936319));
#42914=CARTESIAN_POINT('Ctrl Pts',(6.67604077222952,1.10578868122673,138.749564042709));
#42915=CARTESIAN_POINT('Ctrl Pts',(6.64757559240127,1.27764312715159,138.757780077159));
#42916=CARTESIAN_POINT('Ctrl Pts',(6.61243908087821,1.44858646800505,138.765996111609));
#42917=CARTESIAN_POINT('Ctrl Pts',(6.57070455705608,1.61806385037256,138.774212146059));
#42918=CARTESIAN_POINT('Ctrl Pts',(6.52900554144138,1.78739703945603,138.782421190214));
#42919=CARTESIAN_POINT('Ctrl Pts',(6.48071977902235,1.95526640804378,138.790630234369));
#42920=CARTESIAN_POINT('Ctrl Pts',(6.42597194211774,2.12112555005959,138.798839278523));
#42921=CARTESIAN_POINT('Ctrl Pts',(6.37125972230467,2.28687678972565,138.807042982151));
#42922=CARTESIAN_POINT('Ctrl Pts',(6.3100939139596,2.45062006867249,138.815246685779));
#42923=CARTESIAN_POINT('Ctrl Pts',(6.24264951638908,2.61182235527747,138.823450389408));
#42924=CARTESIAN_POINT('Ctrl Pts',(6.17523549319343,2.77295204254347,138.831650398402));
#42925=CARTESIAN_POINT('Ctrl Pts',(6.10154865225163,2.93154268739914,138.839850407395));
#42926=CARTESIAN_POINT('Ctrl Pts',(6.021812813575,3.08707943504277,138.848050416389));
#42927=CARTESIAN_POINT('Ctrl Pts',(5.94208335074426,3.24260374563989,138.856249769693));
#42928=CARTESIAN_POINT('Ctrl Pts',(5.85630600922196,3.3950743227376,138.864449122997));
#42929=CARTESIAN_POINT('Ctrl Pts',(5.76475160007908,3.54399886983415,138.872648476301));
#42930=CARTESIAN_POINT('Ctrl Pts',(5.67319778784387,3.69292244598668,138.880847776148));
#42931=CARTESIAN_POINT('Ctrl Pts',(5.5758671698464,3.83829973220239,138.889047075995));
#42932=CARTESIAN_POINT('Ctrl Pts',(5.47307505995551,3.97966561259774,138.897246375841));
#42933=CARTESIAN_POINT('Ctrl Pts',(5.37026497274139,4.12105621648725,138.905447109664));
#42934=CARTESIAN_POINT('Ctrl Pts',(5.26199170148207,4.25843372685605,138.913647843487));
#42935=CARTESIAN_POINT('Ctrl Pts',(5.14861221183529,4.39136439983527,138.92184857731));
#42936=CARTESIAN_POINT('Ctrl Pts',(5.03519232486205,4.52434243626452,138.93005223307));
#42937=CARTESIAN_POINT('Ctrl Pts',(4.91666282776165,4.65287020646299,138.93825588883));
#42938=CARTESIAN_POINT('Ctrl Pts',(4.79341908311819,4.77654922445047,138.94645954459));
#42939=CARTESIAN_POINT('Ctrl Pts',(4.67003415484269,4.90036992470359,138.954672598165));
#42940=CARTESIAN_POINT('Ctrl Pts',(4.54192444304752,5.01933052138917,138.96288565174));
#42941=CARTESIAN_POINT('Ctrl Pts',(4.4095208755519,5.13307068411024,138.971098705315));
#42942=CARTESIAN_POINT('Ctrl Pts',(4.27703896189472,5.24687814943753,138.979316618739));
#42943=CARTESIAN_POINT('Ctrl Pts',(4.1402584081641,5.35545880063626,138.987534532162));
#42944=CARTESIAN_POINT('Ctrl Pts',(3.99964084713923,5.45849448968261,138.995752445585));
#42945=CARTESIAN_POINT('Ctrl Pts',(3.85880397015197,5.5616908796481,139.003983176181));
#42946=CARTESIAN_POINT('Ctrl Pts',(3.71411842340981,5.65932482410708,139.012213906777));
#42947=CARTESIAN_POINT('Ctrl Pts',(3.56607341546888,5.75112244657389,139.020444637373));
#42948=CARTESIAN_POINT('Ctrl Pts',(3.43011178152382,5.83542758402129,139.028003579048));
#42949=CARTESIAN_POINT('Ctrl Pts',(3.2913171798409,5.91481066982111,139.035562520724));
#42950=CARTESIAN_POINT('Ctrl Pts',(3.15008384884486,5.98909515246225,139.0431214624));
#42951=CARTESIAN_POINT('Ctrl Pts',(3.13315510240313,5.99799916373436,139.044027504947));
#42952=CARTESIAN_POINT('Ctrl Pts',(3.11618552915106,6.00683301543969,139.044933547494));
#42953=CARTESIAN_POINT('Ctrl Pts',(3.09917575053254,6.01559628526642,139.045839590042));
#42954=CARTESIAN_POINT('Ctrl Pts',(3.09917575053248,6.01559628526645,137.045751582743));
#42955=CARTESIAN_POINT('Ctrl Pts',(2.93382384459259,6.10078395293762,137.054501030655));
#42956=CARTESIAN_POINT('Ctrl Pts',(2.76495772122983,6.17915010267049,137.063250478567));
#42957=CARTESIAN_POINT('Ctrl Pts',(2.59315093316716,6.25042856433175,137.07199992648));
#42958=CARTESIAN_POINT('Ctrl Pts',(2.42134553245626,6.32170645041447,137.08074930374));
#42959=CARTESIAN_POINT('Ctrl Pts',(2.24659977927604,6.38589665313452,137.089498681));
#42960=CARTESIAN_POINT('Ctrl Pts',(2.06950718689937,6.44278115439069,137.09824805826));
#42961=CARTESIAN_POINT('Ctrl Pts',(1.89241596572871,6.49966521519721,137.106997367774));
#42962=CARTESIAN_POINT('Ctrl Pts',(1.712978214572,6.54924360009546,137.115746677289));
#42963=CARTESIAN_POINT('Ctrl Pts',(1.53180337335838,6.59134792173557,137.124495986804));
#42964=CARTESIAN_POINT('Ctrl Pts',(1.35062987477788,6.63345193135303,137.13324523148));
#42965=CARTESIAN_POINT('Ctrl Pts',(1.16771959102968,6.66808192368235,137.141994476156));
#42966=CARTESIAN_POINT('Ctrl Pts',(0.983693746907124,6.69512028363164,137.150743720832));
#42967=CARTESIAN_POINT('Ctrl Pts',(0.799669205420131,6.72215845218864,137.159492903576));
#42968=CARTESIAN_POINT('Ctrl Pts',(0.614529402873715,6.74160505424577,137.16824208632));
#42969=CARTESIAN_POINT('Ctrl Pts',(0.428903127363467,6.75339404354121,137.176991269065));
#42970=CARTESIAN_POINT('Ctrl Pts',(0.243278104163973,6.7651829533033,137.185740392783));
#42971=CARTESIAN_POINT('Ctrl Pts',(0.0571669005390867,6.76931433552276,
137.194489516502));
#42972=CARTESIAN_POINT('Ctrl Pts',(-0.128798404777669,6.76577415902473,
137.20323864022));
#42973=CARTESIAN_POINT('Ctrl Pts',(-0.314762517259109,6.76223400523441,
137.21198770782));
#42974=CARTESIAN_POINT('Ctrl Pts',(-0.500580446819374,6.7510223966509,137.220736775419));
#42975=CARTESIAN_POINT('Ctrl Pts',(-0.685621118842331,6.732177410125,137.229485843018));
#42976=CARTESIAN_POINT('Ctrl Pts',(-0.870660665414054,6.71333253821777,
137.238234857404));
#42977=CARTESIAN_POINT('Ctrl Pts',(-1.05492267885428,6.68685441030621,137.24698387179));
#42978=CARTESIAN_POINT('Ctrl Pts',(-1.23778137635178,6.65283295028191,137.255732886175));
#42979=CARTESIAN_POINT('Ctrl Pts',(-1.4299992297876,6.61707018861884,137.264929696543));
#42980=CARTESIAN_POINT('Ctrl Pts',(-1.62066601233596,6.57297172934437,137.27412650691));
#42981=CARTESIAN_POINT('Ctrl Pts',(-1.80906628500274,6.52070304311325,137.283323317278));
#42982=CARTESIAN_POINT('Ctrl Pts',(-1.98831342545419,6.47097374915064,137.292073315015));
#42983=CARTESIAN_POINT('Ctrl Pts',(-2.16550875896596,6.41384933989564,137.300823312753));
#42984=CARTESIAN_POINT('Ctrl Pts',(-2.34005036713908,6.34952386240514,137.309573310491));
#42985=CARTESIAN_POINT('Ctrl Pts',(-2.51458843546987,6.28519968948637,137.318323130772));
#42986=CARTESIAN_POINT('Ctrl Pts',(-2.68647261717955,6.21367483971142,137.327072951053));
#42987=CARTESIAN_POINT('Ctrl Pts',(-2.85511905908633,6.1351922674389,137.335822771333));
#42988=CARTESIAN_POINT('Ctrl Pts',(-3.02376230488794,6.05671118252982,137.344572425792));
#42989=CARTESIAN_POINT('Ctrl Pts',(-3.18916767379822,5.97127275992677,137.35332208025));
#42990=CARTESIAN_POINT('Ctrl Pts',(-3.35077334102712,5.87916720438039,137.362071734709));
#42991=CARTESIAN_POINT('Ctrl Pts',(-3.51237616037281,5.78706327195695,137.370821234977));
#42992=CARTESIAN_POINT('Ctrl Pts',(-3.67017916302202,5.68829258362361,137.379570735246));
#42993=CARTESIAN_POINT('Ctrl Pts',(-3.82364636566355,5.58319061741116,137.388320235514));
#42994=CARTESIAN_POINT('Ctrl Pts',(-3.97711106778689,5.47809036367781,137.397069593223));
#42995=CARTESIAN_POINT('Ctrl Pts',(-4.12623987481817,5.3666592004331,137.405818950931));
#42996=CARTESIAN_POINT('Ctrl Pts',(-4.27052628213818,5.24927559512425,137.41456830864));
#42997=CARTESIAN_POINT('Ctrl Pts',(-4.41481053024877,5.13189374643124,137.423317535416));
#42998=CARTESIAN_POINT('Ctrl Pts',(-4.55425230136438,5.00855981477437,137.432066762193));
#42999=CARTESIAN_POINT('Ctrl Pts',(-4.68837800630465,4.87969268192156,137.440815988969));
#43000=CARTESIAN_POINT('Ctrl Pts',(-4.8225018822883,4.75082730631876,137.44956509644));
#43001=CARTESIAN_POINT('Ctrl Pts',(-4.95130963052918,4.61642907903578,137.458314203911));
#43002=CARTESIAN_POINT('Ctrl Pts',(-5.07436379033335,4.47695444731725,137.467063311382));
#43003=CARTESIAN_POINT('Ctrl Pts',(-5.19741643562774,4.33748153220623,137.475812311171));
#43004=CARTESIAN_POINT('Ctrl Pts',(-5.31471544462743,4.19293255254628,137.484561310961));
#43005=CARTESIAN_POINT('Ctrl Pts',(-5.42586245275597,4.04379841779643,137.493310310751));
#43006=CARTESIAN_POINT('Ctrl Pts',(-5.53702160019118,3.89464799484392,137.502060266093));
#43007=CARTESIAN_POINT('Ctrl Pts',(-5.64202723081213,3.74091164443907,137.510810221435));
#43008=CARTESIAN_POINT('Ctrl Pts',(-5.74052265232925,3.58311159163299,137.519560176777));
#43009=CARTESIAN_POINT('Ctrl Pts',(-5.83901427066878,3.42531763191851,137.52830979426));
#43010=CARTESIAN_POINT('Ctrl Pts',(-5.93099603115702,3.26346052695681,137.537059411742));
#43011=CARTESIAN_POINT('Ctrl Pts',(-6.01615550622718,3.09809004467146,137.545809029225));
#43012=CARTESIAN_POINT('Ctrl Pts',(-6.10131214578762,2.93272506863905,137.554558355376));
#43013=CARTESIAN_POINT('Ctrl Pts',(-6.17964682328709,2.7638472041698,137.563307681527));
#43014=CARTESIAN_POINT('Ctrl Pts',(-6.25089348288525,2.59203002791687,137.572057007678));
#43015=CARTESIAN_POINT('Ctrl Pts',(-6.32213814889304,2.42021765937099,137.58080608901));
#43016=CARTESIAN_POINT('Ctrl Pts',(-6.3862950841257,2.24546640831963,137.589555170341));
#43017=CARTESIAN_POINT('Ctrl Pts',(-6.44314639819805,2.06836976660061,137.598304251673));
#43018=CARTESIAN_POINT('Ctrl Pts',(-6.50000285283698,1.89125711158286,137.607054124107));
#43019=CARTESIAN_POINT('Ctrl Pts',(-6.5495522767325,1.71179891440255,137.615803996542));
#43020=CARTESIAN_POINT('Ctrl Pts',(-6.59162635926387,1.53060476278421,137.624553868976));
#43021=CARTESIAN_POINT('Ctrl Pts',(-6.63369752055196,1.34942319164695,137.633303133899));
#43022=CARTESIAN_POINT('Ctrl Pts',(-6.66829431424252,1.16650618642713,137.642052398821));
#43023=CARTESIAN_POINT('Ctrl Pts',(-6.69529923745415,0.982474997618747,
137.650801663743));
#43024=CARTESIAN_POINT('Ctrl Pts',(-6.72230554731441,0.798434359177943,
137.659551377923));
#43025=CARTESIAN_POINT('Ctrl Pts',(-6.74171916496701,0.613279706240553,
137.668301092103));
#43026=CARTESIAN_POINT('Ctrl Pts',(-6.75347414817274,0.427639953655605,
137.677050806283));
#43027=CARTESIAN_POINT('Ctrl Pts',(-6.7624883775873,0.285283364200971,137.683760465458));
#43028=CARTESIAN_POINT('Ctrl Pts',(-6.76699999999983,0.142641701109694,
137.690470124634));
#43029=CARTESIAN_POINT('Ctrl Pts',(-6.767,8.32090660346834E-12,137.69717978381));
#43030=CARTESIAN_POINT('',(-6.76699997222249,0.000613140130776506,137.302820216215));
#43031=CARTESIAN_POINT('Ctrl Pts',(3.0991757505325,6.01559628526643,136.651412426306));
#43032=CARTESIAN_POINT('Ctrl Pts',(3.07449030807931,6.02831398123773,136.652724932637));
#43033=CARTESIAN_POINT('Ctrl Pts',(3.04972988437511,6.04087802633221,136.654037438968));
#43034=CARTESIAN_POINT('Ctrl Pts',(3.02489644499519,6.05328757759413,136.655349945299));
#43035=CARTESIAN_POINT('Ctrl Pts',(2.86925552937279,6.1310631080521,136.663575937841));
#43036=CARTESIAN_POINT('Ctrl Pts',(2.71040878682656,6.2029341524034,136.671801930382));
#43037=CARTESIAN_POINT('Ctrl Pts',(2.54884354114607,6.26862709073988,136.680027922924));
#43038=CARTESIAN_POINT('Ctrl Pts',(2.38744767574249,6.33425115852169,136.688245291575));
#43039=CARTESIAN_POINT('Ctrl Pts',(2.22333931178423,6.39370988444081,136.696462660226));
#43040=CARTESIAN_POINT('Ctrl Pts',(2.05702995467596,6.44677568754845,136.704680028878));
#43041=CARTESIAN_POINT('Ctrl Pts',(1.89086167365069,6.49979647625779,136.71289042694));
#43042=CARTESIAN_POINT('Ctrl Pts',(1.72249645736861,6.54643503440276,136.721100825003));
#43043=CARTESIAN_POINT('Ctrl Pts',(1.55246544864081,6.58651197757785,136.729311223065));
#43044=CARTESIAN_POINT('Ctrl Pts',(1.38254466009271,6.62656294144534,136.737516298854));
#43045=CARTESIAN_POINT('Ctrl Pts',(1.21096057751938,6.66006068105089,136.745721374643));
#43046=CARTESIAN_POINT('Ctrl Pts',(1.03825924602322,6.68687570828465,136.753926450431));
#43047=CARTESIAN_POINT('Ctrl Pts',(0.865635325669229,6.71367871602865,136.762127848401));
#43048=CARTESIAN_POINT('Ctrl Pts',(0.691895507423722,6.73380492433716,136.77032924637));
#43049=CARTESIAN_POINT('Ctrl Pts',(0.517595858989442,6.7471759667847,136.77853064434));
#43050=CARTESIAN_POINT('Ctrl Pts',(0.343309863154941,6.76054596190086,136.786731399908));
#43051=CARTESIAN_POINT('Ctrl Pts',(0.168464480763489,6.76716180902418,136.794932155475));
#43052=CARTESIAN_POINT('Ctrl Pts',(-0.00637888808444536,6.76699699348144,
136.803132911043));
#43053=CARTESIAN_POINT('Ctrl Pts',(-0.181221368811281,6.76683217877588,
136.811333624955));
#43054=CARTESIAN_POINT('Ctrl Pts',(-0.356061477640533,6.75988676928104,
136.819534338867));
#43055=CARTESIAN_POINT('Ctrl Pts',(-0.530337721449143,6.74618639686217,
136.827735052778));
#43056=CARTESIAN_POINT('Ctrl Pts',(-0.704644663212336,6.73248361118603,
136.835937211208));
#43057=CARTESIAN_POINT('Ctrl Pts',(-0.878387184796682,6.71202352008909,
136.844139369638));
#43058=CARTESIAN_POINT('Ctrl Pts',(-1.05100876161048,6.68488366263902,136.852341528067));
#43059=CARTESIAN_POINT('Ctrl Pts',(-1.2236920285752,6.65773410615866,136.86054661772));
#43060=CARTESIAN_POINT('Ctrl Pts',(-1.3952531989625,6.62390008358326,136.868751707373));
#43061=CARTESIAN_POINT('Ctrl Pts',(-1.56514572896263,6.58351029824592,136.876956797026));
#43062=CARTESIAN_POINT('Ctrl Pts',(-1.73523234109187,6.54307437235411,136.885171260024));
#43063=CARTESIAN_POINT('Ctrl Pts',(-1.90364615552444,6.49606780460035,136.893385723022));
#43064=CARTESIAN_POINT('Ctrl Pts',(-2.06985456410139,6.44266956187175,136.901600186019));
#43065=CARTESIAN_POINT('Ctrl Pts',(-2.23616144590738,6.38923968237198,136.909819515827));
#43066=CARTESIAN_POINT('Ctrl Pts',(-2.40025998110839,6.32941070176852,136.918038845634));
#43067=CARTESIAN_POINT('Ctrl Pts',(-2.56163746254934,6.26340981498606,136.926258175442));
#43068=CARTESIAN_POINT('Ctrl Pts',(-2.72326498861374,6.19730666383107,136.934490240602));
#43069=CARTESIAN_POINT('Ctrl Pts',(-2.88216270952051,6.12501264421115,136.942722305763));
#43070=CARTESIAN_POINT('Ctrl Pts',(-3.03784124961139,6.04680159606378,136.950954370924));
#43071=CARTESIAN_POINT('Ctrl Pts',(-3.17777629977712,5.97649989012777,136.958353942185));
#43072=CARTESIAN_POINT('Ctrl Pts',(-3.31511053933854,5.90141810395166,136.965753513446));
#43073=CARTESIAN_POINT('Ctrl Pts',(-3.44950926018174,5.82178450854379,136.973153084707));
#43074=CARTESIAN_POINT('Ctrl Pts',(-3.59763719071756,5.73401611599594,136.981308543114));
#43075=CARTESIAN_POINT('Ctrl Pts',(-3.74265481063443,5.64044748463279,136.989464001521));
#43076=CARTESIAN_POINT('Ctrl Pts',(-3.88407107074503,5.54132483413503,136.997619459927));
#43077=CARTESIAN_POINT('Ctrl Pts',(-4.0253152086782,5.44232282893239,137.005764992069));
#43078=CARTESIAN_POINT('Ctrl Pts',(-4.16296641600805,5.33778046811054,137.013910524211));
#43079=CARTESIAN_POINT('Ctrl Pts',(-4.29655805699752,5.22798984915328,137.022056056353));
#43080=CARTESIAN_POINT('Ctrl Pts',(-4.43001519104161,5.11830977304643,137.030193387154));
#43081=CARTESIAN_POINT('Ctrl Pts',(-4.55942061573056,5.00339218907516,137.038330717954));
#43082=CARTESIAN_POINT('Ctrl Pts',(-4.68433653653444,4.88357248461498,137.046468048755));
#43083=CARTESIAN_POINT('Ctrl Pts',(-4.80915293702246,4.76384824032318,137.054598896557));
#43084=CARTESIAN_POINT('Ctrl Pts',(-4.92948669289416,4.63922990373686,137.062729744359));
#43085=CARTESIAN_POINT('Ctrl Pts',(-5.04493299719119,4.51009313139446,137.070860592161));
#43086=CARTESIAN_POINT('Ctrl Pts',(-5.16031157709498,4.38103211469973,137.078986670155));
#43087=CARTESIAN_POINT('Ctrl Pts',(-5.27080817226869,4.24745821278198,137.087112748148));
#43088=CARTESIAN_POINT('Ctrl Pts',(-5.37605478581504,4.10978392861659,137.095238826142));
#43089=CARTESIAN_POINT('Ctrl Pts',(-5.48167458463072,3.97162147658447,137.103393717724));
#43090=CARTESIAN_POINT('Ctrl Pts',(-5.58200683845017,3.82932977235232,137.111548609306));
#43091=CARTESIAN_POINT('Ctrl Pts',(-5.67672003015765,3.68335970266372,137.119703500889));
#43092=CARTESIAN_POINT('Ctrl Pts',(-5.7710638735329,3.53795886521006,137.127826591245));
#43093=CARTESIAN_POINT('Ctrl Pts',(-5.85983221476445,3.38890861778875,137.135949681601));
#43094=CARTESIAN_POINT('Ctrl Pts',(-5.94274068696559,3.23668381642133,137.144072771957));
#43095=CARTESIAN_POINT('Ctrl Pts',(-6.02565566951855,3.08444706166741,137.152196500176));
#43096=CARTESIAN_POINT('Ctrl Pts',(-6.10270969147033,2.92903557768013,137.160320228394));
#43097=CARTESIAN_POINT('Ctrl Pts',(-6.17366436725664,2.77094880509649,137.168443956613));
#43098=CARTESIAN_POINT('Ctrl Pts',(-6.24463811377077,2.61281954299714,137.176569868273));
#43099=CARTESIAN_POINT('Ctrl Pts',(-6.30950910014755,2.45201389415588,137.184695779933));
#43100=CARTESIAN_POINT('Ctrl Pts',(-6.3680871204253,2.28905120665165,137.192821691594));
#43101=CARTESIAN_POINT('Ctrl Pts',(-6.42703975323206,2.12504635582046,137.200999569304));
#43102=CARTESIAN_POINT('Ctrl Pts',(-6.47961852516843,1.95885713505044,137.209177447014));
#43103=CARTESIAN_POINT('Ctrl Pts',(-6.52568076147207,1.79102752612945,137.217355324724));
#43104=CARTESIAN_POINT('Ctrl Pts',(-6.57152315271205,1.62399893153206,137.225494171198));
#43105=CARTESIAN_POINT('Ctrl Pts',(-6.61091105274013,1.45534594316093,137.233633017671));
#43106=CARTESIAN_POINT('Ctrl Pts',(-6.64375543029131,1.28561377655762,137.241771864144));
#43107=CARTESIAN_POINT('Ctrl Pts',(-6.67683607412608,1.11466064030292,137.249969257473));
#43108=CARTESIAN_POINT('Ctrl Pts',(-6.7032786414045,0.942613114501291,137.258166650801));
#43109=CARTESIAN_POINT('Ctrl Pts',(-6.72304544005497,0.770031824638522,
137.26636404413));
#43110=CARTESIAN_POINT('Ctrl Pts',(-6.74281223870545,0.597450534775627,
137.274561437458));
#43111=CARTESIAN_POINT('Ctrl Pts',(-6.75590330159673,0.424335856632697,
137.282758830787));
#43112=CARTESIAN_POINT('Ctrl Pts',(-6.76233423306537,0.251246333927945,
137.290956224115));
#43113=CARTESIAN_POINT('Ctrl Pts',(-6.7654367038518,0.167742849207789,137.29491088814));
#43114=CARTESIAN_POINT('Ctrl Pts',(-6.76699239991745,0.0841857874934056,
137.298865552165));
#43115=CARTESIAN_POINT('Ctrl Pts',(-6.76699997222244,0.000613140658257255,
137.30282021619));
#43116=CARTESIAN_POINT('Ctrl Pts',(-6.76699997222249,0.000613140130961323,
137.302820216215));
#43117=CARTESIAN_POINT('Ctrl Pts',(-6.76701562449587,-0.172135189647376,
137.310994680361));
#43118=CARTESIAN_POINT('Ctrl Pts',(-6.7604121071467,-0.345139132386608,
137.319169144507));
#43119=CARTESIAN_POINT('Ctrl Pts',(-6.74715665970798,-0.517847476925649,
137.327343608653));
#43120=CARTESIAN_POINT('Ctrl Pts',(-6.73391603079622,-0.69036274738927,
137.335508934404));
#43121=CARTESIAN_POINT('Ctrl Pts',(-6.71403830402876,-0.862582718275997,
137.343674260155));
#43122=CARTESIAN_POINT('Ctrl Pts',(-6.68754268485469,-1.03395446623465,
137.351839585906));
#43123=CARTESIAN_POINT('Ctrl Pts',(-6.66107118090542,-1.20517023866385,
137.359997479913));
#43124=CARTESIAN_POINT('Ctrl Pts',(-6.62799383308207,-1.37553896817054,
137.368155373919));
#43125=CARTESIAN_POINT('Ctrl Pts',(-6.58838177335109,-1.54451112283959,
137.376313267926));
#43126=CARTESIAN_POINT('Ctrl Pts',(-6.54879754047434,-1.71336457720498,
137.384465431139));
#43127=CARTESIAN_POINT('Ctrl Pts',(-6.50268782024288,-1.88082305774971,
137.392617594353));
#43128=CARTESIAN_POINT('Ctrl Pts',(-6.45017512153973,-2.04634549904702,
137.400769757566));
#43129=CARTESIAN_POINT('Ctrl Pts',(-6.39768840969953,-2.21178602855718,
137.408917886533));
#43130=CARTESIAN_POINT('Ctrl Pts',(-6.33880514060618,-2.37529208122676,
137.4170660155));
#43131=CARTESIAN_POINT('Ctrl Pts',(-6.27369814580787,-2.53633605330344,
137.425214144468));
#43132=CARTESIAN_POINT('Ctrl Pts',(-6.20860080580003,-2.69735614398595,
137.43336106514));
#43133=CARTESIAN_POINT('Ctrl Pts',(-6.13728170805753,-2.85591454168801,
137.441507985812));
#43134=CARTESIAN_POINT('Ctrl Pts',(-6.05996255435189,-3.01150175823508,
137.449654906484));
#43135=CARTESIAN_POINT('Ctrl Pts',(-5.98264609294616,-3.16708355714072,
137.457801543475));
#43136=CARTESIAN_POINT('Ctrl Pts',(-5.89933015289816,-3.31969405475827,
137.465948180466));
#43137=CARTESIAN_POINT('Ctrl Pts',(-5.81028324683367,-3.4688467235616,137.474094817457));
#43138=CARTESIAN_POINT('Ctrl Pts',(-5.72122269490448,-3.61802224905055,
137.482242702868));
#43139=CARTESIAN_POINT('Ctrl Pts',(-5.62642961453309,-3.76373857806599,
137.490390588279));
#43140=CARTESIAN_POINT('Ctrl Pts',(-5.52621683817355,-3.90553664142166,
137.49853847369));
#43141=CARTESIAN_POINT('Ctrl Pts',(-5.42596985777076,-4.0473831024694,137.50668914009));
#43142=CARTESIAN_POINT('Ctrl Pts',(-5.32029970766465,-4.18530833783343,
137.514839806489));
#43143=CARTESIAN_POINT('Ctrl Pts',(-5.20956060664076,-4.31888495861337,
137.522990472889));
#43144=CARTESIAN_POINT('Ctrl Pts',(-5.09870503425828,-4.45260207042451,
137.531149711864));
#43145=CARTESIAN_POINT('Ctrl Pts',(-4.98277009609973,-4.58196115331192,
137.539308950838));
#43146=CARTESIAN_POINT('Ctrl Pts',(-4.86214867596418,-4.70656979687115,
137.547468189812));
#43147=CARTESIAN_POINT('Ctrl Pts',(-4.74145571725088,-4.83125234376469,
137.555632267897));
#43148=CARTESIAN_POINT('Ctrl Pts',(-4.61607100008085,-4.95117858619476,
137.563796345981));
#43149=CARTESIAN_POINT('Ctrl Pts',(-4.48642163544698,-5.06599545094479,
137.571960424066));
#43150=CARTESIAN_POINT('Ctrl Pts',(-4.35659652926539,-5.18096795157912,
137.580135568674));
#43151=CARTESIAN_POINT('Ctrl Pts',(-4.22249551110337,-5.29081701279263,
137.588310713281));
#43152=CARTESIAN_POINT('Ctrl Pts',(-4.08457661889368,-5.39523149126959,
137.596485857889));
#43153=CARTESIAN_POINT('Ctrl Pts',(-4.01555650236539,-5.44748466236354,
137.600577026434));
#43154=CARTESIAN_POINT('Ctrl Pts',(-3.94558066492359,-5.49837749322565,
137.604668194978));
#43155=CARTESIAN_POINT('Ctrl Pts',(-3.87470887583674,-5.54787528045756,
137.608759363522));
#43156=CARTESIAN_POINT('Ctrl Pts',(-3.73220543769111,-5.64740155109401,
137.616985564541));
#43157=CARTESIAN_POINT('Ctrl Pts',(-3.58566569063898,-5.74157286039979,
137.62521176556));
#43158=CARTESIAN_POINT('Ctrl Pts',(-3.43552915256106,-5.83004532074178,
137.633437966579));
#43159=CARTESIAN_POINT('Ctrl Pts',(-3.28556126124083,-5.91841840092106,
137.641654927195));
#43160=CARTESIAN_POINT('Ctrl Pts',(-3.13200493027858,-6.0011051987528,137.64987188781));
#43161=CARTESIAN_POINT('Ctrl Pts',(-2.97533060905648,-6.07780361370879,
137.658088848426));
#43162=CARTESIAN_POINT('Ctrl Pts',(-2.81880083263286,-6.15443126814163,
137.666298228228));
#43163=CARTESIAN_POINT('Ctrl Pts',(-2.6591591148915,-6.22508138578937,137.674507608029));
#43164=CARTESIAN_POINT('Ctrl Pts',(-2.49690267299663,-6.289496485537,137.682716987831));
#43165=CARTESIAN_POINT('Ctrl Pts',(-2.33476337015323,-6.3538650815921,137.690920440971));
#43166=CARTESIAN_POINT('Ctrl Pts',(-2.17001343504685,-6.41200749375973,
137.699123894112));
#43167=CARTESIAN_POINT('Ctrl Pts',(-2.00317242939371,-6.46371326855678,
137.707327347252));
#43168=CARTESIAN_POINT('Ctrl Pts',(-1.83641840466981,-6.51539208705299,
137.715526523602));
#43169=CARTESIAN_POINT('Ctrl Pts',(-1.66757582293883,-6.56064084737598,
137.723725699952));
#43170=CARTESIAN_POINT('Ctrl Pts',(-1.49718195114939,-6.59929808427779,
137.731924876302));
#43171=CARTESIAN_POINT('Ctrl Pts',(-1.32682014153861,-6.63794804723704,
137.740122509854));
#43172=CARTESIAN_POINT('Ctrl Pts',(-1.15490797131203,-6.67000887197743,
137.748320143405));
#43173=CARTESIAN_POINT('Ctrl Pts',(-0.981995822377504,-6.69536953459875,
137.756517776957));
#43174=CARTESIAN_POINT('Ctrl Pts',(-0.809096127361443,-6.72072837062995,
137.764714820077));
#43175=CARTESIAN_POINT('Ctrl Pts',(-0.635196951828904,-6.73938795269441,
137.772911863198));
#43176=CARTESIAN_POINT('Ctrl Pts',(-0.460856723997039,-6.75128877177882,
137.781108906318));
#43177=CARTESIAN_POINT('Ctrl Pts',(-0.286497366894744,-6.76319089666618,
137.789306848849));
#43178=CARTESIAN_POINT('Ctrl Pts',(-0.111697219000216,-6.76833275666487,
137.797504791381));
#43179=CARTESIAN_POINT('Ctrl Pts',(0.0629822882574094,-6.76670689710777,
137.805702733912));
#43180=CARTESIAN_POINT('Ctrl Pts',(0.237712709839843,-6.76508056365683,
137.81390306592));
#43181=CARTESIAN_POINT('Ctrl Pts',(0.412322062169648,-6.75668258479427,
137.822103397929));
#43182=CARTESIAN_POINT('Ctrl Pts',(0.586250982279984,-6.74155759344795,
137.830303729937));
#43183=CARTESIAN_POINT('Ctrl Pts',(0.760361183333839,-6.72641683777274,
137.838512608908));
#43184=CARTESIAN_POINT('Ctrl Pts',(0.933789177502336,-6.70453509308144,
137.846721487879));
#43185=CARTESIAN_POINT('Ctrl Pts',(1.10598177941889,-6.67600878546407,137.85493036685));
#43186=CARTESIAN_POINT('Ctrl Pts',(1.27826681831792,-6.64746716426314,137.863143652537));
#43187=CARTESIAN_POINT('Ctrl Pts',(1.44931479189869,-6.61227394150192,137.871356938224));
#43188=CARTESIAN_POINT('Ctrl Pts',(1.61858482864857,-6.57057624204062,137.879570223912));
#43189=CARTESIAN_POINT('Ctrl Pts',(1.78810248660039,-6.52881754398408,137.887795524624));
#43190=CARTESIAN_POINT('Ctrl Pts',(1.95583666532564,-6.48053545283601,137.896020825336));
#43191=CARTESIAN_POINT('Ctrl Pts',(2.12126249475715,-6.42592673692571,137.904246126048));
#43192=CARTESIAN_POINT('Ctrl Pts',(2.27087020251983,-6.37653974071551,137.911684918342));
#43193=CARTESIAN_POINT('Ctrl Pts',(2.41858997147528,-6.32197888860733,137.919123710636));
#43194=CARTESIAN_POINT('Ctrl Pts',(2.56404983685379,-6.26242264895384,137.92656250293));
#43195=CARTESIAN_POINT('Ctrl Pts',(2.72346680703007,-6.19715189364311,137.934715059143));
#43196=CARTESIAN_POINT('Ctrl Pts',(2.88063918846917,-6.12568786670864,137.942867615356));
#43197=CARTESIAN_POINT('Ctrl Pts',(3.03504581874679,-6.04820517824153,137.95102017157));
#43198=CARTESIAN_POINT('Ctrl Pts',(3.18927356522068,-5.97081225533702,137.95916328285));
#43199=CARTESIAN_POINT('Ctrl Pts',(3.34074161538607,-5.88741471313523,137.96730639413));
#43200=CARTESIAN_POINT('Ctrl Pts',(3.48894655912745,-5.79823601688934,137.975449505411));
#43201=CARTESIAN_POINT('Ctrl Pts',(3.63701096211187,-5.70914188760294,137.983584894688));
#43202=CARTESIAN_POINT('Ctrl Pts',(3.78181810807352,-5.614277705794,137.991720283965));
#43203=CARTESIAN_POINT('Ctrl Pts',(3.92288708508951,-5.5139138474987,137.999855673243));
#43204=CARTESIAN_POINT('Ctrl Pts',(4.06385193028665,-5.41362407403292,138.007985057281));
#43205=CARTESIAN_POINT('Ctrl Pts',(4.20108380432733,-5.30784291859152,138.01611444132));
#43206=CARTESIAN_POINT('Ctrl Pts',(4.33412882111483,-5.19688525580292,138.024243825359));
#43207=CARTESIAN_POINT('Ctrl Pts',(4.46710357488483,-5.08598619137742,138.032368916151));
#43208=CARTESIAN_POINT('Ctrl Pts',(4.59589559486509,-4.96991629767309,138.040494006943));
#43209=CARTESIAN_POINT('Ctrl Pts',(4.72008228381978,-4.84903209248718,138.048619097735));
#43210=CARTESIAN_POINT('Ctrl Pts',(4.8447430202892,-4.72768644608306,138.05677520376));
#43211=CARTESIAN_POINT('Ctrl Pts',(4.96476289850688,-4.6014898832583,138.064931309785));
#43212=CARTESIAN_POINT('Ctrl Pts',(5.07974981604692,-4.47084229271972,138.07308741581));
#43213=CARTESIAN_POINT('Ctrl Pts',(5.19427393203929,-4.34072053510538,138.081210694984));
#43214=CARTESIAN_POINT('Ctrl Pts',(5.30380529847201,-4.20618380314721,138.089333974157));
#43215=CARTESIAN_POINT('Ctrl Pts',(5.40799537127942,-4.06766211283832,138.09745725333));
#43216=CARTESIAN_POINT('Ctrl Pts',(5.51219931787526,-3.92912197719611,138.105581614187));
#43217=CARTESIAN_POINT('Ctrl Pts',(5.61106033427002,-3.78659611867205,138.113705975044));
#43218=CARTESIAN_POINT('Ctrl Pts',(5.70427196775197,-3.64054533249059,138.1218303359));
#43219=CARTESIAN_POINT('Ctrl Pts',(5.79751374714345,-3.49444731149926,138.129957324286));
#43220=CARTESIAN_POINT('Ctrl Pts',(5.88510230860671,-3.34482240094478,138.138084312671));
#43221=CARTESIAN_POINT('Ctrl Pts',(5.96677611970491,-3.19215784968713,138.146211301057));
#43222=CARTESIAN_POINT('Ctrl Pts',(6.04897794269357,-3.03850633948597,138.154390829497));
#43223=CARTESIAN_POINT('Ctrl Pts',(6.12518809651608,-2.88177608184259,138.162570357937));
#43224=CARTESIAN_POINT('Ctrl Pts',(6.19518864453863,-2.72248538262001,138.170749886377));
#43225=CARTESIAN_POINT('Ctrl Pts',(6.26485953741319,-2.56394483465351,138.178890894781));
#43226=CARTESIAN_POINT('Ctrl Pts',(6.32837911048866,-2.40286827257537,138.187031903184));
#43227=CARTESIAN_POINT('Ctrl Pts',(6.38558237281462,-2.23978274839307,138.195172911588));
#43228=CARTESIAN_POINT('Ctrl Pts',(6.4431916300072,-2.07553973977815,138.203371700046));
#43229=CARTESIAN_POINT('Ctrl Pts',(6.49439447691907,-1.90925950819574,138.211570488505));
#43230=CARTESIAN_POINT('Ctrl Pts',(6.5390746352727,-1.74149129034089,138.219769276963));
#43231=CARTESIAN_POINT('Ctrl Pts',(6.58375479362637,-1.57372307248591,138.227968065421));
#43232=CARTESIAN_POINT('Ctrl Pts',(6.621912244947,-1.40446724488043,138.23616685388));
#43233=CARTESIAN_POINT('Ctrl Pts',(6.65348374684837,-1.23427834398266,138.244365642338));
#43234=CARTESIAN_POINT('Ctrl Pts',(6.68518718196193,-1.06337824573845,138.25259869247));
#43235=CARTESIAN_POINT('Ctrl Pts',(6.71034817818033,-0.891006032119165,
138.260831742602));
#43236=CARTESIAN_POINT('Ctrl Pts',(6.72883277965433,-0.717703576310849,
138.269064792734));
#43237=CARTESIAN_POINT('Ctrl Pts',(6.74729536880935,-0.544607497088091,
138.277288038569));
#43238=CARTESIAN_POINT('Ctrl Pts',(6.7590973571348,-0.370583734199326,138.285511284404));
#43239=CARTESIAN_POINT('Ctrl Pts',(6.76415555074572,-0.196185334100025,
138.293734530239));
#43240=CARTESIAN_POINT('Ctrl Pts',(6.76920873323391,-0.021959709471846,
138.301949629352));
#43241=CARTESIAN_POINT('Ctrl Pts',(6.76753141606382,0.152639457644934,138.310164728466));
#43242=CARTESIAN_POINT('Ctrl Pts',(6.75909205449102,0.327052899263056,138.318379827579));
#43243=CARTESIAN_POINT('Ctrl Pts',(6.75065936519795,0.501328447124589,138.326588431718));
#43244=CARTESIAN_POINT('Ctrl Pts',(6.73547529723366,0.675418205804321,138.334797035857));
#43245=CARTESIAN_POINT('Ctrl Pts',(6.7135603500842,0.848761701408204,138.343005639996));
#43246=CARTESIAN_POINT('Ctrl Pts',(6.69165834560424,1.02200282270295,138.351209396245));
#43247=CARTESIAN_POINT('Ctrl Pts',(6.66303342581454,1.1944982045209,138.359413152494));
#43248=CARTESIAN_POINT('Ctrl Pts',(6.62775803369018,1.36569119747302,138.367616908743));
#43249=CARTESIAN_POINT('Ctrl Pts',(6.59249307866533,1.53683353873298,138.375818237707));
#43250=CARTESIAN_POINT('Ctrl Pts',(6.55058163932144,1.70667390757311,138.384019566671));
#43251=CARTESIAN_POINT('Ctrl Pts',(6.50214754427987,1.8746643199291,138.392220895635));
#43252=CARTESIAN_POINT('Ctrl Pts',(6.45372012876234,2.04263156480367,138.400421093558));
#43253=CARTESIAN_POINT('Ctrl Pts',(6.39877194756112,2.2087490169544,138.408621291481));
#43254=CARTESIAN_POINT('Ctrl Pts',(6.33747714091964,2.37248234731494,138.416821489404));
#43255=CARTESIAN_POINT('Ctrl Pts',(6.27617967955108,2.53622276909692,138.425022042484));
#43256=CARTESIAN_POINT('Ctrl Pts',(6.2085351706833,2.69757852779026,138.433222595563));
#43257=CARTESIAN_POINT('Ctrl Pts',(6.13476650800192,2.85603376946035,138.441423148643));
#43258=CARTESIAN_POINT('Ctrl Pts',(6.06098128201432,3.01452458914686,138.449625542996));
#43259=CARTESIAN_POINT('Ctrl Pts',(5.98106931466843,3.17011326995205,138.45782793735));
#43260=CARTESIAN_POINT('Ctrl Pts',(5.89530022198093,3.32230707381356,138.466030331703));
#43261=CARTESIAN_POINT('Ctrl Pts',(5.80945092011412,3.47464320563636,138.474240396737));
#43262=CARTESIAN_POINT('Ctrl Pts',(5.7177337255637,3.62357780498087,138.48245046177));
#43263=CARTESIAN_POINT('Ctrl Pts',(5.62046300289667,3.76864493327107,138.490660526804));
#43264=CARTESIAN_POINT('Ctrl Pts',(5.5231457281873,3.91378148811548,138.49887452103));
#43265=CARTESIAN_POINT('Ctrl Pts',(5.42026983690323,4.05504659204454,138.507088515255));
#43266=CARTESIAN_POINT('Ctrl Pts',(5.3121909895703,4.19200618920441,138.51530250948));
#43267=CARTESIAN_POINT('Ctrl Pts',(5.20396479477191,4.32915250791073,138.523527702115));
#43268=CARTESIAN_POINT('Ctrl Pts',(5.09052170049427,4.46198131637448,138.531752894751));
#43269=CARTESIAN_POINT('Ctrl Pts',(4.9722561607381,4.59009342737182,138.539978087386));
#43270=CARTESIAN_POINT('Ctrl Pts',(4.86590021414053,4.70530437439686,138.547374985506));
#43271=CARTESIAN_POINT('Ctrl Pts',(4.75564480751625,4.81670112120452,138.554771883625));
#43272=CARTESIAN_POINT('Ctrl Pts',(4.64179987782883,4.92402100870704,138.562168781745));
#43273=CARTESIAN_POINT('Ctrl Pts',(4.50874499689211,5.04944982572152,138.570813816718));
#43274=CARTESIAN_POINT('Ctrl Pts',(4.37048472851995,5.16959417462541,138.579458851691));
#43275=CARTESIAN_POINT('Ctrl Pts',(4.22745515641186,5.28402421460451,138.588103886664));
#43276=CARTESIAN_POINT('Ctrl Pts',(4.0845883862147,5.39832400579028,138.596739081516));
#43277=CARTESIAN_POINT('Ctrl Pts',(3.93696337097964,5.50692226462593,138.605374276369));
#43278=CARTESIAN_POINT('Ctrl Pts',(3.78505167362472,5.60942713902148,138.614009471221));
#43279=CARTESIAN_POINT('Ctrl Pts',(3.63336168653824,5.71178241082807,138.622632063283));
#43280=CARTESIAN_POINT('Ctrl Pts',(3.47739774985327,5.80806186913041,138.631254655344));
#43281=CARTESIAN_POINT('Ctrl Pts',(3.31766296943204,5.89791500627632,138.639877247406));
#43282=CARTESIAN_POINT('Ctrl Pts',(3.24558516275021,5.93845982082378,138.643768056421));
#43283=CARTESIAN_POINT('Ctrl Pts',(3.1727399991916,5.97769671143552,138.647658865436));
#43284=CARTESIAN_POINT('Ctrl Pts',(3.09917575053274,6.01559628526631,138.651549674452));
#43285=CARTESIAN_POINT('Origin',(0.,0.,-3.69717978381041));
#43286=CARTESIAN_POINT('',(3.09917575053271,6.01559628526633,141.045900408649));
#43287=CARTESIAN_POINT('',(3.09917575053259,6.01559628526639,140.651392015123));
#43288=CARTESIAN_POINT('',(3.09917575053259,6.01559628526639,-3.69717978381041));
#43289=CARTESIAN_POINT('',(-6.76699963384649,0.00222610005286933,139.69717978384));
#43290=CARTESIAN_POINT('Ctrl Pts',(-6.76699963384649,0.00222610005305866,
139.69717978384));
#43291=CARTESIAN_POINT('Ctrl Pts',(-6.76705636330936,-0.170222687206146,
139.705337466641));
#43292=CARTESIAN_POINT('Ctrl Pts',(-6.76051690289134,-0.34292831167991,
139.713495149441));
#43293=CARTESIAN_POINT('Ctrl Pts',(-6.74734854687333,-0.515341233559222,
139.721652832242));
#43294=CARTESIAN_POINT('Ctrl Pts',(-6.73419462435496,-0.687565178026157,
139.729801573614));
#43295=CARTESIAN_POINT('Ctrl Pts',(-6.71442629813685,-0.859496697719035,
139.737950314987));
#43296=CARTESIAN_POINT('Ctrl Pts',(-6.68806283453828,-1.03058455318709,
139.746099056359));
#43297=CARTESIAN_POINT('Ctrl Pts',(-6.66172273840259,-1.20152076359161,
139.75424057503));
#43298=CARTESIAN_POINT('Ctrl Pts',(-6.62879919912588,-1.37161443985086,
139.762382093702));
#43299=CARTESIAN_POINT('Ctrl Pts',(-6.58936341206318,-1.5403177671387,139.770523612373));
#43300=CARTESIAN_POINT('Ctrl Pts',(-6.54995431271802,-1.70890692638066,
139.778659621365));
#43301=CARTESIAN_POINT('Ctrl Pts',(-6.50404182458938,-1.87610725598205,
139.786795630357));
#43302=CARTESIAN_POINT('Ctrl Pts',(-6.45174851469608,-2.04137946083451,
139.794931639349));
#43303=CARTESIAN_POINT('Ctrl Pts',(-6.39741451302602,-2.21310124078667,
139.80338514759));
#43304=CARTESIAN_POINT('Ctrl Pts',(-6.33619169653277,-2.38274097428837,
139.811838655831));
#43305=CARTESIAN_POINT('Ctrl Pts',(-6.26827534944102,-2.54970844285972,
139.820292164073));
#43306=CARTESIAN_POINT('Ctrl Pts',(-6.20294787868022,-2.71031134463774,
139.828423436382));
#43307=CARTESIAN_POINT('Ctrl Pts',(-6.13142790803199,-2.8684415826166,139.836554708691));
#43308=CARTESIAN_POINT('Ctrl Pts',(-6.05393904204425,-3.02359241221636,
139.844685981001));
#43309=CARTESIAN_POINT('Ctrl Pts',(-5.97645006524831,-3.17874346368005,
139.852817264938));
#43310=CARTESIAN_POINT('Ctrl Pts',(-5.89299233890733,-3.33091477113788,
139.860948548875));
#43311=CARTESIAN_POINT('Ctrl Pts',(-5.80383613475882,-3.47962284175567,
139.869079832812));
#43312=CARTESIAN_POINT('Ctrl Pts',(-5.71466288010896,-3.62835935175335,
139.8772126718));
#43313=CARTESIAN_POINT('Ctrl Pts',(-5.61978916554424,-3.77363099275641,
139.885345510788));
#43314=CARTESIAN_POINT('Ctrl Pts',(-5.51952939717935,-3.91498202213918,
139.893478349776));
#43315=CARTESIAN_POINT('Ctrl Pts',(-5.41923142313166,-4.0563869157257,139.901614287921));
#43316=CARTESIAN_POINT('Ctrl Pts',(-5.31354351973422,-4.19386792515054,
139.909750226065));
#43317=CARTESIAN_POINT('Ctrl Pts',(-5.20282125064118,-4.32700127500288,
139.917886164209));
#43318=CARTESIAN_POINT('Ctrl Pts',(-5.09198084434003,-4.46027667398758,
139.926030783146));
#43319=CARTESIAN_POINT('Ctrl Pts',(-4.97609558074881,-4.58919487029723,
139.934175402082));
#43320=CARTESIAN_POINT('Ctrl Pts',(-4.85555938568095,-4.71336737928688,
139.942320021019));
#43321=CARTESIAN_POINT('Ctrl Pts',(-4.73494703799582,-4.83761833825205,
139.95046978558));
#43322=CARTESIAN_POINT('Ctrl Pts',(-4.6096781678019,-4.95711738489197,139.958619550142));
#43323=CARTESIAN_POINT('Ctrl Pts',(-4.48018060082227,-5.07151562987001,
139.966769314703));
#43324=CARTESIAN_POINT('Ctrl Pts',(-4.3505146868854,-5.18606259267268,139.974929673966));
#43325=CARTESIAN_POINT('Ctrl Pts',(-4.21660938297347,-5.29549528569637,
139.983090033229));
#43326=CARTESIAN_POINT('Ctrl Pts',(-4.07892293864588,-5.39950707570501,
139.991250392492));
#43327=CARTESIAN_POINT('Ctrl Pts',(-4.04199757380827,-5.42740142152997,
139.993438874041));
#43328=CARTESIAN_POINT('Ctrl Pts',(-4.0048004035001,-5.45490613153912,139.995627355591));
#43329=CARTESIAN_POINT('Ctrl Pts',(-3.96734057255745,-5.48201585015399,
139.99781583714));
#43330=CARTESIAN_POINT('Ctrl Pts',(-3.82782172928879,-5.58298578213995,
140.005966819314));
#43331=CARTESIAN_POINT('Ctrl Pts',(-3.68422662962426,-5.67878465813751,
140.014117801488));
#43332=CARTESIAN_POINT('Ctrl Pts',(-3.53697823196215,-5.76906179431508,
140.022268783663));
#43333=CARTESIAN_POINT('Ctrl Pts',(-3.38990087696121,-5.8592340652319,140.030410297716));
#43334=CARTESIAN_POINT('Ctrl Pts',(-3.23917897983449,-5.94389717472451,
140.038551811769));
#43335=CARTESIAN_POINT('Ctrl Pts',(-3.08526765853149,-6.02274127579955,
140.046693325822));
#43336=CARTESIAN_POINT('Ctrl Pts',(-2.93150273090615,-6.10151038383432,
140.054827096025));
#43337=CARTESIAN_POINT('Ctrl Pts',(-2.7745547418729,-6.17447133680736,140.062960866228));
#43338=CARTESIAN_POINT('Ctrl Pts',(-2.61490681340937,-6.24135813402702,
140.071094636431));
#43339=CARTESIAN_POINT('Ctrl Pts',(-2.45537715778601,-6.30819537913816,
140.079222380849));
#43340=CARTESIAN_POINT('Ctrl Pts',(-2.29315188133859,-6.36896728787685,
140.087350125267));
#43341=CARTESIAN_POINT('Ctrl Pts',(-2.12873767178384,-6.42345428291728,
140.095477869685));
#43342=CARTESIAN_POINT('Ctrl Pts',(-1.9644106992507,-6.4779123675419,140.103601301579));
#43343=CARTESIAN_POINT('Ctrl Pts',(-1.7978974529962,-6.52609206486806,140.111724733473));
#43344=CARTESIAN_POINT('Ctrl Pts',(-1.62972351079848,-6.56782233912814,
140.119848165367));
#43345=CARTESIAN_POINT('Ctrl Pts',(-1.46048273925821,-6.60981733383464,
140.128023129118));
#43346=CARTESIAN_POINT('Ctrl Pts',(-1.28956047779386,-6.64528065816036,
140.136198092869));
#43347=CARTESIAN_POINT('Ctrl Pts',(-1.11750723084254,-6.6740891954644,140.144373056619));
#43348=CARTESIAN_POINT('Ctrl Pts',(-0.946577324580619,-6.70270964098448,
140.152494645792));
#43349=CARTESIAN_POINT('Ctrl Pts',(-0.774531526743982,-6.72476190446661,
140.160616234965));
#43350=CARTESIAN_POINT('Ctrl Pts',(-0.601918838865556,-6.7401767566896,
140.168737824139));
#43351=CARTESIAN_POINT('Ctrl Pts',(-0.42928336257217,-6.75559364398924,
140.176860485528));
#43352=CARTESIAN_POINT('Ctrl Pts',(-0.256081211738418,-6.76437134208855,
140.184983146917));
#43353=CARTESIAN_POINT('Ctrl Pts',(-0.0828653323660814,-6.76649261705737,
140.193105808307));
#43354=CARTESIAN_POINT('Ctrl Pts',(0.0904064004816274,-6.76861457603149,
140.201231088849));
#43355=CARTESIAN_POINT('Ctrl Pts',(0.263691504913624,-6.76407583332543,
140.209356369391));
#43356=CARTESIAN_POINT('Ctrl Pts',(0.436438259753492,-6.7529112718459,140.217481649933));
#43357=CARTESIAN_POINT('Ctrl Pts',(0.611067054643416,-6.74162507478562,
140.225695453721));
#43358=CARTESIAN_POINT('Ctrl Pts',(0.785145317493713,-6.72356786403866,
140.233909257509));
#43359=CARTESIAN_POINT('Ctrl Pts',(0.95811060862046,-6.69882923066777,140.242123061297));
#43360=CARTESIAN_POINT('Ctrl Pts',(1.12950786827785,-6.67431486746914,140.250262402152));
#43361=CARTESIAN_POINT('Ctrl Pts',(1.29981190532521,-6.64323985432275,140.258401743007));
#43362=CARTESIAN_POINT('Ctrl Pts',(1.46848817947352,-6.60574231004711,140.266541083862));
#43363=CARTESIAN_POINT('Ctrl Pts',(1.6394791613353,-6.56773019515146,140.274792119116));
#43364=CARTESIAN_POINT('Ctrl Pts',(1.80879700187877,-6.52311810091999,140.283043154371));
#43365=CARTESIAN_POINT('Ctrl Pts',(1.97590363668063,-6.47210119038263,140.291294189625));
#43366=CARTESIAN_POINT('Ctrl Pts',(2.14301027148261,-6.42108427984524,140.299545224879));
#43367=CARTESIAN_POINT('Ctrl Pts',(2.30790536007158,-6.36366274257922,140.307796260133));
#43368=CARTESIAN_POINT('Ctrl Pts',(2.4700750024516,-6.30008083140714,140.316047295387));
#43369=CARTESIAN_POINT('Ctrl Pts',(2.63186603658003,-6.23664736131115,140.324279067418));
#43370=CARTESIAN_POINT('Ctrl Pts',(2.79144948368518,-6.16688438648224,140.332510839449));
#43371=CARTESIAN_POINT('Ctrl Pts',(2.94829467539587,-6.09096441518356,140.340742611479));
#43372=CARTESIAN_POINT('Ctrl Pts',(3.10495257827362,-6.01513509991752,140.348964553952));
#43373=CARTESIAN_POINT('Ctrl Pts',(3.25887841724637,-5.93316358242239,140.357186496424));
#43374=CARTESIAN_POINT('Ctrl Pts',(3.40955885309962,-5.84527137327687,140.365408438897));
#43375=CARTESIAN_POINT('Ctrl Pts',(3.56008955160476,-5.75746650623547,140.373622210887));
#43376=CARTESIAN_POINT('Ctrl Pts',(3.70738096237336,-5.66375284406863,140.381835982876));
#43377=CARTESIAN_POINT('Ctrl Pts',(3.85094175012746,-5.56439903647512,140.390049754866));
#43378=CARTESIAN_POINT('Ctrl Pts',(3.99438862883727,-5.46512406167048,140.398257009597));
#43379=CARTESIAN_POINT('Ctrl Pts',(4.13411048706786,-5.36021805805965,140.406464264327));
#43380=CARTESIAN_POINT('Ctrl Pts',(4.26964246240572,-5.2499944993516,140.414671519057));
#43381=CARTESIAN_POINT('Ctrl Pts',(4.40509403728806,-5.13983632760708,140.422873905069));
#43382=CARTESIAN_POINT('Ctrl Pts',(4.5363604035007,-5.02436711034961,140.431076291081));
#43383=CARTESIAN_POINT('Ctrl Pts',(4.66300739084778,-4.90394240105846,140.439278677093));
#43384=CARTESIAN_POINT('Ctrl Pts',(4.78961657714103,-4.78355363562206,140.447478614892));
#43385=CARTESIAN_POINT('Ctrl Pts',(4.91160886901698,-4.65821256823187,140.455678552691));
#43386=CARTESIAN_POINT('Ctrl Pts',(5.02858460541446,-4.5283137994389,140.463878490489));
#43387=CARTESIAN_POINT('Ctrl Pts',(5.14554398558485,-4.39843319384647,140.472077281725));
#43388=CARTESIAN_POINT('Ctrl Pts',(5.25748796692467,-4.26399642179446,140.480276072961));
#43389=CARTESIAN_POINT('Ctrl Pts',(5.36405506699925,-4.12543358184321,140.488474864197));
#43390=CARTESIAN_POINT('Ctrl Pts',(5.470626598068,-3.98686498053469,140.496673996333));
#43391=CARTESIAN_POINT('Ctrl Pts',(5.57182058388545,-3.84417025362486,140.50487312847));
#43392=CARTESIAN_POINT('Ctrl Pts',(5.66731699076707,-3.69781112635068,140.513072260606));
#43393=CARTESIAN_POINT('Ctrl Pts',(5.76283469181036,-3.55141936334685,140.521273221017));
#43394=CARTESIAN_POINT('Ctrl Pts',(5.85265208768857,-3.40136187266688,140.529474181428));
#43395=CARTESIAN_POINT('Ctrl Pts',(5.93649346107707,-3.24812782793246,140.537675141839));
#43396=CARTESIAN_POINT('Ctrl Pts',(6.02041341401542,-3.09475016601034,140.545883788524));
#43397=CARTESIAN_POINT('Ctrl Pts',(6.0983459817951,-2.93819031663081,140.554092435209));
#43398=CARTESIAN_POINT('Ctrl Pts',(6.17006184638328,-2.77896128289066,140.562301081894));
#43399=CARTESIAN_POINT('Ctrl Pts',(6.24181195013942,-2.61965622873774,140.570513647617));
#43400=CARTESIAN_POINT('Ctrl Pts',(6.3073392986111,-2.45767978149311,140.578726213341));
#43401=CARTESIAN_POINT('Ctrl Pts',(6.36646346716161,-2.29356314962039,140.586938779064));
#43402=CARTESIAN_POINT('Ctrl Pts',(6.42566876260306,-2.12922132604648,140.595162613613));
#43403=CARTESIAN_POINT('Ctrl Pts',(6.47845321032211,-1.96273379060594,140.603386448162));
#43404=CARTESIAN_POINT('Ctrl Pts',(6.52468648835483,-1.79464626839941,140.611610282711));
#43405=CARTESIAN_POINT('Ctrl Pts',(6.56716617397803,-1.6402054542425,140.619166439685));
#43406=CARTESIAN_POINT('Ctrl Pts',(6.60411580339929,-1.4844142516776,140.626722596659));
#43407=CARTESIAN_POINT('Ctrl Pts',(6.63547272895231,-1.32770127036553,140.634278753633));
#43408=CARTESIAN_POINT('Ctrl Pts',(6.67135117063168,-1.14839103949166,140.642924471686));
#43409=CARTESIAN_POINT('Ctrl Pts',(6.69998922023828,-0.967465284381121,
140.651570189738));
#43410=CARTESIAN_POINT('Ctrl Pts',(6.72125320686374,-0.785521692395489,
140.660215907791));
#43411=CARTESIAN_POINT('Ctrl Pts',(6.74248989486381,-0.603811678903314,
140.668850526503));
#43412=CARTESIAN_POINT('Ctrl Pts',(6.75637136192696,-0.421086735623222,
140.677485145215));
#43413=CARTESIAN_POINT('Ctrl Pts',(6.76281500291947,-0.237954273521913,
140.686119763928));
#43414=CARTESIAN_POINT('Ctrl Pts',(6.76948620828031,-0.0483542842714589,
140.69505932383));
#43415=CARTESIAN_POINT('Ctrl Pts',(6.76818455781633,0.141682223962945,140.703998883732));
#43416=CARTESIAN_POINT('Ctrl Pts',(6.75887674449614,0.331472702811677,140.712938443635));
#43417=CARTESIAN_POINT('Ctrl Pts',(6.74991138668418,0.514280360598753,140.721549096905));
#43418=CARTESIAN_POINT('Ctrl Pts',(6.73351845799152,0.696859420342741,140.730159750176));
#43419=CARTESIAN_POINT('Ctrl Pts',(6.70972102713668,0.878597028221676,140.738770403447));
#43420=CARTESIAN_POINT('Ctrl Pts',(6.68594612214232,1.0601626092955,140.747372906158));
#43421=CARTESIAN_POINT('Ctrl Pts',(6.6547807282305,1.24088802507926,140.755975408869));
#43422=CARTESIAN_POINT('Ctrl Pts',(6.61629982679463,1.4201639348883,140.76457791158));
#43423=CARTESIAN_POINT('Ctrl Pts',(6.57786223483875,1.59923807326943,140.773170732347));
#43424=CARTESIAN_POINT('Ctrl Pts',(6.5321256247305,1.77686566268429,140.781763553115));
#43425=CARTESIAN_POINT('Ctrl Pts',(6.47921635425518,1.95244575718563,140.790356373882));
#43426=CARTESIAN_POINT('Ctrl Pts',(6.47298075640211,1.97313866885272,140.791369076841));
#43427=CARTESIAN_POINT('Ctrl Pts',(6.46664559110848,1.99380315177187,140.792381779799));
#43428=CARTESIAN_POINT('Ctrl Pts',(6.46021111211851,2.0144382310859,140.793394482757));
#43429=CARTESIAN_POINT('Ctrl Pts',(6.40559884401013,2.1895772727539,140.801989740517));
#43430=CARTESIAN_POINT('Ctrl Pts',(6.34389249037932,2.36239098317935,140.810584998277));
#43431=CARTESIAN_POINT('Ctrl Pts',(6.27532428130308,2.53231004509481,140.819180256037));
#43432=CARTESIAN_POINT('Ctrl Pts',(6.20669186100719,2.70238822900503,140.827783562892));
#43433=CARTESIAN_POINT('Ctrl Pts',(6.13118487331445,2.86956607055048,140.836386869746));
#43434=CARTESIAN_POINT('Ctrl Pts',(6.04908273339191,3.03329640565835,140.8449901766));
#43435=CARTESIAN_POINT('Ctrl Pts',(5.96357661027702,3.20381505723776,140.85395017954));
#43436=CARTESIAN_POINT('Ctrl Pts',(5.87091699002684,3.37059390659366,140.86291018248));
#43437=CARTESIAN_POINT('Ctrl Pts',(5.77147029246756,3.53304679606206,140.87187018542));
#43438=CARTESIAN_POINT('Ctrl Pts',(5.67572132086355,3.68945920072163,140.880497028625));
#43439=CARTESIAN_POINT('Ctrl Pts',(5.57368110157995,3.84186132870413,140.88912387183));
#43440=CARTESIAN_POINT('Ctrl Pts',(5.46571913039019,3.98976232220502,140.897750715035));
#43441=CARTESIAN_POINT('Ctrl Pts',(5.35765397484706,4.13780467166864,140.906385803321));
#43442=CARTESIAN_POINT('Ctrl Pts',(5.24365595731899,4.28133705899291,140.915020891607));
#43443=CARTESIAN_POINT('Ctrl Pts',(5.12413421366191,4.41990243788021,140.923655979893));
#43444=CARTESIAN_POINT('Ctrl Pts',(5.0044349562296,4.55867361416278,140.932303893018));
#43445=CARTESIAN_POINT('Ctrl Pts',(4.87919578376329,4.69246281460474,140.940951806143));
#43446=CARTESIAN_POINT('Ctrl Pts',(4.74886298885342,4.82084943895763,140.949599719269));
#43447=CARTESIAN_POINT('Ctrl Pts',(4.73424163334257,4.83525246375888,140.950569883473));
#43448=CARTESIAN_POINT('Ctrl Pts',(4.71955620680024,4.84958753646979,140.951540047677));
#43449=CARTESIAN_POINT('Ctrl Pts',(4.70480736498783,4.86385409509335,140.952510211881));
#43450=CARTESIAN_POINT('Ctrl Pts',(4.57978419058098,4.98478904508226,140.960734112443));
#43451=CARTESIAN_POINT('Ctrl Pts',(4.44993041114769,5.10105975968477,140.968958013006));
#43452=CARTESIAN_POINT('Ctrl Pts',(4.31562816458559,5.21225887164439,140.977181913569));
#43453=CARTESIAN_POINT('Ctrl Pts',(4.18145070678321,5.32335466143615,140.985398172783));
#43454=CARTESIAN_POINT('Ctrl Pts',(4.04283328221031,5.42938800100551,140.993614431996));
#43455=CARTESIAN_POINT('Ctrl Pts',(3.90019509022749,5.52998799801278,141.00183069121));
#43456=CARTESIAN_POINT('Ctrl Pts',(3.75769109599703,5.63049334790417,141.010039220351));
#43457=CARTESIAN_POINT('Ctrl Pts',(3.61117416244117,5.72557533448906,141.018247749493));
#43458=CARTESIAN_POINT('Ctrl Pts',(3.46109660356837,5.81490320648311,141.026456278634));
#43459=CARTESIAN_POINT('Ctrl Pts',(3.34259678803946,5.88543564605894,141.032937655306));
#43460=CARTESIAN_POINT('Ctrl Pts',(3.22187781245033,5.95238139570221,141.039419031978));
#43461=CARTESIAN_POINT('Ctrl Pts',(3.09917575053271,6.01559628526633,141.045900408649));
#43462=CARTESIAN_POINT('Ctrl Pts',(3.09917575053254,6.01559628526642,139.045839590042));
#43463=CARTESIAN_POINT('Ctrl Pts',(2.94611930473484,6.09444945339552,139.0539922918));
#43464=CARTESIAN_POINT('Ctrl Pts',(2.78980507744459,6.16758436117791,139.062144993558));
#43465=CARTESIAN_POINT('Ctrl Pts',(2.63070295282366,6.2347165913139,139.070297695316));
#43466=CARTESIAN_POINT('Ctrl Pts',(2.4717912571062,6.30176847106487,139.078440639127));
#43467=CARTESIAN_POINT('Ctrl Pts',(2.31009863951035,6.36283183385974,139.086583582939));
#43468=CARTESIAN_POINT('Ctrl Pts',(2.14612079442815,6.41766737496757,139.09472652675));
#43469=CARTESIAN_POINT('Ctrl Pts',(1.98230470270438,6.47244882442094,139.102861438083));
#43470=CARTESIAN_POINT('Ctrl Pts',(1.81620821557681,6.52101456742517,139.110996349416));
#43471=CARTESIAN_POINT('Ctrl Pts',(1.6483482856285,6.5631727791721,139.119131260749));
#43472=CARTESIAN_POINT('Ctrl Pts',(1.4806186310235,6.60529827211883,139.127259858613));
#43473=CARTESIAN_POINT('Ctrl Pts',(1.31112861174914,6.64102604678876,139.135388456478));
#43474=CARTESIAN_POINT('Ctrl Pts',(1.14041167024186,6.67021365642632,139.143517054342));
#43475=CARTESIAN_POINT('Ctrl Pts',(0.969791327360429,6.69938475052091,139.151641052714));
#43476=CARTESIAN_POINT('Ctrl Pts',(0.797945804421077,6.72202298805287,139.159765051085));
#43477=CARTESIAN_POINT('Ctrl Pts',(0.62542009786228,6.73803670969445,139.167889049456));
#43478=CARTESIAN_POINT('Ctrl Pts',(0.452933585170598,6.75404679338727,139.176011202242));
#43479=CARTESIAN_POINT('Ctrl Pts',(0.279767559797171,6.76343531791645,139.184133355029));
#43480=CARTESIAN_POINT('Ctrl Pts',(0.106473732171504,6.76616230549914,139.192255507815));
#43481=CARTESIAN_POINT('Ctrl Pts',(-0.0668039513705443,6.76888903903519,
139.20037690394));
#43482=CARTESIAN_POINT('Ctrl Pts',(-0.24020904763952,6.7649554643749,139.208498300064));
#43483=CARTESIAN_POINT('Ctrl Pts',(-0.413188376620589,6.75437372118435,
139.216619696189));
#43484=CARTESIAN_POINT('Ctrl Pts',(-0.586184528439248,6.74379094888269,
139.224741882148));
#43485=CARTESIAN_POINT('Ctrl Pts',(-0.758754465192137,6.72655874263071,
139.232864068107));
#43486=CARTESIAN_POINT('Ctrl Pts',(-0.930348706431284,6.70274125149119,
139.240986254066));
#43487=CARTESIAN_POINT('Ctrl Pts',(-1.10199231154012,6.67891690858601,139.249110776598));
#43488=CARTESIAN_POINT('Ctrl Pts',(-1.27265929991497,6.64850355893192,139.25723529913));
#43489=CARTESIAN_POINT('Ctrl Pts',(-1.44180902181761,6.61161672698935,139.265359821662));
#43490=CARTESIAN_POINT('Ctrl Pts',(-1.61113948018845,6.57469048146895,139.273493025246));
#43491=CARTESIAN_POINT('Ctrl Pts',(-1.77894907559217,6.53127701429676,139.28162622883));
#43492=CARTESIAN_POINT('Ctrl Pts',(-1.94471009998545,6.48154238025291,139.289759432414));
#43493=CARTESIAN_POINT('Ctrl Pts',(-2.1105619282766,6.43178050157393,139.297897091367));
#43494=CARTESIAN_POINT('Ctrl Pts',(-2.27436260371014,6.37569067426807,139.30603475032));
#43495=CARTESIAN_POINT('Ctrl Pts',(-2.4356034118258,6.31348754812287,139.314172409274));
#43496=CARTESIAN_POINT('Ctrl Pts',(-2.59708947912999,6.25118980642457,139.322322446208));
#43497=CARTESIAN_POINT('Ctrl Pts',(-2.75600756303741,6.18276033018469,139.330472483142));
#43498=CARTESIAN_POINT('Ctrl Pts',(-2.91187150330822,6.10846080025251,139.338622520076));
#43499=CARTESIAN_POINT('Ctrl Pts',(-3.0567726788274,6.03938716327792,139.346199320266));
#43500=CARTESIAN_POINT('Ctrl Pts',(-3.19903429087571,5.96524077185426,139.353776120456));
#43501=CARTESIAN_POINT('Ctrl Pts',(-3.33828849068273,5.88626528054719,139.361352920646));
#43502=CARTESIAN_POINT('Ctrl Pts',(-3.48945353901703,5.80053476773534,139.369577788324));
#43503=CARTESIAN_POINT('Ctrl Pts',(-3.63752622077289,5.70885705583353,139.377802656001));
#43504=CARTESIAN_POINT('Ctrl Pts',(-3.78200694796311,5.61148041478884,139.386027523679));
#43505=CARTESIAN_POINT('Ctrl Pts',(-3.92632490144238,5.51421347942969,139.394243125123));
#43506=CARTESIAN_POINT('Ctrl Pts',(-4.06705866364899,5.41126059842744,139.402458726566));
#43507=CARTESIAN_POINT('Ctrl Pts',(-4.20373301473877,5.30291596584326,139.41067432801));
#43508=CARTESIAN_POINT('Ctrl Pts',(-4.34028084749351,5.19467162700414,139.418882324338));
#43509=CARTESIAN_POINT('Ctrl Pts',(-4.47277647341769,5.08104569792874,139.427090320666));
#43510=CARTESIAN_POINT('Ctrl Pts',(-4.60077339315962,4.96237576013692,139.435298316994));
#43511=CARTESIAN_POINT('Ctrl Pts',(-4.72867753604107,4.84379183866709,139.443500363865));
#43512=CARTESIAN_POINT('Ctrl Pts',(-4.85208920566462,4.72017143363979,139.451702410737));
#43513=CARTESIAN_POINT('Ctrl Pts',(-4.97059470455424,4.59189256005162,139.459904457608));
#43514=CARTESIAN_POINT('Ctrl Pts',(-5.08903810327832,4.46368090814818,139.46810220638));
#43515=CARTESIAN_POINT('Ctrl Pts',(-5.20258021017523,4.33081591378342,139.476299955151));
#43516=CARTESIAN_POINT('Ctrl Pts',(-5.31084390006278,4.19371268319206,139.484497703923));
#43517=CARTESIAN_POINT('Ctrl Pts',(-5.41908694082581,4.05663560228841,139.492693889139));
#43518=CARTESIAN_POINT('Ctrl Pts',(-5.52205334290557,3.91532217273589,139.500890074354));
#43519=CARTESIAN_POINT('Ctrl Pts',(-5.61940584465528,3.77022107482494,139.50908625957));
#43520=CARTESIAN_POINT('Ctrl Pts',(-5.71675114448669,3.62513071116562,139.51728183845));
#43521=CARTESIAN_POINT('Ctrl Pts',(-5.80848317041546,3.47625353465381,139.525477417331));
#43522=CARTESIAN_POINT('Ctrl Pts',(-5.89430767840892,3.32406768767569,139.533672996211));
#43523=CARTESIAN_POINT('Ctrl Pts',(-5.98014145205202,3.17186541065013,139.541869459889));
#43524=CARTESIAN_POINT('Ctrl Pts',(-6.06006626081168,3.01635406411403,139.550065923568));
#43525=CARTESIAN_POINT('Ctrl Pts',(-6.13383353959432,2.85803693267737,139.558262387246));
#43526=CARTESIAN_POINT('Ctrl Pts',(-6.20762220346182,2.69967390521001,139.566461227074));
#43527=CARTESIAN_POINT('Ctrl Pts',(-6.27524963022061,2.53850379783761,139.574660066902));
#43528=CARTESIAN_POINT('Ctrl Pts',(-6.33651515021793,2.37505047337076,139.58285890673));
#43529=CARTESIAN_POINT('Ctrl Pts',(-6.39784466379375,2.21142641725664,139.591066310479));
#43530=CARTESIAN_POINT('Ctrl Pts',(-6.45279886827092,2.04551471581172,139.599273714228));
#43531=CARTESIAN_POINT('Ctrl Pts',(-6.50122649370331,1.87785597892124,139.607481117978));
#43532=CARTESIAN_POINT('Ctrl Pts',(-6.54968005953462,1.71010743513894,139.615692918047));
#43533=CARTESIAN_POINT('Ctrl Pts',(-6.59159999092413,1.54061033836585,139.623904718116));
#43534=CARTESIAN_POINT('Ctrl Pts',(-6.62688607665502,1.36991602919153,139.632116518185));
#43535=CARTESIAN_POINT('Ctrl Pts',(-6.66222410843459,1.19897043414319,139.640340407171));
#43536=CARTESIAN_POINT('Ctrl Pts',(-6.69090871860183,1.0268244584136,139.648564296157));
#43537=CARTESIAN_POINT('Ctrl Pts',(-6.71289139029902,0.854036405576067,
139.656788185144));
#43538=CARTESIAN_POINT('Ctrl Pts',(-6.73320299891431,0.694383231886422,
139.664386916394));
#43539=CARTESIAN_POINT('Ctrl Pts',(-6.74779342697931,0.534182153838582,
139.671985647644));
#43540=CARTESIAN_POINT('Ctrl Pts',(-6.756663967453,0.373873014434406,139.679584378894));
#43541=CARTESIAN_POINT('Ctrl Pts',(-6.76351075745563,0.250137260535642,
139.685449513866));
#43542=CARTESIAN_POINT('Ctrl Pts',(-6.76695884701256,0.126211727219041,
139.691314648838));
#43543=CARTESIAN_POINT('Ctrl Pts',(-6.76699963384628,0.00222610069067668,
139.69717978381));
#43544=CARTESIAN_POINT('',(-6.76699900574552,0.00191530820773601,139.30282021619));
#43545=CARTESIAN_POINT('Ctrl Pts',(3.09917575053274,6.01559628526631,138.651549674452));
#43546=CARTESIAN_POINT('Ctrl Pts',(2.93643032011442,6.0994411225101,138.660157271204));
#43547=CARTESIAN_POINT('Ctrl Pts',(2.77016378607077,6.17673784217197,138.668764867957));
#43548=CARTESIAN_POINT('Ctrl Pts',(2.60091889377964,6.24720016551256,138.677372464709));
#43549=CARTESIAN_POINT('Ctrl Pts',(2.43188856515335,6.31757315880528,138.685969149005));
#43550=CARTESIAN_POINT('Ctrl Pts',(2.25988769262987,6.38112892639731,138.694565833301));
#43551=CARTESIAN_POINT('Ctrl Pts',(2.08548129553116,6.43762819414027,138.703162517597));
#43552=CARTESIAN_POINT('Ctrl Pts',(1.96437876055543,6.47685957935186,138.709131795548));
#43553=CARTESIAN_POINT('Ctrl Pts',(1.84211691387169,6.51268963392374,138.715101073499));
#43554=CARTESIAN_POINT('Ctrl Pts',(1.71889077907999,6.54505183246044,138.721070351449));
#43555=CARTESIAN_POINT('Ctrl Pts',(1.54144520074409,6.59165338370827,138.729666108997));
#43556=CARTESIAN_POINT('Ctrl Pts',(1.36220751444305,6.63100720467594,138.738261866544));
#43557=CARTESIAN_POINT('Ctrl Pts',(1.18178355520717,6.66300807658537,138.746857624092));
#43558=CARTESIAN_POINT('Ctrl Pts',(1.00119125428201,6.69503880639649,138.755461401773));
#43559=CARTESIAN_POINT('Ctrl Pts',(0.819410771755674,6.71970283992063,138.764065179455));
#43560=CARTESIAN_POINT('Ctrl Pts',(0.637054201472317,6.73694670784818,138.772668957137));
#43561=CARTESIAN_POINT('Ctrl Pts',(0.447530858517566,6.75486827486396,138.781610870805));
#43562=CARTESIAN_POINT('Ctrl Pts',(0.257385606767702,6.76477462134419,138.790552784473));
#43563=CARTESIAN_POINT('Ctrl Pts',(0.0673054826767739,6.76666527707716,
138.799494698141));
#43564=CARTESIAN_POINT('Ctrl Pts',(-0.116084756870127,6.76848939103662,
138.808121900471));
#43565=CARTESIAN_POINT('Ctrl Pts',(-0.299414079998668,6.76285248166214,
138.816749102802));
#43566=CARTESIAN_POINT('Ctrl Pts',(-0.482070316135283,6.74980719800953,
138.825376305133));
#43567=CARTESIAN_POINT('Ctrl Pts',(-0.664900504379287,6.73674949072096,
138.834011723553));
#43568=CARTESIAN_POINT('Ctrl Pts',(-0.847056022907174,6.71626935705887,
138.842647141974));
#43569=CARTESIAN_POINT('Ctrl Pts',(-1.02793231538164,6.6884709878263,138.851282560394));
#43570=CARTESIAN_POINT('Ctrl Pts',(-1.20907582681324,6.66063155046294,138.859930736415));
#43571=CARTESIAN_POINT('Ctrl Pts',(-1.38893603553696,6.62545232648749,138.868578912437));
#43572=CARTESIAN_POINT('Ctrl Pts',(-1.56691955745236,6.58308834062504,138.877227088458));
#43573=CARTESIAN_POINT('Ctrl Pts',(-1.58574953921025,6.57860639155247,138.878142032689));
#43574=CARTESIAN_POINT('Ctrl Pts',(-1.60455853068165,6.57404407022203,138.879056976921));
#43575=CARTESIAN_POINT('Ctrl Pts',(-1.62334584034992,6.56940159242976,138.879971921153));
#43576=CARTESIAN_POINT('Ctrl Pts',(-1.79225697596518,6.5276624499018,138.888197913694));
#43577=CARTESIAN_POINT('Ctrl Pts',(-1.95977899018776,6.47934982852275,138.896423906235));
#43578=CARTESIAN_POINT('Ctrl Pts',(-2.12536348880185,6.42457150637053,138.904649898777));
#43579=CARTESIAN_POINT('Ctrl Pts',(-2.29077439347098,6.36985061220897,138.912867267428));
#43580=CARTESIAN_POINT('Ctrl Pts',(-2.4542514901066,6.30867762728692,138.92108463608));
#43581=CARTESIAN_POINT('Ctrl Pts',(-2.61525783632606,6.24121105632033,138.929302004731));
#43582=CARTESIAN_POINT('Ctrl Pts',(-2.7761276048758,6.173801715564,138.937512402793));
#43583=CARTESIAN_POINT('Ctrl Pts',(-2.93453046863394,6.10010955917699,138.945722800856));
#43584=CARTESIAN_POINT('Ctrl Pts',(-3.0899457952861,6.0203425136942,138.953933198918));
#43585=CARTESIAN_POINT('Ctrl Pts',(-3.24526037616607,5.94062717606265,138.962138274707));
#43586=CARTESIAN_POINT('Ctrl Pts',(-3.39759095994833,5.85484495648378,138.970343350496));
#43587=CARTESIAN_POINT('Ctrl Pts',(-3.54643793101119,5.76325142619035,138.978548426285));
#43588=CARTESIAN_POINT('Ctrl Pts',(-3.69521818334,5.67169895151494,138.986749824254));
#43589=CARTESIAN_POINT('Ctrl Pts',(-3.84051762937841,5.57434054311842,138.994951222223));
#43590=CARTESIAN_POINT('Ctrl Pts',(-3.98186217922372,5.47147718497187,139.003152620193));
#43591=CARTESIAN_POINT('Ctrl Pts',(-4.12319565778759,5.36862188393958,139.011353375761));
#43592=CARTESIAN_POINT('Ctrl Pts',(-4.26057456260895,5.2602626956497,139.019554131328));
#43593=CARTESIAN_POINT('Ctrl Pts',(-4.39355437305861,5.14674353071703,139.027754886896));
#43594=CARTESIAN_POINT('Ctrl Pts',(-4.52653350803412,5.03322494240769,139.035955600808));
#43595=CARTESIAN_POINT('Ctrl Pts',(-4.65511331988828,4.91454666153035,139.044156314719));
#43596=CARTESIAN_POINT('Ctrl Pts',(-4.77888303653782,4.79109235175978,139.052357028631));
#43597=CARTESIAN_POINT('Ctrl Pts',(-4.9026745546507,4.66761629608333,139.060559187061));
#43598=CARTESIAN_POINT('Ctrl Pts',(-5.02165403577198,4.53936278850447,139.068761345491));
#43599=CARTESIAN_POINT('Ctrl Pts',(-5.13544815388113,4.40675178093785,139.07696350392));
#43600=CARTESIAN_POINT('Ctrl Pts',(-5.24928293884472,4.27409338188359,139.085168593573));
#43601=CARTESIAN_POINT('Ctrl Pts',(-5.35792843607556,4.13707465250544,139.093373683226));
#43602=CARTESIAN_POINT('Ctrl Pts',(-5.46105209899662,3.99614801678374,139.101578772879));
#43603=CARTESIAN_POINT('Ctrl Pts',(-5.56429356850904,3.85506038904415,139.109793235877));
#43604=CARTESIAN_POINT('Ctrl Pts',(-5.66200038950564,3.71005622553704,139.118007698875));
#43605=CARTESIAN_POINT('Ctrl Pts',(-5.75388322105544,3.56161717179945,139.126222161872));
#43606=CARTESIAN_POINT('Ctrl Pts',(-5.8458204902793,3.41309017261341,139.13444149168));
#43607=CARTESIAN_POINT('Ctrl Pts',(-5.93192671545112,3.26112453780743,139.142660821487));
#43608=CARTESIAN_POINT('Ctrl Pts',(-6.01195898185081,3.10622571629034,139.150880151295));
#43609=CARTESIAN_POINT('Ctrl Pts',(-6.09211525339475,2.95108688844114,139.159112216456));
#43610=CARTESIAN_POINT('Ctrl Pts',(-6.16617860691969,2.79300611590146,139.167344281616));
#43611=CARTESIAN_POINT('Ctrl Pts',(-6.23395413846561,2.63250922116285,139.175576346777));
#43612=CARTESIAN_POINT('Ctrl Pts',(-6.29487565276906,2.48824308786293,139.182975918038));
#43613=CARTESIAN_POINT('Ctrl Pts',(-6.35071739569539,2.34202521030278,139.190375489299));
#43614=CARTESIAN_POINT('Ctrl Pts',(-6.40137263913761,2.19424641617581,139.19777506056));
#43615=CARTESIAN_POINT('Ctrl Pts',(-6.46711100489098,2.00246495864534,139.207377930647));
#43616=CARTESIAN_POINT('Ctrl Pts',(-6.52428232460604,1.80756608683193,139.216980800734));
#43617=CARTESIAN_POINT('Ctrl Pts',(-6.57262117171399,1.61026082767266,139.22658367082));
#43618=CARTESIAN_POINT('Ctrl Pts',(-6.62073468961635,1.41387529746773,139.236141777591));
#43619=CARTESIAN_POINT('Ctrl Pts',(-6.66009780047818,1.21510584577315,139.245699884361));
#43620=CARTESIAN_POINT('Ctrl Pts',(-6.69049480540422,1.0146764306217,139.255257991132));
#43621=CARTESIAN_POINT('Ctrl Pts',(-6.72062522273823,0.816004820072558,
139.264732271464));
#43622=CARTESIAN_POINT('Ctrl Pts',(-6.74194604189968,0.615702336556618,
139.274206551796));
#43623=CARTESIAN_POINT('Ctrl Pts',(-6.75429365501373,0.414495140914014,
139.283680832128));
#43624=CARTESIAN_POINT('Ctrl Pts',(-6.76260829568126,0.279006158870459,
139.290060626816));
#43625=CARTESIAN_POINT('Ctrl Pts',(-6.76685507026145,0.143107377020171,
139.296440421503));
#43626=CARTESIAN_POINT('Ctrl Pts',(-6.76699635293221,0.00702562468027349,
139.30282021619));
#43627=CARTESIAN_POINT('Ctrl Pts',(-6.767,8.29220280134288E-12,139.30282021619));
#43628=CARTESIAN_POINT('Ctrl Pts',(-6.76700000000023,-0.186007249407506,
139.311569727996));
#43629=CARTESIAN_POINT('Ctrl Pts',(-6.75932637295483,-0.37201435551949,
139.320319239802));
#43630=CARTESIAN_POINT('Ctrl Pts',(-6.74400518266993,-0.557389537147142,
139.329068751608));
#43631=CARTESIAN_POINT('Ctrl Pts',(-6.7286840570973,-0.742763935803766,
139.337818226458));
#43632=CARTESIAN_POINT('Ctrl Pts',(-6.70571545653094,-0.927506129687686,
139.346567701309));
#43633=CARTESIAN_POINT('Ctrl Pts',(-6.67517739415768,-1.1109886392427,139.35531717616));
#43634=CARTESIAN_POINT('Ctrl Pts',(-6.64463945823201,-1.29447038905986,
139.364066614782));
#43635=CARTESIAN_POINT('Ctrl Pts',(-6.60653217027268,-1.47669218227726,
139.372816053404));
#43636=CARTESIAN_POINT('Ctrl Pts',(-6.56098496116829,-1.65703510503657,
139.381565492026));
#43637=CARTESIAN_POINT('Ctrl Pts',(-6.5154379368764,-1.83737729603586,139.390314895146));
#43638=CARTESIAN_POINT('Ctrl Pts',(-6.46245112202766,-2.01584035396648,
139.399064298266));
#43639=CARTESIAN_POINT('Ctrl Pts',(-6.40220448416371,-2.19181813637767,
139.407813701386));
#43640=CARTESIAN_POINT('Ctrl Pts',(-6.34195808575328,-2.36779521935566,
139.416563069732));
#43641=CARTESIAN_POINT('Ctrl Pts',(-6.27445201489388,-2.54128677544449,
139.425312438077));
#43642=CARTESIAN_POINT('Ctrl Pts',(-6.19991555136349,-2.71170355237462,
139.434061806422));
#43643=CARTESIAN_POINT('Ctrl Pts',(-6.12537937789215,-2.88211966612697,
139.442811140719));
#43644=CARTESIAN_POINT('Ctrl Pts',(-6.04381298133804,-3.04946076210075,
139.451560475016));
#43645=CARTESIAN_POINT('Ctrl Pts',(-5.95549339426503,-3.21315848206489,
139.460309809313));
#43646=CARTESIAN_POINT('Ctrl Pts',(-5.86717414355367,-3.37685557859277,
139.469059110289));
#43647=CARTESIAN_POINT('Ctrl Pts',(-5.77210188986454,-3.53690907466958,
139.477808411264));
#43648=CARTESIAN_POINT('Ctrl Pts',(-5.67059953467293,-3.69277536784559,
139.48655771224));
#43649=CARTESIAN_POINT('Ctrl Pts',(-5.56909755762015,-3.84864108035431,
139.495306980621));
#43650=CARTESIAN_POINT('Ctrl Pts',(-5.46116568338345,-4.00031938103902,
139.504056249001));
#43651=CARTESIAN_POINT('Ctrl Pts',(-5.34717048686417,-4.14729511662828,
139.512805517382));
#43652=CARTESIAN_POINT('Ctrl Pts',(-5.23317570555825,-4.29427031687666,
139.521554753895));
#43653=CARTESIAN_POINT('Ctrl Pts',(-5.11311782179116,-4.43654275986771,
139.530303990407));
#43654=CARTESIAN_POINT('Ctrl Pts',(-4.98740459172328,-4.57362924147307,
139.53905322692));
#43655=CARTESIAN_POINT('Ctrl Pts',(-4.8616918091116,-4.71071523514095,139.547802432291));
#43656=CARTESIAN_POINT('Ctrl Pts',(-4.73032391415777,-4.84261509316186,
139.556551637662));
#43657=CARTESIAN_POINT('Ctrl Pts',(-4.59374707237655,-4.96888084331189,
139.565300843033));
#43658=CARTESIAN_POINT('Ctrl Pts',(-4.45717070537763,-5.09514615452409,
139.57405001799));
#43659=CARTESIAN_POINT('Ctrl Pts',(-4.31538563819868,-5.21577720253336,
139.582799192946));
#43660=CARTESIAN_POINT('Ctrl Pts',(-4.16887341291004,-5.33036429028372,
139.591548367902));
#43661=CARTESIAN_POINT('Ctrl Pts',(-4.02236168477714,-5.44495098920899,
139.60029751317));
#43662=CARTESIAN_POINT('Ctrl Pts',(-3.87112305634835,-5.55349359238483,
139.609046658438));
#43663=CARTESIAN_POINT('Ctrl Pts',(-3.71567117317149,-5.655623461022,139.617795803706));
#43664=CARTESIAN_POINT('Ctrl Pts',(-3.56021980457719,-5.75775299158511,
139.626544920012));
#43665=CARTESIAN_POINT('Ctrl Pts',(-3.40055544862808,-5.85346967275109,
139.635294036318));
#43666=CARTESIAN_POINT('Ctrl Pts',(-3.23722036323824,-5.94244842803332,
139.644043152624));
#43667=CARTESIAN_POINT('Ctrl Pts',(-3.07388580496478,-6.03142689616255,
139.652792240695));
#43668=CARTESIAN_POINT('Ctrl Pts',(-2.90688079258149,-6.11366734484612,
139.661541328766));
#43669=CARTESIAN_POINT('Ctrl Pts',(-2.73677251095066,-6.18889046787102,
139.670290416837));
#43670=CARTESIAN_POINT('Ctrl Pts',(-2.56666476417112,-6.26411335438079,
139.679039477399));
#43671=CARTESIAN_POINT('Ctrl Pts',(-2.39345402972576,-6.33231884350108,
139.687788537962));
#43672=CARTESIAN_POINT('Ctrl Pts',(-2.21772856474536,-6.3932752962087,139.696537598524));
#43673=CARTESIAN_POINT('Ctrl Pts',(-2.04200363768781,-6.45423156231919,
139.705286632304));
#43674=CARTESIAN_POINT('Ctrl Pts',(-1.86376426620618,-6.50793874251905,
139.714035666084));
#43675=CARTESIAN_POINT('Ctrl Pts',(-1.68361578195226,-6.55421443795985,
139.722784699864));
#43676=CARTESIAN_POINT('Ctrl Pts',(-1.50346783420434,-6.6004899955855,139.731533707588));
#43677=CARTESIAN_POINT('Ctrl Pts',(-1.32141106257841,-6.63933404145376,
139.740282715312));
#43678=CARTESIAN_POINT('Ctrl Pts',(-1.13806375959667,-6.67061465526924,
139.749031723036));
#43679=CARTESIAN_POINT('Ctrl Pts',(-0.954716987425224,-6.70189517852395,
139.757780705431));
#43680=CARTESIAN_POINT('Ctrl Pts',(-0.770079973815777,-6.72561226535761,
139.766529687826));
#43681=CARTESIAN_POINT('Ctrl Pts',(-0.584779770558182,-6.74168536939732,
139.775278670221));
#43682=CARTESIAN_POINT('Ctrl Pts',(-0.39149064755964,-6.75845143942361,
139.784404850897));
#43683=CARTESIAN_POINT('Ctrl Pts',(-0.19748021311006,-6.7668997592401,139.793531031573));
#43684=CARTESIAN_POINT('Ctrl Pts',(-0.00346532630350954,-6.76699911271707,
139.802657212249));
#43685=CARTESIAN_POINT('Ctrl Pts',(0.184486595290432,-6.76709536139789,
139.811498199779));
#43686=CARTESIAN_POINT('Ctrl Pts',(0.372442378179701,-6.75935659726801,
139.820339187309));
#43687=CARTESIAN_POINT('Ctrl Pts',(0.55975021771666,-6.74380965729062,139.829180174839));
#43688=CARTESIAN_POINT('Ctrl Pts',(0.74512991445234,-6.72842275717313,139.837930153437));
#43689=CARTESIAN_POINT('Ctrl Pts',(0.929874656308788,-6.70538772273548,
139.846680132035));
#43690=CARTESIAN_POINT('Ctrl Pts',(1.1133568828924,-6.67478280180832,139.855430110632));
#43691=CARTESIAN_POINT('Ctrl Pts',(1.29683723118321,-6.64417819418128,139.864179999657));
#43692=CARTESIAN_POINT('Ctrl Pts',(1.47905480729703,-6.60600390230194,139.872929888682));
#43693=CARTESIAN_POINT('Ctrl Pts',(1.65939064804279,-6.56038959797268,139.881679777707));
#43694=CARTESIAN_POINT('Ctrl Pts',(1.83972470263745,-6.51477574543403,139.890429580068));
#43695=CARTESIAN_POINT('Ctrl Pts',(2.01817678125337,-6.4617220982026,139.899179382429));
#43696=CARTESIAN_POINT('Ctrl Pts',(2.19414072347178,-6.40140886724186,139.90792918479));
#43697=CARTESIAN_POINT('Ctrl Pts',(2.37010298131595,-6.34109621361562,139.916678903396));
#43698=CARTESIAN_POINT('Ctrl Pts',(2.54357687926412,-6.27352420826174,139.925428622001));
#43699=CARTESIAN_POINT('Ctrl Pts',(2.71397317789471,-6.19892237325715,139.934178340607));
#43700=CARTESIAN_POINT('Ctrl Pts',(2.884367902067,-6.12432122757199,139.942927978365));
#43701=CARTESIAN_POINT('Ctrl Pts',(3.05168482125755,-6.0426904971767,139.951677616123));
#43702=CARTESIAN_POINT('Ctrl Pts',(3.21535561996888,-5.954307452352,139.960427253881));
#43703=CARTESIAN_POINT('Ctrl Pts',(3.37902496074775,-5.86592519481807,139.9691768137));
#43704=CARTESIAN_POINT('Ctrl Pts',(3.53904799384366,-5.77079087940544,139.977926373519));
#43705=CARTESIAN_POINT('Ctrl Pts',(3.69488118814473,-5.66922763747358,139.986675933338));
#43706=CARTESIAN_POINT('Ctrl Pts',(3.85071304610322,-5.56766526649405,139.995425418126));
#43707=CARTESIAN_POINT('Ctrl Pts',(4.00235489705458,-5.45967423581087,140.004174902913));
#43708=CARTESIAN_POINT('Ctrl Pts',(4.14929168607147,-5.34562133936722,140.012924387701));
#43709=CARTESIAN_POINT('Ctrl Pts',(4.29622726385251,-5.23156938308946,140.021673800364));
#43710=CARTESIAN_POINT('Ctrl Pts',(4.43845763091563,-5.11145583677639,140.030423213027));
#43711=CARTESIAN_POINT('Ctrl Pts',(4.57549970660462,-4.98568866204671,140.03917262569));
#43712=CARTESIAN_POINT('Ctrl Pts',(4.7125406981481,-4.85992248226632,140.047921969137));
#43713=CARTESIAN_POINT('Ctrl Pts',(4.84439326930845,-4.72850295734483,140.056671312583));
#43714=CARTESIAN_POINT('Ctrl Pts',(4.97060959434245,-4.59187644222172,140.06542065603));
#43715=CARTESIAN_POINT('Ctrl Pts',(5.0968249628008,-4.45525096257162,140.074169933166));
#43716=CARTESIAN_POINT('Ctrl Pts',(5.21740397615422,-4.3134187821883,140.082919210302));
#43717=CARTESIAN_POINT('Ctrl Pts',(5.33193710451536,-4.16686161439187,140.091668487438));
#43718=CARTESIAN_POINT('Ctrl Pts',(5.44646940289003,-4.02030550865029,140.100417701171));
#43719=CARTESIAN_POINT('Ctrl Pts',(5.55495572749303,-3.86902470980653,140.109166914904));
#43720=CARTESIAN_POINT('Ctrl Pts',(5.65702762491113,-3.71353301466304,140.117916128637));
#43721=CARTESIAN_POINT('Ctrl Pts',(5.75909881654827,-3.55804239467423,140.126665281873));
#43722=CARTESIAN_POINT('Ctrl Pts',(5.85475551250471,-3.39834117620089,140.13541443511));
#43723=CARTESIAN_POINT('Ctrl Pts',(5.943672837278,-3.23497174692511,140.144163588346));
#43724=CARTESIAN_POINT('Ctrl Pts',(6.0325895767604,-3.071603393015,140.152912683991));
#43725=CARTESIAN_POINT('Ctrl Pts',(6.11476689685035,-2.90456712830031,140.161661779637));
#43726=CARTESIAN_POINT('Ctrl Pts',(6.18992570525032,-2.73443024476422,140.170410875282));
#43727=CARTESIAN_POINT('Ctrl Pts',(6.26508404388486,-2.56429442463547,140.179159916243));
#43728=CARTESIAN_POINT('Ctrl Pts',(6.3332238428312,-2.39105828656509,140.187908957204));
#43729=CARTESIAN_POINT('Ctrl Pts',(6.39411368719854,-2.21531017132597,140.196657998165));
#43730=CARTESIAN_POINT('Ctrl Pts',(6.45500317120724,-2.03956309620039,140.205406987348));
#43731=CARTESIAN_POINT('Ctrl Pts',(6.50864269269921,-1.86130434439165,140.21415597653));
#43732=CARTESIAN_POINT('Ctrl Pts',(6.55485008446195,-1.68113930720483,140.222904965713));
#43733=CARTESIAN_POINT('Ctrl Pts',(6.60199664749285,-1.49731239212364,140.231831779242));
#43734=CARTESIAN_POINT('Ctrl Pts',(6.64140563640806,-1.31150116500181,140.240758592771));
#43735=CARTESIAN_POINT('Ctrl Pts',(6.67293772282089,-1.12436255156154,140.249685406301));
#43736=CARTESIAN_POINT('Ctrl Pts',(6.70384494949803,-0.940932395056238,
140.258435320456));
#43737=CARTESIAN_POINT('Ctrl Pts',(6.72718449348876,-0.756227260511558,
140.267185234612));
#43738=CARTESIAN_POINT('Ctrl Pts',(6.74287707373892,-0.570874564546478,
140.275935148767));
#43739=CARTESIAN_POINT('Ctrl Pts',(6.75856934538643,-0.385525513637225,
140.284684890851));
#43740=CARTESIAN_POINT('Ctrl Pts',(6.76661493004089,-0.199529212422936,
140.293434632935));
#43741=CARTESIAN_POINT('Ctrl Pts',(6.76698649908906,-0.0135174386050861,
140.302184375019));
#43742=CARTESIAN_POINT('Ctrl Pts',(6.76735806132401,0.172490924441198,140.310933956665));
#43743=CARTESIAN_POINT('Ctrl Pts',(6.76005588896313,0.35851447289691,140.319683538311));
#43744=CARTESIAN_POINT('Ctrl Pts',(6.7451047845462,0.543921359657803,140.328433119957));
#43745=CARTESIAN_POINT('Ctrl Pts',(6.73015393440735,0.729325093146103,140.337182552796));
#43746=CARTESIAN_POINT('Ctrl Pts',(6.70755443556955,0.914111900252082,140.345931985635));
#43747=CARTESIAN_POINT('Ctrl Pts',(6.67738304682388,1.09765415591119,140.354681418474));
#43748=CARTESIAN_POINT('Ctrl Pts',(6.6472121311194,1.28119353390863,140.363430714135));
#43749=CARTESIAN_POINT('Ctrl Pts',(6.60946960955583,1.46348811672254,140.372180009797));
#43750=CARTESIAN_POINT('Ctrl Pts',(6.5642836699128,1.64391876347833,140.380929305458));
#43751=CARTESIAN_POINT('Ctrl Pts',(6.51909837867823,1.8243468210934,140.389678475569));
#43752=CARTESIAN_POINT('Ctrl Pts',(6.46646995272034,2.00291071820082,140.39842764568));
#43753=CARTESIAN_POINT('Ctrl Pts',(6.40657713281668,2.17900400212353,140.407176815791));
#43754=CARTESIAN_POINT('Ctrl Pts',(6.34668509279189,2.3550949930931,140.415925871976));
#43755=CARTESIAN_POINT('Ctrl Pts',(6.27952894037665,2.52871516397778,140.424674928162));
#43756=CARTESIAN_POINT('Ctrl Pts',(6.20533675061595,2.69927486771078,140.433423984348));
#43757=CARTESIAN_POINT('Ctrl Pts',(6.12832117908069,2.87632521635599,140.44250598563));
#43758=CARTESIAN_POINT('Ctrl Pts',(6.04372366626235,3.0500772891969,140.451587986912));
#43759=CARTESIAN_POINT('Ctrl Pts',(5.95185378008025,3.21989527477906,140.460669988195));
#43760=CARTESIAN_POINT('Ctrl Pts',(5.86334450817532,3.38350129286473,140.469419768502));
#43761=CARTESIAN_POINT('Ctrl Pts',(5.7680856205742,3.54345567124695,140.478169548809));
#43762=CARTESIAN_POINT('Ctrl Pts',(5.66640068804651,3.69921508465054,140.486919329116));
#43763=CARTESIAN_POINT('Ctrl Pts',(5.56471941108094,3.85496889852037,140.49566879487));
#43764=CARTESIAN_POINT('Ctrl Pts',(5.45661270815287,4.00652780919401,140.504418260623));
#43765=CARTESIAN_POINT('Ctrl Pts',(5.3424477644929,4.15337704569003,140.513167726377));
#43766=CARTESIAN_POINT('Ctrl Pts',(5.22828631819778,4.30022178356027,140.521916924096));
#43767=CARTESIAN_POINT('Ctrl Pts',(5.10806717844259,4.44235690972461,140.530666121816));
#43768=CARTESIAN_POINT('Ctrl Pts',(4.98219864544916,4.57929969070431,140.539415319535));
#43769=CARTESIAN_POINT('Ctrl Pts',(4.85633329944237,4.71623900429782,140.548164295726));
#43770=CARTESIAN_POINT('Ctrl Pts',(4.72481904033877,4.84798602483394,140.556913271916));
#43771=CARTESIAN_POINT('Ctrl Pts',(4.58810250737444,4.97409332258899,140.565662248106));
#43772=CARTESIAN_POINT('Ctrl Pts',(4.45137708685898,5.10020881821912,140.574411793042));
#43773=CARTESIAN_POINT('Ctrl Pts',(4.30944892636317,5.22068366307714,140.583161337978));
#43774=CARTESIAN_POINT('Ctrl Pts',(4.16280009466937,5.33510865604635,140.591910882915));
#43775=CARTESIAN_POINT('Ctrl Pts',(4.01615988349057,5.44952692272694,140.600659913523));
#43776=CARTESIAN_POINT('Ctrl Pts',(3.8647997823249,5.55789587288446,140.609408944131));
#43777=CARTESIAN_POINT('Ctrl Pts',(3.70923383581317,5.65984746713714,140.618157974739));
#43778=CARTESIAN_POINT('Ctrl Pts',(3.55366577799787,5.76180044505231,140.626907124087));
#43779=CARTESIAN_POINT('Ctrl Pts',(3.39389200027082,5.85733573570919,140.635656273435));
#43780=CARTESIAN_POINT('Ctrl Pts',(3.23045513626279,5.94612887621799,140.644405422784));
#43781=CARTESIAN_POINT('Ctrl Pts',(3.18695122151738,5.96976399206604,140.646734286897));
#43782=CARTESIAN_POINT('Ctrl Pts',(3.14318791262744,5.99292165435291,140.64906315101));
#43783=CARTESIAN_POINT('Ctrl Pts',(3.09917575053259,6.01559628526639,140.651392015123));
#43784=CARTESIAN_POINT('Origin',(0.,0.,-3.69717978381041));
#43785=CARTESIAN_POINT('',(3.09917575053276,6.0155962852663,143.045751582742));
#43786=CARTESIAN_POINT('',(3.09917575053256,6.0155962852664,142.651137628792));
#43787=CARTESIAN_POINT('',(3.09917575053259,6.01559628526639,-3.69717978381041));
#43788=CARTESIAN_POINT('',(-6.767,8.61074883271029E-12,141.69717978381));
#43789=CARTESIAN_POINT('Ctrl Pts',(-6.767,8.61074887974675E-12,141.69717978381));
#43790=CARTESIAN_POINT('Ctrl Pts',(-6.76700000000024,-0.186007249407185,
141.705929295616));
#43791=CARTESIAN_POINT('Ctrl Pts',(-6.75932637295485,-0.372014355519164,
141.714678807422));
#43792=CARTESIAN_POINT('Ctrl Pts',(-6.74400518266996,-0.557389537146815,
141.723428319228));
#43793=CARTESIAN_POINT('Ctrl Pts',(-6.72868405709736,-0.742763935803183,
141.732177794078));
#43794=CARTESIAN_POINT('Ctrl Pts',(-6.70571545653104,-0.927506129686851,
141.740927268929));
#43795=CARTESIAN_POINT('Ctrl Pts',(-6.67517739415786,-1.11098863924161,
141.74967674378));
#43796=CARTESIAN_POINT('Ctrl Pts',(-6.64463945823222,-1.29447038905877,
141.758426182402));
#43797=CARTESIAN_POINT('Ctrl Pts',(-6.60653217027292,-1.47669218227619,
141.767175621023));
#43798=CARTESIAN_POINT('Ctrl Pts',(-6.56098496116856,-1.6570351050355,141.775925059645));
#43799=CARTESIAN_POINT('Ctrl Pts',(-6.5154379368767,-1.8373772960348,141.784674462766));
#43800=CARTESIAN_POINT('Ctrl Pts',(-6.46245112202799,-2.01584035396542,
141.793423865886));
#43801=CARTESIAN_POINT('Ctrl Pts',(-6.40220448416407,-2.19181813637662,
141.802173269006));
#43802=CARTESIAN_POINT('Ctrl Pts',(-6.34195808575363,-2.36779521935474,
141.810922637351));
#43803=CARTESIAN_POINT('Ctrl Pts',(-6.2744520148942,-2.54128677544369,141.819672005697));
#43804=CARTESIAN_POINT('Ctrl Pts',(-6.19991555136379,-2.71170355237395,
141.828421374042));
#43805=CARTESIAN_POINT('Ctrl Pts',(-6.12537937789256,-2.88211966612607,
141.837170708339));
#43806=CARTESIAN_POINT('Ctrl Pts',(-6.04381298133859,-3.04946076209963,
141.845920042636));
#43807=CARTESIAN_POINT('Ctrl Pts',(-5.95549339426575,-3.21315848206357,
141.854669376933));
#43808=CARTESIAN_POINT('Ctrl Pts',(-5.86717414355442,-3.37685557859146,
141.863418677909));
#43809=CARTESIAN_POINT('Ctrl Pts',(-5.77210188986533,-3.5369090746683,141.872167978884));
#43810=CARTESIAN_POINT('Ctrl Pts',(-5.67059953467376,-3.69277536784433,
141.88091727986));
#43811=CARTESIAN_POINT('Ctrl Pts',(-5.5690975576208,-3.84864108035339,141.889666548241));
#43812=CARTESIAN_POINT('Ctrl Pts',(-5.4611656833839,-4.00031938103843,141.898415816621));
#43813=CARTESIAN_POINT('Ctrl Pts',(-5.34717048686439,-4.147295116628,141.907165085002));
#43814=CARTESIAN_POINT('Ctrl Pts',(-5.23317570555848,-4.29427031687638,
141.915914321515));
#43815=CARTESIAN_POINT('Ctrl Pts',(-5.1131178217914,-4.43654275986744,141.924663558027));
#43816=CARTESIAN_POINT('Ctrl Pts',(-4.98740459172353,-4.57362924147281,
141.93341279454));
#43817=CARTESIAN_POINT('Ctrl Pts',(-4.86169180911176,-4.71071523514079,
141.942161999911));
#43818=CARTESIAN_POINT('Ctrl Pts',(-4.73032391415785,-4.84261509316178,
141.950911205282));
#43819=CARTESIAN_POINT('Ctrl Pts',(-4.59374707237654,-4.9688808433119,141.959660410653));
#43820=CARTESIAN_POINT('Ctrl Pts',(-4.45717070537781,-5.09514615452392,
141.96840958561));
#43821=CARTESIAN_POINT('Ctrl Pts',(-4.31538563819906,-5.21577720253303,
141.977158760566));
#43822=CARTESIAN_POINT('Ctrl Pts',(-4.16887341291064,-5.33036429028325,
141.985907935522));
#43823=CARTESIAN_POINT('Ctrl Pts',(-4.02236168477765,-5.44495098920861,
141.99465708079));
#43824=CARTESIAN_POINT('Ctrl Pts',(-3.87112305634876,-5.55349359238454,
142.003406226058));
#43825=CARTESIAN_POINT('Ctrl Pts',(-3.7156711731718,-5.65562346102179,142.012155371326));
#43826=CARTESIAN_POINT('Ctrl Pts',(-3.56021980457752,-5.7577529915849,142.020904487632));
#43827=CARTESIAN_POINT('Ctrl Pts',(-3.40055544862841,-5.8534696727509,142.029653603938));
#43828=CARTESIAN_POINT('Ctrl Pts',(-3.23722036323858,-5.94244842803314,
142.038402720244));
#43829=CARTESIAN_POINT('Ctrl Pts',(-3.07388580496535,-6.03142689616225,
142.047151808315));
#43830=CARTESIAN_POINT('Ctrl Pts',(-2.9068807925823,-6.11366734484573,142.055900896386));
#43831=CARTESIAN_POINT('Ctrl Pts',(-2.73677251095172,-6.18889046787056,
142.064649984457));
#43832=CARTESIAN_POINT('Ctrl Pts',(-2.56666476417208,-6.2641133543804,142.073399045019));
#43833=CARTESIAN_POINT('Ctrl Pts',(-2.39345402972661,-6.33231884350076,
142.082148105582));
#43834=CARTESIAN_POINT('Ctrl Pts',(-2.2177285647461,-6.39327529620845,142.090897166144));
#43835=CARTESIAN_POINT('Ctrl Pts',(-2.04200363768844,-6.454231562319,142.099646199924));
#43836=CARTESIAN_POINT('Ctrl Pts',(-1.86376426620669,-6.50793874251891,
142.108395233704));
#43837=CARTESIAN_POINT('Ctrl Pts',(-1.68361578195264,-6.55421443795975,
142.117144267484));
#43838=CARTESIAN_POINT('Ctrl Pts',(-1.50346783420461,-6.60048999558544,
142.125893275208));
#43839=CARTESIAN_POINT('Ctrl Pts',(-1.32141106257856,-6.63933404145374,
142.134642282932));
#43840=CARTESIAN_POINT('Ctrl Pts',(-1.13806375959669,-6.67061465526923,
142.143391290656));
#43841=CARTESIAN_POINT('Ctrl Pts',(-0.954716987425243,-6.70189517852394,
142.152140273051));
#43842=CARTESIAN_POINT('Ctrl Pts',(-0.770079973815802,-6.7256122653576,
142.160889255446));
#43843=CARTESIAN_POINT('Ctrl Pts',(-0.584779770558209,-6.74168536939732,
142.169638237841));
#43844=CARTESIAN_POINT('Ctrl Pts',(-0.391490647559668,-6.75845143942361,
142.178764418517));
#43845=CARTESIAN_POINT('Ctrl Pts',(-0.197480213110089,-6.7668997592401,
142.187890599193));
#43846=CARTESIAN_POINT('Ctrl Pts',(-0.0034653263035411,-6.76699911271707,
142.197016779869));
#43847=CARTESIAN_POINT('Ctrl Pts',(0.184486595290399,-6.76709536139789,
142.205857767399));
#43848=CARTESIAN_POINT('Ctrl Pts',(0.372442378179669,-6.75935659726801,
142.214698754929));
#43849=CARTESIAN_POINT('Ctrl Pts',(0.559750217716626,-6.74380965729062,
142.223539742459));
#43850=CARTESIAN_POINT('Ctrl Pts',(0.745129914452304,-6.72842275717314,
142.232289721057));
#43851=CARTESIAN_POINT('Ctrl Pts',(0.929874656308751,-6.70538772273548,
142.241039699655));
#43852=CARTESIAN_POINT('Ctrl Pts',(1.11335688289236,-6.67478280180833,142.249789678252));
#43853=CARTESIAN_POINT('Ctrl Pts',(1.29683723118317,-6.64417819418129,142.258539567277));
#43854=CARTESIAN_POINT('Ctrl Pts',(1.47905480729698,-6.60600390230195,142.267289456302));
#43855=CARTESIAN_POINT('Ctrl Pts',(1.65939064804274,-6.56038959797269,142.276039345327));
#43856=CARTESIAN_POINT('Ctrl Pts',(1.83972470263728,-6.51477574543408,142.284789147688));
#43857=CARTESIAN_POINT('Ctrl Pts',(2.01817678125308,-6.46172209820268,142.293538950049));
#43858=CARTESIAN_POINT('Ctrl Pts',(2.19414072347137,-6.401408867242,142.30228875241));
#43859=CARTESIAN_POINT('Ctrl Pts',(2.37010298131555,-6.34109621361577,142.311038471016));
#43860=CARTESIAN_POINT('Ctrl Pts',(2.54357687926371,-6.2735242082619,142.319788189621));
#43861=CARTESIAN_POINT('Ctrl Pts',(2.71397317789431,-6.19892237325733,142.328537908227));
#43862=CARTESIAN_POINT('Ctrl Pts',(2.8843679020666,-6.12432122757218,142.337287545985));
#43863=CARTESIAN_POINT('Ctrl Pts',(3.05168482125716,-6.0426904971769,142.346037183743));
#43864=CARTESIAN_POINT('Ctrl Pts',(3.21535561996849,-5.95430745235221,142.354786821501));
#43865=CARTESIAN_POINT('Ctrl Pts',(3.37902496074748,-5.86592519481823,142.36353638132));
#43866=CARTESIAN_POINT('Ctrl Pts',(3.5390479938435,-5.77079087940554,142.372285941139));
#43867=CARTESIAN_POINT('Ctrl Pts',(3.69488118814467,-5.66922763747361,142.381035500958));
#43868=CARTESIAN_POINT('Ctrl Pts',(3.85071304610327,-5.56766526649402,142.389784985746));
#43869=CARTESIAN_POINT('Ctrl Pts',(4.00235489705474,-5.45967423581076,142.398534470533));
#43870=CARTESIAN_POINT('Ctrl Pts',(4.14929168607172,-5.34562133936703,142.407283955321));
#43871=CARTESIAN_POINT('Ctrl Pts',(4.29622726385275,-5.23156938308926,142.416033367984));
#43872=CARTESIAN_POINT('Ctrl Pts',(4.43845763091587,-5.11145583677619,142.424782780647));
#43873=CARTESIAN_POINT('Ctrl Pts',(4.57549970660485,-4.9856886620465,142.433532193311));
#43874=CARTESIAN_POINT('Ctrl Pts',(4.71254069814832,-4.8599224822661,142.442281536757));
#43875=CARTESIAN_POINT('Ctrl Pts',(4.84439326930866,-4.72850295734461,142.451030880203));
#43876=CARTESIAN_POINT('Ctrl Pts',(4.97060959434265,-4.5918764422215,142.45978022365));
#43877=CARTESIAN_POINT('Ctrl Pts',(5.096824962801,-4.45525096257139,142.468529500786));
#43878=CARTESIAN_POINT('Ctrl Pts',(5.21740397615442,-4.31341878218807,142.477278777922));
#43879=CARTESIAN_POINT('Ctrl Pts',(5.33193710451554,-4.16686161439163,142.486028055058));
#43880=CARTESIAN_POINT('Ctrl Pts',(5.44646940289021,-4.02030550865005,142.494777268791));
#43881=CARTESIAN_POINT('Ctrl Pts',(5.5549557274932,-3.86902470980628,142.503526482524));
#43882=CARTESIAN_POINT('Ctrl Pts',(5.65702762491129,-3.7135330146628,142.512275696257));
#43883=CARTESIAN_POINT('Ctrl Pts',(5.75909881654849,-3.55804239467387,142.521024849493));
#43884=CARTESIAN_POINT('Ctrl Pts',(5.85475551250499,-3.39834117620041,142.52977400273));
#43885=CARTESIAN_POINT('Ctrl Pts',(5.94367283727832,-3.23497174692451,142.538523155966));
#43886=CARTESIAN_POINT('Ctrl Pts',(6.0325895767607,-3.07160339301441,142.547272251611));
#43887=CARTESIAN_POINT('Ctrl Pts',(6.11476689685063,-2.9045671282997,142.556021347257));
#43888=CARTESIAN_POINT('Ctrl Pts',(6.18992570525059,-2.73443024476361,142.564770442902));
#43889=CARTESIAN_POINT('Ctrl Pts',(6.26508404388511,-2.56429442463485,142.573519483863));
#43890=CARTESIAN_POINT('Ctrl Pts',(6.33322384283144,-2.39105828656447,142.582268524824));
#43891=CARTESIAN_POINT('Ctrl Pts',(6.39411368719876,-2.21531017132534,142.591017565785));
#43892=CARTESIAN_POINT('Ctrl Pts',(6.45500317120744,-2.03956309619975,142.599766554968));
#43893=CARTESIAN_POINT('Ctrl Pts',(6.50864269269939,-1.86130434439101,142.60851554415));
#43894=CARTESIAN_POINT('Ctrl Pts',(6.55485008446212,-1.68113930720419,142.617264533333));
#43895=CARTESIAN_POINT('Ctrl Pts',(6.60199664749297,-1.49731239212313,142.626191346862));
#43896=CARTESIAN_POINT('Ctrl Pts',(6.64140563640814,-1.31150116500142,142.635118160391));
#43897=CARTESIAN_POINT('Ctrl Pts',(6.67293772282093,-1.12436255156127,142.644044973921));
#43898=CARTESIAN_POINT('Ctrl Pts',(6.70384494949804,-0.9409323950561,142.652794888076));
#43899=CARTESIAN_POINT('Ctrl Pts',(6.72718449348876,-0.75622726051155,142.661544802232));
#43900=CARTESIAN_POINT('Ctrl Pts',(6.74287707373891,-0.5708745645466,142.670294716387));
#43901=CARTESIAN_POINT('Ctrl Pts',(6.75856934538643,-0.385525513637349,
142.679044458471));
#43902=CARTESIAN_POINT('Ctrl Pts',(6.76661493004089,-0.199529212423061,
142.687794200555));
#43903=CARTESIAN_POINT('Ctrl Pts',(6.76698649908906,-0.0135174386052131,
142.696543942639));
#43904=CARTESIAN_POINT('Ctrl Pts',(6.76735806132401,0.172490924441069,142.705293524285));
#43905=CARTESIAN_POINT('Ctrl Pts',(6.76005588896314,0.358514472896781,142.714043105931));
#43906=CARTESIAN_POINT('Ctrl Pts',(6.74510478454621,0.543921359657673,142.722792687577));
#43907=CARTESIAN_POINT('Ctrl Pts',(6.73015393440736,0.729325093145971,142.731542120416));
#43908=CARTESIAN_POINT('Ctrl Pts',(6.70755443556957,0.914111900251948,142.740291553255));
#43909=CARTESIAN_POINT('Ctrl Pts',(6.6773830468239,1.09765415591105,142.749040986094));
#43910=CARTESIAN_POINT('Ctrl Pts',(6.64721213111942,1.2811935339085,142.757790281755));
#43911=CARTESIAN_POINT('Ctrl Pts',(6.60946960955586,1.4634881167224,142.766539577417));
#43912=CARTESIAN_POINT('Ctrl Pts',(6.56428366991284,1.64391876347819,142.775288873078));
#43913=CARTESIAN_POINT('Ctrl Pts',(6.5190983786783,1.82434682109313,142.784038043189));
#43914=CARTESIAN_POINT('Ctrl Pts',(6.46646995272046,2.00291071820043,142.7927872133));
#43915=CARTESIAN_POINT('Ctrl Pts',(6.40657713281685,2.17900400212303,142.801536383411));
#43916=CARTESIAN_POINT('Ctrl Pts',(6.34668509279207,2.3550949930926,142.810285439596));
#43917=CARTESIAN_POINT('Ctrl Pts',(6.27952894037685,2.52871516397728,142.819034495782));
#43918=CARTESIAN_POINT('Ctrl Pts',(6.20533675061617,2.69927486771029,142.827783551968));
#43919=CARTESIAN_POINT('Ctrl Pts',(6.12832117908092,2.8763252163555,142.83686555325));
#43920=CARTESIAN_POINT('Ctrl Pts',(6.04372366626259,3.05007728919642,142.845947554532));
#43921=CARTESIAN_POINT('Ctrl Pts',(5.9518537800805,3.21989527477858,142.855029555815));
#43922=CARTESIAN_POINT('Ctrl Pts',(5.86334450817565,3.38350129286415,142.863779336122));
#43923=CARTESIAN_POINT('Ctrl Pts',(5.76808562057461,3.54345567124627,142.872529116429));
#43924=CARTESIAN_POINT('Ctrl Pts',(5.66640068804702,3.69921508464976,142.881278896736));
#43925=CARTESIAN_POINT('Ctrl Pts',(5.56471941108154,3.8549688985195,142.89002836249));
#43926=CARTESIAN_POINT('Ctrl Pts',(5.45661270815357,4.00652780919305,142.898777828243));
#43927=CARTESIAN_POINT('Ctrl Pts',(5.34244776449371,4.15337704568899,142.907527293997));
#43928=CARTESIAN_POINT('Ctrl Pts',(5.22828631819854,4.30022178355935,142.916276491716));
#43929=CARTESIAN_POINT('Ctrl Pts',(5.10806717844329,4.4423569097238,142.925025689436));
#43930=CARTESIAN_POINT('Ctrl Pts',(4.98219864544979,4.57929969070362,142.933774887155));
#43931=CARTESIAN_POINT('Ctrl Pts',(4.85633329944285,4.71623900429733,142.942523863346));
#43932=CARTESIAN_POINT('Ctrl Pts',(4.72481904033908,4.84798602483364,142.951272839536));
#43933=CARTESIAN_POINT('Ctrl Pts',(4.58810250737457,4.97409332258887,142.960021815726));
#43934=CARTESIAN_POINT('Ctrl Pts',(4.45137708685902,5.10020881821909,142.968771360662));
#43935=CARTESIAN_POINT('Ctrl Pts',(4.30944892636311,5.22068366307719,142.977520905598));
#43936=CARTESIAN_POINT('Ctrl Pts',(4.16280009466921,5.33510865604648,142.986270450535));
#43937=CARTESIAN_POINT('Ctrl Pts',(4.01615988349061,5.4495269227269,142.995019481143));
#43938=CARTESIAN_POINT('Ctrl Pts',(3.86479978232516,5.55789587288428,143.003768511751));
#43939=CARTESIAN_POINT('Ctrl Pts',(3.70923383581365,5.65984746713683,143.012517542359));
#43940=CARTESIAN_POINT('Ctrl Pts',(3.55366577799846,5.76180044505194,143.021266691707));
#43941=CARTESIAN_POINT('Ctrl Pts',(3.39389200027154,5.85733573570877,143.030015841055));
#43942=CARTESIAN_POINT('Ctrl Pts',(3.23045513626363,5.94612887621753,143.038764990403));
#43943=CARTESIAN_POINT('Ctrl Pts',(3.186951221518,5.96976399206571,143.041093854516));
#43944=CARTESIAN_POINT('Ctrl Pts',(3.14318791262784,5.99292165435271,143.04342271863));
#43945=CARTESIAN_POINT('Ctrl Pts',(3.09917575053276,6.0155962852663,143.045751582743));
#43946=CARTESIAN_POINT('Ctrl Pts',(3.09917575053271,6.01559628526633,141.045900408649));
#43947=CARTESIAN_POINT('Ctrl Pts',(2.94392531879992,6.09557977326476,141.054101057528));
#43948=CARTESIAN_POINT('Ctrl Pts',(2.78549957819497,6.16958901908825,141.062301706407));
#43949=CARTESIAN_POINT('Ctrl Pts',(2.62440023039033,6.23737223762757,141.070502355286));
#43950=CARTESIAN_POINT('Ctrl Pts',(2.46049844904947,6.30633459169672,141.078845660071));
#43951=CARTESIAN_POINT('Ctrl Pts',(2.29382951096609,6.36885211567673,141.087188964856));
#43952=CARTESIAN_POINT('Ctrl Pts',(2.12494493933669,6.42470995491527,141.095532269641));
#43953=CARTESIAN_POINT('Ctrl Pts',(1.958977437471,6.47960298598729,141.103731464151));
#43954=CARTESIAN_POINT('Ctrl Pts',(1.79087057807845,6.5280644314441,141.111930658661));
#43955=CARTESIAN_POINT('Ctrl Pts',(1.62116474209249,6.5699401731672,141.120129853171));
#43956=CARTESIAN_POINT('Ctrl Pts',(1.45143515441507,6.61182177573587,141.128330195223));
#43957=CARTESIAN_POINT('Ctrl Pts',(1.28010649233721,6.6471157521242,141.136530537276));
#43958=CARTESIAN_POINT('Ctrl Pts',(1.10773096853083,6.67571877039153,141.144730879329));
#43959=CARTESIAN_POINT('Ctrl Pts',(0.935300048529582,6.70433098078973,141.152933856719));
#43960=CARTESIAN_POINT('Ctrl Pts',(0.761821950131028,6.72624789093049,141.16113683411));
#43961=CARTESIAN_POINT('Ctrl Pts',(0.587855728529647,6.74141785104846,141.1693398115));
#43962=CARTESIAN_POINT('Ctrl Pts',(0.408647442634721,6.75704492235468,141.177789966386));
#43963=CARTESIAN_POINT('Ctrl Pts',(0.228921566005123,6.765512031444,141.186240121272));
#43964=CARTESIAN_POINT('Ctrl Pts',(0.0492902242368824,6.76682048482112,
141.194690276157));
#43965=CARTESIAN_POINT('Ctrl Pts',(-0.125385348580903,6.76809283986175,
141.202907303489));
#43966=CARTESIAN_POINT('Ctrl Pts',(-0.299971179635794,6.76259637893075,
141.211124330822));
#43967=CARTESIAN_POINT('Ctrl Pts',(-0.473909036402681,6.75038511680748,
141.219341358154));
#43968=CARTESIAN_POINT('Ctrl Pts',(-0.655249151676379,6.73765418104553,
141.227908076816));
#43969=CARTESIAN_POINT('Ctrl Pts',(-0.835884485223362,6.71762445440569,
141.236474795479));
#43970=CARTESIAN_POINT('Ctrl Pts',(-1.01519399128521,6.69041629198501,141.245041514141));
#43971=CARTESIAN_POINT('Ctrl Pts',(-1.19450349734705,6.66320812956433,141.253608232803));
#43972=CARTESIAN_POINT('Ctrl Pts',(-1.37248676300084,6.62882168162202,141.262174951465));
#43973=CARTESIAN_POINT('Ctrl Pts',(-1.54854076241575,6.58743580668054,141.270741670128));
#43974=CARTESIAN_POINT('Ctrl Pts',(-1.71611079516019,6.54804429928992,141.278895562294));
#43975=CARTESIAN_POINT('Ctrl Pts',(-1.8824512869401,6.50219016550125,141.287049454461));
#43976=CARTESIAN_POINT('Ctrl Pts',(-2.04702016246669,6.44996104286335,141.295203346628));
#43977=CARTESIAN_POINT('Ctrl Pts',(-2.21138821798702,6.39779565434711,141.303347288768));
#43978=CARTESIAN_POINT('Ctrl Pts',(-2.37398861583787,6.339270871206,141.311491230908));
#43979=CARTESIAN_POINT('Ctrl Pts',(-2.53428881202539,6.2745254176904,141.319635173048));
#43980=CARTESIAN_POINT('Ctrl Pts',(-2.69442713718199,6.20984534409047,141.327770891441));
#43981=CARTESIAN_POINT('Ctrl Pts',(-2.85226954830692,6.13895724151273,141.335906609834));
#43982=CARTESIAN_POINT('Ctrl Pts',(-3.0072980347807,6.06204977957161,141.344042328227));
#43983=CARTESIAN_POINT('Ctrl Pts',(-3.16220258387119,5.98520380123137,141.352171542527));
#43984=CARTESIAN_POINT('Ctrl Pts',(-3.31429736145067,5.90234820680222,141.360300756827));
#43985=CARTESIAN_POINT('Ctrl Pts',(-3.46308375362178,5.81371997222096,141.368429971127));
#43986=CARTESIAN_POINT('Ctrl Pts',(-3.61178248283268,5.72514395621485,141.376554395803));
#43987=CARTESIAN_POINT('Ctrl Pts',(-3.75717639514937,5.63080225999025,141.384678820478));
#43988=CARTESIAN_POINT('Ctrl Pts',(-3.89879094817286,5.53097804573887,141.392803245154));
#43989=CARTESIAN_POINT('Ctrl Pts',(-4.04126519219066,5.43054783460247,141.400976990288));
#43990=CARTESIAN_POINT('Ctrl Pts',(-4.17991370426195,5.32456848964003,141.409150735422));
#43991=CARTESIAN_POINT('Ctrl Pts',(-4.3142818636197,5.21337328427978,141.417324480556));
#43992=CARTESIAN_POINT('Ctrl Pts',(-4.44778956860342,5.10289014047698,141.425445883418));
#43993=CARTESIAN_POINT('Ctrl Pts',(-4.57707131033809,4.98725799648973,141.43356728628));
#43994=CARTESIAN_POINT('Ctrl Pts',(-4.70171373100924,4.86684466483565,141.441688689142));
#43995=CARTESIAN_POINT('Ctrl Pts',(-4.82636578837591,4.74642202345693,141.449810719909));
#43996=CARTESIAN_POINT('Ctrl Pts',(-4.94637754695109,4.62121771234742,141.457932750675));
#43997=CARTESIAN_POINT('Ctrl Pts',(-5.06137215960588,4.4916367687032,141.466054781441));
#43998=CARTESIAN_POINT('Ctrl Pts',(-5.17639756066847,4.36202113133861,141.474178986782));
#43999=CARTESIAN_POINT('Ctrl Pts',(-5.28640289827642,4.22802680182094,141.482303192123));
#44000=CARTESIAN_POINT('Ctrl Pts',(-5.39105133537233,4.09009223604801,141.490427397464));
#44001=CARTESIAN_POINT('Ctrl Pts',(-5.49683251938946,3.9506646240429,141.498639541707));
#44002=CARTESIAN_POINT('Ctrl Pts',(-5.59713992333364,3.80721128192054,141.506851685949));
#44003=CARTESIAN_POINT('Ctrl Pts',(-5.69167082960152,3.66021477067442,141.515063830192));
#44004=CARTESIAN_POINT('Ctrl Pts',(-5.78533877288137,3.51456017556538,141.523201006608));
#44005=CARTESIAN_POINT('Ctrl Pts',(-5.87333511422548,3.36542717952042,141.531338183025));
#44006=CARTESIAN_POINT('Ctrl Pts',(-5.9554120167134,3.21330930835885,141.539475359441));
#44007=CARTESIAN_POINT('Ctrl Pts',(-6.03862318125308,3.05908924372479,141.547724987596));
#44008=CARTESIAN_POINT('Ctrl Pts',(-6.11574992864197,2.90180155320928,141.555974615752));
#44009=CARTESIAN_POINT('Ctrl Pts',(-6.18658494147511,2.74198026285994,141.564224243907));
#44010=CARTESIAN_POINT('Ctrl Pts',(-6.2574199543082,2.58215897251071,141.572473872063));
#44011=CARTESIAN_POINT('Ctrl Pts',(-6.32196314922586,2.41980446325587,141.580723500218));
#44012=CARTESIAN_POINT('Ctrl Pts',(-6.38006006919299,2.25546503264607,141.588973128374));
#44013=CARTESIAN_POINT('Ctrl Pts',(-6.44833391140206,2.06233802418279,141.59866785593));
#44014=CARTESIAN_POINT('Ctrl Pts',(-6.50787396952278,1.86599841217219,141.608362583487));
#44015=CARTESIAN_POINT('Ctrl Pts',(-6.55841537856759,1.66717627207447,141.618057311044));
#44016=CARTESIAN_POINT('Ctrl Pts',(-6.60874513278828,1.46918674954501,141.627711439498));
#44017=CARTESIAN_POINT('Ctrl Pts',(-6.65015138029429,1.26873551353126,141.637365567952));
#44018=CARTESIAN_POINT('Ctrl Pts',(-6.68241934800761,1.06656488662131,141.647019696406));
#44019=CARTESIAN_POINT('Ctrl Pts',(-6.71440970154839,0.866133614101466,
141.65659076655));
#44020=CARTESIAN_POINT('Ctrl Pts',(-6.73741828367758,0.664012490796059,
141.666161836694));
#44021=CARTESIAN_POINT('Ctrl Pts',(-6.7512827600329,0.46094478420152,141.675732906837));
#44022=CARTESIAN_POINT('Ctrl Pts',(-6.76163861067503,0.309266582599061,
141.682881865828));
#44023=CARTESIAN_POINT('Ctrl Pts',(-6.76689381230157,0.15706068684614,141.690030824819));
#44024=CARTESIAN_POINT('Ctrl Pts',(-6.76699840663235,0.00464377381538438,
141.69717978381));
#44025=CARTESIAN_POINT('',(-6.76796187734296,-0.00130286369752294,141.304484749508));
#44026=CARTESIAN_POINT('Ctrl Pts',(3.09917575053259,6.01559628526639,140.651392015123));
#44027=CARTESIAN_POINT('Ctrl Pts',(2.9338238445927,6.10078395293757,140.660141463035));
#44028=CARTESIAN_POINT('Ctrl Pts',(2.76495772122994,6.17915010267044,140.668890910947));
#44029=CARTESIAN_POINT('Ctrl Pts',(2.59315093316727,6.25042856433171,140.67764035886));
#44030=CARTESIAN_POINT('Ctrl Pts',(2.42134553245637,6.32170645041443,140.68638973612));
#44031=CARTESIAN_POINT('Ctrl Pts',(2.24659977927615,6.38589665313448,140.69513911338));
#44032=CARTESIAN_POINT('Ctrl Pts',(2.06950718689948,6.44278115439066,140.70388849064));
#44033=CARTESIAN_POINT('Ctrl Pts',(1.89241596572883,6.49966521519718,140.712637800154));
#44034=CARTESIAN_POINT('Ctrl Pts',(1.71297821457211,6.54924360009543,140.721387109669));
#44035=CARTESIAN_POINT('Ctrl Pts',(1.5318033733585,6.59134792173555,140.730136419184));
#44036=CARTESIAN_POINT('Ctrl Pts',(1.35062987477787,6.63345193135304,140.73888566386));
#44037=CARTESIAN_POINT('Ctrl Pts',(1.16771959102955,6.66808192368237,140.747634908536));
#44038=CARTESIAN_POINT('Ctrl Pts',(0.983693746906859,6.69512028363168,140.756384153212));
#44039=CARTESIAN_POINT('Ctrl Pts',(0.799669205419866,6.72215845218867,140.765133335956));
#44040=CARTESIAN_POINT('Ctrl Pts',(0.614529402873451,6.74160505424579,140.7738825187));
#44041=CARTESIAN_POINT('Ctrl Pts',(0.428903127363203,6.75339404354122,140.782631701445));
#44042=CARTESIAN_POINT('Ctrl Pts',(0.243278104163965,6.7651829533033,140.791380825163));
#44043=CARTESIAN_POINT('Ctrl Pts',(0.0571669005393323,6.76931433552275,
140.800129948882));
#44044=CARTESIAN_POINT('Ctrl Pts',(-0.128798404777167,6.76577415902474,
140.8088790726));
#44045=CARTESIAN_POINT('Ctrl Pts',(-0.314762517258735,6.76223400523443,
140.8176281402));
#44046=CARTESIAN_POINT('Ctrl Pts',(-0.500580446819129,6.75102239665092,
140.826377207799));
#44047=CARTESIAN_POINT('Ctrl Pts',(-0.685621118842215,6.73217741012502,
140.835126275398));
#44048=CARTESIAN_POINT('Ctrl Pts',(-0.870660665414065,6.71333253821777,
140.843875289784));
#44049=CARTESIAN_POINT('Ctrl Pts',(-1.05492267885442,6.68685441030619,140.85262430417));
#44050=CARTESIAN_POINT('Ctrl Pts',(-1.23778137635204,6.65283295028186,140.861373318555));
#44051=CARTESIAN_POINT('Ctrl Pts',(-1.42999922978786,6.61707018861878,140.870570128923));
#44052=CARTESIAN_POINT('Ctrl Pts',(-1.62066601233622,6.57297172934431,140.87976693929));
#44053=CARTESIAN_POINT('Ctrl Pts',(-1.809066285003,6.52070304311318,140.888963749658));
#44054=CARTESIAN_POINT('Ctrl Pts',(-1.98831342545444,6.47097374915056,140.897713747395));
#44055=CARTESIAN_POINT('Ctrl Pts',(-2.16550875896621,6.41384933989556,140.906463745133));
#44056=CARTESIAN_POINT('Ctrl Pts',(-2.34005036713933,6.34952386240505,140.915213742871));
#44057=CARTESIAN_POINT('Ctrl Pts',(-2.51458843547,6.28519968948631,140.923963563152));
#44058=CARTESIAN_POINT('Ctrl Pts',(-2.68647261717956,6.21367483971142,140.932713383433));
#44059=CARTESIAN_POINT('Ctrl Pts',(-2.85511905908622,6.13519226743895,140.941463203713));
#44060=CARTESIAN_POINT('Ctrl Pts',(-3.02376230488772,6.05671118252993,140.950212858172));
#44061=CARTESIAN_POINT('Ctrl Pts',(-3.18916767379789,5.97127275992695,140.958962512631));
#44062=CARTESIAN_POINT('Ctrl Pts',(-3.35077334102669,5.87916720438064,140.967712167089));
#44063=CARTESIAN_POINT('Ctrl Pts',(-3.5123761603725,5.78706327195715,140.976461667357));
#44064=CARTESIAN_POINT('Ctrl Pts',(-3.67017916302182,5.68829258362374,140.985211167626));
#44065=CARTESIAN_POINT('Ctrl Pts',(-3.82364636566345,5.58319061741122,140.993960667894));
#44066=CARTESIAN_POINT('Ctrl Pts',(-3.9771110677869,5.47809036367781,141.002710025603));
#44067=CARTESIAN_POINT('Ctrl Pts',(-4.12623987481828,5.36665920043301,141.011459383311));
#44068=CARTESIAN_POINT('Ctrl Pts',(-4.27052628213839,5.24927559512408,141.02020874102));
#44069=CARTESIAN_POINT('Ctrl Pts',(-4.41481053024887,5.13189374643114,141.028957967796));
#44070=CARTESIAN_POINT('Ctrl Pts',(-4.55425230136439,5.00855981477436,141.037707194573));
#44071=CARTESIAN_POINT('Ctrl Pts',(-4.68837800630456,4.87969268192165,141.046456421349));
#44072=CARTESIAN_POINT('Ctrl Pts',(-4.82250188228803,4.75082730631903,141.05520552882));
#44073=CARTESIAN_POINT('Ctrl Pts',(-4.95130963052875,4.61642907903623,141.063954636291));
#44074=CARTESIAN_POINT('Ctrl Pts',(-5.07436379033277,4.47695444731792,141.072703743762));
#44075=CARTESIAN_POINT('Ctrl Pts',(-5.19741643562717,4.33748153220692,141.081452743552));
#44076=CARTESIAN_POINT('Ctrl Pts',(-5.31471544462688,4.19293255254697,141.090201743341));
#44077=CARTESIAN_POINT('Ctrl Pts',(-5.42586245275545,4.04379841779714,141.098950743131));
#44078=CARTESIAN_POINT('Ctrl Pts',(-5.53702160019067,3.89464799484464,141.107700698473));
#44079=CARTESIAN_POINT('Ctrl Pts',(-5.64202723081164,3.74091164443981,141.116450653815));
#44080=CARTESIAN_POINT('Ctrl Pts',(-5.74052265232879,3.58311159163374,141.125200609157));
#44081=CARTESIAN_POINT('Ctrl Pts',(-5.8390142706684,3.42531763191916,141.13395022664));
#44082=CARTESIAN_POINT('Ctrl Pts',(-5.93099603115672,3.26346052695737,141.142699844122));
#44083=CARTESIAN_POINT('Ctrl Pts',(-6.01615550622695,3.0980900446719,141.151449461605));
#44084=CARTESIAN_POINT('Ctrl Pts',(-6.10131214578758,2.93272506863916,141.160198787756));
#44085=CARTESIAN_POINT('Ctrl Pts',(-6.17964682328721,2.76384720416956,141.168948113907));
#44086=CARTESIAN_POINT('Ctrl Pts',(-6.2508934828855,2.59203002791627,141.177697440058));
#44087=CARTESIAN_POINT('Ctrl Pts',(-6.32213814889323,2.4202176593705,141.18644652139));
#44088=CARTESIAN_POINT('Ctrl Pts',(-6.38629508412583,2.24546640831925,141.195195602721));
#44089=CARTESIAN_POINT('Ctrl Pts',(-6.44314639819814,2.06836976660036,141.203944684053));
#44090=CARTESIAN_POINT('Ctrl Pts',(-6.50000285283705,1.8912571115826,141.212694556487));
#44091=CARTESIAN_POINT('Ctrl Pts',(-6.54955227673256,1.71179891440229,141.221444428922));
#44092=CARTESIAN_POINT('Ctrl Pts',(-6.59162635926393,1.53060476278395,141.230194301356));
#44093=CARTESIAN_POINT('Ctrl Pts',(-6.63369752055202,1.34942319164669,141.238943566279));
#44094=CARTESIAN_POINT('Ctrl Pts',(-6.66829431424257,1.16650618642687,141.247692831201));
#44095=CARTESIAN_POINT('Ctrl Pts',(-6.69529923745418,0.982474997618482,
141.256442096124));
#44096=CARTESIAN_POINT('Ctrl Pts',(-6.72230554731444,0.798434359177678,
141.265191810303));
#44097=CARTESIAN_POINT('Ctrl Pts',(-6.74171916496703,0.613279706240286,
141.273941524483));
#44098=CARTESIAN_POINT('Ctrl Pts',(-6.75347414817275,0.427639953655338,
141.282691238663));
#44099=CARTESIAN_POINT('Ctrl Pts',(-6.7624883775873,0.285283364200832,141.289400897838));
#44100=CARTESIAN_POINT('Ctrl Pts',(-6.76699999999982,0.142641701109683,
141.296110557014));
#44101=CARTESIAN_POINT('Ctrl Pts',(-6.767,8.4381075191075E-12,141.30282021619));
#44102=CARTESIAN_POINT('Ctrl Pts',(-6.76699803346499,-0.00515898061969993,
141.30282021619));
#44103=CARTESIAN_POINT('Ctrl Pts',(-6.76684551847906,-0.205211798397617,
141.3121990332));
#44104=CARTESIAN_POINT('Ctrl Pts',(-6.7578179217659,-0.404900345085272,
141.32157785021));
#44105=CARTESIAN_POINT('Ctrl Pts',(-6.74003529756579,-0.603500776774318,
141.330956667221));
#44106=CARTESIAN_POINT('Ctrl Pts',(-6.72210344891169,-0.803767781442086,
141.340414187398));
#44107=CARTESIAN_POINT('Ctrl Pts',(-6.69526909379508,-1.00292819836621,
141.349871707575));
#44108=CARTESIAN_POINT('Ctrl Pts',(-6.65970477407413,-1.20025885631984,
141.359329227753));
#44109=CARTESIAN_POINT('Ctrl Pts',(-6.6239923058968,-1.39841152443993,141.368826144635));
#44110=CARTESIAN_POINT('Ctrl Pts',(-6.57947708712788,-1.59471904311785,
141.378323061518));
#44111=CARTESIAN_POINT('Ctrl Pts',(-6.52638211645565,-1.78847014792195,
141.3878199784));
#44112=CARTESIAN_POINT('Ctrl Pts',(-6.47303707337058,-1.98313380255237,
141.397361624885));
#44113=CARTESIAN_POINT('Ctrl Pts',(-6.41103134849624,-2.17521679241845,
141.40690327137));
#44114=CARTESIAN_POINT('Ctrl Pts',(-6.34063841920463,-2.36402060839288,
141.416444917855));
#44115=CARTESIAN_POINT('Ctrl Pts',(-6.32600128567985,-2.40327947561456,
141.418428957375));
#44116=CARTESIAN_POINT('Ctrl Pts',(-6.31100167596679,-2.44239664350668,
141.420412996895));
#44117=CARTESIAN_POINT('Ctrl Pts',(-6.29564229928631,-2.48136596241606,
141.422397036415));
#44118=CARTESIAN_POINT('Ctrl Pts',(-6.23250708629875,-2.64155060405269,
141.430552494822));
#44119=CARTESIAN_POINT('Ctrl Pts',(-6.16315136132801,-2.79958535426697,
141.438707953228));
#44120=CARTESIAN_POINT('Ctrl Pts',(-6.08774025173248,-2.95494629857062,
141.446863411635));
#44121=CARTESIAN_POINT('Ctrl Pts',(-6.01242092736996,-3.11011814818318,
141.455008943777));
#44122=CARTESIAN_POINT('Ctrl Pts',(-5.93106104695123,-3.2626223446625,141.463154475919));
#44123=CARTESIAN_POINT('Ctrl Pts',(-5.84387490999866,-3.41195179278491,
141.471300008061));
#44124=CARTESIAN_POINT('Ctrl Pts',(-5.75677655653961,-3.5611308883272,141.479437338861));
#44125=CARTESIAN_POINT('Ctrl Pts',(-5.6638638079716,-3.70714128589627,141.487574669662));
#44126=CARTESIAN_POINT('Ctrl Pts',(-5.56539828393895,-3.84949749202794,
141.495712000462));
#44127=CARTESIAN_POINT('Ctrl Pts',(-5.46701120723309,-3.99174028319601,
141.503842848264));
#44128=CARTESIAN_POINT('Ctrl Pts',(-5.36308037052578,-4.13033438046218,
141.511973696066));
#44129=CARTESIAN_POINT('Ctrl Pts',(-5.25391238953515,-4.26482046551658,
141.520104543868));
#44130=CARTESIAN_POINT('Ctrl Pts',(-5.14480844987737,-4.39922765685088,
141.528230621862));
#44131=CARTESIAN_POINT('Ctrl Pts',(-5.03047371408059,-4.529531352152,141.536356699856));
#44132=CARTESIAN_POINT('Ctrl Pts',(-4.91125702156631,-4.6553027257221,141.54448277785));
#44133=CARTESIAN_POINT('Ctrl Pts',(-4.79161760843506,-4.78152006161099,
141.552637669432));
#44134=CARTESIAN_POINT('Ctrl Pts',(-4.66706177056764,-4.90317257289954,
141.560792561014));
#44135=CARTESIAN_POINT('Ctrl Pts',(-4.53798203647573,-5.01986135631489,
141.568947452596));
#44136=CARTESIAN_POINT('Ctrl Pts',(-4.40940566821507,-5.13609509427424,
141.577070542953));
#44137=CARTESIAN_POINT('Ctrl Pts',(-4.2763409083398,-5.24740351417476,141.585193633309));
#44138=CARTESIAN_POINT('Ctrl Pts',(-4.13921143707729,-5.35343045898315,
141.593316723665));
#44139=CARTESIAN_POINT('Ctrl Pts',(-4.00207119778253,-5.45946572951139,
141.601440451884));
#44140=CARTESIAN_POINT('Ctrl Pts',(-3.86086590071739,-5.5602184750565,141.609564180102));
#44141=CARTESIAN_POINT('Ctrl Pts',(-3.71605079975729,-5.65537403304355,
141.61768790832));
#44142=CARTESIAN_POINT('Ctrl Pts',(-3.57119677635348,-5.75055516631124,
141.625813819981));
#44143=CARTESIAN_POINT('Ctrl Pts',(-3.42273132276988,-5.84013591572219,
141.633939731641));
#44144=CARTESIAN_POINT('Ctrl Pts',(-3.27113699773397,-5.92384602619413,
141.642065643301));
#44145=CARTESIAN_POINT('Ctrl Pts',(-3.11857321123165,-6.00809147152397,
141.650243521011));
#44146=CARTESIAN_POINT('Ctrl Pts',(-2.96284072425621,-6.08639074903449,
141.658421398721));
#44147=CARTESIAN_POINT('Ctrl Pts',(-2.80445396374326,-6.15851662052192,
141.666599276431));
#44148=CARTESIAN_POINT('Ctrl Pts',(-2.64682314888578,-6.23029825086811,
141.674738122905));
#44149=CARTESIAN_POINT('Ctrl Pts',(-2.48656370337479,-6.29596519292917,
141.682876969378));
#44150=CARTESIAN_POINT('Ctrl Pts',(-2.32419978976134,-6.35534297558152,
141.691015815852));
#44151=CARTESIAN_POINT('Ctrl Pts',(-2.16066791008213,-6.41514789277168,
141.69921320918));
#44152=CARTESIAN_POINT('Ctrl Pts',(-1.99500153066225,-6.46857271123967,
141.707410602509));
#44153=CARTESIAN_POINT('Ctrl Pts',(-1.82774818014213,-6.51549120097535,
141.715607995837));
#44154=CARTESIAN_POINT('Ctrl Pts',(-1.66049482962201,-6.56240969071102,
141.723805389165));
#44155=CARTESIAN_POINT('Ctrl Pts',(-1.49165488423451,-6.60282182449964,
141.732002782494));
#44156=CARTESIAN_POINT('Ctrl Pts',(-1.32178227966414,-6.63665432316358,
141.740200175822));
#44157=CARTESIAN_POINT('Ctrl Pts',(-1.15131252789826,-6.67060575202081,
141.748426385159));
#44158=CARTESIAN_POINT('Ctrl Pts',(-0.979295518889764,-6.69803236714227,
141.756652594496));
#44159=CARTESIAN_POINT('Ctrl Pts',(-0.806271845541212,-6.71879562950739,
141.764878803833));
#44160=CARTESIAN_POINT('Ctrl Pts',(-0.63344255687744,-6.73953556523672,
141.773095771376));
#44161=CARTESIAN_POINT('Ctrl Pts',(-0.45960920873851,-6.75362701250998,
141.781312738919));
#44162=CARTESIAN_POINT('Ctrl Pts',(-0.285323950504457,-6.7609821212061,
141.789529706462));
#44163=CARTESIAN_POINT('Ctrl Pts',(-0.11119951384423,-6.76833044298193,
141.797739091806));
#44164=CARTESIAN_POINT('Ctrl Pts',(0.0633756463752362,-6.76895479045135,
141.805948477149));
#44165=CARTESIAN_POINT('Ctrl Pts',(0.237842774754304,-6.76281892515963,
141.814157862493));
#44166=CARTESIAN_POINT('Ctrl Pts',(0.412183919450204,-6.75668749061034,
141.822361319793));
#44167=CARTESIAN_POINT('Ctrl Pts',(0.586416830726529,-6.7438055791375,141.830564777094));
#44168=CARTESIAN_POINT('Ctrl Pts',(0.759981165075346,-6.72418899412641,
141.838768234394));
#44169=CARTESIAN_POINT('Ctrl Pts',(0.933454984232804,-6.70458263932161,
141.846967413526));
#44170=CARTESIAN_POINT('Ctrl Pts',(1.10626056555226,-6.67824864806033,141.855166592658));
#44171=CARTESIAN_POINT('Ctrl Pts',(1.27784101356949,-6.64525479903064,141.86336577179));
#44172=CARTESIAN_POINT('Ctrl Pts',(1.44938913213254,-6.61226716675316,141.87156340602));
#44173=CARTESIAN_POINT('Ctrl Pts',(1.61971222421063,-6.57262223780582,141.87976104025));
#44174=CARTESIAN_POINT('Ctrl Pts',(1.78826163004924,-6.52643925448584,141.887958674479));
#44175=CARTESIAN_POINT('Ctrl Pts',(1.95679886980705,-6.4802596047042,141.896155716995));
#44176=CARTESIAN_POINT('Ctrl Pts',(2.12356233213615,-6.4275429343452,141.904352759511));
#44177=CARTESIAN_POINT('Ctrl Pts',(2.2880166661251,-6.36845889800145,141.912549802026));
#44178=CARTESIAN_POINT('Ctrl Pts',(2.45248901892003,-6.30936838798344,141.920747742669));
#44179=CARTESIAN_POINT('Ctrl Pts',(2.61465140169011,-6.24390924335047,141.928945683312));
#44180=CARTESIAN_POINT('Ctrl Pts',(2.77398660788165,-6.17230000075282,141.937143623955));
#44181=CARTESIAN_POINT('Ctrl Pts',(2.93336823100454,-6.10066989722069,141.945343952791));
#44182=CARTESIAN_POINT('Ctrl Pts',(3.08992070995639,-6.02288627402341,141.953544281627));
#44183=CARTESIAN_POINT('Ctrl Pts',(3.24314964103395,-5.93921454452198,141.961744610463));
#44184=CARTESIAN_POINT('Ctrl Pts',(3.39653824063363,-5.85545562690731,141.969953484254));
#44185=CARTESIAN_POINT('Ctrl Pts',(3.5465960581434,-5.76579651719551,141.978162358046));
#44186=CARTESIAN_POINT('Ctrl Pts',(3.69285513820632,-5.67054758627623,141.986371231837));
#44187=CARTESIAN_POINT('Ctrl Pts',(3.83919271390396,-5.57524753630653,141.99458451124));
#44188=CARTESIAN_POINT('Ctrl Pts',(3.98172719538239,-5.47435189156545,142.002797790644));
#44189=CARTESIAN_POINT('Ctrl Pts',(4.12002225636718,-5.36821251507791,142.011011070047));
#44190=CARTESIAN_POINT('Ctrl Pts',(4.25851959561478,-5.26191789307011,142.019236362663));
#44191=CARTESIAN_POINT('Ctrl Pts',(4.39276484658754,-5.15036444097716,142.027461655278));
#44192=CARTESIAN_POINT('Ctrl Pts',(4.5223562660631,-5.03394306709957,142.035686947894));
#44193=CARTESIAN_POINT('Ctrl Pts',(4.63955613788398,-4.92865391947789,142.043125737006));
#44194=CARTESIAN_POINT('Ctrl Pts',(4.75294996887623,-4.8193839025031,142.050564526118));
#44195=CARTESIAN_POINT('Ctrl Pts',(4.86226871520141,-4.70644578649044,142.05800331523));
#44196=CARTESIAN_POINT('Ctrl Pts',(4.98315908712159,-4.58155292677796,142.066229516249));
#44197=CARTESIAN_POINT('Ctrl Pts',(5.0994033158173,-4.45182470217961,142.074455717268));
#44198=CARTESIAN_POINT('Ctrl Pts',(5.21059208957854,-4.31764045237923,142.082681918286));
#44199=CARTESIAN_POINT('Ctrl Pts',(5.32165596618666,-4.18360693030277,142.090898878902));
#44200=CARTESIAN_POINT('Ctrl Pts',(5.42767546902388,-4.04512762378935,142.099115839518));
#44201=CARTESIAN_POINT('Ctrl Pts',(5.52827763207056,-3.90261904658247,142.107332800134));
#44202=CARTESIAN_POINT('Ctrl Pts',(5.62878698144326,-3.76024194512348,142.115542179935));
#44203=CARTESIAN_POINT('Ctrl Pts',(5.7238887390716,-3.61384326731823,142.123751559737));
#44204=CARTESIAN_POINT('Ctrl Pts',(5.81324974211918,-3.46387303978527,142.131960939538));
#44205=CARTESIAN_POINT('Ctrl Pts',(5.90254623208519,-3.31401108142111,142.140164392679));
#44206=CARTESIAN_POINT('Ctrl Pts',(5.9861100397044,-3.16058301597431,142.148367845819));
#44207=CARTESIAN_POINT('Ctrl Pts',(6.06365088531202,-3.00406839819848,142.15657129896));
#44208=CARTESIAN_POINT('Ctrl Pts',(6.14115130575638,-2.84763537779144,142.16477047531));
#44209=CARTESIAN_POINT('Ctrl Pts',(6.21263486082306,-2.6881193313531,142.17296965166));
#44210=CARTESIAN_POINT('Ctrl Pts',(6.27785682638096,-2.52602507261152,142.18116882801));
#44211=CARTESIAN_POINT('Ctrl Pts',(6.34306651944176,-2.36396131435091,142.189366461561));
#44212=CARTESIAN_POINT('Ctrl Pts',(6.40201683036049,-2.19932064016115,142.197564095113));
#44213=CARTESIAN_POINT('Ctrl Pts',(6.45451075406156,-2.03262882142897,142.205761728664));
#44214=CARTESIAN_POINT('Ctrl Pts',(6.50700089691177,-1.86594900859882,142.213958771785));
#44215=CARTESIAN_POINT('Ctrl Pts',(6.55303547007303,-1.69721868729407,142.222155814905));
#44216=CARTESIAN_POINT('Ctrl Pts',(6.59246705224555,-1.52697975266763,142.230352858026));
#44217=CARTESIAN_POINT('Ctrl Pts',(6.63190296100066,-1.35672213878032,142.238550800557));
#44218=CARTESIAN_POINT('Ctrl Pts',(6.66473435438957,-1.18495593128793,142.246748743088));
#44219=CARTESIAN_POINT('Ctrl Pts',(6.69086472824702,-1.01223425564438,142.254946685619));
#44220=CARTESIAN_POINT('Ctrl Pts',(6.7170027183976,-0.839462236331058,142.263147017628));
#44221=CARTESIAN_POINT('Ctrl Pts',(6.73643574490875,-0.665734548697585,
142.271347349636));
#44222=CARTESIAN_POINT('Ctrl Pts',(6.74911905885693,-0.491610546443122,
142.279547681645));
#44223=CARTESIAN_POINT('Ctrl Pts',(6.76181559224628,-0.317305059916308,
142.287756560615));
#44224=CARTESIAN_POINT('Ctrl Pts',(6.7677483320653,-0.142602791727504,142.295965439586));
#44225=CARTESIAN_POINT('Ctrl Pts',(6.76692464638334,0.0319347799383077,
142.304174318557));
#44226=CARTESIAN_POINT('Ctrl Pts',(6.7661005185278,0.206566047420996,142.312387604244));
#44227=CARTESIAN_POINT('Ctrl Pts',(6.75851275017981,0.381032084133073,142.320600889932));
#44228=CARTESIAN_POINT('Ctrl Pts',(6.74422072020736,0.554775519580439,142.328814175619));
#44229=CARTESIAN_POINT('Ctrl Pts',(6.72990778275652,0.728773120260453,142.337039476331));
#44230=CARTESIAN_POINT('Ctrl Pts',(6.70887102724182,0.902045651135109,142.345264777043));
#44231=CARTESIAN_POINT('Ctrl Pts',(6.68122138693208,1.07404365777253,142.353490077755));
#44232=CARTESIAN_POINT('Ctrl Pts',(6.65621562258789,1.22959510703063,142.360928870049));
#44233=CARTESIAN_POINT('Ctrl Pts',(6.62580187104475,1.38410407259627,142.368367662343));
#44234=CARTESIAN_POINT('Ctrl Pts',(6.59009727604772,1.53717497124708,142.375806454637));
#44235=CARTESIAN_POINT('Ctrl Pts',(6.55096306011718,1.70494916392396,142.383959783471));
#44236=CARTESIAN_POINT('Ctrl Pts',(6.50535651729762,1.87149037648807,142.392113112305));
#44237=CARTESIAN_POINT('Ctrl Pts',(6.45336732036248,2.03625617948175,142.400266441139));
#44238=CARTESIAN_POINT('Ctrl Pts',(6.40143939672394,2.20082779321088,142.408410160643));
#44239=CARTESIAN_POINT('Ctrl Pts',(6.3431439031148,2.3636278176858,142.416553880147));
#44240=CARTESIAN_POINT('Ctrl Pts',(6.27862157673203,2.52412362934049,142.424697599652));
#44241=CARTESIAN_POINT('Ctrl Pts',(6.21416172815082,2.68446403082892,142.432833433487));
#44242=CARTESIAN_POINT('Ctrl Pts',(6.14348718732535,2.84250432495502,142.440969267323));
#44243=CARTESIAN_POINT('Ctrl Pts',(6.06678858213726,2.99772668861739,142.449105101158));
#44244=CARTESIAN_POINT('Ctrl Pts',(5.98742971644171,3.15833287800792,142.457523123143));
#44245=CARTESIAN_POINT('Ctrl Pts',(5.9016214831714,3.31592176199994,142.465941145128));
#44246=CARTESIAN_POINT('Ctrl Pts',(5.80962999299254,3.46994068314164,142.474359167112));
#44247=CARTESIAN_POINT('Ctrl Pts',(5.72083909529676,3.61860093686423,142.482484307029));
#44248=CARTESIAN_POINT('Ctrl Pts',(5.62628816602592,3.7639351178533,142.490609446946));
#44249=CARTESIAN_POINT('Ctrl Pts',(5.52626372034169,3.90547030371955,142.498734586863));
#44250=CARTESIAN_POINT('Ctrl Pts',(5.42626627486101,4.0469672841371,142.506857533511));
#44251=CARTESIAN_POINT('Ctrl Pts',(5.32079846526247,4.18466701266856,142.51498048016));
#44252=CARTESIAN_POINT('Ctrl Pts',(5.21019023318417,4.31812537266257,142.523103426808));
#44253=CARTESIAN_POINT('Ctrl Pts',(5.09959081698206,4.45157309554256,142.531225726028));
#44254=CARTESIAN_POINT('Ctrl Pts',(4.98385202789909,4.58077984192608,142.539348025249));
#44255=CARTESIAN_POINT('Ctrl Pts',(4.86334417652548,4.70533446427092,142.547470324469));
#44256=CARTESIAN_POINT('Ctrl Pts',(4.7428230054427,4.82990285361373,142.555593521446));
#44257=CARTESIAN_POINT('Ctrl Pts',(4.61753197770552,4.94981783330412,142.563716718422));
#44258=CARTESIAN_POINT('Ctrl Pts',(4.48787830738047,5.06470505539502,142.571839915398));
#44259=CARTESIAN_POINT('Ctrl Pts',(4.35813809382838,5.17966896417685,142.579968534571));
#44260=CARTESIAN_POINT('Ctrl Pts',(4.22402969654757,5.28959817118007,142.588097153744));
#44261=CARTESIAN_POINT('Ctrl Pts',(4.08599388627922,5.39415822545918,142.596225772917));
#44262=CARTESIAN_POINT('Ctrl Pts',(3.94790277331778,5.49876017069816,142.604357648742));
#44263=CARTESIAN_POINT('Ctrl Pts',(3.80588141029657,5.59798846612755,142.612489524566));
#44264=CARTESIAN_POINT('Ctrl Pts',(3.66039937943157,5.6915521066803,142.620621400391));
#44265=CARTESIAN_POINT('Ctrl Pts',(3.51477710291696,5.78520594320757,142.628761115398));
#44266=CARTESIAN_POINT('Ctrl Pts',(3.36568781175504,5.8731840362202,142.636900830405));
#44267=CARTESIAN_POINT('Ctrl Pts',(3.21362597947884,5.95524114239035,142.645040545412));
#44268=CARTESIAN_POINT('Ctrl Pts',(3.17565848841867,5.97572953450231,142.647072906539));
#44269=CARTESIAN_POINT('Ctrl Pts',(3.13750578286208,5.99584903144824,142.649105267665));
#44270=CARTESIAN_POINT('Ctrl Pts',(3.09917575053256,6.0155962852664,142.651137628792));
#44271=CARTESIAN_POINT('Origin',(0.,0.,-3.69717978381041));
#44272=CARTESIAN_POINT('',(3.09917575053269,6.01559628526634,145.045580110739));
#44273=CARTESIAN_POINT('',(3.0991757505327,6.01559628526633,144.651598619988));
#44274=CARTESIAN_POINT('',(3.09917575053259,6.01559628526639,-3.69717978381041));
#44275=CARTESIAN_POINT('',(-6.76789295125885,-0.00152640326764282,143.695634344439));
#44276=CARTESIAN_POINT('Ctrl Pts',(-6.76699890218547,-0.00385458436745586,
143.69717978381));
#44277=CARTESIAN_POINT('Ctrl Pts',(-6.76688822840503,-0.198150331811941,
143.706274939033));
#44278=CARTESIAN_POINT('Ctrl Pts',(-6.75840555936475,-0.392127566114781,
143.715370094256));
#44279=CARTESIAN_POINT('Ctrl Pts',(-6.74165716558243,-0.585104829710985,
143.72446524948));
#44280=CARTESIAN_POINT('Ctrl Pts',(-6.72480840539411,-0.779238528642958,
143.73361490832));
#44281=CARTESIAN_POINT('Ctrl Pts',(-6.69959463942678,-0.972360037544215,
143.74276456716));
#44282=CARTESIAN_POINT('Ctrl Pts',(-6.66617399448702,-1.1637926255244,143.751914226001));
#44283=CARTESIAN_POINT('Ctrl Pts',(-6.63265004861101,-1.35581691858995,
143.761092165813));
#44284=CARTESIAN_POINT('Ctrl Pts',(-6.5908685217642,-1.54614165088267,143.770270105625));
#44285=CARTESIAN_POINT('Ctrl Pts',(-6.54103761856071,-1.73410376638008,
143.779448045438));
#44286=CARTESIAN_POINT('Ctrl Pts',(-6.4910067296831,-1.9228202276341,143.788662818949));
#44287=CARTESIAN_POINT('Ctrl Pts',(-6.43286183228391,-2.10915489027211,
143.79787759246));
#44288=CARTESIAN_POINT('Ctrl Pts',(-6.3668609488963,-2.29245952143529,143.807092365972));
#44289=CARTESIAN_POINT('Ctrl Pts',(-6.34417735930147,-2.35545878463785,
143.810259356015));
#44290=CARTESIAN_POINT('Ctrl Pts',(-6.32056622121258,-2.41810034992914,
143.813426346058));
#44291=CARTESIAN_POINT('Ctrl Pts',(-6.29603925657947,-2.480358578837,143.816593336102));
#44292=CARTESIAN_POINT('Ctrl Pts',(-6.23234122283766,-2.64204702357524,
143.824818203779));
#44293=CARTESIAN_POINT('Ctrl Pts',(-6.16232128426089,-2.80150714443053,
143.833043071457));
#44294=CARTESIAN_POINT('Ctrl Pts',(-6.08615524134657,-2.95820948856392,
143.841267939134));
#44295=CARTESIAN_POINT('Ctrl Pts',(-6.01007500800483,-3.11473528996703,
143.849483540578));
#44296=CARTESIAN_POINT('Ctrl Pts',(-5.92786261372773,-3.26850918163377,
143.857699142021));
#44297=CARTESIAN_POINT('Ctrl Pts',(-5.83974274512548,-3.41901940192716,
143.865914743465));
#44298=CARTESIAN_POINT('Ctrl Pts',(-5.75170444836886,-3.56939029613381,
143.874122739793));
#44299=CARTESIAN_POINT('Ctrl Pts',(-5.6577697480437,-3.71650322799807,143.882330736121));
#44300=CARTESIAN_POINT('Ctrl Pts',(-5.55821031525164,-3.85986879199673,
143.890538732449));
#44301=CARTESIAN_POINT('Ctrl Pts',(-5.458723046787,-4.00313043937784,143.89874077932));
#44302=CARTESIAN_POINT('Ctrl Pts',(-5.35361937030534,-4.14264983562056,
143.906942826192));
#44303=CARTESIAN_POINT('Ctrl Pts',(-5.24321558859412,-4.27796438642535,
143.915144873063));
#44304=CARTESIAN_POINT('Ctrl Pts',(-5.13286966152387,-4.41320802865587,
143.923342621835));
#44305=CARTESIAN_POINT('Ctrl Pts',(-5.01722938852348,-4.5442509377589,143.931540370606));
#44306=CARTESIAN_POINT('Ctrl Pts',(-4.89665292325319,-4.67066153228812,
143.939738119378));
#44307=CARTESIAN_POINT('Ctrl Pts',(-4.77609945552222,-4.79704801653503,
143.947934304593));
#44308=CARTESIAN_POINT('Ctrl Pts',(-4.65061191370683,-4.91880368243128,
143.956130489809));
#44309=CARTESIAN_POINT('Ctrl Pts',(-4.52058728115179,-5.03553171308539,
143.964326675025));
#44310=CARTESIAN_POINT('Ctrl Pts',(-4.39057226752552,-5.15225110846332,
143.972522253905));
#44311=CARTESIAN_POINT('Ctrl Pts',(-4.25602109801748,-5.26394336894143,
143.980717832785));
#44312=CARTESIAN_POINT('Ctrl Pts',(-4.11736595633787,-5.37025014143568,
143.988913411665));
#44313=CARTESIAN_POINT('Ctrl Pts',(-3.97869584539161,-5.47656839085322,
143.997109875344));
#44314=CARTESIAN_POINT('Ctrl Pts',(-3.83592116437346,-5.57749977554788,
144.005306339022));
#44315=CARTESIAN_POINT('Ctrl Pts',(-3.68950539311895,-5.6727276467451,144.013502802701));
#44316=CARTESIAN_POINT('Ctrl Pts',(-3.54304717603013,-5.76798312443859,
144.021701642528));
#44317=CARTESIAN_POINT('Ctrl Pts',(-3.39294606691518,-5.85753159959245,
144.029900482356));
#44318=CARTESIAN_POINT('Ctrl Pts',(-3.23969263340999,-5.9411009620296,144.038099322184));
#44319=CARTESIAN_POINT('Ctrl Pts',(-3.08627912233369,-6.02475761504323,
144.046306725933));
#44320=CARTESIAN_POINT('Ctrl Pts',(-2.92970702395475,-6.10242250591931,
144.054514129682));
#44321=CARTESIAN_POINT('Ctrl Pts',(-2.77049041122545,-6.17387008944211,
144.062721533431));
#44322=CARTESIAN_POINT('Ctrl Pts',(-2.61118851365254,-6.24535594407168,
144.0709333335));
#44323=CARTESIAN_POINT('Ctrl Pts',(-2.44923961032437,-6.31061771827833,
144.079145133569));
#44324=CARTESIAN_POINT('Ctrl Pts',(-2.28517555503982,-6.36947891767046,
144.087356933638));
#44325=CARTESIAN_POINT('Ctrl Pts',(-2.12086997454152,-6.42842676897266,
144.095580822624));
#44326=CARTESIAN_POINT('Ctrl Pts',(-1.95444336144118,-6.48095510677064,
144.10380471161));
#44327=CARTESIAN_POINT('Ctrl Pts',(-1.78644170893756,-6.52693764491191,
144.112028600597));
#44328=CARTESIAN_POINT('Ctrl Pts',(-1.63121108639254,-6.56942471522044,
144.119627331847));
#44329=CARTESIAN_POINT('Ctrl Pts',(-1.47463612428513,-6.60632386487549,
144.127226063098));
#44330=CARTESIAN_POINT('Ctrl Pts',(-1.31715250548996,-6.63757472856476,
144.134824794349));
#44331=CARTESIAN_POINT('Ctrl Pts',(-1.14669261750365,-6.67140058781731,
144.143049642671));
#44332=CARTESIAN_POINT('Ctrl Pts',(-0.974689627855077,-6.6987033178731,
144.151274490993));
#44333=CARTESIAN_POINT('Ctrl Pts',(-0.801683994273585,-6.7193445940304,
144.159499339316));
#44334=CARTESIAN_POINT('Ctrl Pts',(-0.62887320339435,-6.73996262353416,
144.167714924635));
#44335=CARTESIAN_POINT('Ctrl Pts',(-0.455062370104183,-6.75393409596503,
144.175930509954));
#44336=CARTESIAN_POINT('Ctrl Pts',(-0.280803496358166,-6.76117137753755,
144.184146095274));
#44337=CARTESIAN_POINT('Ctrl Pts',(-0.106705864663507,-6.76840196244033,
144.192354078697));
#44338=CARTESIAN_POINT('Ctrl Pts',(0.0678386256527802,-6.76891075117247,
144.200562062121));
#44339=CARTESIAN_POINT('Ctrl Pts',(0.242271380931179,-6.76266172287079,
144.208770045544));
#44340=CARTESIAN_POINT('Ctrl Pts',(0.416577768971264,-6.75641722165719,
144.216972082721));
#44341=CARTESIAN_POINT('Ctrl Pts',(0.590772226114278,-6.74342466747038,
144.225174119898));
#44342=CARTESIAN_POINT('Ctrl Pts',(0.764294586920538,-6.72370008138406,
144.233376157075));
#44343=CARTESIAN_POINT('Ctrl Pts',(0.937726084850511,-6.70398582383762,
144.241573899354));
#44344=CARTESIAN_POINT('Ctrl Pts',(1.11048583192282,-6.67754659747403,144.249771641634));
#44345=CARTESIAN_POINT('Ctrl Pts',(1.28201712896983,-6.6444503972133,144.257969383914));
#44346=CARTESIAN_POINT('Ctrl Pts',(1.45351581217918,-6.61136048964737,144.266165567528));
#44347=CARTESIAN_POINT('Ctrl Pts',(1.62378615750544,-6.57161619110681,144.274361751143));
#44348=CARTESIAN_POINT('Ctrl Pts',(1.79227972119302,-6.52533695689351,144.282557934757));
#44349=CARTESIAN_POINT('Ctrl Pts',(1.96076088140341,-6.47906112947756,144.290753515019));
#44350=CARTESIAN_POINT('Ctrl Pts',(2.12746517421121,-6.426251418611,144.29894909528));
#44351=CARTESIAN_POINT('Ctrl Pts',(2.29185748577107,-6.3670776864206,144.307144675541));
#44352=CARTESIAN_POINT('Ctrl Pts',(2.45626760499938,-6.307897544282,144.315341143582));
#44353=CARTESIAN_POINT('Ctrl Pts',(2.61836490632715,-6.24235212892302,144.323537611623));
#44354=CARTESIAN_POINT('Ctrl Pts',(2.77763244260628,-6.17066017649498,144.331734079664));
#44355=CARTESIAN_POINT('Ctrl Pts',(2.93694620838337,-6.09894741453446,144.339932926837));
#44356=CARTESIAN_POINT('Ctrl Pts',(3.0934282459081,-6.02108470902992,144.348131774011));
#44357=CARTESIAN_POINT('Ctrl Pts',(3.24658443415898,-5.93733766193878,144.356330621185));
#44358=CARTESIAN_POINT('Ctrl Pts',(3.39990068551969,-5.85350309103974,144.364538036951));
#44359=CARTESIAN_POINT('Ctrl Pts',(3.54988382808291,-5.76377206462456,144.372745452717));
#44360=CARTESIAN_POINT('Ctrl Pts',(3.69606620807512,-5.66845513217889,144.380952868483));
#44361=CARTESIAN_POINT('Ctrl Pts',(3.84232693668147,-5.57308711320992,144.389164683136));
#44362=CARTESIAN_POINT('Ctrl Pts',(3.98478254927311,-5.47212742718527,144.397376497788));
#44363=CARTESIAN_POINT('Ctrl Pts',(4.12299704562277,-5.36592809882745,144.40558831244));
#44364=CARTESIAN_POINT('Ctrl Pts',(4.26141508383007,-5.25957237581388,144.413812220238));
#44365=CARTESIAN_POINT('Ctrl Pts',(4.39557924810398,-5.14796181940539,144.422036128036));
#44366=CARTESIAN_POINT('Ctrl Pts',(4.52508813375834,-5.03148749195698,144.430260035834));
#44367=CARTESIAN_POINT('Ctrl Pts',(4.6447519522449,-4.92386736452163,144.437858774754));
#44368=CARTESIAN_POINT('Ctrl Pts',(4.7604416149879,-4.81209539836844,144.445457513675));
#44369=CARTESIAN_POINT('Ctrl Pts',(4.87187081025728,-4.69650548899531,144.453056252595));
#44370=CARTESIAN_POINT('Ctrl Pts',(4.99139819418358,-4.57251500838341,144.461207234769));
#44371=CARTESIAN_POINT('Ctrl Pts',(5.1063768628517,-4.44376376357494,144.469358216943));
#44372=CARTESIAN_POINT('Ctrl Pts',(5.21640031467672,-4.31062138873743,144.477509199118));
#44373=CARTESIAN_POINT('Ctrl Pts',(5.32629596406532,-4.17763367110812,144.48565071317));
#44374=CARTESIAN_POINT('Ctrl Pts',(5.43124762368969,-4.04026525580476,144.493792227223));
#44375=CARTESIAN_POINT('Ctrl Pts',(5.53088471846351,-3.89892334254815,144.501933741276));
#44376=CARTESIAN_POINT('Ctrl Pts',(5.63042704281628,-3.75771586750114,144.510067511479));
#44377=CARTESIAN_POINT('Ctrl Pts',(5.72466465678561,-3.61254271560257,144.518201281682));
#44378=CARTESIAN_POINT('Ctrl Pts',(5.81326647395409,-3.46384495940587,144.526335051884));
#44379=CARTESIAN_POINT('Ctrl Pts',(5.90180265175817,-3.31525736377375,144.534462796302));
#44380=CARTESIAN_POINT('Ctrl Pts',(5.9847111598257,-3.16315067589078,144.54259054072));
#44381=CARTESIAN_POINT('Ctrl Pts',(6.06170357407764,-3.00799580784521,144.550718285138));
#44382=CARTESIAN_POINT('Ctrl Pts',(6.13865513669684,-2.85292326387987,144.558841717031));
#44383=CARTESIAN_POINT('Ctrl Pts',(6.20969669476124,-2.69480608758663,144.566965148925));
#44384=CARTESIAN_POINT('Ctrl Pts',(6.27458523912784,-2.53414069793273,144.575088580819));
#44385=CARTESIAN_POINT('Ctrl Pts',(6.33988541090072,-2.3724561102329,144.58326354457));
#44386=CARTESIAN_POINT('Ctrl Pts',(6.39895404780624,-2.20819119318812,144.591438508321));
#44387=CARTESIAN_POINT('Ctrl Pts',(6.45159209329951,-2.04187376242393,144.599613472072));
#44388=CARTESIAN_POINT('Ctrl Pts',(6.50388646344933,-1.87664222304505,144.607735061245));
#44389=CARTESIAN_POINT('Ctrl Pts',(6.54983387689869,-1.70938525286557,144.615856650418));
#44390=CARTESIAN_POINT('Ctrl Pts',(6.58928884327989,-1.54063673194792,144.62397823959));
#44391=CARTESIAN_POINT('Ctrl Pts',(6.62874901852584,-1.37186593276461,144.63210090098));
#44392=CARTESIAN_POINT('Ctrl Pts',(6.66171495610781,-1.20160354703293,144.640223562369));
#44393=CARTESIAN_POINT('Ctrl Pts',(6.68809209491408,-1.03039464767038,144.648346223758));
#44394=CARTESIAN_POINT('Ctrl Pts',(6.71447773903112,-0.859130541982949,
144.6564715043));
#44395=CARTESIAN_POINT('Ctrl Pts',(6.73427029802455,-0.68691967644226,144.664596784842));
#44396=CARTESIAN_POINT('Ctrl Pts',(6.7474269848792,-0.514313215583638,144.672722065384));
#44397=CARTESIAN_POINT('Ctrl Pts',(6.76072701110826,-0.339826243134885,
144.680935869172));
#44398=CARTESIAN_POINT('Ctrl Pts',(6.76724569597574,-0.164935388005928,
144.68914967296));
#44399=CARTESIAN_POINT('Ctrl Pts',(6.76699291840621,0.00978990501790505,
144.697363476749));
#44400=CARTESIAN_POINT('Ctrl Pts',(6.76674243241313,0.182931211112485,144.705502817604));
#44401=CARTESIAN_POINT('Ctrl Pts',(6.75984283251556,0.355909582581761,144.713642158459));
#44402=CARTESIAN_POINT('Ctrl Pts',(6.74635595661114,0.528176397330839,144.721781499313));
#44403=CARTESIAN_POINT('Ctrl Pts',(6.7326840032492,0.702807192019788,144.730032534568));
#44404=CARTESIAN_POINT('Ctrl Pts',(6.71224271718065,0.876706369439806,144.738283569823));
#44405=CARTESIAN_POINT('Ctrl Pts',(6.68514992355707,1.04931382320304,144.746534605078));
#44406=CARTESIAN_POINT('Ctrl Pts',(6.65805712993348,1.22192127696627,144.754785640333));
#44407=CARTESIAN_POINT('Ctrl Pts',(6.62431296874273,1.39323664339194,144.763036675588));
#44408=CARTESIAN_POINT('Ctrl Pts',(6.58408725713041,1.56271686190845,144.771287710843));
#44409=CARTESIAN_POINT('Ctrl Pts',(6.54395130916204,1.73181888545011,144.779520333919));
#44410=CARTESIAN_POINT('Ctrl Pts',(6.49723756827165,1.8996219445071,144.787752956995));
#44411=CARTESIAN_POINT('Ctrl Pts',(6.44404249761946,2.0655762607259,144.795985580071));
#44412=CARTESIAN_POINT('Ctrl Pts',(6.39091198629422,2.23132916920469,144.804208211759));
#44413=CARTESIAN_POINT('Ctrl Pts',(6.33131591745078,2.39523746481411,144.812430843447));
#44414=CARTESIAN_POINT('Ctrl Pts',(6.26540171352483,2.55676169561424,144.820653475135));
#44415=CARTESIAN_POINT('Ctrl Pts',(6.19955429764811,2.71812226080607,144.828867775181));
#44416=CARTESIAN_POINT('Ctrl Pts',(6.12740163149053,2.87710324275143,144.837082075227));
#44417=CARTESIAN_POINT('Ctrl Pts',(6.04914089969554,3.03318040604753,144.845296375274));
#44418=CARTESIAN_POINT('Ctrl Pts',(5.96963345730859,3.19174391272658,144.853641530918));
#44419=CARTESIAN_POINT('Ctrl Pts',(5.88382178386252,3.34730993633217,144.861986686562));
#44420=CARTESIAN_POINT('Ctrl Pts',(5.79196410820693,3.49934862070682,144.870331842207));
#44421=CARTESIAN_POINT('Ctrl Pts',(5.70168008987063,3.64878265841722,144.87853403304));
#44422=CARTESIAN_POINT('Ctrl Pts',(5.60555574342687,3.79480891683922,144.886736223873));
#44423=CARTESIAN_POINT('Ctrl Pts',(5.50388301182707,3.9369481571544,144.894938414706));
#44424=CARTESIAN_POINT('Ctrl Pts',(5.40224546313339,4.0790382115033,144.903137767247));
#44425=CARTESIAN_POINT('Ctrl Pts',(5.29506356124918,4.2172436355249,144.911337119788));
#44426=CARTESIAN_POINT('Ctrl Pts',(5.18267264513429,4.35111402440534,144.919536472329));
#44427=CARTESIAN_POINT('Ctrl Pts',(5.07030023271001,4.48496237328161,144.927734474954));
#44428=CARTESIAN_POINT('Ctrl Pts',(4.95272074510374,4.61447683477543,144.93593247758));
#44429=CARTESIAN_POINT('Ctrl Pts',(4.83030992278301,4.73923992322229,144.944130480205));
#44430=CARTESIAN_POINT('Ctrl Pts',(4.7040745734996,4.86790103135945,144.952584616083));
#44431=CARTESIAN_POINT('Ctrl Pts',(4.57270135312063,4.99150874150268,144.96103875196));
#44432=CARTESIAN_POINT('Ctrl Pts',(4.43664349550639,5.10964612216745,144.969492887838));
#44433=CARTESIAN_POINT('Ctrl Pts',(4.30464012473797,5.22426304128517,144.977695092785));
#44434=CARTESIAN_POINT('Ctrl Pts',(4.16822762356709,5.33373077776102,144.985897297732));
#44435=CARTESIAN_POINT('Ctrl Pts',(4.02785338214885,5.43770964027246,144.994099502679));
#44436=CARTESIAN_POINT('Ctrl Pts',(3.88101174320888,5.54647907284095,145.002679604023));
#44437=CARTESIAN_POINT('Ctrl Pts',(3.72983501078796,5.64924161019091,145.011259705366));
#44438=CARTESIAN_POINT('Ctrl Pts',(3.57486866209415,5.7456594964179,145.019839806709));
#44439=CARTESIAN_POINT('Ctrl Pts',(3.41990231340035,5.84207738264489,145.028419908052));
#44440=CARTESIAN_POINT('Ctrl Pts',(3.26114675272484,5.93215042579056,145.037000009395));
#44441=CARTESIAN_POINT('Ctrl Pts',(3.09917575053269,6.01559628526634,145.045580110739));
#44442=CARTESIAN_POINT('Ctrl Pts',(3.09917575053276,6.0155962852663,143.045751582743));
#44443=CARTESIAN_POINT('Ctrl Pts',(2.93382384459276,6.10078395293754,143.054501030655));
#44444=CARTESIAN_POINT('Ctrl Pts',(2.76495772122989,6.17915010267047,143.063250478567));
#44445=CARTESIAN_POINT('Ctrl Pts',(2.5931509331671,6.25042856433178,143.07199992648));
#44446=CARTESIAN_POINT('Ctrl Pts',(2.4213455324562,6.3217064504145,143.08074930374));
#44447=CARTESIAN_POINT('Ctrl Pts',(2.24659977927598,6.38589665313455,143.089498681));
#44448=CARTESIAN_POINT('Ctrl Pts',(2.06950718689931,6.44278115439071,143.09824805826));
#44449=CARTESIAN_POINT('Ctrl Pts',(1.89241596572878,6.49966521519719,143.106997367774));
#44450=CARTESIAN_POINT('Ctrl Pts',(1.71297821457219,6.5492436000954,143.115746677289));
#44451=CARTESIAN_POINT('Ctrl Pts',(1.5318033733587,6.5913479217355,143.124495986804));
#44452=CARTESIAN_POINT('Ctrl Pts',(1.35062987477807,6.633451931353,143.13324523148));
#44453=CARTESIAN_POINT('Ctrl Pts',(1.16771959102976,6.66808192368234,143.141994476156));
#44454=CARTESIAN_POINT('Ctrl Pts',(0.983693746907072,6.69512028363165,143.150743720832));
#44455=CARTESIAN_POINT('Ctrl Pts',(0.799669205420081,6.72215845218865,143.159492903576));
#44456=CARTESIAN_POINT('Ctrl Pts',(0.614529402873668,6.74160505424577,143.16824208632));
#44457=CARTESIAN_POINT('Ctrl Pts',(0.428903127363422,6.75339404354121,143.176991269065));
#44458=CARTESIAN_POINT('Ctrl Pts',(0.243278104164058,6.7651829533033,143.185740392783));
#44459=CARTESIAN_POINT('Ctrl Pts',(0.0571669005392994,6.76931433552276,
143.194489516502));
#44460=CARTESIAN_POINT('Ctrl Pts',(-0.128798404777326,6.76577415902473,
143.20323864022));
#44461=CARTESIAN_POINT('Ctrl Pts',(-0.314762517258893,6.76223400523442,
143.21198770782));
#44462=CARTESIAN_POINT('Ctrl Pts',(-0.500580446819286,6.7510223966509,143.220736775419));
#44463=CARTESIAN_POINT('Ctrl Pts',(-0.685621118842369,6.732177410125,143.229485843018));
#44464=CARTESIAN_POINT('Ctrl Pts',(-0.870660665414345,6.71333253821774,
143.238234857404));
#44465=CARTESIAN_POINT('Ctrl Pts',(-1.05492267885482,6.68685441030613,143.24698387179));
#44466=CARTESIAN_POINT('Ctrl Pts',(-1.23778137635257,6.65283295028176,143.255732886175));
#44467=CARTESIAN_POINT('Ctrl Pts',(-1.42999922978838,6.61707018861867,143.264929696543));
#44468=CARTESIAN_POINT('Ctrl Pts',(-1.62066601233674,6.57297172934418,143.27412650691));
#44469=CARTESIAN_POINT('Ctrl Pts',(-1.80906628500351,6.52070304311304,143.283323317278));
#44470=CARTESIAN_POINT('Ctrl Pts',(-1.98831342545495,6.47097374915041,143.292073315015));
#44471=CARTESIAN_POINT('Ctrl Pts',(-2.16550875896671,6.41384933989539,143.300823312753));
#44472=CARTESIAN_POINT('Ctrl Pts',(-2.34005036713982,6.34952386240487,143.309573310491));
#44473=CARTESIAN_POINT('Ctrl Pts',(-2.5145884354706,6.28519968948607,143.318323130772));
#44474=CARTESIAN_POINT('Ctrl Pts',(-2.68647261718028,6.21367483971111,143.327072951053));
#44475=CARTESIAN_POINT('Ctrl Pts',(-2.85511905908704,6.13519226743856,143.335822771333));
#44476=CARTESIAN_POINT('Ctrl Pts',(-3.02376230488864,6.05671118252947,143.344572425792));
#44477=CARTESIAN_POINT('Ctrl Pts',(-3.18916767379891,5.97127275992641,143.353322080251));
#44478=CARTESIAN_POINT('Ctrl Pts',(-3.3507733410278,5.87916720438001,143.362071734709));
#44479=CARTESIAN_POINT('Ctrl Pts',(-3.51237616037359,5.78706327195648,143.370821234978));
#44480=CARTESIAN_POINT('Ctrl Pts',(-3.67017916302289,5.68829258362305,143.379570735246));
#44481=CARTESIAN_POINT('Ctrl Pts',(-3.82364636566451,5.5831906174105,143.388320235514));
#44482=CARTESIAN_POINT('Ctrl Pts',(-3.97711106778804,5.47809036367698,143.397069593223));
#44483=CARTESIAN_POINT('Ctrl Pts',(-4.1262398748195,5.36665920043208,143.405818950931));
#44484=CARTESIAN_POINT('Ctrl Pts',(-4.27052628213968,5.24927559512303,143.41456830864));
#44485=CARTESIAN_POINT('Ctrl Pts',(-4.41481053025033,5.1318937464299,143.423317535416));
#44486=CARTESIAN_POINT('Ctrl Pts',(-4.554252301366,5.00855981477291,143.432066762193));
#44487=CARTESIAN_POINT('Ctrl Pts',(-4.68837800630631,4.87969268191997,143.440815988969));
#44488=CARTESIAN_POINT('Ctrl Pts',(-4.82250188228982,4.75082730631721,143.44956509644));
#44489=CARTESIAN_POINT('Ctrl Pts',(-4.95130963053058,4.61642907903428,143.458314203911));
#44490=CARTESIAN_POINT('Ctrl Pts',(-5.07436379033462,4.47695444731582,143.467063311382));
#44491=CARTESIAN_POINT('Ctrl Pts',(-5.19741643562905,4.33748153220467,143.475812311172));
#44492=CARTESIAN_POINT('Ctrl Pts',(-5.31471544462877,4.19293255254458,143.484561310961));
#44493=CARTESIAN_POINT('Ctrl Pts',(-5.42586245275734,4.0437984177946,143.493310310751));
#44494=CARTESIAN_POINT('Ctrl Pts',(-5.53702160019258,3.89464799484194,143.502060266093));
#44495=CARTESIAN_POINT('Ctrl Pts',(-5.64202723081354,3.74091164443695,143.510810221435));
#44496=CARTESIAN_POINT('Ctrl Pts',(-5.74052265233067,3.58311159163072,143.519560176778));
#44497=CARTESIAN_POINT('Ctrl Pts',(-5.83901427067021,3.42531763191609,143.52830979426));
#44498=CARTESIAN_POINT('Ctrl Pts',(-5.93099603115843,3.26346052695425,143.537059411742));
#44499=CARTESIAN_POINT('Ctrl Pts',(-6.01615550622858,3.09809004466874,143.545809029225));
#44500=CARTESIAN_POINT('Ctrl Pts',(-6.101312145789,2.93272506863618,143.554558355376));
#44501=CARTESIAN_POINT('Ctrl Pts',(-6.17964682328844,2.76384720416678,143.563307681527));
#44502=CARTESIAN_POINT('Ctrl Pts',(-6.25089348288656,2.5920300279137,143.572057007678));
#44503=CARTESIAN_POINT('Ctrl Pts',(-6.32213814889422,2.4202176593679,143.58080608901));
#44504=CARTESIAN_POINT('Ctrl Pts',(-6.38629508412675,2.24546640831663,143.589555170341));
#44505=CARTESIAN_POINT('Ctrl Pts',(-6.44314639819898,2.06836976659772,143.598304251673));
#44506=CARTESIAN_POINT('Ctrl Pts',(-6.50000285283783,1.89125711157993,143.607054124107));
#44507=CARTESIAN_POINT('Ctrl Pts',(-6.54955227673327,1.71179891439961,143.615803996542));
#44508=CARTESIAN_POINT('Ctrl Pts',(-6.59162635926456,1.53060476278125,143.624553868976));
#44509=CARTESIAN_POINT('Ctrl Pts',(-6.63369752055257,1.34942319164398,143.633303133899));
#44510=CARTESIAN_POINT('Ctrl Pts',(-6.66829431424304,1.16650618642415,143.642052398821));
#44511=CARTESIAN_POINT('Ctrl Pts',(-6.69529923745459,0.98247499761575,143.650801663744));
#44512=CARTESIAN_POINT('Ctrl Pts',(-6.72230554731477,0.798434359174936,
143.659551377923));
#44513=CARTESIAN_POINT('Ctrl Pts',(-6.74171916496728,0.613279706237536,
143.668301092103));
#44514=CARTESIAN_POINT('Ctrl Pts',(-6.75347414817293,0.427639953652585,
143.677050806283));
#44515=CARTESIAN_POINT('Ctrl Pts',(-6.76248837758735,0.2852833641991,143.683760465459));
#44516=CARTESIAN_POINT('Ctrl Pts',(-6.76699999999982,0.142641701108978,
143.690470124634));
#44517=CARTESIAN_POINT('Ctrl Pts',(-6.767,8.75965874919443E-12,143.69717978381));
#44518=CARTESIAN_POINT('',(-6.76699974675837,-0.00185131634684238,143.302820216147));
#44519=CARTESIAN_POINT('Ctrl Pts',(3.09917575053256,6.0155962852664,142.651137628792));
#44520=CARTESIAN_POINT('Ctrl Pts',(2.94537248680428,6.09483420661211,142.659292690381));
#44521=CARTESIAN_POINT('Ctrl Pts',(2.7887129155403,6.16807472739275,142.66744775197));
#44522=CARTESIAN_POINT('Ctrl Pts',(2.62971668029715,6.23513265146516,142.675602813559));
#44523=CARTESIAN_POINT('Ctrl Pts',(2.51269282237715,6.28448839229172,142.681605073721));
#44524=CARTESIAN_POINT('Ctrl Pts',(2.39440352898993,6.33049591829624,142.687607333883));
#44525=CARTESIAN_POINT('Ctrl Pts',(2.27506026073269,6.37309891732703,142.693609594045));
#44526=CARTESIAN_POINT('Ctrl Pts',(2.1113620730569,6.43153567570255,142.701842644177));
#44527=CARTESIAN_POINT('Ctrl Pts',(1.94517163699043,6.48374673505441,142.710075694309));
#44528=CARTESIAN_POINT('Ctrl Pts',(1.77700268200559,6.5295138002875,142.718308744441));
#44529=CARTESIAN_POINT('Ctrl Pts',(1.6090339903958,6.57522636398105,142.726531990276));
#44530=CARTESIAN_POINT('Ctrl Pts',(1.43909181369065,6.61451012086672,142.734755236111));
#44531=CARTESIAN_POINT('Ctrl Pts',(1.26770897287109,6.64719511975556,142.742978481946));
#44532=CARTESIAN_POINT('Ctrl Pts',(1.09649592002553,6.67984773780793,142.751193581059));
#44533=CARTESIAN_POINT('Ctrl Pts',(0.923845394888543,6.7059145504386,142.759408680172));
#44534=CARTESIAN_POINT('Ctrl Pts',(0.750304561895766,6.72527561252313,142.767623779286));
#44535=CARTESIAN_POINT('Ctrl Pts',(0.576900932762358,6.74462136747566,142.775832383425));
#44536=CARTESIAN_POINT('Ctrl Pts',(0.402608752152995,6.75727189219634,142.784040987564));
#44537=CARTESIAN_POINT('Ctrl Pts',(0.227984638693499,6.76315843408387,142.792249591703));
#44538=CARTESIAN_POINT('Ctrl Pts',(0.0534636558596394,6.76904149945985,
142.800453347952));
#44539=CARTESIAN_POINT('Ctrl Pts',(-0.121388512277072,6.76816852798543,
142.808657104201));
#44540=CARTESIAN_POINT('Ctrl Pts',(-0.2960107754922,6.76052265884765,142.81686086045));
#44541=CARTESIAN_POINT('Ctrl Pts',(-0.470581372381167,6.75287905192983,
142.825062189414));
#44542=CARTESIAN_POINT('Ctrl Pts',(-0.644921842294491,6.73846655089551,
142.833263518378));
#44543=CARTESIAN_POINT('Ctrl Pts',(-0.818471491392515,6.71732040457932,
142.841464847342));
#44544=CARTESIAN_POINT('Ctrl Pts',(-0.991997206337053,6.6961771745186,142.849665045265));
#44545=CARTESIAN_POINT('Ctrl Pts',(-1.16473196205274,6.66830219121516,142.857865243188));
#44546=CARTESIAN_POINT('Ctrl Pts',(-1.33612055799236,6.63378254501233,142.866065441111));
#44547=CARTESIAN_POINT('Ctrl Pts',(-1.5075165769091,6.59926140373601,142.87426599419));
#44548=CARTESIAN_POINT('Ctrl Pts',(-1.67756596863274,6.55809509690823,142.88246654727));
#44549=CARTESIAN_POINT('Ctrl Pts',(-1.84572403230184,6.51042178330893,142.89066710035));
#44550=CARTESIAN_POINT('Ctrl Pts',(-2.01391985256634,6.462737765602,142.898869494703));
#44551=CARTESIAN_POINT('Ctrl Pts',(-2.18022315434341,6.40854392888582,142.907071889057));
#44552=CARTESIAN_POINT('Ctrl Pts',(-2.34410464082515,6.34802823188918,142.91527428341));
#44553=CARTESIAN_POINT('Ctrl Pts',(-2.50813938530545,6.28745594207779,142.923484348444));
#44554=CARTESIAN_POINT('Ctrl Pts',(-2.66974745302628,6.22055010447293,142.931694413477));
#44555=CARTESIAN_POINT('Ctrl Pts',(-2.82841890151393,6.147547113895,142.939904478511));
#44556=CARTESIAN_POINT('Ctrl Pts',(-2.98716628734198,6.07450918538086,142.948118472737));
#44557=CARTESIAN_POINT('Ctrl Pts',(-3.14297393250963,5.99536844806555,142.956332466962));
#44558=CARTESIAN_POINT('Ctrl Pts',(-3.29535681582956,5.91040713118527,142.964546461187));
#44559=CARTESIAN_POINT('Ctrl Pts',(-3.44794744777205,5.82532998373289,142.972771653822));
#44560=CARTESIAN_POINT('Ctrl Pts',(-3.59710368060713,5.7344165842604,142.980996846458));
#44561=CARTESIAN_POINT('Ctrl Pts',(-3.74236875980682,5.63799299978476,142.989222039093));
#44562=CARTESIAN_POINT('Ctrl Pts',(-3.87300533439763,5.55127947678899,142.996618937213));
#44563=CARTESIAN_POINT('Ctrl Pts',(-4.00049525190842,5.46011034373183,143.004015835333));
#44564=CARTESIAN_POINT('Ctrl Pts',(-4.12452997356337,5.36474990071087,143.011412733452));
#44565=CARTESIAN_POINT('Ctrl Pts',(-4.26950967042598,5.25328653031429,143.020058699943));
#44566=CARTESIAN_POINT('Ctrl Pts',(-4.41009750244017,5.1358434511334,143.028704666434));
#44567=CARTESIAN_POINT('Ctrl Pts',(-4.54579968236004,5.01278308406172,143.037350632925));
#44568=CARTESIAN_POINT('Ctrl Pts',(-4.68132828074351,4.8898801279292,143.04598554005));
#44569=CARTESIAN_POINT('Ctrl Pts',(-4.81198346391476,4.76137441564103,143.054620447174));
#44570=CARTESIAN_POINT('Ctrl Pts',(-4.93730352515229,4.62766927302706,143.063255354298));
#44571=CARTESIAN_POINT('Ctrl Pts',(-5.06678411127458,4.4895252275944,143.07217693337));
#44572=CARTESIAN_POINT('Ctrl Pts',(-5.19056897234715,4.34583075751169,143.081098512442));
#44573=CARTESIAN_POINT('Ctrl Pts',(-5.30818699501875,4.19707515133024,143.090020091513));
#44574=CARTESIAN_POINT('Ctrl Pts',(-5.421711262608,4.05349705965723,143.098631150489));
#44575=CARTESIAN_POINT('Ctrl Pts',(-5.52949049087475,3.90520445058976,143.107242209465));
#44576=CARTESIAN_POINT('Ctrl Pts',(-5.63113892221326,3.75267417167211,143.11585326844));
#44577=CARTESIAN_POINT('Ctrl Pts',(-5.73269149438886,3.60028773584836,143.12445620679));
#44578=CARTESIAN_POINT('Ctrl Pts',(-5.82812462812182,3.44367185071973,143.133059145139));
#44579=CARTESIAN_POINT('Ctrl Pts',(-5.91709398212594,3.28333486057834,143.141662083489));
#44580=CARTESIAN_POINT('Ctrl Pts',(-6.00596371103467,3.1231774107755,143.150255388538));
#44581=CARTESIAN_POINT('Ctrl Pts',(-6.08838395204931,2.95930743465205,143.158848693587));
#44582=CARTESIAN_POINT('Ctrl Pts',(-6.16405458437788,2.79226074728168,143.167441998635));
#44583=CARTESIAN_POINT('Ctrl Pts',(-6.17248553142073,2.77364901203428,143.168399433476));
#44584=CARTESIAN_POINT('Ctrl Pts',(-6.18083273707581,2.7549978698738,143.169356868316));
#44585=CARTESIAN_POINT('Ctrl Pts',(-6.18909582082967,2.73630808217728,143.170314303157));
#44586=CARTESIAN_POINT('Ctrl Pts',(-6.26062697767703,2.57451592624766,143.178602543211));
#44587=CARTESIAN_POINT('Ctrl Pts',(-6.32578739031436,2.40996812569131,143.186890783266));
#44588=CARTESIAN_POINT('Ctrl Pts',(-6.3843812733518,2.24320412724186,143.19517902332));
#44589=CARTESIAN_POINT('Ctrl Pts',(-6.44300346685093,2.07635955441253,143.203471267955));
#44590=CARTESIAN_POINT('Ctrl Pts',(-6.49505269240845,1.9072969767779,143.21176351259));
#44591=CARTESIAN_POINT('Ctrl Pts',(-6.54038305502368,1.73657090081549,143.220055757224));
#44592=CARTESIAN_POINT('Ctrl Pts',(-6.58576627920047,1.56564573429979,143.228357671779));
#44593=CARTESIAN_POINT('Ctrl Pts',(-6.62441490038546,1.39305353014417,143.236659586334));
#44594=CARTESIAN_POINT('Ctrl Pts',(-6.65623394311995,1.21935995278584,143.24496150089));
#44595=CARTESIAN_POINT('Ctrl Pts',(-6.68807450098562,1.0455489287735,143.253269028963));
#44596=CARTESIAN_POINT('Ctrl Pts',(-6.71307622229203,0.870635389273911,
143.261576557037));
#44597=CARTESIAN_POINT('Ctrl Pts',(-6.73119600157738,0.695190181424242,
143.26988408511));
#44598=CARTESIAN_POINT('Ctrl Pts',(-6.74934006901336,0.519509802959734,
143.278202748777));
#44599=CARTESIAN_POINT('Ctrl Pts',(-6.76058374549735,0.343296678059089,
143.286521412444));
#44600=CARTESIAN_POINT('Ctrl Pts',(-6.76493599236578,0.167122766833334,
143.294840076111));
#44601=CARTESIAN_POINT('Ctrl Pts',(-6.76632770385839,0.11078789788809,143.29750012279));
#44602=CARTESIAN_POINT('Ctrl Pts',(-6.76701515159437,0.0544570080009674,
143.300160169469));
#44603=CARTESIAN_POINT('Ctrl Pts',(-6.76699974675837,-0.00185131634684155,
143.302820216148));
#44604=CARTESIAN_POINT('Ctrl Pts',(-6.76699974675812,-0.00185131724654051,
143.30282021619));
#44605=CARTESIAN_POINT('Ctrl Pts',(-6.76694879264479,-0.18810057983288,
143.311618768413));
#44606=CARTESIAN_POINT('Ctrl Pts',(-6.7592084520437,-0.374197992708356,
143.320417320637));
#44607=CARTESIAN_POINT('Ctrl Pts',(-6.74381692552782,-0.559662643888693,
143.32921587286));
#44608=CARTESIAN_POINT('Ctrl Pts',(-6.72942699192261,-0.733058311553397,
143.337441865402));
#44609=CARTESIAN_POINT('Ctrl Pts',(-6.70832640600916,-0.906126217035766,
143.345667857943));
#44610=CARTESIAN_POINT('Ctrl Pts',(-6.68053450457218,-1.07830781005268,
143.353893850484));
#44611=CARTESIAN_POINT('Ctrl Pts',(-6.6527717393516,-1.25030889292472,143.362111219136));
#44612=CARTESIAN_POINT('Ctrl Pts',(-6.61833168465202,-1.42142516287446,
143.370328587787));
#44613=CARTESIAN_POINT('Ctrl Pts',(-6.57728557869943,-1.59110132179961,
143.378545956439));
#44614=CARTESIAN_POINT('Ctrl Pts',(-6.53627429113555,-1.76063354866794,
143.386756354501));
#44615=CARTESIAN_POINT('Ctrl Pts',(-6.48866819670722,-1.9287277512246,143.394966752564));
#44616=CARTESIAN_POINT('Ctrl Pts',(-6.43458991820602,-2.09483688733072,
143.403177150626));
#44617=CARTESIAN_POINT('Ctrl Pts',(-6.3805466951786,-2.26083834555534,143.411382226415));
#44618=CARTESIAN_POINT('Ctrl Pts',(-6.32003975573042,-2.42485696105429,
143.419587302204));
#44619=CARTESIAN_POINT('Ctrl Pts',(-6.25324209995986,-2.58635887673957,
143.427792377993));
#44620=CARTESIAN_POINT('Ctrl Pts',(-6.18647438537625,-2.74778840127588,
143.435993775962));
#44621=CARTESIAN_POINT('Ctrl Pts',(-6.11342170885582,-2.90670314306622,
143.444195173932));
#44622=CARTESIAN_POINT('Ctrl Pts',(-6.03430596010193,-3.06258723628868,
143.452396571901));
#44623=CARTESIAN_POINT('Ctrl Pts',(-5.95519640835219,-3.21845911937109,
143.460597327469));
#44624=CARTESIAN_POINT('Ctrl Pts',(-5.87002488458139,-3.37130050354307,
143.468798083037));
#44625=CARTESIAN_POINT('Ctrl Pts',(-5.77906035557741,-3.52061790124881,
143.476998838604));
#44626=CARTESIAN_POINT('Ctrl Pts',(-5.68809628862993,-3.66993454049323,
143.485199552516));
#44627=CARTESIAN_POINT('Ctrl Pts',(-5.59133946059942,-3.81572692231828,
143.493400266428));
#44628=CARTESIAN_POINT('Ctrl Pts',(-5.48910344561935,-3.95752856758985,
143.50160098034));
#44629=CARTESIAN_POINT('Ctrl Pts',(-5.386849422238,-4.09935519056552,143.50980313877));
#44630=CARTESIAN_POINT('Ctrl Pts',(-5.27911449863336,-4.23718938577961,
143.518005297199));
#44631=CARTESIAN_POINT('Ctrl Pts',(-5.16625402251077,-4.37059588327396,
143.526207455629));
#44632=CARTESIAN_POINT('Ctrl Pts',(-5.05335321319236,-4.50405005654085,
143.534412545282));
#44633=CARTESIAN_POINT('Ctrl Pts',(-4.93532343375856,-4.63307310655719,
143.542617634935));
#44634=CARTESIAN_POINT('Ctrl Pts',(-4.81255856699862,-4.75726486956614,
143.550822724588));
#44635=CARTESIAN_POINT('Ctrl Pts',(-4.68965345589309,-4.88159850698095,
143.559037187586));
#44636=CARTESIAN_POINT('Ctrl Pts',(-4.56200270287097,-5.00108957592308,
143.567251650584));
#44637=CARTESIAN_POINT('Ctrl Pts',(-4.43003590176463,-5.11537593037662,
143.575466113581));
#44638=CARTESIAN_POINT('Ctrl Pts',(-4.29799091449966,-5.22972999588296,
143.583685443389));
#44639=CARTESIAN_POINT('Ctrl Pts',(-4.16162506114506,-5.33887297648314,
143.591904773196));
#44640=CARTESIAN_POINT('Ctrl Pts',(-4.02139880848787,-5.44248478391004,
143.600124103004));
#44641=CARTESIAN_POINT('Ctrl Pts',(-3.88095528375388,-5.54625713155074,
143.608356168165));
#44642=CARTESIAN_POINT('Ctrl Pts',(-3.73663970249292,-5.64448097788017,
143.616588233325));
#44643=CARTESIAN_POINT('Ctrl Pts',(-3.58894026976262,-5.73688040140948,
143.624820298486));
#44644=CARTESIAN_POINT('Ctrl Pts',(-3.45617741423368,-5.81993563791387,
143.632219869747));
#44645=CARTESIAN_POINT('Ctrl Pts',(-3.3206810083165,-5.8982854429643,143.639619441007));
#44646=CARTESIAN_POINT('Ctrl Pts',(-3.18281997537517,-5.97176238679611,
143.647019012268));
#44647=CARTESIAN_POINT('Ctrl Pts',(-3.03087604775185,-6.05274520839092,
143.655174470675));
#44648=CARTESIAN_POINT('Ctrl Pts',(-2.87559151159903,-6.12805730365544,
143.663329929082));
#44649=CARTESIAN_POINT('Ctrl Pts',(-2.71743183989417,-6.19740697352767,
143.671485387488));
#44650=CARTESIAN_POINT('Ctrl Pts',(-2.55946466929967,-6.26667223573574,
143.67963091963));
#44651=CARTESIAN_POINT('Ctrl Pts',(-2.39862965996404,-6.32998937288949,
143.687776451772));
#44652=CARTESIAN_POINT('Ctrl Pts',(-2.23541880552875,-6.3871113786976,143.695921983914));
#44653=CARTESIAN_POINT('Ctrl Pts',(-2.0723722801886,-6.44417587112796,143.704059314714));
#44654=CARTESIAN_POINT('Ctrl Pts',(-1.90695501444588,-6.49505753028614,
143.712196645515));
#44655=CARTESIAN_POINT('Ctrl Pts',(-1.73968101121387,-6.53955648184354,
143.720333976315));
#44656=CARTESIAN_POINT('Ctrl Pts',(-1.57254027491464,-6.58401998115689,
143.728464824117));
#44657=CARTESIAN_POINT('Ctrl Pts',(-1.40354609809013,-6.62211080439482,
143.736595671919));
#44658=CARTESIAN_POINT('Ctrl Pts',(-1.23322975786386,-6.65367818310437,
143.744726519721));
#44659=CARTESIAN_POINT('Ctrl Pts',(-1.0630133305006,-6.68522704340764,143.752852597715));
#44660=CARTESIAN_POINT('Ctrl Pts',(-0.891476642852279,-6.71026001384686,
143.760978675709));
#44661=CARTESIAN_POINT('Ctrl Pts',(-0.719163335925261,-6.72867692018727,
143.769104753703));
#44662=CARTESIAN_POINT('Ctrl Pts',(-0.546239037482381,-6.74715912951398,
143.777259645285));
#44663=CARTESIAN_POINT('Ctrl Pts',(-0.37253296306589,-6.7589781802694,143.785414536867));
#44664=CARTESIAN_POINT('Ctrl Pts',(-0.198602602775026,-6.76408500879247,
143.793569428449));
#44665=CARTESIAN_POINT('Ctrl Pts',(-0.0253505100775911,-6.76917192246981,
143.801692518806));
#44666=CARTESIAN_POINT('Ctrl Pts',(0.148123753687154,-6.76759887689182,
143.809815609162));
#44667=CARTESIAN_POINT('Ctrl Pts',(0.321266709299463,-6.75936954911447,
143.817938699518));
#44668=CARTESIAN_POINT('Ctrl Pts',(0.49442326088739,-6.75113957513271,143.826062427737));
#44669=CARTESIAN_POINT('Ctrl Pts',(0.667248087080589,-6.73625229515411,
143.834186155955));
#44670=CARTESIAN_POINT('Ctrl Pts',(0.839190586537864,-6.71476344776689,
143.842309884173));
#44671=CARTESIAN_POINT('Ctrl Pts',(1.01117929956173,-6.69326882474954,143.850435795834));
#44672=CARTESIAN_POINT('Ctrl Pts',(1.18228485079778,-6.66516914665729,143.858561707494));
#44673=CARTESIAN_POINT('Ctrl Pts',(1.35196465532392,-6.63057166244019,143.866687619154));
#44674=CARTESIAN_POINT('Ctrl Pts',(1.52272957984003,-6.59575292371475,143.874865496864));
#44675=CARTESIAN_POINT('Ctrl Pts',(1.69205009072681,-6.55435305714574,143.883043374575));
#44676=CARTESIAN_POINT('Ctrl Pts',(1.85938724408571,-6.50653272308158,143.891221252285));
#44677=CARTESIAN_POINT('Ctrl Pts',(2.025925733503,-6.45894062510083,143.899360098758));
#44678=CARTESIAN_POINT('Ctrl Pts',(2.19049942769433,-6.40498938475211,143.907498945232));
#44679=CARTESIAN_POINT('Ctrl Pts',(2.35259619403884,-6.34488614143658,143.915637791705));
#44680=CARTESIAN_POINT('Ctrl Pts',(2.5158590047264,-6.28435054497517,143.923835185033));
#44681=CARTESIAN_POINT('Ctrl Pts',(2.67660876875601,-6.21757424780426,143.932032578362));
#44682=CARTESIAN_POINT('Ctrl Pts',(2.83434685429409,-6.14481626328674,143.94022997169));
#44683=CARTESIAN_POINT('Ctrl Pts',(2.99208493983216,-6.07205827876922,143.948427365019));
#44684=CARTESIAN_POINT('Ctrl Pts',(3.14681104284906,-5.99331883019363,143.956624758347));
#44685=CARTESIAN_POINT('Ctrl Pts',(3.29805599559148,-5.90890139111689,143.964822151676));
#44686=CARTESIAN_POINT('Ctrl Pts',(3.44983261439606,-5.82418720238604,143.973048361013));
#44687=CARTESIAN_POINT('Ctrl Pts',(3.59855533709777,-5.73350301216,143.98127457035));
#44688=CARTESIAN_POINT('Ctrl Pts',(3.7437228282438,-5.63709396633462,143.989500779687));
#44689=CARTESIAN_POINT('Ctrl Pts',(3.88872722993242,-5.54079323194213,143.99771774723));
#44690=CARTESIAN_POINT('Ctrl Pts',(4.03018405746355,-5.43878064568041,144.005934714773));
#44691=CARTESIAN_POINT('Ctrl Pts',(4.16761605287158,-5.33134743154553,144.014151682316));
#44692=CARTESIAN_POINT('Ctrl Pts',(4.30492123302262,-5.22401335131771,144.022361067659));
#44693=CARTESIAN_POINT('Ctrl Pts',(4.43820869666726,-5.11126882413304,144.030570453003));
#44694=CARTESIAN_POINT('Ctrl Pts',(4.5670296299557,-4.99344864388397,144.038779838346));
#44695=CARTESIAN_POINT('Ctrl Pts',(4.69575754093226,-4.87571354224188,144.046983295646));
#44696=CARTESIAN_POINT('Ctrl Pts',(4.8200250822395,-4.75291032896131,144.055186752947));
#44697=CARTESIAN_POINT('Ctrl Pts',(4.93941598264742,-4.62541444093038,144.063390210247));
#44698=CARTESIAN_POINT('Ctrl Pts',(5.05874461974385,-4.49798504302693,144.071589389379));
#44699=CARTESIAN_POINT('Ctrl Pts',(5.17320143790893,-4.36586810692125,144.079788568511));
#44700=CARTESIAN_POINT('Ctrl Pts',(5.28240649878178,-4.22947639568162,144.087987747643));
#44701=CARTESIAN_POINT('Ctrl Pts',(5.39159098306766,-4.09311038357981,144.096185381872));
#44702=CARTESIAN_POINT('Ctrl Pts',(5.49552545235458,-3.95247147651687,144.104383016102));
#44703=CARTESIAN_POINT('Ctrl Pts',(5.59386961355452,-3.80800626923742,144.112580650332));
#44704=CARTESIAN_POINT('Ctrl Pts',(5.69220667616514,-3.66355148961492,144.120777692847));
#44705=CARTESIAN_POINT('Ctrl Pts',(5.78495403173994,-3.51527125581709,144.128974735363));
#44706=CARTESIAN_POINT('Ctrl Pts',(5.87181421219092,-3.36364190387632,144.137171777878));
#44707=CARTESIAN_POINT('Ctrl Pts',(5.95868390967129,-3.21199593832746,144.145369718521));
#44708=CARTESIAN_POINT('Ctrl Pts',(6.03966496859387,-3.05700043485392,144.153567659164));
#44709=CARTESIAN_POINT('Ctrl Pts',(6.11450543412456,-2.89915716994805,144.161765599807));
#44710=CARTESIAN_POINT('Ctrl Pts',(6.18936770189748,-2.74126792273742,144.169965928643));
#44711=CARTESIAN_POINT('Ctrl Pts',(6.2580856594678,-2.5805295856471,144.178166257478));
#44712=CARTESIAN_POINT('Ctrl Pts',(6.32045511063464,-2.41746482796597,144.186366586314));
#44713=CARTESIAN_POINT('Ctrl Pts',(6.38288955238794,-2.25423015257616,144.194575460106));
#44714=CARTESIAN_POINT('Ctrl Pts',(6.43896214304632,-2.08866454888237,144.202784333897));
#44715=CARTESIAN_POINT('Ctrl Pts',(6.48851797523371,-1.9213077538669,144.210993207688));
#44716=CARTESIAN_POINT('Ctrl Pts',(6.53810040348953,-1.75386114030583,144.219206487092));
#44717=CARTESIAN_POINT('Ctrl Pts',(6.58115901258738,-1.58462176628159,144.227419766495));
#44718=CARTESIAN_POINT('Ctrl Pts',(6.61758987996973,-1.414140438755,144.235633045898));
#44719=CARTESIAN_POINT('Ctrl Pts',(6.65407403322155,-1.24340975549199,144.243858338514));
#44720=CARTESIAN_POINT('Ctrl Pts',(6.6839110103928,-1.07143384184307,144.252083631129));
#44721=CARTESIAN_POINT('Ctrl Pts',(6.70704853533991,-0.898770796474191,
144.260308923745));
#44722=CARTESIAN_POINT('Ctrl Pts',(6.72797364727505,-0.742617812969376,
144.267747712857));
#44723=CARTESIAN_POINT('Ctrl Pts',(6.74341991850449,-0.585903071393837,
144.27518650197));
#44724=CARTESIAN_POINT('Ctrl Pts',(6.75338540460217,-0.429039132138814,
144.282625291083));
#44725=CARTESIAN_POINT('Ctrl Pts',(6.76440575894322,-0.255570805859548,
144.290851492102));
#44726=CARTESIAN_POINT('Ctrl Pts',(6.76875362779252,-0.081435143226303,
144.299077693121));
#44727=CARTESIAN_POINT('Ctrl Pts',(6.76636347128686,0.0928136543552743,
144.307303894141));
#44728=CARTESIAN_POINT('Ctrl Pts',(6.76397599961829,0.266866720137652,144.315520854757));
#44729=CARTESIAN_POINT('Ctrl Pts',(6.75486557891059,0.44103231246453,144.323737815373));
#44730=CARTESIAN_POINT('Ctrl Pts',(6.73901844382689,0.614751505700547,144.331954775989));
#44731=CARTESIAN_POINT('Ctrl Pts',(6.7231859290136,0.788310428858095,144.34016415579));
#44732=CARTESIAN_POINT('Ctrl Pts',(6.70062910993685,0.961423418208949,144.348373535592));
#44733=CARTESIAN_POINT('Ctrl Pts',(6.67138625310781,1.13353185303462,144.356582915394));
#44734=CARTESIAN_POINT('Ctrl Pts',(6.64216450780107,1.30551603628391,144.364786368535));
#44735=CARTESIAN_POINT('Ctrl Pts',(6.60626639893625,1.47649675739657,144.372989821675));
#44736=CARTESIAN_POINT('Ctrl Pts',(6.56378198500671,1.64592073117187,144.381193274816));
#44737=CARTESIAN_POINT('Ctrl Pts',(6.52131971991186,1.81525637741148,144.389392451166));
#44738=CARTESIAN_POINT('Ctrl Pts',(6.47227807732916,1.98303654611663,144.397591627517));
#44739=CARTESIAN_POINT('Ctrl Pts',(6.41679817313314,2.14871827033588,144.405790803867));
#44740=CARTESIAN_POINT('Ctrl Pts',(6.36132870831835,2.31436881903838,144.413988437419));
#44741=CARTESIAN_POINT('Ctrl Pts',(6.2994235028427,2.47792136806083,144.42218607097));
#44742=CARTESIAN_POINT('Ctrl Pts',(6.23127358718948,2.63884794590266,144.430383704522));
#44743=CARTESIAN_POINT('Ctrl Pts',(6.16312858000278,2.79976293308131,144.438580747643));
#44744=CARTESIAN_POINT('Ctrl Pts',(6.08873989744063,2.9580519951231,144.446777790764));
#44745=CARTESIAN_POINT('Ctrl Pts',(6.0083467689822,3.11320704477893,144.454974833885));
#44746=CARTESIAN_POINT('Ctrl Pts',(5.92794481948514,3.26837911863463,144.463172776416));
#44747=CARTESIAN_POINT('Ctrl Pts',(5.84153727655828,3.42041617646988,144.471370718948));
#44748=CARTESIAN_POINT('Ctrl Pts',(5.74940940996816,3.56883460482125,144.479568661479));
#44749=CARTESIAN_POINT('Ctrl Pts',(5.65725469061115,3.71729629310694,144.487768993488));
#44750=CARTESIAN_POINT('Ctrl Pts',(5.55937651560925,3.86213694634304,144.495969325496));
#44751=CARTESIAN_POINT('Ctrl Pts',(5.45610358890816,4.00290177585006,144.504169657505));
#44752=CARTESIAN_POINT('Ctrl Pts',(5.35272302390506,4.14381332035504,144.512378536476));
#44753=CARTESIAN_POINT('Ctrl Pts',(5.243936686171,4.28064026447128,144.520587415447));
#44754=CARTESIAN_POINT('Ctrl Pts',(5.13011432771665,4.41296000260101,144.528796294418));
#44755=CARTESIAN_POINT('Ctrl Pts',(5.01623086678018,4.54535077303533,144.537009580106));
#44756=CARTESIAN_POINT('Ctrl Pts',(4.8973062397233,4.67322925158298,144.545222865793));
#44757=CARTESIAN_POINT('Ctrl Pts',(4.77374712394494,4.796209690644,144.553436151481));
#44758=CARTESIAN_POINT('Ctrl Pts',(4.65000725640862,4.91937003493026,144.561661452193));
#44759=CARTESIAN_POINT('Ctrl Pts',(4.52161961520314,5.03761777751236,144.569886752906));
#44760=CARTESIAN_POINT('Ctrl Pts',(4.38902498581782,5.15060663163737,144.578112053618));
#44761=CARTESIAN_POINT('Ctrl Pts',(4.26910913819172,5.25279142055012,144.585550845909));
#44762=CARTESIAN_POINT('Ctrl Pts',(4.14575295375266,5.35067537461854,144.5929896382));
#44763=CARTESIAN_POINT('Ctrl Pts',(4.01930215292755,5.44403335804181,144.600428430491));
#44764=CARTESIAN_POINT('Ctrl Pts',(3.87432988710954,5.55106564491353,144.608956795407));
#44765=CARTESIAN_POINT('Ctrl Pts',(3.72484198009896,5.65247813014822,144.617485160323));
#44766=CARTESIAN_POINT('Ctrl Pts',(3.57132008783943,5.74786585005205,144.626013525239));
#44767=CARTESIAN_POINT('Ctrl Pts',(3.4177981955799,5.84325356995589,144.634541890156));
#44768=CARTESIAN_POINT('Ctrl Pts',(3.2602426527421,5.93261620916592,144.643070255072));
#44769=CARTESIAN_POINT('Ctrl Pts',(3.0991757505327,6.01559628526633,144.651598619988));
#44770=CARTESIAN_POINT('Origin',(0.,0.,-3.69717978381041));
#44771=CARTESIAN_POINT('',(3.09917575053267,6.01559628526635,147.045751582742));
#44772=CARTESIAN_POINT('',(3.09917575053262,6.01559628526637,146.651454788324));
#44773=CARTESIAN_POINT('',(3.09917575053259,6.01559628526639,-3.69717978381041));
#44774=CARTESIAN_POINT('',(-6.767,8.90224858076955E-12,145.69717978381));
#44775=CARTESIAN_POINT('Ctrl Pts',(-6.767,8.90224859300312E-12,145.69717978381));
#44776=CARTESIAN_POINT('Ctrl Pts',(-6.76700000000025,-0.186007249406894,
145.705929295616));
#44777=CARTESIAN_POINT('Ctrl Pts',(-6.75932637295486,-0.372014355518876,
145.714678807422));
#44778=CARTESIAN_POINT('Ctrl Pts',(-6.74400518266998,-0.557389537146528,
145.723428319228));
#44779=CARTESIAN_POINT('Ctrl Pts',(-6.72868405709738,-0.742763935803023,
145.732177794078));
#44780=CARTESIAN_POINT('Ctrl Pts',(-6.70571545653105,-0.927506129686817,
145.740927268929));
#44781=CARTESIAN_POINT('Ctrl Pts',(-6.67517739415784,-1.1109886392417,145.74967674378));
#44782=CARTESIAN_POINT('Ctrl Pts',(-6.6446394582322,-1.29447038905887,145.758426182402));
#44783=CARTESIAN_POINT('Ctrl Pts',(-6.6065321702729,-1.47669218227628,145.767175621024));
#44784=CARTESIAN_POINT('Ctrl Pts',(-6.56098496116854,-1.65703510503559,
145.775925059646));
#44785=CARTESIAN_POINT('Ctrl Pts',(-6.51543793687668,-1.83737729603489,
145.784674462766));
#44786=CARTESIAN_POINT('Ctrl Pts',(-6.46245112202797,-2.01584035396551,
145.793423865886));
#44787=CARTESIAN_POINT('Ctrl Pts',(-6.40220448416404,-2.19181813637671,
145.802173269006));
#44788=CARTESIAN_POINT('Ctrl Pts',(-6.34195808575363,-2.3677952193547,145.810922637352));
#44789=CARTESIAN_POINT('Ctrl Pts',(-6.27445201489426,-2.54128677544354,
145.819672005697));
#44790=CARTESIAN_POINT('Ctrl Pts',(-6.1999155513639,-2.71170355237368,145.828421374042));
#44791=CARTESIAN_POINT('Ctrl Pts',(-6.12537937789263,-2.88211966612593,
145.837170708339));
#44792=CARTESIAN_POINT('Ctrl Pts',(-6.04381298133861,-3.0494607620996,145.845920042636));
#44793=CARTESIAN_POINT('Ctrl Pts',(-5.9554933942657,-3.21315848206365,145.854669376933));
#44794=CARTESIAN_POINT('Ctrl Pts',(-5.8671741435545,-3.37685557859132,145.863418677909));
#44795=CARTESIAN_POINT('Ctrl Pts',(-5.77210188986554,-3.53690907466794,
145.872167978884));
#44796=CARTESIAN_POINT('Ctrl Pts',(-5.67059953467412,-3.69277536784376,
145.88091727986));
#44797=CARTESIAN_POINT('Ctrl Pts',(-5.56909755762125,-3.84864108035272,
145.889666548241));
#44798=CARTESIAN_POINT('Ctrl Pts',(-5.46116568338445,-4.00031938103767,
145.898415816621));
#44799=CARTESIAN_POINT('Ctrl Pts',(-5.34717048686504,-4.14729511662716,
145.907165085002));
#44800=CARTESIAN_POINT('Ctrl Pts',(-5.23317570555923,-4.29427031687546,
145.915914321515));
#44801=CARTESIAN_POINT('Ctrl Pts',(-5.11311782179226,-4.43654275986644,
145.924663558027));
#44802=CARTESIAN_POINT('Ctrl Pts',(-4.9874045917245,-4.57362924147174,145.93341279454));
#44803=CARTESIAN_POINT('Ctrl Pts',(-4.86169180911277,-4.71071523513975,
145.942161999911));
#44804=CARTESIAN_POINT('Ctrl Pts',(-4.73032391415889,-4.84261509316077,
145.950911205282));
#44805=CARTESIAN_POINT('Ctrl Pts',(-4.5937470723776,-4.96888084331092,145.959660410653));
#44806=CARTESIAN_POINT('Ctrl Pts',(-4.45717070537871,-5.09514615452315,
145.96840958561));
#44807=CARTESIAN_POINT('Ctrl Pts',(-4.31538563819978,-5.21577720253245,
145.977158760566));
#44808=CARTESIAN_POINT('Ctrl Pts',(-4.16887341291117,-5.33036429028284,
145.985907935522));
#44809=CARTESIAN_POINT('Ctrl Pts',(-4.02236168477819,-5.44495098920821,
145.99465708079));
#44810=CARTESIAN_POINT('Ctrl Pts',(-3.87112305634932,-5.55349359238415,
146.003406226058));
#44811=CARTESIAN_POINT('Ctrl Pts',(-3.71567117317237,-5.65562346102142,
146.012155371326));
#44812=CARTESIAN_POINT('Ctrl Pts',(-3.56021980457809,-5.75775299158455,
146.020904487632));
#44813=CARTESIAN_POINT('Ctrl Pts',(-3.400555448629,-5.85346967275056,146.029653603938));
#44814=CARTESIAN_POINT('Ctrl Pts',(-3.23722036323917,-5.94244842803281,
146.038402720244));
#44815=CARTESIAN_POINT('Ctrl Pts',(-3.07388580496584,-6.03142689616201,
146.047151808315));
#44816=CARTESIAN_POINT('Ctrl Pts',(-2.90688079258268,-6.11366734484556,
146.055900896386));
#44817=CARTESIAN_POINT('Ctrl Pts',(-2.73677251095199,-6.18889046787044,
146.064649984457));
#44818=CARTESIAN_POINT('Ctrl Pts',(-2.56666476417235,-6.26411335438029,
146.073399045019));
#44819=CARTESIAN_POINT('Ctrl Pts',(-2.39345402972688,-6.33231884350066,
146.082148105582));
#44820=CARTESIAN_POINT('Ctrl Pts',(-2.21772856474637,-6.39327529620835,
146.090897166144));
#44821=CARTESIAN_POINT('Ctrl Pts',(-2.04200363768883,-6.45423156231887,
146.099646199924));
#44822=CARTESIAN_POINT('Ctrl Pts',(-1.86376426620721,-6.50793874251876,
146.108395233704));
#44823=CARTESIAN_POINT('Ctrl Pts',(-1.6836157819533,-6.55421443795958,146.117144267484));
#44824=CARTESIAN_POINT('Ctrl Pts',(-1.50346783420502,-6.60048999558536,
146.125893275208));
#44825=CARTESIAN_POINT('Ctrl Pts',(-1.32141106257872,-6.63933404145371,
146.134642282932));
#44826=CARTESIAN_POINT('Ctrl Pts',(-1.1380637595966,-6.67061465526925,146.143391290656));
#44827=CARTESIAN_POINT('Ctrl Pts',(-0.954716987425405,-6.70189517852391,
146.152140273051));
#44828=CARTESIAN_POINT('Ctrl Pts',(-0.770079973816217,-6.72561226535755,
146.160889255446));
#44829=CARTESIAN_POINT('Ctrl Pts',(-0.584779770558881,-6.74168536939726,
146.169638237841));
#44830=CARTESIAN_POINT('Ctrl Pts',(-0.391490647560342,-6.75845143942357,
146.178764418517));
#44831=CARTESIAN_POINT('Ctrl Pts',(-0.197480213110766,-6.76689975924008,
146.187890599193));
#44832=CARTESIAN_POINT('Ctrl Pts',(-0.00346532630421726,-6.76699911271707,
146.197016779869));
#44833=CARTESIAN_POINT('Ctrl Pts',(0.184486595289723,-6.76709536139791,
146.205857767399));
#44834=CARTESIAN_POINT('Ctrl Pts',(0.372442378178995,-6.75935659726805,
146.214698754929));
#44835=CARTESIAN_POINT('Ctrl Pts',(0.559750217715953,-6.74380965729067,
146.223539742459));
#44836=CARTESIAN_POINT('Ctrl Pts',(0.745129914451633,-6.72842275717321,
146.232289721057));
#44837=CARTESIAN_POINT('Ctrl Pts',(0.929874656308079,-6.70538772273558,
146.241039699655));
#44838=CARTESIAN_POINT('Ctrl Pts',(1.11335688289169,-6.67478280180844,146.249789678252));
#44839=CARTESIAN_POINT('Ctrl Pts',(1.29683723118251,-6.64417819418142,146.258539567277));
#44840=CARTESIAN_POINT('Ctrl Pts',(1.47905480729632,-6.6060039023021,146.267289456302));
#44841=CARTESIAN_POINT('Ctrl Pts',(1.65939064804209,-6.56038959797286,146.276039345327));
#44842=CARTESIAN_POINT('Ctrl Pts',(1.83972470263675,-6.51477574543423,146.284789147688));
#44843=CARTESIAN_POINT('Ctrl Pts',(2.01817678125268,-6.46172209820281,146.293538950049));
#44844=CARTESIAN_POINT('Ctrl Pts',(2.1941407234711,-6.4014088672421,146.30228875241));
#44845=CARTESIAN_POINT('Ctrl Pts',(2.37010298131527,-6.34109621361587,146.311038471016));
#44846=CARTESIAN_POINT('Ctrl Pts',(2.54357687926344,-6.27352420826201,146.319788189621));
#44847=CARTESIAN_POINT('Ctrl Pts',(2.71397317789404,-6.19892237325745,146.328537908227));
#44848=CARTESIAN_POINT('Ctrl Pts',(2.88436790206646,-6.12432122757225,146.337287545985));
#44849=CARTESIAN_POINT('Ctrl Pts',(3.05168482125713,-6.04269049717691,146.346037183743));
#44850=CARTESIAN_POINT('Ctrl Pts',(3.21535561996858,-5.95430745235216,146.354786821501));
#44851=CARTESIAN_POINT('Ctrl Pts',(3.37902496074756,-5.86592519481819,146.36353638132));
#44852=CARTESIAN_POINT('Ctrl Pts',(3.53904799384358,-5.77079087940549,146.372285941139));
#44853=CARTESIAN_POINT('Ctrl Pts',(3.69488118814475,-5.66922763747356,146.381035500958));
#44854=CARTESIAN_POINT('Ctrl Pts',(3.85071304610335,-5.56766526649396,146.389784985746));
#44855=CARTESIAN_POINT('Ctrl Pts',(4.00235489705481,-5.4596742358107,146.398534470533));
#44856=CARTESIAN_POINT('Ctrl Pts',(4.14929168607179,-5.34562133936697,146.407283955321));
#44857=CARTESIAN_POINT('Ctrl Pts',(4.29622726385282,-5.2315693830892,146.416033367984));
#44858=CARTESIAN_POINT('Ctrl Pts',(4.43845763091594,-5.11145583677613,146.424782780647));
#44859=CARTESIAN_POINT('Ctrl Pts',(4.57549970660492,-4.98568866204643,146.433532193311));
#44860=CARTESIAN_POINT('Ctrl Pts',(4.71254069814829,-4.85992248226612,146.442281536757));
#44861=CARTESIAN_POINT('Ctrl Pts',(4.84439326930854,-4.72850295734473,146.451030880203));
#44862=CARTESIAN_POINT('Ctrl Pts',(4.97060959434246,-4.59187644222171,146.45978022365));
#44863=CARTESIAN_POINT('Ctrl Pts',(5.09682496280072,-4.4552509625717,146.468529500786));
#44864=CARTESIAN_POINT('Ctrl Pts',(5.21740397615406,-4.31341878218849,146.477278777922));
#44865=CARTESIAN_POINT('Ctrl Pts',(5.33193710451512,-4.16686161439217,146.486028055058));
#44866=CARTESIAN_POINT('Ctrl Pts',(5.44646940288973,-4.02030550865069,146.494777268791));
#44867=CARTESIAN_POINT('Ctrl Pts',(5.55495572749267,-3.86902470980705,146.503526482524));
#44868=CARTESIAN_POINT('Ctrl Pts',(5.65702762491071,-3.71353301466368,146.512275696257));
#44869=CARTESIAN_POINT('Ctrl Pts',(5.75909881654779,-3.55804239467499,146.521024849493));
#44870=CARTESIAN_POINT('Ctrl Pts',(5.8547555125042,-3.39834117620177,146.52977400273));
#44871=CARTESIAN_POINT('Ctrl Pts',(5.94367283727745,-3.23497174692612,146.538523155966));
#44872=CARTESIAN_POINT('Ctrl Pts',(6.03258957675987,-3.07160339301603,146.547272251611));
#44873=CARTESIAN_POINT('Ctrl Pts',(6.11476689684985,-2.90456712830135,146.556021347257));
#44874=CARTESIAN_POINT('Ctrl Pts',(6.18992570524986,-2.73443024476528,146.564770442902));
#44875=CARTESIAN_POINT('Ctrl Pts',(6.26508404388437,-2.56429442463666,146.573519483863));
#44876=CARTESIAN_POINT('Ctrl Pts',(6.3332238428307,-2.39105828656642,146.582268524824));
#44877=CARTESIAN_POINT('Ctrl Pts',(6.39411368719803,-2.21531017132743,146.591017565785));
#44878=CARTESIAN_POINT('Ctrl Pts',(6.45500317120682,-2.03956309620174,146.599766554968));
#44879=CARTESIAN_POINT('Ctrl Pts',(6.50864269269886,-1.86130434439289,146.60851554415));
#44880=CARTESIAN_POINT('Ctrl Pts',(6.55485008446166,-1.68113930720596,146.617264533333));
#44881=CARTESIAN_POINT('Ctrl Pts',(6.60199664749259,-1.49731239212479,146.626191346862));
#44882=CARTESIAN_POINT('Ctrl Pts',(6.64140563640784,-1.31150116500296,146.635118160391));
#44883=CARTESIAN_POINT('Ctrl Pts',(6.67293772282069,-1.1243625515627,146.644044973921));
#44884=CARTESIAN_POINT('Ctrl Pts',(6.70384494949784,-0.940932395057531,
146.652794888076));
#44885=CARTESIAN_POINT('Ctrl Pts',(6.7271844934886,-0.756227260512984,146.661544802232));
#44886=CARTESIAN_POINT('Ctrl Pts',(6.74287707373878,-0.570874564548037,
146.670294716387));
#44887=CARTESIAN_POINT('Ctrl Pts',(6.75856934538633,-0.385525513638917,
146.679044458471));
#44888=CARTESIAN_POINT('Ctrl Pts',(6.76661493004084,-0.199529212424761,
146.687794200555));
#44889=CARTESIAN_POINT('Ctrl Pts',(6.76698649908905,-0.0135174386070417,
146.696543942639));
#44890=CARTESIAN_POINT('Ctrl Pts',(6.76735806132406,0.172490924439112,146.705293524285));
#44891=CARTESIAN_POINT('Ctrl Pts',(6.76005588896325,0.358514472894699,146.714043105931));
#44892=CARTESIAN_POINT('Ctrl Pts',(6.74510478454639,0.543921359655468,146.722792687577));
#44893=CARTESIAN_POINT('Ctrl Pts',(6.7301539344076,0.729325093143771,146.731542120416));
#44894=CARTESIAN_POINT('Ctrl Pts',(6.70755443556987,0.914111900249756,146.740291553255));
#44895=CARTESIAN_POINT('Ctrl Pts',(6.67738304682426,1.09765415590887,146.749040986094));
#44896=CARTESIAN_POINT('Ctrl Pts',(6.64721213111984,1.28119353390633,146.757790281755));
#44897=CARTESIAN_POINT('Ctrl Pts',(6.60946960955634,1.46348811672024,146.766539577417));
#44898=CARTESIAN_POINT('Ctrl Pts',(6.56428366991337,1.64391876347605,146.775288873078));
#44899=CARTESIAN_POINT('Ctrl Pts',(6.5190983786789,1.824346821091,146.784038043189));
#44900=CARTESIAN_POINT('Ctrl Pts',(6.46646995272111,2.00291071819832,146.7927872133));
#44901=CARTESIAN_POINT('Ctrl Pts',(6.40657713281757,2.17900400212094,146.80153638341));
#44902=CARTESIAN_POINT('Ctrl Pts',(6.34668509279284,2.35509499309053,146.810285439596));
#44903=CARTESIAN_POINT('Ctrl Pts',(6.27952894037767,2.52871516397523,146.819034495782));
#44904=CARTESIAN_POINT('Ctrl Pts',(6.20533675061705,2.69927486770826,146.827783551968));
#44905=CARTESIAN_POINT('Ctrl Pts',(6.12832117908181,2.87632521635362,146.83686555325));
#44906=CARTESIAN_POINT('Ctrl Pts',(6.04372366626347,3.05007728919468,146.845947554532));
#44907=CARTESIAN_POINT('Ctrl Pts',(5.95185378008137,3.21989527477697,146.855029555815));
#44908=CARTESIAN_POINT('Ctrl Pts',(5.86334450817657,3.38350129286257,146.863779336122));
#44909=CARTESIAN_POINT('Ctrl Pts',(5.76808562057557,3.54345567124471,146.872529116429));
#44910=CARTESIAN_POINT('Ctrl Pts',(5.66640068804801,3.69921508464823,146.881278896736));
#44911=CARTESIAN_POINT('Ctrl Pts',(5.56471941108251,3.8549688985181,146.890028362489));
#44912=CARTESIAN_POINT('Ctrl Pts',(5.45661270815451,4.00652780919178,146.898777828243));
#44913=CARTESIAN_POINT('Ctrl Pts',(5.3424477644946,4.15337704568785,146.907527293996));
#44914=CARTESIAN_POINT('Ctrl Pts',(5.22828631819954,4.30022178355814,146.916276491716));
#44915=CARTESIAN_POINT('Ctrl Pts',(5.1080671784444,4.44235690972252,146.925025689436));
#44916=CARTESIAN_POINT('Ctrl Pts',(4.98219864545103,4.57929969070227,146.933774887155));
#44917=CARTESIAN_POINT('Ctrl Pts',(4.85633329944421,4.71623900429592,146.942523863345));
#44918=CARTESIAN_POINT('Ctrl Pts',(4.72481904034057,4.84798602483218,146.951272839536));
#44919=CARTESIAN_POINT('Ctrl Pts',(4.58810250737619,4.97409332258737,146.960021815726));
#44920=CARTESIAN_POINT('Ctrl Pts',(4.45137708686068,5.10020881821763,146.968771360662));
#44921=CARTESIAN_POINT('Ctrl Pts',(4.30944892636482,5.22068366307578,146.977520905598));
#44922=CARTESIAN_POINT('Ctrl Pts',(4.16280009467095,5.33510865604512,146.986270450534));
#44923=CARTESIAN_POINT('Ctrl Pts',(4.01615988349229,5.44952692272567,146.995019481143));
#44924=CARTESIAN_POINT('Ctrl Pts',(3.86479978232677,5.55789587288316,147.003768511751));
#44925=CARTESIAN_POINT('Ctrl Pts',(3.70923383581518,5.65984746713583,147.012517542359));
#44926=CARTESIAN_POINT('Ctrl Pts',(3.55366577800002,5.76180044505098,147.021266691707));
#44927=CARTESIAN_POINT('Ctrl Pts',(3.39389200027312,5.85733573570785,147.030015841055));
#44928=CARTESIAN_POINT('Ctrl Pts',(3.23045513626524,5.94612887621666,147.038764990403));
#44929=CARTESIAN_POINT('Ctrl Pts',(3.18695122151905,5.96976399206515,147.041093854516));
#44930=CARTESIAN_POINT('Ctrl Pts',(3.14318791262833,5.99292165435246,147.043422718629));
#44931=CARTESIAN_POINT('Ctrl Pts',(3.09917575053267,6.01559628526635,147.045751582743));
#44932=CARTESIAN_POINT('Ctrl Pts',(3.09917575053269,6.01559628526634,145.045580110739));
#44933=CARTESIAN_POINT('Ctrl Pts',(2.9439233683427,6.09558077812104,145.05380430615));
#44934=CARTESIAN_POINT('Ctrl Pts',(2.78571726968034,6.16947671695349,145.062028501561));
#44935=CARTESIAN_POINT('Ctrl Pts',(2.62508186159937,6.23708539462961,145.070252696972));
#44936=CARTESIAN_POINT('Ctrl Pts',(2.49964395324186,6.28988005065112,145.076674854344));
#44937=CARTESIAN_POINT('Ctrl Pts',(2.37272511858934,6.33884180682753,145.083097011717));
#44938=CARTESIAN_POINT('Ctrl Pts',(2.24458091329037,6.38389736161951,145.089519169089));
#44939=CARTESIAN_POINT('Ctrl Pts',(2.0720689977826,6.44455262139732,145.098164887149));
#44940=CARTESIAN_POINT('Ctrl Pts',(1.89694273773663,6.4982653745132,145.106810605209));
#44941=CARTESIAN_POINT('Ctrl Pts',(1.71977518678143,6.54481950147832,145.115456323269));
#44942=CARTESIAN_POINT('Ctrl Pts',(1.54283508285712,6.59131386243156,145.124090941989));
#44943=CARTESIAN_POINT('Ctrl Pts',(1.36385920719454,6.63066784586529,145.132725560709));
#44944=CARTESIAN_POINT('Ctrl Pts',(1.18343739809782,6.66271453123901,145.141360179429));
#44945=CARTESIAN_POINT('Ctrl Pts',(0.996643791826336,6.69589298100611,145.150299739327));
#44946=CARTESIAN_POINT('Ctrl Pts',(0.808300551939153,6.72123844830351,145.159239299226));
#44947=CARTESIAN_POINT('Ctrl Pts',(0.619078821817926,6.73862229334577,145.168178859125));
#44948=CARTESIAN_POINT('Ctrl Pts',(0.436818986978534,6.75536654742401,145.176789512402));
#44949=CARTESIAN_POINT('Ctrl Pts',(0.253744494266675,6.76472450344558,145.18540016568));
#44950=CARTESIAN_POINT('Ctrl Pts',(0.0704653816734188,6.76663310886482,
145.194010818958));
#44951=CARTESIAN_POINT('Ctrl Pts',(-0.112640244974695,6.76853990766132,
145.202613321676));
#44952=CARTESIAN_POINT('Ctrl Pts',(-0.295949801375999,6.76301141110478,
145.211215824394));
#44953=CARTESIAN_POINT('Ctrl Pts',(-0.478849452261388,6.75003645931405,
145.219818327112));
#44954=CARTESIAN_POINT('Ctrl Pts',(-0.661543253267038,6.73707611057069,
145.228411147886));
#44955=CARTESIAN_POINT('Ctrl Pts',(-0.84382776553683,6.71668604764664,145.237003968661));
#44956=CARTESIAN_POINT('Ctrl Pts',(-1.02509026510326,6.68890715650849,145.245596789435));
#44957=CARTESIAN_POINT('Ctrl Pts',(-1.04645287332205,6.68563328811566,145.246609492361));
#44958=CARTESIAN_POINT('Ctrl Pts',(-1.06780128811058,6.68225685065292,145.247622195287));
#44959=CARTESIAN_POINT('Ctrl Pts',(-1.08913450867068,6.67877795873038,145.248634898213));
#44960=CARTESIAN_POINT('Ctrl Pts',(-1.27019898926127,6.64925106394149,145.25723015596));
#44961=CARTESIAN_POINT('Ctrl Pts',(-1.44995535059435,6.61237420054901,145.265825413708));
#44962=CARTESIAN_POINT('Ctrl Pts',(-1.62780734683736,6.56829751469757,145.274420671455));
#44963=CARTESIAN_POINT('Ctrl Pts',(-1.80582589392731,6.52417955290033,145.283023978297));
#44964=CARTESIAN_POINT('Ctrl Pts',(-1.98193621989576,6.47284838414931,145.291627285139));
#44965=CARTESIAN_POINT('Ctrl Pts',(-2.15555740029556,6.41450397879922,145.30023059198));
#44966=CARTESIAN_POINT('Ctrl Pts',(-2.33637697543853,6.35374059403776,145.309190594927));
#44967=CARTESIAN_POINT('Ctrl Pts',(-2.51449624819373,6.28537017245824,145.318150597873));
#44968=CARTESIAN_POINT('Ctrl Pts',(-2.6892834913913,6.20967336523671,145.327110600819));
#44969=CARTESIAN_POINT('Ctrl Pts',(-2.85757162120232,6.13679119210479,145.335737444011));
#44970=CARTESIAN_POINT('Ctrl Pts',(-3.02277079659474,6.05711781313992,145.344364287202));
#44971=CARTESIAN_POINT('Ctrl Pts',(-3.18434321852858,5.97095028170651,145.352991130394));
#44972=CARTESIAN_POINT('Ctrl Pts',(-3.34607006285292,5.88470039589586,145.361626218667));
#44973=CARTESIAN_POINT('Ctrl Pts',(-3.50416297030758,5.79194411997024,145.370261306939));
#44974=CARTESIAN_POINT('Ctrl Pts',(-3.65811206393917,5.69302249491979,145.378896395212));
#44975=CARTESIAN_POINT('Ctrl Pts',(-3.81228980286979,5.59395395140424,145.387544308324));
#44976=CARTESIAN_POINT('Ctrl Pts',(-3.96231117723578,5.48870193191362,145.396192221436));
#44977=CARTESIAN_POINT('Ctrl Pts',(-4.10769718875882,5.37764937546721,145.404840134547));
#44978=CARTESIAN_POINT('Ctrl Pts',(-4.12400728703292,5.3651909684289,145.40581029881));
#44979=CARTESIAN_POINT('Ctrl Pts',(-4.14025908368601,5.35265959902519,145.406780463073));
#44980=CARTESIAN_POINT('Ctrl Pts',(-4.15645193036076,5.34005583777925,145.407750627336));
#44981=CARTESIAN_POINT('Ctrl Pts',(-4.29185953005773,5.23466083887976,145.41586332159));
#44982=CARTESIAN_POINT('Ctrl Pts',(-4.42346060361134,5.12395270312488,145.423976015843));
#44983=CARTESIAN_POINT('Ctrl Pts',(-4.55080472908244,5.00823974244054,145.432088710096));
#44984=CARTESIAN_POINT('Ctrl Pts',(-4.67801292831267,4.89265029297204,145.440192744916));
#44985=CARTESIAN_POINT('Ctrl Pts',(-4.80097295277972,4.77206689778212,145.448296779735));
#44986=CARTESIAN_POINT('Ctrl Pts',(-4.91926491135886,4.64683997269903,145.456400814555));
#44987=CARTESIAN_POINT('Ctrl Pts',(-5.03745599628963,4.52171983506759,145.464497938646));
#44988=CARTESIAN_POINT('Ctrl Pts',(-5.15098668773628,4.39196431732556,145.472595062737));
#44989=CARTESIAN_POINT('Ctrl Pts',(-5.25947168751103,4.25796272509165,145.480692186829));
#44990=CARTESIAN_POINT('Ctrl Pts',(-5.36788744554687,4.12404666084116,145.488784142842));
#44991=CARTESIAN_POINT('Ctrl Pts',(-5.47126369259091,3.98589020426211,145.496876098855));
#44992=CARTESIAN_POINT('Ctrl Pts',(-5.56925343928991,3.84391793993544,145.504968054869));
#44993=CARTESIAN_POINT('Ctrl Pts',(-5.66721119758169,3.70199202195374,145.513057369291));
#44994=CARTESIAN_POINT('Ctrl Pts',(-5.75978574337875,3.55625307726772,145.521146683714));
#44995=CARTESIAN_POINT('Ctrl Pts',(-5.84667163970565,3.40715713424868,145.529235998137));
#44996=CARTESIAN_POINT('Ctrl Pts',(-5.93354430905497,3.25808388868432,145.537324081092));
#44997=CARTESIAN_POINT('Ctrl Pts',(-6.01472986596867,3.10565498064337,145.545412164047));
#44998=CARTESIAN_POINT('Ctrl Pts',(-6.08996739788074,2.95035355385582,145.553500247002));
#44999=CARTESIAN_POINT('Ctrl Pts',(-6.16520808407557,2.79504561616076,145.561588669045));
#45000=CARTESIAN_POINT('Ctrl Pts',(-6.2345000875311,2.63686525240069,145.569677091087));
#45001=CARTESIAN_POINT('Ctrl Pts',(-6.29762951322042,2.47631813671328,145.577765513129));
#45002=CARTESIAN_POINT('Ctrl Pts',(-6.36077384375081,2.3157331158934,145.585855844846));
#45003=CARTESIAN_POINT('Ctrl Pts',(-6.41775256505008,2.15278057455462,145.593946176563));
#45004=CARTESIAN_POINT('Ctrl Pts',(-6.46840080796771,1.9879839002071,145.60203650828));
#45005=CARTESIAN_POINT('Ctrl Pts',(-6.51909944905326,1.82302324286654,145.610134890383));
#45006=CARTESIAN_POINT('Ctrl Pts',(-6.5634549203035,1.65621514058114,145.618233272485));
#45007=CARTESIAN_POINT('Ctrl Pts',(-6.60135270114207,1.48809660812874,145.626331654588));
#45008=CARTESIAN_POINT('Ctrl Pts',(-6.63926980182875,1.31989237080289,145.634434165152));
#45009=CARTESIAN_POINT('Ctrl Pts',(-6.67072258577455,1.15037673503887,145.642536675715));
#45010=CARTESIAN_POINT('Ctrl Pts',(-6.69564817523386,0.980094135013302,
145.650639186279));
#45011=CARTESIAN_POINT('Ctrl Pts',(-6.72061010657903,0.809563260385306,
145.658753510425));
#45012=CARTESIAN_POINT('Ctrl Pts',(-6.73902578995366,0.63826355426418,145.666867834572));
#45013=CARTESIAN_POINT('Ctrl Pts',(-6.75088439156448,0.466742896819157,
145.674982158718));
#45014=CARTESIAN_POINT('Ctrl Pts',(-6.76163788249994,0.311206359239643,
145.682340303803));
#45015=CARTESIAN_POINT('Ctrl Pts',(-6.76700013085047,0.155488341605922,
145.689698448888));
#45016=CARTESIAN_POINT('Ctrl Pts',(-6.76699999999761,-5.6946322475613E-6,
145.697056593973));
#45017=CARTESIAN_POINT('',(-6.76699866775558,0.00424624472223871,145.302820216218));
#45018=CARTESIAN_POINT('Ctrl Pts',(3.0991757505327,6.01559628526633,144.651598619988));
#45019=CARTESIAN_POINT('Ctrl Pts',(2.94554257394182,6.09474657939993,144.65973337502));
#45020=CARTESIAN_POINT('Ctrl Pts',(2.78871523524756,6.16808998521787,144.667868130051));
#45021=CARTESIAN_POINT('Ctrl Pts',(2.62917701709088,6.23536023119764,144.676002885083));
#45022=CARTESIAN_POINT('Ctrl Pts',(2.46975342994266,6.30258214232559,144.684131795151));
#45023=CARTESIAN_POINT('Ctrl Pts',(2.30762317732625,6.36373944112315,144.692260705218));
#45024=CARTESIAN_POINT('Ctrl Pts',(2.14329310126062,6.41861228631927,144.700389615286));
#45025=CARTESIAN_POINT('Ctrl Pts',(1.97904658299517,6.4734572300238,144.708514392003));
#45026=CARTESIAN_POINT('Ctrl Pts',(1.81260281499707,6.52202396866606,144.716639168719));
#45027=CARTESIAN_POINT('Ctrl Pts',(1.64448752408125,6.56414120682524,144.724763945436));
#45028=CARTESIAN_POINT('Ctrl Pts',(1.47639578656538,6.6062525442472,144.73288758385));
#45029=CARTESIAN_POINT('Ctrl Pts',(1.30663334483601,6.6419160836238,144.741011222264));
#45030=CARTESIAN_POINT('Ctrl Pts',(1.13574020417337,6.67101065721111,144.749134860678));
#45031=CARTESIAN_POINT('Ctrl Pts',(0.964853908587294,6.70010406542349,144.757258173702));
#45032=CARTESIAN_POINT('Ctrl Pts',(0.792837364671338,6.72262896917097,144.765381486726));
#45033=CARTESIAN_POINT('Ctrl Pts',(0.620239680184277,6.73851554417773,144.77350479975));
#45034=CARTESIAN_POINT('Ctrl Pts',(0.447616073412362,6.75440450517434,144.781629332806));
#45035=CARTESIAN_POINT('Ctrl Pts',(0.274411516545912,6.76365311816404,144.789753865863));
#45036=CARTESIAN_POINT('Ctrl Pts',(0.101179091980249,6.76624355099239,144.79787839892));
#45037=CARTESIAN_POINT('Ctrl Pts',(-0.0721123087947992,6.76883486572208,
144.806005697938));
#45038=CARTESIAN_POINT('Ctrl Pts',(-0.24543123060132,6.76476348102892,144.814132996955));
#45039=CARTESIAN_POINT('Ctrl Pts',(-0.418225783397205,6.75406368004491,
144.822260295973));
#45040=CARTESIAN_POINT('Ctrl Pts',(-0.591219031196919,6.74335157544968,
144.830396940504));
#45041=CARTESIAN_POINT('Ctrl Pts',(-0.7636863400305,6.72599585161625,144.838533585035));
#45042=CARTESIAN_POINT('Ctrl Pts',(-0.935081153500462,6.70208267901615,
144.846670229565));
#45043=CARTESIAN_POINT('Ctrl Pts',(-1.10657756852881,6.6781553308669,144.854811697438));
#45044=CARTESIAN_POINT('Ctrl Pts',(-1.27699986206859,6.64766285280158,144.86295316531));
#45045=CARTESIAN_POINT('Ctrl Pts',(-1.44581314006289,6.61074227027657,144.871094633183));
#45046=CARTESIAN_POINT('Ctrl Pts',(-1.61489533330733,6.57376287420443,144.879249070206));
#45047=CARTESIAN_POINT('Ctrl Pts',(-1.78236303600487,6.53033500518731,144.887403507229));
#45048=CARTESIAN_POINT('Ctrl Pts',(-1.94769672303461,6.4806455291954,144.895557944253));
#45049=CARTESIAN_POINT('Ctrl Pts',(-2.10093493824198,6.43459123286666,144.903115819468));
#45050=CARTESIAN_POINT('Ctrl Pts',(-2.25233994001898,6.38315859856928,144.910673694684));
#45051=CARTESIAN_POINT('Ctrl Pts',(-2.40151557817402,6.32653237783444,144.918231569899));
#45052=CARTESIAN_POINT('Ctrl Pts',(-2.56401766669649,6.26484751260877,144.92646462003));
#45053=CARTESIAN_POINT('Ctrl Pts',(-2.72437915358357,6.19680745619827,144.934697670162));
#45054=CARTESIAN_POINT('Ctrl Pts',(-2.88206742583381,6.12257922390129,144.942930720293));
#45055=CARTESIAN_POINT('Ctrl Pts',(-3.03956791559096,6.04843938601893,144.951153966127));
#45056=CARTESIAN_POINT('Ctrl Pts',(-3.19440120872991,5.96812619713585,144.959377211961));
#45057=CARTESIAN_POINT('Ctrl Pts',(-3.34605151341352,5.88185585249954,144.967600457795));
#45058=CARTESIAN_POINT('Ctrl Pts',(-3.49755157903101,5.79567097538695,144.975815556908));
#45059=CARTESIAN_POINT('Ctrl Pts',(-3.64587462697365,5.703540871759,144.984030656021));
#45060=CARTESIAN_POINT('Ctrl Pts',(-3.79052637866044,5.60572910268409,144.992245755134));
#45061=CARTESIAN_POINT('Ctrl Pts',(-3.93506376660752,5.50799466499003,145.000454359272));
#45062=CARTESIAN_POINT('Ctrl Pts',(-4.07593534427567,5.40458770875781,145.00866296341));
#45063=CARTESIAN_POINT('Ctrl Pts',(-4.21267283740553,5.29581689307567,145.016871567548));
#45064=CARTESIAN_POINT('Ctrl Pts',(-4.34932957523257,5.1871103159572,145.025075323796));
#45065=CARTESIAN_POINT('Ctrl Pts',(-4.48185681282941,5.07304641250351,145.033279080045));
#45066=CARTESIAN_POINT('Ctrl Pts',(-4.60981652639567,4.95397624065451,145.041482836293));
#45067=CARTESIAN_POINT('Ctrl Pts',(-4.73773837990794,4.83494129866817,145.049684165256));
#45068=CARTESIAN_POINT('Ctrl Pts',(-4.86109513684568,4.71090327970509,145.05788549422));
#45069=CARTESIAN_POINT('Ctrl Pts',(-4.9794828705545,4.58225264928226,145.066086823184));
#45070=CARTESIAN_POINT('Ctrl Pts',(-5.09785427746469,4.4536197610095,145.074287021106));
#45071=CARTESIAN_POINT('Ctrl Pts',(-5.2112577828604,4.32037579122047,145.082487219028));
#45072=CARTESIAN_POINT('Ctrl Pts',(-5.31932726298064,4.18294710333647,145.09068741695));
#45073=CARTESIAN_POINT('Ctrl Pts',(-5.4274014236763,4.04551246330632,145.098887970029));
#45074=CARTESIAN_POINT('Ctrl Pts',(-5.53014087731727,3.90389302571494,145.107088523108));
#45075=CARTESIAN_POINT('Ctrl Pts',(-5.62722061241426,3.75854721657452,145.115289076187));
#45076=CARTESIAN_POINT('Ctrl Pts',(-5.72432214486191,3.61316877288308,145.123491470539));
#45077=CARTESIAN_POINT('Ctrl Pts',(-5.81576122877437,3.46406258908148,145.131693864892));
#45078=CARTESIAN_POINT('Ctrl Pts',(-5.9012568753538,3.31171500752851,145.139896259244));
#45079=CARTESIAN_POINT('Ctrl Pts',(-5.98683247539223,3.15922495420528,145.148106324277));
#45080=CARTESIAN_POINT('Ctrl Pts',(-6.06645335779164,3.00348775974395,145.156316389311));
#45081=CARTESIAN_POINT('Ctrl Pts',(-6.13988467878509,2.84501408278062,145.164526454344));
#45082=CARTESIAN_POINT('Ctrl Pts',(-6.21335114270621,2.6864645631266,145.172740448568));
#45083=CARTESIAN_POINT('Ctrl Pts',(-6.28062200120726,2.52517628027051,145.180954442793));
#45084=CARTESIAN_POINT('Ctrl Pts',(-6.341511105684,2.36167861837434,145.189168437017));
#45085=CARTESIAN_POINT('Ctrl Pts',(-6.40248322228989,2.19795805471039,145.197393629652));
#45086=CARTESIAN_POINT('Ctrl Pts',(-6.4570560849287,2.03202243269057,145.205618822286));
#45087=CARTESIAN_POINT('Ctrl Pts',(-6.50509349167212,1.86441617258728,145.213844014921));
#45088=CARTESIAN_POINT('Ctrl Pts',(-6.54829342872336,1.71368822166918,145.22124091305));
#45089=CARTESIAN_POINT('Ctrl Pts',(-6.58620854212007,1.56160951137961,145.228637811178));
#45090=CARTESIAN_POINT('Ctrl Pts',(-6.61877538971471,1.408581321936,145.236034709307));
#45091=CARTESIAN_POINT('Ctrl Pts',(-6.66778227040013,1.17830314718247,145.247165627121));
#45092=CARTESIAN_POINT('Ctrl Pts',(-6.70477811017182,0.945412940415503,
145.258296544934));
#45093=CARTESIAN_POINT('Ctrl Pts',(-6.72954515647865,0.710992958414298,
145.269427462748));
#45094=CARTESIAN_POINT('Ctrl Pts',(-6.75431220278549,0.476572976413092,
145.280558380562));
#45095=CARTESIAN_POINT('Ctrl Pts',(-6.76685034307383,0.24062281924469,145.291689298376));
#45096=CARTESIAN_POINT('Ctrl Pts',(-6.7669986677552,0.00424624532204132,
145.30282021619));
#45097=CARTESIAN_POINT('Ctrl Pts',(-6.76699866775558,0.00424624472224321,
145.302820216218));
#45098=CARTESIAN_POINT('Ctrl Pts',(-6.76710532578424,-0.165728588349608,
145.31082429152));
#45099=CARTESIAN_POINT('Ctrl Pts',(-6.76080360179688,-0.335917030645911,
145.318828366822));
#45100=CARTESIAN_POINT('Ctrl Pts',(-6.74807175566877,-0.505783135687022,
145.326832442124));
#45101=CARTESIAN_POINT('Ctrl Pts',(-6.73534832620318,-0.67553694706182,
145.334831226159));
#45102=CARTESIAN_POINT('Ctrl Pts',(-6.71620325708614,-0.844968469928021,
145.342830010194));
#45103=CARTESIAN_POINT('Ctrl Pts',(-6.69066686053985,-1.01354129727105,
145.350828794229));
#45104=CARTESIAN_POINT('Ctrl Pts',(-6.66514176758924,-1.18203950644778,
145.35882403763));
#45105=CARTESIAN_POINT('Ctrl Pts',(-6.63323103058441,-1.34967940315641,
145.366819281032));
#45106=CARTESIAN_POINT('Ctrl Pts',(-6.59501682831114,-1.51592942919285,
145.374814524433));
#45107=CARTESIAN_POINT('Ctrl Pts',(-6.56295873406291,-1.65539744596142,
145.381521775959));
#45108=CARTESIAN_POINT('Ctrl Pts',(-6.52646542676354,-1.79388728555138,
145.388229027485));
#45109=CARTESIAN_POINT('Ctrl Pts',(-6.48561325923976,-1.93109027535571,
145.39493627901));
#45110=CARTESIAN_POINT('Ctrl Pts',(-6.43325868069639,-2.10692438995726,
145.403532036545));
#45111=CARTESIAN_POINT('Ctrl Pts',(-6.37378001956298,-2.2805249665359,145.41212779408));
#45112=CARTESIAN_POINT('Ctrl Pts',(-6.30740207231591,-2.45131966461843,
145.420723551615));
#45113=CARTESIAN_POINT('Ctrl Pts',(-6.24096219218916,-2.62227371995626,
145.429327329284));
#45114=CARTESIAN_POINT('Ctrl Pts',(-6.16761028752212,-2.7904163866458,145.437931106953));
#45115=CARTESIAN_POINT('Ctrl Pts',(-6.08761862570831,-2.95519685772865,
145.446534884621));
#45116=CARTESIAN_POINT('Ctrl Pts',(-6.00448322145325,-3.12645334579485,
145.455476798296));
#45117=CARTESIAN_POINT('Ctrl Pts',(-5.91417578569463,-3.29407768641138,
145.46441871197));
#45118=CARTESIAN_POINT('Ctrl Pts',(-5.81705280286035,-3.4574825652105,145.473360625644));
#45119=CARTESIAN_POINT('Ctrl Pts',(-5.72334807106682,-3.61513639641286,
145.481987827962));
#45120=CARTESIAN_POINT('Ctrl Pts',(-5.6232995659211,-3.7688624904389,145.490615030279));
#45121=CARTESIAN_POINT('Ctrl Pts',(-5.51727027242546,-3.91816509874332,
145.499242232597));
#45122=CARTESIAN_POINT('Ctrl Pts',(-5.41114000225819,-4.06760989492768,
145.507877651004));
#45123=CARTESIAN_POINT('Ctrl Pts',(-5.29901775843554,-4.21262255349265,
145.51651306941));
#45124=CARTESIAN_POINT('Ctrl Pts',(-5.18130661292036,-4.35274060597548,
145.525148487817));
#45125=CARTESIAN_POINT('Ctrl Pts',(-5.06342156595441,-4.4930656629225,145.533796663825));
#45126=CARTESIAN_POINT('Ctrl Pts',(-4.93993131965913,-4.62848143545159,
145.542444839833));
#45127=CARTESIAN_POINT('Ctrl Pts',(-4.81127657989389,-4.75856140779591,
145.55109301584));
#45128=CARTESIAN_POINT('Ctrl Pts',(-4.79766539534225,-4.77232337656039,
145.552007960132));
#45129=CARTESIAN_POINT('Ctrl Pts',(-4.78399643654703,-4.78602565922484,
145.552922904423));
#45130=CARTESIAN_POINT('Ctrl Pts',(-4.77027024711876,-4.79966777698764,
145.553837848714));
#45131=CARTESIAN_POINT('Ctrl Pts',(-4.64686215219463,-4.92232000852181,
145.56206384126));
#45132=CARTESIAN_POINT('Ctrl Pts',(-4.51855863337628,-5.04037059823362,
145.570289833807));
#45133=CARTESIAN_POINT('Ctrl Pts',(-4.38573665410778,-5.15340693142076,
145.578515826354));
#45134=CARTESIAN_POINT('Ctrl Pts',(-4.2530539215162,-5.26632476062344,145.58673319501));
#45135=CARTESIAN_POINT('Ctrl Pts',(-4.1158624322524,-5.37423857123331,145.594950563667));
#45136=CARTESIAN_POINT('Ctrl Pts',(-3.97457654674478,-5.47677188442849,
145.603167932324));
#45137=CARTESIAN_POINT('Ctrl Pts',(-3.83341051053263,-5.57921822116947,
145.611378330392));
#45138=CARTESIAN_POINT('Ctrl Pts',(-3.68815728371712,-5.6762929413398,145.619588728459));
#45139=CARTESIAN_POINT('Ctrl Pts',(-3.53926498510135,-5.76765917554389,
145.627799126527));
#45140=CARTESIAN_POINT('Ctrl Pts',(-3.39046920379679,-5.8589661828884,145.636004202321));
#45141=CARTESIAN_POINT('Ctrl Pts',(-3.23803935388692,-5.9445718885637,145.644209278115));
#45142=CARTESIAN_POINT('Ctrl Pts',(-3.08245334911492,-6.02418213125485,
145.652414353909));
#45143=CARTESIAN_POINT('Ctrl Pts',(-2.9269370837608,-6.10375668968255,145.660615751884));
#45144=CARTESIAN_POINT('Ctrl Pts',(-2.76826780034502,-6.17734097632867,
145.668817149859));
#45145=CARTESIAN_POINT('Ctrl Pts',(-2.60694895810223,-6.24468623149712,
145.677018547834));
#45146=CARTESIAN_POINT('Ctrl Pts',(-2.44564275169426,-6.31202621162449,
145.685219303407));
#45147=CARTESIAN_POINT('Ctrl Pts',(-2.28168772685584,-6.37312798772671,
145.69342005898));
#45148=CARTESIAN_POINT('Ctrl Pts',(-2.11560866349979,-6.42779036550856,
145.701620814553));
#45149=CARTESIAN_POINT('Ctrl Pts',(-1.94953044374658,-6.48245246563147,
145.70982152847));
#45150=CARTESIAN_POINT('Ctrl Pts',(-1.78132854704235,-6.53067511953306,
145.718022242387));
#45151=CARTESIAN_POINT('Ctrl Pts',(-1.61154419120836,-6.57230662094995,
145.726222956304));
#45152=CARTESIAN_POINT('Ctrl Pts',(-1.44172992864499,-6.61394545556336,
145.734425114739));
#45153=CARTESIAN_POINT('Ctrl Pts',(-1.27033299967155,-6.6489907392495,145.742627273174));
#45154=CARTESIAN_POINT('Ctrl Pts',(-1.09790617863893,-6.67734161346463,
145.750829431609));
#45155=CARTESIAN_POINT('Ctrl Pts',(-0.925417737055973,-6.70570261949372,
145.759034521267));
#45156=CARTESIAN_POINT('Ctrl Pts',(-0.751899023627536,-6.72736439215343,
145.767239610926));
#45157=CARTESIAN_POINT('Ctrl Pts',(-0.577909376777984,-6.74227778664096,
145.775444700584));
#45158=CARTESIAN_POINT('Ctrl Pts',(-0.40372096732874,-6.75720821791838,
145.783659163587));
#45159=CARTESIAN_POINT('Ctrl Pts',(-0.229060907082588,-6.76537483871306,
145.79187362659));
#45160=CARTESIAN_POINT('Ctrl Pts',(-0.0544910606802038,-6.76678060264303,
145.800088089593));
#45161=CARTESIAN_POINT('Ctrl Pts',(0.12018221283816,-6.7681871994437,145.808307419406));
#45162=CARTESIAN_POINT('Ctrl Pts',(0.29476480836678,-6.76282496567511,145.816526749218));
#45163=CARTESIAN_POINT('Ctrl Pts',(0.468698637813905,-6.75074889082029,
145.824746079031));
#45164=CARTESIAN_POINT('Ctrl Pts',(0.642901967182734,-6.73865410481976,
145.832978144197));
#45165=CARTESIAN_POINT('Ctrl Pts',(0.816454165608605,-6.71982472772884,
145.841210209363));
#45166=CARTESIAN_POINT('Ctrl Pts',(0.988804675396828,-6.6943673572574,145.849442274529));
#45167=CARTESIAN_POINT('Ctrl Pts',(1.14372568761367,-6.67148444494887,145.856841845726));
#45168=CARTESIAN_POINT('Ctrl Pts',(1.29767573289346,-6.64324703872476,145.864241416924));
#45169=CARTESIAN_POINT('Ctrl Pts',(1.45026540971424,-6.60976695817533,145.871640988122));
#45170=CARTESIAN_POINT('Ctrl Pts',(1.61844255534776,-6.57286679232076,145.879796446531));
#45171=CARTESIAN_POINT('Ctrl Pts',(1.78548477583121,-6.52948366823578,145.88795190494));
#45172=CARTESIAN_POINT('Ctrl Pts',(1.95084858414145,-6.47969743134302,145.896107363348));
#45173=CARTESIAN_POINT('Ctrl Pts',(2.11601112296054,-6.42997179084476,145.904252895492));
#45174=CARTESIAN_POINT('Ctrl Pts',(2.2794989698499,-6.37385865492978,145.912398427636));
#45175=CARTESIAN_POINT('Ctrl Pts',(2.44077743612675,-6.31148908794862,145.92054395978));
#45176=CARTESIAN_POINT('Ctrl Pts',(2.60189351893728,-6.24918231785978,145.928681290583));
#45177=CARTESIAN_POINT('Ctrl Pts',(2.76080431140704,-6.18063178833523,145.936818621386));
#45178=CARTESIAN_POINT('Ctrl Pts',(2.91698893908493,-6.10601871347085,145.944955952188));
#45179=CARTESIAN_POINT('Ctrl Pts',(3.07304913471808,-6.03146508272467,145.953086799993));
#45180=CARTESIAN_POINT('Ctrl Pts',(3.22638716187806,-5.95085868063015,145.961217647797));
#45181=CARTESIAN_POINT('Ctrl Pts',(3.37650084473444,-5.86442930262678,145.969348495601));
#45182=CARTESIAN_POINT('Ctrl Pts',(3.52652646623596,-5.77805062678448,145.977474573597));
#45183=CARTESIAN_POINT('Ctrl Pts',(3.67333119436201,-5.68585595972377,145.985600651593));
#45184=CARTESIAN_POINT('Ctrl Pts',(3.81643625478613,-5.58812162655342,145.993726729589));
#45185=CARTESIAN_POINT('Ctrl Pts',(3.96004873955535,-5.49004074533051,146.00188162117));
#45186=CARTESIAN_POINT('Ctrl Pts',(4.09993493891927,-5.38638100644084,146.01003651275));
#45187=CARTESIAN_POINT('Ctrl Pts',(4.23563868442833,-5.27746662092469,146.018191404331));
#45188=CARTESIAN_POINT('Ctrl Pts',(4.37081323283637,-5.16897696338387,146.02631449469));
#45189=CARTESIAN_POINT('Ctrl Pts',(4.50183761251203,-5.05527381211952,146.034437585048));
#45190=CARTESIAN_POINT('Ctrl Pts',(4.62829291269694,-4.93671892194394,146.042560675407));
#45191=CARTESIAN_POINT('Ctrl Pts',(4.75475814272944,-4.81815472229703,146.050684403627));
#45192=CARTESIAN_POINT('Ctrl Pts',(4.87665331169783,-4.69473827504831,146.058808131848));
#45193=CARTESIAN_POINT('Ctrl Pts',(4.99359546364005,-4.56686909660366,146.066931860069));
#45194=CARTESIAN_POINT('Ctrl Pts',(5.11056904651986,-4.43896555032756,146.075057771731));
#45195=CARTESIAN_POINT('Ctrl Pts',(5.2225867148445,-4.3066071596935,146.083183683394));
#45196=CARTESIAN_POINT('Ctrl Pts',(5.32930502132712,-4.17022745059038,146.091309595056));
#45197=CARTESIAN_POINT('Ctrl Pts',(5.43670580239076,-4.03297557917606,146.099487472763));
#45198=CARTESIAN_POINT('Ctrl Pts',(5.53873897495106,-3.89165107307566,146.107665350469));
#45199=CARTESIAN_POINT('Ctrl Pts',(5.63509850285464,-3.74672575232367,146.115843228175));
#45200=CARTESIAN_POINT('Ctrl Pts',(5.73099812770412,-3.60249212858475,146.12398207465));
#45201=CARTESIAN_POINT('Ctrl Pts',(5.82127800915604,-3.45469233096788,146.132120921126));
#45202=CARTESIAN_POINT('Ctrl Pts',(5.90568266291211,-3.30381616997366,146.140259767602));
#45203=CARTESIAN_POINT('Ctrl Pts',(5.9906944820993,-3.15185468032441,146.148457160923));
#45204=CARTESIAN_POINT('Ctrl Pts',(6.06974605637035,-2.99677273730642,146.156654554244));
#45205=CARTESIAN_POINT('Ctrl Pts',(6.14262582048684,-2.83909088080822,146.164851947565));
#45206=CARTESIAN_POINT('Ctrl Pts',(6.21550558460327,-2.68140902431015,146.173049340887));
#45207=CARTESIAN_POINT('Ctrl Pts',(6.28221345195744,-2.52112762147068,146.181246734208));
#45208=CARTESIAN_POINT('Ctrl Pts',(6.34258911909827,-2.35878194547446,146.189444127529));
#45209=CARTESIAN_POINT('Ctrl Pts',(6.40317702262229,-2.19586558163773,146.197670336849));
#45210=CARTESIAN_POINT('Ctrl Pts',(6.45756855974203,-2.03038557931949,146.205896546168));
#45211=CARTESIAN_POINT('Ctrl Pts',(6.50554111361607,-1.86285367623198,146.214122755487));
#45212=CARTESIAN_POINT('Ctrl Pts',(6.55345977238034,-1.69550998806275,146.222339723013));
#45213=CARTESIAN_POINT('Ctrl Pts',(6.59497371003025,-1.52611933109708,146.230556690538));
#45214=CARTESIAN_POINT('Ctrl Pts',(6.62990852064688,-1.35521290130148,146.238773658064));
#45215=CARTESIAN_POINT('Ctrl Pts',(6.66481109519662,-1.1844641752691,146.246983043389));
#45216=CARTESIAN_POINT('Ctrl Pts',(6.69314656173241,-1.01220281108887,146.255192428715));
#45217=CARTESIAN_POINT('Ctrl Pts',(6.71479042235199,-0.838974721842076,
146.263401814041));
#45218=CARTESIAN_POINT('Ctrl Pts',(6.73641865381941,-0.665871721562182,
146.271605271324));
#45219=CARTESIAN_POINT('Ctrl Pts',(6.75136485969259,-0.491803741093733,
146.279808728607));
#45220=CARTESIAN_POINT('Ctrl Pts',(6.75955567154628,-0.317326524681699,
146.288012185889));
#45221=CARTESIAN_POINT('Ctrl Pts',(6.76774221182591,-0.142940299536919,
146.296211365004));
#45222=CARTESIAN_POINT('Ctrl Pts',(6.769180359736,0.0318543789915835,146.304410544118));
#45223=CARTESIAN_POINT('Ctrl Pts',(6.76384861027529,0.206496918323283,146.312609723232));
#45224=CARTESIAN_POINT('Ctrl Pts',(6.75851786543104,0.381106551238395,146.320807357444));
#45225=CARTESIAN_POINT('Ctrl Pts',(6.74641976878472,0.555563743767707,146.329004991656));
#45226=CARTESIAN_POINT('Ctrl Pts',(6.72758493374229,0.729307863171511,146.337202625868));
#45227=CARTESIAN_POINT('Ctrl Pts',(6.70875145821885,0.903039441534751,146.345399668366));
#45228=CARTESIAN_POINT('Ctrl Pts',(6.68318225050078,1.07605769259408,146.353596710864));
#45229=CARTESIAN_POINT('Ctrl Pts',(6.65095980993641,1.24780711915372,146.361793753362));
#45230=CARTESIAN_POINT('Ctrl Pts',(6.61873383884821,1.41957536382374,146.369991693987));
#45231=CARTESIAN_POINT('Ctrl Pts',(6.57985324873458,1.59007415442005,146.378189634613));
#45232=CARTESIAN_POINT('Ctrl Pts',(6.53445168184405,1.75875814643328,146.386387575238));
#45233=CARTESIAN_POINT('Ctrl Pts',(6.48903688873982,1.92749127883262,146.394587904056));
#45234=CARTESIAN_POINT('Ctrl Pts',(6.43709742815154,2.09440821331476,146.402788232875));
#45235=CARTESIAN_POINT('Ctrl Pts',(6.37881684499615,2.2589786758607,146.410988561693));
#45236=CARTESIAN_POINT('Ctrl Pts',(6.32047553195928,2.42372062510332,146.419197435467));
#45237=CARTESIAN_POINT('Ctrl Pts',(6.25578001523389,2.58611087894923,146.427406309242));
#45238=CARTESIAN_POINT('Ctrl Pts',(6.18496242640183,2.74563813784657,146.435615183016));
#45239=CARTESIAN_POINT('Ctrl Pts',(6.1141068305503,2.90525101326567,146.443828462402));
#45240=CARTESIAN_POINT('Ctrl Pts',(6.03712277050334,3.06199750896016,146.452041741788));
#45241=CARTESIAN_POINT('Ctrl Pts',(5.95428836567338,3.21539096509378,146.460255021174));
#45242=CARTESIAN_POINT('Ctrl Pts',(5.87133280250385,3.36900878327216,146.468480313773));
#45243=CARTESIAN_POINT('Ctrl Pts',(5.7825099763599,3.51926345212565,146.476705606371));
#45244=CARTESIAN_POINT('Ctrl Pts',(5.688142047697,3.66569625654136,146.48493089897));
#45245=CARTESIAN_POINT('Ctrl Pts',(5.60279758952673,3.79812714199456,146.492369688292));
#45246=CARTESIAN_POINT('Ctrl Pts',(5.51291844001722,3.92743235224374,146.499808477615));
#45247=CARTESIAN_POINT('Ctrl Pts',(5.41877068292729,4.0532965948531,146.507247266937));
#45248=CARTESIAN_POINT('Ctrl Pts',(5.31465068167149,4.19249253008954,146.515473981811));
#45249=CARTESIAN_POINT('Ctrl Pts',(5.20501825343316,4.32786854475823,146.523700696685));
#45250=CARTESIAN_POINT('Ctrl Pts',(5.09018299449507,4.45896020194767,146.531927411558));
#45251=CARTESIAN_POINT('Ctrl Pts',(4.97547307725163,4.58990877372399,146.540145147044));
#45252=CARTESIAN_POINT('Ctrl Pts',(4.85557187037958,4.71658203140227,146.548362882529));
#45253=CARTESIAN_POINT('Ctrl Pts',(4.73083148838794,4.8385454868666,146.556580618015));
#45254=CARTESIAN_POINT('Ctrl Pts',(4.60623003637546,4.96037310516212,146.564789200973));
#45255=CARTESIAN_POINT('Ctrl Pts',(4.47680040494159,5.07750112571033,146.57299778393));
#45256=CARTESIAN_POINT('Ctrl Pts',(4.34293390232146,5.18952927731089,146.581206366888));
#45257=CARTESIAN_POINT('Ctrl Pts',(4.20915413810584,5.30148484060192,146.589409631119));
#45258=CARTESIAN_POINT('Ctrl Pts',(4.07094350009997,5.4083468846326,146.597612895349));
#45259=CARTESIAN_POINT('Ctrl Pts',(3.92872934099403,5.50975269546761,146.60581615958));
#45260=CARTESIAN_POINT('Ctrl Pts',(3.78658379393986,5.61110958247685,146.614015466098));
#45261=CARTESIAN_POINT('Ctrl Pts',(3.64043886376392,5.70701527105099,146.622214772615));
#45262=CARTESIAN_POINT('Ctrl Pts',(3.49075412609444,5.79714797388808,146.630414079133));
#45263=CARTESIAN_POINT('Ctrl Pts',(3.36271593860724,5.87424620103042,146.637427648864));
#45264=CARTESIAN_POINT('Ctrl Pts',(3.23208837159504,5.94712101654775,146.644441218594));
#45265=CARTESIAN_POINT('Ctrl Pts',(3.09917575053262,6.01559628526637,146.651454788324));
#45266=CARTESIAN_POINT('Origin',(0.,0.,-3.69717978381041));
#45267=CARTESIAN_POINT('',(3.09917575053273,6.01559628526631,149.045786479356));
#45268=CARTESIAN_POINT('',(3.09917575053258,6.01559628526639,148.651204821489));
#45269=CARTESIAN_POINT('',(3.09917575053259,6.01559628526639,-3.69717978381041));
#45270=CARTESIAN_POINT('',(-6.767,3.61801146291416E-8,147.697179782109));
#45271=CARTESIAN_POINT('Ctrl Pts',(-6.76699999998963,1.18489098065876E-5,
147.697431498484));
#45272=CARTESIAN_POINT('Ctrl Pts',(-6.76700030221227,-0.172589739342158,
147.705556329219));
#45273=CARTESIAN_POINT('Ctrl Pts',(-6.76039261620527,-0.345365153995567,
147.713681159955));
#45274=CARTESIAN_POINT('Ctrl Pts',(-6.74716305906021,-0.517764091506218,
147.72180599069));
#45275=CARTESIAN_POINT('Ctrl Pts',(-6.73394247234798,-0.69004613220238,
147.729925312303));
#45276=CARTESIAN_POINT('Ctrl Pts',(-6.71410898296127,-0.861951839635234,
147.738044633917));
#45277=CARTESIAN_POINT('Ctrl Pts',(-6.68770077749777,-1.03293141624008,
147.74616395553));
#45278=CARTESIAN_POINT('Ctrl Pts',(-6.66130489176939,-1.20383122888302,
147.754279489385));
#45279=CARTESIAN_POINT('Ctrl Pts',(-6.62834045449182,-1.3738054093097,147.76239502324));
#45280=CARTESIAN_POINT('Ctrl Pts',(-6.58889743896392,-1.54230980636663,
147.770510557096));
#45281=CARTESIAN_POINT('Ctrl Pts',(-6.54945813819784,-1.7107983335999,147.778625326626));
#45282=CARTESIAN_POINT('Ctrl Pts',(-6.50354154946792,-1.87781699413692,
147.786740096157));
#45283=CARTESIAN_POINT('Ctrl Pts',(-6.45128870527251,-2.0428321128334,147.794854865687));
#45284=CARTESIAN_POINT('Ctrl Pts',(-6.39903587011488,-2.20784720298848,
147.802969633814));
#45285=CARTESIAN_POINT('Ctrl Pts',(-6.34044689170832,-2.37085840179826,
147.811084401941));
#45286=CARTESIAN_POINT('Ctrl Pts',(-6.27571253911645,-2.53134768974485,
147.819199170068));
#45287=CARTESIAN_POINT('Ctrl Pts',(-6.21096579408922,-2.69186770099439,
147.827315491647));
#45288=CARTESIAN_POINT('Ctrl Pts',(-6.14007146962038,-2.8498644996653,147.835431813226));
#45289=CARTESIAN_POINT('Ctrl Pts',(-6.06326826634064,-3.00484058319016,
147.843548134806));
#45290=CARTESIAN_POINT('Ctrl Pts',(-5.98643564276011,-3.15987603198623,
147.85166756543));
#45291=CARTESIAN_POINT('Ctrl Pts',(-5.90368979646056,-3.31188813315499,
147.859786996055));
#45292=CARTESIAN_POINT('Ctrl Pts',(-5.81531506766974,-3.46040455203338,
147.867906426679));
#45293=CARTESIAN_POINT('Ctrl Pts',(-5.72684077024805,-3.60908829902345,
147.876035005174));
#45294=CARTESIAN_POINT('Ctrl Pts',(-5.63272511365515,-3.75426818334733,
147.88416358367));
#45295=CARTESIAN_POINT('Ctrl Pts',(-5.53329587632421,-3.89550070530779,
147.892292162165));
#45296=CARTESIAN_POINT('Ctrl Pts',(-5.433803534497,-4.03682286294679,147.900425899604));
#45297=CARTESIAN_POINT('Ctrl Pts',(-5.32899111528955,-4.17419237636698,
147.908559637043));
#45298=CARTESIAN_POINT('Ctrl Pts',(-5.21922603288083,-4.30719962594016,
147.916693374482));
#45299=CARTESIAN_POINT('Ctrl Pts',(-5.10930377981723,-4.44039732621095,
147.924838758473));
#45300=CARTESIAN_POINT('Ctrl Pts',(-4.99441494525329,-4.56922001643452,
147.932984142465));
#45301=CARTESIAN_POINT('Ctrl Pts',(-4.87496369336073,-4.6932950033441,147.941129526457));
#45302=CARTESIAN_POINT('Ctrl Pts',(-4.81399306195092,-4.75662569410024,
147.945287115408));
#45303=CARTESIAN_POINT('Ctrl Pts',(-4.75183431668322,-4.818720103377,147.949444704359));
#45304=CARTESIAN_POINT('Ctrl Pts',(-4.6885443610219,-4.87953284390317,147.953602293311));
#45305=CARTESIAN_POINT('Ctrl Pts',(-4.5644196466217,-4.99879922623558,147.961756186543));
#45306=CARTESIAN_POINT('Ctrl Pts',(-4.43553781951026,-5.11352168817597,
147.969910079775));
#45307=CARTESIAN_POINT('Ctrl Pts',(-4.30226700957082,-5.22329279079381,
147.978063973008));
#45308=CARTESIAN_POINT('Ctrl Pts',(-4.16915882717726,-5.33292994206074,
147.986207916217));
#45309=CARTESIAN_POINT('Ctrl Pts',(-4.03167260190153,-5.43762753094104,
147.994351859426));
#45310=CARTESIAN_POINT('Ctrl Pts',(-3.89021417056718,-5.53701387998245,
148.002495802636));
#45311=CARTESIAN_POINT('Ctrl Pts',(-3.74889858379892,-5.63629986879952,
148.0106315221));
#45312=CARTESIAN_POINT('Ctrl Pts',(-3.60361907328117,-5.73028508639669,
148.018767241564));
#45313=CARTESIAN_POINT('Ctrl Pts',(-3.45481550655504,-5.81863719574153,
148.026902961029));
#45314=CARTESIAN_POINT('Ctrl Pts',(-3.30613090065821,-5.90691867210069,
148.035032176402));
#45315=CARTESIAN_POINT('Ctrl Pts',(-3.1539281610335,-5.98957582110507,148.043161391776));
#45316=CARTESIAN_POINT('Ctrl Pts',(-2.998677167291,-6.06631883817259,148.051290607149));
#45317=CARTESIAN_POINT('Ctrl Pts',(-2.84351764533614,-6.14301663929146,
148.059415032899));
#45318=CARTESIAN_POINT('Ctrl Pts',(-2.68531377287162,-6.21380708614292,
148.067539458649));
#45319=CARTESIAN_POINT('Ctrl Pts',(-2.52456112158583,-6.27844567893816,
148.075663884398));
#45320=CARTESIAN_POINT('Ctrl Pts',(-2.36283263342434,-6.34347665544801,
148.083837628863));
#45321=CARTESIAN_POINT('Ctrl Pts',(-2.19852464358827,-6.40228065315007,
148.092011373328));
#45322=CARTESIAN_POINT('Ctrl Pts',(-2.0321639654529,-6.45465712625503,148.100185117793));
#45323=CARTESIAN_POINT('Ctrl Pts',(-1.86686857706813,-6.50669820688264,
148.108306521727));
#45324=CARTESIAN_POINT('Ctrl Pts',(-1.69954707236529,-6.55239375033596,
148.116427925661));
#45325=CARTESIAN_POINT('Ctrl Pts',(-1.53073283787493,-6.59159661835062,
148.124549329596));
#45326=CARTESIAN_POINT('Ctrl Pts',(-1.36190555159674,-6.63080251731536,
148.132671361432));
#45327=CARTESIAN_POINT('Ctrl Pts',(-1.1915856621398,-6.66351465811254,148.140793393268));
#45328=CARTESIAN_POINT('Ctrl Pts',(-1.02031796570017,-6.68963678004041,
148.148915425105));
#45329=CARTESIAN_POINT('Ctrl Pts',(-0.849004414479253,-6.71576589583937,
148.157039631514));
#45330=CARTESIAN_POINT('Ctrl Pts',(-0.676742912638536,-6.73530142438346,
148.165163837922));
#45331=CARTESIAN_POINT('Ctrl Pts',(-0.504084569463769,-6.74819885205145,
148.173288044331));
#45332=CARTESIAN_POINT('Ctrl Pts',(-0.32955738407196,-6.76123588060333,
148.1815001866));
#45333=CARTESIAN_POINT('Ctrl Pts',(-0.154625098924222,-6.76749023865297,
148.189712328869));
#45334=CARTESIAN_POINT('Ctrl Pts',(0.0201426923150803,-6.76697002150492,
148.197924471137));
#45335=CARTESIAN_POINT('Ctrl Pts',(0.19331511027857,-6.76645455317546,148.206061648608));
#45336=CARTESIAN_POINT('Ctrl Pts',(0.366325662320664,-6.75928775695696,
148.214198826078));
#45337=CARTESIAN_POINT('Ctrl Pts',(0.538625371183535,-6.74552975751478,
148.222336003548));
#45338=CARTESIAN_POINT('Ctrl Pts',(0.713306080042034,-6.73158163705134,
148.230585628216));
#45339=CARTESIAN_POINT('Ctrl Pts',(0.887255765966873,-6.71085885889615,
148.238835252884));
#45340=CARTESIAN_POINT('Ctrl Pts',(1.05991347156252,-6.68347757030727,148.247084877552));
#45341=CARTESIAN_POINT('Ctrl Pts',(1.23257117715829,-6.65609628171836,148.255334502221));
#45342=CARTESIAN_POINT('Ctrl Pts',(1.40393653734784,-6.62205661971031,148.263584126889));
#45343=CARTESIAN_POINT('Ctrl Pts',(1.57346533802009,-6.58152686160661,148.271833751557));
#45344=CARTESIAN_POINT('Ctrl Pts',(1.74248533610249,-6.5411187444619,148.280058616831));
#45345=CARTESIAN_POINT('Ctrl Pts',(1.91018504262813,-6.49413881720199,148.288283482105));
#45346=CARTESIAN_POINT('Ctrl Pts',(2.07601559175624,-6.44068694028712,148.29650834738));
#45347=CARTESIAN_POINT('Ctrl Pts',(2.24165931412539,-6.38729528292152,148.304723946418));
#45348=CARTESIAN_POINT('Ctrl Pts',(2.40543773395594,-6.32744630395622,148.312939545457));
#45349=CARTESIAN_POINT('Ctrl Pts',(2.56681265041902,-6.26129074693461,148.321155144495));
#45350=CARTESIAN_POINT('Ctrl Pts',(2.72803818340686,-6.19519642958537,148.329363138419));
#45351=CARTESIAN_POINT('Ctrl Pts',(2.88686431410104,-6.12280729580259,148.337571132343));
#45352=CARTESIAN_POINT('Ctrl Pts',(3.04276839207491,-6.04432374316514,148.345779126267));
#45353=CARTESIAN_POINT('Ctrl Pts',(3.19855946508222,-5.96589707827147,148.353981170738));
#45354=CARTESIAN_POINT('Ctrl Pts',(3.35143238488852,-5.8813849539298,148.362183215208));
#45355=CARTESIAN_POINT('Ctrl Pts',(3.50088479236352,-5.79103571657073,148.370385259679));
#45356=CARTESIAN_POINT('Ctrl Pts',(3.65025888270915,-5.70073382467119,148.378583006054));
#45357=CARTESIAN_POINT('Ctrl Pts',(3.79621572525279,-5.60460109855421,148.38678075243));
#45358=CARTESIAN_POINT('Ctrl Pts',(3.93827780206285,-5.50293166900871,148.394978498806));
#45359=CARTESIAN_POINT('Ctrl Pts',(4.08031278365309,-5.40128163067305,148.403174681642));
#45360=CARTESIAN_POINT('Ctrl Pts',(4.21845418407797,-5.2940971958665,148.411370864478));
#45361=CARTESIAN_POINT('Ctrl Pts',(4.35225346470765,-5.18171581418166,148.419567047314));
#45362=CARTESIAN_POINT('Ctrl Pts',(4.4860428473285,-5.06934274608343,148.427762623824));
#45363=CARTESIAN_POINT('Ctrl Pts',(4.61549047452351,-4.95177372684966,148.435958200335));
#45364=CARTESIAN_POINT('Ctrl Pts',(4.74018095837061,-4.82938644984026,148.444153776845));
#45365=CARTESIAN_POINT('Ctrl Pts',(4.8648849040407,-4.70698595966649,148.452350238166));
#45366=CARTESIAN_POINT('Ctrl Pts',(4.98483042699659,-4.57976642674965,148.460546699486));
#45367=CARTESIAN_POINT('Ctrl Pts',(5.09963904573666,-4.44814237667794,148.468743160807));
#45368=CARTESIAN_POINT('Ctrl Pts',(5.21448094762456,-4.31648016864593,148.476941998291));
#45369=CARTESIAN_POINT('Ctrl Pts',(5.32418274320228,-4.18041117043751,148.485140835775));
#45370=CARTESIAN_POINT('Ctrl Pts',(5.42840625351473,-4.04038297031385,148.493339673259));
#45371=CARTESIAN_POINT('Ctrl Pts',(5.53273862871813,-3.90020850612087,148.501547074699));
#45372=CARTESIAN_POINT('Ctrl Pts',(5.63158107181388,-3.7560668660245,148.509754476139));
#45373=CARTESIAN_POINT('Ctrl Pts',(5.72463821485365,-3.6084354378369,148.517961877579));
#45374=CARTESIAN_POINT('Ctrl Pts',(5.81774520441193,-3.46072493014529,148.526173675354));
#45375=CARTESIAN_POINT('Ctrl Pts',(5.90506053685541,-3.30952121826683,148.534385473129));
#45376=CARTESIAN_POINT('Ctrl Pts',(5.98633491887672,-3.15532616999214,148.542597270904));
#45377=CARTESIAN_POINT('Ctrl Pts',(6.06772894864998,-3.00090412410236,148.550821157644));
#45378=CARTESIAN_POINT('Ctrl Pts',(6.14306410036819,-2.84348226485778,148.559045044384));
#45379=CARTESIAN_POINT('Ctrl Pts',(6.21213881171551,-2.68358349674047,148.567268931124));
#45380=CARTESIAN_POINT('Ctrl Pts',(6.27596290606529,-2.53583920851005,148.574867690684));
#45381=CARTESIAN_POINT('Ctrl Pts',(6.33444260790102,-2.38598066718417,148.582466450244));
#45382=CARTESIAN_POINT('Ctrl Pts',(6.38745708405515,-2.23443079985791,148.590065209804));
#45383=CARTESIAN_POINT('Ctrl Pts',(6.44483961693894,-2.07039418427202,148.598290058976));
#45384=CARTESIAN_POINT('Ctrl Pts',(6.49597967538635,-1.90391545841032,148.606514908149));
#45385=CARTESIAN_POINT('Ctrl Pts',(6.54066455293232,-1.73551035894767,148.614739757322));
#45386=CARTESIAN_POINT('Ctrl Pts',(6.58529910532507,-1.56729492124308,148.622955343477));
#45387=CARTESIAN_POINT('Ctrl Pts',(6.62349286201827,-1.39715777363023,148.631170929632));
#45388=CARTESIAN_POINT('Ctrl Pts',(6.65508168916922,-1.2256331875747,148.639386515787));
#45389=CARTESIAN_POINT('Ctrl Pts',(6.68664128706593,-1.05426731382947,148.647594500031));
#45390=CARTESIAN_POINT('Ctrl Pts',(6.71160806215666,-0.881516908974152,
148.655802484276));
#45391=CARTESIAN_POINT('Ctrl Pts',(6.72986806023965,-0.707930004849491,
148.66401046852));
#45392=CARTESIAN_POINT('Ctrl Pts',(6.74811482989324,-0.534468855508366,
148.672212506501));
#45393=CARTESIAN_POINT('Ctrl Pts',(6.75966446280209,-0.360172769293801,
148.680414544483));
#45394=CARTESIAN_POINT('Ctrl Pts',(6.76445431274541,-0.185598628173927,
148.688616582465));
#45395=CARTESIAN_POINT('Ctrl Pts',(6.7692416545327,-0.0111159010211107,
148.696814325533));
#45396=CARTESIAN_POINT('Ctrl Pts',(6.76727625517002,0.163644233189768,148.705012068601));
#45397=CARTESIAN_POINT('Ctrl Pts',(6.75854741509987,0.338121040231024,148.713209811669));
#45398=CARTESIAN_POINT('Ctrl Pts',(6.74982023470305,0.512564672818135,148.721405996045));
#45399=CARTESIAN_POINT('Ctrl Pts',(6.7343321867894,0.686724727267406,148.729602180421));
#45400=CARTESIAN_POINT('Ctrl Pts',(6.71212468128308,0.860041430926754,148.737798364797));
#45401=CARTESIAN_POINT('Ctrl Pts',(6.68991881060401,1.03334537570733,148.745993945803));
#45402=CARTESIAN_POINT('Ctrl Pts',(6.66099451217594,1.20580573731151,148.754189526809));
#45403=CARTESIAN_POINT('Ctrl Pts',(6.62544497345568,1.37686887673116,148.762385107815));
#45404=CARTESIAN_POINT('Ctrl Pts',(6.58989158393448,1.54795054607048,148.770581576583));
#45405=CARTESIAN_POINT('Ctrl Pts',(6.54771159734892,1.71763434029412,148.778778045352));
#45406=CARTESIAN_POINT('Ctrl Pts',(6.49904913891051,1.88537775791128,148.78697451412));
#45407=CARTESIAN_POINT('Ctrl Pts',(6.45037255566012,2.05316986489414,148.795173362003));
#45408=CARTESIAN_POINT('Ctrl Pts',(6.39520985258252,2.21902012888161,148.803372209887));
#45409=CARTESIAN_POINT('Ctrl Pts',(6.33375475728329,2.38240208079814,148.81157105777));
#45410=CARTESIAN_POINT('Ctrl Pts',(6.27223543567658,2.54595478209566,148.819778474214));
#45411=CARTESIAN_POINT('Ctrl Pts',(6.2044107100859,2.70703368127936,148.827985890659));
#45412=CARTESIAN_POINT('Ctrl Pts',(6.13052252148254,2.86513221572677,148.836193307103));
#45413=CARTESIAN_POINT('Ctrl Pts',(6.05659473155843,3.02331548510802,148.844405122417));
#45414=CARTESIAN_POINT('Ctrl Pts',(5.97659716433209,3.17851488671776,148.852616937731));
#45415=CARTESIAN_POINT('Ctrl Pts',(5.89081726300164,3.33024938614541,148.860828753045));
#45416=CARTESIAN_POINT('Ctrl Pts',(5.80491103808832,3.48220733704962,148.869052661471));
#45417=CARTESIAN_POINT('Ctrl Pts',(5.71320564995931,3.63068988310866,148.877276569897));
#45418=CARTESIAN_POINT('Ctrl Pts',(5.61603204282505,3.77524477272168,148.885500478323));
#45419=CARTESIAN_POINT('Ctrl Pts',(5.52624553783209,3.9088106523958,148.893099208232));
#45420=CARTESIAN_POINT('Ctrl Pts',(5.43179119289796,4.03902350447473,148.900697938142));
#45421=CARTESIAN_POINT('Ctrl Pts',(5.33295947919684,4.16555304770502,148.908296668051));
#45422=CARTESIAN_POINT('Ctrl Pts',(5.22693461647475,4.30129163756545,148.916448447124));
#45423=CARTESIAN_POINT('Ctrl Pts',(5.11555741577803,4.43319289296123,148.924600226197));
#45424=CARTESIAN_POINT('Ctrl Pts',(4.99913698328774,4.56080238799323,148.932752005271));
#45425=CARTESIAN_POINT('Ctrl Pts',(4.88284860610434,4.68826713600216,148.940894537808));
#45426=CARTESIAN_POINT('Ctrl Pts',(4.76152862715262,4.8114495455013,148.949037070345));
#45427=CARTESIAN_POINT('Ctrl Pts',(4.63552842812275,4.92992547530547,148.957179602883));
#45428=CARTESIAN_POINT('Ctrl Pts',(4.50967383726271,5.04826449212506,148.965312725759));
#45429=CARTESIAN_POINT('Ctrl Pts',(4.37915006662856,5.16190761644505,148.973445848634));
#45430=CARTESIAN_POINT('Ctrl Pts',(4.24434734603993,5.27046531211086,148.98157897151));
#45431=CARTESIAN_POINT('Ctrl Pts',(4.10963473767697,5.37895043968956,148.989706657598));
#45432=CARTESIAN_POINT('Ctrl Pts',(3.9706491556476,5.48235667595469,148.997834343685));
#45433=CARTESIAN_POINT('Ctrl Pts',(3.82781643569586,5.58033245735562,149.005962029773));
#45434=CARTESIAN_POINT('Ctrl Pts',(3.68505784274448,5.67825739150822,149.014085497773));
#45435=CARTESIAN_POINT('Ctrl Pts',(3.53845638861122,5.77075727651909,149.022208965772));
#45436=CARTESIAN_POINT('Ctrl Pts',(3.38846954371261,5.85752192922332,149.030332433772));
#45437=CARTESIAN_POINT('Ctrl Pts',(3.2933581315994,5.91254214546822,149.0354837823));
#45438=CARTESIAN_POINT('Ctrl Pts',(3.19688601129499,5.96525692464893,149.040635130828));
#45439=CARTESIAN_POINT('Ctrl Pts',(3.09917575053273,6.01559628526631,149.045786479356));
#45440=CARTESIAN_POINT('Ctrl Pts',(3.09917575053267,6.01559628526635,147.045751582743));
#45441=CARTESIAN_POINT('Ctrl Pts',(2.9338238445929,6.10078395293747,147.054501030655));
#45442=CARTESIAN_POINT('Ctrl Pts',(2.76495772123027,6.17915010267029,147.063250478567));
#45443=CARTESIAN_POINT('Ctrl Pts',(2.59315093316772,6.25042856433152,147.07199992648));
#45444=CARTESIAN_POINT('Ctrl Pts',(2.42134553245695,6.32170645041421,147.08074930374));
#45445=CARTESIAN_POINT('Ctrl Pts',(2.24659977927686,6.38589665313423,147.089498681));
#45446=CARTESIAN_POINT('Ctrl Pts',(2.06950718690031,6.44278115439039,147.09824805826));
#45447=CARTESIAN_POINT('Ctrl Pts',(1.89241596572979,6.49966521519689,147.106997367774));
#45448=CARTESIAN_POINT('Ctrl Pts',(1.71297821457321,6.54924360009514,147.115746677289));
#45449=CARTESIAN_POINT('Ctrl Pts',(1.53180337335973,6.59134792173526,147.124495986804));
#45450=CARTESIAN_POINT('Ctrl Pts',(1.35062987477911,6.63345193135279,147.13324523148));
#45451=CARTESIAN_POINT('Ctrl Pts',(1.1677195910308,6.66808192368215,147.141994476156));
#45452=CARTESIAN_POINT('Ctrl Pts',(0.98369374690812,6.6951202836315,147.150743720832));
#45453=CARTESIAN_POINT('Ctrl Pts',(0.79966920542126,6.7221584521885,147.159492903576));
#45454=CARTESIAN_POINT('Ctrl Pts',(0.614529402874977,6.74160505424565,147.16824208632));
#45455=CARTESIAN_POINT('Ctrl Pts',(0.428903127364861,6.75339404354112,147.176991269065));
#45456=CARTESIAN_POINT('Ctrl Pts',(0.243278104165756,6.76518295330323,147.185740392783));
#45457=CARTESIAN_POINT('Ctrl Pts',(0.0571669005412571,6.76931433552273,
147.194489516502));
#45458=CARTESIAN_POINT('Ctrl Pts',(-0.128798404775113,6.76577415902478,
147.20323864022));
#45459=CARTESIAN_POINT('Ctrl Pts',(-0.314762517256553,6.76223400523453,
147.21198770782));
#45460=CARTESIAN_POINT('Ctrl Pts',(-0.500580446816821,6.75102239665108,
147.220736775419));
#45461=CARTESIAN_POINT('Ctrl Pts',(-0.685621118839784,6.73217741012526,
147.229485843018));
#45462=CARTESIAN_POINT('Ctrl Pts',(-0.870660665411512,6.7133325382181,147.238234857404));
#45463=CARTESIAN_POINT('Ctrl Pts',(-1.05492267885174,6.68685441030661,147.246983871789));
#45464=CARTESIAN_POINT('Ctrl Pts',(-1.23778137634926,6.65283295028238,147.255732886175));
#45465=CARTESIAN_POINT('Ctrl Pts',(-1.42999922904426,6.61707018875721,147.264929696507));
#45466=CARTESIAN_POINT('Ctrl Pts',(-1.62066601086376,6.57297172968495,147.274126506839));
#45467=CARTESIAN_POINT('Ctrl Pts',(-1.8090662828219,6.52070304371829,147.283323317171));
#45468=CARTESIAN_POINT('Ctrl Pts',(-1.98831342328973,6.4709737498157,147.292073314909));
#45469=CARTESIAN_POINT('Ctrl Pts',(-2.16550875682036,6.41384934062005,147.300823312647));
#45470=CARTESIAN_POINT('Ctrl Pts',(-2.34005036501476,6.34952386318803,147.309573310384));
#45471=CARTESIAN_POINT('Ctrl Pts',(-2.51458843336683,6.28519969032774,147.318323130665));
#45472=CARTESIAN_POINT('Ctrl Pts',(-2.68647261510021,6.21367484061042,147.327072950946));
#45473=CARTESIAN_POINT('Ctrl Pts',(-2.85511905703302,6.13519226839444,147.335822771227));
#45474=CARTESIAN_POINT('Ctrl Pts',(-3.02376230286066,6.05671118354192,147.344572425685));
#45475=CARTESIAN_POINT('Ctrl Pts',(-3.18916767179931,5.97127276099435,147.353322080144));
#45476=CARTESIAN_POINT('Ctrl Pts',(-3.35077333905882,5.8791672055022,147.362071734602));
#45477=CARTESIAN_POINT('Ctrl Pts',(-3.51237615843546,5.7870632731328,147.370821234871));
#45478=CARTESIAN_POINT('Ctrl Pts',(-3.67017916111784,5.68829258485222,147.379570735139));
#45479=CARTESIAN_POINT('Ctrl Pts',(-3.82364636379465,5.58319061869107,147.388320235408));
#45480=CARTESIAN_POINT('Ctrl Pts',(-3.97711106595286,5.47809036500931,147.397069593116));
#45481=CARTESIAN_POINT('Ctrl Pts',(-4.12623987302113,5.36665920181476,147.405818950825));
#45482=CARTESIAN_POINT('Ctrl Pts',(-4.27052628038016,5.24927559655448,147.414568308533));
#45483=CARTESIAN_POINT('Ctrl Pts',(-4.41481052852976,5.13189374791003,147.42331753531));
#45484=CARTESIAN_POINT('Ctrl Pts',(-4.5542522996864,5.00855981630014,147.432066762086));
#45485=CARTESIAN_POINT('Ctrl Pts',(-4.68837800466957,4.87969268349254,147.440815988863));
#45486=CARTESIAN_POINT('Ctrl Pts',(-4.82250188069621,4.75082730793486,147.449565096333));
#45487=CARTESIAN_POINT('Ctrl Pts',(-4.95130962898196,4.61642908069523,147.458314203804));
#45488=CARTESIAN_POINT('Ctrl Pts',(-5.07436378883271,4.47695444901814,147.467063311275));
#45489=CARTESIAN_POINT('Ctrl Pts',(-5.19741643417376,4.33748153394847,147.475812311065));
#45490=CARTESIAN_POINT('Ctrl Pts',(-5.31471544322182,4.19293255432793,147.484561310855));
#45491=CARTESIAN_POINT('Ctrl Pts',(-5.42586245140029,4.04379841961546,147.493310310644));
#45492=CARTESIAN_POINT('Ctrl Pts',(-5.53702159888527,3.89464799670051,147.502060265986));
#45493=CARTESIAN_POINT('Ctrl Pts',(-5.64202722955755,3.74091164633121,147.510810221329));
#45494=CARTESIAN_POINT('Ctrl Pts',(-5.7405226511274,3.58311159355849,147.519560176671));
#45495=CARTESIAN_POINT('Ctrl Pts',(-5.83901426951965,3.42531763387737,147.528309794153));
#45496=CARTESIAN_POINT('Ctrl Pts',(-5.930996030062,3.26346052894687,147.537059411636));
#45497=CARTESIAN_POINT('Ctrl Pts',(-6.01615550518748,3.09809004669044,147.545809029118));
#45498=CARTESIAN_POINT('Ctrl Pts',(-6.1013121448033,2.93272507068684,147.554558355269));
#45499=CARTESIAN_POINT('Ctrl Pts',(-6.17964682235935,2.76384720624411,147.56330768142));
#45500=CARTESIAN_POINT('Ctrl Pts',(-6.25089348201509,2.59203003001534,147.572057007571));
#45501=CARTESIAN_POINT('Ctrl Pts',(-6.32213814808036,2.42021766149385,147.580806088903));
#45502=CARTESIAN_POINT('Ctrl Pts',(-6.38629508337152,2.24546641046453,147.589555170234));
#45503=CARTESIAN_POINT('Ctrl Pts',(-6.44314639750321,2.0683697687651,147.598304251566));
#45504=CARTESIAN_POINT('Ctrl Pts',(-6.50000285220132,1.89125711376742,147.607054124));
#45505=CARTESIAN_POINT('Ctrl Pts',(-6.54955227615689,1.71179891660476,147.615803996435));
#45506=CARTESIAN_POINT('Ctrl Pts',(-6.59162635874899,1.53060476500157,147.624553868869));
#45507=CARTESIAN_POINT('Ctrl Pts',(-6.63369752009797,1.34942319387872,147.633303133791));
#45508=CARTESIAN_POINT('Ctrl Pts',(-6.66829431385002,1.1665061886708,147.642052398714));
#45509=CARTESIAN_POINT('Ctrl Pts',(-6.69529923712354,0.982474999871755,
147.650801663636));
#45510=CARTESIAN_POINT('Ctrl Pts',(-6.72230554704547,0.798434361441817,
147.659551377816));
#45511=CARTESIAN_POINT('Ctrl Pts',(-6.74171916476026,0.613279708512756,
147.668301091996));
#45512=CARTESIAN_POINT('Ctrl Pts',(-6.75347414802849,0.427639955933567,
147.677050806175));
#45513=CARTESIAN_POINT('Ctrl Pts',(-6.76248837677719,0.285283377755817,
147.68376046482));
#45514=CARTESIAN_POINT('Ctrl Pts',(-6.76699999923736,0.142641725985062,
147.690470123464));
#45515=CARTESIAN_POINT('Ctrl Pts',(-6.767,3.61801116239577E-8,147.697179782109));
#45516=CARTESIAN_POINT('',(-6.76699988085942,0.00126982229687558,147.302820216159));
#45517=CARTESIAN_POINT('Ctrl Pts',(3.09917575053262,6.01559628526637,146.651454788324));
#45518=CARTESIAN_POINT('Ctrl Pts',(2.94383551293841,6.095626040357,146.659651824689));
#45519=CARTESIAN_POINT('Ctrl Pts',(2.78537370919825,6.16964506113875,146.667848861055));
#45520=CARTESIAN_POINT('Ctrl Pts',(2.62429879734114,6.23741491503282,146.67604589742));
#45521=CARTESIAN_POINT('Ctrl Pts',(2.46321043893686,6.30519042635998,146.684243618075));
#45522=CARTESIAN_POINT('Ctrl Pts',(2.29950886843622,6.36671559218961,146.69244133873));
#45523=CARTESIAN_POINT('Ctrl Pts',(2.13372239599045,6.42180019440412,146.700639059385));
#45524=CARTESIAN_POINT('Ctrl Pts',(1.96789195217928,6.47689940664764,146.708838954312));
#45525=CARTESIAN_POINT('Ctrl Pts',(1.79997584528955,6.52555453960363,146.717038849239));
#45526=CARTESIAN_POINT('Ctrl Pts',(1.6305174559355,6.56762528056296,146.725238744166));
#45527=CARTESIAN_POINT('Ctrl Pts',(1.45862578677847,6.61030012194282,146.733556382681));
#45528=CARTESIAN_POINT('Ctrl Pts',(1.28514757403759,6.64619993402496,146.741874021196));
#45529=CARTESIAN_POINT('Ctrl Pts',(1.11065980228004,6.675232116084,146.750191659711));
#45530=CARTESIAN_POINT('Ctrl Pts',(0.938374859555118,6.70389778000326,146.75840429181));
#45531=CARTESIAN_POINT('Ctrl Pts',(0.765106062686008,6.72586821508305,146.766616923908));
#45532=CARTESIAN_POINT('Ctrl Pts',(0.591412879740036,6.74110671964757,146.774829556007));
#45533=CARTESIAN_POINT('Ctrl Pts',(0.414388444682558,6.75663748266257,146.78319969773));
#45534=CARTESIAN_POINT('Ctrl Pts',(0.236923576271659,6.76517546696643,146.791569839453));
#45535=CARTESIAN_POINT('Ctrl Pts',(0.0596090533561449,6.76673745321614,
146.799939981176));
#45536=CARTESIAN_POINT('Ctrl Pts',(-0.117705469559497,6.76829943946584,
146.808310122899));
#45537=CARTESIAN_POINT('Ctrl Pts',(-0.294869260590996,6.76288549758536,
146.816680264622));
#45538=CARTESIAN_POINT('Ctrl Pts',(-0.471298878222098,6.75056785517979,
146.825050406345));
#45539=CARTESIAN_POINT('Ctrl Pts',(-0.643142130747061,6.73857041527806,
146.833202962572));
#45540=CARTESIAN_POINT('Ctrl Pts',(-0.814795756546637,6.71998823285555,
146.841355518798));
#45541=CARTESIAN_POINT('Ctrl Pts',(-0.985710125587109,6.69482371301254,
146.849508075025));
#45542=CARTESIAN_POINT('Ctrl Pts',(-1.15642648621514,6.66968834687178,146.857651186319));
#45543=CARTESIAN_POINT('Ctrl Pts',(-1.32640493695681,6.63798587589216,146.865794297613));
#45544=CARTESIAN_POINT('Ctrl Pts',(-1.49509738735121,6.5997706628591,146.873937408907));
#45545=CARTESIAN_POINT('Ctrl Pts',(-1.66362986896612,6.56159168879803,146.882072798198));
#45546=CARTESIAN_POINT('Ctrl Pts',(-1.83087842402008,6.5169123484129,146.890208187489));
#45547=CARTESIAN_POINT('Ctrl Pts',(-1.99630161783497,6.46583860381849,146.89834357678));
#45548=CARTESIAN_POINT('Ctrl Pts',(-2.16160270246582,6.41480255994268,146.906472960832));
#45549=CARTESIAN_POINT('Ctrl Pts',(-2.32508076097357,6.35738161781102,146.914602344885));
#45550=CARTESIAN_POINT('Ctrl Pts',(-2.48620607010074,6.29373246785993,146.922731728937));
#45551=CARTESIAN_POINT('Ctrl Pts',(-2.64724628660119,6.23011693195363,146.930856819744));
#45552=CARTESIAN_POINT('Ctrl Pts',(-2.80593588901788,6.16027987283074,146.93898191055));
#45553=CARTESIAN_POINT('Ctrl Pts',(-2.96176180886218,6.08442733439766,146.947107001356));
#45554=CARTESIAN_POINT('Ctrl Pts',(-3.11818254958853,6.0082852505933,146.955263107373));
#45555=CARTESIAN_POINT('Ctrl Pts',(-3.27171734868893,5.92608178937322,146.963419213389));
#45556=CARTESIAN_POINT('Ctrl Pts',(-3.42186849673354,5.83807373977604,146.971575319406));
#45557=CARTESIAN_POINT('Ctrl Pts',(-3.57141531398624,5.75041990641363,146.979698598594));
#45558=CARTESIAN_POINT('Ctrl Pts',(-3.71760535988774,5.65700832756984,146.987821877781));
#45559=CARTESIAN_POINT('Ctrl Pts',(-3.859972841208,5.55813805740165,146.995945156969));
#45560=CARTESIAN_POINT('Ctrl Pts',(-4.00235927996356,5.45925462182005,147.00406951784));
#45561=CARTESIAN_POINT('Ctrl Pts',(-4.14092183978618,5.35491125581414,147.012193878712));
#45562=CARTESIAN_POINT('Ctrl Pts',(-4.27522504620788,5.24544943777717,147.020318239583));
#45563=CARTESIAN_POINT('Ctrl Pts',(-4.40957168811507,5.13595221829794,147.028445227983));
#45564=CARTESIAN_POINT('Ctrl Pts',(-4.53965595009455,5.02133348140751,147.036572216383));
#45565=CARTESIAN_POINT('Ctrl Pts',(-4.66507671893109,4.90197390920098,147.044699204784));
#45566=CARTESIAN_POINT('Ctrl Pts',(-4.79130831812865,4.78184269154912,147.052878733198));
#45567=CARTESIAN_POINT('Ctrl Pts',(-4.91281564503122,4.65690938727829,147.061058261612));
#45568=CARTESIAN_POINT('Ctrl Pts',(-5.02922924669246,4.52759783817128,147.069237790026));
#45569=CARTESIAN_POINT('Ctrl Pts',(-5.14509461975249,4.39889525819394,147.077378798444));
#45570=CARTESIAN_POINT('Ctrl Pts',(-5.2559139558375,4.26585590360896,147.085519806863));
#45571=CARTESIAN_POINT('Ctrl Pts',(-5.36136533585237,4.12892852148359,147.093660815281));
#45572=CARTESIAN_POINT('Ctrl Pts',(-5.46756514649457,3.99102931095266,147.101859603693));
#45573=CARTESIAN_POINT('Ctrl Pts',(-5.56832030529724,3.84918698802021,147.110058392105));
#45574=CARTESIAN_POINT('Ctrl Pts',(-5.66334819405037,3.70388663878181,147.118257180517));
#45575=CARTESIAN_POINT('Ctrl Pts',(-5.75837608280357,3.55858628954329,147.126455968929));
#45576=CARTESIAN_POINT('Ctrl Pts',(-5.84767656591252,3.40982826574327,147.134654757341));
#45577=CARTESIAN_POINT('Ctrl Pts',(-5.93101572523069,3.25811931443068,147.142853545753));
#45578=CARTESIAN_POINT('Ctrl Pts',(-6.02009273654493,3.09596529124274,147.151616815914));
#45579=CARTESIAN_POINT('Ctrl Pts',(-6.10260743088169,2.92998977387308,147.160380086075));
#45580=CARTESIAN_POINT('Ctrl Pts',(-6.17823994314578,2.76073182415788,147.169143356237));
#45581=CARTESIAN_POINT('Ctrl Pts',(-6.253739347016,2.59177175763023,147.177891203602));
#45582=CARTESIAN_POINT('Ctrl Pts',(-6.32238060641745,2.41954103964781,147.186639050967));
#45583=CARTESIAN_POINT('Ctrl Pts',(-6.38388932885875,2.24460375943804,147.195386898333));
#45584=CARTESIAN_POINT('Ctrl Pts',(-6.44683896903127,2.06556835754892,147.204339674818));
#45585=CARTESIAN_POINT('Ctrl Pts',(-6.50231761661049,1.88369826451708,147.213292451304));
#45586=CARTESIAN_POINT('Ctrl Pts',(-6.5500813497716,1.69962446186629,147.222245227789));
#45587=CARTESIAN_POINT('Ctrl Pts',(-6.59655721135478,1.52051391068235,147.230956607181));
#45588=CARTESIAN_POINT('Ctrl Pts',(-6.63572867129488,1.33931724643213,147.239667986573));
#45589=CARTESIAN_POINT('Ctrl Pts',(-6.66741942644637,1.1566361536134,147.248379365964));
#45590=CARTESIAN_POINT('Ctrl Pts',(-6.70042743386985,0.966361771098127,
147.257452840997));
#45591=CARTESIAN_POINT('Ctrl Pts',(-6.725319414712,0.774477178504855,147.266526316029));
#45592=CARTESIAN_POINT('Ctrl Pts',(-6.74195345813885,0.581680813066479,
147.275599791062));
#45593=CARTESIAN_POINT('Ctrl Pts',(-6.7585875015657,0.388884447627976,147.284673266094));
#45594=CARTESIAN_POINT('Ctrl Pts',(-6.76696349439261,0.195176652538027,
147.293746741127));
#45595=CARTESIAN_POINT('Ctrl Pts',(-6.76699988085942,0.0012698222966961,
147.302820216159));
#45596=CARTESIAN_POINT('Ctrl Pts',(-6.76699988085954,0.00126982163972021,
147.30282021619));
#45597=CARTESIAN_POINT('Ctrl Pts',(-6.76703393944407,-0.180231603618993,
147.311313205573));
#45598=CARTESIAN_POINT('Ctrl Pts',(-6.75976143043599,-0.361630771729502,
147.319806194955));
#45599=CARTESIAN_POINT('Ctrl Pts',(-6.74523311582971,-0.542327588376448,
147.328299184338));
#45600=CARTESIAN_POINT('Ctrl Pts',(-6.73069223038859,-0.723180755563819,
147.336799522402));
#45601=CARTESIAN_POINT('Ctrl Pts',(-6.70888303755105,-0.903330040991249,
147.345299860467));
#45602=CARTESIAN_POINT('Ctrl Pts',(-6.67990792922329,-1.0821825433354,147.353800198532));
#45603=CARTESIAN_POINT('Ctrl Pts',(-6.64955444747541,-1.26954322906799,
147.362704905751));
#45604=CARTESIAN_POINT('Ctrl Pts',(-6.61133672238485,-1.45548034105547,
147.37160961297));
#45605=CARTESIAN_POINT('Ctrl Pts',(-6.56543161974002,-1.63932810825592,
147.380514320189));
#45606=CARTESIAN_POINT('Ctrl Pts',(-6.52149101612976,-1.8153081496402,147.38903795237));
#45607=CARTESIAN_POINT('Ctrl Pts',(-6.4705074268006,-1.98937366922607,147.397561584551));
#45608=CARTESIAN_POINT('Ctrl Pts',(-6.41268614305828,-2.16095937736654,
147.406085216732));
#45609=CARTESIAN_POINT('Ctrl Pts',(-6.35480723427398,-2.33271608886416,
147.414617343617));
#45610=CARTESIAN_POINT('Ctrl Pts',(-6.29007714417336,-2.50198775953929,
147.423149470501));
#45611=CARTESIAN_POINT('Ctrl Pts',(-6.21874885537241,-2.66823006388211,
147.431681597386));
#45612=CARTESIAN_POINT('Ctrl Pts',(-6.14730614356766,-2.83473904984793,
147.440227411289));
#45613=CARTESIAN_POINT('Ctrl Pts',(-6.0692442182562,-2.99820867128655,147.448773225192));
#45614=CARTESIAN_POINT('Ctrl Pts',(-5.98486208498972,-3.15811887421175,
147.457319039094));
#45615=CARTESIAN_POINT('Ctrl Pts',(-5.97387667941093,-3.17893700676326,
147.458431587783));
#45616=CARTESIAN_POINT('Ctrl Pts',(-5.96278421573265,-3.19969485310094,
147.459544136472));
#45617=CARTESIAN_POINT('Ctrl Pts',(-5.95158540696316,-3.22039130287348,
147.460656685161));
#45618=CARTESIAN_POINT('Ctrl Pts',(-5.86455592316925,-3.38122995787209,
147.469302652788));
#45619=CARTESIAN_POINT('Ctrl Pts',(-5.77092524741157,-3.53868192027616,
147.477948620414));
#45620=CARTESIAN_POINT('Ctrl Pts',(-5.67097279947118,-3.69220212172331,
147.486594588041));
#45621=CARTESIAN_POINT('Ctrl Pts',(-5.57114820444209,-3.84552594974385,
147.495229496288));
#45622=CARTESIAN_POINT('Ctrl Pts',(-5.46501812760932,-3.99492779111802,
147.503864404535));
#45623=CARTESIAN_POINT('Ctrl Pts',(-5.35290746851323,-4.13988775615177,
147.512499312781));
#45624=CARTESIAN_POINT('Ctrl Pts',(-5.2370748484061,-4.28966024608161,147.521420891288));
#45625=CARTESIAN_POINT('Ctrl Pts',(-5.11485785024722,-4.43469056379052,
147.530342469795));
#45626=CARTESIAN_POINT('Ctrl Pts',(-4.9866647519595,-4.57443588342483,147.539264048302));
#45627=CARTESIAN_POINT('Ctrl Pts',(-4.86293345640356,-4.70931732148341,
147.54787510835));
#45628=CARTESIAN_POINT('Ctrl Pts',(-4.73363525331509,-4.83927517159217,
147.556486168397));
#45629=CARTESIAN_POINT('Ctrl Pts',(-4.59917969044027,-4.96385285590153,
147.565097228445));
#45630=CARTESIAN_POINT('Ctrl Pts',(-4.46485092571184,-5.08831305738522,
147.573700167844));
#45631=CARTESIAN_POINT('Ctrl Pts',(-4.32537472098508,-5.20740300223337,
147.582303107243));
#45632=CARTESIAN_POINT('Ctrl Pts',(-4.18119829727038,-5.32070200245262,
147.590906046641));
#45633=CARTESIAN_POINT('Ctrl Pts',(-4.03718331838328,-5.43387413354107,
147.599499352703));
#45634=CARTESIAN_POINT('Ctrl Pts',(-3.8884788596687,-5.54126806845471,147.608092658764));
#45635=CARTESIAN_POINT('Ctrl Pts',(-3.73556628575502,-5.64250241690072,
147.616685964826));
#45636=CARTESIAN_POINT('Ctrl Pts',(-3.71852941001364,-5.65378152215081,
147.617643394839));
#45637=CARTESIAN_POINT('Ctrl Pts',(-3.70144033134603,-5.66498420615577,
147.618600824852));
#45638=CARTESIAN_POINT('Ctrl Pts',(-3.68429974104188,-5.67610997234539,
147.619558254864));
#45639=CARTESIAN_POINT('Ctrl Pts',(-3.53041242883121,-5.7759965121217,147.628154010825));
#45640=CARTESIAN_POINT('Ctrl Pts',(-3.37255098090347,-5.8695626523731,147.636749766786));
#45641=CARTESIAN_POINT('Ctrl Pts',(-3.21125769516597,-5.95651853142735,
147.645345522747));
#45642=CARTESIAN_POINT('Ctrl Pts',(-3.04981391785115,-6.04355554298091,
147.653949298812));
#45643=CARTESIAN_POINT('Ctrl Pts',(-2.8849321801368,-6.12396983774937,147.662553074876));
#45644=CARTESIAN_POINT('Ctrl Pts',(-2.71717694824763,-6.1975187318726,147.671156850941));
#45645=CARTESIAN_POINT('Ctrl Pts',(-2.54282874066887,-6.27395818306215,
147.68009876541));
#45646=CARTESIAN_POINT('Ctrl Pts',(-2.36537695821387,-6.34298154504423,
147.689040679879));
#45647=CARTESIAN_POINT('Ctrl Pts',(-2.18547384835621,-6.40437296369841,
147.697982594348));
#45648=CARTESIAN_POINT('Ctrl Pts',(-2.0119024912119,-6.46360368995572,147.706609795017));
#45649=CARTESIAN_POINT('Ctrl Pts',(-1.83604971473384,-6.51573049723694,
147.715236995687));
#45650=CARTESIAN_POINT('Ctrl Pts',(-1.65851332944963,-6.56061144528754,
147.723864196357));
#45651=CARTESIAN_POINT('Ctrl Pts',(-1.48080786809786,-6.6055351355298,147.732499613107));
#45652=CARTESIAN_POINT('Ctrl Pts',(-1.30141589509124,-6.64319912676801,
147.741135029856));
#45653=CARTESIAN_POINT('Ctrl Pts',(-1.12094415059955,-6.67351280895127,
147.749770446606));
#45654=CARTESIAN_POINT('Ctrl Pts',(-0.940205784786006,-6.7038712752864,
147.758418620955));
#45655=CARTESIAN_POINT('Ctrl Pts',(-0.758384761661105,-6.72685769002199,
147.767066795305));
#45656=CARTESIAN_POINT('Ctrl Pts',(-0.576093150510847,-6.74243321672039,
147.775714969654));
#45657=CARTESIAN_POINT('Ctrl Pts',(-0.556807229401932,-6.74408106204492,
147.776629921292));
#45658=CARTESIAN_POINT('Ctrl Pts',(-0.537516040892551,-6.74564600519852,
147.77754487293));
#45659=CARTESIAN_POINT('Ctrl Pts',(-0.518220309308166,-6.74712803428396,
147.778459824568));
#45660=CARTESIAN_POINT('Ctrl Pts',(-0.344739502314164,-6.76045241126372,
147.78668581734));
#45661=CARTESIAN_POINT('Ctrl Pts',(-0.170516782363119,-6.76709922487563,
147.794911810112));
#45662=CARTESIAN_POINT('Ctrl Pts',(0.00389331571225554,-6.76699888001267,
147.803137802884));
#45663=CARTESIAN_POINT('Ctrl Pts',(0.178120567359625,-6.76689864034833,
147.811355171766));
#45664=CARTESIAN_POINT('Ctrl Pts',(0.352534450596516,-6.76006532841609,
147.819572540649));
#45665=CARTESIAN_POINT('Ctrl Pts',(0.526575400606224,-6.74648110850956,
147.827789909531));
#45666=CARTESIAN_POINT('Ctrl Pts',(0.700468716025642,-6.73290841175744,
147.836000307825));
#45667=CARTESIAN_POINT('Ctrl Pts',(0.873989373075183,-6.71259624010123,
147.844210706118));
#45668=CARTESIAN_POINT('Ctrl Pts',(1.04657779932796,-6.68557880141681,147.852421104412));
#45669=CARTESIAN_POINT('Ctrl Pts',(1.21905434759662,-6.65857887640143,147.860626180432));
#45670=CARTESIAN_POINT('Ctrl Pts',(1.39059951608976,-6.62488239767228,147.868831256452));
#45671=CARTESIAN_POINT('Ctrl Pts',(1.56065875125951,-6.58457540484708,147.877036332472));
#45672=CARTESIAN_POINT('Ctrl Pts',(1.73064175957193,-6.5442864791112,147.885237730673));
#45673=CARTESIAN_POINT('Ctrl Pts',(1.89913981362772,-6.49739302505692,147.893439128874));
#45674=CARTESIAN_POINT('Ctrl Pts',(2.0656083602185,-6.4440322083456,147.901640527075));
#45675=CARTESIAN_POINT('Ctrl Pts',(2.23206386758617,-6.39067557130431,147.909841282872));
#45676=CARTESIAN_POINT('Ctrl Pts',(2.39648984055659,-6.33085268162535,147.91804203867));
#45677=CARTESIAN_POINT('Ctrl Pts',(2.55835634539918,-6.26475073805461,147.926242794468));
#45678=CARTESIAN_POINT('Ctrl Pts',(2.7202220280246,-6.19864913025533,147.93444350861));
#45679=CARTESIAN_POINT('Ctrl Pts',(2.87952793624065,-6.12626866659616,147.942644222751));
#45680=CARTESIAN_POINT('Ctrl Pts',(3.03576371935655,-6.04784487567584,147.950844936892));
#45681=CARTESIAN_POINT('Ctrl Pts',(3.19202702266656,-5.96940727077575,147.959047095551));
#45682=CARTESIAN_POINT('Ctrl Pts',(3.34521880315717,-5.88492437854656,147.967249254209));
#45683=CARTESIAN_POINT('Ctrl Pts',(3.49485289058715,-5.79467792661116,147.975451412867));
#45684=CARTESIAN_POINT('Ctrl Pts',(3.64454045305823,-5.70439922311592,147.983656502748));
#45685=CARTESIAN_POINT('Ctrl Pts',(3.79066748304104,-5.6083530417684,147.991861592629));
#45686=CARTESIAN_POINT('Ctrl Pts',(3.93277635253836,-5.50686473058083,148.000066682509));
#45687=CARTESIAN_POINT('Ctrl Pts',(4.075047564563,-5.40526048103565,148.008281145732));
#45688=CARTESIAN_POINT('Ctrl Pts',(4.21329115361369,-5.29820188968842,148.016495608954));
#45689=CARTESIAN_POINT('Ctrl Pts',(4.34708135694208,-5.18605559902,148.024710072177));
#45690=CARTESIAN_POINT('Ctrl Pts',(4.48095082671527,-5.07384286523736,148.032929402208));
#45691=CARTESIAN_POINT('Ctrl Pts',(4.61036138616766,-4.95653666375602,148.041148732239));
#45692=CARTESIAN_POINT('Ctrl Pts',(4.73492389474723,-4.8345407962858,148.04936806227));
#45693=CARTESIAN_POINT('Ctrl Pts',(4.85967940531258,-4.71235590368316,148.05760012765));
#45694=CARTESIAN_POINT('Ctrl Pts',(4.97957160763023,-4.58546708439416,148.06583219303));
#45695=CARTESIAN_POINT('Ctrl Pts',(5.094250563344,-4.45431253931169,148.07406425841));
#45696=CARTESIAN_POINT('Ctrl Pts',(5.19733220223208,-4.33642146356397,148.081463826932));
#45697=CARTESIAN_POINT('Ctrl Pts',(5.29620213894733,-4.21508438956819,148.088863395454));
#45698=CARTESIAN_POINT('Ctrl Pts',(5.39063649034132,-4.09063897563701,148.096262963976));
#45699=CARTESIAN_POINT('Ctrl Pts',(5.49471763035978,-3.9534810414655,148.104418423467));
#45700=CARTESIAN_POINT('Ctrl Pts',(5.59373040297787,-3.81212447922415,148.112573882958));
#45701=CARTESIAN_POINT('Ctrl Pts',(5.68731290183461,-3.66698254108546,148.12072934245));
#45702=CARTESIAN_POINT('Ctrl Pts',(5.78078149854195,-3.522017259682,148.12887487568));
#45703=CARTESIAN_POINT('Ctrl Pts',(5.86883278182236,-3.37327607722917,148.137020408909));
#45704=CARTESIAN_POINT('Ctrl Pts',(5.95114476016919,-3.22120552643119,148.145165942139));
#45705=CARTESIAN_POINT('Ctrl Pts',(6.03337386261268,-3.06928808802974,148.15330327403));
#45706=CARTESIAN_POINT('Ctrl Pts',(6.10987499165739,-2.91404827390774,148.161440605921));
#45707=CARTESIAN_POINT('Ctrl Pts',(6.18036919521648,-2.75596183043583,148.169577937812));
#45708=CARTESIAN_POINT('Ctrl Pts',(6.25080723617763,-2.59800133413285,148.177708786706));
#45709=CARTESIAN_POINT('Ctrl Pts',(6.3152477324257,-2.43719905642263,148.1858396356));
#45710=CARTESIAN_POINT('Ctrl Pts',(6.37345747199705,-2.27405559576826,148.193970484495));
#45711=CARTESIAN_POINT('Ctrl Pts',(6.43163306393536,-2.11100784011223,148.202096563581));
#45712=CARTESIAN_POINT('Ctrl Pts',(6.4835850558457,-1.94562198001445,148.210222642668));
#45713=CARTESIAN_POINT('Ctrl Pts',(6.52912822500949,-1.77841885431537,148.218348721755));
#45714=CARTESIAN_POINT('Ctrl Pts',(6.57483287196891,-1.61062289345233,148.226503612656));
#45715=CARTESIAN_POINT('Ctrl Pts',(6.61408302073444,-1.44099709884985,148.234658503557));
#45716=CARTESIAN_POINT('Ctrl Pts',(6.64674171189912,-1.27008409772752,148.242813394458));
#45717=CARTESIAN_POINT('Ctrl Pts',(6.67927305267028,-1.09983756048281,148.250936485905));
#45718=CARTESIAN_POINT('Ctrl Pts',(6.70526419716062,-0.928314202450003,
148.259059577352));
#45719=CARTESIAN_POINT('Ctrl Pts',(6.72463089436373,-0.756061065370284,
148.267182668798));
#45720=CARTESIAN_POINT('Ctrl Pts',(6.74399911232347,-0.583794402231071,
148.275306398105));
#45721=CARTESIAN_POINT('Ctrl Pts',(6.7567418059398,-0.410798209435841,148.283430127412));
#45722=CARTESIAN_POINT('Ctrl Pts',(6.76282658223518,-0.237624953683721,
148.291553856719));
#45723=CARTESIAN_POINT('Ctrl Pts',(6.7689129939542,-0.0644051536344399,
148.299679769465));
#45724=CARTESIAN_POINT('Ctrl Pts',(6.76833791234505,0.108991438684712,148.307805682211));
#45725=CARTESIAN_POINT('Ctrl Pts',(6.76112107417796,0.282012092483061,148.315931594957));
#45726=CARTESIAN_POINT('Ctrl Pts',(6.75385808633422,0.456139165331137,148.324109470659));
#45727=CARTESIAN_POINT('Ctrl Pts',(6.73986811838416,0.629885099653434,148.332287346361));
#45728=CARTESIAN_POINT('Ctrl Pts',(6.71922421894785,0.802692279459984,148.340465222064));
#45729=CARTESIAN_POINT('Ctrl Pts',(6.69867884061792,0.97467475293634,148.348604069608));
#45730=CARTESIAN_POINT('Ctrl Pts',(6.67154302027316,1.14572706080913,148.356742917153));
#45731=CARTESIAN_POINT('Ctrl Pts',(6.6379399531208,1.31531067765859,148.364881764697));
#45732=CARTESIAN_POINT('Ctrl Pts',(6.60409518114556,1.48611409917312,148.373079154478));
#45733=CARTESIAN_POINT('Ctrl Pts',(6.56368986228207,1.65542725416067,148.381276544259));
#45734=CARTESIAN_POINT('Ctrl Pts',(6.51690055096956,1.82271671105869,148.38947393404));
#45735=CARTESIAN_POINT('Ctrl Pts',(6.47011123965706,1.99000616795671,148.397671323821));
#45736=CARTESIAN_POINT('Ctrl Pts',(6.416938108077,2.15527159113971,148.405868713602));
#45737=CARTESIAN_POINT('Ctrl Pts',(6.35760628504209,2.31800157989449,148.414066103384));
#45738=CARTESIAN_POINT('Ctrl Pts',(6.29805504077451,2.48133337747458,148.422293808791));
#45739=CARTESIAN_POINT('Ctrl Pts',(6.23212231044813,2.64259718578998,148.430521514198));
#45740=CARTESIAN_POINT('Ctrl Pts',(6.15997062115693,2.80125881461952,148.438749219605));
#45741=CARTESIAN_POINT('Ctrl Pts',(6.08790258433046,2.95973649160482,148.446967385834));
#45742=CARTESIAN_POINT('Ctrl Pts',(6.00963009503864,3.11561767361745,148.455185552063));
#45743=CARTESIAN_POINT('Ctrl Pts',(5.92536500898667,3.26838469435231,148.463403718292));
#45744=CARTESIAN_POINT('Ctrl Pts',(5.84119797321572,3.42097395642084,148.471612321918));
#45745=CARTESIAN_POINT('Ctrl Pts',(5.75105241082793,3.57045596734108,148.479820925545));
#45746=CARTESIAN_POINT('Ctrl Pts',(5.65518754507125,3.71633459608672,148.488029529171));
#45747=CARTESIAN_POINT('Ctrl Pts',(5.55938678915395,3.86211566817921,148.496232643276));
#45748=CARTESIAN_POINT('Ctrl Pts',(5.45787454183872,4.00429785801297,148.504435757381));
#45749=CARTESIAN_POINT('Ctrl Pts',(5.3509553530199,4.14241062788175,148.512638871486));
#45750=CARTESIAN_POINT('Ctrl Pts',(5.24408823251829,4.28045613854671,148.520837990776));
#45751=CARTESIAN_POINT('Ctrl Pts',(5.13181963362406,4.41443589324564,148.529037110066));
#45752=CARTESIAN_POINT('Ctrl Pts',(5.01449675683676,4.54390925037832,148.537236229356));
#45753=CARTESIAN_POINT('Ctrl Pts',(4.89720969107976,4.67334308773068,148.545432845989));
#45754=CARTESIAN_POINT('Ctrl Pts',(4.77487166154099,4.79827300251162,148.553629462623));
#45755=CARTESIAN_POINT('Ctrl Pts',(4.64786942653458,4.9182922639759,148.561826079256));
#45756=CARTESIAN_POINT('Ctrl Pts',(4.52085719900817,5.03832096854069,148.570023340798));
#45757=CARTESIAN_POINT('Ctrl Pts',(4.38918028835731,5.153437996135,148.57822060234));
#45758=CARTESIAN_POINT('Ctrl Pts',(4.25326179248185,5.26327399292627,148.586417863882));
#45759=CARTESIAN_POINT('Ctrl Pts',(4.11733958182613,5.3731129916386,148.594615349463));
#45760=CARTESIAN_POINT('Ctrl Pts',(3.97717583715614,5.47767045050518,148.602812835043));
#45761=CARTESIAN_POINT('Ctrl Pts',(3.83322589023906,5.57661799609772,148.611010320624));
#45762=CARTESIAN_POINT('Ctrl Pts',(3.68919908197937,5.67561837422939,148.619212183211));
#45763=CARTESIAN_POINT('Ctrl Pts',(3.54138233098872,5.76900265545213,148.627414045797));
#45764=CARTESIAN_POINT('Ctrl Pts',(3.39025952851201,5.85648609059507,148.635615908384));
#45765=CARTESIAN_POINT('Ctrl Pts',(3.29451541302883,5.91191137374175,148.640812212752));
#45766=CARTESIAN_POINT('Ctrl Pts',(3.19744483268801,5.96496902539041,148.646008517121));
#45767=CARTESIAN_POINT('Ctrl Pts',(3.09917575053258,6.01559628526639,148.651204821489));
#45768=CARTESIAN_POINT('Origin',(0.,0.,-3.69717978381041));
#45769=CARTESIAN_POINT('',(3.09917575053262,6.01559628526637,151.045614412788));
#45770=CARTESIAN_POINT('',(3.09917575053255,6.01559628526641,150.651392015123));
#45771=CARTESIAN_POINT('',(3.09917575053259,6.01559628526639,-3.69717978381041));
#45772=CARTESIAN_POINT('',(-6.76699997627813,0.000566614310235722,149.697179783767));
#45773=CARTESIAN_POINT('Ctrl Pts',(-6.76699997627821,0.000566613400196833,
149.69717978381));
#45774=CARTESIAN_POINT('Ctrl Pts',(-6.76700396482936,-0.0470682034863547,
149.699411627096));
#45775=CARTESIAN_POINT('Ctrl Pts',(-6.76650495248852,-0.094704481331748,
149.701643470382));
#45776=CARTESIAN_POINT('Ctrl Pts',(-6.76550302050593,-0.142330177844389,
149.703875313668));
#45777=CARTESIAN_POINT('Ctrl Pts',(-6.76164443078019,-0.325743849067885,
149.712470475538));
#45778=CARTESIAN_POINT('Ctrl Pts',(-6.75032524002114,-0.508892452664186,
149.721065637408));
#45779=CARTESIAN_POINT('Ctrl Pts',(-6.73161054280729,-0.691164596869533,
149.729660799278));
#45780=CARTESIAN_POINT('Ctrl Pts',(-6.7128783227168,-0.873607405460162,
149.738264008939));
#45781=CARTESIAN_POINT('Ctrl Pts',(-6.68673680573006,-1.05517181285975,
149.746867218599));
#45782=CARTESIAN_POINT('Ctrl Pts',(-6.65330256622685,-1.23525461433637,
149.75547042826));
#45783=CARTESIAN_POINT('Ctrl Pts',(-6.61848155058639,-1.42280684043653,
149.764430479471));
#45784=CARTESIAN_POINT('Ctrl Pts',(-6.57575002775779,-1.60875156095252,
149.773390530682));
#45785=CARTESIAN_POINT('Ctrl Pts',(-6.52529734598111,-1.79242393047288,
149.782350581893));
#45786=CARTESIAN_POINT('Ctrl Pts',(-6.47672146268755,-1.96926383812271,
149.790977326529));
#45787=CARTESIAN_POINT('Ctrl Pts',(-6.42098863317139,-2.14399713628271,
149.799604071166));
#45788=CARTESIAN_POINT('Ctrl Pts',(-6.35831760155604,-2.316049714005,149.808230815803));
#45789=CARTESIAN_POINT('Ctrl Pts',(-6.29558667263248,-2.48826672952273,
149.816865805378));
#45790=CARTESIAN_POINT('Ctrl Pts',(-6.22590441835218,-2.65779762737199,
149.825500794953));
#45791=CARTESIAN_POINT('Ctrl Pts',(-6.14953704952157,-2.82408977841738,
149.834135784528));
#45792=CARTESIAN_POINT('Ctrl Pts',(-6.07305625398113,-2.99062891939909,
149.842783599456));
#45793=CARTESIAN_POINT('Ctrl Pts',(-5.98987063636119,-3.15391942696104,
149.851431414384));
#45794=CARTESIAN_POINT('Ctrl Pts',(-5.90029221948735,-3.31343337410866,
149.860079229312));
#45795=CARTESIAN_POINT('Ctrl Pts',(-5.89023820993247,-3.33133673526112,
149.861049833805));
#45796=CARTESIAN_POINT('Ctrl Pts',(-5.88010371402478,-3.34919255304436,
149.862020438298));
#45797=CARTESIAN_POINT('Ctrl Pts',(-5.86988920644516,-3.36700010455281,
149.862991042791));
#45798=CARTESIAN_POINT('Ctrl Pts',(-5.78333435411803,-3.51789626661514,
149.871215671137));
#45799=CARTESIAN_POINT('Ctrl Pts',(-5.69084309843223,-3.66565158696293,
149.879440299483));
#45800=CARTESIAN_POINT('Ctrl Pts',(-5.59266957079819,-3.80976850633578,
149.887664927829));
#45801=CARTESIAN_POINT('Ctrl Pts',(-5.49459923989674,-3.95373393481747,
149.895880910721));
#45802=CARTESIAN_POINT('Ctrl Pts',(-5.39085873155815,-4.09406828460298,
149.904096893612));
#45803=CARTESIAN_POINT('Ctrl Pts',(-5.28174781080178,-4.23029893306497,
149.912312876503));
#45804=CARTESIAN_POINT('Ctrl Pts',(-5.17272972786479,-4.3664136686903,149.920521868766));
#45805=CARTESIAN_POINT('Ctrl Pts',(-5.05835055591938,-4.49843137887082,
149.928730861029));
#45806=CARTESIAN_POINT('Ctrl Pts',(-4.9389531043467,-4.62590869268559,149.936939853291));
#45807=CARTESIAN_POINT('Ctrl Pts',(-4.81963333329541,-4.7533030691841,149.945143504747));
#45808=CARTESIAN_POINT('Ctrl Pts',(-4.69530203017841,-4.87616267276169,
149.953347156202));
#45809=CARTESIAN_POINT('Ctrl Pts',(-4.56634204662254,-4.99407742363363,
149.961550807657));
#45810=CARTESIAN_POINT('Ctrl Pts',(-4.43744014567412,-5.1119390665879,149.969750764249));
#45811=CARTESIAN_POINT('Ctrl Pts',(-4.30391398159691,-5.22486005251954,
149.977950720842));
#45812=CARTESIAN_POINT('Ctrl Pts',(-4.16618306273024,-5.33246731708875,
149.986150677434));
#45813=CARTESIAN_POINT('Ctrl Pts',(-4.02846316007205,-5.44006597484643,
149.994349978164));
#45814=CARTESIAN_POINT('Ctrl Pts',(-3.88653944934674,-5.54235153041358,
150.002549278895));
#45815=CARTESIAN_POINT('Ctrl Pts',(-3.74086459358734,-5.63899114136959,
150.010748579625));
#45816=CARTESIAN_POINT('Ctrl Pts',(-3.59519068936305,-5.7356301210843,150.018947826799));
#45817=CARTESIAN_POINT('Ctrl Pts',(-3.44576598706677,-5.82662303054573,
150.027147073972));
#45818=CARTESIAN_POINT('Ctrl Pts',(-3.29307210356225,-5.91168039737773,
150.035346321146));
#45819=CARTESIAN_POINT('Ctrl Pts',(-3.14035151623339,-5.996752639442,150.043547002242));
#45820=CARTESIAN_POINT('Ctrl Pts',(-2.98436092183173,-6.07588709629209,
150.051747683339));
#45821=CARTESIAN_POINT('Ctrl Pts',(-2.82560654218276,-6.14884027022771,
150.059948364435));
#45822=CARTESIAN_POINT('Ctrl Pts',(-2.66679559782668,-6.22181943761892,
150.068151967461));
#45823=CARTESIAN_POINT('Ctrl Pts',(-2.50521923212617,-6.28861278517178,
150.076355570487));
#45824=CARTESIAN_POINT('Ctrl Pts',(-2.34140368498817,-6.34902494749578,
150.084559173513));
#45825=CARTESIAN_POINT('Ctrl Pts',(-2.1774004699578,-6.40950631828855,150.092772174627));
#45826=CARTESIAN_POINT('Ctrl Pts',(-2.01115328531376,-6.46359177480447,
150.100985175741));
#45827=CARTESIAN_POINT('Ctrl Pts',(-1.84320460156978,-6.51113552283717,
150.109198176854));
#45828=CARTESIAN_POINT('Ctrl Pts',(-1.67515653678631,-6.5587074041484,150.117416037885));
#45829=CARTESIAN_POINT('Ctrl Pts',(-1.50540531381688,-6.59972977664111,
150.125633898915));
#45830=CARTESIAN_POINT('Ctrl Pts',(-1.3345035309375,-6.63410802790514,150.133851759945));
#45831=CARTESIAN_POINT('Ctrl Pts',(-1.16333518430878,-6.66853990058492,
150.14208243877));
#45832=CARTESIAN_POINT('Ctrl Pts',(-0.991013045163549,-6.69630688502552,
150.150313117594));
#45833=CARTESIAN_POINT('Ctrl Pts',(-0.818096122069102,-6.71736613078783,
150.158543796418));
#45834=CARTESIAN_POINT('Ctrl Pts',(-0.659278447110338,-6.73670825409481,
150.166103364625));
#45835=CARTESIAN_POINT('Ctrl Pts',(-0.499959279506673,-6.75039250432336,
150.173662932831));
#45836=CARTESIAN_POINT('Ctrl Pts',(-0.340570660280462,-6.75842441885356,
150.181222501038));
#45837=CARTESIAN_POINT('Ctrl Pts',(-0.168647099917588,-6.76708799439156,
150.1893765831));
#45838=CARTESIAN_POINT('Ctrl Pts',(0.00388881049175518,-6.7692012821825,
150.197530665162));
#45839=CARTESIAN_POINT('Ctrl Pts',(0.176491945955157,-6.76469804152506,
150.205684747223));
#45840=CARTESIAN_POINT('Ctrl Pts',(0.348884466162331,-6.76020029584998,
150.213828879442));
#45841=CARTESIAN_POINT('Ctrl Pts',(0.521343686668807,-6.74910210203667,
150.221973011661));
#45842=CARTESIAN_POINT('Ctrl Pts',(0.693319462283189,-6.73138894458041,
150.23011714388));
#45843=CARTESIAN_POINT('Ctrl Pts',(0.865121581854534,-6.71369367334575,
150.238253052396));
#45844=CARTESIAN_POINT('Ctrl Pts',(1.03644086740629,-6.68939677341782,150.246388960911));
#45845=CARTESIAN_POINT('Ctrl Pts',(1.20672727565984,-6.65853574610654,150.254524869427));
#45846=CARTESIAN_POINT('Ctrl Pts',(1.37687754983429,-6.62769939039164,150.262654273756));
#45847=CARTESIAN_POINT('Ctrl Pts',(1.54599623272606,-6.59030942079538,150.270783678086));
#45848=CARTESIAN_POINT('Ctrl Pts',(1.71353850991623,-6.54645513045297,150.278913082416));
#45849=CARTESIAN_POINT('Ctrl Pts',(1.88098207103713,-6.5026266791002,150.287037696893));
#45850=CARTESIAN_POINT('Ctrl Pts',(2.0468507233365,-6.45234158439991,150.29516231137));
#45851=CARTESIAN_POINT('Ctrl Pts',(2.21060996053383,-6.3957401919081,150.303286925847));
#45852=CARTESIAN_POINT('Ctrl Pts',(2.37535707894493,-6.33879735026647,150.31146055224));
#45853=CARTESIAN_POINT('Ctrl Pts',(2.53796888007013,-6.27546182363841,150.319634178634));
#45854=CARTESIAN_POINT('Ctrl Pts',(2.69791614876294,-6.2059276062684,150.327807805027));
#45855=CARTESIAN_POINT('Ctrl Pts',(2.85684515792853,-6.13683605903512,150.335929396315));
#45856=CARTESIAN_POINT('Ctrl Pts',(3.01314313174157,-6.06162468484079,150.344050987603));
#45857=CARTESIAN_POINT('Ctrl Pts',(3.16631085115103,-5.98053213300316,150.352172578891));
#45858=CARTESIAN_POINT('Ctrl Pts',(3.31949039946434,-5.89943331851433,150.360294797397));
#45859=CARTESIAN_POINT('Ctrl Pts',(3.46953888837857,-5.81245259286801,150.368417015903));
#45860=CARTESIAN_POINT('Ctrl Pts',(3.61598184378114,-5.71987450084747,150.376539234409));
#45861=CARTESIAN_POINT('Ctrl Pts',(3.76246399203482,-5.62727163194801,150.384663626682));
#45862=CARTESIAN_POINT('Ctrl Pts',(3.90533837616407,-5.52906860929183,150.392788018955));
#45863=CARTESIAN_POINT('Ctrl Pts',(4.04415968501874,-5.4255931880366,150.400912411228));
#45864=CARTESIAN_POINT('Ctrl Pts',(4.18447445378208,-5.32100456309202,150.4091242069));
#45865=CARTESIAN_POINT('Ctrl Pts',(4.32064812564791,-5.21102966677564,150.417336002571));
#45866=CARTESIAN_POINT('Ctrl Pts',(4.45225600858948,-5.096048021161,150.425547798243));
#45867=CARTESIAN_POINT('Ctrl Pts',(4.58267093414513,-4.98210862469067,150.433685158234));
#45868=CARTESIAN_POINT('Ctrl Pts',(4.7086022792593,-4.86325316794276,150.441822518225));
#45869=CARTESIAN_POINT('Ctrl Pts',(4.82967494894583,-4.73988701210536,150.449959878216));
#45870=CARTESIAN_POINT('Ctrl Pts',(4.95240886869547,-4.61482813705478,150.458208891727));
#45871=CARTESIAN_POINT('Ctrl Pts',(5.07014954707028,-4.48513416966097,150.466457905239));
#45872=CARTESIAN_POINT('Ctrl Pts',(5.18254967333258,-4.35126049363175,150.47470691875));
#45873=CARTESIAN_POINT('Ctrl Pts',(5.29494979959488,-4.21738681760252,150.482955932262));
#45874=CARTESIAN_POINT('Ctrl Pts',(5.40200918801733,-4.07933377557342,150.491204945774));
#45875=CARTESIAN_POINT('Ctrl Pts',(5.50342733123436,-3.93758512413671,150.499453959285));
#45876=CARTESIAN_POINT('Ctrl Pts',(5.60454655662779,-3.79625425986352,150.507678659818));
#45877=CARTESIAN_POINT('Ctrl Pts',(5.70036008965199,-3.65082725855684,150.515903360351));
#45878=CARTESIAN_POINT('Ctrl Pts',(5.79051899991666,-3.50173938373548,150.524128060883));
#45879=CARTESIAN_POINT('Ctrl Pts',(5.88057634176751,-3.35281946368334,150.532343495889));
#45880=CARTESIAN_POINT('Ctrl Pts',(5.96499156158994,-3.20024718656367,150.540558930896));
#45881=CARTESIAN_POINT('Ctrl Pts',(6.04345714430163,-3.04448924205516,150.548774365902));
#45882=CARTESIAN_POINT('Ctrl Pts',(6.12185009874917,-2.8888754681339,150.556982196647));
#45883=CARTESIAN_POINT('Ctrl Pts',(6.19430422302675,-2.73008221757033,150.565190027391));
#45884=CARTESIAN_POINT('Ctrl Pts',(6.26055630029154,-2.56860347482438,150.573397858136));
#45885=CARTESIAN_POINT('Ctrl Pts',(6.32676036273262,-2.40724176045984,150.581599740426));
#45886=CARTESIAN_POINT('Ctrl Pts',(6.38677119532312,-2.24319876107158,150.589801622715));
#45887=CARTESIAN_POINT('Ctrl Pts',(6.4403723410656,-2.07699135974064,150.598003505004));
#45888=CARTESIAN_POINT('Ctrl Pts',(6.49394540526051,-1.91087103417984,150.606201090341));
#45889=CARTESIAN_POINT('Ctrl Pts',(6.54111536246229,-1.74258890629774,150.614398675679));
#45890=CARTESIAN_POINT('Ctrl Pts',(6.58171453172264,-1.57268014005107,150.622596261016));
#45891=CARTESIAN_POINT('Ctrl Pts',(6.62230596857683,-1.40280373416089,150.630792285064));
#45892=CARTESIAN_POINT('Ctrl Pts',(6.6563290208704,-1.23130165416054,150.638988309111));
#45893=CARTESIAN_POINT('Ctrl Pts',(6.68366629150933,-1.05872277001204,150.647184333159));
#45894=CARTESIAN_POINT('Ctrl Pts',(6.71100154442281,-0.886156623667957,
150.65537975227));
#45895=CARTESIAN_POINT('Ctrl Pts',(6.73165194140962,-0.712514185737677,
150.66357517138));
#45896=CARTESIAN_POINT('Ctrl Pts',(6.74555150261371,-0.538352974902165,
150.671770590491));
#45897=CARTESIAN_POINT('Ctrl Pts',(6.7594525670483,-0.364172928619752,150.679966895932));
#45898=CARTESIAN_POINT('Ctrl Pts',(6.76660131256587,-0.189474355435032,
150.688163201373));
#45899=CARTESIAN_POINT('Ctrl Pts',(6.76698377532349,-0.0148183841432244,
150.696359506814));
#45900=CARTESIAN_POINT('Ctrl Pts',(6.76736634903676,0.159888256305075,150.704558190072));
#45901=CARTESIAN_POINT('Ctrl Pts',(6.7609787292514,0.334551911487722,150.71275687333));
#45902=CARTESIAN_POINT('Ctrl Pts',(6.74785906062422,0.508612915635836,150.720955556588));
#45903=CARTESIAN_POINT('Ctrl Pts',(6.73472568236196,0.682855807979336,150.729162807208));
#45904=CARTESIAN_POINT('Ctrl Pts',(6.71484622770233,0.856494432818047,150.737370057828));
#45905=CARTESIAN_POINT('Ctrl Pts',(6.68831070415793,1.02897469582418,150.745577308449));
#45906=CARTESIAN_POINT('Ctrl Pts',(6.66176096118246,1.20154738478935,150.753788957039));
#45907=CARTESIAN_POINT('Ctrl Pts',(6.62854810712325,1.37296012253397,150.762000605629));
#45908=CARTESIAN_POINT('Ctrl Pts',(6.58881298834815,1.5426705431085,150.770212254219));
#45909=CARTESIAN_POINT('Ctrl Pts',(6.54901935243595,1.71263089292084,150.778435995945));
#45910=CARTESIAN_POINT('Ctrl Pts',(6.50268435133856,1.88088356948477,150.78665973767));
#45911=CARTESIAN_POINT('Ctrl Pts',(6.4499986631602,2.0469016207995,150.794883479395));
#45912=CARTESIAN_POINT('Ctrl Pts',(6.4013048591865,2.20034083221205,150.802484125441));
#45913=CARTESIAN_POINT('Ctrl Pts',(6.3471868848032,2.35187120945674,150.810084771486));
#45914=CARTESIAN_POINT('Ctrl Pts',(6.28783096916308,2.50109390132272,150.817685417532));
#45915=CARTESIAN_POINT('Ctrl Pts',(6.22358991167221,2.66259799781795,150.825911615954));
#45916=CARTESIAN_POINT('Ctrl Pts',(6.15303221576947,2.82185231328987,150.834137814376));
#45917=CARTESIAN_POINT('Ctrl Pts',(6.07633550844756,2.97832768324431,150.842364012798));
#45918=CARTESIAN_POINT('Ctrl Pts',(5.99737722358098,3.13941708677773,150.850832779464));
#45919=CARTESIAN_POINT('Ctrl Pts',(5.91191238708636,3.29756077071774,150.859301546131));
#45920=CARTESIAN_POINT('Ctrl Pts',(5.82018977794054,3.45219929157581,150.867770312797));
#45921=CARTESIAN_POINT('Ctrl Pts',(5.73130494264953,3.60205350510196,150.875977067241));
#45922=CARTESIAN_POINT('Ctrl Pts',(5.6365439549662,3.7486158563877,150.884183821685));
#45923=CARTESIAN_POINT('Ctrl Pts',(5.53618142010418,3.89139875670603,150.89239057613));
#45924=CARTESIAN_POINT('Ctrl Pts',(5.43588628825688,4.0340857646882,150.900591818955));
#45925=CARTESIAN_POINT('Ctrl Pts',(5.32999730572402,4.17299808375075,150.908793061781));
#45926=CARTESIAN_POINT('Ctrl Pts',(5.21883357252479,4.30767514354183,150.916994304607));
#45927=CARTESIAN_POINT('Ctrl Pts',(5.1077242642446,4.44228626646785,150.925191532167));
#45928=CARTESIAN_POINT('Ctrl Pts',(4.99134557668544,4.57266598397942,150.933388759727));
#45929=CARTESIAN_POINT('Ctrl Pts',(4.87005829085282,4.69838496120696,150.941585987286));
#45930=CARTESIAN_POINT('Ctrl Pts',(4.74880831326354,4.82406526699287,150.94978069336));
#45931=CARTESIAN_POINT('Ctrl Pts',(4.62265299463237,4.94508743108714,150.957975399434));
#45932=CARTESIAN_POINT('Ctrl Pts',(4.49199157550546,5.0610572695424,150.966170105508));
#45933=CARTESIAN_POINT('Ctrl Pts',(4.36132600684613,5.17703079095632,150.974365071829));
#45934=CARTESIAN_POINT('Ctrl Pts',(4.22615431604807,5.28795142348739,150.98256003815));
#45935=CARTESIAN_POINT('Ctrl Pts',(4.08691081441889,5.3934635434928,150.99075500447));
#45936=CARTESIAN_POINT('Ctrl Pts',(3.94766332851582,5.49897868259197,150.998950205279));
#45937=CARTESIAN_POINT('Ctrl Pts',(3.80434408879023,5.59908478839752,151.007145406088));
#45938=CARTESIAN_POINT('Ctrl Pts',(3.65741831470865,5.69346821113755,151.015340606898));
#45939=CARTESIAN_POINT('Ctrl Pts',(3.51043154852579,5.7878908145,151.023539209714));
#45940=CARTESIAN_POINT('Ctrl Pts',(3.35983556333475,5.87658580209414,151.03173781253));
#45941=CARTESIAN_POINT('Ctrl Pts',(3.2061225495812,5.95928411783387,151.039936415346));
#45942=CARTESIAN_POINT('Ctrl Pts',(3.17063755624633,5.97837520915509,151.04182908116));
#45943=CARTESIAN_POINT('Ctrl Pts',(3.13498654744956,5.9971469166337,151.043721746974));
#45944=CARTESIAN_POINT('Ctrl Pts',(3.09917575053262,6.01559628526637,151.045614412788));
#45945=CARTESIAN_POINT('Ctrl Pts',(3.09917575053273,6.01559628526631,149.045786479356));
#45946=CARTESIAN_POINT('Ctrl Pts',(2.94512620286167,6.09496108966518,149.053908071751));
#45947=CARTESIAN_POINT('Ctrl Pts',(2.78799803146464,6.16841903677227,149.062029664145));
#45948=CARTESIAN_POINT('Ctrl Pts',(2.6282914520702,6.23573356093529,149.070151256539));
#45949=CARTESIAN_POINT('Ctrl Pts',(2.4685751060542,6.30305220161929,149.078273345598));
#45950=CARTESIAN_POINT('Ctrl Pts',(2.30628037506223,6.36422652839151,149.086395434656));
#45951=CARTESIAN_POINT('Ctrl Pts',(2.14192748660438,6.41906812879632,149.094517523714));
#45952=CARTESIAN_POINT('Ctrl Pts',(1.97753325073724,6.47392352608732,149.102641656104));
#45953=CARTESIAN_POINT('Ctrl Pts',(1.81108017339957,6.52244290859249,149.110765788493));
#45954=CARTESIAN_POINT('Ctrl Pts',(1.64310362371349,6.56448775471016,149.118889920882));
#45955=CARTESIAN_POINT('Ctrl Pts',(1.47505282556408,6.60655118535775,149.127017644275));
#45956=CARTESIAN_POINT('Ctrl Pts',(1.30547756869858,6.64213429208963,149.135145367667));
#45957=CARTESIAN_POINT('Ctrl Pts',(1.13492334272837,6.67114967648982,149.14327309106));
#45958=CARTESIAN_POINT('Ctrl Pts',(0.964166382420434,6.700199550887,149.151410475712));
#45959=CARTESIAN_POINT('Ctrl Pts',(0.792428489986612,6.72266605231141,149.159547860364));
#45960=CARTESIAN_POINT('Ctrl Pts',(0.620261075322537,6.73851357485015,149.167685245016));
#45961=CARTESIAN_POINT('Ctrl Pts',(0.447975890638217,6.75437193778545,149.175828195994));
#45962=CARTESIAN_POINT('Ctrl Pts',(0.275260962282223,6.76360228215639,149.183971146972));
#45963=CARTESIAN_POINT('Ctrl Pts',(0.102667306064882,6.76622113326674,149.19211409795));
#45964=CARTESIAN_POINT('Ctrl Pts',(-0.070176194071899,6.76884377538563,
149.200268836538));
#45965=CARTESIAN_POINT('Ctrl Pts',(-0.24289770757871,6.76483582292493,149.208423575127));
#45966=CARTESIAN_POINT('Ctrl Pts',(-0.414950837277496,6.75426567456764,
149.216578313715));
#45967=CARTESIAN_POINT('Ctrl Pts',(-0.484926364438568,6.7499667018912,149.21989491791));
#45968=CARTESIAN_POINT('Ctrl Pts',(-0.554791444068832,6.74458285327622,
149.223211522104));
#45969=CARTESIAN_POINT('Ctrl Pts',(-0.624509858585915,6.7381211354894,149.226528126298));
#45970=CARTESIAN_POINT('Ctrl Pts',(-0.797549664132813,6.72208327236423,
149.234759876099));
#45971=CARTESIAN_POINT('Ctrl Pts',(-0.97022531043997,6.69935190517954,149.2429916259));
#45972=CARTESIAN_POINT('Ctrl Pts',(-1.14197910143897,6.66994548192687,149.251223375702));
#45973=CARTESIAN_POINT('Ctrl Pts',(-1.31352780205097,6.6405741727447,149.25944529601));
#45974=CARTESIAN_POINT('Ctrl Pts',(-1.48415648957198,6.60454373877506,149.267667216317));
#45975=CARTESIAN_POINT('Ctrl Pts',(-1.65331051605781,6.56192451476643,149.275889136625));
#45976=CARTESIAN_POINT('Ctrl Pts',(-1.8222964485577,6.51934764289916,149.284102886537));
#45977=CARTESIAN_POINT('Ctrl Pts',(-1.98981029334086,6.47019510725002,149.292316636449));
#45978=CARTESIAN_POINT('Ctrl Pts',(-2.1553054588549,6.41458863677401,149.300530386361));
#45979=CARTESIAN_POINT('Ctrl Pts',(-2.32066931320966,6.35902628692279,149.308737619122));
#45980=CARTESIAN_POINT('Ctrl Pts',(-2.48401734042951,6.29702031544894,149.316944851883));
#45981=CARTESIAN_POINT('Ctrl Pts',(-2.6448159412813,6.22874286166513,149.325152084644));
#45982=CARTESIAN_POINT('Ctrl Pts',(-2.8055191552641,6.16050591055053,149.333354448816));
#45983=CARTESIAN_POINT('Ctrl Pts',(-2.96367562670376,6.08600502804842,149.341556812988));
#45984=CARTESIAN_POINT('Ctrl Pts',(-3.11876956394421,6.00546129843622,149.34975917716));
#45985=CARTESIAN_POINT('Ctrl Pts',(-3.27381721439687,5.92494160658195,149.357959093389));
#45986=CARTESIAN_POINT('Ctrl Pts',(-3.4258038319085,5.83838282150255,149.366159009619));
#45987=CARTESIAN_POINT('Ctrl Pts',(-3.57423594106801,5.74605311823496,149.374358925848));
#45988=CARTESIAN_POINT('Ctrl Pts',(-3.72264729859076,5.65373632317486,149.382557695683));
#45989=CARTESIAN_POINT('Ctrl Pts',(-3.86750483280932,5.55565040534534,149.390756465519));
#45990=CARTESIAN_POINT('Ctrl Pts',(-4.00834189494613,5.45210823931621,149.398955235354));
#45991=CARTESIAN_POINT('Ctrl Pts',(-4.14918481625368,5.34856176567642,149.407154346278));
#45992=CARTESIAN_POINT('Ctrl Pts',(-4.28600664340828,5.23955880387085,149.415353457203));
#45993=CARTESIAN_POINT('Ctrl Pts',(-4.41837177039249,5.12545411632948,149.423552568127));
#45994=CARTESIAN_POINT('Ctrl Pts',(-4.55076641610839,5.01132398231489,149.431753507535));
#45995=CARTESIAN_POINT('Ctrl Pts',(-4.67870211068835,4.89209009050625,149.439954446942));
#45996=CARTESIAN_POINT('Ctrl Pts',(-4.80177820549031,4.76814587290262,149.448155386349));
#45997=CARTESIAN_POINT('Ctrl Pts',(-4.9249696591013,4.64408548280138,149.456364012469));
#45998=CARTESIAN_POINT('Ctrl Pts',(-5.04329215966144,4.51530620073256,149.464572638589));
#45999=CARTESIAN_POINT('Ctrl Pts',(-5.15638302138738,4.38223722962917,149.472781264709));
#46000=CARTESIAN_POINT('Ctrl Pts',(-5.26952787890707,4.24910472408447,149.480993810079));
#46001=CARTESIAN_POINT('Ctrl Pts',(-5.37743589602003,4.11167872763715,149.489206355448));
#46002=CARTESIAN_POINT('Ctrl Pts',(-5.4797863068807,3.97041950314104,149.497418900818));
#46003=CARTESIAN_POINT('Ctrl Pts',(-5.58227716442797,3.82896644073198,149.505642715558));
#46004=CARTESIAN_POINT('Ctrl Pts',(-5.67919497535735,3.68366993616677,149.513866530299));
#46005=CARTESIAN_POINT('Ctrl Pts',(-5.77026307927509,3.53501810404909,149.52209034504));
#46006=CARTESIAN_POINT('Ctrl Pts',(-5.8539405746149,3.39843007317805,149.529646758208));
#46007=CARTESIAN_POINT('Ctrl Pts',(-5.9326797234281,3.25900969930774,149.537203171376));
#46008=CARTESIAN_POINT('Ctrl Pts',(-6.0063013658658,3.11715140832116,149.544759584544));
#46009=CARTESIAN_POINT('Ctrl Pts',(-6.09117194522075,2.95361803764797,149.553470571453));
#46010=CARTESIAN_POINT('Ctrl Pts',(-6.16943201730198,2.78647759071529,149.562181558361));
#46011=CARTESIAN_POINT('Ctrl Pts',(-6.24078436680482,2.61627588129475,149.570892545269));
#46012=CARTESIAN_POINT('Ctrl Pts',(-6.31203988881782,2.44630514120322,149.579591711081));
#46013=CARTESIAN_POINT('Ctrl Pts',(-6.37640626983225,2.27328169467997,149.588290876892));
#46014=CARTESIAN_POINT('Ctrl Pts',(-6.43363275134785,2.09777468303541,149.596990042704));
#46015=CARTESIAN_POINT('Ctrl Pts',(-6.49075166015386,1.92259758447119,149.605672856072));
#46016=CARTESIAN_POINT('Ctrl Pts',(-6.54075736032535,1.74494651626455,149.61435566944));
#46017=CARTESIAN_POINT('Ctrl Pts',(-6.5834477071965,1.56540898381516,149.623038482807));
#46018=CARTESIAN_POINT('Ctrl Pts',(-6.62608942416789,1.38607596814402,149.631711405313));
#46019=CARTESIAN_POINT('Ctrl Pts',(-6.66143233574533,1.20486105875168,149.640384327818));
#46020=CARTESIAN_POINT('Ctrl Pts',(-6.68932389964516,1.02236723619061,149.649057250324));
#46021=CARTESIAN_POINT('Ctrl Pts',(-6.71717092613002,0.840164820849831,
149.657716323855));
#46022=CARTESIAN_POINT('Ctrl Pts',(-6.73759030209038,0.656687857839354,
149.666375397386));
#46023=CARTESIAN_POINT('Ctrl Pts',(-6.75048041214476,0.472549685482899,
149.675034470918));
#46024=CARTESIAN_POINT('Ctrl Pts',(-6.7614690981279,0.315573791173186,149.682416241867));
#46025=CARTESIAN_POINT('Ctrl Pts',(-6.76698678421464,0.158117688653368,
149.689798012817));
#46026=CARTESIAN_POINT('Ctrl Pts',(-6.76699997627813,0.000566614310398829,
149.697179783767));
#46027=CARTESIAN_POINT('',(-6.767,9.01944948036252E-12,149.30282021619));
#46028=CARTESIAN_POINT('Ctrl Pts',(3.09917575053258,6.01559628526639,148.651204821489));
#46029=CARTESIAN_POINT('Ctrl Pts',(2.94388516761211,6.09560045875987,148.659416327252));
#46030=CARTESIAN_POINT('Ctrl Pts',(2.78560087384593,6.16953292422705,148.667627833014));
#46031=CARTESIAN_POINT('Ctrl Pts',(2.62484376789698,6.23718559882039,148.675839338777));
#46032=CARTESIAN_POINT('Ctrl Pts',(2.46398377506222,6.30488157210938,148.684056100022));
#46033=CARTESIAN_POINT('Ctrl Pts',(2.30064815032346,6.36628961790689,148.692272861268));
#46034=CARTESIAN_POINT('Ctrl Pts',(2.13537375161274,6.4212512753297,148.700489622514));
#46035=CARTESIAN_POINT('Ctrl Pts',(1.96988497674041,6.47628422309903,148.708717041658));
#46036=CARTESIAN_POINT('Ctrl Pts',(1.80245274945248,6.52485398647728,148.716944460801));
#46037=CARTESIAN_POINT('Ctrl Pts',(1.6336257460409,6.56685281713184,148.725171879945));
#46038=CARTESIAN_POINT('Ctrl Pts',(1.5878156857973,6.57824891445967,148.727404334227));
#46039=CARTESIAN_POINT('Ctrl Pts',(1.54190297044554,6.58916150686769,148.729636788509));
#46040=CARTESIAN_POINT('Ctrl Pts',(1.49589863188773,6.59958909956646,148.731869242791));
#46041=CARTESIAN_POINT('Ctrl Pts',(1.32638072773533,6.63801294642667,148.740095444554));
#46042=CARTESIAN_POINT('Ctrl Pts',(1.1551444957387,6.66995491392575,148.748321646317));
#46043=CARTESIAN_POINT('Ctrl Pts',(0.982726700329653,6.69526229751002,148.75654784808));
#46044=CARTESIAN_POINT('Ctrl Pts',(0.810502580265703,6.72054125353996,148.764764809425));
#46045=CARTESIAN_POINT('Ctrl Pts',(0.637099891296366,6.73920041413438,148.77298177077));
#46046=CARTESIAN_POINT('Ctrl Pts',(0.463068282913116,6.75113744233962,148.781198732115));
#46047=CARTESIAN_POINT('Ctrl Pts',(0.289197233144874,6.76306345764476,148.789408112631));
#46048=CARTESIAN_POINT('Ctrl Pts',(0.114698775060923,6.76827966714148,148.797617493147));
#46049=CARTESIAN_POINT('Ctrl Pts',(-0.0598694812759922,6.7667351540615,
148.805826873663));
#46050=CARTESIAN_POINT('Ctrl Pts',(-0.234311709875384,6.76519175602669,
148.814030327502));
#46051=CARTESIAN_POINT('Ctrl Pts',(-0.40882327918961,6.75689736035804,148.822233781341));
#46052=CARTESIAN_POINT('Ctrl Pts',(-0.582843623452481,6.74185303240888,
148.83043723518));
#46053=CARTESIAN_POINT('Ctrl Pts',(-0.75677324356916,6.72681654770249,148.838636412212));
#46054=CARTESIAN_POINT('Ctrl Pts',(-0.930211792370118,6.70503717205541,
148.846835589244));
#46055=CARTESIAN_POINT('Ctrl Pts',(-1.10260078454534,6.67656801881925,148.855034766277));
#46056=CARTESIAN_POINT('Ctrl Pts',(-1.27495733857424,6.64810422257571,148.863232400484));
#46057=CARTESIAN_POINT('Ctrl Pts',(-1.44626437487053,6.61295320838439,148.871430034691));
#46058=CARTESIAN_POINT('Ctrl Pts',(-1.61597028789769,6.57121975196629,148.879627668898));
#46059=CARTESIAN_POINT('Ctrl Pts',(-1.78566397759705,6.52948930146418,148.887824712658));
#46060=CARTESIAN_POINT('Ctrl Pts',(-1.95375642518749,6.48117743774689,148.896021756418));
#46061=CARTESIAN_POINT('Ctrl Pts',(-2.11970800408929,6.42643968130098,148.904218800178));
#46062=CARTESIAN_POINT('Ctrl Pts',(-2.28567779148569,6.37169591893364,148.912416743332));
#46063=CARTESIAN_POINT('Ctrl Pts',(-2.44950590150521,6.31052497153085,148.920614686485));
#46064=CARTESIAN_POINT('Ctrl Pts',(-2.61066956059549,6.24313170174875,148.928812629639));
#46065=CARTESIAN_POINT('Ctrl Pts',(-2.77188019416391,6.17571878880579,148.937012962253));
#46066=CARTESIAN_POINT('Ctrl Pts',(-2.93042449906161,6.10208007930452,148.945213294867));
#46067=CARTESIAN_POINT('Ctrl Pts',(-3.08580126436238,6.0224678958762,148.95341362748));
#46068=CARTESIAN_POINT('Ctrl Pts',(-3.24133997366222,5.94277273533523,148.961622507026));
#46069=CARTESIAN_POINT('Ctrl Pts',(-3.39370422798857,5.85709182613359,148.969831386572));
#46070=CARTESIAN_POINT('Ctrl Pts',(-3.54241807360485,5.76572312826394,148.978040266118));
#46071=CARTESIAN_POINT('Ctrl Pts',(-3.69121175197275,5.67430538173623,148.986253552364));
#46072=CARTESIAN_POINT('Ctrl Pts',(-3.83635081725048,5.57719395889699,148.994466838611));
#46073=CARTESIAN_POINT('Ctrl Pts',(-3.97738984309682,5.47472912900997,149.002680124858));
#46074=CARTESIAN_POINT('Ctrl Pts',(-4.11863519109865,5.37211440610975,149.010905426097));
#46075=CARTESIAN_POINT('Ctrl Pts',(-4.25576823160249,5.26413084759802,149.019130727337));
#46076=CARTESIAN_POINT('Ctrl Pts',(-4.38837708282492,5.1511586637316,149.027356028577));
#46077=CARTESIAN_POINT('Ctrl Pts',(-4.50830565974434,5.04898906405793,149.034794813117));
#46078=CARTESIAN_POINT('Ctrl Pts',(-4.62453422653369,4.94273989356865,149.042233597658));
#46079=CARTESIAN_POINT('Ctrl Pts',(-4.73678561079548,4.83271673878792,149.049672382199));
#46080=CARTESIAN_POINT('Ctrl Pts',(-4.85803307738912,4.71387607707551,149.057707327923));
#46081=CARTESIAN_POINT('Ctrl Pts',(-4.97502002374452,4.59025882254214,149.065742273648));
#46082=CARTESIAN_POINT('Ctrl Pts',(-5.08733491019311,4.46220937558184,149.073777219373));
#46083=CARTESIAN_POINT('Ctrl Pts',(-5.19951770846345,4.33431052146556,149.081802715582));
#46084=CARTESIAN_POINT('Ctrl Pts',(-5.30703913411327,4.20199012627802,149.08982821179));
#46085=CARTESIAN_POINT('Ctrl Pts',(-5.4095220371579,4.06563160277749,149.097853707999));
#46086=CARTESIAN_POINT('Ctrl Pts',(-5.51190724024873,3.92940307385215,149.105871553267));
#46087=CARTESIAN_POINT('Ctrl Pts',(-5.60926325531765,3.7891443765773,149.113889398535));
#46088=CARTESIAN_POINT('Ctrl Pts',(-5.70125112887812,3.64527427849619,149.121907243803));
#46089=CARTESIAN_POINT('Ctrl Pts',(-5.79316596150943,3.50151841727303,149.129918722679));
#46090=CARTESIAN_POINT('Ctrl Pts',(-5.87972093833214,3.35415718109323,149.137930201555));
#46091=CARTESIAN_POINT('Ctrl Pts',(-5.9606187667796,3.20364057239804,149.14594168043));
#46092=CARTESIAN_POINT('Ctrl Pts',(-6.04148158251528,3.053189107536,149.153949691925));
#46093=CARTESIAN_POINT('Ctrl Pts',(-6.11669194310629,2.89958531797667,149.16195770342));
#46094=CARTESIAN_POINT('Ctrl Pts',(-6.1859970691669,2.74330626439312,149.169965714915));
#46095=CARTESIAN_POINT('Ctrl Pts',(-6.25528612372444,2.58706345112009,149.177971869393));
#46096=CARTESIAN_POINT('Ctrl Pts',(-6.31867251662192,2.42814695248479,149.185978023871));
#46097=CARTESIAN_POINT('Ctrl Pts',(-6.37595052568969,2.26705621764379,149.193984178349));
#46098=CARTESIAN_POINT('Ctrl Pts',(-6.43322675806054,2.10597047964916,149.201990084485));
#46099=CARTESIAN_POINT('Ctrl Pts',(-6.48439485906697,1.94271099495298,149.209995990622));
#46100=CARTESIAN_POINT('Ctrl Pts',(-6.52929820438422,1.77779468955923,149.218001896758));
#46101=CARTESIAN_POINT('Ctrl Pts',(-6.57422542585116,1.61279069434266,149.226012059821));
#46102=CARTESIAN_POINT('Ctrl Pts',(-6.61288113874827,1.44612848236859,149.234022222883));
#46103=CARTESIAN_POINT('Ctrl Pts',(-6.64515922493019,1.27833793471255,149.242032385946));
#46104=CARTESIAN_POINT('Ctrl Pts',(-6.67744680380719,1.11049804136435,149.250044904725));
#46105=CARTESIAN_POINT('Ctrl Pts',(-6.70335296096843,0.941529523093904,
149.258057423504));
#46106=CARTESIAN_POINT('Ctrl Pts',(-6.72282324652257,0.771969297327177,
149.266069942284));
#46107=CARTESIAN_POINT('Ctrl Pts',(-6.74231191257035,0.602249001969103,
149.274090025105));
#46108=CARTESIAN_POINT('Ctrl Pts',(-6.75535254533619,0.431936258650848,
149.282110107926));
#46109=CARTESIAN_POINT('Ctrl Pts',(-6.7619427611625,0.261570439388989,149.290130190747));
#46110=CARTESIAN_POINT('Ctrl Pts',(-6.76531612817425,0.174364428269627,
149.294235470988));
#46111=CARTESIAN_POINT('Ctrl Pts',(-6.76700022446772,0.0871444901626732,
149.29834075123));
#46112=CARTESIAN_POINT('Ctrl Pts',(-6.76699999997756,-1.74287689782069E-5,
149.302446031472));
#46113=CARTESIAN_POINT('Ctrl Pts',(-6.767,9.01944950864228E-12,149.30282021619));
#46114=CARTESIAN_POINT('Ctrl Pts',(-6.76700000000025,-0.18600724940665,
149.311569727996));
#46115=CARTESIAN_POINT('Ctrl Pts',(-6.75932637295488,-0.372014355518504,
149.320319239802));
#46116=CARTESIAN_POINT('Ctrl Pts',(-6.74400518267002,-0.557389537146031,
149.329068751608));
#46117=CARTESIAN_POINT('Ctrl Pts',(-6.72868405709744,-0.742763935802529,
149.337818226458));
#46118=CARTESIAN_POINT('Ctrl Pts',(-6.70571545653112,-0.92750612968633,
149.346567701309));
#46119=CARTESIAN_POINT('Ctrl Pts',(-6.67517739415792,-1.11098863924122,
149.35531717616));
#46120=CARTESIAN_POINT('Ctrl Pts',(-6.64463945823232,-1.29447038905826,
149.364066614782));
#46121=CARTESIAN_POINT('Ctrl Pts',(-6.60653217027305,-1.47669218227555,
149.372816053404));
#46122=CARTESIAN_POINT('Ctrl Pts',(-6.56098496116875,-1.65703510503474,
149.381565492025));
#46123=CARTESIAN_POINT('Ctrl Pts',(-6.51543793687688,-1.83737729603417,
149.390314895146));
#46124=CARTESIAN_POINT('Ctrl Pts',(-6.46245112202815,-2.01584035396493,
149.399064298266));
#46125=CARTESIAN_POINT('Ctrl Pts',(-6.4022044841642,-2.19181813637625,149.407813701386));
#46126=CARTESIAN_POINT('Ctrl Pts',(-6.3419580857538,-2.36779521935426,149.416563069732));
#46127=CARTESIAN_POINT('Ctrl Pts',(-6.27445201489444,-2.5412867754431,149.425312438077));
#46128=CARTESIAN_POINT('Ctrl Pts',(-6.19991555136409,-2.71170355237325,
149.434061806422));
#46129=CARTESIAN_POINT('Ctrl Pts',(-6.12537937789278,-2.88211966612562,
149.442811140719));
#46130=CARTESIAN_POINT('Ctrl Pts',(-6.04381298133871,-3.04946076209941,
149.451560475016));
#46131=CARTESIAN_POINT('Ctrl Pts',(-5.95549339426575,-3.21315848206357,
149.460309809313));
#46132=CARTESIAN_POINT('Ctrl Pts',(-5.86717414355448,-3.37685557859135,
149.469059110289));
#46133=CARTESIAN_POINT('Ctrl Pts',(-5.77210188986546,-3.53690907466809,
149.477808411264));
#46134=CARTESIAN_POINT('Ctrl Pts',(-5.67059953467396,-3.69277536784401,
149.48655771224));
#46135=CARTESIAN_POINT('Ctrl Pts',(-5.56909755762115,-3.84864108035286,
149.495306980621));
#46136=CARTESIAN_POINT('Ctrl Pts',(-5.46116568338442,-4.00031938103771,
149.504056249001));
#46137=CARTESIAN_POINT('Ctrl Pts',(-5.34717048686509,-4.14729511662709,
149.512805517382));
#46138=CARTESIAN_POINT('Ctrl Pts',(-5.23317570555944,-4.2942703168752,149.521554753895));
#46139=CARTESIAN_POINT('Ctrl Pts',(-5.11311782179264,-4.436542759866,149.530303990407));
#46140=CARTESIAN_POINT('Ctrl Pts',(-4.98740459172507,-4.57362924147112,
149.53905322692));
#46141=CARTESIAN_POINT('Ctrl Pts',(-4.86169180911318,-4.71071523513934,
149.547802432291));
#46142=CARTESIAN_POINT('Ctrl Pts',(-4.73032391415912,-4.84261509316055,
149.556551637662));
#46143=CARTESIAN_POINT('Ctrl Pts',(-4.59374707237765,-4.96888084331087,
149.565300843033));
#46144=CARTESIAN_POINT('Ctrl Pts',(-4.45717070537876,-5.09514615452311,
149.57405001799));
#46145=CARTESIAN_POINT('Ctrl Pts',(-4.31538563819983,-5.21577720253241,
149.582799192946));
#46146=CARTESIAN_POINT('Ctrl Pts',(-4.16887341291121,-5.3303642902828,149.591548367902));
#46147=CARTESIAN_POINT('Ctrl Pts',(-4.02236168477824,-5.44495098920818,
149.60029751317));
#46148=CARTESIAN_POINT('Ctrl Pts',(-3.87112305634937,-5.55349359238412,
149.609046658438));
#46149=CARTESIAN_POINT('Ctrl Pts',(-3.71567117317242,-5.65562346102138,
149.617795803706));
#46150=CARTESIAN_POINT('Ctrl Pts',(-3.56021980457814,-5.75775299158452,
149.626544920012));
#46151=CARTESIAN_POINT('Ctrl Pts',(-3.40055544862904,-5.85346967275053,
149.635294036318));
#46152=CARTESIAN_POINT('Ctrl Pts',(-3.23722036323922,-5.94244842803279,
149.644043152624));
#46153=CARTESIAN_POINT('Ctrl Pts',(-3.07388580496577,-6.03142689616205,
149.652792240695));
#46154=CARTESIAN_POINT('Ctrl Pts',(-2.90688079258249,-6.11366734484565,
149.661541328766));
#46155=CARTESIAN_POINT('Ctrl Pts',(-2.73677251095168,-6.18889046787057,
149.670290416837));
#46156=CARTESIAN_POINT('Ctrl Pts',(-2.56666476417227,-6.26411335438031,
149.679039477399));
#46157=CARTESIAN_POINT('Ctrl Pts',(-2.39345402972704,-6.33231884350059,
149.687788537962));
#46158=CARTESIAN_POINT('Ctrl Pts',(-2.21772856474678,-6.39327529620821,
149.696537598524));
#46159=CARTESIAN_POINT('Ctrl Pts',(-2.04200363768948,-6.45423156231866,
149.705286632304));
#46160=CARTESIAN_POINT('Ctrl Pts',(-1.86376426620811,-6.50793874251849,
149.714035666084));
#46161=CARTESIAN_POINT('Ctrl Pts',(-1.68361578195445,-6.55421443795928,
149.722784699864));
#46162=CARTESIAN_POINT('Ctrl Pts',(-1.50346783420668,-6.60048999558496,
149.731533707588));
#46163=CARTESIAN_POINT('Ctrl Pts',(-1.32141106258089,-6.63933404145327,
149.740282715312));
#46164=CARTESIAN_POINT('Ctrl Pts',(-1.13806375959929,-6.67061465526879,
149.749031723036));
#46165=CARTESIAN_POINT('Ctrl Pts',(-0.954716987427849,-6.70189517852357,
149.757780705431));
#46166=CARTESIAN_POINT('Ctrl Pts',(-0.770079973818414,-6.72561226535731,
149.766529687826));
#46167=CARTESIAN_POINT('Ctrl Pts',(-0.584779770560826,-6.7416853693971,
149.775278670221));
#46168=CARTESIAN_POINT('Ctrl Pts',(-0.391490647562162,-6.75845143942346,
149.784404850897));
#46169=CARTESIAN_POINT('Ctrl Pts',(-0.197480213112457,-6.76689975924003,
149.793531031573));
#46170=CARTESIAN_POINT('Ctrl Pts',(-0.00346532630577843,-6.76699911271707,
149.802657212249));
#46171=CARTESIAN_POINT('Ctrl Pts',(0.184486595288163,-6.76709536139795,
149.811498199779));
#46172=CARTESIAN_POINT('Ctrl Pts',(0.372442378177437,-6.75935659726813,
149.820339187309));
#46173=CARTESIAN_POINT('Ctrl Pts',(0.5597502177144,-6.7438096572908,149.829180174839));
#46174=CARTESIAN_POINT('Ctrl Pts',(0.745129914450085,-6.72842275717338,
149.837930153437));
#46175=CARTESIAN_POINT('Ctrl Pts',(0.929874656306541,-6.70538772273579,
149.846680132035));
#46176=CARTESIAN_POINT('Ctrl Pts',(1.11335688289016,-6.67478280180869,149.855430110632));
#46177=CARTESIAN_POINT('Ctrl Pts',(1.29683723118086,-6.64417819418173,149.864179999657));
#46178=CARTESIAN_POINT('Ctrl Pts',(1.47905480729456,-6.60600390230249,149.872929888682));
#46179=CARTESIAN_POINT('Ctrl Pts',(1.65939064804022,-6.56038959797333,149.881679777707));
#46180=CARTESIAN_POINT('Ctrl Pts',(1.8397247026349,-6.51477574543475,149.890429580068));
#46181=CARTESIAN_POINT('Ctrl Pts',(2.01817678125084,-6.46172209820339,149.899179382429));
#46182=CARTESIAN_POINT('Ctrl Pts',(2.19414072346928,-6.40140886724272,149.90792918479));
#46183=CARTESIAN_POINT('Ctrl Pts',(2.37010298131359,-6.3410962136165,149.916678903395));
#46184=CARTESIAN_POINT('Ctrl Pts',(2.5435768792619,-6.27352420826264,149.925428622001));
#46185=CARTESIAN_POINT('Ctrl Pts',(2.71397317789264,-6.19892237325806,149.934178340606));
#46186=CARTESIAN_POINT('Ctrl Pts',(2.88436790206507,-6.1243212275729,149.942927978365));
#46187=CARTESIAN_POINT('Ctrl Pts',(3.05168482125576,-6.04269049717761,149.951677616123));
#46188=CARTESIAN_POINT('Ctrl Pts',(3.21535561996723,-5.95430745235289,149.960427253881));
#46189=CARTESIAN_POINT('Ctrl Pts',(3.37902496074624,-5.86592519481895,149.9691768137));
#46190=CARTESIAN_POINT('Ctrl Pts',(3.53904799384228,-5.77079087940629,149.977926373519));
#46191=CARTESIAN_POINT('Ctrl Pts',(3.69488118814347,-5.66922763747439,149.986675933338));
#46192=CARTESIAN_POINT('Ctrl Pts',(3.85071304610209,-5.56766526649483,149.995425418126));
#46193=CARTESIAN_POINT('Ctrl Pts',(4.00235489705358,-5.45967423581161,150.004174902913));
#46194=CARTESIAN_POINT('Ctrl Pts',(4.14929168607059,-5.3456213393679,150.012924387701));
#46195=CARTESIAN_POINT('Ctrl Pts',(4.29622726385165,-5.23156938309016,150.021673800364));
#46196=CARTESIAN_POINT('Ctrl Pts',(4.43845763091479,-5.11145583677712,150.030423213027));
#46197=CARTESIAN_POINT('Ctrl Pts',(4.5754997066038,-4.98568866204746,150.039172625691));
#46198=CARTESIAN_POINT('Ctrl Pts',(4.7125406981473,-4.85992248226709,150.047921969137));
#46199=CARTESIAN_POINT('Ctrl Pts',(4.84439326930767,-4.72850295734563,150.056671312583));
#46200=CARTESIAN_POINT('Ctrl Pts',(4.97060959434169,-4.59187644222254,150.06542065603));
#46201=CARTESIAN_POINT('Ctrl Pts',(5.09682496279998,-4.45525096257255,150.074169933166));
#46202=CARTESIAN_POINT('Ctrl Pts',(5.21740397615335,-4.31341878218936,150.082919210302));
#46203=CARTESIAN_POINT('Ctrl Pts',(5.33193710451443,-4.16686161439305,150.091668487438));
#46204=CARTESIAN_POINT('Ctrl Pts',(5.44646940288906,-4.0203055086516,150.100417701171));
#46205=CARTESIAN_POINT('Ctrl Pts',(5.55495572749203,-3.86902470980796,150.109166914904));
#46206=CARTESIAN_POINT('Ctrl Pts',(5.65702762491009,-3.71353301466462,150.117916128637));
#46207=CARTESIAN_POINT('Ctrl Pts',(5.75909881654742,-3.55804239467561,150.126665281873));
#46208=CARTESIAN_POINT('Ctrl Pts',(5.85475551250403,-3.39834117620207,150.13541443511));
#46209=CARTESIAN_POINT('Ctrl Pts',(5.94367283727747,-3.23497174692608,150.144163588346));
#46210=CARTESIAN_POINT('Ctrl Pts',(6.03258957675983,-3.07160339301611,150.152912683991));
#46211=CARTESIAN_POINT('Ctrl Pts',(6.11476689684975,-2.90456712830154,150.161661779637));
#46212=CARTESIAN_POINT('Ctrl Pts',(6.18992570524972,-2.73443024476559,150.170410875282));
#46213=CARTESIAN_POINT('Ctrl Pts',(6.26508404388419,-2.56429442463709,150.179159916243));
#46214=CARTESIAN_POINT('Ctrl Pts',(6.33322384283048,-2.39105828656697,150.187908957204));
#46215=CARTESIAN_POINT('Ctrl Pts',(6.3941136871978,-2.21531017132811,150.196657998165));
#46216=CARTESIAN_POINT('Ctrl Pts',(6.45500317120656,-2.03956309620255,150.205406987348));
#46217=CARTESIAN_POINT('Ctrl Pts',(6.50864269269859,-1.86130434439383,150.21415597653));
#46218=CARTESIAN_POINT('Ctrl Pts',(6.55485008446139,-1.68113930720703,150.222904965713));
#46219=CARTESIAN_POINT('Ctrl Pts',(6.60199664749235,-1.49731239212586,150.231831779242));
#46220=CARTESIAN_POINT('Ctrl Pts',(6.64140563640763,-1.31150116500403,150.240758592771));
#46221=CARTESIAN_POINT('Ctrl Pts',(6.67293772282051,-1.12436255156377,150.249685406301));
#46222=CARTESIAN_POINT('Ctrl Pts',(6.70384494949771,-0.940932395058484,
150.258435320456));
#46223=CARTESIAN_POINT('Ctrl Pts',(6.72718449348851,-0.756227260513811,
150.267185234612));
#46224=CARTESIAN_POINT('Ctrl Pts',(6.74287707373872,-0.570874564548736,
150.275935148767));
#46225=CARTESIAN_POINT('Ctrl Pts',(6.7585693453863,-0.385525513639488,150.284684890851));
#46226=CARTESIAN_POINT('Ctrl Pts',(6.76661493004083,-0.199529212425204,
150.293434632935));
#46227=CARTESIAN_POINT('Ctrl Pts',(6.76698649908905,-0.0135174386073543,
150.302184375019));
#46228=CARTESIAN_POINT('Ctrl Pts',(6.76735806132407,0.172490924438802,150.310933956665));
#46229=CARTESIAN_POINT('Ctrl Pts',(6.76005588896326,0.358514472894389,150.319683538311));
#46230=CARTESIAN_POINT('Ctrl Pts',(6.74510478454641,0.54392135965516,150.328433119957));
#46231=CARTESIAN_POINT('Ctrl Pts',(6.73015393440765,0.729325093143337,150.337182552796));
#46232=CARTESIAN_POINT('Ctrl Pts',(6.70755443556994,0.914111900249198,150.345931985635));
#46233=CARTESIAN_POINT('Ctrl Pts',(6.67738304682437,1.09765415590819,150.354681418474));
#46234=CARTESIAN_POINT('Ctrl Pts',(6.64721213111997,1.28119353390565,150.363430714135));
#46235=CARTESIAN_POINT('Ctrl Pts',(6.60946960955649,1.46348811671957,150.372180009797));
#46236=CARTESIAN_POINT('Ctrl Pts',(6.56428366991354,1.64391876347538,150.380929305458));
#46237=CARTESIAN_POINT('Ctrl Pts',(6.51909837867908,1.82434682109034,150.389678475569));
#46238=CARTESIAN_POINT('Ctrl Pts',(6.46646995272131,2.00291071819767,150.39842764568));
#46239=CARTESIAN_POINT('Ctrl Pts',(6.40657713281779,2.17900400212029,150.40717681579));
#46240=CARTESIAN_POINT('Ctrl Pts',(6.34668509279304,2.35509499309002,150.415925871976));
#46241=CARTESIAN_POINT('Ctrl Pts',(6.27952894037783,2.52871516397484,150.424674928162));
#46242=CARTESIAN_POINT('Ctrl Pts',(6.20533675061716,2.699274867708,150.433423984348));
#46243=CARTESIAN_POINT('Ctrl Pts',(6.12832117908193,2.87632521635336,150.44250598563));
#46244=CARTESIAN_POINT('Ctrl Pts',(6.0437236662636,3.05007728919442,150.451587986912));
#46245=CARTESIAN_POINT('Ctrl Pts',(5.95185378008151,3.21989527477672,150.460669988195));
#46246=CARTESIAN_POINT('Ctrl Pts',(5.86334450817671,3.38350129286232,150.469419768502));
#46247=CARTESIAN_POINT('Ctrl Pts',(5.76808562057572,3.54345567124447,150.478169548809));
#46248=CARTESIAN_POINT('Ctrl Pts',(5.66640068804817,3.69921508464799,150.486919329116));
#46249=CARTESIAN_POINT('Ctrl Pts',(5.56471941108274,3.85496889851777,150.495668794869));
#46250=CARTESIAN_POINT('Ctrl Pts',(5.45661270815482,4.00652780919135,150.504418260623));
#46251=CARTESIAN_POINT('Ctrl Pts',(5.342447764495,4.15337704568733,150.513167726376));
#46252=CARTESIAN_POINT('Ctrl Pts',(5.22828631819995,4.30022178355763,150.521916924096));
#46253=CARTESIAN_POINT('Ctrl Pts',(5.10806717844484,4.44235690972202,150.530666121816));
#46254=CARTESIAN_POINT('Ctrl Pts',(4.98219864545147,4.57929969070179,150.539415319535));
#46255=CARTESIAN_POINT('Ctrl Pts',(4.85633329944467,4.71623900429546,150.548164295725));
#46256=CARTESIAN_POINT('Ctrl Pts',(4.72481904034104,4.84798602483173,150.556913271916));
#46257=CARTESIAN_POINT('Ctrl Pts',(4.58810250737667,4.97409332258693,150.565662248106));
#46258=CARTESIAN_POINT('Ctrl Pts',(4.45137708686117,5.10020881821721,150.574411793042));
#46259=CARTESIAN_POINT('Ctrl Pts',(4.30944892636532,5.22068366307537,150.583161337978));
#46260=CARTESIAN_POINT('Ctrl Pts',(4.16280009467146,5.33510865604472,150.591910882914));
#46261=CARTESIAN_POINT('Ctrl Pts',(4.01615988349291,5.44952692272521,150.600659913523));
#46262=CARTESIAN_POINT('Ctrl Pts',(3.8647997823275,5.55789587288265,150.609408944131));
#46263=CARTESIAN_POINT('Ctrl Pts',(3.70923383581604,5.65984746713526,150.618157974739));
#46264=CARTESIAN_POINT('Ctrl Pts',(3.55366577800089,5.76180044505044,150.626907124087));
#46265=CARTESIAN_POINT('Ctrl Pts',(3.39389200027401,5.85733573570734,150.635656273435));
#46266=CARTESIAN_POINT('Ctrl Pts',(3.23045513626613,5.94612887621617,150.644405422783));
#46267=CARTESIAN_POINT('Ctrl Pts',(3.18695122151961,5.96976399206486,150.646734286896));
#46268=CARTESIAN_POINT('Ctrl Pts',(3.14318791262855,5.99292165435235,150.649063151009));
#46269=CARTESIAN_POINT('Ctrl Pts',(3.09917575053255,6.01559628526641,150.651392015123));
#46270=CARTESIAN_POINT('Origin',(0.,0.,-3.69717978381041));
#46271=CARTESIAN_POINT('',(3.09917575053261,6.01559628526638,153.045781927116));
#46272=CARTESIAN_POINT('',(3.0991757505326,6.01559628526638,152.651615498439));
#46273=CARTESIAN_POINT('',(3.09917575053259,6.01559628526639,-3.69717978381041));
#46274=CARTESIAN_POINT('',(-6.76699781313954,-0.0054403092439294,151.697179783855));
#46275=CARTESIAN_POINT('Ctrl Pts',(-6.76699781313954,-0.00544030924374474,
151.697179783855));
#46276=CARTESIAN_POINT('Ctrl Pts',(-6.76682066285936,-0.225790937285296,
151.707538286931));
#46277=CARTESIAN_POINT('Ctrl Pts',(-6.75587712910279,-0.445703616568735,
151.717896790007));
#46278=CARTESIAN_POINT('Ctrl Pts',(-6.73431712015831,-0.664275488892024,
151.728255293083));
#46279=CARTESIAN_POINT('Ctrl Pts',(-6.71240037143604,-0.886463931197475,
151.738785191732));
#46280=CARTESIAN_POINT('Ctrl Pts',(-6.67951292140793,-1.10726700774589,
151.749315090381));
#46281=CARTESIAN_POINT('Ctrl Pts',(-6.63586112722697,-1.32575868850933,
151.75984498903));
#46282=CARTESIAN_POINT('Ctrl Pts',(-6.61854007886523,-1.41245626967753,
151.764023256777));
#46283=CARTESIAN_POINT('Ctrl Pts',(-6.599524712548,-1.49879014981483,151.768201524525));
#46284=CARTESIAN_POINT('Ctrl Pts',(-6.57883001468178,-1.58470332804665,
151.772379792272));
#46285=CARTESIAN_POINT('Ctrl Pts',(-6.53601859897826,-1.7624331413288,151.781023434166));
#46286=CARTESIAN_POINT('Ctrl Pts',(-6.48596221488716,-1.9385873517263,151.78966707606));
#46287=CARTESIAN_POINT('Ctrl Pts',(-6.42879045362175,-2.11256770386701,
151.798310717954));
#46288=CARTESIAN_POINT('Ctrl Pts',(-6.37169244615921,-2.28632361456472,
151.806943209212));
#46289=CARTESIAN_POINT('Ctrl Pts',(-6.30749745980911,-2.45791097036454,
151.815575700471));
#46290=CARTESIAN_POINT('Ctrl Pts',(-6.23638551469233,-2.62674412764847,
151.824208191729));
#46291=CARTESIAN_POINT('Ctrl Pts',(-6.16273537061777,-2.8016034475293,151.833148802535));
#46292=CARTESIAN_POINT('Ctrl Pts',(-6.08166543488737,-2.97350801273204,
151.84208941334));
#46293=CARTESIAN_POINT('Ctrl Pts',(-5.99343230693078,-3.1418240215261,151.851030024146));
#46294=CARTESIAN_POINT('Ctrl Pts',(-5.90847739352962,-3.30388641557568,
151.859638455405));
#46295=CARTESIAN_POINT('Ctrl Pts',(-5.81688210052459,-3.4626217765525,151.868246886663));
#46296=CARTESIAN_POINT('Ctrl Pts',(-5.71892465582685,-3.61748390196497,
151.876855317922));
#46297=CARTESIAN_POINT('Ctrl Pts',(-5.62106020070992,-3.77219901900898,
151.885455577321));
#46298=CARTESIAN_POINT('Ctrl Pts',(-5.5168457975921,-3.92304797382831,151.894055836721));
#46299=CARTESIAN_POINT('Ctrl Pts',(-5.40660531102839,-4.06950955408139,
151.90265609612));
#46300=CARTESIAN_POINT('Ctrl Pts',(-5.29648918255778,-4.21580591660546,
151.911246653895));
#46301=CARTESIAN_POINT('Ctrl Pts',(-5.18036071515962,-4.35772453466346,
151.91983721167));
#46302=CARTESIAN_POINT('Ctrl Pts',(-5.05858687090311,-4.4947733946804,151.928427769444));
#46303=CARTESIAN_POINT('Ctrl Pts',(-5.04409142298777,-4.51108711643535,
151.929450353428));
#46304=CARTESIAN_POINT('Ctrl Pts',(-5.02951603259424,-4.52733187070495,
151.930472937412));
#46305=CARTESIAN_POINT('Ctrl Pts',(-5.01486135872867,-4.54350685624332,
151.931495521396));
#46306=CARTESIAN_POINT('Ctrl Pts',(-4.89152421449246,-4.6796392971741,151.940101826078));
#46307=CARTESIAN_POINT('Ctrl Pts',(-4.76271597648191,-4.8106636564498,151.948708130761));
#46308=CARTESIAN_POINT('Ctrl Pts',(-4.62888841512035,-4.93616055658288,
151.957314435443));
#46309=CARTESIAN_POINT('Ctrl Pts',(-4.49493053380187,-5.06177966435729,
151.96592912086));
#46310=CARTESIAN_POINT('Ctrl Pts',(-4.35594379387702,-5.18186036088778,
151.974543806276));
#46311=CARTESIAN_POINT('Ctrl Pts',(-4.21241341248116,-5.29602324790487,
151.983158491693));
#46312=CARTESIAN_POINT('Ctrl Pts',(-4.06322305990135,-5.41468802953486,
151.992112888262));
#46313=CARTESIAN_POINT('Ctrl Pts',(-3.90912375108719,-5.52695858495553,
152.001067284831));
#46314=CARTESIAN_POINT('Ctrl Pts',(-3.75069272947807,-5.63245888125607,
152.0100216814));
#46315=CARTESIAN_POINT('Ctrl Pts',(-3.5978452869411,-5.73424103422492,152.018660498477));
#46316=CARTESIAN_POINT('Ctrl Pts',(-3.44096652223121,-5.82972188038494,
152.027299315554));
#46317=CARTESIAN_POINT('Ctrl Pts',(-3.28059960474056,-5.91861092093205,
152.035938132631));
#46318=CARTESIAN_POINT('Ctrl Pts',(-3.12007657215159,-6.00758649379843,
152.044585359483));
#46319=CARTESIAN_POINT('Ctrl Pts',(-2.95605887790096,-6.08995731281826,
152.053232586336));
#46320=CARTESIAN_POINT('Ctrl Pts',(-2.78911142845873,-6.16548022782013,
152.061879813188));
#46321=CARTESIAN_POINT('Ctrl Pts',(-2.62191369320887,-6.24111636595801,
152.070540003869));
#46322=CARTESIAN_POINT('Ctrl Pts',(-2.45177770476479,-6.30988396628493,
152.079200194551));
#46323=CARTESIAN_POINT('Ctrl Pts',(-2.27928676565387,-6.37158856486474,
152.087860385232));
#46324=CARTESIAN_POINT('Ctrl Pts',(-2.26102314405801,-6.37812194827024,
152.088777340328));
#46325=CARTESIAN_POINT('Ctrl Pts',(-2.24273313349377,-6.3845761955102,152.089694295423));
#46326=CARTESIAN_POINT('Ctrl Pts',(-2.22441743461814,-6.39095110891695,
152.090611250519));
#46327=CARTESIAN_POINT('Ctrl Pts',(-2.06044476477771,-6.44802299999824,
152.098820359882));
#46328=CARTESIAN_POINT('Ctrl Pts',(-1.89405170220875,-6.49885770803804,
152.107029469246));
#46329=CARTESIAN_POINT('Ctrl Pts',(-1.72575409940623,-6.54324550879627,
152.115238578609));
#46330=CARTESIAN_POINT('Ctrl Pts',(-1.55763559982528,-6.58758607181623,
152.123438951794));
#46331=CARTESIAN_POINT('Ctrl Pts',(-1.38761694091712,-6.62549329787349,
152.131639324979));
#46332=CARTESIAN_POINT('Ctrl Pts',(-1.21623222764221,-6.65680615373803,
152.139839698164));
#46333=CARTESIAN_POINT('Ctrl Pts',(-1.04499519193563,-6.68809202816225,
152.148033005309));
#46334=CARTESIAN_POINT('Ctrl Pts',(-0.872394798051353,-6.71279478400163,
152.156226312454));
#46335=CARTESIAN_POINT('Ctrl Pts',(-0.698978604547322,-6.73080366006802,
152.1644196196));
#46336=CARTESIAN_POINT('Ctrl Pts',(-0.525676726956045,-6.74880066468767,
152.172607525719));
#46337=CARTESIAN_POINT('Ctrl Pts',(-0.351560477592479,-6.76011254137418,
152.180795431838));
#46338=CARTESIAN_POINT('Ctrl Pts',(-0.177185936192593,-6.76467989959729,
152.188983337957));
#46339=CARTESIAN_POINT('Ctrl Pts',(-0.00289104353758479,-6.76924517159641,
152.197167504101));
#46340=CARTESIAN_POINT('Ctrl Pts',(0.171661547038031,-6.76707205286047,
152.205351670245));
#46341=CARTESIAN_POINT('Ctrl Pts',(0.345912251864701,-6.75815312892582,
152.213535836389));
#46342=CARTESIAN_POINT('Ctrl Pts',(0.52014864388683,-6.74923493758399,152.221719330293));
#46343=CARTESIAN_POINT('Ctrl Pts',(0.694082839869698,-6.73357205407506,
152.229902824196));
#46344=CARTESIAN_POINT('Ctrl Pts',(0.867156516699929,-6.71120917387805,
152.2380863181));
#46345=CARTESIAN_POINT('Ctrl Pts',(1.04022887084597,-6.68884646458529,152.246269749463));
#46346=CARTESIAN_POINT('Ctrl Pts',(1.21244036167865,-6.65978390559459,152.254453180825));
#46347=CARTESIAN_POINT('Ctrl Pts',(1.38323918504562,-6.6241179304836,152.262636612188));
#46348=CARTESIAN_POINT('Ctrl Pts',(1.55406802980395,-6.58844568634701,152.270821481956));
#46349=CARTESIAN_POINT('Ctrl Pts',(1.72348335993138,-6.54616778734753,152.279006351725));
#46350=CARTESIAN_POINT('Ctrl Pts',(1.89094490308364,-6.497431521263,152.287191221493));
#46351=CARTESIAN_POINT('Ctrl Pts',(2.05846659610467,-6.44867774978616,152.295379031154));
#46352=CARTESIAN_POINT('Ctrl Pts',(2.22403275876064,-6.39346109100412,152.303566840814));
#46353=CARTESIAN_POINT('Ctrl Pts',(2.38711954936351,-6.33197830516234,152.311754650474));
#46354=CARTESIAN_POINT('Ctrl Pts',(2.55039578527835,-6.27042409952316,152.31995197128));
#46355=CARTESIAN_POINT('Ctrl Pts',(2.71118655795087,-6.20258935209995,152.328149292086));
#46356=CARTESIAN_POINT('Ctrl Pts',(2.86898826530126,-6.12871889823344,152.336346612891));
#46357=CARTESIAN_POINT('Ctrl Pts',(3.02688424282071,-6.05480431442504,152.344548830747));
#46358=CARTESIAN_POINT('Ctrl Pts',(3.18178727646132,-5.97484700216473,152.352751048602));
#46359=CARTESIAN_POINT('Ctrl Pts',(3.33321970147719,-5.88913706935782,152.360953266457));
#46360=CARTESIAN_POINT('Ctrl Pts',(3.48489273404859,-5.80329095397696,152.369168516631));
#46361=CARTESIAN_POINT('Ctrl Pts',(3.63308383197254,-5.71167414139782,152.377383766805));
#46362=CARTESIAN_POINT('Ctrl Pts',(3.77734444563583,-5.61462001733191,152.385599016979));
#46363=CARTESIAN_POINT('Ctrl Pts',(3.91339829548935,-5.52308715269189,152.393346914241));
#46364=CARTESIAN_POINT('Ctrl Pts',(4.04595622289335,-5.42671854493955,152.401094811504));
#46365=CARTESIAN_POINT('Ctrl Pts',(4.17467077253493,-5.32582509485081,152.408842708766));
#46366=CARTESIAN_POINT('Ctrl Pts',(4.31045240636619,-5.21939208060285,152.41701600504));
#46367=CARTESIAN_POINT('Ctrl Pts',(4.44237888345318,-5.10759238998213,152.425189301315));
#46368=CARTESIAN_POINT('Ctrl Pts',(4.56999418349115,-4.99073563343693,152.433362597589));
#46369=CARTESIAN_POINT('Ctrl Pts',(4.6974537140481,-4.87402151430523,152.441525917394));
#46370=CARTESIAN_POINT('Ctrl Pts',(4.82061227768349,-4.75226286039346,152.449689237199));
#46371=CARTESIAN_POINT('Ctrl Pts',(4.93904408494467,-4.6258115533356,152.457852557004));
#46372=CARTESIAN_POINT('Ctrl Pts',(5.05735599433471,-4.49948826292183,152.466007612436));
#46373=CARTESIAN_POINT('Ctrl Pts',(5.1709504277376,-4.36848204158194,152.474162667868));
#46374=CARTESIAN_POINT('Ctrl Pts',(5.27943585967152,-4.23318390855092,152.482317723299));
#46375=CARTESIAN_POINT('Ctrl Pts',(5.38783404239173,-4.09799458880029,152.490466220042));
#46376=CARTESIAN_POINT('Ctrl Pts',(5.49113117897016,-3.95852051332946,152.498614716785));
#46377=CARTESIAN_POINT('Ctrl Pts',(5.58897370801332,-3.81518831660193,152.506763213529));
#46378=CARTESIAN_POINT('Ctrl Pts',(5.68675790427688,-3.6719415731586,152.514906852216));
#46379=CARTESIAN_POINT('Ctrl Pts',(5.77909376505791,-3.52484158931778,152.523050490903));
#46380=CARTESIAN_POINT('Ctrl Pts',(5.86566902263997,-3.37434673927293,152.53119412959));
#46381=CARTESIAN_POINT('Ctrl Pts',(5.95243595276715,-3.22351870245232,152.539355797816));
#46382=CARTESIAN_POINT('Ctrl Pts',(6.03341652519195,-3.06928104646432,152.547517466042));
#46383=CARTESIAN_POINT('Ctrl Pts',(6.10834065229936,-2.91212353368931,152.555679134268));
#46384=CARTESIAN_POINT('Ctrl Pts',(6.18306921713104,-2.75537622363578,152.563819499418));
#46385=CARTESIAN_POINT('Ctrl Pts',(6.25177276618944,-2.59572461526402,152.571959864567));
#46386=CARTESIAN_POINT('Ctrl Pts',(6.31422997937869,-2.43367803283742,152.580100229717));
#46387=CARTESIAN_POINT('Ctrl Pts',(6.37669114641939,-2.27162119205822,152.588241110191));
#46388=CARTESIAN_POINT('Ctrl Pts',(6.43290505884602,-2.1071694150306,152.596381990666));
#46389=CARTESIAN_POINT('Ctrl Pts',(6.48269916034021,-1.94085048278437,152.604522871141));
#46390=CARTESIAN_POINT('Ctrl Pts',(6.53250579729907,-1.77448968041626,152.61266580105));
#46391=CARTESIAN_POINT('Ctrl Pts',(6.57588930064009,-1.60626113560997,152.620808730959));
#46392=CARTESIAN_POINT('Ctrl Pts',(6.61272745042785,-1.43670618651064,152.628951660868));
#46393=CARTESIAN_POINT('Ctrl Pts',(6.64971916818584,-1.26644441012698,152.63712853638));
#46394=CARTESIAN_POINT('Ctrl Pts',(6.68011076325744,-1.0948455081302,152.645305411892));
#46395=CARTESIAN_POINT('Ctrl Pts',(6.703830722841,-0.922465522116235,152.653482287404));
#46396=CARTESIAN_POINT('Ctrl Pts',(6.72748854798329,-0.750537085527412,
152.661637743588));
#46397=CARTESIAN_POINT('Ctrl Pts',(6.74450966163421,-0.577832019655981,
152.669793199773));
#46398=CARTESIAN_POINT('Ctrl Pts',(6.75487538359512,-0.404904374020209,
152.677948655957));
#46399=CARTESIAN_POINT('Ctrl Pts',(6.76528194204491,-0.231295467792647,
152.686136241133));
#46400=CARTESIAN_POINT('Ctrl Pts',(6.7689805684702,-0.0574625941143888,
152.694323826309));
#46401=CARTESIAN_POINT('Ctrl Pts',(6.76600505955837,0.116036778784197,152.702511411485));
#46402=CARTESIAN_POINT('Ctrl Pts',(6.76302955064653,0.289536151682656,152.710698996661));
#46403=CARTESIAN_POINT('Ctrl Pts',(6.75337998421799,0.462701662475575,152.718886581837));
#46404=CARTESIAN_POINT('Ctrl Pts',(6.73714210211013,0.634984484830179,152.727074167013));
#46405=CARTESIAN_POINT('Ctrl Pts',(6.72080726251413,0.80829601952519,152.735310640812));
#46406=CARTESIAN_POINT('Ctrl Pts',(6.69775835998404,0.981212097610075,152.74354711461));
#46407=CARTESIAN_POINT('Ctrl Pts',(6.66801914461703,1.15317374537436,152.751783588409));
#46408=CARTESIAN_POINT('Ctrl Pts',(6.63831273267355,1.32494571326005,152.760010977081));
#46409=CARTESIAN_POINT('Ctrl Pts',(6.60193076403463,1.49576499809945,152.768238365753));
#46410=CARTESIAN_POINT('Ctrl Pts',(6.55894885626404,1.66507624477458,152.776465754426));
#46411=CARTESIAN_POINT('Ctrl Pts',(6.51600580488551,1.83423443113852,152.784685705395));
#46412=CARTESIAN_POINT('Ctrl Pts',(6.46647478491051,2.00188695012239,152.792905656365));
#46413=CARTESIAN_POINT('Ctrl Pts',(6.41048273242969,2.16748705583697,152.801125607335));
#46414=CARTESIAN_POINT('Ctrl Pts',(6.35453015777041,2.33297040334873,152.809339762736));
#46415=CARTESIAN_POINT('Ctrl Pts',(6.29212573879177,2.49640388273475,152.817553918138));
#46416=CARTESIAN_POINT('Ctrl Pts',(6.22344669317352,2.65725427033763,152.825768073539));
#46417=CARTESIAN_POINT('Ctrl Pts',(6.15480240948141,2.81802324345311,152.833978071343));
#46418=CARTESIAN_POINT('Ctrl Pts',(6.07988996652485,2.97621140154097,152.842188069146));
#46419=CARTESIAN_POINT('Ctrl Pts',(5.99893534885182,3.13130383072229,152.85039806695));
#46420=CARTESIAN_POINT('Ctrl Pts',(5.91799446527066,3.28636994820293,152.858606671913));
#46421=CARTESIAN_POINT('Ctrl Pts',(5.83101360838452,3.438341063342,152.866815276876));
#46422=CARTESIAN_POINT('Ctrl Pts',(5.73826566776904,3.58672498612636,152.875023881839));
#46423=CARTESIAN_POINT('Ctrl Pts',(5.64552342457804,3.73509979381675,152.883231982555));
#46424=CARTESIAN_POINT('Ctrl Pts',(5.54701499199426,3.87988754437472,152.89144008327));
#46425=CARTESIAN_POINT('Ctrl Pts',(5.44305769737916,4.02062332269531,152.899648183986));
#46426=CARTESIAN_POINT('Ctrl Pts',(5.33908805214441,4.16137582109384,152.907857259863));
#46427=CARTESIAN_POINT('Ctrl Pts',(5.22966846758373,4.29807510049649,152.91606633574));
#46428=CARTESIAN_POINT('Ctrl Pts',(5.11515785859708,4.43028769738857,152.924275411617));
#46429=CARTESIAN_POINT('Ctrl Pts',(5.00061300646012,4.56253983101763,152.932486942329));
#46430=CARTESIAN_POINT('Ctrl Pts',(4.88097433125103,4.69030233929231,152.94069847304));
#46431=CARTESIAN_POINT('Ctrl Pts',(4.75663908369482,4.81317708249623,152.948910003752));
#46432=CARTESIAN_POINT('Ctrl Pts',(4.6321733316871,4.93618079718074,152.95713015343));
#46433=CARTESIAN_POINT('Ctrl Pts',(4.5030014132024,5.05428624544385,152.965350303108));
#46434=CARTESIAN_POINT('Ctrl Pts',(4.36955604258135,5.16713353715006,152.973570452786));
#46435=CARTESIAN_POINT('Ctrl Pts',(4.2360385128263,5.28004184980293,152.981795047421));
#46436=CARTESIAN_POINT('Ctrl Pts',(4.09824320547279,5.38768611750558,152.990019642055));
#46437=CARTESIAN_POINT('Ctrl Pts',(3.95663349822709,5.48974866097778,152.99824423669));
#46438=CARTESIAN_POINT('Ctrl Pts',(3.81481632539584,5.59196073138394,153.006480880783));
#46439=CARTESIAN_POINT('Ctrl Pts',(3.66917388251207,5.68857453730499,153.014717524877));
#46440=CARTESIAN_POINT('Ctrl Pts',(3.5201970339267,5.77931672798209,153.02295416897));
#46441=CARTESIAN_POINT('Ctrl Pts',(3.38543950074021,5.86139789621528,153.0304046544));
#46442=CARTESIAN_POINT('Ctrl Pts',(3.24795419331786,5.93867531269824,153.03785513983));
#46443=CARTESIAN_POINT('Ctrl Pts',(3.10811898405032,6.01098040098169,153.04530562526));
#46444=CARTESIAN_POINT('Ctrl Pts',(3.10513914377014,6.01252119757833,153.045464392545));
#46445=CARTESIAN_POINT('Ctrl Pts',(3.10215806480747,6.01405982642792,153.045623159831));
#46446=CARTESIAN_POINT('Ctrl Pts',(3.09917575053261,6.01559628526638,153.045781927116));
#46447=CARTESIAN_POINT('Ctrl Pts',(3.09917575053262,6.01559628526637,151.045614412788));
#46448=CARTESIAN_POINT('Ctrl Pts',(2.94387213756178,6.09560717171302,151.053822491478));
#46449=CARTESIAN_POINT('Ctrl Pts',(2.78556183173075,6.16955175392866,151.062030570168));
#46450=CARTESIAN_POINT('Ctrl Pts',(2.62476468355848,6.23721887991308,151.070238648858));
#46451=CARTESIAN_POINT('Ctrl Pts',(2.46387447321858,6.30492516859095,151.078451478015));
#46452=CARTESIAN_POINT('Ctrl Pts',(2.30049488689371,6.36634663295596,151.086664307172));
#46453=CARTESIAN_POINT('Ctrl Pts',(2.13516212173171,6.42132164853328,151.09487713633));
#46454=CARTESIAN_POINT('Ctrl Pts',(1.96959745390637,6.47637377437072,151.103101485145));
#46455=CARTESIAN_POINT('Ctrl Pts',(1.80207447805811,6.52496128703662,151.111325833961));
#46456=CARTESIAN_POINT('Ctrl Pts',(1.633141877495,6.56697316942685,151.119550182777));
#46457=CARTESIAN_POINT('Ctrl Pts',(1.52108161702273,6.5948414581283,151.125005747111));
#46458=CARTESIAN_POINT('Ctrl Pts',(1.40840128980731,6.61981737147946,151.130461311445));
#46459=CARTESIAN_POINT('Ctrl Pts',(1.295262361097,6.64188109016756,151.135916875779));
#46460=CARTESIAN_POINT('Ctrl Pts',(1.12619762638398,6.67485114556148,151.144069185045));
#46461=CARTESIAN_POINT('Ctrl Pts',(0.955608083129771,6.70141354431739,151.152221494311));
#46462=CARTESIAN_POINT('Ctrl Pts',(0.78402508820873,6.72142794806723,151.160373803576));
#46463=CARTESIAN_POINT('Ctrl Pts',(0.61264136654608,6.74141910746555,151.168516644904));
#46464=CARTESIAN_POINT('Ctrl Pts',(0.440266849311369,6.75487736779777,151.176659486231));
#46465=CARTESIAN_POINT('Ctrl Pts',(0.267444897019827,6.76171296544434,151.184802327558));
#46466=CARTESIAN_POINT('Ctrl Pts',(0.0947873154990069,6.76854206176143,
151.192937424238));
#46467=CARTESIAN_POINT('Ctrl Pts',(-0.0783164910748943,6.76876102111578,
151.201072520918));
#46468=CARTESIAN_POINT('Ctrl Pts',(-0.251316192730467,6.76233163718488,
151.209207617598));
#46469=CARTESIAN_POINT('Ctrl Pts',(-0.424187713524088,6.75590701698458,
151.217336686732));
#46470=CARTESIAN_POINT('Ctrl Pts',(-0.596954919196228,6.74284387543872,
151.225465755865));
#46471=CARTESIAN_POINT('Ctrl Pts',(-0.769065619154389,6.72315603518427,
151.233594824999));
#46472=CARTESIAN_POINT('Ctrl Pts',(-0.941084955812843,6.70347864602932,
151.241719578895));
#46473=CARTESIAN_POINT('Ctrl Pts',(-1.11244811839762,6.67718360315843,151.249844332791));
#46474=CARTESIAN_POINT('Ctrl Pts',(-1.28260618693369,6.64433671401739,151.257969086686));
#46475=CARTESIAN_POINT('Ctrl Pts',(-1.45379845852855,6.6112901848974,151.266143221992));
#46476=CARTESIAN_POINT('Ctrl Pts',(-1.6237705644435,6.5716119233359,151.274317357298));
#46477=CARTESIAN_POINT('Ctrl Pts',(-1.79197154642861,6.52542159379685,151.282491492604));
#46478=CARTESIAN_POINT('Ctrl Pts',(-1.95911821829167,6.4795207924841,151.290614391148));
#46479=CARTESIAN_POINT('Ctrl Pts',(-2.12451555646846,6.42718945040662,151.298737289692));
#46480=CARTESIAN_POINT('Ctrl Pts',(-2.28763618556708,6.36859558163997,151.306860188237));
#46481=CARTESIAN_POINT('Ctrl Pts',(-2.45077822839969,6.30999402093683,151.314984153118));
#46482=CARTESIAN_POINT('Ctrl Pts',(-2.61164262248649,6.24512841972122,151.323108118));
#46483=CARTESIAN_POINT('Ctrl Pts',(-2.76972026942334,6.17421562865645,151.331232082881));
#46484=CARTESIAN_POINT('Ctrl Pts',(-2.92784874914383,6.10328003427549,151.339358660174));
#46485=CARTESIAN_POINT('Ctrl Pts',(-3.08318836359391,6.02629352742905,151.347485237466));
#46486=CARTESIAN_POINT('Ctrl Pts',(-3.23525303135444,5.94351973355115,151.355611814758));
#46487=CARTESIAN_POINT('Ctrl Pts',(-3.38890446546756,5.8598822106234,151.363823191364));
#46488=CARTESIAN_POINT('Ctrl Pts',(-3.53921188552433,5.77033612681724,151.372034567969));
#46489=CARTESIAN_POINT('Ctrl Pts',(-3.68570311014295,5.67519881448066,151.380245944575));
#46490=CARTESIAN_POINT('Ctrl Pts',(-3.83093187624985,5.58088139364305,151.388386555697));
#46491=CARTESIAN_POINT('Ctrl Pts',(-3.97240970507219,5.48106900138085,151.39652716682));
#46492=CARTESIAN_POINT('Ctrl Pts',(-4.10970947800898,5.3761116995802,151.404667777942));
#46493=CARTESIAN_POINT('Ctrl Pts',(-4.24879954984783,5.26978582346835,151.41291453729));
#46494=CARTESIAN_POINT('Ctrl Pts',(-4.38360155522664,5.15818018942659,151.421161296637));
#46495=CARTESIAN_POINT('Ctrl Pts',(-4.51370994905373,5.0416972832384,151.429408055984));
#46496=CARTESIAN_POINT('Ctrl Pts',(-4.64381834288091,4.92521437705012,151.437654815331));
#46497=CARTESIAN_POINT('Ctrl Pts',(-4.76923289663995,4.80385451259961,151.445901574678));
#46498=CARTESIAN_POINT('Ctrl Pts',(-4.88959050076544,4.67805448181447,151.454148334026));
#46499=CARTESIAN_POINT('Ctrl Pts',(-5.0088099671827,4.55344405396111,151.462317109536));
#46500=CARTESIAN_POINT('Ctrl Pts',(-5.12345180751663,4.424075684855,151.470485885046));
#46501=CARTESIAN_POINT('Ctrl Pts',(-5.2331094156714,4.29032106532965,151.478654660556));
#46502=CARTESIAN_POINT('Ctrl Pts',(-5.34263232504818,4.1567307443341,151.486813401887));
#46503=CARTESIAN_POINT('Ctrl Pts',(-5.44718296239913,4.0187651788118,151.494972143218));
#46504=CARTESIAN_POINT('Ctrl Pts',(-5.54639079289593,3.87683352395732,151.503130884549));
#46505=CARTESIAN_POINT('Ctrl Pts',(-5.64547523653223,3.73507839248016,151.511279478683));
#46506=CARTESIAN_POINT('Ctrl Pts',(-5.7392299068261,3.58936729755277,151.519428072816));
#46507=CARTESIAN_POINT('Ctrl Pts',(-5.82732409670485,3.44014285633068,151.527576666949));
#46508=CARTESIAN_POINT('Ctrl Pts',(-5.91535540066671,3.29102493877173,151.53571944422));
#46509=CARTESIAN_POINT('Ctrl Pts',(-5.9977340828456,3.13839897948418,151.54386222149));
#46510=CARTESIAN_POINT('Ctrl Pts',(-6.07417207465694,2.98273743521916,151.552004998761));
#46511=CARTESIAN_POINT('Ctrl Pts',(-6.15056996188726,2.82715756161119,151.560143503776));
#46512=CARTESIAN_POINT('Ctrl Pts',(-6.22103320390696,2.66854560029287,151.56828200879));
#46513=CARTESIAN_POINT('Ctrl Pts',(-6.28531914140873,2.50739950758572,151.576420513805));
#46514=CARTESIAN_POINT('Ctrl Pts',(-6.34958351078944,2.34630747986649,151.584556288327));
#46515=CARTESIAN_POINT('Ctrl Pts',(-6.40767456819633,2.18268335226831,151.592692062849));
#46516=CARTESIAN_POINT('Ctrl Pts',(-6.45939737997885,2.01704598051764,151.600827837371));
#46517=CARTESIAN_POINT('Ctrl Pts',(-6.51112495630825,1.85139335076001,151.608964361336));
#46518=CARTESIAN_POINT('Ctrl Pts',(-6.55648299694826,1.68372745157347,151.617100885301));
#46519=CARTESIAN_POINT('Ctrl Pts',(-6.59532603339712,1.51458361049967,151.625237409265));
#46520=CARTESIAN_POINT('Ctrl Pts',(-6.63416951338339,1.34543783802121,151.633374026139));
#46521=CARTESIAN_POINT('Ctrl Pts',(-6.66649776433342,1.17481444681058,151.641510643012));
#46522=CARTESIAN_POINT('Ctrl Pts',(-6.69221627720592,1.00325983628379,151.649647259886));
#46523=CARTESIAN_POINT('Ctrl Pts',(-6.71795126802431,0.831595310086349,
151.65778908992));
#46524=CARTESIAN_POINT('Ctrl Pts',(-6.73706800780001,0.658998734044302,
151.665930919953));
#46525=CARTESIAN_POINT('Ctrl Pts',(-6.7495237187244,0.486023219997578,151.674072749987));
#46526=CARTESIAN_POINT('Ctrl Pts',(-6.76130708652667,0.322384699870326,
151.681775094595));
#46527=CARTESIAN_POINT('Ctrl Pts',(-6.76712953799064,0.158407349923215,
151.689477439202));
#46528=CARTESIAN_POINT('Ctrl Pts',(-6.7669978131403,-0.0054403082953369,
151.69717978381));
#46529=CARTESIAN_POINT('',(-6.767,9.16835936326781E-12,151.30282021619));
#46530=CARTESIAN_POINT('Ctrl Pts',(3.09917575053255,6.01559628526641,150.651392015123));
#46531=CARTESIAN_POINT('Ctrl Pts',(2.93382384459255,6.10078395293764,150.660141463035));
#46532=CARTESIAN_POINT('Ctrl Pts',(2.76495772122967,6.17915010267057,150.668890910947));
#46533=CARTESIAN_POINT('Ctrl Pts',(2.59315093316688,6.25042856433187,150.67764035886));
#46534=CARTESIAN_POINT('Ctrl Pts',(2.42134553245598,6.32170645041458,150.68638973612));
#46535=CARTESIAN_POINT('Ctrl Pts',(2.24659977927575,6.38589665313463,150.69513911338));
#46536=CARTESIAN_POINT('Ctrl Pts',(2.06950718689908,6.44278115439079,150.70388849064));
#46537=CARTESIAN_POINT('Ctrl Pts',(1.89241596572854,6.49966521519726,150.712637800154));
#46538=CARTESIAN_POINT('Ctrl Pts',(1.71297821457195,6.54924360009547,150.721387109669));
#46539=CARTESIAN_POINT('Ctrl Pts',(1.53180337335846,6.59134792173556,150.730136419184));
#46540=CARTESIAN_POINT('Ctrl Pts',(1.35062987477783,6.63345193135305,150.73888566386));
#46541=CARTESIAN_POINT('Ctrl Pts',(1.16771959102951,6.66808192368238,150.747634908536));
#46542=CARTESIAN_POINT('Ctrl Pts',(0.983693746906821,6.69512028363169,150.756384153212));
#46543=CARTESIAN_POINT('Ctrl Pts',(0.799669205419827,6.72215845218868,150.765133335956));
#46544=CARTESIAN_POINT('Ctrl Pts',(0.614529402873411,6.7416050542458,150.773882518701));
#46545=CARTESIAN_POINT('Ctrl Pts',(0.428903127363162,6.75339404354123,150.782631701445));
#46546=CARTESIAN_POINT('Ctrl Pts',(0.243278104163796,6.7651829533033,150.791380825163));
#46547=CARTESIAN_POINT('Ctrl Pts',(0.0571669005390366,6.76931433552276,
150.800129948882));
#46548=CARTESIAN_POINT('Ctrl Pts',(-0.128798404777591,6.76577415902473,
150.808879072601));
#46549=CARTESIAN_POINT('Ctrl Pts',(-0.314762517259159,6.76223400523441,
150.8176281402));
#46550=CARTESIAN_POINT('Ctrl Pts',(-0.500580446819552,6.75102239665089,
150.826377207799));
#46551=CARTESIAN_POINT('Ctrl Pts',(-0.685621118842636,6.73217741012497,
150.835126275398));
#46552=CARTESIAN_POINT('Ctrl Pts',(-0.870660665414486,6.71333253821772,
150.843875289784));
#46553=CARTESIAN_POINT('Ctrl Pts',(-1.05492267885483,6.68685441030613,150.85262430417));
#46554=CARTESIAN_POINT('Ctrl Pts',(-1.23778137635246,6.65283295028178,150.861373318555));
#46555=CARTESIAN_POINT('Ctrl Pts',(-1.42999922978828,6.61707018861869,150.870570128923));
#46556=CARTESIAN_POINT('Ctrl Pts',(-1.62066601233663,6.5729717293442,150.87976693929));
#46557=CARTESIAN_POINT('Ctrl Pts',(-1.8090662850034,6.52070304311307,150.888963749658));
#46558=CARTESIAN_POINT('Ctrl Pts',(-1.98831342545485,6.47097374915044,150.897713747395));
#46559=CARTESIAN_POINT('Ctrl Pts',(-2.16550875896661,6.41384933989542,150.906463745133));
#46560=CARTESIAN_POINT('Ctrl Pts',(-2.34005036713973,6.3495238624049,150.915213742871));
#46561=CARTESIAN_POINT('Ctrl Pts',(-2.51458843547051,6.28519968948611,150.923963563152));
#46562=CARTESIAN_POINT('Ctrl Pts',(-2.68647261718019,6.21367483971115,150.932713383433));
#46563=CARTESIAN_POINT('Ctrl Pts',(-2.85511905908695,6.1351922674386,150.941463203714));
#46564=CARTESIAN_POINT('Ctrl Pts',(-3.02376230488844,6.05671118252957,150.950212858172));
#46565=CARTESIAN_POINT('Ctrl Pts',(-3.1891676737986,5.97127275992657,150.958962512631));
#46566=CARTESIAN_POINT('Ctrl Pts',(-3.35077334102739,5.87916720438024,150.967712167089));
#46567=CARTESIAN_POINT('Ctrl Pts',(-3.51237616037319,5.78706327195673,150.976461667358));
#46568=CARTESIAN_POINT('Ctrl Pts',(-3.6701791630225,5.68829258362331,150.985211167626));
#46569=CARTESIAN_POINT('Ctrl Pts',(-3.82364636566412,5.58319061741077,150.993960667894));
#46570=CARTESIAN_POINT('Ctrl Pts',(-3.97711106778755,5.47809036367733,151.002710025603));
#46571=CARTESIAN_POINT('Ctrl Pts',(-4.12623987481892,5.36665920043252,151.011459383311));
#46572=CARTESIAN_POINT('Ctrl Pts',(-4.27052628213902,5.24927559512357,151.02020874102));
#46573=CARTESIAN_POINT('Ctrl Pts',(-4.41481053024948,5.13189374643062,151.028957967796));
#46574=CARTESIAN_POINT('Ctrl Pts',(-4.55425230136499,5.00855981477382,151.037707194573));
#46575=CARTESIAN_POINT('Ctrl Pts',(-4.68837800630515,4.87969268192109,151.046456421349));
#46576=CARTESIAN_POINT('Ctrl Pts',(-4.82250188228878,4.75082730631827,151.05520552882));
#46577=CARTESIAN_POINT('Ctrl Pts',(-4.95130963052965,4.61642907903527,151.063954636291));
#46578=CARTESIAN_POINT('Ctrl Pts',(-5.07436379033381,4.47695444731674,151.072703743762));
#46579=CARTESIAN_POINT('Ctrl Pts',(-5.19741643562819,4.3374815322057,151.081452743552));
#46580=CARTESIAN_POINT('Ctrl Pts',(-5.31471544462785,4.19293255254574,151.090201743341));
#46581=CARTESIAN_POINT('Ctrl Pts',(-5.42586245275639,4.04379841779588,151.098950743131));
#46582=CARTESIAN_POINT('Ctrl Pts',(-5.53702160019166,3.89464799484325,151.107700698473));
#46583=CARTESIAN_POINT('Ctrl Pts',(-5.64202723081266,3.74091164443829,151.116450653815));
#46584=CARTESIAN_POINT('Ctrl Pts',(-5.74052265232982,3.58311159163208,151.125200609158));
#46585=CARTESIAN_POINT('Ctrl Pts',(-5.83901427066933,3.42531763191758,151.13395022664));
#46586=CARTESIAN_POINT('Ctrl Pts',(-5.93099603115754,3.26346052695587,151.142699844122));
#46587=CARTESIAN_POINT('Ctrl Pts',(-6.01615550622767,3.0980900446705,151.151449461605));
#46588=CARTESIAN_POINT('Ctrl Pts',(-6.10131214578814,2.93272506863797,151.160198787756));
#46589=CARTESIAN_POINT('Ctrl Pts',(-6.17964682328764,2.76384720416858,151.168948113907));
#46590=CARTESIAN_POINT('Ctrl Pts',(-6.25089348288581,2.59203002791552,151.177697440058));
#46591=CARTESIAN_POINT('Ctrl Pts',(-6.32213814889342,2.42021765936998,151.18644652139));
#46592=CARTESIAN_POINT('Ctrl Pts',(-6.38629508412592,2.24546640831898,151.195195602721));
#46593=CARTESIAN_POINT('Ctrl Pts',(-6.44314639819815,2.06836976660032,151.203944684053));
#46594=CARTESIAN_POINT('Ctrl Pts',(-6.50000285283702,1.89125711158269,151.212694556487));
#46595=CARTESIAN_POINT('Ctrl Pts',(-6.5495522767325,1.7117989144025,151.221444428922));
#46596=CARTESIAN_POINT('Ctrl Pts',(-6.59162635926386,1.53060476278429,151.230194301356));
#46597=CARTESIAN_POINT('Ctrl Pts',(-6.63369752055195,1.34942319164703,151.238943566279));
#46598=CARTESIAN_POINT('Ctrl Pts',(-6.66829431424251,1.16650618642721,151.247692831201));
#46599=CARTESIAN_POINT('Ctrl Pts',(-6.69529923745413,0.982474997618827,
151.256442096124));
#46600=CARTESIAN_POINT('Ctrl Pts',(-6.7223055473144,0.798434359178024,151.265191810303));
#46601=CARTESIAN_POINT('Ctrl Pts',(-6.741719164967,0.61327970624063,151.273941524483));
#46602=CARTESIAN_POINT('Ctrl Pts',(-6.75347414817273,0.427639953655683,
151.282691238663));
#46603=CARTESIAN_POINT('Ctrl Pts',(-6.76248837758728,0.285283364201305,
151.289400897838));
#46604=CARTESIAN_POINT('Ctrl Pts',(-6.76699999999981,0.142641701110285,
151.296110557014));
#46605=CARTESIAN_POINT('Ctrl Pts',(-6.767,9.16835937808996E-12,151.30282021619));
#46606=CARTESIAN_POINT('Ctrl Pts',(-6.76699999999368,9.25253348153785E-6,
151.303021482695));
#46607=CARTESIAN_POINT('Ctrl Pts',(-6.76700023307113,-0.170455966723974,
151.311077178856));
#46608=CARTESIAN_POINT('Ctrl Pts',(-6.7605549706658,-0.341193029931809,
151.319132875017));
#46609=CARTESIAN_POINT('Ctrl Pts',(-6.74762845049654,-0.511663262360731,
151.327188571179));
#46610=CARTESIAN_POINT('Ctrl Pts',(-6.73471557880108,-0.681953503696206,
151.335235761728));
#46611=CARTESIAN_POINT('Ctrl Pts',(-6.7153350949022,-0.851977105275738,
151.343282952278));
#46612=CARTESIAN_POINT('Ctrl Pts',(-6.68950320557243,-1.02119335222872,
151.351330142828));
#46613=CARTESIAN_POINT('Ctrl Pts',(-6.66369290553083,-1.19026817482549,
151.359370607848));
#46614=CARTESIAN_POINT('Ctrl Pts',(-6.63144198725326,-1.35853661800618,
151.367411072869));
#46615=CARTESIAN_POINT('Ctrl Pts',(-6.59281860865363,-1.52546117400293,
151.37545153789));
#46616=CARTESIAN_POINT('Ctrl Pts',(-6.55421901968788,-1.69228291470446,
151.383487050477));
#46617=CARTESIAN_POINT('Ctrl Pts',(-6.50925486776001,-1.85776205259014,
151.391522563065));
#46618=CARTESIAN_POINT('Ctrl Pts',(-6.45804570416447,-2.02136950677575,
151.399558075652));
#46619=CARTESIAN_POINT('Ctrl Pts',(-6.40685048307061,-2.18493241625405,
151.407591400444));
#46620=CARTESIAN_POINT('Ctrl Pts',(-6.34941374018606,-2.34662429780411,
151.415624725237));
#46621=CARTESIAN_POINT('Ctrl Pts',(-6.28590539453114,-2.5059294425431,151.423658050029));
#46622=CARTESIAN_POINT('Ctrl Pts',(-6.22240468799061,-2.66521542523004,
151.431690408531));
#46623=CARTESIAN_POINT('Ctrl Pts',(-6.15283396955282,-2.82211489426953,
151.439722767033));
#46624=CARTESIAN_POINT('Ctrl Pts',(-6.07741190738215,-2.97613062683909,
151.447755125536));
#46625=CARTESIAN_POINT('Ctrl Pts',(-6.00198391720787,-3.13015846469711,
151.455788115363));
#46626=CARTESIAN_POINT('Ctrl Pts',(-5.92070383231666,-3.28130177849347,
151.46382110519));
#46627=CARTESIAN_POINT('Ctrl Pts',(-5.83383695003169,-3.42908667730126,
151.471854095018));
#46628=CARTESIAN_POINT('Ctrl Pts',(-5.74694596005494,-3.57691259004551,
151.479889314197));
#46629=CARTESIAN_POINT('Ctrl Pts',(-5.65446527656626,-3.72137791018506,
151.487924533376));
#46630=CARTESIAN_POINT('Ctrl Pts',(-5.55670421255499,-3.86203667695863,
151.495959752556));
#46631=CARTESIAN_POINT('Ctrl Pts',(-5.4588363892755,-4.0028490491288,151.504003746538));
#46632=CARTESIAN_POINT('Ctrl Pts',(-5.35567688177833,-4.13984625728533,
151.512047740521));
#46633=CARTESIAN_POINT('Ctrl Pts',(-5.24757659962024,-4.2726138172222,151.520091734503));
#46634=CARTESIAN_POINT('Ctrl Pts',(-5.13941661942993,-4.40545469761589,
151.528140170756));
#46635=CARTESIAN_POINT('Ctrl Pts',(-5.02631067726316,-4.53406099736127,
151.536188607008));
#46636=CARTESIAN_POINT('Ctrl Pts',(-4.90864705673056,-4.6580546446398,151.544237043261));
#46637=CARTESIAN_POINT('Ctrl Pts',(-4.79079680301249,-4.78224496553134,
151.552298245611));
#46638=CARTESIAN_POINT('Ctrl Pts',(-4.66837469570844,-4.90180775598046,
151.560359447961));
#46639=CARTESIAN_POINT('Ctrl Pts',(-4.54180352305622,-5.01640406645578,
151.568420650312));
#46640=CARTESIAN_POINT('Ctrl Pts',(-4.41788460963826,-5.12859904717882,
151.576312932694));
#46641=CARTESIAN_POINT('Ctrl Pts',(-4.28998908925523,-5.23603348263788,
151.584205215077));
#46642=CARTESIAN_POINT('Ctrl Pts',(-4.15853970958954,-5.33843015162388,
151.59209749746));
#46643=CARTESIAN_POINT('Ctrl Pts',(-4.02143734872161,-5.44523038985015,
151.600329187484));
#46644=CARTESIAN_POINT('Ctrl Pts',(-3.88001749945412,-5.5469018433012,151.608560877509));
#46645=CARTESIAN_POINT('Ctrl Pts',(-3.73469941990389,-5.64307622161615,
151.616792567533));
#46646=CARTESIAN_POINT('Ctrl Pts',(-3.58955421119695,-5.73913619058896,
151.625014465113));
#46647=CARTESIAN_POINT('Ctrl Pts',(-3.44052030213288,-5.82971190998977,
151.633236362693));
#46648=CARTESIAN_POINT('Ctrl Pts',(-3.28805023937711,-5.91447500826,151.641458260274));
#46649=CARTESIAN_POINT('Ctrl Pts',(-3.1357310102289,-5.99915425319096,151.649672024201));
#46650=CARTESIAN_POINT('Ctrl Pts',(-2.97998270806837,-6.07803215569456,
151.657885788129));
#46651=CARTESIAN_POINT('Ctrl Pts',(-2.82128717941016,-6.15082333117249,
151.666099552057));
#46652=CARTESIAN_POINT('Ctrl Pts',(-2.66271686202538,-6.22355707418303,
151.674306835299));
#46653=CARTESIAN_POINT('Ctrl Pts',(-2.5012042740145,-6.29021350692185,151.682514118542));
#46654=CARTESIAN_POINT('Ctrl Pts',(-2.33725628959949,-6.3505528922077,151.690721401784));
#46655=CARTESIAN_POINT('Ctrl Pts',(-2.17340483629631,-6.41085675020136,
151.698923852651));
#46656=CARTESIAN_POINT('Ctrl Pts',(-2.00712117853895,-6.46485084687705,
151.707126303518));
#46657=CARTESIAN_POINT('Ctrl Pts',(-1.8389327045801,-6.51234331926886,151.715328754385));
#46658=CARTESIAN_POINT('Ctrl Pts',(-1.67079343048949,-6.55982189877414,
151.723528805804));
#46659=CARTESIAN_POINT('Ctrl Pts',(-1.50075079345592,-6.60080254146056,
151.731728857223));
#46660=CARTESIAN_POINT('Ctrl Pts',(-1.32934814206397,-6.6351429914653,151.739928908642));
#46661=CARTESIAN_POINT('Ctrl Pts',(-1.15796877252919,-6.66947877695963,
151.748127846236));
#46662=CARTESIAN_POINT('Ctrl Pts',(-0.985230107706917,-6.69717609494801,
151.756326783831));
#46663=CARTESIAN_POINT('Ctrl Pts',(-0.811686528474478,-6.71814364087975,
151.764525721426));
#46664=CARTESIAN_POINT('Ctrl Pts',(-0.638135043440735,-6.7391121419909,
151.772725032524));
#46665=CARTESIAN_POINT('Ctrl Pts',(-0.463778926784342,-6.75335021722072,
151.780924343623));
#46666=CARTESIAN_POINT('Ctrl Pts',(-0.289178593508561,-6.76081834847354,
151.789123654721));
#46667=CARTESIAN_POINT('Ctrl Pts',(-0.114538636257731,-6.76828817455156,
151.797324826579));
#46668=CARTESIAN_POINT('Ctrl Pts',(0.06034528998886,-6.76898498131176,151.805525998438));
#46669=CARTESIAN_POINT('Ctrl Pts',(0.234911792673331,-6.76292136947215,
151.813727170296));
#46670=CARTESIAN_POINT('Ctrl Pts',(0.409642357685587,-6.75685205888588,
151.821936049838));
#46671=CARTESIAN_POINT('Ctrl Pts',(0.584054544452102,-6.74400964817368,
151.83014492938));
#46672=CARTESIAN_POINT('Ctrl Pts',(0.757590160048227,-6.72445879973981,
151.838353808921));
#46673=CARTESIAN_POINT('Ctrl Pts',(0.93120923168094,-6.70489854899208,151.846566636244));
#46674=CARTESIAN_POINT('Ctrl Pts',(1.10395053750502,-6.67862348196518,151.854779463566));
#46675=CARTESIAN_POINT('Ctrl Pts',(1.27526519165629,-6.64574959586576,151.862992290889));
#46676=CARTESIAN_POINT('Ctrl Pts',(1.44681431562433,-6.61283071691918,151.871216358698));
#46677=CARTESIAN_POINT('Ctrl Pts',(1.61693253645797,-6.57329505057456,151.879440426508));
#46678=CARTESIAN_POINT('Ctrl Pts',(1.78508407526776,-6.52730908140755,151.887664494317));
#46679=CARTESIAN_POINT('Ctrl Pts',(1.93663282517774,-6.48586363172575,151.895076541834));
#46680=CARTESIAN_POINT('Ctrl Pts',(2.08658411908769,-6.43917948131312,151.902488589351));
#46681=CARTESIAN_POINT('Ctrl Pts',(2.23455979943223,-6.38741195655654,151.909900636867));
#46682=CARTESIAN_POINT('Ctrl Pts',(2.40712446113371,-6.32704227029496,151.918544337435));
#46683=CARTESIAN_POINT('Ctrl Pts',(2.57739622972982,-6.25962118194966,151.927188038003));
#46684=CARTESIAN_POINT('Ctrl Pts',(2.74479281837802,-6.18533761278885,151.935831738571));
#46685=CARTESIAN_POINT('Ctrl Pts',(2.91197428131449,-6.11114950737562,151.944464330895));
#46686=CARTESIAN_POINT('Ctrl Pts',(3.07628765451557,-6.03011663009837,151.953096923219));
#46687=CARTESIAN_POINT('Ctrl Pts',(3.23716825738057,-5.94247681303071,151.961729515542));
#46688=CARTESIAN_POINT('Ctrl Pts',(3.40345588027828,-5.85189151814839,151.970652239794));
#46689=CARTESIAN_POINT('Ctrl Pts',(3.56607566392043,-5.75424753404614,151.979574964047));
#46690=CARTESIAN_POINT('Ctrl Pts',(3.72442631529256,-5.64986173476452,151.988497688299));
#46691=CARTESIAN_POINT('Ctrl Pts',(3.87720327285403,-5.5491501513976,151.997106346695));
#46692=CARTESIAN_POINT('Ctrl Pts',(4.02600619613065,-5.4421634199807,152.005715005091));
#46693=CARTESIAN_POINT('Ctrl Pts',(4.17031943446256,-5.32923304186858,152.014323663487));
#46694=CARTESIAN_POINT('Ctrl Pts',(4.31449624953625,-5.21640941993707,152.022924183882));
#46695=CARTESIAN_POINT('Ctrl Pts',(4.45419160182225,-5.09765354092595,152.031524704278));
#46696=CARTESIAN_POINT('Ctrl Pts',(4.58891927497414,-4.97333981221581,152.040125224673));
#46697=CARTESIAN_POINT('Ctrl Pts',(4.72349583075759,-4.84916552006763,152.04871609829));
#46698=CARTESIAN_POINT('Ctrl Pts',(4.8531155994263,-4.71944602131146,152.057306971907));
#46699=CARTESIAN_POINT('Ctrl Pts',(4.97732572854776,-4.58459568467456,152.065897845524));
#46700=CARTESIAN_POINT('Ctrl Pts',(4.99132318199891,-4.56939916790657,152.066865965873));
#46701=CARTESIAN_POINT('Ctrl Pts',(5.00525197158645,-4.55413753382398,152.067834086222));
#46702=CARTESIAN_POINT('Ctrl Pts',(5.01911147663452,-4.53881140664774,152.068802206571));
#46703=CARTESIAN_POINT('Ctrl Pts',(5.14232916496506,-4.40255473982118,152.077409263679));
#46704=CARTESIAN_POINT('Ctrl Pts',(5.25992018472983,-4.26136041845833,152.086016320786));
#46705=CARTESIAN_POINT('Ctrl Pts',(5.37151197477263,-4.11571963390052,152.094623377894));
#46706=CARTESIAN_POINT('Ctrl Pts',(5.48321209879413,-3.96993746039604,152.103238790784));
#46707=CARTESIAN_POINT('Ctrl Pts',(5.58890118275948,-3.81970044793657,152.111854203674));
#46708=CARTESIAN_POINT('Ctrl Pts',(5.68824976275295,-3.66552910731057,152.120469616565));
#46709=CARTESIAN_POINT('Ctrl Pts',(5.79129726639236,-3.5056176945325,152.129405796541));
#46710=CARTESIAN_POINT('Ctrl Pts',(5.8875228850268,-3.34147368997647,152.138341976516));
#46711=CARTESIAN_POINT('Ctrl Pts',(5.97661157035904,-3.17370495431609,152.147278156492));
#46712=CARTESIAN_POINT('Ctrl Pts',(6.06274189604705,-3.01150729937476,152.155917593575));
#46713=CARTESIAN_POINT('Ctrl Pts',(6.14220158827863,-2.84592206877392,152.164557030658));
#46714=CARTESIAN_POINT('Ctrl Pts',(6.21475528363058,-2.67751858342492,152.173196467741));
#46715=CARTESIAN_POINT('Ctrl Pts',(6.2910470338892,-2.50043874504311,152.182281019163));
#46716=CARTESIAN_POINT('Ctrl Pts',(6.35970227598654,-2.32024297721477,152.191365570586));
#46717=CARTESIAN_POINT('Ctrl Pts',(6.42050674934671,-2.13761130273804,152.200450122008));
#46718=CARTESIAN_POINT('Ctrl Pts',(6.48131122270687,-1.95497962826131,152.20953467343));
#46719=CARTESIAN_POINT('Ctrl Pts',(6.5342648734388,-1.76991243252498,152.218619224853));
#46720=CARTESIAN_POINT('Ctrl Pts',(6.57921538620068,-1.58310261890388,152.227703776275));
#46721=CARTESIAN_POINT('Ctrl Pts',(6.61984056596085,-1.41426845455237,152.235914172818));
#46722=CARTESIAN_POINT('Ctrl Pts',(6.6540176064454,-1.24364128244219,152.24412456936));
#46723=CARTESIAN_POINT('Ctrl Pts',(6.68158884294507,-1.07175535166938,152.252334965903));
#46724=CARTESIAN_POINT('Ctrl Pts',(6.70913081273306,-0.900051876840416,
152.260536647156));
#46725=CARTESIAN_POINT('Ctrl Pts',(6.7300808845267,-0.727092656219492,152.268738328409));
#46726=CARTESIAN_POINT('Ctrl Pts',(6.74433165425905,-0.553425277123611,
152.276940009663));
#46727=CARTESIAN_POINT('Ctrl Pts',(6.75857018037254,-0.379907105210154,
152.285134644401));
#46728=CARTESIAN_POINT('Ctrl Pts',(6.76612083765613,-0.205682343029822,
152.293329279139));
#46729=CARTESIAN_POINT('Ctrl Pts',(6.76692757997545,-0.0313069859245526,
152.301523913878));
#46730=CARTESIAN_POINT('Ctrl Pts',(6.76773379236648,0.142953828495147,152.309713165771));
#46731=CARTESIAN_POINT('Ctrl Pts',(6.76180491155083,0.317364682295511,152.317902417665));
#46732=CARTESIAN_POINT('Ctrl Pts',(6.74913685369885,0.491366187322597,152.326091669559));
#46733=CARTESIAN_POINT('Ctrl Pts',(6.73647455518912,0.665288585178814,152.334277198332));
#46734=CARTESIAN_POINT('Ctrl Pts',(6.71707920940525,0.838801646880461,152.342462727106));
#46735=CARTESIAN_POINT('Ctrl Pts',(6.69099880037581,1.01134764219304,152.350648255879));
#46736=CARTESIAN_POINT('Ctrl Pts',(6.66492049002162,1.18387975283048,152.358833125967));
#46737=CARTESIAN_POINT('Ctrl Pts',(6.63215823275973,1.35544459521934,152.367017996056));
#46738=CARTESIAN_POINT('Ctrl Pts',(6.59281174209825,1.52549084994028,152.375202866145));
#46739=CARTESIAN_POINT('Ctrl Pts',(6.55346549401829,1.69553605628104,152.383387685771));
#46740=CARTESIAN_POINT('Ctrl Pts',(6.50753517343739,1.86406234266953,152.391572505398));
#46741=CARTESIAN_POINT('Ctrl Pts',(6.45517133322181,2.03052999454611,152.399757325025));
#46742=CARTESIAN_POINT('Ctrl Pts',(6.40279822069086,2.19702712364512,152.407943593977));
#46743=CARTESIAN_POINT('Ctrl Pts',(6.34398942696614,2.36146454864155,152.416129862929));
#46744=CARTESIAN_POINT('Ctrl Pts',(6.27894496928143,2.52331905884599,152.42431613188));
#46745=CARTESIAN_POINT('Ctrl Pts',(6.21387707493509,2.68523188807598,152.432505350489));
#46746=CARTESIAN_POINT('Ctrl Pts',(6.1425691752523,2.84455961492315,152.440694569097));
#46747=CARTESIAN_POINT('Ctrl Pts',(6.0652688930922,3.00080026900961,152.448883787706));
#46748=CARTESIAN_POINT('Ctrl Pts',(5.98787905783168,3.15722192935625,152.457082493601));
#46749=CARTESIAN_POINT('Ctrl Pts',(5.90448313068335,3.31054904906628,152.465281199496));
#46750=CARTESIAN_POINT('Ctrl Pts',(5.81537457033345,3.46030455404131,152.47347990539));
#46751=CARTESIAN_POINT('Ctrl Pts',(5.72621270366357,3.61014964541337,152.481683515897));
#46752=CARTESIAN_POINT('Ctrl Pts',(5.63133158775056,3.75641856193982,152.489887126403));
#46753=CARTESIAN_POINT('Ctrl Pts',(5.53106716917532,3.89866451109492,152.498090736909));
#46754=CARTESIAN_POINT('Ctrl Pts',(5.43064447048977,4.04113501353463,152.506307297855));
#46755=CARTESIAN_POINT('Ctrl Pts',(5.32482170495855,4.17956957168957,152.514523858802));
#46756=CARTESIAN_POINT('Ctrl Pts',(5.21397499711123,4.31355465127068,152.522740419748));
#46757=CARTESIAN_POINT('Ctrl Pts',(5.11159675800477,4.43730353637919,152.530329251726));
#46758=CARTESIAN_POINT('Ctrl Pts',(5.00493346792305,4.55725707086845,152.537918083705));
#46759=CARTESIAN_POINT('Ctrl Pts',(4.89430773789984,4.67311895490942,152.545506915683));
#46760=CARTESIAN_POINT('Ctrl Pts',(4.77510884212814,4.79795979109479,152.553683859617));
#46761=CARTESIAN_POINT('Ctrl Pts',(4.65093988341982,4.9184364187114,152.56186080355));
#46762=CARTESIAN_POINT('Ctrl Pts',(4.52215398777142,5.03412478102034,152.570037747484));
#46763=CARTESIAN_POINT('Ctrl Pts',(4.39356713560064,5.14963434258532,152.578202053641));
#46764=CARTESIAN_POINT('Ctrl Pts',(4.26037783138535,5.26037014250751,152.586366359798));
#46765=CARTESIAN_POINT('Ctrl Pts',(4.12297796141772,5.36594276242897,152.594530665956));
#46766=CARTESIAN_POINT('Ctrl Pts',(3.98570080863105,5.47142109132739,152.602687680253));
#46767=CARTESIAN_POINT('Ctrl Pts',(3.84422085959967,5.57174519650159,152.61084469455));
#46768=CARTESIAN_POINT('Ctrl Pts',(3.69896574212059,5.66656345933038,152.619001708847));
#46769=CARTESIAN_POINT('Ctrl Pts',(3.55383767118573,5.76129878991671,152.627151588658));
#46770=CARTESIAN_POINT('Ctrl Pts',(3.40494131244847,5.85053767288747,152.63530146847));
#46771=CARTESIAN_POINT('Ctrl Pts',(3.25273593142272,5.93396983143929,152.643451348282));
#46772=CARTESIAN_POINT('Ctrl Pts',(3.20191196779873,5.96182924720193,152.646172731668));
#46773=CARTESIAN_POINT('Ctrl Pts',(3.15071929826171,5.9890415589112,152.648894115053));
#46774=CARTESIAN_POINT('Ctrl Pts',(3.0991757505326,6.01559628526638,152.651615498439));
#46775=CARTESIAN_POINT('Origin',(0.,0.,-3.69717978381041));
#46776=CARTESIAN_POINT('',(-6.76724014394675,0.000669971015295954,153.303235821163));
#46777=CARTESIAN_POINT('Ctrl Pts',(3.0991757505326,6.01559628526638,152.651615498439));
#46778=CARTESIAN_POINT('Ctrl Pts',(2.94492830563623,6.09506304435979,152.659759416587));
#46779=CARTESIAN_POINT('Ctrl Pts',(2.78753676423252,6.16863743062611,152.667903334736));
#46780=CARTESIAN_POINT('Ctrl Pts',(2.62749618569209,6.2360686970377,152.676047252884));
#46781=CARTESIAN_POINT('Ctrl Pts',(2.46748507374941,6.30348754803553,152.684189671578));
#46782=CARTESIAN_POINT('Ctrl Pts',(2.30482622857547,6.36476538464918,152.692332090272));
#46783=CARTESIAN_POINT('Ctrl Pts',(2.14003647277271,6.41969881654915,152.700474508966));
#46784=CARTESIAN_POINT('Ctrl Pts',(1.9752567367852,6.47462890829708,152.708616432572));
#46785=CARTESIAN_POINT('Ctrl Pts',(1.80834669322798,6.52321524757542,152.716758356177));
#46786=CARTESIAN_POINT('Ctrl Pts',(1.63984005988312,6.56530376890533,152.724900279783));
#46787=CARTESIAN_POINT('Ctrl Pts',(1.47131194816819,6.6073976549667,152.733043241182));
#46788=CARTESIAN_POINT('Ctrl Pts',(1.30118719458042,6.64299198541091,152.741186202582));
#46789=CARTESIAN_POINT('Ctrl Pts',(1.13001146939226,6.67198344415227,152.749329163982));
#46790=CARTESIAN_POINT('Ctrl Pts',(0.958781697811568,6.70098405654995,152.757474696411));
#46791=CARTESIAN_POINT('Ctrl Pts',(0.786500652576645,6.72337758510041,152.765620228839));
#46792=CARTESIAN_POINT('Ctrl Pts',(0.61372089513729,6.73911237945116,152.773765761268));
#46793=CARTESIAN_POINT('Ctrl Pts',(0.440760318609443,6.75486364072613,152.781919818235));
#46794=CARTESIAN_POINT('Ctrl Pts',(0.267300350225355,6.76394221637646,152.790073875202));
#46795=CARTESIAN_POINT('Ctrl Pts',(0.0938962172301893,6.76634853524335,
152.79822793217));
#46796=CARTESIAN_POINT('Ctrl Pts',(-0.0796068153495014,6.76875622653391,
152.806386639735));
#46797=CARTESIAN_POINT('Ctrl Pts',(-0.253053585947054,6.76448408648889,
152.814545347299));
#46798=CARTESIAN_POINT('Ctrl Pts',(-0.425892454205106,6.75358457542742,
152.822704054864));
#46799=CARTESIAN_POINT('Ctrl Pts',(-0.598973669275219,6.74266978156651,
152.830874202199));
#46800=CARTESIAN_POINT('Ctrl Pts',(-0.771444917987083,6.72510909096235,
152.839044349533));
#46801=CARTESIAN_POINT('Ctrl Pts',(-0.942762205668032,6.70100652316978,
152.847214496867));
#46802=CARTESIAN_POINT('Ctrl Pts',(-1.05526312990229,6.68517880846691,152.852579682942));
#46803=CARTESIAN_POINT('Ctrl Pts',(-1.16726664649183,6.66653108608735,152.857944869016));
#46804=CARTESIAN_POINT('Ctrl Pts',(-1.27862215391275,6.64510454300935,152.863310055091));
#46805=CARTESIAN_POINT('Ctrl Pts',(-1.44960357757298,6.61220504010695,152.87154805943));
#46806=CARTESIAN_POINT('Ctrl Pts',(-1.61954544372369,6.57265771547668,152.879786063768));
#46807=CARTESIAN_POINT('Ctrl Pts',(-1.78789346599803,6.5265401212466,152.888024068107));
#46808=CARTESIAN_POINT('Ctrl Pts',(-1.95605633052642,6.4804732495001,152.896253011868));
#46809=CARTESIAN_POINT('Ctrl Pts',(-2.12262850043843,6.42785059227623,152.904481955629));
#46810=CARTESIAN_POINT('Ctrl Pts',(-2.28706429538294,6.36880097889583,152.91271089939));
#46811=CARTESIAN_POINT('Ctrl Pts',(-2.45135192060478,6.3098045739111,152.920932428218));
#46812=CARTESIAN_POINT('Ctrl Pts',(-2.61350667061379,6.24439286696381,152.929153957047));
#46813=CARTESIAN_POINT('Ctrl Pts',(-2.77299638335608,6.17274493705143,152.937375485875));
#46814=CARTESIAN_POINT('Ctrl Pts',(-2.93237407528811,6.10114733050489,152.945591240147));
#46815=CARTESIAN_POINT('Ctrl Pts',(-3.08909013388998,6.02332237190325,152.95380699442));
#46816=CARTESIAN_POINT('Ctrl Pts',(-3.24263070343066,5.93949788460008,152.962022748692));
#46817=CARTESIAN_POINT('Ctrl Pts',(-3.39609393362528,5.85571562021592,152.970234364637));
#46818=CARTESIAN_POINT('Ctrl Pts',(-3.54638454856016,5.76594001872067,152.978445980583));
#46819=CARTESIAN_POINT('Ctrl Pts',(-3.69301161604868,5.67044567946202,152.986657596528));
#46820=CARTESIAN_POINT('Ctrl Pts',(-3.83961411264868,5.5749673425746,152.99486783642));
#46821=CARTESIAN_POINT('Ctrl Pts',(-3.98255398204806,5.47377236626722,153.003078076312));
#46822=CARTESIAN_POINT('Ctrl Pts',(-4.12136742791459,5.36717984831184,153.011288316203));
#46823=CARTESIAN_POINT('Ctrl Pts',(-4.26017257550486,5.26059370246369,153.019498065287));
#46824=CARTESIAN_POINT('Ctrl Pts',(-4.39485150688813,5.14861087458011,153.02770781437));
#46825=CARTESIAN_POINT('Ctrl Pts',(-4.52497185228122,5.03159206773191,153.035917563453));
#46826=CARTESIAN_POINT('Ctrl Pts',(-4.65510784230526,4.9145591914771,153.044128299611));
#46827=CARTESIAN_POINT('Ctrl Pts',(-4.78068388857562,4.79248936891971,153.052339035768));
#46828=CARTESIAN_POINT('Ctrl Pts',(-4.90130292896311,4.66578167068902,153.060549771926));
#46829=CARTESIAN_POINT('Ctrl Pts',(-5.02195818455962,4.53903592916301,153.068762973313));
#46830=CARTESIAN_POINT('Ctrl Pts',(-5.13765322320199,4.40764979685971,153.076976174699));
#46831=CARTESIAN_POINT('Ctrl Pts',(-5.24802983011563,4.27205710427852,153.085189376086));
#46832=CARTESIAN_POINT('Ctrl Pts',(-5.35852196341923,4.1363224927281,153.093411173873));
#46833=CARTESIAN_POINT('Ctrl Pts',(-5.4636843178522,3.99637280217192,153.10163297166));
#46834=CARTESIAN_POINT('Ctrl Pts',(-5.56320016391786,3.85267347905118,153.109854769447));
#46835=CARTESIAN_POINT('Ctrl Pts',(-5.66276990172245,3.70889633710346,153.11808101966));
#46836=CARTESIAN_POINT('Ctrl Pts',(-5.75668684323546,3.56136581550566,153.126307269874));
#46837=CARTESIAN_POINT('Ctrl Pts',(-5.84467922020521,3.41057382457871,153.134533520087));
#46838=CARTESIAN_POINT('Ctrl Pts',(-5.93279963002372,3.25956242455254,153.142771739863));
#46839=CARTESIAN_POINT('Ctrl Pts',(-6.01497807970119,3.10528038679674,153.151009959638));
#46840=CARTESIAN_POINT('Ctrl Pts',(-6.09098957038893,2.94824270598831,153.159248179414));
#46841=CARTESIAN_POINT('Ctrl Pts',(-6.15823680080461,2.80931174950108,153.166536517775));
#46842=CARTESIAN_POINT('Ctrl Pts',(-6.22065785029642,2.66822442975674,153.173824856137));
#46843=CARTESIAN_POINT('Ctrl Pts',(-6.2781292976951,2.52534780207054,153.181113194498));
#46844=CARTESIAN_POINT('Ctrl Pts',(-6.3504164459868,2.34563866926717,153.190280410912));
#46845=CARTESIAN_POINT('Ctrl Pts',(-6.41505133711675,2.16265535962499,153.199447627326));
#46846=CARTESIAN_POINT('Ctrl Pts',(-6.47175761011487,1.9770286886943,153.20861484374));
#46847=CARTESIAN_POINT('Ctrl Pts',(-6.52820740822629,1.79224158236338,153.21774059806));
#46848=CARTESIAN_POINT('Ctrl Pts',(-6.57680004080532,1.60483515921502,153.22686635238));
#46849=CARTESIAN_POINT('Ctrl Pts',(-6.61730875284526,1.41545535765617,153.235992106701));
#46850=CARTESIAN_POINT('Ctrl Pts',(-6.65769786423432,1.22663469378369,153.245090917529));
#46851=CARTESIAN_POINT('Ctrl Pts',(-6.69005060763174,1.03585247477288,153.254189728358));
#46852=CARTESIAN_POINT('Ctrl Pts',(-6.71418957826771,0.843769700262641,
153.263288539186));
#46853=CARTESIAN_POINT('Ctrl Pts',(-6.73821397325754,0.652598646816766,
153.272344162501));
#46854=CARTESIAN_POINT('Ctrl Pts',(-6.75410229271552,0.460139554458451,
153.281399785815));
#46855=CARTESIAN_POINT('Ctrl Pts',(-6.76172810895751,0.267061754158045,
153.29045540913));
#46856=CARTESIAN_POINT('Ctrl Pts',(-6.76519894482116,0.179183770675106,
153.294577011483));
#46857=CARTESIAN_POINT('Ctrl Pts',(-6.76695883519318,0.0911778433954226,
153.298698613836));
#46858=CARTESIAN_POINT('Ctrl Pts',(-6.76699928620785,0.00310812845892864,
153.302820216189));
#46859=CARTESIAN_POINT('',(3.92888236737299,-5.50964357679747,154.));
#46860=CARTESIAN_POINT('Ctrl Pts',(-6.767,9.31121846292626E-12,153.30282021619));
#46861=CARTESIAN_POINT('Ctrl Pts',(-6.76700000000026,-0.186008656853188,
153.3115697942));
#46862=CARTESIAN_POINT('Ctrl Pts',(-6.75932625676188,-0.37201717040645,
153.32031937221));
#46863=CARTESIAN_POINT('Ctrl Pts',(-6.7440048348797,-0.557393745138262,
153.329068950221));
#46864=CARTESIAN_POINT('Ctrl Pts',(-6.72868354559113,-0.742768715596703,
153.337818452511));
#46865=CARTESIAN_POINT('Ctrl Pts',(-6.70571473370896,-0.927511472541724,
153.346567954801));
#46866=CARTESIAN_POINT('Ctrl Pts',(-6.67517641362661,-1.11099453057292,
153.355317457091));
#46867=CARTESIAN_POINT('Ctrl Pts',(-6.64463834768126,-1.29447606167556,
153.364066886569));
#46868=CARTESIAN_POINT('Ctrl Pts',(-6.60653094664505,-1.47669763213353,
153.372816316047));
#46869=CARTESIAN_POINT('Ctrl Pts',(-6.56098364152038,-1.65704033013745,
153.381565745524));
#46870=CARTESIAN_POINT('Ctrl Pts',(-6.51543670030484,-1.83738158725801,
153.390315105097));
#46871=CARTESIAN_POINT('Ctrl Pts',(-6.46245004412932,-2.01584372410336,
153.399064464669));
#46872=CARTESIAN_POINT('Ctrl Pts',(-6.40220363820689,-2.19182060737882,
153.407813824241));
#46873=CARTESIAN_POINT('Ctrl Pts',(-6.34195769362181,-2.36779614310984,
153.416563116816));
#46874=CARTESIAN_POINT('Ctrl Pts',(-6.27445220335668,-2.54128619222773,
153.42531240939));
#46875=CARTESIAN_POINT('Ctrl Pts',(-6.19991644125039,-2.71170151777682,
153.434061701964));
#46876=CARTESIAN_POINT('Ctrl Pts',(-6.12538122514392,-2.88211559497567,
153.442810930446));
#46877=CARTESIAN_POINT('Ctrl Pts',(-6.04381595508577,-3.04945473112789,
153.451560158929));
#46878=CARTESIAN_POINT('Ctrl Pts',(-5.95549765311986,-3.213150588392,153.460309387411));
#46879=CARTESIAN_POINT('Ctrl Pts',(-5.86717996878046,-3.37684530090017,
153.469058554709));
#46880=CARTESIAN_POINT('Ctrl Pts',(-5.77210948310036,-3.53689653331464,
153.477807722007));
#46881=CARTESIAN_POINT('Ctrl Pts',(-5.67060908169332,-3.69276070746769,
153.486556889304));
#46882=CARTESIAN_POINT('Ctrl Pts',(-5.5691093563862,-3.84862384340065,153.495305998323));
#46883=CARTESIAN_POINT('Ctrl Pts',(-5.46117995742809,-4.00029973676548,
153.504055107342));
#46884=CARTESIAN_POINT('Ctrl Pts',(-5.34718743797362,-4.14727326121358,
153.512804216361));
#46885=CARTESIAN_POINT('Ctrl Pts',(-5.23319563997062,-4.2942458554755,153.521553270007));
#46886=CARTESIAN_POINT('Ctrl Pts',(-5.11314097386879,-4.43651591395998,
153.530302323653));
#46887=CARTESIAN_POINT('Ctrl Pts',(-4.98743116787335,-4.57360026081483,
153.5390513773));
#46888=CARTESIAN_POINT('Ctrl Pts',(-4.86172211573906,-4.71068378559727,
153.547800378479));
#46889=CARTESIAN_POINT('Ctrl Pts',(-4.73035818522944,-4.84258144980424,
153.556549379659));
#46890=CARTESIAN_POINT('Ctrl Pts',(-4.5937855075914,-4.96884530955063,153.565298380838));
#46891=CARTESIAN_POINT('Ctrl Pts',(-4.45241612228613,-5.09954381050499,
153.574354664571));
#46892=CARTESIAN_POINT('Ctrl Pts',(-4.30546569332165,-5.22420535248028,
153.583410948304));
#46893=CARTESIAN_POINT('Ctrl Pts',(-4.15346891903191,-5.34237633816974,
153.592467232036));
#46894=CARTESIAN_POINT('Ctrl Pts',(-4.00661345260036,-5.45655017707648,
153.60121718596));
#46895=CARTESIAN_POINT('Ctrl Pts',(-3.85504768195733,-5.56466517980614,
153.609967139885));
#46896=CARTESIAN_POINT('Ctrl Pts',(-3.69928645877247,-5.66635409200155,
153.618717093809));
#46897=CARTESIAN_POINT('Ctrl Pts',(-3.54352834466741,-5.76804097443025,
153.627466873079));
#46898=CARTESIAN_POINT('Ctrl Pts',(-3.38357518563572,-5.86330186629665,
153.63621665235));
#46899=CARTESIAN_POINT('Ctrl Pts',(-3.21997030268213,-5.95181319009974,
153.64496643162));
#46900=CARTESIAN_POINT('Ctrl Pts',(-3.05636846790294,-6.0403228648203,153.653716047871));
#46901=CARTESIAN_POINT('Ctrl Pts',(-2.88911529745392,-6.12208308673445,
153.662465664121));
#46902=CARTESIAN_POINT('Ctrl Pts',(-2.71877888751091,-6.19681614708916,
153.671215280372));
#46903=CARTESIAN_POINT('Ctrl Pts',(-2.548445424774,-6.27154791439248,153.679964745234));
#46904=CARTESIAN_POINT('Ctrl Pts',(-2.37502909175458,-6.33925264829314,
153.688714210096));
#46905=CARTESIAN_POINT('Ctrl Pts',(-2.1991188982138,-6.3997003891994,153.697463674959));
#46906=CARTESIAN_POINT('Ctrl Pts',(-2.02321151455511,-6.46014716455032,
153.706213000062));
#46907=CARTESIAN_POINT('Ctrl Pts',(-1.84481062111901,-6.5133370857405,153.714962325166));
#46908=CARTESIAN_POINT('Ctrl Pts',(-1.66452213842223,-6.55908949860438,
153.72371165027));
#46909=CARTESIAN_POINT('Ctrl Pts',(-1.48423629599081,-6.60484124143928,
153.732460847242));
#46910=CARTESIAN_POINT('Ctrl Pts',(-1.30206319737382,-6.64315562342162,
153.741210044215));
#46911=CARTESIAN_POINT('Ctrl Pts',(-1.11862155689613,-6.67390251745164,
153.749959241188));
#46912=CARTESIAN_POINT('Ctrl Pts',(-0.935182359145258,-6.704649002053,153.758708321655));
#46913=CARTESIAN_POINT('Ctrl Pts',(-0.750474935937235,-6.72782815298643,
153.767457402123));
#46914=CARTESIAN_POINT('Ctrl Pts',(-0.565126592231362,-6.74336124901766,
153.77620648259));
#46915=CARTESIAN_POINT('Ctrl Pts',(-0.379780470417673,-6.75889415884347,
153.784955458177));
#46916=CARTESIAN_POINT('Ctrl Pts',(-0.193793729005098,-6.76678117325788,
153.793704433763));
#46917=CARTESIAN_POINT('Ctrl Pts',(-0.00779800265608266,-6.7669955069554,
153.80245340935));
#46918=CARTESIAN_POINT('Ctrl Pts',(0.17821673193395,-6.76720986255722,153.811203279057));
#46919=CARTESIAN_POINT('Ctrl Pts',(0.364240166675858,-6.75974996789178,
153.819953148765));
#46920=CARTESIAN_POINT('Ctrl Pts',(0.549640413288921,-6.74464116288477,
153.828703018472));
#46921=CARTESIAN_POINT('Ctrl Pts',(0.735033738525658,-6.72953292192083,
153.837452561528));
#46922=CARTESIAN_POINT('Ctrl Pts',(0.91980363650705,-6.70677636530813,153.846202104585));
#46923=CARTESIAN_POINT('Ctrl Pts',(1.10332252380503,-6.67644878722697,153.854951647641));
#46924=CARTESIAN_POINT('Ctrl Pts',(1.28683553553499,-6.64612218011807,153.863700910571));
#46925=CARTESIAN_POINT('Ctrl Pts',(1.46909733398482,-6.60822508332242,153.872450173501));
#46926=CARTESIAN_POINT('Ctrl Pts',(1.64948889425487,-6.56288620865316,153.881199436431));
#46927=CARTESIAN_POINT('Ctrl Pts',(1.82987563779965,-6.51754854459987,153.889948465742));
#46928=CARTESIAN_POINT('Ctrl Pts',(2.00839196519895,-6.46476957015119,153.898697495054));
#46929=CARTESIAN_POINT('Ctrl Pts',(2.18443160482961,-6.4047285316258,153.907446524365));
#46930=CARTESIAN_POINT('Ctrl Pts',(2.3604849227005,-6.34468282792527,153.916196233474));
#46931=CARTESIAN_POINT('Ctrl Pts',(2.53406089643084,-6.27737402346287,153.924945942583));
#46932=CARTESIAN_POINT('Ctrl Pts',(2.70456994115639,-6.20303074580429,153.933695651692));
#46933=CARTESIAN_POINT('Ctrl Pts',(2.87506802043528,-6.12869224916626,153.942444798107));
#46934=CARTESIAN_POINT('Ctrl Pts',(3.04249930269661,-6.04732029912513,153.951193944521));
#46935=CARTESIAN_POINT('Ctrl Pts',(3.20629514779787,-5.9591912559682,153.959943090936));
#46936=CARTESIAN_POINT('Ctrl Pts',(3.37009610080391,-5.871059464544,153.968692510189));
#46937=CARTESIAN_POINT('Ctrl Pts',(3.53026113741014,-5.77617029410984,153.977441929442));
#46938=CARTESIAN_POINT('Ctrl Pts',(3.68624626164006,-5.67484603302545,153.986191348695));
#46939=CARTESIAN_POINT('Ctrl Pts',(3.76830672481212,-5.62154148981211,153.990794232464));
#46940=CARTESIAN_POINT('Ctrl Pts',(3.84921079545831,-5.56645673171636,153.995397116232));
#46941=CARTESIAN_POINT('Ctrl Pts',(3.92888236737299,-5.50964357679747,154.));
#46942=CARTESIAN_POINT('',(-3.92888236737363,-5.50964357679701,154.));
#46943=CARTESIAN_POINT('Origin',(0.,0.,154.));
#46944=CARTESIAN_POINT('',(-6.76699995627346,0.000769282111940907,153.697179783839));
#46945=CARTESIAN_POINT('Ctrl Pts',(-6.76699995627346,0.000769282111748204,
153.697179783839));
#46946=CARTESIAN_POINT('Ctrl Pts',(-6.76701947092661,-0.170891614425859,
153.705273779468));
#46947=CARTESIAN_POINT('Ctrl Pts',(-6.76050280836558,-0.342746040058435,
153.713367775097));
#46948=CARTESIAN_POINT('Ctrl Pts',(-6.74743188915907,-0.514248870839024,
153.721461770727));
#46949=CARTESIAN_POINT('Ctrl Pts',(-6.73437014253476,-0.685631348659959,
153.729550086355));
#46950=CARTESIAN_POINT('Ctrl Pts',(-6.7147633219503,-0.856662354601882,
153.737638401983));
#46951=CARTESIAN_POINT('Ctrl Pts',(-6.68864541020004,-1.02679675525875,
153.745726717611));
#46952=CARTESIAN_POINT('Ctrl Pts',(-6.66253954073297,-1.19685271141162,
153.753811303929));
#46953=CARTESIAN_POINT('Ctrl Pts',(-6.62992861067414,-1.36601251921381,
153.761895890246));
#46954=CARTESIAN_POINT('Ctrl Pts',(-6.59089844295224,-1.53373619462076,
153.769980476564));
#46955=CARTESIAN_POINT('Ctrl Pts',(-6.55187966162554,-1.70141093946542,
153.77806270434));
#46956=CARTESIAN_POINT('Ctrl Pts',(-6.50644545638599,-1.86765002537015,
153.786144932116));
#46957=CARTESIAN_POINT('Ctrl Pts',(-6.45473272074018,-2.03192384301332,
153.794227159892));
#46958=CARTESIAN_POINT('Ctrl Pts',(-6.40301193775555,-2.19622322432188,
153.802310645393));
#46959=CARTESIAN_POINT('Ctrl Pts',(-6.3450107770592,-2.35855637023451,153.810394130895));
#46960=CARTESIAN_POINT('Ctrl Pts',(-6.28091605110546,-2.51840873548472,
153.818477616396));
#46961=CARTESIAN_POINT('Ctrl Pts',(-6.22169455239901,-2.66610726295361,
153.825946501223));
#46962=CARTESIAN_POINT('Ctrl Pts',(-6.15727148173902,-2.81168785811568,
153.83341538605));
#46963=CARTESIAN_POINT('Ctrl Pts',(-6.08783061025201,-2.95476013592959,
153.840884270877));
#46964=CARTESIAN_POINT('Ctrl Pts',(-5.99896118095524,-3.13786198078316,
153.850442842332));
#46965=CARTESIAN_POINT('Ctrl Pts',(-5.901916903247,-3.3167679087119,153.860001413788));
#46966=CARTESIAN_POINT('Ctrl Pts',(-5.79710256826938,-3.49082953077983,
153.869559985244));
#46967=CARTESIAN_POINT('Ctrl Pts',(-5.69197696941553,-3.66540805824244,
153.879146942492));
#46968=CARTESIAN_POINT('Ctrl Pts',(-5.57903518394445,-3.83511339336938,
153.888733899741));
#46969=CARTESIAN_POINT('Ctrl Pts',(-5.45872656148091,-3.99932410876923,
153.89832085699));
#46970=CARTESIAN_POINT('Ctrl Pts',(-5.33816688849719,-4.16387748610534,
153.907927819542));
#46971=CARTESIAN_POINT('Ctrl Pts',(-5.2102096778897,-4.32291321352696,153.917534782095));
#46972=CARTESIAN_POINT('Ctrl Pts',(-5.07534690357434,-4.47583989977058,
153.927141744648));
#46973=CARTESIAN_POINT('Ctrl Pts',(-4.94048239335081,-4.62876855443496,
153.936748830859));
#46974=CARTESIAN_POINT('Ctrl Pts',(-4.79871221545128,-4.77558793666736,
153.946355917069));
#46975=CARTESIAN_POINT('Ctrl Pts',(-4.65056698131552,-4.91574162790294,
153.955963003279));
#46976=CARTESIAN_POINT('Ctrl Pts',(-4.50269287672303,-5.05563881540073,
153.965552506981));
#46977=CARTESIAN_POINT('Ctrl Pts',(-4.34846710060624,-5.18889461150784,
153.975142010682));
#46978=CARTESIAN_POINT('Ctrl Pts',(-4.18845473229509,-5.31499162327796,
153.984731514384));
#46979=CARTESIAN_POINT('Ctrl Pts',(-4.1035304018323,-5.38191585176705,153.989821009589));
#46980=CARTESIAN_POINT('Ctrl Pts',(-4.01697672380024,-5.44682420222127,
153.994910504795));
#46981=CARTESIAN_POINT('Ctrl Pts',(-3.92888236737363,-5.50964357679701,
154.));
#46982=CARTESIAN_POINT('Ctrl Pts',(3.09917575053261,6.01559628526638,153.045781927116));
#46983=CARTESIAN_POINT('Ctrl Pts',(2.94639732302355,6.09430622112099,153.053915280607));
#46984=CARTESIAN_POINT('Ctrl Pts',(2.79037452573701,6.16731781408541,153.062048634097));
#46985=CARTESIAN_POINT('Ctrl Pts',(2.63157606100013,6.23434811629661,153.070181987587));
#46986=CARTESIAN_POINT('Ctrl Pts',(2.47296115830906,6.30130093526874,153.078305939381));
#46987=CARTESIAN_POINT('Ctrl Pts',(2.31157730937803,6.36228608395666,153.086429891174));
#46988=CARTESIAN_POINT('Ctrl Pts',(2.14791895551187,6.41706577499038,153.094553842968));
#46989=CARTESIAN_POINT('Ctrl Pts',(1.98441500867196,6.47179378293556,153.102670130043));
#46990=CARTESIAN_POINT('Ctrl Pts',(1.81864117473825,6.52032787233376,153.110786417118));
#46991=CARTESIAN_POINT('Ctrl Pts',(1.65111305741791,6.56247778446709,153.118902704193));
#46992=CARTESIAN_POINT('Ctrl Pts',(1.48370742648437,6.60459687914409,153.127013057131));
#46993=CARTESIAN_POINT('Ctrl Pts',(1.31455042063434,6.64034100076727,153.13512341007));
#46994=CARTESIAN_POINT('Ctrl Pts',(1.14417401210083,6.66956931368384,153.143233763009));
#46995=CARTESIAN_POINT('Ctrl Pts',(0.973886012015048,6.69878246000665,153.151339907479));
#46996=CARTESIAN_POINT('Ctrl Pts',(0.802380230570611,6.72148646861295,153.159446051949));
#46997=CARTESIAN_POINT('Ctrl Pts',(0.630200046847709,6.73759132783765,153.16755219642));
#46998=CARTESIAN_POINT('Ctrl Pts',(0.456747704672164,6.75381517829787,153.175718233382));
#46999=CARTESIAN_POINT('Ctrl Pts',(0.282611322577518,6.76334188447178,153.183884270344));
#47000=CARTESIAN_POINT('Ctrl Pts',(0.108353414412268,6.76613246527033,153.192050307306));
#47001=CARTESIAN_POINT('Ctrl Pts',(-0.0645940545419908,6.76890206058514,
153.200154934744));
#47002=CARTESIAN_POINT('Ctrl Pts',(-0.237660855314371,6.76503651809403,
153.208259562183));
#47003=CARTESIAN_POINT('Ctrl Pts',(-0.410295751295052,6.7545500513705,153.216364189622));
#47004=CARTESIAN_POINT('Ctrl Pts',(-0.582956388774257,6.74406202101543,
153.224470025538));
#47005=CARTESIAN_POINT('Ctrl Pts',(-0.755184626184368,6.72695112247535,
153.232575861453));
#47006=CARTESIAN_POINT('Ctrl Pts',(-0.926433189663243,6.70328356442501,
153.240681697369));
#47007=CARTESIAN_POINT('Ctrl Pts',(-1.0977402072223,6.67960792767719,153.248790300135));
#47008=CARTESIAN_POINT('Ctrl Pts',(-1.26806652102535,6.64937122536387,153.256898902901));
#47009=CARTESIAN_POINT('Ctrl Pts',(-1.43687397087053,6.6126909947339,153.265007505667));
#47010=CARTESIAN_POINT('Ctrl Pts',(-1.60780895651683,6.57554847109535,153.273218303821));
#47011=CARTESIAN_POINT('Ctrl Pts',(-1.77718615438182,6.53179898737637,153.281429101974));
#47012=CARTESIAN_POINT('Ctrl Pts',(-1.94446249311462,6.48161666660953,153.289639900127));
#47013=CARTESIAN_POINT('Ctrl Pts',(-2.10995223596933,6.43197031840232,153.297763002804));
#47014=CARTESIAN_POINT('Ctrl Pts',(-2.27338545253408,6.37602805559977,153.305886105482));
#47015=CARTESIAN_POINT('Ctrl Pts',(-2.43425670380338,6.31400691320403,153.314009208159));
#47016=CARTESIAN_POINT('Ctrl Pts',(-2.59773305835091,6.25098141807217,153.32226385405));
#47017=CARTESIAN_POINT('Ctrl Pts',(-2.75856339751926,6.181678644642,153.330518499941));
#47018=CARTESIAN_POINT('Ctrl Pts',(-2.91624400533904,6.10637453005662,153.338773145833));
#47019=CARTESIAN_POINT('Ctrl Pts',(-3.07392461315882,6.03107041547123,153.347027791724));
#47020=CARTESIAN_POINT('Ctrl Pts',(-3.22845517768015,5.94976520392367,153.355282437615));
#47021=CARTESIAN_POINT('Ctrl Pts',(-3.37936374480091,5.86278003001351,153.363537083506));
#47022=CARTESIAN_POINT('Ctrl Pts',(-3.53143289885957,5.77512588244229,153.371855213098));
#47023=CARTESIAN_POINT('Ctrl Pts',(-3.68029464888091,5.68143320994216,153.380173342689));
#47024=CARTESIAN_POINT('Ctrl Pts',(-3.82544302852417,5.58195974864705,153.38849147228));
#47025=CARTESIAN_POINT('Ctrl Pts',(-3.97041383648347,5.48260798123564,153.396799425634));
#47026=CARTESIAN_POINT('Ctrl Pts',(-4.11168003741536,5.37748970785892,153.405107378989));
#47027=CARTESIAN_POINT('Ctrl Pts',(-4.24876047979325,5.26690833272681,153.413415332343));
#47028=CARTESIAN_POINT('Ctrl Pts',(-4.38569876832377,5.15644163163315,153.421714670263));
#47029=CARTESIAN_POINT('Ctrl Pts',(-4.51845967542282,5.04052333296863,153.430014008184));
#47030=CARTESIAN_POINT('Ctrl Pts',(-4.64659109393952,4.91949999549974,153.438313346104));
#47031=CARTESIAN_POINT('Ctrl Pts',(-4.77461350413703,4.79857961912153,153.446605623329));
#47032=CARTESIAN_POINT('Ctrl Pts',(-4.89801402012995,4.67256309620952,153.454897900554));
#47033=CARTESIAN_POINT('Ctrl Pts',(-5.01637354724699,4.54183723117425,153.463190177779));
#47034=CARTESIAN_POINT('Ctrl Pts',(-5.13465441379185,4.41119824525717,153.471476944039));
#47035=CARTESIAN_POINT('Ctrl Pts',(-5.24790073360115,4.27585641233802,153.479763710298));
#47036=CARTESIAN_POINT('Ctrl Pts',(-5.35573009431797,4.13623550548284,153.488050476558));
#47037=CARTESIAN_POINT('Ctrl Pts',(-5.46351089017542,3.99667748196166,153.496333510572));
#47038=CARTESIAN_POINT('Ctrl Pts',(-5.56587937520239,3.85284450095779,153.504616544586));
#47039=CARTESIAN_POINT('Ctrl Pts',(-5.66249312863783,3.7051937288257,153.512899578601));
#47040=CARTESIAN_POINT('Ctrl Pts',(-5.75908395288089,3.55757799842255,153.521180646815));
#47041=CARTESIAN_POINT('Ctrl Pts',(-5.84992257501593,3.40614657410768,153.52946171503));
#47042=CARTESIAN_POINT('Ctrl Pts',(-5.93470952527804,3.25138614295106,153.537742783244));
#47043=CARTESIAN_POINT('Ctrl Pts',(-6.01949065779634,3.0966363308406,153.546023283245));
#47044=CARTESIAN_POINT('Ctrl Pts',(-6.09822077806186,2.93855827358451,153.554303783245));
#47045=CARTESIAN_POINT('Ctrl Pts',(-6.17064598217405,2.77766397584,153.562584283246));
#47046=CARTESIAN_POINT('Ctrl Pts',(-6.24307843517748,2.61675357451276,153.570865612025));
#47047=CARTESIAN_POINT('Ctrl Pts',(-6.30920457180915,2.4530266900129,153.579146940804));
#47048=CARTESIAN_POINT('Ctrl Pts',(-6.36881824749775,2.28701620683801,153.587428269583));
#47049=CARTESIAN_POINT('Ctrl Pts',(-6.42847284618091,2.12089176246176,153.595715283245));
#47050=CARTESIAN_POINT('Ctrl Pts',(-6.48160593226592,1.95248091625491,153.604002296907));
#47051=CARTESIAN_POINT('Ctrl Pts',(-6.52806068577934,1.78233349370487,153.612289310569));
#47052=CARTESIAN_POINT('Ctrl Pts',(-6.57453174707025,1.61212634150182,153.620579233358));
#47053=CARTESIAN_POINT('Ctrl Pts',(-6.6143197184717,1.44018173706329,153.628869156146));
#47054=CARTESIAN_POINT('Ctrl Pts',(-6.64731869275697,1.26706084973208,153.637159078935));
#47055=CARTESIAN_POINT('Ctrl Pts',(-6.68035304300543,1.09375437123414,153.645457888788));
#47056=CARTESIAN_POINT('Ctrl Pts',(-6.70658379608069,0.919269435204907,
153.653756698641));
#47057=CARTESIAN_POINT('Ctrl Pts',(-6.72595667241432,0.74417460370888,153.662055508495));
#47058=CARTESIAN_POINT('Ctrl Pts',(-6.74129614728042,0.605534232466989,
153.668626519581));
#47059=CARTESIAN_POINT('Ctrl Pts',(-6.75233709758221,0.466511658131155,
153.675197530667));
#47060=CARTESIAN_POINT('Ctrl Pts',(-6.75907576279589,0.327389420698271,
153.681768541753));
#47061=CARTESIAN_POINT('Ctrl Pts',(-6.76434391201384,0.218626530260761,
153.686905622439));
#47062=CARTESIAN_POINT('Ctrl Pts',(-6.76698757074323,0.109718671431278,
153.692042703124));
#47063=CARTESIAN_POINT('Ctrl Pts',(-6.76699995627339,0.000769282719978384,
153.69717978381));
#47064=CARTESIAN_POINT('Origin',(0.,0.,0.));
#47065=CARTESIAN_POINT('',(-7.91099862725341,0.00453934634078324,0.642148860446907));
#47066=CARTESIAN_POINT('',(3.42067962509757,7.13322310757503,0.));
#47067=CARTESIAN_POINT('Ctrl Pts',(-7.91099862725342,0.00453934634078324,
0.642148860446907));
#47068=CARTESIAN_POINT('Ctrl Pts',(-7.90966797736711,2.20467810308481,0.553622307310889));
#47069=CARTESIAN_POINT('Ctrl Pts',(-6.94102417781289,4.38711985141806,0.465095754174871));
#47070=CARTESIAN_POINT('Ctrl Pts',(-3.67820201488296,7.34180684107626,0.287981765306128));
#47071=CARTESIAN_POINT('Ctrl Pts',(-1.40868175871758,8.08992666571333,0.199394329573404));
#47072=CARTESIAN_POINT('Ctrl Pts',(1.69567364519644,7.7814699249772,0.0738712625604527));
#47073=CARTESIAN_POINT('Ctrl Pts',(2.59296389908065,7.53014751000291,0.0369356312802263));
#47074=CARTESIAN_POINT('Ctrl Pts',(3.42067962509757,7.13322310757503,0.));
#47075=CARTESIAN_POINT('',(-3.42067962509618,7.1332231075757,0.));
#47076=CARTESIAN_POINT('Origin',(0.,0.,0.));
#47077=CARTESIAN_POINT('',(-7.9109995421887,0.00269137328987276,0.357668491799685));
#47078=CARTESIAN_POINT('Ctrl Pts',(-3.42067962509618,7.1332231075757,-6.22634595477876E-14));
#47079=CARTESIAN_POINT('Ctrl Pts',(-3.62731135360407,7.03413452826928,0.00922064556105209));
#47080=CARTESIAN_POINT('Ctrl Pts',(-3.82949148083065,6.926132808479,0.0184412911221664));
#47081=CARTESIAN_POINT('Ctrl Pts',(-4.02653219998454,6.80962256241031,0.0276619366832808));
#47082=CARTESIAN_POINT('Ctrl Pts',(-4.22390059962538,6.69291855875524,0.0368979162608378));
#47083=CARTESIAN_POINT('Ctrl Pts',(-4.41611240780442,6.5676777773061,0.0461338958383948));
#47084=CARTESIAN_POINT('Ctrl Pts',(-4.60250654856346,6.43434957633097,0.0553698754159518));
#47085=CARTESIAN_POINT('Ctrl Pts',(-4.78893874977624,6.30099415061687,0.0646077409196011));
#47086=CARTESIAN_POINT('Ctrl Pts',(-4.96955083114128,6.15954806785506,0.0738456064232504));
#47087=CARTESIAN_POINT('Ctrl Pts',(-5.14371259147606,6.01050262260076,0.0830834719268997));
#47088=CARTESIAN_POINT('Ctrl Pts',(-5.31770286349601,5.86160393489066,0.0923122413695945));
#47089=CARTESIAN_POINT('Ctrl Pts',(-5.48525542973374,5.70512090210243,0.101541010812289));
#47090=CARTESIAN_POINT('Ctrl Pts',(-5.64577433139744,5.54158399728216,0.110769780254984));
#47091=CARTESIAN_POINT('Ctrl Pts',(-5.80575143797907,5.37859907412792,0.119967400083236));
#47092=CARTESIAN_POINT('Ctrl Pts',(-5.95874220013166,5.20860787913774,0.129165019911488));
#47093=CARTESIAN_POINT('Ctrl Pts',(-6.10419004227923,5.03217496990507,0.13836263973974));
#47094=CARTESIAN_POINT('Ctrl Pts',(-6.21358399872687,4.89947658329754,0.145280336200942));
#47095=CARTESIAN_POINT('Ctrl Pts',(-6.31871173245749,4.76313504531534,0.152198032662144));
#47096=CARTESIAN_POINT('Ctrl Pts',(-6.41934941157972,4.62340503655597,0.159115729123346));
#47097=CARTESIAN_POINT('Ctrl Pts',(-6.53431466778682,4.4637819570399,0.167018283643299));
#47098=CARTESIAN_POINT('Ctrl Pts',(-6.64335809141854,4.29981903155955,0.174920838163251));
#47099=CARTESIAN_POINT('Ctrl Pts',(-6.74614773335647,4.13199851884404,0.182823392683204));
#47100=CARTESIAN_POINT('Ctrl Pts',(-6.84892595283971,3.96419665511074,0.19072506903519));
#47101=CARTESIAN_POINT('Ctrl Pts',(-6.94545159618463,3.79253835114268,0.198626745387175));
#47102=CARTESIAN_POINT('Ctrl Pts',(-7.03543686180464,3.61753357462795,0.20652842173916));
#47103=CARTESIAN_POINT('Ctrl Pts',(-7.12542708494852,3.44251915664191,0.214430533415183));
#47104=CARTESIAN_POINT('Ctrl Pts',(-7.20887605615657,3.26415820451004,0.222332645091205));
#47105=CARTESIAN_POINT('Ctrl Pts',(-7.28554250781484,3.08298416584046,0.230234756767228));
#47106=CARTESIAN_POINT('Ctrl Pts',(-7.36225435229779,2.90170285728692,0.238141547141196));
#47107=CARTESIAN_POINT('Ctrl Pts',(-7.43217551890899,2.71760545062612,0.246048337515164));
#47108=CARTESIAN_POINT('Ctrl Pts',(-7.49511303977695,2.53124505351923,0.253955127889132));
#47109=CARTESIAN_POINT('Ctrl Pts',(-7.55807012074251,2.34482673821814,0.261864375582507));
#47110=CARTESIAN_POINT('Ctrl Pts',(-7.61403912746857,2.15614435839489,0.269773623275881));
#47111=CARTESIAN_POINT('Ctrl Pts',(-7.66287724009551,1.9657653479564,0.277682870969256));
#47112=CARTESIAN_POINT('Ctrl Pts',(-7.71176225471301,1.77520350583035,0.28559971435871));
#47113=CARTESIAN_POINT('Ctrl Pts',(-7.75350261574405,1.58294211241716,0.293516557748164));
#47114=CARTESIAN_POINT('Ctrl Pts',(-7.78800659475649,1.38955902358606,0.301433401137619));
#47115=CARTESIAN_POINT('Ctrl Pts',(-7.81241025252054,1.25278480645919,0.30703275350733));
#47116=CARTESIAN_POINT('Ctrl Pts',(-7.83319511826985,1.11544967373295,0.312632105877042));
#47117=CARTESIAN_POINT('Ctrl Pts',(-7.85034443405357,0.977759309198411,
0.318231458246754));
#47118=CARTESIAN_POINT('Ctrl Pts',(-7.89060612247121,0.654501715431181,
0.331377136085626));
#47119=CARTESIAN_POINT('Ctrl Pts',(-7.91088858436064,0.328839751290012,
0.344522813924497));
#47120=CARTESIAN_POINT('Ctrl Pts',(-7.91099954218839,0.00269137419092156,
0.357668491763368));
#47121=CARTESIAN_POINT('',(-7.91099984610374,0.00110339172886062,2.35766849176338));
#47122=CARTESIAN_POINT('Ctrl Pts',(-7.9109995421887,0.00269137328987276,
0.357668491799686));
#47123=CARTESIAN_POINT('Ctrl Pts',(-7.91106612671522,-0.193026612311905,
0.365557065733029));
#47124=CARTESIAN_POINT('Ctrl Pts',(-7.90386535789137,-0.38893260034787,
0.373445639666373));
#47125=CARTESIAN_POINT('Ctrl Pts',(-7.88938173600258,-0.58444574053446,
0.381334213599717));
#47126=CARTESIAN_POINT('Ctrl Pts',(-7.8749084006657,-0.779820023460108,
0.38921718491337));
#47127=CARTESIAN_POINT('Ctrl Pts',(-7.85316254236865,-0.974801671083165,
0.397100156227022));
#47128=CARTESIAN_POINT('Ctrl Pts',(-7.82418072132649,-1.16881009579097,
0.404983127540675));
#47129=CARTESIAN_POINT('Ctrl Pts',(-7.79521407261338,-1.36271695477407,
0.412861972024807));
#47130=CARTESIAN_POINT('Ctrl Pts',(-7.7590190599732,-1.55565126495248,0.420740816508939));
#47131=CARTESIAN_POINT('Ctrl Pts',(-7.7156840782254,-1.74703755111877,0.428619660993071));
#47132=CARTESIAN_POINT('Ctrl Pts',(-7.67236369316935,-1.93835937189216,
0.436495851615135));
#47133=CARTESIAN_POINT('Ctrl Pts',(-7.62190820812512,-2.12813387105543,
0.444372042237198));
#47134=CARTESIAN_POINT('Ctrl Pts',(-7.56445716738786,-2.315795492429,0.452248232859261));
#47135=CARTESIAN_POINT('Ctrl Pts',(-7.50700354853349,-2.50346553512323,
0.460124776925605));
#47136=CARTESIAN_POINT('Ctrl Pts',(-7.44255383927082,-2.68902217738124,
0.46800132099195));
#47137=CARTESIAN_POINT('Ctrl Pts',(-7.37129771049221,-2.87191418104586,
0.475877865058294));
#47138=CARTESIAN_POINT('Ctrl Pts',(-7.30003652999233,-3.05481915088534,
0.483754967534222));
#47139=CARTESIAN_POINT('Ctrl Pts',(-7.22196809318516,-3.23505878302041,
0.491632070010151));
#47140=CARTESIAN_POINT('Ctrl Pts',(-7.13733056290994,-3.4121010295347,0.499509172486079));
#47141=CARTESIAN_POINT('Ctrl Pts',(-7.05267271493674,-3.58918577600005,
0.507388165903161));
#47142=CARTESIAN_POINT('Ctrl Pts',(-6.9614427801441,-3.76307129523202,0.515267159320242));
#47143=CARTESIAN_POINT('Ctrl Pts',(-6.86392539657377,-3.93324918486862,
0.523146152737324));
#47144=CARTESIAN_POINT('Ctrl Pts',(-6.76636810703079,-4.10349671454231,
0.531028370388735));
#47145=CARTESIAN_POINT('Ctrl Pts',(-6.66251841354984,-4.27003329147758,
0.538910588040146));
#47146=CARTESIAN_POINT('Ctrl Pts',(-6.55270499322013,-4.43237839898942,
0.546792805691557));
#47147=CARTESIAN_POINT('Ctrl Pts',(-6.44276429118574,-4.59491167623469,
0.554684159403901));
#47148=CARTESIAN_POINT('Ctrl Pts',(-6.32684624659744,-4.75324349162964,
0.562575513116245));
#47149=CARTESIAN_POINT('Ctrl Pts',(-6.20532139862745,-4.90692442775883,
0.570466866828589));
#47150=CARTESIAN_POINT('Ctrl Pts',(-6.08372134841189,-5.06070046502733,
0.578363103883966));
#47151=CARTESIAN_POINT('Ctrl Pts',(-5.95650780183018,-5.2098196229548,0.586259340939343));
#47152=CARTESIAN_POINT('Ctrl Pts',(-5.82408922820781,-5.35386828955231,
0.594155577994721));
#47153=CARTESIAN_POINT('Ctrl Pts',(-5.69147314761481,-5.49813180981411,
0.602063592566027));
#47154=CARTESIAN_POINT('Ctrl Pts',(-5.55363677011433,-5.63730948165375,
0.609971607137334));
#47155=CARTESIAN_POINT('Ctrl Pts',(-5.41102385846469,-5.77102606155317,
0.617879621708641));
#47156=CARTESIAN_POINT('Ctrl Pts',(-5.29931365386042,-5.87576767524552,
0.624074053303617));
#47157=CARTESIAN_POINT('Ctrl Pts',(-5.18467339594249,-5.97715926774425,
0.630268484898594));
#47158=CARTESIAN_POINT('Ctrl Pts',(-5.06732899452634,-6.07503891849531,
0.636462916493571));
#47159=CARTESIAN_POINT('Ctrl Pts',(-4.91907023871337,-6.19870493975095,
0.644289269605917));
#47160=CARTESIAN_POINT('Ctrl Pts',(-4.76603844546121,-6.31714329989183,
0.652115622718264));
#47161=CARTESIAN_POINT('Ctrl Pts',(-4.6086409765581,-6.42995718097637,0.65994197583061));
#47162=CARTESIAN_POINT('Ctrl Pts',(-4.45143333327123,-6.54263500546073,
0.667758890148847));
#47163=CARTESIAN_POINT('Ctrl Pts',(-4.28987078075816,-6.64970165296909,
0.675575804467085));
#47164=CARTESIAN_POINT('Ctrl Pts',(-4.12439613246084,-6.75079828927973,
0.683392718785321));
#47165=CARTESIAN_POINT('Ctrl Pts',(-3.95908852051114,-6.8517928748348,0.691201742415584));
#47166=CARTESIAN_POINT('Ctrl Pts',(-3.78987697509584,-6.94682926645249,
0.699010766045846));
#47167=CARTESIAN_POINT('Ctrl Pts',(-3.61723601415294,-7.03558985572034,
0.706819789676109));
#47168=CARTESIAN_POINT('Ctrl Pts',(-3.4447354099442,-7.12427828281785,0.714622464586765));
#47169=CARTESIAN_POINT('Ctrl Pts',(-3.26881125517591,-7.20670090797966,
0.72242513949742));
#47170=CARTESIAN_POINT('Ctrl Pts',(-3.08996572640634,-7.28258421232698,
0.730227814408076));
#47171=CARTESIAN_POINT('Ctrl Pts',(-2.9112304847738,-7.35842072236838,0.738025677710171));
#47172=CARTESIAN_POINT('Ctrl Pts',(-2.72957778154651,-7.42772580607952,
0.745823541012267));
#47173=CARTESIAN_POINT('Ctrl Pts',(-2.54553314591733,-7.49027249190817,
0.753621404314362));
#47174=CARTESIAN_POINT('Ctrl Pts',(-2.3615658817154,-7.55279288342873,0.76141598943445));
#47175=CARTESIAN_POINT('Ctrl Pts',(-2.17520902235627,-7.60856042377065,
0.769210574554537));
#47176=CARTESIAN_POINT('Ctrl Pts',(-1.98700692466844,-7.65739671698676,
0.777005159674624));
#47177=CARTESIAN_POINT('Ctrl Pts',(-1.79881702477839,-7.70622984501377,
0.784799239610262));
#47178=CARTESIAN_POINT('Ctrl Pts',(-1.60878246449003,-7.74813252360481,
0.792593319545901));
#47179=CARTESIAN_POINT('Ctrl Pts',(-1.41746199545339,-7.78297645450925,
0.800387399481539));
#47180=CARTESIAN_POINT('Ctrl Pts',(-1.22613925784472,-7.81782079857369,
0.808181571835054));
#47181=CARTESIAN_POINT('Ctrl Pts',(-1.033530928811,-7.84560616405464,0.81597574418857));
#47182=CARTESIAN_POINT('Ctrl Pts',(-0.840205128118094,-7.86625554776121,
0.823769916542086));
#47183=CARTESIAN_POINT('Ctrl Pts',(-0.646842666975414,-7.88690884721877,
0.831565566907657));
#47184=CARTESIAN_POINT('Ctrl Pts',(-0.452762814686121,-7.9004234319023,
0.839361217273228));
#47185=CARTESIAN_POINT('Ctrl Pts',(-0.258538107664255,-7.90677425040613,
0.8471568676388));
#47186=CARTESIAN_POINT('Ctrl Pts',(-0.0642420383565574,-7.91312740233567,
0.854955382292021));
#47187=CARTESIAN_POINT('Ctrl Pts',(0.130198638675183,-7.91231153399614,
0.862753896945242));
#47188=CARTESIAN_POINT('Ctrl Pts',(0.324211961902205,-7.90435371195897,
0.870552411598464));
#47189=CARTESIAN_POINT('Ctrl Pts',(0.518434713335572,-7.89638729982929,
0.878359344379414));
#47190=CARTESIAN_POINT('Ctrl Pts',(0.71222883633158,-7.88126355082138,0.886166277160364));
#47191=CARTESIAN_POINT('Ctrl Pts',(0.905027021324463,-7.85906146372915,
0.893973209941314));
#47192=CARTESIAN_POINT('Ctrl Pts',(1.09794061974251,-7.83684608595726,0.901784816131675));
#47193=CARTESIAN_POINT('Ctrl Pts',(1.28985674377954,-7.80754397955293,0.909596422322036));
#47194=CARTESIAN_POINT('Ctrl Pts',(1.48021879727392,-7.77128517763934,0.917408028512397));
#47195=CARTESIAN_POINT('Ctrl Pts',(1.67084401425626,-7.7349762502275,0.925230433753797));
#47196=CARTESIAN_POINT('Ctrl Pts',(1.85991052628593,-7.69169149718788,0.933052838995197));
#47197=CARTESIAN_POINT('Ctrl Pts',(2.04687628812262,-7.64161098598466,0.940875244236597));
#47198=CARTESIAN_POINT('Ctrl Pts',(2.15697474602777,-7.61212009417424,0.945481621071194));
#47199=CARTESIAN_POINT('Ctrl Pts',(2.26634507620393,-7.58027358173682,0.950087997905792));
#47200=CARTESIAN_POINT('Ctrl Pts',(2.37488002166888,-7.54611594680853,0.954694374740389));
#47201=CARTESIAN_POINT('Ctrl Pts',(2.56153944077685,-7.4873713252813,0.962616464906417));
#47202=CARTESIAN_POINT('Ctrl Pts',(2.74626565333976,-7.42161887265386,0.970538555072446));
#47203=CARTESIAN_POINT('Ctrl Pts',(2.92849514242134,-7.34900246297514,0.978460645238474));
#47204=CARTESIAN_POINT('Ctrl Pts',(3.11052681834732,-7.2764648796226,0.986374135843243));
#47205=CARTESIAN_POINT('Ctrl Pts',(3.29006685295937,-7.19707830715971,0.994287626448011));
#47206=CARTESIAN_POINT('Ctrl Pts',(3.46656583453685,-7.11103665542668,1.00220111705278));
#47207=CARTESIAN_POINT('Ctrl Pts',(3.6429057122888,-7.02507256536467,1.01010747409441));
#47208=CARTESIAN_POINT('Ctrl Pts',(3.81620969119175,-6.93246549712835,1.01801383113605));
#47209=CARTESIAN_POINT('Ctrl Pts',(3.98594705941756,-6.83345791232525,1.02592018817768));
#47210=CARTESIAN_POINT('Ctrl Pts',(4.15556265334386,-6.73452135831173,1.03382087297931));
#47211=CARTESIAN_POINT('Ctrl Pts',(4.32161643909138,-6.62919360925994,1.04172155778094));
#47212=CARTESIAN_POINT('Ctrl Pts',(4.48360083903562,-6.51776376652293,1.04962224258256));
#47213=CARTESIAN_POINT('Ctrl Pts',(4.64549882763955,-6.40639336655981,1.05751871272671));
#47214=CARTESIAN_POINT('Ctrl Pts',(4.80333147379025,-6.28892755392932,1.06541518287086));
#47215=CARTESIAN_POINT('Ctrl Pts',(4.95661856809418,-6.16569974702174,1.073311653015));
#47216=CARTESIAN_POINT('Ctrl Pts',(5.10985208654935,-6.04251500984797,1.08120536323933));
#47217=CARTESIAN_POINT('Ctrl Pts',(5.25854295211118,-5.91357250740162,1.08909907346365));
#47218=CARTESIAN_POINT('Ctrl Pts',(5.40224231930561,-5.77924726270676,1.09699278368797));
#47219=CARTESIAN_POINT('Ctrl Pts',(5.54594160696548,-5.64492209235808,1.1048864895433));
#47220=CARTESIAN_POINT('Ctrl Pts',(5.68464914485778,-5.50521441413616,1.11278019539862));
#47221=CARTESIAN_POINT('Ctrl Pts',(5.81795097104388,-5.36053798592358,1.12067390125394));
#47222=CARTESIAN_POINT('Ctrl Pts',(5.9512596551405,-5.21585411461716,1.12856801321269));
#47223=CARTESIAN_POINT('Ctrl Pts',(6.07916183988643,-5.0662012364696,1.13646212517144));
#47224=CARTESIAN_POINT('Ctrl Pts',(6.20128205197944,-4.91202828898589,1.14435623713019));
#47225=CARTESIAN_POINT('Ctrl Pts',(6.32342890329766,-4.75782171031371,1.15225207110549));
#47226=CARTESIAN_POINT('Ctrl Pts',(6.43979105508588,-4.59909336699831,1.16014790508079));
#47227=CARTESIAN_POINT('Ctrl Pts',(6.55003462754972,-4.43632363313359,1.16804373905609));
#47228=CARTESIAN_POINT('Ctrl Pts',(6.66032062550205,-4.27349125992113,1.17594261161773));
#47229=CARTESIAN_POINT('Ctrl Pts',(6.76448315945939,-4.10661468149927,1.18384148417937));
#47230=CARTESIAN_POINT('Ctrl Pts',(6.86223267518691,-3.93620168583841,1.19174035674102));
#47231=CARTESIAN_POINT('Ctrl Pts',(6.96008394357878,-3.76561129823632,1.19964745165877));
#47232=CARTESIAN_POINT('Ctrl Pts',(7.05150868835067,-3.59147743864202,1.20755454657653));
#47233=CARTESIAN_POINT('Ctrl Pts',(7.13626366989418,-3.41433182830089,1.21546164149429));
#47234=CARTESIAN_POINT('Ctrl Pts',(7.2210691804526,-3.23708060772867,1.2233734504443));
#47235=CARTESIAN_POINT('Ctrl Pts',(7.29919686339688,-3.05681437116568,1.23128525939432));
#47236=CARTESIAN_POINT('Ctrl Pts',(7.37045221679219,-2.87408335299851,1.23919706834434));
#47237=CARTESIAN_POINT('Ctrl Pts',(7.4417980846851,-2.69112021463941,1.24711892753448));
#47238=CARTESIAN_POINT('Ctrl Pts',(7.50625407293359,-2.50568636444544,1.25504078672463));
#47239=CARTESIAN_POINT('Ctrl Pts',(7.56367564732459,-2.31834676053195,1.26296264591478));
#47240=CARTESIAN_POINT('Ctrl Pts',(7.58774835862122,-2.23980881991876,1.26628370827225));
#47241=CARTESIAN_POINT('Ctrl Pts',(7.61058537722258,-2.16093606269547,1.26960477062973));
#47242=CARTESIAN_POINT('Ctrl Pts',(7.6321787424618,-2.08177055486773,1.27292583298721));
#47243=CARTESIAN_POINT('Ctrl Pts',(7.68325789520957,-1.89450437278393,1.28078181326463));
#47244=CARTESIAN_POINT('Ctrl Pts',(7.72751443554771,-1.70508658561529,1.28863779354205));
#47245=CARTESIAN_POINT('Ctrl Pts',(7.76476293192005,-1.51405997605129,1.29649377381948));
#47246=CARTESIAN_POINT('Ctrl Pts',(7.80197079559645,-1.32324174875495,1.30434118436419));
#47247=CARTESIAN_POINT('Ctrl Pts',(7.83218577261682,-1.13081853413889,1.3121885949089));
#47248=CARTESIAN_POINT('Ctrl Pts',(7.85527200877326,-0.937348744162689,
1.32003600545361));
#47249=CARTESIAN_POINT('Ctrl Pts',(7.87833750629953,-0.744052750313094,
1.32787636657962));
#47250=CARTESIAN_POINT('Ctrl Pts',(7.89428697580821,-0.54971239878627,1.33571672770562));
#47251=CARTESIAN_POINT('Ctrl Pts',(7.90303543735866,-0.354896993299682,
1.34355708883162));
#47252=CARTESIAN_POINT('Ctrl Pts',(7.91177772381033,-0.160219098204852,
1.35139191584123));
#47253=CARTESIAN_POINT('Ctrl Pts',(7.91332911110288,0.0349328347151123,
1.35922674285084));
#47254=CARTESIAN_POINT('Ctrl Pts',(7.90765632864982,0.229983451501376,1.36706156986045));
#47255=CARTESIAN_POINT('Ctrl Pts',(7.90198645884924,0.424933920843567,1.37489237413015));
#47256=CARTESIAN_POINT('Ctrl Pts',(7.88909981890886,0.619782828602985,1.38272317839985));
#47257=CARTESIAN_POINT('Ctrl Pts',(7.86901521296409,0.81395367075759,1.39055398266955));
#47258=CARTESIAN_POINT('Ctrl Pts',(7.84893705567685,1.00806216957978,1.39838227266662));
#47259=CARTESIAN_POINT('Ctrl Pts',(7.82166557348624,1.20149268878542,1.4062105626637));
#47260=CARTESIAN_POINT('Ctrl Pts',(7.7872715374635,1.39367248728343,1.41403885266077));
#47261=CARTESIAN_POINT('Ctrl Pts',(7.75287507181378,1.58586586154281,1.4218676956556));
#47262=CARTESIAN_POINT('Ctrl Pts',(7.71135510037303,1.77680799242736,1.42969653865042));
#47263=CARTESIAN_POINT('Ctrl Pts',(7.66283385940022,1.96593444530317,1.43752538164525));
#47264=CARTESIAN_POINT('Ctrl Pts',(7.61430794975743,2.15507909575548,1.44535497792428));
#47265=CARTESIAN_POINT('Ctrl Pts',(7.55877951482502,2.34240738059906,1.45318457420331));
#47266=CARTESIAN_POINT('Ctrl Pts',(7.49642118890176,2.52736826730588,1.46101417048234));
#47267=CARTESIAN_POINT('Ctrl Pts',(7.4340459945453,2.71237918743351,1.4688458847307));
#47268=CARTESIAN_POINT('Ctrl Pts',(7.36483734020135,2.89502110168799,1.47667759897906));
#47269=CARTESIAN_POINT('Ctrl Pts',(7.28901675181659,3.07476109506693,1.48450931322742));
#47270=CARTESIAN_POINT('Ctrl Pts',(7.21316243784266,3.254581038197,1.49234451108337));
#47271=CARTESIAN_POINT('Ctrl Pts',(7.13069046659174,3.43149616657611,1.50017970893932));
#47272=CARTESIAN_POINT('Ctrl Pts',(7.04186929690232,3.60499622820114,1.50801490679527));
#47273=CARTESIAN_POINT('Ctrl Pts',(6.952943867529,3.77869994692328,1.51585930172951));
#47274=CARTESIAN_POINT('Ctrl Pts',(6.85765451363545,3.94898028053856,1.52370369666375));
#47275=CARTESIAN_POINT('Ctrl Pts',(6.75631476749142,4.11535317592274,1.531548091598));
#47276=CARTESIAN_POINT('Ctrl Pts',(6.65490817317078,4.28183581822377,1.53939766104193));
#47277=CARTESIAN_POINT('Ctrl Pts',(6.54744342477946,4.44440559427355,1.54724723048585));
#47278=CARTESIAN_POINT('Ctrl Pts',(6.43427573884808,4.6026097723434,1.55509679992978));
#47279=CARTESIAN_POINT('Ctrl Pts',(6.32094554126904,4.76104113559808,1.56295764155316));
#47280=CARTESIAN_POINT('Ctrl Pts',(6.20189626204498,4.91509410335571,1.57081848317654));
#47281=CARTESIAN_POINT('Ctrl Pts',(6.0775222946626,5.06435027993513,1.57867932479992));
#47282=CARTESIAN_POINT('Ctrl Pts',(6.01171364190726,5.1433245870416,1.58283864694462));
#47283=CARTESIAN_POINT('Ctrl Pts',(5.94441486145594,5.22095658309199,1.58699796908932));
#47284=CARTESIAN_POINT('Ctrl Pts',(5.87568825599643,5.29718873727807,1.59115729123402));
#47285=CARTESIAN_POINT('Ctrl Pts',(5.74512415958285,5.4420115793553,1.5990590075182));
#47286=CARTESIAN_POINT('Ctrl Pts',(5.60901247919307,5.58221516921733,1.60696072380238));
#47287=CARTESIAN_POINT('Ctrl Pts',(5.46771201489397,5.71734609081733,1.61486244008655));
#47288=CARTESIAN_POINT('Ctrl Pts',(5.32657659542006,5.85231917387486,1.62275492683713));
#47289=CARTESIAN_POINT('Ctrl Pts',(5.18026471049383,5.98223115281326,1.63064741358771));
#47290=CARTESIAN_POINT('Ctrl Pts',(5.02917515824721,6.10666179083705,1.63853990033829));
#47291=CARTESIAN_POINT('Ctrl Pts',(4.87823377477048,6.23097040364931,1.64642464717545));
#47292=CARTESIAN_POINT('Ctrl Pts',(4.72252432185267,6.34980816445695,1.65430939401261));
#47293=CARTESIAN_POINT('Ctrl Pts',(4.56248235630436,6.46279163739722,1.66219414084976));
#47294=CARTESIAN_POINT('Ctrl Pts',(4.40256736252464,6.57568547315181,1.67007263220107));
#47295=CARTESIAN_POINT('Ctrl Pts',(4.23832698504589,6.68273407523877,1.67795112355238));
#47296=CARTESIAN_POINT('Ctrl Pts',(4.07022996932809,6.78359410613456,1.68582961490369));
#47297=CARTESIAN_POINT('Ctrl Pts',(3.90223483919664,6.88439300457452,1.69370333100835));
#47298=CARTESIAN_POINT('Ctrl Pts',(3.73038802416106,6.97901062793922,1.70157704711301));
#47299=CARTESIAN_POINT('Ctrl Pts',(3.55518759034413,7.06714668005859,1.70945076321767));
#47300=CARTESIAN_POINT('Ctrl Pts',(3.38006054681664,7.15524581257545,1.71732118107534));
#47301=CARTESIAN_POINT('Ctrl Pts',(3.20158299270792,7.23686862926661,1.72519159893301));
#47302=CARTESIAN_POINT('Ctrl Pts',(3.02027818423293,7.31176043712091,1.73306201679067));
#47303=CARTESIAN_POINT('Ctrl Pts',(2.83899039489044,7.38664521486051,1.74093169585004));
#47304=CARTESIAN_POINT('Ctrl Pts',(2.65487619711691,7.45480010438969,1.74880137490941));
#47305=CARTESIAN_POINT('Ctrl Pts',(2.46847990812357,7.51601809093021,1.75667105396878));
#47306=CARTESIAN_POINT('Ctrl Pts',(2.28208477794308,7.57723569688274,1.7645406841029));
#47307=CARTESIAN_POINT('Ctrl Pts',(2.09340791355454,7.63151637715714,1.77241031423701));
#47308=CARTESIAN_POINT('Ctrl Pts',(1.90300999933721,7.67870262104365,1.78027994437113));
#47309=CARTESIAN_POINT('Ctrl Pts',(1.71258097184564,7.72589657572128,1.78815086049602));
#47310=CARTESIAN_POINT('Ctrl Pts',(1.52043067021317,7.76599370087157,1.79602177662091));
#47311=CARTESIAN_POINT('Ctrl Pts',(1.32713143109919,7.79888730298038,1.80389269274579));
#47312=CARTESIAN_POINT('Ctrl Pts',(1.13376781522621,7.83179186003917,1.81176623021608));
#47313=CARTESIAN_POINT('Ctrl Pts',(0.939254840577545,7.85748805622527,1.81963976768636));
#47314=CARTESIAN_POINT('Ctrl Pts',(0.744171676952125,7.87592086776031,1.82751330515665));
#47315=CARTESIAN_POINT('Ctrl Pts',(0.548897500175621,7.89437172754384,1.83539455189909));
#47316=CARTESIAN_POINT('Ctrl Pts',(0.353052364075873,7.90554496486019,1.84327579864153));
#47317=CARTESIAN_POINT('Ctrl Pts',(0.157218223899022,7.90943761781292,1.85115704538398));
#47318=CARTESIAN_POINT('Ctrl Pts',(-0.0387248944192319,7.9133324369563,
1.85904267789706));
#47319=CARTESIAN_POINT('Ctrl Pts',(-0.23465665926724,7.90993860042775,1.86692831041015));
#47320=CARTESIAN_POINT('Ctrl Pts',(-0.429998259737013,7.89930519075084,
1.87481394292323));
#47321=CARTESIAN_POINT('Ctrl Pts',(-0.625581418376249,7.88865863186776,
1.88270932675887));
#47322=CARTESIAN_POINT('Ctrl Pts',(-0.820572611094728,7.87075464924748,
1.89060471059451));
#47323=CARTESIAN_POINT('Ctrl Pts',(-1.01440016151281,7.84569393440267,1.89850009443015));
#47324=CARTESIAN_POINT('Ctrl Pts',(-1.10350376009476,7.83417338497152,1.90212964611371));
#47325=CARTESIAN_POINT('Ctrl Pts',(-1.19236160753875,7.82114111686436,1.90575919779728));
#47326=CARTESIAN_POINT('Ctrl Pts',(-1.28091912361697,7.80661048078821,1.90938874948084));
#47327=CARTESIAN_POINT('Ctrl Pts',(-1.4840743942043,7.77327649136997,1.91771511845594));
#47328=CARTESIAN_POINT('Ctrl Pts',(-1.68610102522148,7.73197959767553,1.92604148743103));
#47329=CARTESIAN_POINT('Ctrl Pts',(-1.88636669581931,7.68280819029759,1.93436785640613));
#47330=CARTESIAN_POINT('Ctrl Pts',(-2.08638212157466,7.63369822575735,1.94268382104739));
#47331=CARTESIAN_POINT('Ctrl Pts',(-2.28464069384541,7.57673344200757,1.95099978568865));
#47332=CARTESIAN_POINT('Ctrl Pts',(-2.48051884884997,7.5120534636343,1.95931575032991));
#47333=CARTESIAN_POINT('Ctrl Pts',(-2.67616425723196,7.44745033939779,1.96762183376373));
#47334=CARTESIAN_POINT('Ctrl Pts',(-2.86943461406105,7.37515039661436,1.97592791719754));
#47335=CARTESIAN_POINT('Ctrl Pts',(-3.05971929268036,7.29534364166621,1.98423400063136));
#47336=CARTESIAN_POINT('Ctrl Pts',(-3.24971045937864,7.21565998771666,1.99252727202732));
#47337=CARTESIAN_POINT('Ctrl Pts',(-3.43672487057012,7.12849274219435,2.00082054342329));
#47338=CARTESIAN_POINT('Ctrl Pts',(-3.62016967077566,7.03408078961253,2.00911381481925));
#47339=CARTESIAN_POINT('Ctrl Pts',(-3.80344077058155,6.93975823391673,2.01739923347394));
#47340=CARTESIAN_POINT('Ctrl Pts',(-3.98314874143098,6.83820478400954,2.02568465212862));
#47341=CARTESIAN_POINT('Ctrl Pts',(-4.15872150952731,6.72970700745544,2.0339700707833));
#47342=CARTESIAN_POINT('Ctrl Pts',(-4.33408484153599,6.6213386550147,2.04224560598232));
#47343=CARTESIAN_POINT('Ctrl Pts',(-4.5053225664823,6.50604265857243,2.05052114118135));
#47344=CARTESIAN_POINT('Ctrl Pts',(-4.67188775381832,6.38415114292593,2.05879667638038));
#47345=CARTESIAN_POINT('Ctrl Pts',(-4.73701876376317,6.33648861725212,2.062032610455));
#47346=CARTESIAN_POINT('Ctrl Pts',(-4.80143561405838,6.28781813039693,2.06526854452963));
#47347=CARTESIAN_POINT('Ctrl Pts',(-4.86510669996793,6.23816141166026,2.06850447860425));
#47348=CARTESIAN_POINT('Ctrl Pts',(-5.0277096124292,6.11134832257107,2.07676839145496));
#47349=CARTESIAN_POINT('Ctrl Pts',(-5.18525920588905,5.97824633454064,2.08503230430567));
#47350=CARTESIAN_POINT('Ctrl Pts',(-5.33728610071854,5.83928917583953,2.09329621715638));
#47351=CARTESIAN_POINT('Ctrl Pts',(-5.48945000238128,5.70020678876818,2.10156757745598));
#47352=CARTESIAN_POINT('Ctrl Pts',(-5.63608105236553,5.555258895159,2.10983893775559));
#47353=CARTESIAN_POINT('Ctrl Pts',(-5.77674712300957,5.40491569562381,2.11811029805519));
#47354=CARTESIAN_POINT('Ctrl Pts',(-5.91754923325907,5.25442709763217,2.12638965767252));
#47355=CARTESIAN_POINT('Ctrl Pts',(-6.05237464655406,5.09853299112444,2.13466901728984));
#47356=CARTESIAN_POINT('Ctrl Pts',(-6.18083133164794,4.93773683479781,2.14294837690717));
#47357=CARTESIAN_POINT('Ctrl Pts',(-6.30950271264577,4.77667193203648,2.15124157422081));
#47358=CARTESIAN_POINT('Ctrl Pts',(-6.43178390076399,4.61068882953579,2.15953477153444));
#47359=CARTESIAN_POINT('Ctrl Pts',(-6.54732487325436,4.44032183564038,2.16782796884807));
#47360=CARTESIAN_POINT('Ctrl Pts',(-6.66297109400047,4.26979965152494,2.17612872057754));
#47361=CARTESIAN_POINT('Ctrl Pts',(-6.77186468438994,4.09488585158791,2.18442947230701));
#47362=CARTESIAN_POINT('Ctrl Pts',(-6.87370083924785,3.91614067322964,2.19273022403647));
#47363=CARTESIAN_POINT('Ctrl Pts',(-6.97569398705812,3.73711993720412,2.20104377239522));
#47364=CARTESIAN_POINT('Ctrl Pts',(-7.07060781210317,3.55425627498662,2.20935732075396));
#47365=CARTESIAN_POINT('Ctrl Pts',(-7.15818420681603,3.36813299340889,2.21767086911271));
#47366=CARTESIAN_POINT('Ctrl Pts',(-7.19312024006662,3.29388457092897,2.22098731531769));
#47367=CARTESIAN_POINT('Ctrl Pts',(-7.22688915641556,3.21911762542658,2.22430376152268));
#47368=CARTESIAN_POINT('Ctrl Pts',(-7.25947675683652,3.14386994275374,2.22762020772766));
#47369=CARTESIAN_POINT('Ctrl Pts',(-7.3438421092644,2.94906280181453,2.23620608546266));
#47370=CARTESIAN_POINT('Ctrl Pts',(-7.42043412903276,2.75069165235358,2.24479196319766));
#47371=CARTESIAN_POINT('Ctrl Pts',(-7.48896670490833,2.54937221542372,2.25337784093267));
#47372=CARTESIAN_POINT('Ctrl Pts',(-7.55833747050121,2.34559053510414,2.26206872850189));
#47373=CARTESIAN_POINT('Ctrl Pts',(-7.61945019851203,2.13878817759546,2.27075961607112));
#47374=CARTESIAN_POINT('Ctrl Pts',(-7.67205674126729,1.9296285546123,2.27945050364034));
#47375=CARTESIAN_POINT('Ctrl Pts',(-7.72377724630503,1.72399175037445,2.28799501294972));
#47376=CARTESIAN_POINT('Ctrl Pts',(-7.76727569579189,1.51607669808758,2.2965395222591));
#47377=CARTESIAN_POINT('Ctrl Pts',(-7.80236435240672,1.30653416040025,2.30508403156849));
#47378=CARTESIAN_POINT('Ctrl Pts',(-7.83835467867448,1.09160702935836,2.31384810826763));
#47379=CARTESIAN_POINT('Ctrl Pts',(-7.86549709841624,0.874967868526115,
2.32261218496678));
#47380=CARTESIAN_POINT('Ctrl Pts',(-7.88364311573386,0.65733722223991,2.33137626166593));
#47381=CARTESIAN_POINT('Ctrl Pts',(-7.90178913305148,0.439706575953708,
2.34014033836508));
#47382=CARTESIAN_POINT('Ctrl Pts',(-7.91093863592887,0.221084715389548,
2.34890441506423));
#47383=CARTESIAN_POINT('Ctrl Pts',(-7.91099969220747,0.00220678346617059,
2.35766849176338));
#47384=CARTESIAN_POINT('',(-7.91099895811926,-0.0034257496853649,4.35766849176336));
#47385=CARTESIAN_POINT('Ctrl Pts',(-7.911,-8.44935232890975E-12,2.35766849176337));
#47386=CARTESIAN_POINT('Ctrl Pts',(-7.91099999999765,-2.20167589667518,
2.4462559274961));
#47387=CARTESIAN_POINT('Ctrl Pts',(-6.94214576671906,-4.38610418339417,
2.53484336322882));
#47388=CARTESIAN_POINT('Ctrl Pts',(-3.67820201487515,-7.34180684108017,
2.71201823469427));
#47389=CARTESIAN_POINT('Ctrl Pts',(-1.40868175870898,-8.08992666571483,
2.800605670427));
#47390=CARTESIAN_POINT('Ctrl Pts',(2.97309270522067,-7.65454228024948,2.97778054189244));
#47391=CARTESIAN_POINT('Ctrl Pts',(5.05102072676269,-6.47444880833704,3.06636797762517));
#47392=CARTESIAN_POINT('Ctrl Pts',(7.66951518848171,-2.93425195366922,3.24354284909062));
#47393=CARTESIAN_POINT('Ctrl Pts',(8.18956872247132,-0.60188196009084,3.33213028482334));
#47394=CARTESIAN_POINT('Ctrl Pts',(7.32306689760967,3.71537198233187,3.50930515628879));
#47395=CARTESIAN_POINT('Ctrl Pts',(5.94329958849633,5.66643518937106,3.59789259202151));
#47396=CARTESIAN_POINT('Ctrl Pts',(2.1615450163706,7.92205913233211,3.77506746348696));
#47397=CARTESIAN_POINT('Ctrl Pts',(-0.21081652930848,8.20894963712981,3.86365489921969));
#47398=CARTESIAN_POINT('Ctrl Pts',(-4.42123908577114,6.91982244717397,4.04082977068514));
#47399=CARTESIAN_POINT('Ctrl Pts',(-6.22631625634709,5.35390358802913,4.12941720641786));
#47400=CARTESIAN_POINT('Ctrl Pts',(-7.65317280859724,2.31334857513753,4.26455925868818));
#47401=CARTESIAN_POINT('Ctrl Pts',(-7.91100000000124,1.157028378357,4.31111387522578));
#47402=CARTESIAN_POINT('Ctrl Pts',(-7.911,-8.4471318828605E-12,4.35766849176337));
#47403=CARTESIAN_POINT('',(-7.91099998419434,-0.000500077126143346,6.35761307316525));
#47404=CARTESIAN_POINT('Ctrl Pts',(-7.91099853652232,-0.00481197898119207,
4.35766849176336));
#47405=CARTESIAN_POINT('Ctrl Pts',(-7.91085957146424,-0.233273569392922,
4.36684708997177));
#47406=CARTESIAN_POINT('Ctrl Pts',(-7.90081999409514,-0.461398660723006,
4.37602568818018));
#47407=CARTESIAN_POINT('Ctrl Pts',(-7.88099117191259,-0.688403332528123,
4.38520428638859));
#47408=CARTESIAN_POINT('Ctrl Pts',(-7.86107949738137,-0.91635651605244,
4.3944212362657));
#47409=CARTESIAN_POINT('Ctrl Pts',(-7.8312966797031,-1.14317980272321,4.40363818614281));
#47410=CARTESIAN_POINT('Ctrl Pts',(-7.7918056249086,-1.36809579476098,4.41285513601991));
#47411=CARTESIAN_POINT('Ctrl Pts',(-7.75212623634786,-1.59408441643826,
4.42211604174709));
#47412=CARTESIAN_POINT('Ctrl Pts',(-7.70264584886791,-1.81814741536919,
4.43137694747427));
#47413=CARTESIAN_POINT('Ctrl Pts',(-7.64357920451689,-2.03951414417183,
4.44063785320145));
#47414=CARTESIAN_POINT('Ctrl Pts',(-7.61253384831106,-2.15586422674899,
4.44550537395275));
#47415=CARTESIAN_POINT('Ctrl Pts',(-7.57884106698765,-2.27146976033907,
4.45037289470406));
#47416=CARTESIAN_POINT('Ctrl Pts',(-7.54253741009926,-2.38622094895949,
4.45524041545537));
#47417=CARTESIAN_POINT('Ctrl Pts',(-7.48354424394224,-2.57269075716126,
4.4631500996323));
#47418=CARTESIAN_POINT('Ctrl Pts',(-7.41755723275975,-2.75720789205596,
4.47105978380923));
#47419=CARTESIAN_POINT('Ctrl Pts',(-7.34472350009437,-2.9392103883801,4.47896946798616));
#47420=CARTESIAN_POINT('Ctrl Pts',(-7.27196366407615,-3.12102822611597,
4.48687112704727));
#47421=CARTESIAN_POINT('Ctrl Pts',(-7.19237107077791,-3.30033619002059,
4.49477278610837));
#47422=CARTESIAN_POINT('Ctrl Pts',(-7.1061427904712,-3.47658678036867,4.50267444516947));
#47423=CARTESIAN_POINT('Ctrl Pts',(-7.01998602260213,-3.65269119930631,
4.51056955108004));
#47424=CARTESIAN_POINT('Ctrl Pts',(-6.92720468165589,-3.82574298818843,
4.51846465699062));
#47425=CARTESIAN_POINT('Ctrl Pts',(-6.82804426171055,-3.99521370643945,
4.52635976290119));
#47426=CARTESIAN_POINT('Ctrl Pts',(-6.72894771435978,-4.16457526284459,
4.53424978330588));
#47427=CARTESIAN_POINT('Ctrl Pts',(-6.62348044823339,-4.33036004812295,
4.54213980371057));
#47428=CARTESIAN_POINT('Ctrl Pts',(-6.51193442959602,-4.49206311004665,
4.55002982411526));
#47429=CARTESIAN_POINT('Ctrl Pts',(-6.40043960678927,-4.65369195576192,
4.5579162232688));
#47430=CARTESIAN_POINT('Ctrl Pts',(-6.28287178631894,-4.8112425281299,4.56580262242234));
#47431=CARTESIAN_POINT('Ctrl Pts',(-6.15956704404111,-4.96423758798495,
4.57368902157588));
#47432=CARTESIAN_POINT('Ctrl Pts',(-6.03629606567186,-5.11719075398323,
4.58157326123697));
#47433=CARTESIAN_POINT('Ctrl Pts',(-5.90729151261009,-5.26559062571781,
4.58945750089806));
#47434=CARTESIAN_POINT('Ctrl Pts',(-5.77293081815939,-5.4089916591492,4.59734174055915));
#47435=CARTESIAN_POINT('Ctrl Pts',(-5.63855444253181,-5.5524094288514,4.60522690038635));
#47436=CARTESIAN_POINT('Ctrl Pts',(-5.49882090709427,-5.69082693830027,
4.61311206021354));
#47437=CARTESIAN_POINT('Ctrl Pts',(-5.35414614578648,-5.82383379309195,
4.62099722004074));
#47438=CARTESIAN_POINT('Ctrl Pts',(-5.20945334281543,-5.95685723450084,
4.62888336318663));
#47439=CARTESIAN_POINT('Ctrl Pts',(-5.05981833949993,-6.08446844284659,
4.63676950633253));
#47440=CARTESIAN_POINT('Ctrl Pts',(-4.90569192378809,-6.20629581545066,
4.64465564947842));
#47441=CARTESIAN_POINT('Ctrl Pts',(-4.75152042760113,-6.32815882137438,
4.65254409924436));
#47442=CARTESIAN_POINT('Ctrl Pts',(-4.59285517151457,-6.4442344065822,4.6604325490103));
#47443=CARTESIAN_POINT('Ctrl Pts',(-4.43017801577483,-6.55419283730235,
4.66832099877624));
#47444=CARTESIAN_POINT('Ctrl Pts',(-4.26742598311092,-6.66420187960985,
4.67621307943216));
#47445=CARTESIAN_POINT('Ctrl Pts',(-4.10065865629295,-6.76808796386108,
4.68410516008808));
#47446=CARTESIAN_POINT('Ctrl Pts',(-3.93038490874541,-6.86556592489697,
4.691997240744));
#47447=CARTESIAN_POINT('Ctrl Pts',(-3.75991376502587,-6.96315689088305,
4.69989847058782));
#47448=CARTESIAN_POINT('Ctrl Pts',(-3.58592838021548,-7.05432472362902,
4.70779970043163));
#47449=CARTESIAN_POINT('Ctrl Pts',(-3.40896119455936,-7.13883075678282,
4.71570093027545));
#47450=CARTESIAN_POINT('Ctrl Pts',(-3.23187674743201,-7.22339278507346,
4.72360739560873));
#47451=CARTESIAN_POINT('Ctrl Pts',(-3.05180687590208,-7.30128407735721,
4.73151386094202));
#47452=CARTESIAN_POINT('Ctrl Pts',(-2.8693020520652,-7.37231488299397,4.7394203262753));
#47453=CARTESIAN_POINT('Ctrl Pts',(-2.68654579668107,-7.44344354569001,
4.74733768411416));
#47454=CARTESIAN_POINT('Ctrl Pts',(-2.50134821293216,-7.50769273055924,
4.75525504195302));
#47455=CARTESIAN_POINT('Ctrl Pts',(-2.31427405444284,-7.56492277560933,
4.76317239979188));
#47456=CARTESIAN_POINT('Ctrl Pts',(-2.23315417186469,-7.58973910819045,
4.76660555776199));
#47457=CARTESIAN_POINT('Ctrl Pts',(-2.15168155942537,-7.61323628552008,
4.77003871573209));
#47458=CARTESIAN_POINT('Ctrl Pts',(-2.06990271671669,-7.63540593179753,
4.77347187370219));
#47459=CARTESIAN_POINT('Ctrl Pts',(-1.88311267735236,-7.68604334562849,
4.78131350719979));
#47460=CARTESIAN_POINT('Ctrl Pts',(-1.69416914107881,-7.72990202532652,
4.78915514069739));
#47461=CARTESIAN_POINT('Ctrl Pts',(-1.50361088955,-7.76679311510398,4.79699677419498));
#47462=CARTESIAN_POINT('Ctrl Pts',(-1.31327700440735,-7.80364076871205,
4.8048291748257));
#47463=CARTESIAN_POINT('Ctrl Pts',(-1.12133253093889,-7.83353710127725,
4.81266157545642));
#47464=CARTESIAN_POINT('Ctrl Pts',(-0.928332353797759,-7.85634266315391,
4.82049397608713));
#47465=CARTESIAN_POINT('Ctrl Pts',(-0.735521847410999,-7.87912581288469,
4.82831867943302));
#47466=CARTESIAN_POINT('Ctrl Pts',(-0.541658049914513,-7.89483202798421,
4.8361433827789));
#47467=CARTESIAN_POINT('Ctrl Pts',(-0.347307203557107,-7.90337261593792,
4.84396808612479));
#47468=CARTESIAN_POINT('Ctrl Pts',(-0.153109544359171,-7.91190647220801,
4.85178662204664));
#47469=CARTESIAN_POINT('Ctrl Pts',(0.0415740495560627,-7.91328593479967,
4.8596051579685));
#47470=CARTESIAN_POINT('Ctrl Pts',(0.236170833643165,-7.90747395426228,
4.86742369389036));
#47471=CARTESIAN_POINT('Ctrl Pts',(0.430652079913269,-7.90166542446816,
4.87523758771817));
#47472=CARTESIAN_POINT('Ctrl Pts',(0.62504626851744,-7.88867396726732,4.88305148154599));
#47473=CARTESIAN_POINT('Ctrl Pts',(0.818779071836284,-7.86851458863253,
4.8908653753738));
#47474=CARTESIAN_POINT('Ctrl Pts',(1.01243451497338,-7.84836325991581,4.89867614900598));
#47475=CARTESIAN_POINT('Ctrl Pts',(1.20542874968516,-7.82104974875847,4.90648692263816));
#47476=CARTESIAN_POINT('Ctrl Pts',(1.39719080189449,-7.78664105138419,4.91429769627034));
#47477=CARTESIAN_POINT('Ctrl Pts',(1.588945233428,-7.75223372142084,4.92210815950027));
#47478=CARTESIAN_POINT('Ctrl Pts',(1.77946723227763,-7.71073182016129,4.92991862273019));
#47479=CARTESIAN_POINT('Ctrl Pts',(1.96819380720538,-7.66225385492274,4.93772908596012));
#47480=CARTESIAN_POINT('Ctrl Pts',(2.15692558742979,-7.61377455260598,4.94553976461163));
#47481=CARTESIAN_POINT('Ctrl Pts',(2.34386150397228,-7.55831888982698,4.95335044326314));
#47482=CARTESIAN_POINT('Ctrl Pts',(2.52845160510943,-7.49605586162614,4.96116112191465));
#47483=CARTESIAN_POINT('Ctrl Pts',(2.71307930626593,-7.43378015077844,4.96897339155976));
#47484=CARTESIAN_POINT('Ctrl Pts',(2.89535990668359,-7.36469442473456,4.97678566120486));
#47485=CARTESIAN_POINT('Ctrl Pts',(3.07476124264891,-7.28901668956137,4.98459793084996));
#47486=CARTESIAN_POINT('Ctrl Pts',(3.25423071902528,-7.21331021038828,4.99241316775984));
#47487=CARTESIAN_POINT('Ctrl Pts',(3.43081842859891,-7.13100687135934,5.00022840466972));
#47488=CARTESIAN_POINT('Ctrl Pts',(3.6040145761508,-7.04237175494822,5.0080436415796));
#47489=CARTESIAN_POINT('Ctrl Pts',(3.77739908255753,-6.95364024373122,5.01586737792262));
#47490=CARTESIAN_POINT('Ctrl Pts',(3.94738434664408,-6.85856336193265,5.02369111426563));
#47491=CARTESIAN_POINT('Ctrl Pts',(4.11348654706754,-6.75745140027617,5.03151485060864));
#47492=CARTESIAN_POINT('Ctrl Pts',(4.27968952566926,-6.6562780915739,5.03934333379963));
#47493=CARTESIAN_POINT('Ctrl Pts',(4.442004452746,-6.54906259908174,5.04717181699063));
#47494=CARTESIAN_POINT('Ctrl Pts',(4.59997859179379,-6.43615707973623,5.05500030018163));
#47495=CARTESIAN_POINT('Ctrl Pts',(4.75817014634896,-6.32309617159784,5.06283955750095));
#47496=CARTESIAN_POINT('Ctrl Pts',(4.91200870294541,-6.2043298095686,5.07067881482026));
#47497=CARTESIAN_POINT('Ctrl Pts',(5.0610756728966,-6.08024950419094,5.07851807213958));
#47498=CARTESIAN_POINT('Ctrl Pts',(5.14465020246199,-6.01068377038913,5.08291315874272));
#47499=CARTESIAN_POINT('Ctrl Pts',(5.22672555110569,-5.93944836820004,5.08730824534587));
#47500=CARTESIAN_POINT('Ctrl Pts',(5.30723332611136,-5.86661703388017,5.09170333194901));
#47501=CARTESIAN_POINT('Ctrl Pts',(5.45212403513974,-5.73554169776082,5.09961321660458));
#47502=CARTESIAN_POINT('Ctrl Pts',(5.59235160506865,-5.59891857292677,5.10752310126014));
#47503=CARTESIAN_POINT('Ctrl Pts',(5.72746461096192,-5.45711188543709,5.1154329859157));
#47504=CARTESIAN_POINT('Ctrl Pts',(5.86243072674516,-5.31545936519276,5.12333427122274));
#47505=CARTESIAN_POINT('Ctrl Pts',(5.99229311804405,-5.1686347545401,5.13123555652978));
#47506=CARTESIAN_POINT('Ctrl Pts',(6.11663398779495,-5.01704192322046,5.13913684183683));
#47507=CARTESIAN_POINT('Ctrl Pts',(6.24086278404226,-4.86558572871025,5.14703100539276));
#47508=CARTESIAN_POINT('Ctrl Pts',(6.35957975544661,-4.70937014007884,5.15492516894869));
#47509=CARTESIAN_POINT('Ctrl Pts',(6.47240430642796,-4.54883539976254,5.16281933250462));
#47510=CARTESIAN_POINT('Ctrl Pts',(6.58514812299098,-4.38841553407917,5.17070784719514));
#47511=CARTESIAN_POINT('Ctrl Pts',(6.69200772217223,-4.22368295542573,5.17859636188567));
#47512=CARTESIAN_POINT('Ctrl Pts',(6.7926429574596,-4.05511068313486,5.18648487657619));
#47513=CARTESIAN_POINT('Ctrl Pts',(6.89322487109512,-3.88662772898379,5.19436921153153));
#47514=CARTESIAN_POINT('Ctrl Pts',(6.98758881606287,-3.71430943059956,5.20225354648687));
#47515=CARTESIAN_POINT('Ctrl Pts',(7.07543798704275,-3.53865769629,5.21013788144221));
#47516=CARTESIAN_POINT('Ctrl Pts',(7.16325692412841,-3.36306641372852,5.21801950294965));
#47517=CARTESIAN_POINT('Ctrl Pts',(7.244565401664,-3.18414428984217,5.22590112445708));
#47518=CARTESIAN_POINT('Ctrl Pts',(7.31911246602694,-3.00241797717257,5.23378274596451));
#47519=CARTESIAN_POINT('Ctrl Pts',(7.39366050701541,-2.82068928374447,5.24166447072743));
#47520=CARTESIAN_POINT('Ctrl Pts',(7.46144681901013,-2.63615664400992,5.24954619549034));
#47521=CARTESIAN_POINT('Ctrl Pts',(7.52226830598668,-2.44936737398625,5.25742792025325));
#47522=CARTESIAN_POINT('Ctrl Pts',(7.58309345699017,-2.26256685134525,5.26531011982948));
#47523=CARTESIAN_POINT('Ctrl Pts',(7.636952839462,-2.07350975555625,5.27319231940571));
#47524=CARTESIAN_POINT('Ctrl Pts',(7.68369301820594,-1.88275930537426,5.28107451898194));
#47525=CARTESIAN_POINT('Ctrl Pts',(7.73044387766686,-1.69196526632228,5.28895851973962));
#47526=CARTESIAN_POINT('Ctrl Pts',(7.77007220956591,-1.49947743699353,5.2968425204973));
#47527=CARTESIAN_POINT('Ctrl Pts',(7.80247550177028,-1.30587022489777,5.30472652125498));
#47528=CARTESIAN_POINT('Ctrl Pts',(7.8348916511138,-1.11218619237123,5.31261365026562));
#47529=CARTESIAN_POINT('Ctrl Pts',(7.86007699153326,-0.91738223213148,5.32050077927626));
#47530=CARTESIAN_POINT('Ctrl Pts',(7.87798073737355,-0.722039127451784,
5.3283879082869));
#47531=CARTESIAN_POINT('Ctrl Pts',(7.89590358450976,-0.526487613510565,
5.33628345198274));
#47532=CARTESIAN_POINT('Ctrl Pts',(7.90652928827996,-0.330396149926966,
5.34417899567859));
#47533=CARTESIAN_POINT('Ctrl Pts',(7.90985914163195,-0.134347904864651,
5.35207453937443));
#47534=CARTESIAN_POINT('Ctrl Pts',(7.91319102275443,0.0618197270910941,
5.3599748911951));
#47535=CARTESIAN_POINT('Ctrl Pts',(7.90921820287093,0.257943743998826,5.36787524301577));
#47536=CARTESIAN_POINT('Ctrl Pts',(7.89799398724836,0.453444569257142,5.37577559483644));
#47537=CARTESIAN_POINT('Ctrl Pts',(7.88675515720779,0.649199945111568,5.38368623325954));
#47538=CARTESIAN_POINT('Ctrl Pts',(7.8682461047889,0.844330166108271,5.39159687168265));
#47539=CARTESIAN_POINT('Ctrl Pts',(7.8425716791579,1.03826319267825,5.39950751010575));
#47540=CARTESIAN_POINT('Ctrl Pts',(7.83129090286285,1.1234730867729,5.40298327013578));
#47541=CARTESIAN_POINT('Ctrl Pts',(7.81862748948768,1.20845201665567,5.4064590301658));
#47542=CARTESIAN_POINT('Ctrl Pts',(7.80459339720012,1.2931523129084,5.40993479019582));
#47543=CARTESIAN_POINT('Ctrl Pts',(7.77265570572528,1.48590663389456,5.41784465349193));
#47544=CARTESIAN_POINT('Ctrl Pts',(7.73352983042176,1.67773721077236,5.42575451678803));
#47545=CARTESIAN_POINT('Ctrl Pts',(7.68727814727843,1.8680673666588,5.43366438008413));
#47546=CARTESIAN_POINT('Ctrl Pts',(7.64107673028992,2.05819067244958,5.44156564697063));
#47547=CARTESIAN_POINT('Ctrl Pts',(7.58776501155819,2.2468164730727,5.44946691385713));
#47548=CARTESIAN_POINT('Ctrl Pts',(7.52745689775621,2.4333749510551,5.45736818074362));
#47549=CARTESIAN_POINT('Ctrl Pts',(7.46720311987403,2.61976534507904,5.46526232881017));
#47550=CARTESIAN_POINT('Ctrl Pts',(7.3999656095018,2.80409180073171,5.47315647687672));
#47551=CARTESIAN_POINT('Ctrl Pts',(7.32590898403179,2.98579613464856,5.48105062494327));
#47552=CARTESIAN_POINT('Ctrl Pts',(7.25190532428576,3.16737051258193,5.48893912706977));
#47553=CARTESIAN_POINT('Ctrl Pts',(7.17109239582628,3.34632618696021,5.49682762919627));
#47554=CARTESIAN_POINT('Ctrl Pts',(7.08368425729333,3.52212128453502,5.50471613132277));
#47555=CARTESIAN_POINT('Ctrl Pts',(6.99632239972878,3.69782330190595,5.51260045663548));
#47556=CARTESIAN_POINT('Ctrl Pts',(6.9023724436189,3.87036776890524,5.5204847819482));
#47557=CARTESIAN_POINT('Ctrl Pts',(6.80209618146223,4.03923365728414,5.52836910726092));
#47558=CARTESIAN_POINT('Ctrl Pts',(6.70185439298216,4.20804149176372,5.53625072204499));
#47559=CARTESIAN_POINT('Ctrl Pts',(6.5952908090014,4.3731729718368,5.54413233682906));
#47560=CARTESIAN_POINT('Ctrl Pts',(6.48271282612842,4.53413226692276,5.55201395161314));
#47561=CARTESIAN_POINT('Ctrl Pts',(6.37013330588394,4.69509376007823,5.559895674029));
#47562=CARTESIAN_POINT('Ctrl Pts',(6.25153941333028,4.85188266684265,5.56777739644486));
#47563=CARTESIAN_POINT('Ctrl Pts',(6.12728180067544,5.00403224760907,5.57565911886072));
#47564=CARTESIAN_POINT('Ctrl Pts',(6.00301665946148,5.15619104686191,5.58354131881685));
#47565=CARTESIAN_POINT('Ctrl Pts',(5.87308733223298,5.30370969227481,5.59142351877298));
#47566=CARTESIAN_POINT('Ctrl Pts',(5.73788469627472,5.4461546261795,5.5993057187291));
#47567=CARTESIAN_POINT('Ctrl Pts',(5.60265111798718,5.58863215987797,5.607189722597));
#47568=CARTESIAN_POINT('Ctrl Pts',(5.46214206372018,5.72603341797021,5.6150737264649));
#47569=CARTESIAN_POINT('Ctrl Pts',(5.31678535237621,5.85796163496807,5.6229577303328));
#47570=CARTESIAN_POINT('Ctrl Pts',(5.17137091527017,5.98994224484682,5.63084486518878));
#47571=CARTESIAN_POINT('Ctrl Pts',(5.02110524036368,6.11644525098225,5.63873200004477));
#47572=CARTESIAN_POINT('Ctrl Pts',(4.86644947338875,6.23711395782972,5.64661913490075));
#47573=CARTESIAN_POINT('Ctrl Pts',(4.71162862559173,6.3579114674352,5.65451468854855));
#47574=CARTESIAN_POINT('Ctrl Pts',(4.55240859789324,6.47286202630655,5.66241024219636));
#47575=CARTESIAN_POINT('Ctrl Pts',(4.38928069598927,6.58165146234712,5.67030579584416));
#47576=CARTESIAN_POINT('Ctrl Pts',(4.22605340599731,6.69050717996132,5.67820615997486));
#47577=CARTESIAN_POINT('Ctrl Pts',(4.05891378832009,6.79319411100993,5.68610652410555));
#47578=CARTESIAN_POINT('Ctrl Pts',(3.88837824456623,6.88944378213394,5.69400688823624));
#47579=CARTESIAN_POINT('Ctrl Pts',(3.71762058035253,6.98581881727732,5.70191754249458));
#47580=CARTESIAN_POINT('Ctrl Pts',(3.54345846071086,7.07573968723102,5.70982819675292));
#47581=CARTESIAN_POINT('Ctrl Pts',(3.36642981088409,7.15898535606764,5.71773885101126));
#47582=CARTESIAN_POINT('Ctrl Pts',(3.28864660744725,7.19556200510547,5.72121465015505));
#47583=CARTESIAN_POINT('Ctrl Pts',(3.21031022542822,7.23085060300295,5.72469044929885));
#47584=CARTESIAN_POINT('Ctrl Pts',(3.13146723383428,7.26483543952802,5.72816624844264));
#47585=CARTESIAN_POINT('Ctrl Pts',(2.95365582650221,7.34148006561724,5.73600507754929));
#47586=CARTESIAN_POINT('Ctrl Pts',(2.77276024579775,7.41170845372168,5.74384390665593));
#47587=CARTESIAN_POINT('Ctrl Pts',(2.58928861157229,7.47525955977329,5.75168273576258));
#47588=CARTESIAN_POINT('Ctrl Pts',(2.40602264600011,7.53873942609104,5.75951277767205));
#47589=CARTESIAN_POINT('Ctrl Pts',(2.22018670579099,7.59555680085031,5.76734281958153));
#47590=CARTESIAN_POINT('Ctrl Pts',(2.03231158941905,7.64549740720073,5.775172861491));
#47591=CARTESIAN_POINT('Ctrl Pts',(1.84461051228267,7.69539175077233,5.78299564999441));
#47592=CARTESIAN_POINT('Ctrl Pts',(1.65487435830366,7.7384219224363,5.79081843849782));
#47593=CARTESIAN_POINT('Ctrl Pts',(1.46365208603583,7.77442239468907,5.79864122700123));
#47594=CARTESIAN_POINT('Ctrl Pts',(1.27256975658462,7.8103965205993,5.80645829052792));
#47595=CARTESIAN_POINT('Ctrl Pts',(1.08000381908775,7.83935112883234,5.81427535405461));
#47596=CARTESIAN_POINT('Ctrl Pts',(0.88651670175689,7.86117097750113,5.8220924175813));
#47597=CARTESIAN_POINT('Ctrl Pts',(0.693133560898,7.8829791005785,5.82990528035965));
#47598=CARTESIAN_POINT('Ctrl Pts',(0.498830574925137,7.89766006236304,5.83771814313801));
#47599=CARTESIAN_POINT('Ctrl Pts',(0.304178823781853,7.90514998233194,5.84553100591636));
#47600=CARTESIAN_POINT('Ctrl Pts',(0.109593833991573,7.91263733341981,5.85334118905126));
#47601=CARTESIAN_POINT('Ctrl Pts',(-0.085339331573861,7.9129385432862,5.86115137218617));
#47602=CARTESIAN_POINT('Ctrl Pts',(-0.280045841120314,7.90604169776957,
5.86896155532107));
#47603=CARTESIAN_POINT('Ctrl Pts',(-0.47476113216939,7.89914454119675,5.87677209070482));
#47604=CARTESIAN_POINT('Ctrl Pts',(-0.669249394896092,7.8850486838601,5.88458262608857));
#47605=CARTESIAN_POINT('Ctrl Pts',(-0.862936648121897,7.86379433488238,
5.89239316147232));
#47606=CARTESIAN_POINT('Ctrl Pts',(-1.05663942563658,7.84253828234054,5.90020432288079));
#47607=CARTESIAN_POINT('Ctrl Pts',(-1.24954071573259,7.81412263277778,5.90801548428925));
#47608=CARTESIAN_POINT('Ctrl Pts',(-1.44107259283951,7.77863939144673,5.91582664569772));
#47609=CARTESIAN_POINT('Ctrl Pts',(-1.6326535540037,7.74314705679151,5.92363980887999));
#47610=CARTESIAN_POINT('Ctrl Pts',(-1.82286405703168,7.70058358625159,5.93145297206225));
#47611=CARTESIAN_POINT('Ctrl Pts',(-2.0111471371933,7.65109196079613,5.93926613524452));
#47612=CARTESIAN_POINT('Ctrl Pts',(-2.19951163212073,7.6015789348564,5.94708267688677));
#47613=CARTESIAN_POINT('Ctrl Pts',(-2.38594670398052,7.54513187565361,5.95489921852901));
#47614=CARTESIAN_POINT('Ctrl Pts',(-2.5699111494959,7.48194344296298,5.96271576017126));
#47615=CARTESIAN_POINT('Ctrl Pts',(-2.75409028479262,7.41868126824703,5.97054142385669));
#47616=CARTESIAN_POINT('Ctrl Pts',(-2.93579270219555,7.3486621210581,5.97836708754212));
#47617=CARTESIAN_POINT('Ctrl Pts',(-3.11449674320316,7.27212699535541,5.98619275122755));
#47618=CARTESIAN_POINT('Ctrl Pts',(-3.29331726924069,7.19554198160118,5.99402351593175));
#47619=CARTESIAN_POINT('Ctrl Pts',(-3.46913520710748,7.11243267504027,6.00185428063595));
#47620=CARTESIAN_POINT('Ctrl Pts',(-3.6414540154819,7.02308576432972,6.00968504534016));
#47621=CARTESIAN_POINT('Ctrl Pts',(-3.81402180621436,6.93360975683211,6.01752712466683));
#47622=CARTESIAN_POINT('Ctrl Pts',(-3.98308006430326,6.83787831662013,6.02536920399351));
#47623=CARTESIAN_POINT('Ctrl Pts',(-4.14816070635285,6.73622177145841,6.03321128332018));
#47624=CARTESIAN_POINT('Ctrl Pts',(-4.24068817453482,6.67924342056785,6.03760675777661));
#47625=CARTESIAN_POINT('Ctrl Pts',(-4.3319666145367,6.6204043905575,6.04200223223303));
#47626=CARTESIAN_POINT('Ctrl Pts',(-4.42191828936477,6.55976826131696,6.04639770668946));
#47627=CARTESIAN_POINT('Ctrl Pts',(-4.58340604536027,6.45090989417677,6.05428878051171));
#47628=CARTESIAN_POINT('Ctrl Pts',(-4.7411067374536,6.33592622752953,6.06217985433396));
#47629=CARTESIAN_POINT('Ctrl Pts',(-4.89452224960557,6.21510844218474,6.07007092815622));
#47630=CARTESIAN_POINT('Ctrl Pts',(-5.04776084545647,6.09442998196677,6.07795290211906));
#47631=CARTESIAN_POINT('Ctrl Pts',(-5.19672383319295,5.96793101483532,6.0858348760819));
#47632=CARTESIAN_POINT('Ctrl Pts',(-5.34094036450682,5.83594696881164,6.09371685004475));
#47633=CARTESIAN_POINT('Ctrl Pts',(-5.48501781815481,5.70409020384851,6.10159122289188));
#47634=CARTESIAN_POINT('Ctrl Pts',(-5.62435767852726,5.56675912887002,6.10946559573902));
#47635=CARTESIAN_POINT('Ctrl Pts',(-5.75852041490217,5.42433070812934,6.11733996858615));
#47636=CARTESIAN_POINT('Ctrl Pts',(-5.89257909164205,5.28201275807434,6.12520823389265));
#47637=CARTESIAN_POINT('Ctrl Pts',(-6.0214684068441,5.13460558984344,6.13307649919915));
#47638=CARTESIAN_POINT('Ctrl Pts',(-6.14478392051677,4.98252461811867,6.14094476450564));
#47639=CARTESIAN_POINT('Ctrl Pts',(-6.26802705681479,4.83053290703224,6.14880841170393));
#47640=CARTESIAN_POINT('Ctrl Pts',(-6.38570269162808,4.67387312693333,6.15667205890222));
#47641=CARTESIAN_POINT('Ctrl Pts',(-6.49744493742192,4.51299571074139,6.16453570610051));
#47642=CARTESIAN_POINT('Ctrl Pts',(-6.61176264344172,4.34841035594743,6.17258059639487));
#47643=CARTESIAN_POINT('Ctrl Pts',(-6.71986989774841,4.17941087149798,6.18062548668924));
#47644=CARTESIAN_POINT('Ctrl Pts',(-6.82141967250549,4.00651402737531,6.1886703769836));
#47645=CARTESIAN_POINT('Ctrl Pts',(-6.92063477014604,3.8375921630737,6.19653031146373));
#47646=CARTESIAN_POINT('Ctrl Pts',(-7.01359042491432,3.66495049636911,6.20439024594387));
#47647=CARTESIAN_POINT('Ctrl Pts',(-7.10000779725799,3.48909877746042,6.212250180424));
#47648=CARTESIAN_POINT('Ctrl Pts',(-7.18642677923157,3.31324378309705,6.22011026130508));
#47649=CARTESIAN_POINT('Ctrl Pts',(-7.26630708264474,3.13417892894322,6.22797034218617));
#47650=CARTESIAN_POINT('Ctrl Pts',(-7.33941668836165,2.95243690442293,6.23583042306725));
#47651=CARTESIAN_POINT('Ctrl Pts',(-7.41254015222441,2.77066043015481,6.24369199385033));
#47652=CARTESIAN_POINT('Ctrl Pts',(-7.47889023200438,2.58620609670518,6.25155356463341));
#47653=CARTESIAN_POINT('Ctrl Pts',(-7.5382836731742,2.39962502544777,6.25941513541648));
#47654=CARTESIAN_POINT('Ctrl Pts',(-7.60010670235002,2.20541154354125,6.26759829689555));
#47655=CARTESIAN_POINT('Ctrl Pts',(-7.65439183267923,2.00889405926646,6.27578145837461));
#47656=CARTESIAN_POINT('Ctrl Pts',(-7.70099040580724,1.81070918970022,6.28396461985367));
#47657=CARTESIAN_POINT('Ctrl Pts',(-7.74581800068916,1.62005633386632,6.29183678037303));
#47658=CARTESIAN_POINT('Ctrl Pts',(-7.78353249133439,1.42786084217599,6.29970894089239));
#47659=CARTESIAN_POINT('Ctrl Pts',(-7.81405419343074,1.23469755897039,6.30758110141175));
#47660=CARTESIAN_POINT('Ctrl Pts',(-7.84459391678191,1.04142022430274,6.31545790997499));
#47661=CARTESIAN_POINT('Ctrl Pts',(-7.86793234444799,0.847174302690902,
6.32333471853823));
#47662=CARTESIAN_POINT('Ctrl Pts',(-7.88404177619998,0.652538329244746,
6.33121152710147));
#47663=CARTESIAN_POINT('Ctrl Pts',(-7.90016949112144,0.457681456480474,
6.33909727533608));
#47664=CARTESIAN_POINT('Ctrl Pts',(-7.90905181413018,0.262433993324727,
6.3469830235707));
#47665=CARTESIAN_POINT('Ctrl Pts',(-7.91071310043852,0.067373901106895,
6.35486877180531));
#47666=CARTESIAN_POINT('Ctrl Pts',(-7.9109058139321,0.0447464276609003,
6.35578353892529));
#47667=CARTESIAN_POINT('Ctrl Pts',(-7.91100141416754,0.0221214693622712,
6.35669830604527));
#47668=CARTESIAN_POINT('Ctrl Pts',(-7.91099998419434,-0.000500077126143346,
6.35761307316525));
#47669=CARTESIAN_POINT('',(-7.911,-8.41493541514637E-12,8.35766849176337));
#47670=CARTESIAN_POINT('Ctrl Pts',(-7.9109999835323,-0.000497167457162866,
6.35768849598628));
#47671=CARTESIAN_POINT('Ctrl Pts',(-7.9108541427804,-2.20200474133999,6.44626926364471));
#47672=CARTESIAN_POINT('Ctrl Pts',(-6.9420229263903,-4.38621542289884,6.53485003130312));
#47673=CARTESIAN_POINT('Ctrl Pts',(-3.67820201487512,-7.34180684108019,
6.71201823469427));
#47674=CARTESIAN_POINT('Ctrl Pts',(-1.40868175870894,-8.08992666571484,
6.800605670427));
#47675=CARTESIAN_POINT('Ctrl Pts',(2.97309270522073,-7.65454228024946,6.97778054189245));
#47676=CARTESIAN_POINT('Ctrl Pts',(5.05102072676276,-6.47444880833699,7.06636797762517));
#47677=CARTESIAN_POINT('Ctrl Pts',(7.66951518848174,-2.93425195366914,7.24354284909062));
#47678=CARTESIAN_POINT('Ctrl Pts',(8.18956872247132,-0.601881960090737,
7.33213028482335));
#47679=CARTESIAN_POINT('Ctrl Pts',(7.32306689760962,3.71537198233198,7.5093051562888));
#47680=CARTESIAN_POINT('Ctrl Pts',(5.94329958849624,5.66643518937116,7.59789259202152));
#47681=CARTESIAN_POINT('Ctrl Pts',(2.16154501637046,7.92205913233216,7.77506746348697));
#47682=CARTESIAN_POINT('Ctrl Pts',(-0.210816529308643,8.2089496371298,7.8636548992197));
#47683=CARTESIAN_POINT('Ctrl Pts',(-4.4212390857713,6.91982244717388,8.04082977068514));
#47684=CARTESIAN_POINT('Ctrl Pts',(-6.22631625634721,5.35390358802899,8.12941720641787));
#47685=CARTESIAN_POINT('Ctrl Pts',(-7.65317280859726,2.31334857513741,8.26455925868819));
#47686=CARTESIAN_POINT('Ctrl Pts',(-7.91100000000123,1.15702837835696,8.31111387522578));
#47687=CARTESIAN_POINT('Ctrl Pts',(-7.911,-8.41493541514637E-12,8.35766849176337));
#47688=CARTESIAN_POINT('',(-7.90360519151496,-0.00207662742780917,10.3576684917634));
#47689=CARTESIAN_POINT('Ctrl Pts',(-7.911,-8.41493541514637E-12,8.35766849176337));
#47690=CARTESIAN_POINT('Ctrl Pts',(-7.91099999999766,-2.20167589667516,
8.4462559274961));
#47691=CARTESIAN_POINT('Ctrl Pts',(-6.94214576671907,-4.38610418339416,
8.53484336322882));
#47692=CARTESIAN_POINT('Ctrl Pts',(-3.67820201487515,-7.34180684108018,
8.71201823469427));
#47693=CARTESIAN_POINT('Ctrl Pts',(-1.40868175870897,-8.08992666571483,
8.800605670427));
#47694=CARTESIAN_POINT('Ctrl Pts',(2.9730927052207,-7.65454228024947,8.97778054189244));
#47695=CARTESIAN_POINT('Ctrl Pts',(5.05102072676273,-6.47444880833701,9.06636797762517));
#47696=CARTESIAN_POINT('Ctrl Pts',(7.66951518848173,-2.93425195366917,9.24354284909062));
#47697=CARTESIAN_POINT('Ctrl Pts',(8.18956872247132,-0.601881960090768,
9.33213028482334));
#47698=CARTESIAN_POINT('Ctrl Pts',(7.32306689760963,3.71537198233196,9.50930515628879));
#47699=CARTESIAN_POINT('Ctrl Pts',(5.94329958849626,5.66643518937113,9.59789259202152));
#47700=CARTESIAN_POINT('Ctrl Pts',(2.16154501637049,7.92205913233215,9.77506746348697));
#47701=CARTESIAN_POINT('Ctrl Pts',(-0.210816529308611,8.2089496371298,9.86365489921969));
#47702=CARTESIAN_POINT('Ctrl Pts',(-4.42123908577128,6.91982244717389,10.0408297706851));
#47703=CARTESIAN_POINT('Ctrl Pts',(-6.22631625634721,5.353903588029,10.1294172064179));
#47704=CARTESIAN_POINT('Ctrl Pts',(-7.65317280859726,2.31334857513742,10.2645592586882));
#47705=CARTESIAN_POINT('Ctrl Pts',(-7.91100000000123,1.15702837835698,10.3111138752258));
#47706=CARTESIAN_POINT('Ctrl Pts',(-7.911,-8.38551450499381E-12,10.3576684917634));
#47707=CARTESIAN_POINT('',(-7.91571978525191,-0.0020331227406836,12.3575752383775));
#47708=CARTESIAN_POINT('Ctrl Pts',(-7.89834820152432,-0.00355290765606358,
10.3576684917634));
#47709=CARTESIAN_POINT('Ctrl Pts',(-7.90111396095795,-1.2014871786324,10.4056583685572));
#47710=CARTESIAN_POINT('Ctrl Pts',(-7.08241423273656,-5.0426308771058,10.5597253981002));
#47711=CARTESIAN_POINT('Ctrl Pts',(-2.32675483040277,-8.41269614686096,
10.7668310040172));
#47712=CARTESIAN_POINT('Ctrl Pts',(3.05913169433092,-7.63406331823264,10.9789853095152));
#47713=CARTESIAN_POINT('Ctrl Pts',(7.4923240719073,-4.47798219086958,11.191139615013));
#47714=CARTESIAN_POINT('Ctrl Pts',(8.91679478215701,2.84829431800013,11.4563324968853));
#47715=CARTESIAN_POINT('Ctrl Pts',(2.41200260105483,9.04380386318945,11.7745639551321));
#47716=CARTESIAN_POINT('Ctrl Pts',(-5.80949993071132,7.0346858171147,12.0749618174482));
#47717=CARTESIAN_POINT('Ctrl Pts',(-7.89632373226713,2.18652121168757,12.2692825270153));
#47718=CARTESIAN_POINT('Ctrl Pts',(-7.91703408569381,-0.00202294616919351,
12.3575260838335));
#47719=CARTESIAN_POINT('',(-7.91661424246722,0.00191610784238723,14.357737223299));
#47720=CARTESIAN_POINT('Ctrl Pts',(-7.91099971462202,-0.00206967004347107,
12.3577517679683));
#47721=CARTESIAN_POINT('Ctrl Pts',(-7.9103927569587,-2.20304480169943,12.4463114449661));
#47722=CARTESIAN_POINT('Ctrl Pts',(-6.94163439087416,-4.38656726580578,
12.5348711219638));
#47723=CARTESIAN_POINT('Ctrl Pts',(-3.67820201487507,-7.34180684108022,
12.7120182346943));
#47724=CARTESIAN_POINT('Ctrl Pts',(-1.40868175870889,-8.08992666571485,
12.800605670427));
#47725=CARTESIAN_POINT('Ctrl Pts',(2.97309270522078,-7.65454228024944,12.9777805418925));
#47726=CARTESIAN_POINT('Ctrl Pts',(5.0510207267628,-6.47444880833696,13.0663679776252));
#47727=CARTESIAN_POINT('Ctrl Pts',(7.66951518848176,-2.93425195366909,13.2435428490906));
#47728=CARTESIAN_POINT('Ctrl Pts',(8.18956872247133,-0.601881960090685,
13.3321302848233));
#47729=CARTESIAN_POINT('Ctrl Pts',(7.3230668976096,3.71537198233203,13.5093051562888));
#47730=CARTESIAN_POINT('Ctrl Pts',(5.9432995884962,5.6664351893712,13.5978925920215));
#47731=CARTESIAN_POINT('Ctrl Pts',(2.16154501637041,7.92205913233217,13.775067463487));
#47732=CARTESIAN_POINT('Ctrl Pts',(-0.210816529308695,8.2089496371298,13.8636548992197));
#47733=CARTESIAN_POINT('Ctrl Pts',(-4.42123908577134,6.91982244717385,14.0408297706851));
#47734=CARTESIAN_POINT('Ctrl Pts',(-6.22631625634725,5.35390358802895,14.1294172064179));
#47735=CARTESIAN_POINT('Ctrl Pts',(-7.65289632442553,2.31393774812261,14.2645330720065));
#47736=CARTESIAN_POINT('Ctrl Pts',(-7.91070987367968,1.15832918971538,14.3110615018624));
#47737=CARTESIAN_POINT('Ctrl Pts',(-7.91099975527532,0.00195246306002456,
14.3575899317182));
#47738=CARTESIAN_POINT('',(-7.90441257296093,0.00229462530749312,16.3576684917634));
#47739=CARTESIAN_POINT('Ctrl Pts',(-7.91882171999131,0.00190181386983465,
14.3577951347062));
#47740=CARTESIAN_POINT('Ctrl Pts',(-7.90092880425392,-2.31733288374248,
14.4514124495886));
#47741=CARTESIAN_POINT('Ctrl Pts',(-5.60174024730873,-7.29337738801806,
14.65110691722));
#47742=CARTESIAN_POINT('Ctrl Pts',(2.87741498209291,-8.90744030178522,14.9568785376003));
#47743=CARTESIAN_POINT('Ctrl Pts',(8.00355842970691,-3.48285758573526,15.2220714194727));
#47744=CARTESIAN_POINT('Ctrl Pts',(7.9874613863806,1.95899721059107,15.4342257249706));
#47745=CARTESIAN_POINT('Ctrl Pts',(5.483858582018,6.79076870116109,15.6463800304684));
#47746=CARTESIAN_POINT('Ctrl Pts',(-1.57046161563201,9.22798244595634,15.9115729123407));
#47747=CARTESIAN_POINT('Ctrl Pts',(-7.21150187483662,4.76683328138724,16.166348591564));
#47748=CARTESIAN_POINT('Ctrl Pts',(-7.90585355722926,1.066076564084,16.3150471180381));
#47749=CARTESIAN_POINT('Ctrl Pts',(-7.90052382745844,0.00364920788198668,
16.3576684917634));
#47750=CARTESIAN_POINT('',(-7.911,-8.60200799479571E-12,18.3576684917634));
#47751=CARTESIAN_POINT('Ctrl Pts',(-7.911,-8.60422844084496E-12,16.3576684917634));
#47752=CARTESIAN_POINT('Ctrl Pts',(-7.9109999999976,-2.20167589667533,16.4462559274961));
#47753=CARTESIAN_POINT('Ctrl Pts',(-6.94214576671898,-4.38610418339429,
16.5348433632288));
#47754=CARTESIAN_POINT('Ctrl Pts',(-3.67820201487504,-7.34180684108023,
16.7120182346943));
#47755=CARTESIAN_POINT('Ctrl Pts',(-1.40868175870887,-8.08992666571484,
16.800605670427));
#47756=CARTESIAN_POINT('Ctrl Pts',(2.97309270522075,-7.65454228024944,16.9777805418924));
#47757=CARTESIAN_POINT('Ctrl Pts',(5.05102072676276,-6.47444880833699,17.0663679776252));
#47758=CARTESIAN_POINT('Ctrl Pts',(7.66951518848173,-2.93425195366916,17.2435428490906));
#47759=CARTESIAN_POINT('Ctrl Pts',(8.18956872247132,-0.601881960090787,
17.3321302848233));
#47760=CARTESIAN_POINT('Ctrl Pts',(7.32306689760966,3.7153719823319,17.5093051562888));
#47761=CARTESIAN_POINT('Ctrl Pts',(5.94329958849631,5.66643518937107,17.5978925920215));
#47762=CARTESIAN_POINT('Ctrl Pts',(2.1615450163706,7.92205913233211,17.775067463487));
#47763=CARTESIAN_POINT('Ctrl Pts',(-0.210816529308475,8.2089496371298,17.8636548992197));
#47764=CARTESIAN_POINT('Ctrl Pts',(-4.42123908577112,6.91982244717398,18.0408297706851));
#47765=CARTESIAN_POINT('Ctrl Pts',(-6.22631625634706,5.35390358802916,18.1294172064179));
#47766=CARTESIAN_POINT('Ctrl Pts',(-7.65317280859725,2.31334857513751,18.2645592586882));
#47767=CARTESIAN_POINT('Ctrl Pts',(-7.91100000000126,1.15702837835691,18.3111138752258));
#47768=CARTESIAN_POINT('Ctrl Pts',(-7.911,-8.60200799479571E-12,18.3576684917634));
#47769=CARTESIAN_POINT('',(-7.911,-8.71303029725823E-12,20.3576684917634));
#47770=CARTESIAN_POINT('Ctrl Pts',(-7.911,-8.60200799479571E-12,18.3576684917634));
#47771=CARTESIAN_POINT('Ctrl Pts',(-7.91099999999761,-2.20167589667534,
18.4462559274961));
#47772=CARTESIAN_POINT('Ctrl Pts',(-6.94214576671897,-4.38610418339433,
18.5348433632288));
#47773=CARTESIAN_POINT('Ctrl Pts',(-3.67820201487497,-7.34180684108027,
18.7120182346943));
#47774=CARTESIAN_POINT('Ctrl Pts',(-1.40868175870878,-8.08992666571486,
18.800605670427));
#47775=CARTESIAN_POINT('Ctrl Pts',(2.97309270522088,-7.6545422802494,18.9777805418925));
#47776=CARTESIAN_POINT('Ctrl Pts',(5.05102072676288,-6.47444880833689,19.0663679776252));
#47777=CARTESIAN_POINT('Ctrl Pts',(7.6695151884818,-2.93425195366899,19.2435428490906));
#47778=CARTESIAN_POINT('Ctrl Pts',(8.18956872247134,-0.601881960090575,
19.3321302848234));
#47779=CARTESIAN_POINT('Ctrl Pts',(7.32306689760955,3.71537198233213,19.5093051562888));
#47780=CARTESIAN_POINT('Ctrl Pts',(5.94329958849612,5.66643518937128,19.5978925920215));
#47781=CARTESIAN_POINT('Ctrl Pts',(2.1615450163703,7.9220591323322,19.775067463487));
#47782=CARTESIAN_POINT('Ctrl Pts',(-0.210816529308805,8.2089496371298,19.8636548992197));
#47783=CARTESIAN_POINT('Ctrl Pts',(-4.42123908577143,6.91982244717379,20.0408297706851));
#47784=CARTESIAN_POINT('Ctrl Pts',(-6.22631625634732,5.35390358802887,20.1294172064179));
#47785=CARTESIAN_POINT('Ctrl Pts',(-7.65317280859733,2.31334857513722,20.2645592586882));
#47786=CARTESIAN_POINT('Ctrl Pts',(-7.91100000000127,1.15702837835671,20.3111138752258));
#47787=CARTESIAN_POINT('Ctrl Pts',(-7.911,-8.71303029725823E-12,20.3576684917634));
#47788=CARTESIAN_POINT('',(-7.911,-8.76687611395255E-12,22.3576684917634));
#47789=CARTESIAN_POINT('Ctrl Pts',(-7.911,-8.71303029725823E-12,20.3576684917634));
#47790=CARTESIAN_POINT('Ctrl Pts',(-7.91099999999757,-2.20167589667551,
20.4462559274961));
#47791=CARTESIAN_POINT('Ctrl Pts',(-6.94214576671885,-4.38610418339453,
20.5348433632288));
#47792=CARTESIAN_POINT('Ctrl Pts',(-3.67820201487467,-7.34180684108043,
20.7120182346943));
#47793=CARTESIAN_POINT('Ctrl Pts',(-1.40868175870837,-8.08992666571495,
20.800605670427));
#47794=CARTESIAN_POINT('Ctrl Pts',(2.97309270522137,-7.65454228024923,20.9777805418925));
#47795=CARTESIAN_POINT('Ctrl Pts',(5.05102072676335,-6.47444880833655,21.0663679776252));
#47796=CARTESIAN_POINT('Ctrl Pts',(7.66951518848206,-2.93425195366835,21.2435428490907));
#47797=CARTESIAN_POINT('Ctrl Pts',(8.18956872247141,-0.601881960089817,
21.3321302848234));
#47798=CARTESIAN_POINT('Ctrl Pts',(7.32306689760917,3.71537198233291,21.5093051562888));
#47799=CARTESIAN_POINT('Ctrl Pts',(5.94329958849549,5.66643518937196,21.5978925920216));
#47800=CARTESIAN_POINT('Ctrl Pts',(2.1615450163693,7.92205913233249,21.775067463487));
#47801=CARTESIAN_POINT('Ctrl Pts',(-0.210816529309916,8.20894963712979,
21.8636548992197));
#47802=CARTESIAN_POINT('Ctrl Pts',(-4.42123908577247,6.91982244717315,22.0408297706852));
#47803=CARTESIAN_POINT('Ctrl Pts',(-6.22631625634817,5.3539035880279,22.1294172064179));
#47804=CARTESIAN_POINT('Ctrl Pts',(-7.65317280859753,2.31334857513634,22.2645592586882));
#47805=CARTESIAN_POINT('Ctrl Pts',(-7.91100000000128,1.15702837835624,22.3111138752258));
#47806=CARTESIAN_POINT('Ctrl Pts',(-7.911,-8.76687611395255E-12,22.3576684917634));
#47807=CARTESIAN_POINT('',(-7.90652056602762,-0.000845387666311545,24.3576684917634));
#47808=CARTESIAN_POINT('Ctrl Pts',(-7.911,-8.76687611395255E-12,22.3576684917634));
#47809=CARTESIAN_POINT('Ctrl Pts',(-7.91099999999756,-2.20167589667553,
22.4462559274961));
#47810=CARTESIAN_POINT('Ctrl Pts',(-6.94214576671886,-4.38610418339451,
22.5348433632288));
#47811=CARTESIAN_POINT('Ctrl Pts',(-3.67820201487475,-7.34180684108038,
22.7120182346943));
#47812=CARTESIAN_POINT('Ctrl Pts',(-1.40868175870851,-8.08992666571492,
22.800605670427));
#47813=CARTESIAN_POINT('Ctrl Pts',(2.97309270522117,-7.65454228024929,22.9777805418925));
#47814=CARTESIAN_POINT('Ctrl Pts',(5.05102072676315,-6.4744488083367,23.0663679776252));
#47815=CARTESIAN_POINT('Ctrl Pts',(7.66951518848194,-2.93425195366865,23.2435428490906));
#47816=CARTESIAN_POINT('Ctrl Pts',(8.18956872247137,-0.60188196009019,23.3321302848234));
#47817=CARTESIAN_POINT('Ctrl Pts',(7.32306689760936,3.71537198233251,23.5093051562888));
#47818=CARTESIAN_POINT('Ctrl Pts',(5.94329958849582,5.6664351893716,23.5978925920215));
#47819=CARTESIAN_POINT('Ctrl Pts',(2.16154501636984,7.92205913233233,23.775067463487));
#47820=CARTESIAN_POINT('Ctrl Pts',(-0.210816529309308,8.20894963712979,
23.8636548992197));
#47821=CARTESIAN_POINT('Ctrl Pts',(-4.42123908577189,6.91982244717351,24.0408297706852));
#47822=CARTESIAN_POINT('Ctrl Pts',(-6.22631625634769,5.35390358802845,24.1294172064179));
#47823=CARTESIAN_POINT('Ctrl Pts',(-7.65317280859741,2.31334857513685,24.2645592586882));
#47824=CARTESIAN_POINT('Ctrl Pts',(-7.91100000000127,1.15702837835653,24.3111138752258));
#47825=CARTESIAN_POINT('Ctrl Pts',(-7.911,-8.70858940515973E-12,24.3576684917634));
#47826=CARTESIAN_POINT('',(-7.91126158341924,-0.001405488932413,26.3574794111892));
#47827=CARTESIAN_POINT('Ctrl Pts',(-7.90426632794342,-0.00127082201034442,
24.3576684917634));
#47828=CARTESIAN_POINT('Ctrl Pts',(-7.9058497364464,-1.21571962861209,24.4063864228439));
#47829=CARTESIAN_POINT('Ctrl Pts',(-7.05373471379606,-5.07204213544585,
24.5611815066734));
#47830=CARTESIAN_POINT('Ctrl Pts',(-1.05237152432548,-9.30131839492834,
24.8220537432516));
#47831=CARTESIAN_POINT('Ctrl Pts',(7.26337396731614,-5.90351958362561,25.1402852014985));
#47832=CARTESIAN_POINT('Ctrl Pts',(8.88769428104811,2.91399200048715,25.4585166597452));
#47833=CARTESIAN_POINT('Ctrl Pts',(2.35795283017753,9.05804632986584,25.7767481179922));
#47834=CARTESIAN_POINT('Ctrl Pts',(-5.84663248951178,7.00016475381016,26.0764023684734));
#47835=CARTESIAN_POINT('Ctrl Pts',(-7.88980521203094,2.17032634514267,26.2699794662058));
#47836=CARTESIAN_POINT('Ctrl Pts',(-7.91126158341924,-0.001405488932413,
26.3574794111892));
#47837=CARTESIAN_POINT('',(-7.91099988262543,0.00136275470605475,28.3577729727994));
#47838=CARTESIAN_POINT('Ctrl Pts',(-7.91099986978392,-0.00139804521138159,
26.3577247441145));
#47839=CARTESIAN_POINT('Ctrl Pts',(-7.91058982688626,-2.20260059530338,
26.4462934290635));
#47840=CARTESIAN_POINT('Ctrl Pts',(-6.94180033678989,-4.38641699152991,
26.5348621140125));
#47841=CARTESIAN_POINT('Ctrl Pts',(-3.67820201487476,-7.34180684108038,
26.7120182346943));
#47842=CARTESIAN_POINT('Ctrl Pts',(-1.40868175870852,-8.08992666571491,
26.800605670427));
#47843=CARTESIAN_POINT('Ctrl Pts',(2.97309270522116,-7.6545422802493,26.9777805418925));
#47844=CARTESIAN_POINT('Ctrl Pts',(5.05102072676314,-6.4744488083367,27.0663679776252));
#47845=CARTESIAN_POINT('Ctrl Pts',(7.66951518848193,-2.93425195366865,27.2435428490906));
#47846=CARTESIAN_POINT('Ctrl Pts',(8.18956872247137,-0.601881960090193,
27.3321302848234));
#47847=CARTESIAN_POINT('Ctrl Pts',(7.32306689760936,3.7153719823325,27.5093051562888));
#47848=CARTESIAN_POINT('Ctrl Pts',(5.94329958849583,5.6664351893716,27.5978925920215));
#47849=CARTESIAN_POINT('Ctrl Pts',(2.16154501636984,7.92205913233233,27.775067463487));
#47850=CARTESIAN_POINT('Ctrl Pts',(-0.210816529309305,8.20894963712979,
27.8636548992197));
#47851=CARTESIAN_POINT('Ctrl Pts',(-4.42123908577189,6.91982244717351,28.0408297706852));
#47852=CARTESIAN_POINT('Ctrl Pts',(-6.22631625634769,5.35390358802845,28.1294172064179));
#47853=CARTESIAN_POINT('Ctrl Pts',(-7.65298073882793,2.31375786554483,28.2645410671589));
#47854=CARTESIAN_POINT('Ctrl Pts',(-7.91079846890045,1.1579320415085,28.3110774921671));
#47855=CARTESIAN_POINT('Ctrl Pts',(-7.91099988189791,0.00135634950828223,
28.3576139171754));
#47856=CARTESIAN_POINT('',(-7.91116372059493,0.00341841640445254,30.3575613031839));
#47857=CARTESIAN_POINT('Ctrl Pts',(-7.91099988262543,0.00136275470605475,
28.3577729727994));
#47858=CARTESIAN_POINT('Ctrl Pts',(-7.91103304674915,-0.191160065200167,
28.3655621021175));
#47859=CARTESIAN_POINT('Ctrl Pts',(-7.9040340849586,-0.383975128877379,
28.3733512314357));
#47860=CARTESIAN_POINT('Ctrl Pts',(-7.88996501489689,-0.576518051498078,
28.3811403607538));
#47861=CARTESIAN_POINT('Ctrl Pts',(-7.87591085565761,-0.768856911354393,
28.3889212349191));
#47862=CARTESIAN_POINT('Ctrl Pts',(-7.85480153216924,-0.960923852310489,
28.3967021090843));
#47863=CARTESIAN_POINT('Ctrl Pts',(-7.8266510171243,-1.15215227125028,28.4044829832496));
#47864=CARTESIAN_POINT('Ctrl Pts',(-7.7985247063564,-1.34321626884203,28.4122571672909));
#47865=CARTESIAN_POINT('Ctrl Pts',(-7.76336931069869,-1.53344282962111,
28.4200313513323));
#47866=CARTESIAN_POINT('Ctrl Pts',(-7.7212507718984,-1.72226813169681,28.4278055353736));
#47867=CARTESIAN_POINT('Ctrl Pts',(-7.67916003024605,-1.91096881394933,
28.4355745886543));
#47868=CARTESIAN_POINT('Ctrl Pts',(-7.63011537485797,-2.09826973266808,
28.4433436419349));
#47869=CARTESIAN_POINT('Ctrl Pts',(-7.57423424038156,-2.28361482562879,
28.4511126952156));
#47870=CARTESIAN_POINT('Ctrl Pts',(-7.51737570576517,-2.47220173394455,
28.4590176346738));
#47871=CARTESIAN_POINT('Ctrl Pts',(-7.45343937646802,-2.65876339351354,
28.4669225741321));
#47872=CARTESIAN_POINT('Ctrl Pts',(-7.38260290411685,-2.84272674735462,
28.4748275135903));
#47873=CARTESIAN_POINT('Ctrl Pts',(-7.31302578234416,-3.02341954934032,
28.4825919168283));
#47874=CARTESIAN_POINT('Ctrl Pts',(-7.23679194854965,-3.20160531616111,
28.4903563200663));
#47875=CARTESIAN_POINT('Ctrl Pts',(-7.15411941173772,-3.37675827423248,
28.4981207233043));
#47876=CARTESIAN_POINT('Ctrl Pts',(-7.07144832537299,-3.55190815933518,
28.5058849903198));
#47877=CARTESIAN_POINT('Ctrl Pts',(-6.98233891285306,-3.72402501899075,
28.5136492573354));
#47878=CARTESIAN_POINT('Ctrl Pts',(-6.88705639282087,-3.89260519987646,
28.5214135243509));
#47879=CARTESIAN_POINT('Ctrl Pts',(-6.79175831210266,-4.06121291176431,
28.5291790593569));
#47880=CARTESIAN_POINT('Ctrl Pts',(-6.69028529202385,-4.22628248442844,
28.5369445943628));
#47881=CARTESIAN_POINT('Ctrl Pts',(-6.58294740138362,-4.3873368357828,28.5447101293687));
#47882=CARTESIAN_POINT('Ctrl Pts',(-6.47222914983099,-4.55346322489422,
28.5527202221058));
#47883=CARTESIAN_POINT('Ctrl Pts',(-6.35527081706428,-4.71531701900264,
28.5607303148429));
#47884=CARTESIAN_POINT('Ctrl Pts',(-6.23245913855011,-4.87240947440824,
28.5687404075799));
#47885=CARTESIAN_POINT('Ctrl Pts',(-6.1132398452078,-5.02490679184133,28.5765161957401));
#47886=CARTESIAN_POINT('Ctrl Pts',(-5.98850508880372,-5.17291715927829,
28.5842919839002));
#47887=CARTESIAN_POINT('Ctrl Pts',(-5.8586475387481,-5.31602953497446,28.5920677720604));
#47888=CARTESIAN_POINT('Ctrl Pts',(-5.72292057371531,-5.46561042883512,
28.6001950170859));
#47889=CARTESIAN_POINT('Ctrl Pts',(-5.58159729495791,-5.60983996416175,
28.6083222621114));
#47890=CARTESIAN_POINT('Ctrl Pts',(-5.43516607510868,-5.74829459370235,
28.6164495071369));
#47891=CARTESIAN_POINT('Ctrl Pts',(-5.28873485525947,-5.88674922324294,
28.6245767521624));
#47892=CARTESIAN_POINT('Ctrl Pts',(-5.13719606725288,-6.01942870847893,
28.632703997188));
#47893=CARTESIAN_POINT('Ctrl Pts',(-4.98107366476083,-6.14596014844109,
28.6408312422135));
#47894=CARTESIAN_POINT('Ctrl Pts',(-4.82135188567672,-6.27540875016794,
28.6491458595509));
#47895=CARTESIAN_POINT('Ctrl Pts',(-4.65644385003665,-6.39873902158748,
28.6574604768884));
#47896=CARTESIAN_POINT('Ctrl Pts',(-4.48683443849475,-6.51553817589441,
28.6657750942259));
#47897=CARTESIAN_POINT('Ctrl Pts',(-4.31743465568261,-6.63219297230204,
28.6740794351131));
#47898=CARTESIAN_POINT('Ctrl Pts',(-4.14334532639385,-6.74233258546919,
28.6823837760004));
#47899=CARTESIAN_POINT('Ctrl Pts',(-3.96508381650821,-6.84558480541032,
28.6906881168877));
#47900=CARTESIAN_POINT('Ctrl Pts',(-3.78703084525463,-6.94871623608675,
28.6989827429695));
#47901=CARTESIAN_POINT('Ctrl Pts',(-3.60481568117551,-7.04497619738786,
28.7072773690513));
#47902=CARTESIAN_POINT('Ctrl Pts',(-3.41898474863096,-7.1340356242893,28.7155719951331));
#47903=CARTESIAN_POINT('Ctrl Pts',(-3.23343362076888,-7.22296095486823,
28.723854132039));
#47904=CARTESIAN_POINT('Ctrl Pts',(-3.04427785290794,-7.30470726108928,
28.7321362689448));
#47905=CARTESIAN_POINT('Ctrl Pts',(-2.85208860341916,-7.37899123175022,
28.7404184058506));
#47906=CARTESIAN_POINT('Ctrl Pts',(-2.66007658993801,-7.45320669808832,
28.7486929050094));
#47907=CARTESIAN_POINT('Ctrl Pts',(-2.46503694599074,-7.51997344672542,
28.7569674041682));
#47908=CARTESIAN_POINT('Ctrl Pts',(-2.26756262496539,-7.57905539904941,
28.7652419033269));
#47909=CARTESIAN_POINT('Ctrl Pts',(-2.07031543065522,-7.6380693977798,28.7735068855024));
#47910=CARTESIAN_POINT('Ctrl Pts',(-1.87063942731905,-7.68941615348493,
28.7817718676779));
#47911=CARTESIAN_POINT('Ctrl Pts',(-1.66914488557447,-7.73290866045633,
28.7900368498533));
#47912=CARTESIAN_POINT('Ctrl Pts',(-1.58861091931513,-7.75029188115623,
28.7933402236812));
#47913=CARTESIAN_POINT('Ctrl Pts',(-1.50778664199549,-7.76642096191549,
28.796643597509));
#47914=CARTESIAN_POINT('Ctrl Pts',(-1.42671173387857,-7.7812861808581,28.7999469713369));
#47915=CARTESIAN_POINT('Ctrl Pts',(-1.22383658821642,-7.81848367547545,
28.8082130608344));
#47916=CARTESIAN_POINT('Ctrl Pts',(-1.01962085420059,-7.84772174840313,
28.816479150332));
#47917=CARTESIAN_POINT('Ctrl Pts',(-0.814700864793647,-7.86893788899776,
28.8247452398296));
#47918=CARTESIAN_POINT('Ctrl Pts',(-0.609596590557578,-7.89017310929688,
28.8330187630328));
#47919=CARTESIAN_POINT('Ctrl Pts',(-0.40378708867809,-7.90337196488202,
28.8412922862361));
#47920=CARTESIAN_POINT('Ctrl Pts',(-0.19791119255603,-7.90852401904812,
28.8495658094393));
#47921=CARTESIAN_POINT('Ctrl Pts',(0.00816323896655843,-7.91368104157214,
28.8578473111737));
#47922=CARTESIAN_POINT('Ctrl Pts',(0.214303899246248,-7.9107757632299,28.866128812908));
#47923=CARTESIAN_POINT('Ctrl Pts',(0.419873743605476,-7.89984981119456,
28.8744103146424));
#47924=CARTESIAN_POINT('Ctrl Pts',(0.625785857325099,-7.88890566768456,
28.8827056048987));
#47925=CARTESIAN_POINT('Ctrl Pts',(0.831124961246783,-7.8699141674667,28.8910008951549));
#47926=CARTESIAN_POINT('Ctrl Pts',(1.03525887144275,-7.84296883004766,28.8992961854112));
#47927=CARTESIAN_POINT('Ctrl Pts',(1.23957791186844,-7.81599905574548,28.9075989987144));
#47928=CARTESIAN_POINT('Ctrl Pts',(1.44268928701813,-7.78106109062025,28.9159018120176));
#47929=CARTESIAN_POINT('Ctrl Pts',(1.6439714750191,-7.73829947658551,28.9242046253209));
#47930=CARTESIAN_POINT('Ctrl Pts',(1.84556233314544,-7.69547228678921,28.9325201711487));
#47931=CARTESIAN_POINT('Ctrl Pts',(2.04531811129274,-7.64479753368419,28.9408357169766));
#47932=CARTESIAN_POINT('Ctrl Pts',(2.24263107276241,-7.58646998751597,28.9491512628045));
#47933=CARTESIAN_POINT('Ctrl Pts',(2.32102460846675,-7.5632961294023,28.9524550753564));
#47934=CARTESIAN_POINT('Ctrl Pts',(2.39903274847824,-7.53891480491464,28.9557588879083));
#47935=CARTESIAN_POINT('Ctrl Pts',(2.47661825383057,-7.51334033734618,28.9590627004603));
#47936=CARTESIAN_POINT('Ctrl Pts',(2.66236678009493,-7.45211215252913,28.9669724035651));
#47937=CARTESIAN_POINT('Ctrl Pts',(2.84607876551478,-7.38391403888483,28.9748821066698));
#47938=CARTESIAN_POINT('Ctrl Pts',(3.0271940501256,-7.30889986132552,28.9827918097746));
#47939=CARTESIAN_POINT('Ctrl Pts',(3.2081255844522,-7.23396178930571,28.9906934881001));
#47940=CARTESIAN_POINT('Ctrl Pts',(3.38646534987413,-7.15222155880661,28.9985951664255));
#47941=CARTESIAN_POINT('Ctrl Pts',(3.56166825101636,-7.06388280407469,29.006496844751));
#47942=CARTESIAN_POINT('Ctrl Pts',(3.73672585699575,-6.97561730836798,29.0143919702418));
#47943=CARTESIAN_POINT('Ctrl Pts',(3.90865147509959,-6.88076434409402,29.0222870957326));
#47944=CARTESIAN_POINT('Ctrl Pts',(4.07691964949858,-6.77957573683873,29.0301822212234));
#47945=CARTESIAN_POINT('Ctrl Pts',(4.24507944322176,-6.67845230465102,29.0380722615041));
#47946=CARTESIAN_POINT('Ctrl Pts',(4.40958619258182,-6.57100153701387,29.0459623017847));
#47947=CARTESIAN_POINT('Ctrl Pts',(4.56993848670113,-6.45752144617173,29.0538523420653));
#47948=CARTESIAN_POINT('Ctrl Pts',(4.73021719035728,-6.34409343473693,29.0617387613705));
#47949=CARTESIAN_POINT('Ctrl Pts',(4.88634495736857,-6.22464181268815,29.0696251806757));
#47950=CARTESIAN_POINT('Ctrl Pts',(5.03784861781131,-6.09950836576332,29.0775115999808));
#47951=CARTESIAN_POINT('Ctrl Pts',(5.18931079779809,-5.9744091793469,29.0853958600493));
#47952=CARTESIAN_POINT('Ctrl Pts',(5.33615112921285,-5.84363148792599,29.0932801201177));
#47953=CARTESIAN_POINT('Ctrl Pts',(5.477928631778,-5.707558050966,29.1011643801862));
#47954=CARTESIAN_POINT('Ctrl Pts',(5.61972268679212,-5.5714687275037,29.1090495607379));
#47955=CARTESIAN_POINT('Ctrl Pts',(5.75645247847028,-5.43008265680269,29.1169347412895));
#47956=CARTESIAN_POINT('Ctrl Pts',(5.88771263608965,-5.28382067398491,29.1248199218412));
#47957=CARTESIAN_POINT('Ctrl Pts',(6.01898916572442,-5.13754044798137,29.1327060859076));
#47958=CARTESIAN_POINT('Ctrl Pts',(6.14479447103222,-4.98638335416747,29.140592249974));
#47959=CARTESIAN_POINT('Ctrl Pts',(6.26476238886679,-4.830804613213,29.1484784140404));
#47960=CARTESIAN_POINT('Ctrl Pts',(6.38476539877375,-4.67518036358808,29.1563668849055));
#47961=CARTESIAN_POINT('Ctrl Pts',(6.49892740802877,-4.51513216233616,29.1642553557706));
#47962=CARTESIAN_POINT('Ctrl Pts',(6.60692449258012,-4.3511457972981,29.1721438266358));
#47963=CARTESIAN_POINT('Ctrl Pts',(6.71497128802812,-4.18708394958124,29.1800359285522));
#47964=CARTESIAN_POINT('Ctrl Pts',(6.81684731459258,-4.01908061335109,29.1879280304687));
#47965=CARTESIAN_POINT('Ctrl Pts',(6.9122735380583,-3.8476480523898,29.1958201323852));
#47966=CARTESIAN_POINT('Ctrl Pts',(7.00781038930819,-3.6760167493672,29.2037213836289));
#47967=CARTESIAN_POINT('Ctrl Pts',(7.09688233433858,-3.50094858194217,29.2116226348727));
#47968=CARTESIAN_POINT('Ctrl Pts',(7.17925711742028,-3.32297882057204,29.2195238861164));
#47969=CARTESIAN_POINT('Ctrl Pts',(7.26168648444222,-3.14489113123344,29.2274303729603));
#47970=CARTESIAN_POINT('Ctrl Pts',(7.33740971002179,-2.96389833188598,29.2353368598041));
#47971=CARTESIAN_POINT('Ctrl Pts',(7.40624366716349,-2.78055313608653,29.243243346648));
#47972=CARTESIAN_POINT('Ctrl Pts',(7.4751724545044,-2.59695535185308,29.2511607259896));
#47973=CARTESIAN_POINT('Ctrl Pts',(7.53719290699625,-2.41099902363484,29.2590781053312));
#47974=CARTESIAN_POINT('Ctrl Pts',(7.59217215418576,-2.22325054395728,29.2669954846728));
#47975=CARTESIAN_POINT('Ctrl Pts',(7.6160105701153,-2.14184480310993,29.2704283760176));
#47976=CARTESIAN_POINT('Ctrl Pts',(7.63852589598784,-2.06010225280555,29.2738612673623));
#47977=CARTESIAN_POINT('Ctrl Pts',(7.65971031677736,-1.97806947882386,29.2772941587071));
#47978=CARTESIAN_POINT('Ctrl Pts',(7.70810110523076,-1.79068504894333,29.2851357853674));
#47979=CARTESIAN_POINT('Ctrl Pts',(7.74968780417034,-1.60122867415708,29.2929774120277));
#47980=CARTESIAN_POINT('Ctrl Pts',(7.78428804038756,-1.41024136383784,29.3008190386881));
#47981=CARTESIAN_POINT('Ctrl Pts',(7.81884753743351,-1.219478926687,29.3086514324238));
#47982=CARTESIAN_POINT('Ctrl Pts',(7.84643688910024,-1.02718948531261,29.3164838261596));
#47983=CARTESIAN_POINT('Ctrl Pts',(7.86692331808896,-0.833929557761398,
29.3243162198953));
#47984=CARTESIAN_POINT('Ctrl Pts',(7.88738961390277,-0.640859557694782,
29.3321409162938));
#47985=CARTESIAN_POINT('Ctrl Pts',(7.90076685114784,-0.446821317721075,
29.3399656126923));
#47986=CARTESIAN_POINT('Ctrl Pts',(7.90697314235659,-0.252382103271008,
29.3477903090908));
#47987=CARTESIAN_POINT('Ctrl Pts',(7.9131745417304,-0.0580961469445164,
29.355608838018));
#47988=CARTESIAN_POINT('Ctrl Pts',(7.91221624117949,0.136589804671775,29.3634273669451));
#47989=CARTESIAN_POINT('Ctrl Pts',(7.90406807064486,0.331102604357672,29.3712458958722));
#47990=CARTESIAN_POINT('Ctrl Pts',(7.89592473796643,0.525499914934816,29.379059782663));
#47991=CARTESIAN_POINT('Ctrl Pts',(7.88060005345888,0.71972392801215,29.3868736694538));
#47992=CARTESIAN_POINT('Ctrl Pts',(7.85811591774078,0.913200538408173,29.3946875562446));
#47993=CARTESIAN_POINT('Ctrl Pts',(7.83564076036415,1.10659988992728,29.4024983228023));
#47994=CARTESIAN_POINT('Ctrl Pts',(7.8060118882968,1.2992520845273,29.41030908936));
#47995=CARTESIAN_POINT('Ctrl Pts',(7.76930314839567,1.49058699455251,29.4181198559177));
#47996=CARTESIAN_POINT('Ctrl Pts',(7.73259586748839,1.68191429994578,29.4259303120354));
#47997=CARTESIAN_POINT('Ctrl Pts',(7.68880933669557,1.87192407799625,29.4337407681532));
#47998=CARTESIAN_POINT('Ctrl Pts',(7.63806881440613,2.06005480179451,29.4415512242709));
#47999=CARTESIAN_POINT('Ctrl Pts',(7.5873268927913,2.24819071387396,29.4493618957859));
#48000=CARTESIAN_POINT('Ctrl Pts',(7.52963068854188,2.43444712842404,29.4571725673009));
#48001=CARTESIAN_POINT('Ctrl Pts',(7.46515578756604,2.61827616331228,29.4649832388159));
#48002=CARTESIAN_POINT('Ctrl Pts',(7.40066775354943,2.80214264275912,29.4727955013046));
#48003=CARTESIAN_POINT('Ctrl Pts',(7.32939838869323,2.9835804254994,29.4806077637932));
#48004=CARTESIAN_POINT('Ctrl Pts',(7.25157207281655,3.16206000460887,29.4884200262818));
#48005=CARTESIAN_POINT('Ctrl Pts',(7.17371619699191,3.34060737373271,29.4962352560196));
#48006=CARTESIAN_POINT('Ctrl Pts',(7.08929854984644,3.51619397882489,29.5040504857575));
#48007=CARTESIAN_POINT('Ctrl Pts',(6.99859031562769,3.68831324510301,29.5118657154953));
#48008=CARTESIAN_POINT('Ctrl Pts',(6.90778343180112,3.86061969943813,29.5196894446748));
#48009=CARTESIAN_POINT('Ctrl Pts',(6.81067246089798,4.02945097199532,29.5275131738543));
#48010=CARTESIAN_POINT('Ctrl Pts',(6.70757348027875,4.19432700282908,29.5353369030338));
#48011=CARTESIAN_POINT('Ctrl Pts',(6.60441194707415,4.35930306784294,29.5431653790546));
#48012=CARTESIAN_POINT('Ctrl Pts',(6.49525536064069,4.52031881834257,29.5509938550753));
#48013=CARTESIAN_POINT('Ctrl Pts',(6.38046128827864,4.67692577969521,29.558822331096));
#48014=CARTESIAN_POINT('Ctrl Pts',(6.26550922710007,4.83374827611838,29.5666615812937));
#48015=CARTESIAN_POINT('Ctrl Pts',(6.14490440061826,4.98614958906298,29.5745008314915));
#48016=CARTESIAN_POINT('Ctrl Pts',(6.01904331686938,5.13371586179544,29.5823400816893));
#48017=CARTESIAN_POINT('Ctrl Pts',(5.94847764981573,5.21645082767864,29.5867352601108));
#48018=CARTESIAN_POINT('Ctrl Pts',(5.87626036670645,5.29766660895056,29.5911304385324));
#48019=CARTESIAN_POINT('Ctrl Pts',(5.80246602453022,5.37729569897104,29.5955256169539));
#48020=CARTESIAN_POINT('Ctrl Pts',(5.66966033730927,5.52060202451148,29.6034355010117));
#48021=CARTESIAN_POINT('Ctrl Pts',(5.53136325581621,5.65917893213775,29.6113453850695));
#48022=CARTESIAN_POINT('Ctrl Pts',(5.38794440026323,5.79257940296654,29.6192552691272));
#48023=CARTESIAN_POINT('Ctrl Pts',(5.24468146505712,5.92583484511269,29.6271565538146));
#48024=CARTESIAN_POINT('Ctrl Pts',(5.09630809708073,6.05392482701331,29.6350578385019));
#48025=CARTESIAN_POINT('Ctrl Pts',(4.94323315358624,6.1764364312511,29.6429591231892));
#48026=CARTESIAN_POINT('Ctrl Pts',(4.79029618321246,6.29883761043843,29.6508532861042));
#48027=CARTESIAN_POINT('Ctrl Pts',(4.63266634681972,6.41567021398392,29.6587474490191));
#48028=CARTESIAN_POINT('Ctrl Pts',(4.47078842503838,6.5265589600143,29.666641611934));
#48029=CARTESIAN_POINT('Ctrl Pts',(4.30902633946936,6.63736835654359,29.674530125963));
#48030=CARTESIAN_POINT('Ctrl Pts',(4.14302250828464,6.74224217535166,29.6824186399919));
#48031=CARTESIAN_POINT('Ctrl Pts',(3.97325400095765,6.84084597428374,29.6903071540208));
#48032=CARTESIAN_POINT('Ctrl Pts',(3.80357544603444,6.93939752766759,29.6981914882945));
#48033=CARTESIAN_POINT('Ctrl Pts',(3.63013648728671,7.0316855081978,29.7060758225682));
#48034=CARTESIAN_POINT('Ctrl Pts',(3.45344256066231,7.11741915867024,29.7139601568419));
#48035=CARTESIAN_POINT('Ctrl Pts',(3.27680944490404,7.20312330310565,29.7218417776483));
#48036=CARTESIAN_POINT('Ctrl Pts',(3.09692390389205,7.28227746279696,29.7297233984547));
#48037=CARTESIAN_POINT('Ctrl Pts',(2.91431556546067,7.35463702604783,29.7376050192611));
#48038=CARTESIAN_POINT('Ctrl Pts',(2.73170483534119,7.42699753701832,29.745486743296));
#48039=CARTESIAN_POINT('Ctrl Pts',(2.54637155407258,7.49256313870811,29.7533684673308));
#48040=CARTESIAN_POINT('Ctrl Pts',(2.35886543682323,7.5511373216861,29.7612501913657));
#48041=CARTESIAN_POINT('Ctrl Pts',(2.1713480241709,7.60971503318365,29.7691323901971));
#48042=CARTESIAN_POINT('Ctrl Pts',(1.98165784401353,7.66130038323983,29.7770145890284));
#48043=CARTESIAN_POINT('Ctrl Pts',(1.79035991680783,7.70574671062369,29.7848967878598));
#48044=CARTESIAN_POINT('Ctrl Pts',(1.59901827601724,7.75020319446003,29.7927807878563));
#48045=CARTESIAN_POINT('Ctrl Pts',(1.40606849224416,7.78751732682527,29.8006647878529));
#48046=CARTESIAN_POINT('Ctrl Pts',(1.21208616243327,7.81759350022996,29.8085487878495));
#48047=CARTESIAN_POINT('Ctrl Pts',(1.01802686373275,7.8476816073488,29.8164359160831));
#48048=CARTESIAN_POINT('Ctrl Pts',(0.822934543366754,7.87052598017935,29.8243230443168));
#48049=CARTESIAN_POINT('Ctrl Pts',(0.627390552475897,7.88608281053807,29.8322101725505));
#48050=CARTESIAN_POINT('Ctrl Pts',(0.431637938485425,7.90165623825759,29.840105715449));
#48051=CARTESIAN_POINT('Ctrl Pts',(0.235433035532845,7.90992656620909,29.8480012583475));
#48052=CARTESIAN_POINT('Ctrl Pts',(0.0393589541391628,7.91090208969426,
29.855896801246));
#48053=CARTESIAN_POINT('Ctrl Pts',(-0.156834529575379,7.91187820723944,
29.8637971522565));
#48054=CARTESIAN_POINT('Ctrl Pts',(-0.352896688958301,7.90555067515392,
29.871697503267));
#48055=CARTESIAN_POINT('Ctrl Pts',(-0.548248629333389,7.89197975418298,
29.8795978542775));
#48056=CARTESIAN_POINT('Ctrl Pts',(-0.743854926148637,7.87839116330233,
29.8875084918772));
#48057=CARTESIAN_POINT('Ctrl Pts',(-0.938748814827542,7.85754038185277,
29.8954191294769));
#48058=CARTESIAN_POINT('Ctrl Pts',(-1.13235955610086,7.82953912026162,29.9033297670766));
#48059=CARTESIAN_POINT('Ctrl Pts',(-1.21742808270823,7.81723594921315,29.9068055364513));
#48060=CARTESIAN_POINT('Ctrl Pts',(-1.30224905815058,7.80355300658742,29.910281305826));
#48061=CARTESIAN_POINT('Ctrl Pts',(-1.38677495964398,7.78850282219275,29.9137570752007));
#48062=CARTESIAN_POINT('Ctrl Pts',(-1.57913194171663,7.75425287041884,29.9216669406442));
#48063=CARTESIAN_POINT('Ctrl Pts',(-1.77047892991408,7.71282634107011,29.9295768060876));
#48064=CARTESIAN_POINT('Ctrl Pts',(-1.96024003766932,7.664292530607,29.9374866715311));
#48065=CARTESIAN_POINT('Ctrl Pts',(-2.1497949144898,7.61581146632153,29.9453879405926));
#48066=CARTESIAN_POINT('Ctrl Pts',(-2.33776701266895,7.56023859084218,29.9532892096542));
#48067=CARTESIAN_POINT('Ctrl Pts',(-2.52358792335832,7.49769464522796,29.9611904787158));
#48068=CARTESIAN_POINT('Ctrl Pts',(-2.70924141526446,7.43520704973728,29.969084628983));
#48069=CARTESIAN_POINT('Ctrl Pts',(-2.89274725574595,7.36576100509929,29.9769787792503));
#48070=CARTESIAN_POINT('Ctrl Pts',(-3.07354927817775,7.28952781972969,29.9848729295175));
#48071=CARTESIAN_POINT('Ctrl Pts',(-3.25422199054022,7.21334915652943,29.9927614338682));
#48072=CARTESIAN_POINT('Ctrl Pts',(-3.43219442100778,7.13039315718868,30.000649938219));
#48073=CARTESIAN_POINT('Ctrl Pts',(-3.60692730560232,7.04088037194926,30.0085384425697));
#48074=CARTESIAN_POINT('Ctrl Pts',(-3.78156767291515,6.95141498179285,30.0164227701281));
#48075=CARTESIAN_POINT('Ctrl Pts',(-3.95297160594728,6.85539988037804,30.0243070976864));
#48076=CARTESIAN_POINT('Ctrl Pts',(-4.1206212574183,6.75310309805147,30.0321914252448));
#48077=CARTESIAN_POINT('Ctrl Pts',(-4.28821327354627,6.65084148376785,30.040073042294));
#48078=CARTESIAN_POINT('Ctrl Pts',(-4.45205328631158,6.5423026720551,30.0479546593431));
#48079=CARTESIAN_POINT('Ctrl Pts',(-4.61164919190898,6.42779999150295,30.0558362763923));
#48080=CARTESIAN_POINT('Ctrl Pts',(-4.77124727740716,6.3132957469728,30.0637180010955));
#48081=CARTESIAN_POINT('Ctrl Pts',(-4.92660085465792,6.19282766497068,30.0715997257987));
#48082=CARTESIAN_POINT('Ctrl Pts',(-5.07724742815115,6.06675197723893,30.0794814505019));
#48083=CARTESIAN_POINT('Ctrl Pts',(-5.22790312932432,5.94066865057788,30.087363652759));
#48084=CARTESIAN_POINT('Ctrl Pts',(-5.37385099334685,5.80897726222848,30.0952458550161));
#48085=CARTESIAN_POINT('Ctrl Pts',(-5.51466218728181,5.6720738676576,30.1031280572732));
#48086=CARTESIAN_POINT('Ctrl Pts',(-5.65550560731773,5.53513914132613,30.111012063454));
#48087=CARTESIAN_POINT('Ctrl Pts',(-5.79120976731282,5.39299027245297,30.1188960696348));
#48088=CARTESIAN_POINT('Ctrl Pts',(-5.9213830674542,5.24605981365697,30.1267800758155));
#48089=CARTESIAN_POINT('Ctrl Pts',(-6.05160806369479,5.0990710039429,30.1346672129945));
#48090=CARTESIAN_POINT('Ctrl Pts',(-6.17629759474949,4.94729707861559,30.1425543501735));
#48091=CARTESIAN_POINT('Ctrl Pts',(-6.29510052804808,4.79120343356122,30.1504414873524));
#48092=CARTESIAN_POINT('Ctrl Pts',(-6.41403027258995,4.63494317284637,30.1583370433275));
#48093=CARTESIAN_POINT('Ctrl Pts',(-6.52706065970622,4.47435425713783,30.1662325993025));
#48094=CARTESIAN_POINT('Ctrl Pts',(-6.63388343936781,4.30993172949195,30.1741281552776));
#48095=CARTESIAN_POINT('Ctrl Pts',(-6.74077130244694,4.14540902489829,30.1820285217413));
#48096=CARTESIAN_POINT('Ctrl Pts',(-6.84144384140127,3.97704834722757,30.189928888205));
#48097=CARTESIAN_POINT('Ctrl Pts',(-6.93563880299297,3.80536928489447,30.1978292546686));
#48098=CARTESIAN_POINT('Ctrl Pts',(-7.02995645221743,3.63346661296065,30.2057399112502));
#48099=CARTESIAN_POINT('Ctrl Pts',(-7.11777951762511,3.4582372306317,30.2136505678318));
#48100=CARTESIAN_POINT('Ctrl Pts',(-7.19889343844244,3.28022167878185,30.2215612244134));
#48101=CARTESIAN_POINT('Ctrl Pts',(-7.2345331231562,3.2020055343994,30.2250369940914));
#48102=CARTESIAN_POINT('Ctrl Pts',(-7.26887822907425,3.1232517273169,30.2285127637695));
#48103=CARTESIAN_POINT('Ctrl Pts',(-7.301913606672,3.04400701061911,30.2319885334476));
#48104=CARTESIAN_POINT('Ctrl Pts',(-7.38494034361703,2.84484384900301,30.2407240720043));
#48105=CARTESIAN_POINT('Ctrl Pts',(-7.45989208854214,2.642096526646,30.2494596105611));
#48106=CARTESIAN_POINT('Ctrl Pts',(-7.52647707587245,2.43640387176807,30.2581951491179));
#48107=CARTESIAN_POINT('Ctrl Pts',(-7.59279172313769,2.23154634456583,30.2668952207299));
#48108=CARTESIAN_POINT('Ctrl Pts',(-7.65080730516922,2.02376754660903,30.275595292342));
#48109=CARTESIAN_POINT('Ctrl Pts',(-7.70028122495755,1.81372270663579,30.2842953639541));
#48110=CARTESIAN_POINT('Ctrl Pts',(-7.74963017704213,1.60420842541853,30.2929734597863));
#48111=CARTESIAN_POINT('Ctrl Pts',(-7.79048045122216,1.39243973004719,30.3016515556185));
#48112=CARTESIAN_POINT('Ctrl Pts',(-7.82263844849393,1.17908808158871,30.3103296514507));
#48113=CARTESIAN_POINT('Ctrl Pts',(-7.85465833584681,0.966652720877075,
30.3189704772035));
#48114=CARTESIAN_POINT('Ctrl Pts',(-7.87806035896862,0.752648180903682,
30.3276113029563));
#48115=CARTESIAN_POINT('Ctrl Pts',(-7.89270170464743,0.537755336054983,
30.3362521287091));
#48116=CARTESIAN_POINT('Ctrl Pts',(-7.90479793956879,0.360217397177362,
30.3433909163939));
#48117=CARTESIAN_POINT('Ctrl Pts',(-7.91091536010079,0.182073519787902,
30.3505297040786));
#48118=CARTESIAN_POINT('Ctrl Pts',(-7.910999127499,0.00371546903165411,
30.3576684917634));
#48119=CARTESIAN_POINT('',(-7.91099855363492,-0.00392369634145859,32.3576684917634));
#48120=CARTESIAN_POINT('Ctrl Pts',(-7.911,-8.98392471526677E-12,30.3576684917634));
#48121=CARTESIAN_POINT('Ctrl Pts',(-7.9109999999975,-2.20167589667574,30.4462559274961));
#48122=CARTESIAN_POINT('Ctrl Pts',(-6.94214576671874,-4.3861041833947,30.5348433632288));
#48123=CARTESIAN_POINT('Ctrl Pts',(-3.67820201487455,-7.34180684108048,
30.7120182346943));
#48124=CARTESIAN_POINT('Ctrl Pts',(-1.40868175870829,-8.08992666571496,
30.800605670427));
#48125=CARTESIAN_POINT('Ctrl Pts',(2.97309270522138,-7.65454228024921,30.9777805418925));
#48126=CARTESIAN_POINT('Ctrl Pts',(5.05102072676332,-6.47444880833656,31.0663679776252));
#48127=CARTESIAN_POINT('Ctrl Pts',(7.66951518848202,-2.93425195366844,31.2435428490907));
#48128=CARTESIAN_POINT('Ctrl Pts',(8.18956872247139,-0.601881960089965,
31.3321302848234));
#48129=CARTESIAN_POINT('Ctrl Pts',(7.32306689760926,3.71537198233271,31.5093051562888));
#48130=CARTESIAN_POINT('Ctrl Pts',(5.94329958849567,5.66643518937176,31.5978925920216));
#48131=CARTESIAN_POINT('Ctrl Pts',(2.16154501636962,7.92205913233239,31.775067463487));
#48132=CARTESIAN_POINT('Ctrl Pts',(-0.210816529309534,8.20894963712979,
31.8636548992197));
#48133=CARTESIAN_POINT('Ctrl Pts',(-4.42123908577208,6.91982244717338,32.0408297706852));
#48134=CARTESIAN_POINT('Ctrl Pts',(-6.22631625634784,5.35390358802828,32.1294172064179));
#48135=CARTESIAN_POINT('Ctrl Pts',(-7.65317280859749,2.31334857513661,32.2645592586882));
#48136=CARTESIAN_POINT('Ctrl Pts',(-7.91100000000132,1.15702837835623,32.3111138752258));
#48137=CARTESIAN_POINT('Ctrl Pts',(-7.911,-9.0383256434734E-12,32.3576684917634));
#48138=CARTESIAN_POINT('',(-7.91722079586035,-0.00170382440757721,34.3576684917634));
#48139=CARTESIAN_POINT('Ctrl Pts',(-7.91099785005971,-0.00583235378789637,
32.3576684917634));
#48140=CARTESIAN_POINT('Ctrl Pts',(-7.91082541404672,-0.239724359934149,
32.3670578153675));
#48141=CARTESIAN_POINT('Ctrl Pts',(-7.90027652667228,-0.473177135982916,
32.3764471389717));
#48142=CARTESIAN_POINT('Ctrl Pts',(-7.87949087824595,-0.705368343235573,
32.3858364625758));
#48143=CARTESIAN_POINT('Ctrl Pts',(-7.85856304809976,-0.939147826422932,
32.395290012715));
#48144=CARTESIAN_POINT('Ctrl Pts',(-7.82725802231293,-1.17164840009605,
32.4047435628543));
#48145=CARTESIAN_POINT('Ctrl Pts',(-7.78576728881217,-1.40205161262427,
32.4141971129935));
#48146=CARTESIAN_POINT('Ctrl Pts',(-7.74394622875813,-1.63428916965886,
32.4237259271344));
#48147=CARTESIAN_POINT('Ctrl Pts',(-7.69177667750553,-1.86439581611647,
32.4332547412752));
#48148=CARTESIAN_POINT('Ctrl Pts',(-7.62950321232089,-2.0915548601902,32.4427835554161));
#48149=CARTESIAN_POINT('Ctrl Pts',(-7.5928507809301,-2.22525436210524,32.4483919506691));
#48150=CARTESIAN_POINT('Ctrl Pts',(-7.55269908749128,-2.35793316962834,
32.4540003459222));
#48151=CARTESIAN_POINT('Ctrl Pts',(-7.5091056755644,-2.48942823821185,32.4596087411753));
#48152=CARTESIAN_POINT('Ctrl Pts',(-7.44817536530196,-2.67321828750213,
32.4674475692857));
#48153=CARTESIAN_POINT('Ctrl Pts',(-7.38040138015807,-2.8550476425854,32.4752863973962));
#48154=CARTESIAN_POINT('Ctrl Pts',(-7.30592644173637,-3.03436316678432,
32.4831252255067));
#48155=CARTESIAN_POINT('Ctrl Pts',(-7.23153498856715,-3.2134776810579,32.4909552664122));
#48156=CARTESIAN_POINT('Ctrl Pts',(-7.15045767286685,-3.39008365418208,
32.4987853073178));
#48157=CARTESIAN_POINT('Ctrl Pts',(-7.06288723091396,-3.56364209249365,
32.5066153482233));
#48158=CARTESIAN_POINT('Ctrl Pts',(-6.97539791045116,-3.73703975373455,
32.5144381357158));
#48159=CARTESIAN_POINT('Ctrl Pts',(-6.88142759951014,-3.90739519048686,
32.5222609232083));
#48160=CARTESIAN_POINT('Ctrl Pts',(-6.78121752641135,-4.07418824546578,
32.5300837107009));
#48161=CARTESIAN_POINT('Ctrl Pts',(-6.6810807904657,-4.24085923559197,32.5379007732104));
#48162=CARTESIAN_POINT('Ctrl Pts',(-6.5747135677808,-4.40397273637294,32.5457178357199));
#48163=CARTESIAN_POINT('Ctrl Pts',(-6.46240360873286,-4.56303195231379,
32.5535348982294));
#48164=CARTESIAN_POINT('Ctrl Pts',(-6.35015400311001,-4.72200569258928,
32.561347759985));
#48165=CARTESIAN_POINT('Ctrl Pts',(-6.23196822504431,-4.87692920145537,
32.5691606217407));
#48166=CARTESIAN_POINT('Ctrl Pts',(-6.10817814816965,-5.02733335976667,
32.5769734834963));
#48167=CARTESIAN_POINT('Ctrl Pts',(-5.98443052870422,-5.17768593259502,
32.5847836656036));
#48168=CARTESIAN_POINT('Ctrl Pts',(-5.85508266347596,-5.32352197197867,
32.592593847711));
#48169=CARTESIAN_POINT('Ctrl Pts',(-5.72050774440121,-5.46440409800061,
32.6004040298183));
#48170=CARTESIAN_POINT('Ctrl Pts',(-5.58592675591156,-5.6052925778965,32.6082145641698));
#48171=CARTESIAN_POINT('Ctrl Pts',(-5.44611847888516,-5.74122643729883,
32.6160250985214));
#48172=CARTESIAN_POINT('Ctrl Pts',(-5.30149448147925,-5.87180357836032,
32.6238356328729));
#48173=CARTESIAN_POINT('Ctrl Pts',(-5.15685889232388,-6.00239118530252,
32.6316467932461));
#48174=CARTESIAN_POINT('Ctrl Pts',(-5.00740707463034,-6.12762098210182,
32.6394579536193));
#48175=CARTESIAN_POINT('Ctrl Pts',(-4.85358526859605,-6.24712982420466,
32.6472691139925));
#48176=CARTESIAN_POINT('Ctrl Pts',(-4.69972404254289,-6.36666929291978,
32.6550822761371));
#48177=CARTESIAN_POINT('Ctrl Pts',(-4.54149087503321,-6.48048467031655,
32.6628954382817));
#48178=CARTESIAN_POINT('Ctrl Pts',(-4.37936280483853,-6.58825488453481,
32.6707086004263));
#48179=CARTESIAN_POINT('Ctrl Pts',(-4.21716462949364,-6.69607169924025,
32.6785251410291));
#48180=CARTESIAN_POINT('Ctrl Pts',(-4.05106848925646,-6.7978379490441,32.6863416816319));
#48181=CARTESIAN_POINT('Ctrl Pts',(-3.88157806155302,-6.89327735928784,
32.6941582222347));
#48182=CARTESIAN_POINT('Ctrl Pts',(-3.71188983543504,-6.98882814906071,
32.7019838848826));
#48183=CARTESIAN_POINT('Ctrl Pts',(-3.53879971682521,-7.07803717952283,
32.7098095475306));
#48184=CARTESIAN_POINT('Ctrl Pts',(-3.36283450243718,-7.16067490598603,
32.7176352101785));
#48185=CARTESIAN_POINT('Ctrl Pts',(-3.18675458827304,-7.24336649837244,
32.7254659738446));
#48186=CARTESIAN_POINT('Ctrl Pts',(-3.00779616625427,-7.31947811357063,
32.7332967375108));
#48187=CARTESIAN_POINT('Ctrl Pts',(-2.82650347640145,-7.38882934556554,
32.7411275011769));
#48188=CARTESIAN_POINT('Ctrl Pts',(-2.64494883766978,-7.4582807828003,32.7489695794733));
#48189=CARTESIAN_POINT('Ctrl Pts',(-2.46105352628233,-7.52095221383441,
32.7568116577697));
#48190=CARTESIAN_POINT('Ctrl Pts',(-2.2753754692137,-7.5767135008591,32.7646537360662));
#48191=CARTESIAN_POINT('Ctrl Pts',(-2.1713028495594,-7.60796772285804,32.7690492238515));
#48192=CARTESIAN_POINT('Ctrl Pts',(-2.06667033537943,-7.63705197311932,
32.7734447116368));
#48193=CARTESIAN_POINT('Ctrl Pts',(-1.9615771006619,-7.66395043552337,32.7778401994221));
#48194=CARTESIAN_POINT('Ctrl Pts',(-1.7722981957133,-7.7123960992459,32.7857567234205));
#48195=CARTESIAN_POINT('Ctrl Pts',(-1.58095632328446,-7.75389396916855,
32.793673247419));
#48196=CARTESIAN_POINT('Ctrl Pts',(-1.38810369409898,-7.78826611861901,
32.8015897714174));
#48197=CARTESIAN_POINT('Ctrl Pts',(-1.1954732428881,-7.82259866925984,32.8094971750981));
#48198=CARTESIAN_POINT('Ctrl Pts',(-1.00133583748493,-7.8498217908875,32.8174045787787));
#48199=CARTESIAN_POINT('Ctrl Pts',(-0.806258457722267,-7.86980738642003,
32.8253119824594));
#48200=CARTESIAN_POINT('Ctrl Pts',(-0.611369670154704,-7.88977366076148,
32.8332117416114));
#48201=CARTESIAN_POINT('Ctrl Pts',(-0.415543058806255,-7.90251631235472,
32.8411115007634));
#48202=CARTESIAN_POINT('Ctrl Pts',(-0.219355684610209,-7.90795827528378,
32.8490112599154));
#48203=CARTESIAN_POINT('Ctrl Pts',(-0.0233216339860801,-7.91339598523174,
32.8569048452792));
#48204=CARTESIAN_POINT('Ctrl Pts',(0.173072274956343,-7.91154436430064,
32.8647984306431));
#48205=CARTESIAN_POINT('Ctrl Pts',(0.369243681633338,-7.9023781296249,32.8726920160069));
#48206=CARTESIAN_POINT('Ctrl Pts',(0.565298106723887,-7.89321736098874,
32.8805808942416));
#48207=CARTESIAN_POINT('Ctrl Pts',(0.761129950722925,-7.87675068606911,
32.8884697724763));
#48208=CARTESIAN_POINT('Ctrl Pts',(0.956156384946896,-7.85300490051581,
32.8963586507111));
#48209=CARTESIAN_POINT('Ctrl Pts',(1.15110263112005,-7.82926887839927,32.9042442853149));
#48210=CARTESIAN_POINT('Ctrl Pts',(1.34524378597666,-7.79825975198306,32.9121299199187));
#48211=CARTESIAN_POINT('Ctrl Pts',(1.53800139065524,-7.76005623190596,32.9200155545225));
#48212=CARTESIAN_POINT('Ctrl Pts',(1.73074184827965,-7.72185611028274,32.9279004876474));
#48213=CARTESIAN_POINT('Ctrl Pts',(1.92209866181779,-7.67646293069589,32.9357854207723));
#48214=CARTESIAN_POINT('Ctrl Pts',(2.11150230940953,-7.62400675480802,32.9436703538971));
#48215=CARTESIAN_POINT('Ctrl Pts',(2.30090530032556,-7.57155076078938,32.9515552596844));
#48216=CARTESIAN_POINT('Ctrl Pts',(2.48835480642252,-7.51203191072139,32.9594401654716));
#48217=CARTESIAN_POINT('Ctrl Pts',(2.6732951422396,-7.44563053625938,32.9673250712589));
#48218=CARTESIAN_POINT('Ctrl Pts',(2.85826586544687,-7.37921825144368,32.9752112726084));
#48219=CARTESIAN_POINT('Ctrl Pts',(3.04072627246391,-7.30592130542255,32.9830974739578));
#48220=CARTESIAN_POINT('Ctrl Pts',(3.2201391468173,-7.22596878453919,32.9909836753073));
#48221=CARTESIAN_POINT('Ctrl Pts',(3.39961160169132,-7.14598971253548,32.9988724955545));
#48222=CARTESIAN_POINT('Ctrl Pts',(3.57603419278762,-7.0593508020727,33.0067613158018));
#48223=CARTESIAN_POINT('Ctrl Pts',(3.7488926380972,-6.9663279414639,33.014650136049));
#48224=CARTESIAN_POINT('Ctrl Pts',(3.92191839442842,-6.87321504331127,33.0225465919462));
#48225=CARTESIAN_POINT('Ctrl Pts',(4.09137281065589,-6.77370601614417,33.0304430478434));
#48226=CARTESIAN_POINT('Ctrl Pts',(4.25676811904696,-6.6681216381126,33.0383395037406));
#48227=CARTESIAN_POINT('Ctrl Pts',(4.42225484159113,-6.56247890348921,33.0462403240168));
#48228=CARTESIAN_POINT('Ctrl Pts',(4.58367770042664,-6.45075431881464,33.0541411442931));
#48229=CARTESIAN_POINT('Ctrl Pts',(4.74058034280286,-6.33331027294819,33.0620419645694));
#48230=CARTESIAN_POINT('Ctrl Pts',(4.89767364313631,-6.21572351666251,33.0699523854122));
#48231=CARTESIAN_POINT('Ctrl Pts',(5.0502354880613,-6.09240363288114,33.077862806255));
#48232=CARTESIAN_POINT('Ctrl Pts',(5.1978440257412,-5.96375204750051,33.0857732270978));
#48233=CARTESIAN_POINT('Ctrl Pts',(5.26190030067285,-5.90792234108201,33.0892060372882));
#48234=CARTESIAN_POINT('Ctrl Pts',(5.32502424256473,-5.85108901776739,33.0926388474785));
#48235=CARTESIAN_POINT('Ctrl Pts',(5.38718366354049,-5.79328690600444,33.0960716576689));
#48236=CARTESIAN_POINT('Ctrl Pts',(5.53774013787773,-5.65328428018089,33.1043862750063));
#48237=CARTESIAN_POINT('Ctrl Pts',(5.68296554276837,-5.5072890821744,33.1127008923437));
#48238=CARTESIAN_POINT('Ctrl Pts',(5.82238320800562,-5.35572355327776,33.1210155096811));
#48239=CARTESIAN_POINT('Ctrl Pts',(5.9616285599979,-5.20434535177658,33.1293198505683));
#48240=CARTESIAN_POINT('Ctrl Pts',(6.09508029100375,-5.04741076523861,33.1376241914556));
#48241=CARTESIAN_POINT('Ctrl Pts',(6.22229735421852,-4.88537988652727,33.1459285323428));
#48242=CARTESIAN_POINT('Ctrl Pts',(6.34936559297583,-4.72353855909943,33.1542231584245));
#48243=CARTESIAN_POINT('Ctrl Pts',(6.47021353080071,-4.55661306047075,33.1625177845062));
#48244=CARTESIAN_POINT('Ctrl Pts',(6.58443876735422,-4.3850983020866,33.1708124105879));
#48245=CARTESIAN_POINT('Ctrl Pts',(6.69849201555532,-4.21384179259385,33.1790945474937));
#48246=CARTESIAN_POINT('Ctrl Pts',(6.8059423005254,-4.03801005667824,33.1873766843994));
#48247=CARTESIAN_POINT('Ctrl Pts',(6.90642905759138,-3.85812890822189,33.1956588213052));
#48248=CARTESIAN_POINT('Ctrl Pts',(7.00682314625146,-3.67841364529878,33.203933320464));
#48249=CARTESIAN_POINT('Ctrl Pts',(7.10026637039486,-3.49465667183419,33.2122078196228));
#48250=CARTESIAN_POINT('Ctrl Pts',(7.18644187709675,-3.30741200141593,33.2204823187816));
#48251=CARTESIAN_POINT('Ctrl Pts',(7.27251826832934,-3.12038269199865,33.228747300957));
#48252=CARTESIAN_POINT('Ctrl Pts',(7.35134349972627,-2.92987395591469,33.2370122831324));
#48253=CARTESIAN_POINT('Ctrl Pts',(7.4226468798375,-2.73646383079307,33.2452772653078));
#48254=CARTESIAN_POINT('Ctrl Pts',(7.45114563696957,-2.65916106935138,33.248580639136));
#48255=CARTESIAN_POINT('Ctrl Pts',(7.47844332087114,-2.58139509025245,33.2518840129641));
#48256=CARTESIAN_POINT('Ctrl Pts',(7.50452474429773,-2.50320381955268,33.2551873867923));
#48257=CARTESIAN_POINT('Ctrl Pts',(7.56978874149768,-2.30754444971906,33.2634534762899));
#48258=CARTESIAN_POINT('Ctrl Pts',(7.62735976619017,-2.10944218308649,33.2717195657876));
#48259=CARTESIAN_POINT('Ctrl Pts',(7.67708674047127,-1.90951831079991,33.2799856552852));
#48260=CARTESIAN_POINT('Ctrl Pts',(7.72685843428924,-1.70941464669802,33.2882591784886));
#48261=CARTESIAN_POINT('Ctrl Pts',(7.76877192402986,-1.50748639153828,33.296532701692));
#48262=CARTESIAN_POINT('Ctrl Pts',(7.80272734130214,-1.30436461056564,33.3048062248954));
#48263=CARTESIAN_POINT('Ctrl Pts',(7.83671550331287,-1.10104695010966,33.3130877266299));
#48264=CARTESIAN_POINT('Ctrl Pts',(7.8627302231974,-0.896533755392057,33.3213692283644));
#48265=CARTESIAN_POINT('Ctrl Pts',(7.88072343325758,-0.691461617521098,
33.3296507300989));
#48266=CARTESIAN_POINT('Ctrl Pts',(7.89874660162455,-0.486048038962156,
33.3379460203553));
#48267=CARTESIAN_POINT('Ctrl Pts',(7.90872153303988,-0.280073949757042,
33.3462413106116));
#48268=CARTESIAN_POINT('Ctrl Pts',(7.91065222120185,-0.0741784011299107,
33.354536600868));
#48269=CARTESIAN_POINT('Ctrl Pts',(7.91258466031614,0.131903875366846,33.3628394141713));
#48270=CARTESIAN_POINT('Ctrl Pts',(7.9064582978321,0.33790717583952,33.3711422274745));
#48271=CARTESIAN_POINT('Ctrl Pts',(7.89232914057703,0.54319585491661,33.3794450407778));
#48272=CARTESIAN_POINT('Ctrl Pts',(7.87817831598618,0.748799348151595,33.3877605866058));
#48273=CARTESIAN_POINT('Ctrl Pts',(7.85600019236455,0.953685737009395,33.3960761324338));
#48274=CARTESIAN_POINT('Ctrl Pts',(7.82590244114712,1.15722598555663,33.4043916782618));
#48275=CARTESIAN_POINT('Ctrl Pts',(7.81394443739188,1.23809365699453,33.4076954908131));
#48276=CARTESIAN_POINT('Ctrl Pts',(7.80073687067036,1.31874896723893,33.4109993033644));
#48277=CARTESIAN_POINT('Ctrl Pts',(7.78628870373272,1.39915303742095,33.4143031159157));
#48278=CARTESIAN_POINT('Ctrl Pts',(7.75169814839391,1.59164952857453,33.4222128190205));
#48279=CARTESIAN_POINT('Ctrl Pts',(7.70992103064171,1.78310643945418,33.4301225221252));
#48280=CARTESIAN_POINT('Ctrl Pts',(7.66103118836468,1.97294757429174,33.43803222523));
#48281=CARTESIAN_POINT('Ctrl Pts',(7.61219094721578,2.1625961060442,33.4459339035554));
#48282=CARTESIAN_POINT('Ctrl Pts',(7.55625244095167,2.3506317960854,33.4538355818808));
#48283=CARTESIAN_POINT('Ctrl Pts',(7.49334089691572,2.53648638920267,33.4617372602062));
#48284=CARTESIAN_POINT('Ctrl Pts',(7.43048152520646,2.72218685374625,33.469632385697));
#48285=CARTESIAN_POINT('Ctrl Pts',(7.36066074571401,2.9057095001494,33.4775275111878));
#48286=CARTESIAN_POINT('Ctrl Pts',(7.28405425401273,3.08649876471692,33.4854226366786));
#48287=CARTESIAN_POINT('Ctrl Pts',(7.20749710416343,3.26717158383793,33.4933126769592));
#48288=CARTESIAN_POINT('Ctrl Pts',(7.12416308422304,3.44511421271346,33.5012027172398));
#48289=CARTESIAN_POINT('Ctrl Pts',(7.03427699053538,3.6197884220524,33.5090927575204));
#48290=CARTESIAN_POINT('Ctrl Pts',(6.94443214826451,3.79438246817234,33.5169791768256));
#48291=CARTESIAN_POINT('Ctrl Pts',(6.8480413815963,3.96571077798305,33.5248655961307));
#48292=CARTESIAN_POINT('Ctrl Pts',(6.74537678638158,4.13325694939771,33.5327520154358));
#48293=CARTESIAN_POINT('Ctrl Pts',(6.64274029988734,4.30075724805079,33.5406362755043));
#48294=CARTESIAN_POINT('Ctrl Pts',(6.53383358841617,4.46447717872594,33.5485205355728));
#48295=CARTESIAN_POINT('Ctrl Pts',(6.41897382861698,4.62392646865522,33.5564047956413));
#48296=CARTESIAN_POINT('Ctrl Pts',(6.30410065900207,4.78339437420407,33.5642899761929));
#48297=CARTESIAN_POINT('Ctrl Pts',(6.18327324819839,4.9385903590711,33.5721751567445));
#48298=CARTESIAN_POINT('Ctrl Pts',(6.05685146349842,5.08905407213531,33.5800603372962));
#48299=CARTESIAN_POINT('Ctrl Pts',(5.93041391027072,5.2395365524653,33.5879465013626));
#48300=CARTESIAN_POINT('Ctrl Pts',(5.79838081400447,5.38528532036431,33.595832665429));
#48301=CARTESIAN_POINT('Ctrl Pts',(5.66115158322437,5.52587402604839,33.6037188294953));
#48302=CARTESIAN_POINT('Ctrl Pts',(5.52388221122846,5.66650385563546,33.6116073003605));
#48303=CARTESIAN_POINT('Ctrl Pts',(5.38141391657862,5.80197036847344,33.6194957712256));
#48304=CARTESIAN_POINT('Ctrl Pts',(5.23418229322077,5.93188475287022,33.6273842420907));
#48305=CARTESIAN_POINT('Ctrl Pts',(5.08688289936547,6.06185893666509,33.6352763440072));
#48306=CARTESIAN_POINT('Ctrl Pts',(4.9348160658088,6.186275671494,33.6431684459237));
#48307=CARTESIAN_POINT('Ctrl Pts',(4.77844989257998,6.30478688173537,33.6510605478402));
#48308=CARTESIAN_POINT('Ctrl Pts',(4.62190244378021,6.42343548222463,33.6589617990839));
#48309=CARTESIAN_POINT('Ctrl Pts',(4.46104597428791,6.53616467480275,33.6668630503276));
#48310=CARTESIAN_POINT('Ctrl Pts',(4.29637791989264,6.64266947615633,33.6747643015714));
#48311=CARTESIAN_POINT('Ctrl Pts',(4.13160075162838,6.7492448507063,33.6826707884152));
#48312=CARTESIAN_POINT('Ctrl Pts',(3.96300725859472,6.84958743595584,33.6905772752591));
#48313=CARTESIAN_POINT('Ctrl Pts',(3.79111903307485,6.94343844770425,33.698483762103));
#48314=CARTESIAN_POINT('Ctrl Pts',(3.61899400299996,7.03741875479565,33.7064011414445));
#48315=CARTESIAN_POINT('Ctrl Pts',(3.44356548136039,7.12488947176204,33.7143185207861));
#48316=CARTESIAN_POINT('Ctrl Pts',(3.26537564802098,7.20563965774806,33.7222359001277));
#48317=CARTESIAN_POINT('Ctrl Pts',(3.18811443439959,7.24065207822409,33.7256687914726));
#48318=CARTESIAN_POINT('Ctrl Pts',(3.11033430007697,7.27440167281522,33.7291016828176));
#48319=CARTESIAN_POINT('Ctrl Pts',(3.0320802757189,7.30687417447409,33.7325345741626));
#48320=CARTESIAN_POINT('Ctrl Pts',(2.8533275037777,7.38104990832296,33.7403762008229));
#48321=CARTESIAN_POINT('Ctrl Pts',(2.67156962090182,7.44877910061264,33.7482178274832));
#48322=CARTESIAN_POINT('Ctrl Pts',(2.48731673635885,7.50980535387098,33.7560594541435));
#48323=CARTESIAN_POINT('Ctrl Pts',(2.30328079570511,7.57075975331405,33.7638918478793));
#48324=CARTESIAN_POINT('Ctrl Pts',(2.11675603282264,7.62502681902685,33.771724241615));
#48325=CARTESIAN_POINT('Ctrl Pts',(1.92827486361654,7.67239708633127,33.7795566353508));
#48326=CARTESIAN_POINT('Ctrl Pts',(1.7399789255388,7.719720800189,33.7873813317492));
#48327=CARTESIAN_POINT('Ctrl Pts',(1.54973074833863,7.76016112808362,33.7952060281477));
#48328=CARTESIAN_POINT('Ctrl Pts',(1.35808052161118,7.79355748659239,33.8030307245462));
#48329=CARTESIAN_POINT('Ctrl Pts',(1.16658135471028,7.82692752189659,33.8108492534733));
#48330=CARTESIAN_POINT('Ctrl Pts',(0.973682683985094,7.8532645856887,33.8186677824005));
#48331=CARTESIAN_POINT('Ctrl Pts',(0.779947771138422,7.87245847714018,33.8264863113276));
#48332=CARTESIAN_POINT('Ctrl Pts',(0.586327885542514,7.89164097250133,33.8343001981183));
#48333=CARTESIAN_POINT('Ctrl Pts',(0.391873095806411,7.90368870919852,33.8421140849091));
#48334=CARTESIAN_POINT('Ctrl Pts',(0.197154910023527,7.90854290887099,33.8499279716999));
#48335=CARTESIAN_POINT('Ctrl Pts',(0.00251447890120057,7.91339517016957,
33.8577387382576));
#48336=CARTESIAN_POINT('Ctrl Pts',(-0.192388787611445,7.91105960878699,
33.8655495048153));
#48337=CARTESIAN_POINT('Ctrl Pts',(-0.386980039243796,7.90152943734483,
33.873360271373));
#48338=CARTESIAN_POINT('Ctrl Pts',(-0.581563556820466,7.89199964468062,
33.8811707274908));
#48339=CARTESIAN_POINT('Ctrl Pts',(-0.775834732537457,7.87527581978102,
33.8889811836085));
#48340=CARTESIAN_POINT('Ctrl Pts',(-0.969220026476353,7.85140328478147,
33.8967916397262));
#48341=CARTESIAN_POINT('Ctrl Pts',(-1.16261065360724,7.82753009142361,33.9046023112412));
#48342=CARTESIAN_POINT('Ctrl Pts',(-1.35511500086208,7.79650783757462,33.9124129827562));
#48343=CARTESIAN_POINT('Ctrl Pts',(-1.54616598484776,7.75843358850869,33.9202236542712));
#48344=CARTESIAN_POINT('Ctrl Pts',(-1.73725588444708,7.72035158401153,33.9280359167599));
#48345=CARTESIAN_POINT('Ctrl Pts',(-1.92689148591203,7.67521479159519,33.9358481792485));
#48346=CARTESIAN_POINT('Ctrl Pts',(-2.11451706105623,7.62317116418765,33.9436604417371));
#48347=CARTESIAN_POINT('Ctrl Pts',(-2.30221390004129,7.5711077695987,33.9514756714749));
#48348=CARTESIAN_POINT('Ctrl Pts',(-2.48789885315812,7.51213240844658,33.9592909012126));
#48349=CARTESIAN_POINT('Ctrl Pts',(-2.67103233821561,7.44644259013701,33.9671061309504));
#48350=CARTESIAN_POINT('Ctrl Pts',(-2.85436498982844,7.38068133096108,33.9749298601299));
#48351=CARTESIAN_POINT('Ctrl Pts',(-3.0351402999016,7.30819114865378,33.9827535893095));
#48352=CARTESIAN_POINT('Ctrl Pts',(-3.21283864744986,7.22921771877515,33.990577318489));
#48353=CARTESIAN_POINT('Ctrl Pts',(-3.39064480878037,7.15019637385234,33.9984057945097));
#48354=CARTESIAN_POINT('Ctrl Pts',(-3.5653699720372,7.0646840963973,34.0062342705304));
#48355=CARTESIAN_POINT('Ctrl Pts',(-3.73651997483667,6.97297206918589,34.0140627465511));
#48356=CARTESIAN_POINT('Ctrl Pts',(-3.90790552800753,6.88113382052127,34.0219019967488));
#48357=CARTESIAN_POINT('Ctrl Pts',(-4.07570579018091,6.78307895642799,34.0297412469466));
#48358=CARTESIAN_POINT('Ctrl Pts',(-4.23945541750854,6.67914206788248,34.0375804971443));
#48359=CARTESIAN_POINT('Ctrl Pts',(-4.33126379336439,6.62086848836599,34.041975675566));
#48360=CARTESIAN_POINT('Ctrl Pts',(-4.42179945894131,6.5607466756324,34.0463708539876));
#48361=CARTESIAN_POINT('Ctrl Pts',(-4.51098512448502,6.49884098948996,34.0507660324093));
#48362=CARTESIAN_POINT('Ctrl Pts',(-4.6706035382721,6.38804641991181,34.0586322226059));
#48363=CARTESIAN_POINT('Ctrl Pts',(-4.8263653571498,6.27120966955334,34.0664984128024));
#48364=CARTESIAN_POINT('Ctrl Pts',(-4.9777792821485,6.14862866159708,34.074364602999));
#48365=CARTESIAN_POINT('Ctrl Pts',(-5.12902791675357,6.02618146869817,34.0822222061011));
#48366=CARTESIAN_POINT('Ctrl Pts',(-5.27593784087924,5.89800272393123,34.0900798092033));
#48367=CARTESIAN_POINT('Ctrl Pts',(-5.41804577754358,5.76443413983039,34.0979374123054));
#48368=CARTESIAN_POINT('Ctrl Pts',(-5.56002581550766,5.63098576891893,34.1057879434786));
#48369=CARTESIAN_POINT('Ctrl Pts',(-5.69721222110953,5.49215745811834,34.1136384746519));
#48370=CARTESIAN_POINT('Ctrl Pts',(-5.82917376449969,5.34833191035004,34.1214890058251));
#48371=CARTESIAN_POINT('Ctrl Pts',(-5.96104181941303,5.20460825614136,34.1293339752704));
#48372=CARTESIAN_POINT('Ctrl Pts',(-6.0876921504874,5.05589467364254,34.1371789447157));
#48373=CARTESIAN_POINT('Ctrl Pts',(-6.20872931340659,4.9026116828529,34.145023914161));
#48374=CARTESIAN_POINT('Ctrl Pts',(-6.32970390662075,4.74940793112742,34.1528648281789));
#48375=CARTESIAN_POINT('Ctrl Pts',(-6.44507089687165,4.59163975082454,34.1607057421968));
#48376=CARTESIAN_POINT('Ctrl Pts',(-6.55447404215888,4.4297619609484,34.1685466562148));
#48377=CARTESIAN_POINT('Ctrl Pts',(-6.66442361566216,4.26707565142955,34.176426732696));
#48378=CARTESIAN_POINT('Ctrl Pts',(-6.76834937075488,4.10023883530814,34.1843068091772));
#48379=CARTESIAN_POINT('Ctrl Pts',(-6.86593240988546,3.92974466637266,34.1921868856584));
#48380=CARTESIAN_POINT('Ctrl Pts',(-6.96300230492519,3.76014704745341,34.2000255244602));
#48381=CARTESIAN_POINT('Ctrl Pts',(-7.05379587419109,3.58693076493575,34.2078641632621));
#48382=CARTESIAN_POINT('Ctrl Pts',(-7.13804420136761,3.41060786067854,34.215702802064));
#48383=CARTESIAN_POINT('Ctrl Pts',(-7.22229999029257,3.23426933976521,34.2235421351224));
#48384=CARTESIAN_POINT('Ctrl Pts',(-7.30000923125475,3.05482396421545,34.2313814681808));
#48385=CARTESIAN_POINT('Ctrl Pts',(-7.37095025389119,2.87280583309443,34.2392208012392));
#48386=CARTESIAN_POINT('Ctrl Pts',(-7.44190986601797,2.69074000567355,34.247062188528));
#48387=CARTESIAN_POINT('Ctrl Pts',(-7.50609759982208,2.50610040520851,34.2549035758168));
#48388=CARTESIAN_POINT('Ctrl Pts',(-7.56334089624944,2.31943861464809,34.2627449631057));
#48389=CARTESIAN_POINT('Ctrl Pts',(-7.62108722234317,2.13113651991079,34.2706552571605));
#48390=CARTESIAN_POINT('Ctrl Pts',(-7.67176637387579,1.94077687265887,34.2785655512153));
#48391=CARTESIAN_POINT('Ctrl Pts',(-7.71525345212281,1.74893829779871,34.2864758452701));
#48392=CARTESIAN_POINT('Ctrl Pts',(-7.75842621094329,1.55848630932855,34.2943289646608));
#48393=CARTESIAN_POINT('Ctrl Pts',(-7.79451051461208,1.36657705616842,34.3021820840515));
#48394=CARTESIAN_POINT('Ctrl Pts',(-7.823436143118,1.17378358931916,34.3100352034423));
#48395=CARTESIAN_POINT('Ctrl Pts',(-7.85267766133815,0.978884672172183,
34.3179740848291));
#48396=CARTESIAN_POINT('Ctrl Pts',(-7.87460319983354,0.783082483421094,
34.325912966216));
#48397=CARTESIAN_POINT('Ctrl Pts',(-7.88919428051167,0.586970701434065,
34.3338518476028));
#48398=CARTESIAN_POINT('Ctrl Pts',(-7.9037853611898,0.390858919447036,34.3417907289897));
#48399=CARTESIAN_POINT('Ctrl Pts',(-7.91104202717494,0.194437909010654,
34.3497296103765));
#48400=CARTESIAN_POINT('Ctrl Pts',(-7.91099981680841,-0.00170248562263939,
34.3576684917634));
#48401=CARTESIAN_POINT('',(-7.91065253198049,0.0049220711787074,36.3576684917634));
#48402=CARTESIAN_POINT('Ctrl Pts',(-7.92256293040024,-0.00170497406090317,
34.3576684917634));
#48403=CARTESIAN_POINT('Ctrl Pts',(-7.92283402357086,-0.0951406271396644,
34.3614448247277));
#48404=CARTESIAN_POINT('Ctrl Pts',(-7.92132116720036,-0.188567197001396,
34.3652211576919));
#48405=CARTESIAN_POINT('Ctrl Pts',(-7.824618403598,-2.90446889716205,34.4750746434051));
#48406=CARTESIAN_POINT('Ctrl Pts',(-4.77929028327528,-8.04776548189143,
34.6872289489031));
#48407=CARTESIAN_POINT('Ctrl Pts',(4.19818763349781,-8.36643474264993,35.0054604071498));
#48408=CARTESIAN_POINT('Ctrl Pts',(8.44002877177934,-2.22556932755547,35.2706532890221));
#48409=CARTESIAN_POINT('Ctrl Pts',(7.59677957168971,3.15057924978888,35.48280759452));
#48410=CARTESIAN_POINT('Ctrl Pts',(4.38769321310667,7.54555450367134,35.694961900018));
#48411=CARTESIAN_POINT('Ctrl Pts',(-2.95515982338205,8.8819502434627,35.9601547818902));
#48412=CARTESIAN_POINT('Ctrl Pts',(-7.54111000579349,3.94981135115549,36.1987365045968));
#48413=CARTESIAN_POINT('Ctrl Pts',(-7.91666636458249,0.66324315570486,36.3312410745546));
#48414=CARTESIAN_POINT('Ctrl Pts',(-7.91054183245,0.0064901895060634,36.3576684917634));
#48415=CARTESIAN_POINT('',(-7.911,-9.20097331658098E-12,38.3576684917634));
#48416=CARTESIAN_POINT('Ctrl Pts',(-7.911,-9.14712749988666E-12,36.3576684917634));
#48417=CARTESIAN_POINT('Ctrl Pts',(-7.91099999999745,-2.20167589667591,
36.4462559274961));
#48418=CARTESIAN_POINT('Ctrl Pts',(-6.94214576671865,-4.38610418339484,
36.5348433632289));
#48419=CARTESIAN_POINT('Ctrl Pts',(-3.6782020148744,-7.34180684108056,36.7120182346943));
#48420=CARTESIAN_POINT('Ctrl Pts',(-1.40868175870812,-8.08992666571498,
36.800605670427));
#48421=CARTESIAN_POINT('Ctrl Pts',(2.97309270522153,-7.65454228024915,36.9777805418925));
#48422=CARTESIAN_POINT('Ctrl Pts',(5.05102072676346,-6.47444880833645,37.0663679776252));
#48423=CARTESIAN_POINT('Ctrl Pts',(7.66951518848208,-2.93425195366828,37.2435428490907));
#48424=CARTESIAN_POINT('Ctrl Pts',(8.1895687224714,-0.601881960089796,37.3321302848234));
#48425=CARTESIAN_POINT('Ctrl Pts',(7.32306689760918,3.71537198233286,37.5093051562888));
#48426=CARTESIAN_POINT('Ctrl Pts',(5.94329958849555,5.66643518937189,37.5978925920216));
#48427=CARTESIAN_POINT('Ctrl Pts',(2.16154501636946,7.92205913233244,37.775067463487));
#48428=CARTESIAN_POINT('Ctrl Pts',(-0.210816529309703,8.20894963712978,
37.8636548992197));
#48429=CARTESIAN_POINT('Ctrl Pts',(-4.42123908577222,6.91982244717329,38.0408297706852));
#48430=CARTESIAN_POINT('Ctrl Pts',(-6.22631625634795,5.35390358802815,38.1294172064179));
#48431=CARTESIAN_POINT('Ctrl Pts',(-7.65317280859754,2.31334857513645,38.2645592586882));
#48432=CARTESIAN_POINT('Ctrl Pts',(-7.91100000000134,1.15702837835607,38.3111138752258));
#48433=CARTESIAN_POINT('Ctrl Pts',(-7.911,-9.20097331658098E-12,38.3576684917634));
#48434=CARTESIAN_POINT('',(-7.911,-9.14324171930048E-12,40.3576684917634));
#48435=CARTESIAN_POINT('Ctrl Pts',(-7.911,-9.20097331658098E-12,38.3576684917634));
#48436=CARTESIAN_POINT('Ctrl Pts',(-7.91099999999744,-2.20167589667592,
38.4462559274961));
#48437=CARTESIAN_POINT('Ctrl Pts',(-6.94214576671865,-4.38610418339481,
38.5348433632289));
#48438=CARTESIAN_POINT('Ctrl Pts',(-3.67820201487448,-7.3418068410805,38.7120182346943));
#48439=CARTESIAN_POINT('Ctrl Pts',(-1.40868175870826,-8.08992666571495,
38.800605670427));
#48440=CARTESIAN_POINT('Ctrl Pts',(2.97309270522133,-7.65454228024922,38.9777805418925));
#48441=CARTESIAN_POINT('Ctrl Pts',(5.05102072676325,-6.4744488083366,39.0663679776252));
#48442=CARTESIAN_POINT('Ctrl Pts',(7.66951518848195,-2.93425195366858,39.2435428490906));
#48443=CARTESIAN_POINT('Ctrl Pts',(8.18956872247136,-0.601881960090168,
39.3321302848234));
#48444=CARTESIAN_POINT('Ctrl Pts',(7.32306689760937,3.71537198233245,39.5093051562888));
#48445=CARTESIAN_POINT('Ctrl Pts',(5.94329958849588,5.66643518937152,39.5978925920215));
#48446=CARTESIAN_POINT('Ctrl Pts',(2.16154501637,7.92205913233228,39.775067463487));
#48447=CARTESIAN_POINT('Ctrl Pts',(-0.210816529309095,8.20894963712979,
39.8636548992197));
#48448=CARTESIAN_POINT('Ctrl Pts',(-4.42123908577165,6.91982244717365,40.0408297706852));
#48449=CARTESIAN_POINT('Ctrl Pts',(-6.22631625634747,5.35390358802869,40.1294172064179));
#48450=CARTESIAN_POINT('Ctrl Pts',(-7.65317280859742,2.31334857513695,40.2645592586882));
#48451=CARTESIAN_POINT('Ctrl Pts',(-7.91100000000134,1.15702837835635,40.3111138752258));
#48452=CARTESIAN_POINT('Ctrl Pts',(-7.911,-9.14324171930048E-12,40.3576684917634));
#48453=CARTESIAN_POINT('',(-7.91099967169525,0.00226142970142933,42.3575775000139));
#48454=CARTESIAN_POINT('Ctrl Pts',(-7.911,-9.14324171930048E-12,40.3576684917634));
#48455=CARTESIAN_POINT('Ctrl Pts',(-7.91099999999746,-2.2016758966759,40.4462559274961));
#48456=CARTESIAN_POINT('Ctrl Pts',(-6.94214576671865,-4.38610418339484,
40.5348433632289));
#48457=CARTESIAN_POINT('Ctrl Pts',(-3.6782020148744,-7.34180684108056,40.7120182346943));
#48458=CARTESIAN_POINT('Ctrl Pts',(-1.40868175870813,-8.08992666571498,
40.800605670427));
#48459=CARTESIAN_POINT('Ctrl Pts',(2.97309270522157,-7.65454228024915,40.9777805418925));
#48460=CARTESIAN_POINT('Ctrl Pts',(5.05102072676352,-6.47444880833642,41.0663679776252));
#48461=CARTESIAN_POINT('Ctrl Pts',(7.66951518848214,-2.93425195366815,41.2435428490907));
#48462=CARTESIAN_POINT('Ctrl Pts',(8.18956872247142,-0.601881960089605,
41.3321302848234));
#48463=CARTESIAN_POINT('Ctrl Pts',(7.32306689760907,3.7153719823331,41.5093051562888));
#48464=CARTESIAN_POINT('Ctrl Pts',(5.94329958849534,5.66643518937212,41.5978925920216));
#48465=CARTESIAN_POINT('Ctrl Pts',(2.16154501636909,7.92205913233254,41.775067463487));
#48466=CARTESIAN_POINT('Ctrl Pts',(-0.210816529310129,8.20894963712978,
41.8636548992198));
#48467=CARTESIAN_POINT('Ctrl Pts',(-4.42123908577265,6.91982244717303,42.0408297706852));
#48468=CARTESIAN_POINT('Ctrl Pts',(-6.22631625634831,5.35390358802774,42.1294172064179));
#48469=CARTESIAN_POINT('Ctrl Pts',(-7.65285257229365,2.31403098157547,42.2645289281051));
#48470=CARTESIAN_POINT('Ctrl Pts',(-7.91066394919783,1.15853502979653,42.3110532140595));
#48471=CARTESIAN_POINT('Ctrl Pts',(-7.91099967169525,0.00226142970142933,
42.3575775000139));
#48472=CARTESIAN_POINT('',(-7.91099966078395,0.00163815081257414,44.3576684917634));
#48473=CARTESIAN_POINT('Ctrl Pts',(-7.91099967460919,0.00226899390551966,
42.3577662811419));
#48474=CARTESIAN_POINT('Ctrl Pts',(-7.91105523449881,-0.19144429357958,
42.3655880831917));
#48475=CARTESIAN_POINT('Ctrl Pts',(-7.9039914899811,-0.38540394722232,42.3734098852415));
#48476=CARTESIAN_POINT('Ctrl Pts',(-7.88978036946687,-0.579039481879457,
42.3812316872913));
#48477=CARTESIAN_POINT('Ctrl Pts',(-7.87558204539206,-0.772500656929422,
42.3890464461796));
#48478=CARTESIAN_POINT('Ctrl Pts',(-7.8542491874259,-0.965637944728926,
42.3968612050679));
#48479=CARTESIAN_POINT('Ctrl Pts',(-7.82580574136786,-1.15787974262179,
42.4046759639563));
#48480=CARTESIAN_POINT('Ctrl Pts',(-7.79738233777216,-1.34998607876402,
42.412485216233));
#48481=CARTESIAN_POINT('Ctrl Pts',(-7.76185837669972,-1.54119783421374,
42.4202944685097));
#48482=CARTESIAN_POINT('Ctrl Pts',(-7.71930972670178,-1.73094723872432,
42.4281037207864));
#48483=CARTESIAN_POINT('Ctrl Pts',(-7.67678273016845,-1.92060007772652,
42.4359089988509));
#48484=CARTESIAN_POINT('Ctrl Pts',(-7.62723824307516,-2.10879170477572,
42.4437142769153));
#48485=CARTESIAN_POINT('Ctrl Pts',(-7.57080348232179,-2.29496310037094,
42.4515195549797));
#48486=CARTESIAN_POINT('Ctrl Pts',(-7.51311269925965,-2.48527796043738,
42.4594985487336));
#48487=CARTESIAN_POINT('Ctrl Pts',(-7.44822142064704,-2.67348124129677,
42.4674775424875));
#48488=CARTESIAN_POINT('Ctrl Pts',(-7.37632005783899,-2.85898992728588,
42.4754565362414));
#48489=CARTESIAN_POINT('Ctrl Pts',(-7.30600106045762,-3.04041604071181,
42.4832599327137));
#48490=CARTESIAN_POINT('Ctrl Pts',(-7.22897744319996,-3.21926458296378,
42.4910633291859));
#48491=CARTESIAN_POINT('Ctrl Pts',(-7.1454767238172,-3.39500859930968,42.4988667256582));
#48492=CARTESIAN_POINT('Ctrl Pts',(-7.06196661380801,-3.57077238011288,
42.5066709997131));
#48493=CARTESIAN_POINT('Ctrl Pts',(-6.97197810182106,-3.74343062041715,
42.514475273768));
#48494=CARTESIAN_POINT('Ctrl Pts',(-6.87578554007716,-3.91247929155744,
42.5222795478228));
#48495=CARTESIAN_POINT('Ctrl Pts',(-6.77956510754424,-4.08157694278271,
42.5300860830845));
#48496=CARTESIAN_POINT('Ctrl Pts',(-6.67713721925833,-4.24706263493058,
42.5378926183462));
#48497=CARTESIAN_POINT('Ctrl Pts',(-6.56882064692729,-4.40845962990495,
42.5456991536079));
#48498=CARTESIAN_POINT('Ctrl Pts',(-6.45629780081742,-4.57612417871097,
42.5538088412301));
#48499=CARTESIAN_POINT('Ctrl Pts',(-6.3374200012213,-4.73937577021939,42.5619185288522));
#48500=CARTESIAN_POINT('Ctrl Pts',(-6.21259151317871,-4.89771657922137,
42.5700282164743));
#48501=CARTESIAN_POINT('Ctrl Pts',(-6.09223400357626,-5.05038609992736,
42.5778474396433));
#48502=CARTESIAN_POINT('Ctrl Pts',(-5.96634494839708,-5.19849028389335,
42.5856666628123));
#48503=CARTESIAN_POINT('Ctrl Pts',(-5.83532506711406,-5.34161982558758,
42.5934858859812));
#48504=CARTESIAN_POINT('Ctrl Pts',(-5.70421447027605,-5.48484846732435,
42.6013105230245));
#48505=CARTESIAN_POINT('Ctrl Pts',(-5.56796621521892,-5.62309535359634,
42.6091351600679));
#48506=CARTESIAN_POINT('Ctrl Pts',(-5.42701555307506,-5.75599020036356,
42.6169597971111));
#48507=CARTESIAN_POINT('Ctrl Pts',(-5.28588402170887,-5.88905557905466,
42.6247944748027));
#48508=CARTESIAN_POINT('Ctrl Pts',(-5.14003830250138,-6.01675497905471,
42.6326291524942));
#48509=CARTESIAN_POINT('Ctrl Pts',(-4.9899448138045,-6.13875978966319,42.6404638301857));
#48510=CARTESIAN_POINT('Ctrl Pts',(-4.97365081118194,-6.1520045128106,42.6413143551483));
#48511=CARTESIAN_POINT('Ctrl Pts',(-4.95730677432316,-6.16518216827127,
42.6421648801108));
#48512=CARTESIAN_POINT('Ctrl Pts',(-4.94091331848041,-6.17829236757722,
42.6430154050734));
#48513=CARTESIAN_POINT('Ctrl Pts',(-4.78976977061013,-6.29916511432414,
42.6508570317337));
#48514=CARTESIAN_POINT('Ctrl Pts',(-4.6339499961255,-6.41467861723858,42.6586986583941));
#48515=CARTESIAN_POINT('Ctrl Pts',(-4.47387290355124,-6.52444497584814,
42.6665402850544));
#48516=CARTESIAN_POINT('Ctrl Pts',(-4.31398428969263,-6.63408209284067,
42.6743726787902));
#48517=CARTESIAN_POINT('Ctrl Pts',(-4.14984862551579,-6.73798534271742,
42.682205072526));
#48518=CARTESIAN_POINT('Ctrl Pts',(-3.98191927558171,-6.83580572301107,
42.6900374662618));
#48519=CARTESIAN_POINT('Ctrl Pts',(-3.81415495933828,-6.9335299696724,42.6978621626603));
#48520=CARTESIAN_POINT('Ctrl Pts',(-3.64260468331891,-7.02518307570911,
42.7056868590588));
#48521=CARTESIAN_POINT('Ctrl Pts',(-3.46775245403099,-7.11045806664817,
42.7135115554573));
#48522=CARTESIAN_POINT('Ctrl Pts',(-3.29303804429053,-7.19566584334176,
42.7213300843844));
#48523=CARTESIAN_POINT('Ctrl Pts',(-3.11502717932611,-7.27450536421443,
42.7291486133116));
#48524=CARTESIAN_POINT('Ctrl Pts',(-2.9342304073972,-7.34671443002283,42.7369671422387));
#48525=CARTESIAN_POINT('Ctrl Pts',(-2.75354098088784,-7.41888062276231,
42.7447810290295));
#48526=CARTESIAN_POINT('Ctrl Pts',(-2.5700692679648,-7.48442407223109,42.7525949158203));
#48527=CARTESIAN_POINT('Ctrl Pts',(-2.38434801111233,-7.5431296927671,42.7604088026111));
#48528=CARTESIAN_POINT('Ctrl Pts',(-2.19870091627492,-7.60181187103706,
42.7682195691689));
#48529=CARTESIAN_POINT('Ctrl Pts',(-2.01080640209859,-7.65366155461945,
42.7760303357267));
#48530=CARTESIAN_POINT('Ctrl Pts',(-1.82121485153133,-7.69851267872968,
42.7838411022845));
#48531=CARTESIAN_POINT('Ctrl Pts',(-1.63163083630754,-7.74336202022554,
42.7916515584023));
#48532=CARTESIAN_POINT('Ctrl Pts',(-1.44035025919597,-7.78121326662324,
42.7994620145201));
#48533=CARTESIAN_POINT('Ctrl Pts',(-1.24793670675543,-7.81195077915449,
42.8072724706378));
#48534=CARTESIAN_POINT('Ctrl Pts',(-1.0555178479215,-7.84268913936685,42.8150831421529));
#48535=CARTESIAN_POINT('Ctrl Pts',(-0.86196629896923,-7.86631331859884,
42.8228938136679));
#48536=CARTESIAN_POINT('Ctrl Pts',(-0.667853804383722,-7.88275918038666,
42.8307044851829));
#48537=CARTESIAN_POINT('Ctrl Pts',(-0.473701770577963,-7.89920839206988,
42.8385167476716));
#48538=CARTESIAN_POINT('Ctrl Pts',(-0.27898891418997,-7.908476343858,42.8463290101603));
#48539=CARTESIAN_POINT('Ctrl Pts',(-0.0842901939676469,-7.91055093929626,
42.854141272649));
#48540=CARTESIAN_POINT('Ctrl Pts',(0.110482476612491,-7.91262632270618,
42.8619565023867));
#48541=CARTESIAN_POINT('Ctrl Pts',(0.305240648751071,-7.907502903694,42.8697717321245));
#48542=CARTESIAN_POINT('Ctrl Pts',(0.499411121469912,-7.89522067657087,
42.8775869618623));
#48543=CARTESIAN_POINT('Ctrl Pts',(0.693792764004116,-7.88292509192949,
42.8854106910419));
#48544=CARTESIAN_POINT('Ctrl Pts',(0.887585079272827,-7.86345517138622,
42.8932344202214));
#48545=CARTESIAN_POINT('Ctrl Pts',(1.0802206752646,-7.83690272318924,42.9010581494009));
#48546=CARTESIAN_POINT('Ctrl Pts',(1.27297314782017,-7.8103341649951,42.9088866254217));
#48547=CARTESIAN_POINT('Ctrl Pts',(1.464567156976,-7.77667457607048,42.9167151014424));
#48548=CARTESIAN_POINT('Ctrl Pts',(1.65444713907479,-7.73606654986934,42.9245435774631));
#48549=CARTESIAN_POINT('Ctrl Pts',(1.84458844924595,-7.69540263564307,42.9323828276609));
#48550=CARTESIAN_POINT('Ctrl Pts',(2.03301068071,-7.64777126942025,42.9402220778587));
#48551=CARTESIAN_POINT('Ctrl Pts',(2.21917390866053,-7.59336474582384,42.9480613280565));
#48552=CARTESIAN_POINT('Ctrl Pts',(2.32354876361187,-7.56286101492435,42.9524565064778));
#48553=CARTESIAN_POINT('Ctrl Pts',(2.42721386694964,-7.53022843219252,42.956851684899));
#48554=CARTESIAN_POINT('Ctrl Pts',(2.5300771028892,-7.49550737798555,42.9612468633203));
#48555=CARTESIAN_POINT('Ctrl Pts',(2.71519729417709,-7.43302083322734,42.9691567473781));
#48556=CARTESIAN_POINT('Ctrl Pts',(2.89825112111964,-7.36358785461777,42.9770666314358));
#48557=CARTESIAN_POINT('Ctrl Pts',(3.07867941314536,-7.28736262793851,42.9849765154936));
#48558=CARTESIAN_POINT('Ctrl Pts',(3.25891154936043,-7.21122027086337,42.992877800181));
#48559=CARTESIAN_POINT('Ctrl Pts',(3.43652352126279,-7.12830050708488,43.0007790848683));
#48560=CARTESIAN_POINT('Ctrl Pts',(3.61097120465141,-7.0388072824292,43.0086803695556));
#48561=CARTESIAN_POINT('Ctrl Pts',(3.78526165073689,-6.94939472191891,43.0165745324706));
#48562=CARTESIAN_POINT('Ctrl Pts',(3.95639318493084,-6.85342065991789,43.0244686953856));
#48563=CARTESIAN_POINT('Ctrl Pts',(4.12384131043278,-6.75113722615442,43.0323628583005));
#48564=CARTESIAN_POINT('Ctrl Pts',(4.29116961380941,-6.64892698412351,43.0402513723294));
#48565=CARTESIAN_POINT('Ctrl Pts',(4.45481946661778,-6.54041654446315,43.0481398863583));
#48566=CARTESIAN_POINT('Ctrl Pts',(4.61429041088716,-6.42590421683943,43.0560284003873));
#48567=CARTESIAN_POINT('Ctrl Pts',(4.77367685895037,-6.31145256395047,43.063912734661));
#48568=CARTESIAN_POINT('Ctrl Pts',(4.92888853101546,-6.19100556059785,43.0717970689347));
#48569=CARTESIAN_POINT('Ctrl Pts',(5.07945320974837,-6.0649052828529,43.0796814032084));
#48570=CARTESIAN_POINT('Ctrl Pts',(5.22996607024078,-5.93884840369633,43.0875630240149));
#48571=CARTESIAN_POINT('Ctrl Pts',(5.37583486070327,-5.80714234904797,43.0954446448213));
#48572=CARTESIAN_POINT('Ctrl Pts',(5.51661955856436,-5.67017016023903,43.1033262656277));
#48573=CARTESIAN_POINT('Ctrl Pts',(5.65740610033338,-5.53319617745597,43.1112079896626));
#48574=CARTESIAN_POINT('Ctrl Pts',(5.79310816325151,-5.3909561571011,43.1190897136975));
#48575=CARTESIAN_POINT('Ctrl Pts',(5.9233213853265,-5.24387116223633,43.1269714377324));
#48576=CARTESIAN_POINT('Ctrl Pts',(6.05354245146998,-5.09677730694437,43.1348536365637));
#48577=CARTESIAN_POINT('Ctrl Pts',(6.17827378864938,-4.94483815361627,43.1427358353951));
#48578=CARTESIAN_POINT('Ctrl Pts',(6.29715024632641,-4.78850913909447,43.1506180342265));
#48579=CARTESIAN_POINT('Ctrl Pts',(6.41605386852112,-4.63214440175283,43.158502034223));
#48580=CARTESIAN_POINT('Ctrl Pts',(6.52909973635385,-4.471388079023,43.1663860342195));
#48581=CARTESIAN_POINT('Ctrl Pts',(6.63596494679445,-4.30672616089244,43.174270034216));
#48582=CARTESIAN_POINT('Ctrl Pts',(6.74287255953469,-4.14199890771071,43.1821571624497));
#48583=CARTESIAN_POINT('Ctrl Pts',(6.84359444060331,-3.97336326049963,43.1900442906835));
#48584=CARTESIAN_POINT('Ctrl Pts',(6.93785258916042,-3.8013316681237,43.1979314189172));
#48585=CARTESIAN_POINT('Ctrl Pts',(7.03221130039376,-3.629116537692,43.2058269618157));
#48586=CARTESIAN_POINT('Ctrl Pts',(7.12009233889316,-3.45349852796777,43.2137225047142));
#48587=CARTESIAN_POINT('Ctrl Pts',(7.20126451919202,-3.27501302663458,43.2216180476127));
#48588=CARTESIAN_POINT('Ctrl Pts',(7.28248613053575,-3.09641883381627,43.2295183986233));
#48589=CARTESIAN_POINT('Ctrl Pts',(7.35699060808092,-2.91495398644879,43.2374187496338));
#48590=CARTESIAN_POINT('Ctrl Pts',(7.42459590233919,-2.73117130311668,43.2453191006443));
#48591=CARTESIAN_POINT('Ctrl Pts',(7.49228922153324,-2.54714932700325,43.2532297382441));
#48592=CARTESIAN_POINT('Ctrl Pts',(7.55306530770237,-2.36080381382491,43.2611403758438));
#48593=CARTESIAN_POINT('Ctrl Pts',(7.6067923898368,-2.17270120769538,43.2690510134435));
#48594=CARTESIAN_POINT('Ctrl Pts',(7.63039895053558,-2.0900528409353,43.272526782818));
#48595=CARTESIAN_POINT('Ctrl Pts',(7.65264534020375,-2.00706537838969,43.2760025521925));
#48596=CARTESIAN_POINT('Ctrl Pts',(7.67352353208574,-1.92378730698753,43.279478321567));
#48597=CARTESIAN_POINT('Ctrl Pts',(7.72103637620601,-1.73427003233409,43.2873881870105));
#48598=CARTESIAN_POINT('Ctrl Pts',(7.76158824895091,-1.54273577210148,43.2952980524539));
#48599=CARTESIAN_POINT('Ctrl Pts',(7.79500657608151,-1.34973830013301,43.3032079178973));
#48600=CARTESIAN_POINT('Ctrl Pts',(7.82838858442728,-1.15695057635546,43.3111091869589));
#48601=CARTESIAN_POINT('Ctrl Pts',(7.8546524309102,-0.962703145096539,43.3190104560205));
#48602=CARTESIAN_POINT('Ctrl Pts',(7.87367553765369,-0.767564021925151,
43.326911725082));
#48603=CARTESIAN_POINT('Ctrl Pts',(7.89268150517765,-0.572600712952502,
43.3348058753493));
#48604=CARTESIAN_POINT('Ctrl Pts',(7.90445969534575,-0.376747653637676,
43.3427000256165));
#48605=CARTESIAN_POINT('Ctrl Pts',(7.9089386771246,-0.180582395273219,43.3505941758837));
#48606=CARTESIAN_POINT('Ctrl Pts',(7.91341445552419,0.0154425651954087,
43.3584826802344));
#48607=CARTESIAN_POINT('Ctrl Pts',(7.91060141846242,0.211778936393597,43.3663711845851));
#48608=CARTESIAN_POINT('Ctrl Pts',(7.90047998062532,0.407844425901003,43.3742596889358));
#48609=CARTESIAN_POINT('Ctrl Pts',(7.89036390187049,0.603806102975317,43.3821440164942));
#48610=CARTESIAN_POINT('Ctrl Pts',(7.87294715080648,0.799496840469732,43.3900283440526));
#48611=CARTESIAN_POINT('Ctrl Pts',(7.84826222883147,0.994334444488994,43.3979126716109));
#48612=CARTESIAN_POINT('Ctrl Pts',(7.82358579314876,1.18910506637002,43.4057942886601));
#48613=CARTESIAN_POINT('Ctrl Pts',(7.79164620979011,1.38302279749853,43.4136759057093));
#48614=CARTESIAN_POINT('Ctrl Pts',(7.75252784787185,1.5755103833271,43.4215575227585));
#48615=CARTESIAN_POINT('Ctrl Pts',(7.7134089516409,1.76800059831891,43.4294392474617));
#48616=CARTESIAN_POINT('Ctrl Pts',(7.66711114124667,1.95906028924922,43.4373209721648));
#48617=CARTESIAN_POINT('Ctrl Pts',(7.61377005084622,2.14812164758823,43.445202696868));
#48618=CARTESIAN_POINT('Ctrl Pts',(7.56042572850756,2.33719446116041,43.4530848991251));
#48619=CARTESIAN_POINT('Ctrl Pts',(7.50003736894496,2.52426836850037,43.4609671013822));
#48620=CARTESIAN_POINT('Ctrl Pts',(7.43279072190796,2.70878996681524,43.4688493036393));
#48621=CARTESIAN_POINT('Ctrl Pts',(7.36552868477923,2.8933537948092,43.4767333098201));
#48622=CARTESIAN_POINT('Ctrl Pts',(7.29140535068825,3.07536382558975,43.4846173160008));
#48623=CARTESIAN_POINT('Ctrl Pts',(7.21065501198952,3.25428568169274,43.4925013221815));
#48624=CARTESIAN_POINT('Ctrl Pts',(7.12987260467482,3.43327859355085,43.5003884593605));
#48625=CARTESIAN_POINT('Ctrl Pts',(7.04245809050236,3.60918057272071,43.5082755965394));
#48626=CARTESIAN_POINT('Ctrl Pts',(6.94869229507463,3.78148071373773,43.5161627337184));
#48627=CARTESIAN_POINT('Ctrl Pts',(6.85482641325402,3.95396476936381,43.5240582896934));
#48628=CARTESIAN_POINT('Ctrl Pts',(6.7545958738127,4.12283900429356,43.5319538456684));
#48629=CARTESIAN_POINT('Ctrl Pts',(6.6483261086347,4.28761949725559,43.5398494016435));
#48630=CARTESIAN_POINT('Ctrl Pts',(6.54199159697163,4.45250038526138,43.5477497681071));
#48631=CARTESIAN_POINT('Ctrl Pts',(6.42961072118199,4.61328227678453,43.5556501345708));
#48632=CARTESIAN_POINT('Ctrl Pts',(6.31155014000222,4.76951316490875,43.5635505010344));
#48633=CARTESIAN_POINT('Ctrl Pts',(6.193335786551,4.92594754160046,43.571461157616));
#48634=CARTESIAN_POINT('Ctrl Pts',(6.06942716860398,5.0778188082938,43.5793718141975));
#48635=CARTESIAN_POINT('Ctrl Pts',(5.94022958811885,5.22470989055253,43.587282470779));
#48636=CARTESIAN_POINT('Ctrl Pts',(5.8834629938259,5.28925062297586,43.5907582404573));
#48637=CARTESIAN_POINT('Ctrl Pts',(5.82567580896491,5.35283041298148,43.5942340101355));
#48638=CARTESIAN_POINT('Ctrl Pts',(5.76690448498989,5.41541629618661,43.5977097798138));
#48639=CARTESIAN_POINT('Ctrl Pts',(5.63435879033588,5.55656488369309,43.6055486079242));
#48640=CARTESIAN_POINT('Ctrl Pts',(5.49642770460188,5.69305753192045,43.6133874360346));
#48641=CARTESIAN_POINT('Ctrl Pts',(5.35347325052906,5.82445234814998,43.6212262641451));
#48642=CARTESIAN_POINT('Ctrl Pts',(5.21067904618544,5.95569987282532,43.6290563050506));
#48643=CARTESIAN_POINT('Ctrl Pts',(5.06287294244189,6.08186070890334,43.636886345956));
#48644=CARTESIAN_POINT('Ctrl Pts',(4.91045639755445,6.2025268212009,43.6447163868615));
#48645=CARTESIAN_POINT('Ctrl Pts',(4.75818104479671,6.3230811536035,43.652539174354));
#48646=CARTESIAN_POINT('Ctrl Pts',(4.60130402998158,6.43815068211475,43.6603619618465));
#48647=CARTESIAN_POINT('Ctrl Pts',(4.4402628923503,6.54736484754111,43.668184749339));
#48648=CARTESIAN_POINT('Ctrl Pts',(4.2793396101219,6.65649908631235,43.6760018118485));
#48649=CARTESIAN_POINT('Ctrl Pts',(4.11425856448946,6.75978630029101,43.683818874358));
#48650=CARTESIAN_POINT('Ctrl Pts',(3.94548968584606,6.85689668427944,43.6916359368675));
#48651=CARTESIAN_POINT('Ctrl Pts',(3.77681150067302,6.95395488283058,43.6994487986231));
#48652=CARTESIAN_POINT('Ctrl Pts',(3.6044497343129,7.04484268857589,43.7072616603787));
#48653=CARTESIAN_POINT('Ctrl Pts',(3.4289027180311,7.12927395674194,43.7150745221343));
#48654=CARTESIAN_POINT('Ctrl Pts',(3.25341591070757,7.21367626674733,43.7228847042415));
#48655=CARTESIAN_POINT('Ctrl Pts',(3.07474634675879,7.29162629907549,43.7306948863488));
#48656=CARTESIAN_POINT('Ctrl Pts',(2.8934165052976,7.36288407669654,43.7385050684561));
#48657=CARTESIAN_POINT('Ctrl Pts',(2.71207848574386,7.43414506808922,43.7463156028076));
#48658=CARTESIAN_POINT('Ctrl Pts',(2.52808027299092,7.49871306450029,43.7541261371591));
#48659=CARTESIAN_POINT('Ctrl Pts',(2.34196433521704,7.55639623448714,43.7619366715106));
#48660=CARTESIAN_POINT('Ctrl Pts',(2.15583348007587,7.61408402783426,43.7697478318838));
#48661=CARTESIAN_POINT('Ctrl Pts',(1.96758489780044,7.66488579049288,43.777558992257));
#48662=CARTESIAN_POINT('Ctrl Pts',(1.7777761413379,7.70865961054772,43.7853701526301));
#48663=CARTESIAN_POINT('Ctrl Pts',(1.58791874245647,7.75244464854915,43.7931833147747));
#48664=CARTESIAN_POINT('Ctrl Pts',(1.39650071577984,7.78919807689108,43.8009964769192));
#48665=CARTESIAN_POINT('Ctrl Pts',(1.20408987311681,7.81882910527258,43.8088096390638));
#48666=CARTESIAN_POINT('Ctrl Pts',(1.01159583085082,7.84847294628855,43.8166261796665));
#48667=CARTESIAN_POINT('Ctrl Pts',(0.818108464844139,7.87098819881346,43.8244427202693));
#48668=CARTESIAN_POINT('Ctrl Pts',(0.624200925947996,7.88633591752505,43.832259260872));
#48669=CARTESIAN_POINT('Ctrl Pts',(0.430067093424239,7.90170154730375,43.8400849235199));
#48670=CARTESIAN_POINT('Ctrl Pts',(0.235512459454907,7.90988290886475,43.8479105861679));
#48671=CARTESIAN_POINT('Ctrl Pts',(0.0411115081473399,7.91089317611468,
43.8557362488158));
#48672=CARTESIAN_POINT('Ctrl Pts',(-0.153416159942628,7.91190410188925,
43.8635670124819));
#48673=CARTESIAN_POINT('Ctrl Pts',(-0.34778959534068,7.90573462937797,43.871397776148));
#48674=CARTESIAN_POINT('Ctrl Pts',(-0.541439143345873,7.89244985122192,
43.8792285398141));
#48675=CARTESIAN_POINT('Ctrl Pts',(-0.735368494589738,7.87914587795805,
43.8870706181105));
#48676=CARTESIAN_POINT('Ctrl Pts',(-0.928571520869114,7.85870610168352,
43.8949126964069));
#48677=CARTESIAN_POINT('Ctrl Pts',(-1.12048728004616,7.83124697958472,43.9027547747032));
#48678=CARTESIAN_POINT('Ctrl Pts',(-1.22805613405249,7.8158561314915,43.9071502624891));
#48679=CARTESIAN_POINT('Ctrl Pts',(-1.33522080975073,7.79826099232864,43.9115457502749));
#48680=CARTESIAN_POINT('Ctrl Pts',(-1.4418846728385,7.77848890146624,43.9159412380607));
#48681=CARTESIAN_POINT('Ctrl Pts',(-1.63399236896911,7.74287823902345,43.9238577620592));
#48682=CARTESIAN_POINT('Ctrl Pts',(-1.82505123055244,7.70009627128783,43.9317742860576));
#48683=CARTESIAN_POINT('Ctrl Pts',(-2.01448541291256,7.65021369120906,43.9396908100561));
#48684=CARTESIAN_POINT('Ctrl Pts',(-2.2037013555568,7.60038857890071,43.9475982137368));
#48685=CARTESIAN_POINT('Ctrl Pts',(-2.39129601721905,7.54347923481972,43.9555056174174));
#48686=CARTESIAN_POINT('Ctrl Pts',(-2.57670109950925,7.47960777339212,43.9634130210981));
#48687=CARTESIAN_POINT('Ctrl Pts',(-2.76192694035415,7.41579806007261,43.9713127802501));
#48688=CARTESIAN_POINT('Ctrl Pts',(-2.94496709509954,7.34503974866953,43.9792125394021));
#48689=CARTESIAN_POINT('Ctrl Pts',(-3.12526557042166,7.26750549462035,43.9871122985541));
#48690=CARTESIAN_POINT('Ctrl Pts',(-3.30542313960086,7.19003183483112,43.9950058839179));
#48691=CARTESIAN_POINT('Ctrl Pts',(-3.48284298314604,7.10579291813421,44.0028994692818));
#48692=CARTESIAN_POINT('Ctrl Pts',(-3.65698606732593,7.01501061320538,44.0107930546456));
#48693=CARTESIAN_POINT('Ctrl Pts',(-3.83102530592119,6.92428244388333,44.0186819328803));
#48694=CARTESIAN_POINT('Ctrl Pts',(-4.00179137401646,6.82701882018973,44.026570811115));
#48695=CARTESIAN_POINT('Ctrl Pts',(-4.16876670559107,6.72348906107204,44.0344596893497));
#48696=CARTESIAN_POINT('Ctrl Pts',(-4.33567338274859,6.62000186977078,44.0423453239536));
#48697=CARTESIAN_POINT('Ctrl Pts',(-4.49879213724428,6.51025385902708,44.0502309585574));
#48698=CARTESIAN_POINT('Ctrl Pts',(-4.65763119171931,6.39455961594881,44.0581165931612));
#48699=CARTESIAN_POINT('Ctrl Pts',(-4.81645611641754,6.27887566463308,44.0660015262861));
#48700=CARTESIAN_POINT('Ctrl Pts',(-4.97100181737944,6.15724673240566,44.073886459411));
#48701=CARTESIAN_POINT('Ctrl Pts',(-5.12080621286675,6.03003024289806,44.0817713925359));
#48702=CARTESIAN_POINT('Ctrl Pts',(-5.27061008897105,5.90281419445952,44.0896562983231));
#48703=CARTESIAN_POINT('Ctrl Pts',(-5.41567242922947,5.77001085004406,44.0975412041103));
#48704=CARTESIAN_POINT('Ctrl Pts',(-5.55556483856092,5.63201742935385,44.1054261098976));
#48705=CARTESIAN_POINT('Ctrl Pts',(-5.6954802334969,5.49400133508035,44.113312311247));
#48706=CARTESIAN_POINT('Ctrl Pts',(-5.83022375950345,5.35079370740464,44.1211985125965));
#48707=CARTESIAN_POINT('Ctrl Pts',(-5.95940427454596,5.20282823976762,44.129084713946));
#48708=CARTESIAN_POINT('Ctrl Pts',(-6.08862768864053,5.05481363485707,44.1369735341933));
#48709=CARTESIAN_POINT('Ctrl Pts',(-6.21228418432807,4.90203830134548,44.1448623544405));
#48710=CARTESIAN_POINT('Ctrl Pts',(-6.33002310350414,4.74496875744233,44.1527511746878));
#48711=CARTESIAN_POINT('Ctrl Pts',(-6.44787598308759,4.58774718471699,44.1606476305849));
#48712=CARTESIAN_POINT('Ctrl Pts',(-6.55979963871181,4.42622337539335,44.1685440864821));
#48713=CARTESIAN_POINT('Ctrl Pts',(-6.66548634053808,4.26089343261484,44.1764405423793));
#48714=CARTESIAN_POINT('Ctrl Pts',(-6.77123145551075,4.09547211181068,44.1843413626556));
#48715=CARTESIAN_POINT('Ctrl Pts',(-6.87073256935227,3.92624075975176,44.1922421829319));
#48716=CARTESIAN_POINT('Ctrl Pts',(-6.96372794869085,3.75372002906743,44.2001430032082));
#48717=CARTESIAN_POINT('Ctrl Pts',(-7.05683633000814,3.58098966233368,44.208053424051));
#48718=CARTESIAN_POINT('Ctrl Pts',(-7.14342303419475,3.40496224139899,44.2159638448938));
#48719=CARTESIAN_POINT('Ctrl Pts',(-7.22327404246507,3.22617933590962,44.2238742657366));
#48720=CARTESIAN_POINT('Ctrl Pts',(-7.25792622600135,3.14859461671368,44.2273070759269));
#48721=CARTESIAN_POINT('Ctrl Pts',(-7.29131056197855,3.07049119303736,44.2307398861171));
#48722=CARTESIAN_POINT('Ctrl Pts',(-7.32341248565942,2.99191419744746,44.2341726963074));
#48723=CARTESIAN_POINT('Ctrl Pts',(-7.40518696717657,2.79175195366992,44.2429172275151));
#48724=CARTESIAN_POINT('Ctrl Pts',(-7.4788016471458,2.58811213538503,44.2516617587229));
#48725=CARTESIAN_POINT('Ctrl Pts',(-7.54398366782736,2.38164468793185,44.2604062899307));
#48726=CARTESIAN_POINT('Ctrl Pts',(-7.60897890274335,2.17576889412544,44.2691257627874));
#48727=CARTESIAN_POINT('Ctrl Pts',(-7.66558964318761,1.96708185281294,44.2778452356441));
#48728=CARTESIAN_POINT('Ctrl Pts',(-7.71359248493486,1.75624940608001,44.2865647085008));
#48729=CARTESIAN_POINT('Ctrl Pts',(-7.76150465931262,1.54581517792442,44.2952677120894));
#48730=CARTESIAN_POINT('Ctrl Pts',(-7.80084132689146,1.33324384238952,44.3039707156781));
#48731=CARTESIAN_POINT('Ctrl Pts',(-7.83142878147297,1.11921590442453,44.3126737192668));
#48732=CARTESIAN_POINT('Ctrl Pts',(-7.86191715276629,0.905881276581177,
44.3213485308328));
#48733=CARTESIAN_POINT('Ctrl Pts',(-7.88371282848472,0.691099677687127,
44.3300233423988));
#48734=CARTESIAN_POINT('Ctrl Pts',(-7.89669319590675,0.475560269282509,
44.3386981539648));
#48735=CARTESIAN_POINT('Ctrl Pts',(-7.90615514801457,0.318444257588431,
44.3450215998977));
#48736=CARTESIAN_POINT('Ctrl Pts',(-7.91093403175593,0.160925906523633,
44.3513450458305));
#48737=CARTESIAN_POINT('Ctrl Pts',(-7.91099932156789,0.00327630163417495,
44.3576684917634));
#48738=CARTESIAN_POINT('',(-7.90417282333004,-0.00298459611092975,46.3576684917634));
#48739=CARTESIAN_POINT('Ctrl Pts',(-7.911,-9.02666830171484E-12,44.3576684917634));
#48740=CARTESIAN_POINT('Ctrl Pts',(-7.91099999999749,-2.20167589667567,
44.4462559274961));
#48741=CARTESIAN_POINT('Ctrl Pts',(-6.94214576671882,-4.38610418339452,
44.5348433632288));
#48742=CARTESIAN_POINT('Ctrl Pts',(-3.67820201487491,-7.34180684108027,
44.7120182346943));
#48743=CARTESIAN_POINT('Ctrl Pts',(-1.40868175870882,-8.08992666571483,
44.800605670427));
#48744=CARTESIAN_POINT('Ctrl Pts',(2.97309270522065,-7.65454228024946,44.9777805418924));
#48745=CARTESIAN_POINT('Ctrl Pts',(5.0510207267626,-6.47444880833709,45.0663679776252));
#48746=CARTESIAN_POINT('Ctrl Pts',(7.66951518848159,-2.93425195366947,45.2435428490906));
#48747=CARTESIAN_POINT('Ctrl Pts',(8.18956872247127,-0.601881960091208,
45.3321302848233));
#48748=CARTESIAN_POINT('Ctrl Pts',(7.32306689760989,3.71537198233139,45.5093051562888));
#48749=CARTESIAN_POINT('Ctrl Pts',(5.94329958849675,5.66643518937059,45.5978925920215));
#48750=CARTESIAN_POINT('Ctrl Pts',(2.16154501637136,7.92205913233188,45.7750674634869));
#48751=CARTESIAN_POINT('Ctrl Pts',(-0.210816529307585,8.20894963712981,
45.8636548992197));
#48752=CARTESIAN_POINT('Ctrl Pts',(-4.42123908577024,6.91982244717452,46.0408297706851));
#48753=CARTESIAN_POINT('Ctrl Pts',(-6.22631625634631,5.35390358803,46.1294172064178));
#48754=CARTESIAN_POINT('Ctrl Pts',(-7.65317280859711,2.3133485751382,46.2645592586882));
#48755=CARTESIAN_POINT('Ctrl Pts',(-7.91100000000129,1.15702837835713,46.3111138752258));
#48756=CARTESIAN_POINT('Ctrl Pts',(-7.911,-8.85624906743487E-12,46.3576684917634));
#48757=CARTESIAN_POINT('',(-7.91868218107619,-0.00107497954501803,48.3576177169414));
#48758=CARTESIAN_POINT('Ctrl Pts',(-7.90000441911832,-0.00480687251647904,
46.3576684917634));
#48759=CARTESIAN_POINT('Ctrl Pts',(-7.90593017288142,-0.869079961314315,
46.3923766291873));
#48760=CARTESIAN_POINT('Ctrl Pts',(-7.5759867787326,-3.05033090647266,46.4801233429855));
#48761=CARTESIAN_POINT('Ctrl Pts',(-5.56852494667735,-6.05216815598226,
46.6209086331589));
#48762=CARTESIAN_POINT('Ctrl Pts',(-0.809224834445862,-8.69093778987658,
46.8330629386561));
#48763=CARTESIAN_POINT('Ctrl Pts',(6.41510616868783,-6.81677508456639,47.0982558205292));
#48764=CARTESIAN_POINT('Ctrl Pts',(9.19981120649332,1.72383834166179,47.4164872787754));
#48765=CARTESIAN_POINT('Ctrl Pts',(3.5235845388455,8.66411051463959,47.7347187370226));
#48766=CARTESIAN_POINT('Ctrl Pts',(-5.25815706812825,7.6698522869705,48.0484059832181));
#48767=CARTESIAN_POINT('Ctrl Pts',(-7.9149434973087,2.51016233332767,48.2560160766646));
#48768=CARTESIAN_POINT('Ctrl Pts',(-7.92423877845688,-0.00105786062598127,
48.3575490173622));
#48769=CARTESIAN_POINT('',(-7.911,-8.51485548736264E-12,50.3576684917634));
#48770=CARTESIAN_POINT('Ctrl Pts',(-7.91099991958436,-0.00109864726889428,
48.3577126973937));
#48771=CARTESIAN_POINT('Ctrl Pts',(-7.91067767249818,-2.20240257181979,
48.4462853979163));
#48772=CARTESIAN_POINT('Ctrl Pts',(-6.94187431232755,-4.38635000211155,
48.5348580984389));
#48773=CARTESIAN_POINT('Ctrl Pts',(-3.67820201487496,-7.34180684108027,
48.7120182346943));
#48774=CARTESIAN_POINT('Ctrl Pts',(-1.40868175870879,-8.08992666571486,
48.800605670427));
#48775=CARTESIAN_POINT('Ctrl Pts',(2.97309270522083,-7.65454228024941,48.9777805418925));
#48776=CARTESIAN_POINT('Ctrl Pts',(5.05102072676283,-6.47444880833693,49.0663679776252));
#48777=CARTESIAN_POINT('Ctrl Pts',(7.66951518848176,-2.93425195366908,49.2435428490906));
#48778=CARTESIAN_POINT('Ctrl Pts',(8.18956872247132,-0.601881960090703,
49.3321302848234));
#48779=CARTESIAN_POINT('Ctrl Pts',(7.32306689760962,3.71537198233198,49.5093051562888));
#48780=CARTESIAN_POINT('Ctrl Pts',(5.94329958849625,5.66643518937114,49.5978925920215));
#48781=CARTESIAN_POINT('Ctrl Pts',(2.16154501637051,7.92205913233214,49.775067463487));
#48782=CARTESIAN_POINT('Ctrl Pts',(-0.21081652930856,8.2089496371298,49.8636548992197));
#48783=CARTESIAN_POINT('Ctrl Pts',(-4.42123908577119,6.91982244717394,50.0408297706851));
#48784=CARTESIAN_POINT('Ctrl Pts',(-6.22631625634712,5.3539035880291,50.1294172064179));
#48785=CARTESIAN_POINT('Ctrl Pts',(-7.65317280859725,2.31334857513749,50.2645592586882));
#48786=CARTESIAN_POINT('Ctrl Pts',(-7.91100000000124,1.15702837835694,50.3111138752258));
#48787=CARTESIAN_POINT('Ctrl Pts',(-7.911,-8.51485548736264E-12,50.3576684917634));
#48788=CARTESIAN_POINT('',(-7.90335554000322,-0.000571285354785519,52.3576684917634));
#48789=CARTESIAN_POINT('Ctrl Pts',(-7.911,-8.51485548736264E-12,50.3576684917634));
#48790=CARTESIAN_POINT('Ctrl Pts',(-7.91099999999763,-2.20167589667524,
50.4462559274961));
#48791=CARTESIAN_POINT('Ctrl Pts',(-6.94214576671903,-4.38610418339421,
50.5348433632288));
#48792=CARTESIAN_POINT('Ctrl Pts',(-3.67820201487512,-7.34180684108019,
50.7120182346943));
#48793=CARTESIAN_POINT('Ctrl Pts',(-1.40868175870896,-8.08992666571483,
50.800605670427));
#48794=CARTESIAN_POINT('Ctrl Pts',(2.97309270522067,-7.65454228024948,50.9777805418925));
#48795=CARTESIAN_POINT('Ctrl Pts',(5.05102072676269,-6.47444880833704,51.0663679776252));
#48796=CARTESIAN_POINT('Ctrl Pts',(7.66951518848169,-2.93425195366925,51.2435428490906));
#48797=CARTESIAN_POINT('Ctrl Pts',(8.18956872247131,-0.601881960090878,
51.3321302848233));
#48798=CARTESIAN_POINT('Ctrl Pts',(7.3230668976097,3.71537198233182,51.5093051562888));
#48799=CARTESIAN_POINT('Ctrl Pts',(5.94329958849637,5.66643518937101,51.5978925920215));
#48800=CARTESIAN_POINT('Ctrl Pts',(2.16154501637069,7.92205913233209,51.775067463487));
#48801=CARTESIAN_POINT('Ctrl Pts',(-0.210816529308383,8.20894963712981,
51.8636548992197));
#48802=CARTESIAN_POINT('Ctrl Pts',(-4.42123908577105,6.91982244717403,52.0408297706851));
#48803=CARTESIAN_POINT('Ctrl Pts',(-6.226316256347,5.35390358802923,52.1294172064179));
#48804=CARTESIAN_POINT('Ctrl Pts',(-7.65317280859717,2.31334857513772,52.2645592586882));
#48805=CARTESIAN_POINT('Ctrl Pts',(-7.91100000000119,1.15702837835726,52.3111138752258));
#48806=CARTESIAN_POINT('Ctrl Pts',(-7.911,-8.11961609059608E-12,52.3576684917634));
#48807=CARTESIAN_POINT('',(-7.91378807792777,-0.00677265886045676,54.3576684917634));
#48808=CARTESIAN_POINT('Ctrl Pts',(-7.89842547330135,-0.000939718817194635,
52.3576684917634));
#48809=CARTESIAN_POINT('Ctrl Pts',(-7.90062068210384,-1.25239052911004,
52.4078425314172));
#48810=CARTESIAN_POINT('Ctrl Pts',(-7.03041977659177,-5.14763933039878,
52.5640937238196));
#48811=CARTESIAN_POINT('Ctrl Pts',(-0.910171092806715,-9.31630818999036,
52.8264220689717));
#48812=CARTESIAN_POINT('Ctrl Pts',(5.95294509739285,-6.38354832108906,53.091614950844));
#48813=CARTESIAN_POINT('Ctrl Pts',(8.10656207347067,-1.3859512325431,53.3037692563418));
#48814=CARTESIAN_POINT('Ctrl Pts',(7.73558219899898,4.04326755765096,53.5159235618395));
#48815=CARTESIAN_POINT('Ctrl Pts',(2.23661238370502,9.08953105248759,53.781116443712));
#48816=CARTESIAN_POINT('Ctrl Pts',(-5.90135440155818,6.93085732631015,54.0793776124781));
#48817=CARTESIAN_POINT('Ctrl Pts',(-7.89488553833502,2.12997361947987,54.2715616284952));
#48818=CARTESIAN_POINT('Ctrl Pts',(-7.91378807792777,-0.00677265886045676,
54.3576684917634));
#48819=CARTESIAN_POINT('',(-7.91688330362235,0.00331809628778629,56.3576684917634));
#48820=CARTESIAN_POINT('Ctrl Pts',(-7.91378807792777,-0.00677265886045676,
54.3576684917634));
#48821=CARTESIAN_POINT('Ctrl Pts',(-7.91817203959193,-0.502336428179145,
54.3776387812441));
#48822=CARTESIAN_POINT('Ctrl Pts',(-7.64902003038262,-3.6253689198465,54.5036862234736));
#48823=CARTESIAN_POINT('Ctrl Pts',(-3.50021070610332,-8.68082195856808,
54.7358108184526));
#48824=CARTESIAN_POINT('Ctrl Pts',(5.42135646210964,-7.63091762632114,55.0540422766991));
#48825=CARTESIAN_POINT('Ctrl Pts',(8.68027656630637,-0.916538724054716,
55.3192351585718));
#48826=CARTESIAN_POINT('Ctrl Pts',(7.02947994193568,4.26891335306067,55.5313894640693));
#48827=CARTESIAN_POINT('Ctrl Pts',(3.18951819903458,8.12491342466588,55.7435437695676));
#48828=CARTESIAN_POINT('Ctrl Pts',(-4.27115340882762,8.32942124443492,56.0087366514396));
#48829=CARTESIAN_POINT('Ctrl Pts',(-7.79718755544591,3.13560819023932,56.2311244176299));
#48830=CARTESIAN_POINT('Ctrl Pts',(-7.92357763626265,0.256741869022418,
56.3474350310711));
#48831=CARTESIAN_POINT('Ctrl Pts',(-7.92188845760677,0.00332019403032202,
56.3576684917634));
#48832=CARTESIAN_POINT('',(-7.91099861016705,0.00331586588032432,58.3576684917633));
#48833=CARTESIAN_POINT('Ctrl Pts',(-7.9109993051824,0.0033156302070531,
56.3576684917634));
#48834=CARTESIAN_POINT('Ctrl Pts',(-7.91108018991349,-0.189673036065407,
56.3654723476325));
#48835=CARTESIAN_POINT('Ctrl Pts',(-7.90409495673348,-0.382940414989945,
56.3732762035016));
#48836=CARTESIAN_POINT('Ctrl Pts',(-7.89000870977794,-0.575919751031557,
56.3810800593707));
#48837=CARTESIAN_POINT('Ctrl Pts',(-7.87593671431612,-0.768703843882773,
56.3888760198363));
#48838=CARTESIAN_POINT('Ctrl Pts',(-7.85477803540268,-0.961200123166922,
56.3966719803019));
#48839=CARTESIAN_POINT('Ctrl Pts',(-7.82654975269139,-1.15283995795008,
56.4044679407676));
#48840=CARTESIAN_POINT('Ctrl Pts',(-7.79834443083918,-1.34432391306864,
56.4122575600062));
#48841=CARTESIAN_POINT('Ctrl Pts',(-7.76308100786333,-1.53495246175189,
56.4200471792447));
#48842=CARTESIAN_POINT('Ctrl Pts',(-7.72082851955789,-1.72416007713366,
56.4278367984833));
#48843=CARTESIAN_POINT('Ctrl Pts',(-7.67860202482051,-1.91325129271923,
56.4356216255782));
#48844=CARTESIAN_POINT('Ctrl Pts',(-7.62939510544607,-2.1009229707498,56.443406452673));
#48845=CARTESIAN_POINT('Ctrl Pts',(-7.57332824800153,-2.28661764359985,
56.4511912797678));
#48846=CARTESIAN_POINT('Ctrl Pts',(-7.51510904103691,-2.47944094570087,
56.4592749584414));
#48847=CARTESIAN_POINT('Ctrl Pts',(-7.44949282727851,-2.67013205625295,
56.467358637115));
#48848=CARTESIAN_POINT('Ctrl Pts',(-7.37667233441845,-2.85808087195332,
56.4754423157885));
#48849=CARTESIAN_POINT('Ctrl Pts',(-7.30657826779504,-3.03899281434856,
56.4832233385371));
#48850=CARTESIAN_POINT('Ctrl Pts',(-7.22980973278331,-3.21736372312977,
56.4910043612857));
#48851=CARTESIAN_POINT('Ctrl Pts',(-7.14658865764285,-3.39266732210079,
56.4987853840343));
#48852=CARTESIAN_POINT('Ctrl Pts',(-7.06336557376309,-3.56797515244263,
56.5065665945964));
#48853=CARTESIAN_POINT('Ctrl Pts',(-6.97368979141322,-3.740215204408,56.5143478051585));
#48854=CARTESIAN_POINT('Ctrl Pts',(-6.87783030434885,-3.90888363917125,
56.5221290157207));
#48855=CARTESIAN_POINT('Ctrl Pts',(-6.78195130289631,-4.07758641024703,
56.529911810326));
#48856=CARTESIAN_POINT('Ctrl Pts',(-6.6798862651892,-4.2427158073662,56.5376946049312));
#48857=CARTESIAN_POINT('Ctrl Pts',(-6.57194887027541,-4.4037948460942,56.5454773995365));
#48858=CARTESIAN_POINT('Ctrl Pts',(-6.46397013174474,-4.56493558345842,
56.5532631752113));
#48859=CARTESIAN_POINT('Ctrl Pts',(-6.35011475401019,-4.72202257807922,
56.5610489508861));
#48860=CARTESIAN_POINT('Ctrl Pts',(-6.23073829652345,-4.87460985928475,
56.5688347265609));
#48861=CARTESIAN_POINT('Ctrl Pts',(-6.11123756686666,-5.0273559854833,56.5766286073115));
#48862=CARTESIAN_POINT('Ctrl Pts',(-5.9862044999284,-5.1755927654553,56.5844224880622));
#48863=CARTESIAN_POINT('Ctrl Pts',(-5.85603390862543,-5.31890852158873,
56.5922163688128));
#48864=CARTESIAN_POINT('Ctrl Pts',(-5.72578300336415,-5.46231270211623,
56.6000150583102));
#48865=CARTESIAN_POINT('Ctrl Pts',(-5.59038850528388,-5.60078955638088,
56.6078137478076));
#48866=CARTESIAN_POINT('Ctrl Pts',(-5.45028024240838,-5.7339660165729,56.615612437305));
#48867=CARTESIAN_POINT('Ctrl Pts',(-5.30999619300789,-5.86730956631885,
56.6234209114111));
#48868=CARTESIAN_POINT('Ctrl Pts',(-5.16498683685651,-5.9953392122672,56.6312293855172));
#48869=CARTESIAN_POINT('Ctrl Pts',(-5.01571372673485,-6.11772317218127,
56.6390378596233));
#48870=CARTESIAN_POINT('Ctrl Pts',(-4.97644965923604,-6.14991444935719,
56.6410917623933));
#48871=CARTESIAN_POINT('Ctrl Pts',(-4.93689074131798,-6.18171535351921,
56.6431456651633));
#48872=CARTESIAN_POINT('Ctrl Pts',(-4.89704567766127,-6.21312036185515,
56.6451995679333));
#48873=CARTESIAN_POINT('Ctrl Pts',(-4.74359679161102,-6.33406542012052,
56.6531094333768));
#48874=CARTESIAN_POINT('Ctrl Pts',(-4.58545758517985,-6.449485602999,56.6610192988203));
#48875=CARTESIAN_POINT('Ctrl Pts',(-4.42306262451535,-6.55899672355577,
56.6689291642637));
#48876=CARTESIAN_POINT('Ctrl Pts',(-4.26084415346442,-6.66838882825596,
56.6768304333253));
#48877=CARTESIAN_POINT('Ctrl Pts',(-4.09437942407764,-6.77188447093364,
56.6847317023869));
#48878=CARTESIAN_POINT('Ctrl Pts',(-3.92413646662417,-6.86913924675504,
56.6926329714486));
#48879=CARTESIAN_POINT('Ctrl Pts',(-3.75404689270852,-6.96630639908934,
56.7005271217158));
#48880=CARTESIAN_POINT('Ctrl Pts',(-3.58018616951,-7.05724371560999,56.7084212719831));
#48881=CARTESIAN_POINT('Ctrl Pts',(-3.40305196903901,-7.14164955007033,
56.7163154222503));
#48882=CARTESIAN_POINT('Ctrl Pts',(-3.22604445540244,-7.22599501726141,
56.7242039266011));
#48883=CARTESIAN_POINT('Ctrl Pts',(-3.04576843906962,-7.30381816143088,
56.7320924309518));
#48884=CARTESIAN_POINT('Ctrl Pts',(-2.862747145676,-7.37486269566586,56.7399809353026));
#48885=CARTESIAN_POINT('Ctrl Pts',(-2.67982275809595,-7.44586961335764,
56.747865262861));
#48886=CARTESIAN_POINT('Ctrl Pts',(-2.49415631067576,-7.5101049483499,56.7557495904194));
#48887=CARTESIAN_POINT('Ctrl Pts',(-2.30629226597316,-7.56735997451637,
56.7636339179779));
#48888=CARTESIAN_POINT('Ctrl Pts',(-2.11849280600797,-7.62459531729512,
56.7715155350271));
#48889=CARTESIAN_POINT('Ctrl Pts',(-1.92849758407093,-7.67485503349543,
56.7793971520763));
#48890=CARTESIAN_POINT('Ctrl Pts',(-1.73686779353118,-7.71797974004818,
56.7872787691255));
#48891=CARTESIAN_POINT('Ctrl Pts',(-1.54523538554448,-7.76110503563581,
56.7951604938287));
#48892=CARTESIAN_POINT('Ctrl Pts',(-1.35196869898921,-7.79709504277689,
56.8030422185319));
#48893=CARTESIAN_POINT('Ctrl Pts',(-1.15764129969557,-7.82584101686452,
56.8109239432351));
#48894=CARTESIAN_POINT('Ctrl Pts',(-0.96330212609917,-7.85458873267156,
56.8188061454923));
#48895=CARTESIAN_POINT('Ctrl Pts',(-0.767902453074723,-7.87609148971396,
56.8266883477494));
#48896=CARTESIAN_POINT('Ctrl Pts',(-0.572023223356488,-7.89029216391515,
56.8345705500066));
#48897=CARTESIAN_POINT('Ctrl Pts',(-0.376099164647193,-7.90449608808776,
56.8424545561874));
#48898=CARTESIAN_POINT('Ctrl Pts',(-0.179695674738636,-7.91139457442694,
56.8503385623682));
#48899=CARTESIAN_POINT('Ctrl Pts',(0.0166037853955017,-7.910982575781,56.8582225685489));
#48900=CARTESIAN_POINT('Ctrl Pts',(0.212981202500519,-7.91057041351684,
56.8661097057279));
#48901=CARTESIAN_POINT('Ctrl Pts',(0.409254162712939,-7.9028419820523,56.8739968429068));
#48902=CARTESIAN_POINT('Ctrl Pts',(0.60484156639343,-7.88784429863843,56.8818839800857));
#48903=CARTESIAN_POINT('Ctrl Pts',(0.800637741703501,-7.87283060657191,
56.8897795360607));
#48904=CARTESIAN_POINT('Ctrl Pts',(0.995746554669449,-7.85053219041334,
56.8976750920358));
#48905=CARTESIAN_POINT('Ctrl Pts',(1.18959326027058,-7.82104781184202,56.9055706480108));
#48906=CARTESIAN_POINT('Ctrl Pts',(1.38355806995182,-7.79154546946059,56.9134710144745));
#48907=CARTESIAN_POINT('Ctrl Pts',(1.57625890119976,-7.75484850062344,56.9213713809383));
#48908=CARTESIAN_POINT('Ctrl Pts',(1.76713324526486,-7.71110634691804,56.929271747402));
#48909=CARTESIAN_POINT('Ctrl Pts',(1.95825620051916,-7.66730721966335,56.9371824039836));
#48910=CARTESIAN_POINT('Ctrl Pts',(2.14754758453539,-7.6164446677572,56.9450930605651));
#48911=CARTESIAN_POINT('Ctrl Pts',(2.33446093623429,-7.55871769132808,56.9530037171467));
#48912=CARTESIAN_POINT('Ctrl Pts',(2.41658657947439,-7.5333537190465,56.9564794868245));
#48913=CARTESIAN_POINT('Ctrl Pts',(2.49825340183972,-7.50666517179851,56.9599552565024));
#48914=CARTESIAN_POINT('Ctrl Pts',(2.57941640384201,-7.47867180825518,56.9634310261802));
#48915=CARTESIAN_POINT('Ctrl Pts',(2.76246156522894,-7.41553898146043,56.9712698542906));
#48916=CARTESIAN_POINT('Ctrl Pts',(2.94346399646625,-7.34558651675808,56.979108682401));
#48917=CARTESIAN_POINT('Ctrl Pts',(3.12187231452425,-7.26896376740227,56.9869475105114));
#48918=CARTESIAN_POINT('Ctrl Pts',(3.30008063962085,-7.19242691096178,56.9947775514169));
#48919=CARTESIAN_POINT('Ctrl Pts',(3.47570032209801,-7.10923479600866,57.0026075923224));
#48920=CARTESIAN_POINT('Ctrl Pts',(3.64819472148541,-7.01958661703992,57.0104376332279));
#48921=CARTESIAN_POINT('Ctrl Pts',(3.82052932948186,-6.93002148428756,57.0182604207203));
#48922=CARTESIAN_POINT('Ctrl Pts',(3.98974411005337,-6.83401235865384,57.0260832082128));
#48923=CARTESIAN_POINT('Ctrl Pts',(4.1553218400315,-6.73180669699875,57.0339059957052));
#48924=CARTESIAN_POINT('Ctrl Pts',(4.32077839457395,-6.62967583293619,57.0417230582147));
#48925=CARTESIAN_POINT('Ctrl Pts',(4.48260290197556,-6.52135764885481,57.0495401207242));
#48926=CARTESIAN_POINT('Ctrl Pts',(4.64030205779981,-6.40714583979317,57.0573571832337));
#48927=CARTESIAN_POINT('Ctrl Pts',(4.79791646883156,-6.29299540617776,57.0651700449893));
#48928=CARTESIAN_POINT('Ctrl Pts',(4.95140966024248,-6.17295786235636,57.0729829067449));
#48929=CARTESIAN_POINT('Ctrl Pts',(5.10031653177235,-6.04737069111277,57.0807957685006));
#48930=CARTESIAN_POINT('Ctrl Pts',(5.24917233135645,-5.92182659364496,57.0886059506078));
#48931=CARTESIAN_POINT('Ctrl Pts',(5.39344467663459,-5.79073688768173,57.0964161327151));
#48932=CARTESIAN_POINT('Ctrl Pts',(5.53270070042722,-5.65447999019293,57.1042263148224));
#48933=CARTESIAN_POINT('Ctrl Pts',(5.67196300475582,-5.51821694743067,57.1120368491738));
#48934=CARTESIAN_POINT('Ctrl Pts',(5.80620827769993,-5.37678648696057,57.1198473835253));
#48935=CARTESIAN_POINT('Ctrl Pts',(5.93503939241925,-5.23060497556752,57.1276579178768));
#48936=CARTESIAN_POINT('Ctrl Pts',(6.06388083307358,-5.08441174758886,57.13546907825));
#48937=CARTESIAN_POINT('Ctrl Pts',(6.18730701767793,-4.93346697367534,57.1432802386232));
#48938=CARTESIAN_POINT('Ctrl Pts',(6.30496018621139,-4.77822122240999,57.1510913989963));
#48939=CARTESIAN_POINT('Ctrl Pts',(6.42264350580237,-4.62293568621037,57.1589045611409));
#48940=CARTESIAN_POINT('Ctrl Pts',(6.53455064947415,-4.4633472573478,57.1667177232854));
#48941=CARTESIAN_POINT('Ctrl Pts',(6.64036629668823,-4.29993679555956,57.17453088543));
#48942=CARTESIAN_POINT('Ctrl Pts',(6.74622769922347,-4.13645567410656,57.1823474260327));
#48943=CARTESIAN_POINT('Ctrl Pts',(6.84599216719703,-3.969149522604,57.1901639666355));
#48944=CARTESIAN_POINT('Ctrl Pts',(6.93938949391331,-3.79852529960846,57.1979805072383));
#48945=CARTESIAN_POINT('Ctrl Pts',(7.03289581700968,-3.62770195503938,57.2058061698862));
#48946=CARTESIAN_POINT('Ctrl Pts',(7.12001998885442,-3.45355311365304,57.2136318325341));
#48947=CARTESIAN_POINT('Ctrl Pts',(7.20053880696445,-3.27660829050392,57.221457495182));
#48948=CARTESIAN_POINT('Ctrl Pts',(7.28111010982523,-3.09954812903815,57.2292882588481));
#48949=CARTESIAN_POINT('Ctrl Pts',(7.35506734541584,-2.91968867812484,57.2371190225142));
#48950=CARTESIAN_POINT('Ctrl Pts',(7.42223665583889,-2.73757630482174,57.2449497861802));
#48951=CARTESIAN_POINT('Ctrl Pts',(7.48950301885456,-2.55520079828319,57.2527918644766));
#48952=CARTESIAN_POINT('Ctrl Pts',(7.54996175821235,-2.3705662006234,57.260633942773));
#48953=CARTESIAN_POINT('Ctrl Pts',(7.60348944494689,-2.18423196125806,57.2684760210694));
#48954=CARTESIAN_POINT('Ctrl Pts',(7.63349173316116,-2.07979155116989,57.2728715088552));
#48955=CARTESIAN_POINT('Ctrl Pts',(7.66131748299645,-1.97481734345205,57.2772669966411));
#48956=CARTESIAN_POINT('Ctrl Pts',(7.68695207033227,-1.86940869485901,57.281662484427));
#48957=CARTESIAN_POINT('Ctrl Pts',(7.73312142302325,-1.67956171156966,57.2895790084254));
#48958=CARTESIAN_POINT('Ctrl Pts',(7.77231871117484,-1.48773533706874,57.2974955324239));
#48959=CARTESIAN_POINT('Ctrl Pts',(7.80437265176402,-1.29448387877096,57.3054120564223));
#48960=CARTESIAN_POINT('Ctrl Pts',(7.83638966426137,-1.10145505792322,57.313319460103));
#48961=CARTESIAN_POINT('Ctrl Pts',(7.86127966514113,-0.90700475994466,57.3212268637836));
#48962=CARTESIAN_POINT('Ctrl Pts',(7.87892137472227,-0.711701461951944,
57.3291342674642));
#48963=CARTESIAN_POINT('Ctrl Pts',(7.89654602907775,-0.516586974561875,
57.3370340266162));
#48964=CARTESIAN_POINT('Ctrl Pts',(7.9069363203028,-0.32062147063296,57.3449337857683));
#48965=CARTESIAN_POINT('Ctrl Pts',(7.9100221172548,-0.124382894884864,57.3528335449203));
#48966=CARTESIAN_POINT('Ctrl Pts',(7.9131055026071,0.0717023172764458,57.3607271302841));
#48967=CARTESIAN_POINT('Ctrl Pts',(7.908895761514,0.268059833174569,57.3686207156479));
#48968=CARTESIAN_POINT('Ctrl Pts',(7.89737460578694,0.464107030620674,57.3765143010118));
#48969=CARTESIAN_POINT('Ctrl Pts',(7.8858603203938,0.660037320549568,57.3844031792465));
#48970=CARTESIAN_POINT('Ctrl Pts',(7.8670433281466,0.855657317763265,57.3922920574812));
#48971=CARTESIAN_POINT('Ctrl Pts',(7.84095742123833,1.05038455735388,57.400180935716));
#48972=CARTESIAN_POINT('Ctrl Pts',(7.81488223994292,1.24503173191201,57.4080665703198));
#48973=CARTESIAN_POINT('Ctrl Pts',(7.78154414606342,1.43878653940533,57.4159522049237));
#48974=CARTESIAN_POINT('Ctrl Pts',(7.74102879056715,1.6310715078164,57.4238378395275));
#48975=CARTESIAN_POINT('Ctrl Pts',(7.70051703917778,1.82333937121696,57.4317227726523));
#48976=CARTESIAN_POINT('Ctrl Pts',(7.65282936290027,2.01413731767258,57.4396077057772));
#48977=CARTESIAN_POINT('Ctrl Pts',(7.59810265271002,2.20289742813436,57.4474926389021));
#48978=CARTESIAN_POINT('Ctrl Pts',(7.54337613226107,2.39165688415176,57.4553775446893));
#48979=CARTESIAN_POINT('Ctrl Pts',(7.4816107219699,2.57837818700974,57.4632624504765));
#48980=CARTESIAN_POINT('Ctrl Pts',(7.41299341303602,2.76250785669192,57.4711473562638));
#48981=CARTESIAN_POINT('Ctrl Pts',(7.34436482965015,2.94666778056437,57.4790335576132));
#48982=CARTESIAN_POINT('Ctrl Pts',(7.26888222472407,3.12823489977492,57.4869197589627));
#48983=CARTESIAN_POINT('Ctrl Pts',(7.18678111885874,3.30667478739828,57.4948059603121));
#48984=CARTESIAN_POINT('Ctrl Pts',(7.10465274835829,3.48517393242599,57.5026947805594));
#48985=CARTESIAN_POINT('Ctrl Pts',(7.01590164162071,3.66054346372422,57.5105836008065));
#48986=CARTESIAN_POINT('Ctrl Pts',(6.9208098424507,3.83227244916611,57.5184724210538));
#48987=CARTESIAN_POINT('Ctrl Pts',(6.82562600319492,4.00416765241737,57.5263688769509));
#48988=CARTESIAN_POINT('Ctrl Pts',(6.72408937990399,4.17241496977283,57.5342653328481));
#48989=CARTESIAN_POINT('Ctrl Pts',(6.61652658460578,4.33653052049735,57.5421617887453));
#48990=CARTESIAN_POINT('Ctrl Pts',(6.50890433924238,4.50073677805189,57.5500626090216));
#48991=CARTESIAN_POINT('Ctrl Pts',(6.39524948026097,4.66080643540534,57.5579634292978));
#48992=CARTESIAN_POINT('Ctrl Pts',(6.27592985017476,4.81628752419178,57.5658642495741));
#48993=CARTESIAN_POINT('Ctrl Pts',(6.15646523058092,4.9719575435548,57.5737746704169));
#48994=CARTESIAN_POINT('Ctrl Pts',(6.03132230951853,5.12302759211004,57.5816850912596));
#48995=CARTESIAN_POINT('Ctrl Pts',(5.90090754944437,5.26908066866607,57.5895955121024));
#48996=CARTESIAN_POINT('Ctrl Pts',(5.84431269485101,5.33246193491155,57.5930283222929));
#48997=CARTESIAN_POINT('Ctrl Pts',(5.78672549096251,5.39489888412984,57.5964611324833));
#48998=CARTESIAN_POINT('Ctrl Pts',(5.72818115022042,5.45635974897729,57.5998939426738));
#48999=CARTESIAN_POINT('Ctrl Pts',(5.58638076990835,5.60522424893074,57.6082085600112));
#49000=CARTESIAN_POINT('Ctrl Pts',(5.43865226372989,5.7486861063339,57.6165231773487));
#49001=CARTESIAN_POINT('Ctrl Pts',(5.285423566284,5.88627375552393,57.6248377946862));
#49002=CARTESIAN_POINT('Ctrl Pts',(5.13238425182783,6.0236913532759,57.6331421355734));
#49003=CARTESIAN_POINT('Ctrl Pts',(4.97385852141849,6.15524902792256,57.6414464764606));
#49004=CARTESIAN_POINT('Ctrl Pts',(4.81031173073891,6.28051128914801,57.6497508173479));
#49005=CARTESIAN_POINT('Ctrl Pts',(4.64695626472553,6.40562701273603,57.6580454434296));
#49006=CARTESIAN_POINT('Ctrl Pts',(4.47859168602644,6.52446183427147,57.6663400695114));
#49007=CARTESIAN_POINT('Ctrl Pts',(4.30571770233826,6.63661932521152,57.6746346955932));
#49008=CARTESIAN_POINT('Ctrl Pts',(4.13310401412025,6.74860794119297,57.6829168324991));
#49009=CARTESIAN_POINT('Ctrl Pts',(3.95599471622409,6.85393913170547,57.6911989694049));
#49010=CARTESIAN_POINT('Ctrl Pts',(3.77491991420195,6.95225867192537,57.6994811063108));
#49011=CARTESIAN_POINT('Ctrl Pts',(3.59401209849676,7.05048754233522,57.7077556054696));
#49012=CARTESIAN_POINT('Ctrl Pts',(3.40914632805054,7.14171751741097,57.7160301046284));
#49013=CARTESIAN_POINT('Ctrl Pts',(3.22088038120729,7.22563841954149,57.7243046037872));
#49014=CARTESIAN_POINT('Ctrl Pts',(3.03283096999261,7.30946279935558,57.7325695859627));
#49015=CARTESIAN_POINT('Ctrl Pts',(2.84138945325158,7.38599476194414,57.7408345681381));
#49016=CARTESIAN_POINT('Ctrl Pts',(2.64713707734078,7.45497057631804,57.7490995503136));
#49017=CARTESIAN_POINT('Ctrl Pts',(2.56949768248666,7.48253904472132,57.7524029241415));
#49018=CARTESIAN_POINT('Ctrl Pts',(2.49140952558729,7.50890096427389,57.7557062979693));
#49019=CARTESIAN_POINT('Ctrl Pts',(2.41291071232974,7.53404160423371,57.7590096717972));
#49020=CARTESIAN_POINT('Ctrl Pts',(2.21648177341447,7.59695146268921,57.7672757612948));
#49021=CARTESIAN_POINT('Ctrl Pts',(2.01770248929773,7.65213956951669,57.7755418507925));
#49022=CARTESIAN_POINT('Ctrl Pts',(1.81719592044119,7.69946231802792,57.7838079402902));
#49023=CARTESIAN_POINT('Ctrl Pts',(1.61650903574976,7.74682762395239,57.7920814634935));
#49024=CARTESIAN_POINT('Ctrl Pts',(1.41409205108396,7.78631338306703,57.8003549866969));
#49025=CARTESIAN_POINT('Ctrl Pts',(1.21057718538857,7.81782731186976,57.8086285099003));
#49026=CARTESIAN_POINT('Ctrl Pts',(1.00686606113847,7.84937163097394,57.8169100116349));
#49027=CARTESIAN_POINT('Ctrl Pts',(0.802055232110211,7.87292872709926,57.8251915133695));
#49028=CARTESIAN_POINT('Ctrl Pts',(0.596781820702515,7.88845818005515,57.8334730151041));
#49029=CARTESIAN_POINT('Ctrl Pts',(0.391166633492497,7.90401348921525,57.8417683053604));
#49030=CARTESIAN_POINT('Ctrl Pts',(0.185087617456562,7.91151441118359,57.8500635956168));
#49031=CARTESIAN_POINT('Ctrl Pts',(-0.0208162702095703,7.91097261295314,
57.8583588858731));
#49032=CARTESIAN_POINT('Ctrl Pts',(-0.226906893306216,7.91043032336272,
57.8666616991764));
#49033=CARTESIAN_POINT('Ctrl Pts',(-0.432821777805041,7.90183076150704,
57.8749645124796));
#49034=CARTESIAN_POINT('Ctrl Pts',(-0.637925996679285,7.88523756286142,
57.8832673257828));
#49035=CARTESIAN_POINT('Ctrl Pts',(-0.843344746839667,7.86861891822478,
57.8915828716108));
#49036=CARTESIAN_POINT('Ctrl Pts',(-1.04795005433127,7.84398216412009,57.8998984174388));
#49037=CARTESIAN_POINT('Ctrl Pts',(-1.25111422146588,7.81144251754091,57.9082139632668));
#49038=CARTESIAN_POINT('Ctrl Pts',(-1.33183247366865,7.79851433519354,57.9115177758181));
#49039=CARTESIAN_POINT('Ctrl Pts',(-1.4123233755187,7.7843392299535,57.9148215883693));
#49040=CARTESIAN_POINT('Ctrl Pts',(-1.49254815857286,7.76892663077344,57.9181254009206));
#49041=CARTESIAN_POINT('Ctrl Pts',(-1.68461541594747,7.7320271149277,57.9260351040254));
#49042=CARTESIAN_POINT('Ctrl Pts',(-1.87555687338099,7.68795403783527,57.9339448071301));
#49043=CARTESIAN_POINT('Ctrl Pts',(-2.06479726327526,7.63678815088981,57.9418545102349));
#49044=CARTESIAN_POINT('Ctrl Pts',(-2.25384565956987,7.58567417423063,57.9497561885603));
#49045=CARTESIAN_POINT('Ctrl Pts',(-2.44119609606983,7.52748181085078,57.9576578668857));
#49046=CARTESIAN_POINT('Ctrl Pts',(-2.62628186223298,7.46234310254534,57.9655595452111));
#49047=CARTESIAN_POINT('Ctrl Pts',(-2.81121413740715,7.39725841354656,57.9734546707019));
#49048=CARTESIAN_POINT('Ctrl Pts',(-2.99388516044192,7.32523896940155,57.9813497961927));
#49049=CARTESIAN_POINT('Ctrl Pts',(-3.17374151740871,7.24646712410098,57.9892449216835));
#49050=CARTESIAN_POINT('Ctrl Pts',(-3.35348202981113,7.16774601534515,57.9971349619641));
#49051=CARTESIAN_POINT('Ctrl Pts',(-3.53041117367976,7.08228130859005,58.0050250022447));
#49052=CARTESIAN_POINT('Ctrl Pts',(-3.70399345783124,6.99030424690824,58.0129150425254));
#49053=CARTESIAN_POINT('Ctrl Pts',(-3.87749607988108,6.89836939625086,58.0208014618305));
#49054=CARTESIAN_POINT('Ctrl Pts',(-4.04765459908768,6.79992830735376,58.0286878811357));
#49055=CARTESIAN_POINT('Ctrl Pts',(-4.21395591786019,6.69525925729028,58.0365743004408));
#49056=CARTESIAN_POINT('Ctrl Pts',(-4.38021170470164,6.59061886475041,58.0444585605094));
#49057=CARTESIAN_POINT('Ctrl Pts',(-4.5426121046703,6.47975409309515,58.0523428205779));
#49058=CARTESIAN_POINT('Ctrl Pts',(-4.70067068893039,6.36298798319082,58.0602270806464));
#49059=CARTESIAN_POINT('Ctrl Pts',(-4.85874772644488,6.24620824090617,58.0681122611981));
#49060=CARTESIAN_POINT('Ctrl Pts',(-5.01248165408357,6.12352598296695,58.0759974417497));
#49061=CARTESIAN_POINT('Ctrl Pts',(-5.16141647512,5.99530657851288,58.0838826223013));
#49062=CARTESIAN_POINT('Ctrl Pts',(-5.31036987272421,5.86707118131486,58.0917687863677));
#49063=CARTESIAN_POINT('Ctrl Pts',(-5.45452270916307,5.73329748584274,58.0996549504341));
#49064=CARTESIAN_POINT('Ctrl Pts',(-5.59345346139795,5.59438999133733,58.1075411145005));
#49065=CARTESIAN_POINT('Ctrl Pts',(-5.73242485256491,5.45544186470301,58.1154295853656));
#49066=CARTESIAN_POINT('Ctrl Pts',(-5.86617087174895,5.31135719017599,58.1233180562307));
#49067=CARTESIAN_POINT('Ctrl Pts',(-5.99430796580337,5.16257619906053,58.1312065270958));
#49068=CARTESIAN_POINT('Ctrl Pts',(-6.12250404117033,5.01372672427763,58.1390986290123));
#49069=CARTESIAN_POINT('Ctrl Pts',(-6.24508582190272,4.86017688609706,58.1469907309287));
#49070=CARTESIAN_POINT('Ctrl Pts',(-6.36171087831312,4.70239893041335,58.1548828328452));
#49071=CARTESIAN_POINT('Ctrl Pts',(-6.47847113835094,4.54443806247567,58.1627840840889));
#49072=CARTESIAN_POINT('Ctrl Pts',(-6.58926067549652,4.38223956342015,58.1706853353326));
#49073=CARTESIAN_POINT('Ctrl Pts',(-6.69378050152099,4.21630449534393,58.1785865865763));
#49074=CARTESIAN_POINT('Ctrl Pts',(-6.79836958543951,4.05025947383781,58.1864930734202));
#49075=CARTESIAN_POINT('Ctrl Pts',(-6.89668050385122,3.88047324462845,58.1943995602641));
#49076=CARTESIAN_POINT('Ctrl Pts',(-6.9884607543749,3.70747046981656,58.202306047108));
#49077=CARTESIAN_POINT('Ctrl Pts',(-7.08036744742426,3.53422935497321,58.2102234264496));
#49078=CARTESIAN_POINT('Ctrl Pts',(-7.16572535208359,3.35776315241992,58.2181408057912));
#49079=CARTESIAN_POINT('Ctrl Pts',(-7.24433005307879,3.17861653586264,58.2260581851327));
#49080=CARTESIAN_POINT('Ctrl Pts',(-7.2784122141163,3.10094047123132,58.2294910764776));
#49081=CARTESIAN_POINT('Ctrl Pts',(-7.31122540923108,3.02276068703856,58.2329239678225));
#49082=CARTESIAN_POINT('Ctrl Pts',(-7.34275591312242,2.9441223820191,58.2363568591674));
#49083=CARTESIAN_POINT('Ctrl Pts',(-7.42407168264268,2.74131768506709,58.2452101335189));
#49084=CARTESIAN_POINT('Ctrl Pts',(-7.49705846057189,2.53495023216138,58.2540634078704));
#49085=CARTESIAN_POINT('Ctrl Pts',(-7.56142423142031,2.32567938299537,58.2629166822218));
#49086=CARTESIAN_POINT('Ctrl Pts',(-7.62548007002129,2.11741620892984,58.2717273265359));
#49087=CARTESIAN_POINT('Ctrl Pts',(-7.68099762436967,1.90627770533604,58.28053797085));
#49088=CARTESIAN_POINT('Ctrl Pts',(-7.72773460272532,1.6929379521535,58.2893486151641));
#49089=CARTESIAN_POINT('Ctrl Pts',(-7.77432731373501,1.48025673448315,58.2981320628489));
#49090=CARTESIAN_POINT('Ctrl Pts',(-7.81219346255932,1.26538800816939,58.3069155105338));
#49091=CARTESIAN_POINT('Ctrl Pts',(-7.84113994178214,1.04902116918052,58.3156989582187));
#49092=CARTESIAN_POINT('Ctrl Pts',(-7.86993795650493,0.833764060819869,
58.3244373562048));
#49093=CARTESIAN_POINT('Ctrl Pts',(-7.88990747454002,0.617024352549807,
58.3331757541909));
#49094=CARTESIAN_POINT('Ctrl Pts',(-7.90090634659527,0.399499564869185,
58.341914152177));
#49095=CARTESIAN_POINT('Ctrl Pts',(-7.90751625250328,0.268775398608426,
58.3471655987057));
#49096=CARTESIAN_POINT('Ctrl Pts',(-7.91088728971183,0.137768043901693,
58.3524170452345));
#49097=CARTESIAN_POINT('Ctrl Pts',(-7.91099722033409,0.00663173176848126,
58.3576684917633));
#49098=CARTESIAN_POINT('',(-7.91099844885794,-0.00350301049124394,60.3576684917633));
#49099=CARTESIAN_POINT('Ctrl Pts',(-7.911,-7.83262343873048E-12,58.3576684917633));
#49100=CARTESIAN_POINT('Ctrl Pts',(-7.91099999999782,-2.20167589667448,
58.4462559274961));
#49101=CARTESIAN_POINT('Ctrl Pts',(-6.94214576671948,-4.38610418339347,
58.5348433632288));
#49102=CARTESIAN_POINT('Ctrl Pts',(-3.67820201487602,-7.34180684107971,
58.7120182346942));
#49103=CARTESIAN_POINT('Ctrl Pts',(-1.40868175871005,-8.08992666571462,
58.800605670427));
#49104=CARTESIAN_POINT('Ctrl Pts',(2.9730927052195,-7.65454228024991,58.9777805418924));
#49105=CARTESIAN_POINT('Ctrl Pts',(5.05102072676162,-6.47444880833785,59.0663679776251));
#49106=CARTESIAN_POINT('Ctrl Pts',(7.66951518848115,-2.93425195367063,59.2435428490906));
#49107=CARTESIAN_POINT('Ctrl Pts',(8.18956872247118,-0.601881960092444,
59.3321302848233));
#49108=CARTESIAN_POINT('Ctrl Pts',(7.32306689761046,3.71537198233028,59.5093051562887));
#49109=CARTESIAN_POINT('Ctrl Pts',(5.9432995884976,5.66643518936969,59.5978925920214));
#49110=CARTESIAN_POINT('Ctrl Pts',(2.16154501637256,7.92205913233156,59.7750674634869));
#49111=CARTESIAN_POINT('Ctrl Pts',(-0.210816529306346,8.20894963712984,
59.8636548992196));
#49112=CARTESIAN_POINT('Ctrl Pts',(-4.4212390857692,6.91982244717519,60.0408297706851));
#49113=CARTESIAN_POINT('Ctrl Pts',(-6.22631625634551,5.35390358803094,60.1294172064178));
#49114=CARTESIAN_POINT('Ctrl Pts',(-7.65317280859673,2.31334857513943,60.2645592586881));
#49115=CARTESIAN_POINT('Ctrl Pts',(-7.91100000000109,1.15702837835847,60.3111138752257));
#49116=CARTESIAN_POINT('Ctrl Pts',(-7.911,-7.43738404196392E-12,60.3576684917633));
#49117=CARTESIAN_POINT('',(-7.91099999260072,-0.000333258038948825,62.3576819008605));
#49118=CARTESIAN_POINT('Ctrl Pts',(-7.91099689771587,-0.0070060209750505,
60.3576684917633));
#49119=CARTESIAN_POINT('Ctrl Pts',(-7.91078925208212,-0.241473484075867,
60.3670821951403));
#49120=CARTESIAN_POINT('Ctrl Pts',(-7.90015416056753,-0.475476672476813,
60.3764958985172));
#49121=CARTESIAN_POINT('Ctrl Pts',(-7.87923780643971,-0.708189656498227,
60.3859096018942));
#49122=CARTESIAN_POINT('Ctrl Pts',(-7.85816685921297,-0.942622625806779,
60.3953928820993));
#49123=CARTESIAN_POINT('Ctrl Pts',(-7.82666220554321,-1.17574623517179,
60.4048761623045));
#49124=CARTESIAN_POINT('Ctrl Pts',(-7.78492189767097,-1.40673808762081,
60.4143594425097));
#49125=CARTESIAN_POINT('Ctrl Pts',(-7.74280977313407,-1.63978758229913,
60.4239271984122));
#49126=CARTESIAN_POINT('Ctrl Pts',(-7.69027887464612,-1.87066716028862,
60.4334949543147));
#49127=CARTESIAN_POINT('Ctrl Pts',(-7.62758081045792,-2.09855473598716,
60.4430627102172));
#49128=CARTESIAN_POINT('Ctrl Pts',(-7.58189647615823,-2.26460280024169,
60.4500341624432));
#49129=CARTESIAN_POINT('Ctrl Pts',(-7.53081522856453,-2.42906283056237,
60.4570056146692));
#49130=CARTESIAN_POINT('Ctrl Pts',(-7.47445012798801,-2.59162425598698,
60.4639770668951));
#49131=CARTESIAN_POINT('Ctrl Pts',(-7.41104955360762,-2.77447654647518,
60.4718186935554));
#49132=CARTESIAN_POINT('Ctrl Pts',(-7.340835215822,-2.95528893057795,60.4796603202158));
#49133=CARTESIAN_POINT('Ctrl Pts',(-7.26395463026879,-3.13350987383104,
60.4875019468761));
#49134=CARTESIAN_POINT('Ctrl Pts',(-7.18716456581266,-3.31152097535113,
60.4953343406118));
#49135=CARTESIAN_POINT('Ctrl Pts',(-7.10372401991034,-3.48694639223469,
60.5031667343475));
#49136=CARTESIAN_POINT('Ctrl Pts',(-7.01383039931391,-3.65924912101652,
60.5109991280833));
#49137=CARTESIAN_POINT('Ctrl Pts',(-6.92402512227369,-3.83138251814048,
60.5188238244817));
#49138=CARTESIAN_POINT('Ctrl Pts',(-6.82777956102114,-4.00039902913049,
60.5266485208802));
#49139=CARTESIAN_POINT('Ctrl Pts',(-6.7253394560609,-4.16578086326567,60.5344732172787));
#49140=CARTESIAN_POINT('Ctrl Pts',(-6.62298009498893,-4.3310323424745,60.5422917462058));
#49141=CARTESIAN_POINT('Ctrl Pts',(-6.5144360989321,-4.49265455325189,60.5501102751329));
#49142=CARTESIAN_POINT('Ctrl Pts',(-6.39999953864532,-4.65015342815048,
60.55792880406));
#49143=CARTESIAN_POINT('Ctrl Pts',(-6.28563092338073,-4.80755879041183,
60.5657426908507));
#49144=CARTESIAN_POINT('Ctrl Pts',(-6.16537691916071,-4.96084540978745,
60.5735565776415));
#49145=CARTESIAN_POINT('Ctrl Pts',(-6.03957349621163,-5.10954723863651,
60.5813704644322));
#49146=CARTESIAN_POINT('Ctrl Pts',(-5.91382030895259,-5.25818968802828,
60.5891812309899));
#49147=CARTESIAN_POINT('Ctrl Pts',(-5.78252234485846,-5.40225072637248,
60.5969919975476));
#49148=CARTESIAN_POINT('Ctrl Pts',(-5.64605663851594,-5.54129636769864,
60.6048027641053));
#49149=CARTESIAN_POINT('Ctrl Pts',(-5.50959635602139,-5.68033648263695,
60.612613220223));
#49150=CARTESIAN_POINT('Ctrl Pts',(-5.36796898031928,-5.81436134035106,
60.6204236763408));
#49151=CARTESIAN_POINT('Ctrl Pts',(-5.22158960635568,-5.94297257126418,
60.6282341324585));
#49152=CARTESIAN_POINT('Ctrl Pts',(-5.0752061955324,-6.07158734902599,60.6360448039735));
#49153=CARTESIAN_POINT('Ctrl Pts',(-4.92407078928556,-6.19478796965872,
60.6438554754885));
#49154=CARTESIAN_POINT('Ctrl Pts',(-4.76863284851574,-6.31221528118748,
60.6516661470034));
#49155=CARTESIAN_POINT('Ctrl Pts',(-4.61316324623443,-6.42966651175527,
60.6594784094921));
#49156=CARTESIAN_POINT('Ctrl Pts',(-4.45338964439313,-6.54134187845383,
60.6672906719807));
#49157=CARTESIAN_POINT('Ctrl Pts',(-4.2897919745336,-6.64692453810235,60.6751029344693));
#49158=CARTESIAN_POINT('Ctrl Pts',(-4.12613216709922,-6.7525473000972,60.6829181642071));
#49159=CARTESIAN_POINT('Ctrl Pts',(-3.95864569386522,-6.85207255478377,
60.6907333939448));
#49160=CARTESIAN_POINT('Ctrl Pts',(-3.78783877802627,-6.94522846216598,
60.6985486236826));
#49161=CARTESIAN_POINT('Ctrl Pts',(-3.61684610137414,-7.03848568111994,
60.7063723528621));
#49162=CARTESIAN_POINT('Ctrl Pts',(-3.44252607862198,-7.12535954905826,
60.7141960820416));
#49163=CARTESIAN_POINT('Ctrl Pts',(-3.26540764991057,-7.2056251553842,60.7220198112211));
#49164=CARTESIAN_POINT('Ctrl Pts',(-3.08818175926735,-7.28593946074827,
60.7298482872418));
#49165=CARTESIAN_POINT('Ctrl Pts',(-2.90815440362756,-7.35963738128823,
60.7376767632625));
#49166=CARTESIAN_POINT('Ctrl Pts',(-2.72587159942505,-7.42654327553862,
60.7455052392832));
#49167=CARTESIAN_POINT('Ctrl Pts',(-2.54333792299625,-7.49354125105097,
60.7533444894809));
#49168=CARTESIAN_POINT('Ctrl Pts',(-2.35854293136561,-7.55372842099553,
60.7611837396787));
#49169=CARTESIAN_POINT('Ctrl Pts',(-2.17204591570938,-7.60697952804201,
60.7690229898764));
#49170=CARTESIAN_POINT('Ctrl Pts',(-2.06748391828869,-7.63683545950584,
60.7734181682983));
#49171=CARTESIAN_POINT('Ctrl Pts',(-1.96238706989977,-7.66451201217708,
60.7778133467202));
#49172=CARTESIAN_POINT('Ctrl Pts',(-1.85685482900996,-7.68999422262347,
60.7822085251421));
#49173=CARTESIAN_POINT('Ctrl Pts',(-1.66693130152836,-7.73585386944991,
60.7901184091998));
#49174=CARTESIAN_POINT('Ctrl Pts',(-1.475051451079,-7.7747352926267,60.7980282932576));
#49175=CARTESIAN_POINT('Ctrl Pts',(-1.28177052722043,-7.80647073366378,
60.8059381773153));
#49176=CARTESIAN_POINT('Ctrl Pts',(-1.08869973213889,-7.83817167295448,
60.8138394620027));
#49177=CARTESIAN_POINT('Ctrl Pts',(-0.894231234931356,-7.86274204905463,
60.82174074669));
#49178=CARTESIAN_POINT('Ctrl Pts',(-0.698934092500138,-7.88006422146045,
60.8296420313773));
#49179=CARTESIAN_POINT('Ctrl Pts',(-0.503812979898112,-7.89737078063705,
60.8375361942922));
#49180=CARTESIAN_POINT('Ctrl Pts',(-0.307865051381116,-7.90744212028735,
60.8454303572072));
#49181=CARTESIAN_POINT('Ctrl Pts',(-0.111668455390341,-7.91021182750947,
60.8533245201221));
#49182=CARTESIAN_POINT('Ctrl Pts',(0.0843877467139504,-7.91297955279118,
60.861213034151));
#49183=CARTESIAN_POINT('Ctrl Pts',(0.280691918259379,-7.9084560504733,60.8691015481799));
#49184=CARTESIAN_POINT('Ctrl Pts',(0.476661619744055,-7.89662679251483,
60.8769900622088));
#49185=CARTESIAN_POINT('Ctrl Pts',(0.672527486035284,-7.88480380232774,
60.8848743964825));
#49186=CARTESIAN_POINT('Ctrl Pts',(0.868058891883867,-7.86568279062602,
60.8927587307562));
#49187=CARTESIAN_POINT('Ctrl Pts',(1.06267394828886,-7.83930131323118,60.9006430650299));
#49188=CARTESIAN_POINT('Ctrl Pts',(1.25722202610392,-7.81292891526827,60.9085246858363));
#49189=CARTESIAN_POINT('Ctrl Pts',(1.45085404158705,-7.77930107796768,60.9164063066427));
#49190=CARTESIAN_POINT('Ctrl Pts',(1.64299349497953,-7.73850718003511,60.9242879274491));
#49191=CARTESIAN_POINT('Ctrl Pts',(1.83513546489242,-7.69771274781001,60.9321696514839));
#49192=CARTESIAN_POINT('Ctrl Pts',(2.02578449446142,-7.64975213068483,60.9400513755187));
#49193=CARTESIAN_POINT('Ctrl Pts',(2.21437397475913,-7.59476588842009,60.9479330995536));
#49194=CARTESIAN_POINT('Ctrl Pts',(2.40297481572181,-7.53977633377402,60.9558152983849));
#49195=CARTESIAN_POINT('Ctrl Pts',(2.58951552864162,-7.4777604066923,60.9636974972163));
#49196=CARTESIAN_POINT('Ctrl Pts',(2.77344434461483,-7.40890865562021,60.9715796960476));
#49197=CARTESIAN_POINT('Ctrl Pts',(2.9574151902524,-7.34004117120056,60.9794636960441));
#49198=CARTESIAN_POINT('Ctrl Pts',(3.13877262644362,-7.26433487113398,60.9873476960406));
#49199=CARTESIAN_POINT('Ctrl Pts',(3.31698433008067,-7.18202867955839,60.9952316960371));
#49200=CARTESIAN_POINT('Ctrl Pts',(3.49526674509232,-7.09968983028511,61.0031188242708));
#49201=CARTESIAN_POINT('Ctrl Pts',(3.67040062743373,-7.01074601604411,61.0110059525044));
#49202=CARTESIAN_POINT('Ctrl Pts',(3.84187752886709,-6.91548248882072,61.0188930807381));
#49203=CARTESIAN_POINT('Ctrl Pts',(4.01353737656521,-6.82011732629645,61.0267886236366));
#49204=CARTESIAN_POINT('Ctrl Pts',(4.18153214850993,-6.7184191509624,61.0346841665351));
#49205=CARTESIAN_POINT('Ctrl Pts',(4.34538076693062,-6.61071758513321,61.0425797094336));
#49206=CARTESIAN_POINT('Ctrl Pts',(4.50932916348269,-6.50295043278221,61.0504800604441));
#49207=CARTESIAN_POINT('Ctrl Pts',(4.66912609253968,-6.38917280111203,61.0583804114547));
#49208=CARTESIAN_POINT('Ctrl Pts',(4.82432274712431,-6.26975526089966,61.0662807624652));
#49209=CARTESIAN_POINT('Ctrl Pts',(4.97972147427797,-6.15018223402939,61.0741914000649));
#49210=CARTESIAN_POINT('Ctrl Pts',(5.1305076981577,-6.02495485036458,61.0821020376646));
#49211=CARTESIAN_POINT('Ctrl Pts',(5.27626787837343,-5.8944820192825,61.0900126752643));
#49212=CARTESIAN_POINT('Ctrl Pts',(5.34031186522947,-5.83715497518498,61.0934884446391));
#49213=CARTESIAN_POINT('Ctrl Pts',(5.40338605588324,-5.77881573223792,61.0969642140139));
#49214=CARTESIAN_POINT('Ctrl Pts',(5.46545780336309,-5.71950102715765,61.1004399833887));
#49215=CARTESIAN_POINT('Ctrl Pts',(5.60671549841262,-5.58451757877156,61.1083498488321));
#49216=CARTESIAN_POINT('Ctrl Pts',(5.74316021425428,-5.44411577413464,61.1162597142756));
#49217=CARTESIAN_POINT('Ctrl Pts',(5.87435065001632,-5.29867204501777,61.1241695797191));
#49218=CARTESIAN_POINT('Ctrl Pts',(6.00539850900617,-5.15338638304439,61.1320708487807));
#49219=CARTESIAN_POINT('Ctrl Pts',(6.1312032329654,-5.00306996473738,61.1399721178423));
#49220=CARTESIAN_POINT('Ctrl Pts',(6.25135822035415,-4.84813793128976,61.1478733869039));
#49221=CARTESIAN_POINT('Ctrl Pts',(6.3714049518872,-4.69334548671999,61.1557675371712));
#49222=CARTESIAN_POINT('Ctrl Pts',(6.48581187689786,-4.53394598196298,61.1636616874385));
#49223=CARTESIAN_POINT('Ctrl Pts',(6.59421057600542,-4.37038990014601,61.1715558377058));
#49224=CARTESIAN_POINT('Ctrl Pts',(6.70253174808528,-4.20695079405837,61.1794443420565));
#49225=CARTESIAN_POINT('Ctrl Pts',(6.80485306569523,-4.03936132005771,61.1873328464072));
#49226=CARTESIAN_POINT('Ctrl Pts',(6.90084743965403,-3.86810361994355,61.195221350758));
#49227=CARTESIAN_POINT('Ctrl Pts',(6.99679098666944,-3.69693659707506,61.2031056783164));
#49228=CARTESIAN_POINT('Ctrl Pts',(7.0864140970039,-3.52210551845024,61.2109900058748));
#49229=CARTESIAN_POINT('Ctrl Pts',(7.16943379640047,-3.34412021898596,61.2188743334333));
#49230=CARTESIAN_POINT('Ctrl Pts',(7.25242495491509,-3.16619610810051,61.2267559504825));
#49231=CARTESIAN_POINT('Ctrl Pts',(7.32881708129936,-2.98512024980436,61.2346375675317));
#49232=CARTESIAN_POINT('Ctrl Pts',(7.39837371244669,-2.80142596028841,61.2425191845809));
#49233=CARTESIAN_POINT('Ctrl Pts',(7.4679312936594,-2.61772916171497,61.2504009092841));
#49234=CARTESIAN_POINT('Ctrl Pts',(7.53065306293866,-2.43141418001852,61.2582826339873));
#49235=CARTESIAN_POINT('Ctrl Pts',(7.58635096178516,-2.24303367888701,61.2661643586905));
#49236=CARTESIAN_POINT('Ctrl Pts',(7.64205223536903,-2.05464176377526,61.2740465609477));
#49237=CARTESIAN_POINT('Ctrl Pts',(7.69072869204972,-1.86418441069174,61.2819287632048));
#49238=CARTESIAN_POINT('Ctrl Pts',(7.73224235045464,-1.67222882221175,61.289810965462));
#49239=CARTESIAN_POINT('Ctrl Pts',(7.77376550969032,-1.48022930270693,61.2976949716428));
#49240=CARTESIAN_POINT('Ctrl Pts',(7.80812253118399,-1.28673120184782,61.3055789778236));
#49241=CARTESIAN_POINT('Ctrl Pts',(7.83522664353816,-1.09231151435374,61.3134629840044));
#49242=CARTESIAN_POINT('Ctrl Pts',(7.86234151982677,-0.897814616407488,
61.3213501211833));
#49243=CARTESIAN_POINT('Ctrl Pts',(7.88219769998987,-0.702395744051026,
61.3292372583623));
#49244=CARTESIAN_POINT('Ctrl Pts',(7.89476029409556,-0.506636850981302,
61.3371243955412));
#49245=CARTESIAN_POINT('Ctrl Pts',(7.90733629761916,-0.310669003233389,
61.3450199515163));
#49246=CARTESIAN_POINT('Ctrl Pts',(7.91260314256511,-0.114360754286667,
61.3529155074914));
#49247=CARTESIAN_POINT('Ctrl Pts',(7.91057806332336,0.0817049818996074,
61.3608110634664));
#49248=CARTESIAN_POINT('Ctrl Pts',(7.90855175027101,0.277890174144436,61.3687114299301));
#49249=CARTESIAN_POINT('Ctrl Pts',(7.89922467226719,0.473832215323574,61.3766117963938));
#49250=CARTESIAN_POINT('Ctrl Pts',(7.88266595834452,0.668953204010979,61.3845121628575));
#49251=CARTESIAN_POINT('Ctrl Pts',(7.86608567692635,0.864328335083012,61.3924228194391));
#49252=CARTESIAN_POINT('Ctrl Pts',(7.84225498728872,1.0588799361571,61.4003334760207));
#49253=CARTESIAN_POINT('Ctrl Pts',(7.81129433698851,1.25203904928371,61.4082441326023));
#49254=CARTESIAN_POINT('Ctrl Pts',(7.79769090364407,1.3369089436435,61.4117199022801));
#49255=CARTESIAN_POINT('Ctrl Pts',(7.78271166383436,1.42151018952133,61.4151956719579));
#49256=CARTESIAN_POINT('Ctrl Pts',(7.76636987437531,1.50579546233731,61.4186714416357));
#49257=CARTESIAN_POINT('Ctrl Pts',(7.7295145903776,1.6958822135001,61.4265102697461));
#49258=CARTESIAN_POINT('Ctrl Pts',(7.68562068403171,1.88490219238425,61.4343490978565));
#49259=CARTESIAN_POINT('Ctrl Pts',(7.63475875621671,2.07228852585065,61.4421879259669));
#49260=CARTESIAN_POINT('Ctrl Pts',(7.58395384383499,2.25946480213964,61.4500179668724));
#49261=CARTESIAN_POINT('Ctrl Pts',(7.52619655453168,2.4450107436099,61.4578480077779));
#49262=CARTESIAN_POINT('Ctrl Pts',(7.46160890470589,2.62836708874803,61.4656780486834));
#49263=CARTESIAN_POINT('Ctrl Pts',(7.39708108610036,2.81155358045593,61.4735008361758));
#49264=CARTESIAN_POINT('Ctrl Pts',(7.32573562359224,2.99255418583702,61.4813236236683));
#49265=CARTESIAN_POINT('Ctrl Pts',(7.24774504098589,3.17082210489086,61.4891464111607));
#49266=CARTESIAN_POINT('Ctrl Pts',(7.16981153455072,3.34895956139493,61.4969634736702));
#49267=CARTESIAN_POINT('Ctrl Pts',(7.08524273430716,3.52436799398476,61.5047805361796));
#49268=CARTESIAN_POINT('Ctrl Pts',(6.99426029815046,3.69651780486936,61.5125975986891));
#49269=CARTESIAN_POINT('Ctrl Pts',(6.90332675437798,3.86857510542941,61.5204104604447));
#49270=CARTESIAN_POINT('Ctrl Pts',(6.80598660427244,4.0373769623895,61.5282233222002));
#49271=CARTESIAN_POINT('Ctrl Pts',(6.70250881419265,4.20241556675085,61.5360361839558));
#49272=CARTESIAN_POINT('Ctrl Pts',(6.59906651483257,4.36739756631958,61.5438463660631));
#49273=CARTESIAN_POINT('Ctrl Pts',(6.48949095637755,4.52861858731441,61.5516565481703));
#49274=CARTESIAN_POINT('Ctrl Pts',(6.37409615292086,4.68559699860322,61.5594667302775));
#49275=CARTESIAN_POINT('Ctrl Pts',(6.25869614508426,4.84258248971942,61.567277264629));
#49276=CARTESIAN_POINT('Ctrl Pts',(6.13747656880136,4.99532469993766,61.5750877989805));
#49277=CARTESIAN_POINT('Ctrl Pts',(6.01079402253949,5.14337206690353,61.582898333332));
#49278=CARTESIAN_POINT('Ctrl Pts',(5.88410132255246,5.29143130000503,61.5907094937051));
#49279=CARTESIAN_POINT('Ctrl Pts',(5.75194500859647,5.43479467224237,61.5985206540783));
#49280=CARTESIAN_POINT('Ctrl Pts',(5.6147210607534,5.57304480602231,61.6063318144514));
#49281=CARTESIAN_POINT('Ctrl Pts',(5.47746194643577,5.71133036925818,61.614144976596));
#49282=CARTESIAN_POINT('Ctrl Pts',(5.33513285896086,5.84449983381412,61.6219581387405));
#49283=CARTESIAN_POINT('Ctrl Pts',(5.18816571862437,5.97217359728356,61.629771300885));
#49284=CARTESIAN_POINT('Ctrl Pts',(5.04113502881494,6.09990256765408,61.6375878414877));
#49285=CARTESIAN_POINT('Ctrl Pts',(4.88946255643335,6.2221308725666,61.6454043820905));
#49286=CARTESIAN_POINT('Ctrl Pts',(4.73361238585418,6.33851992033534,61.6532209226932));
#49287=CARTESIAN_POINT('Ctrl Pts',(4.57758033528857,6.45504479624178,61.6610465853411));
#49288=CARTESIAN_POINT('Ctrl Pts',(4.41736113078819,6.56571659384646,61.668872247989));
#49289=CARTESIAN_POINT('Ctrl Pts',(4.25344777839035,6.67024010036417,61.6766979106369));
#49290=CARTESIAN_POINT('Ctrl Pts',(4.08942758200694,6.77483173865918,61.6845286743029));
#49291=CARTESIAN_POINT('Ctrl Pts',(3.92170874145689,6.87326692191954,61.692359437969));
#49292=CARTESIAN_POINT('Ctrl Pts',(3.75080786426145,6.96529693303842,61.700190201635));
#49293=CARTESIAN_POINT('Ctrl Pts',(3.57966005326413,7.05745991784887,61.7080322799314));
#49294=CARTESIAN_POINT('Ctrl Pts',(3.40532133696547,7.14319909102459,61.7158743582278));
#49295=CARTESIAN_POINT('Ctrl Pts',(3.22832834390742,7.22231383310944,61.7237164365241));
#49296=CARTESIAN_POINT('Ctrl Pts',(3.1291237058251,7.26665767531414,61.7281119243102));
#49297=CARTESIAN_POINT('Ctrl Pts',(3.0290854894646,7.30892127559068,61.7325074120962));
#49298=CARTESIAN_POINT('Ctrl Pts',(2.92831002128822,7.34907622897075,61.7369028998823));
#49299=CARTESIAN_POINT('Ctrl Pts',(2.74680765997869,7.42139758841114,61.7448194238808));
#49300=CARTESIAN_POINT('Ctrl Pts',(2.56236828562723,7.48709311749584,61.7527359478793));
#49301=CARTESIAN_POINT('Ctrl Pts',(2.37551672861666,7.54591553570953,61.7606524718777));
#49302=CARTESIAN_POINT('Ctrl Pts',(2.18888043598011,7.60467018691481,61.7685598755584));
#49303=CARTESIAN_POINT('Ctrl Pts',(1.99983782129082,7.65656739646813,61.7764672792391));
#49304=CARTESIAN_POINT('Ctrl Pts',(1.80893475291605,7.70140740772052,61.7843746829197));
#49305=CARTESIAN_POINT('Ctrl Pts',(1.6182162411962,7.74620406963048,61.7922744420718));
#49306=CARTESIAN_POINT('Ctrl Pts',(1.42564119176957,7.78395704594293,61.8001742012238));
#49307=CARTESIAN_POINT('Ctrl Pts',(1.23177201580282,7.81451589678369,61.8080739603758));
#49308=CARTESIAN_POINT('Ctrl Pts',(1.03805435169923,7.84505086539355,61.8159675457397));
#49309=CARTESIAN_POINT('Ctrl Pts',(0.843044914796897,7.86840285650722,61.8238611311036));
#49310=CARTESIAN_POINT('Ctrl Pts',(0.647318013532443,7.88447210594066,61.8317547164674));
#49311=CARTESIAN_POINT('Ctrl Pts',(0.451707828785264,7.90053177290579,61.8396435947022));
#49312=CARTESIAN_POINT('Ctrl Pts',(0.255381374618466,7.90931732363015,61.8475324729369));
#49313=CARTESIAN_POINT('Ctrl Pts',(0.058920102984681,7.91078058231072,61.8554213511717));
#49314=CARTESIAN_POINT('Ctrl Pts',(-0.137460390642674,7.91224323935048,
61.8633069857755));
#49315=CARTESIAN_POINT('Ctrl Pts',(-0.333975247228655,7.90638960191985,
61.8711926203793));
#49316=CARTESIAN_POINT('Ctrl Pts',(-0.530040690244659,7.89322354090425,
61.8790782549832));
#49317=CARTESIAN_POINT('Ctrl Pts',(-0.726088691952936,7.88005865109617,
61.8869631881081));
#49318=CARTESIAN_POINT('Ctrl Pts',(-0.921687015649926,7.85958265032517,
61.8948481212329));
#49319=CARTESIAN_POINT('Ctrl Pts',(-1.11625416202244,7.83185148261684,61.9027330543578));
#49320=CARTESIAN_POINT('Ctrl Pts',(-1.31082063381719,7.80412041105439,61.9106179601451));
#49321=CARTESIAN_POINT('Ctrl Pts',(-1.5043555940604,7.76913427075128,61.9185028659324));
#49322=CARTESIAN_POINT('Ctrl Pts',(-1.69628481823644,7.72700063513784,61.9263877717197));
#49323=CARTESIAN_POINT('Ctrl Pts',(-1.88824557814089,7.68486007658239,61.9342739730691));
#49324=CARTESIAN_POINT('Ctrl Pts',(-2.07859973958628,7.63556975658473,61.9421601744186));
#49325=CARTESIAN_POINT('Ctrl Pts',(-2.26678514152769,7.57928796933784,61.9500463757681));
#49326=CARTESIAN_POINT('Ctrl Pts',(-2.45503303722391,7.52298749169214,61.9579351960153));
#49327=CARTESIAN_POINT('Ctrl Pts',(-2.64111040837763,7.45969101943708,61.9658240162626));
#49328=CARTESIAN_POINT('Ctrl Pts',(-2.82447183645689,7.38960620365266,61.9737128365099));
#49329=CARTESIAN_POINT('Ctrl Pts',(-3.00801074147592,7.31945355223476,61.9816092924071));
#49330=CARTESIAN_POINT('Ctrl Pts',(-3.18882813050841,7.24249955629964,61.9895057483043));
#49331=CARTESIAN_POINT('Ctrl Pts',(-3.36639912302167,7.15899978659861,61.9974022042014));
#49332=CARTESIAN_POINT('Ctrl Pts',(-3.54406825920082,7.07545386649101,62.0053030244777));
#49333=CARTESIAN_POINT('Ctrl Pts',(-3.71848711581281,6.98535511714533,62.013203844754));
#49334=CARTESIAN_POINT('Ctrl Pts',(-3.88915663111816,6.88900440547323,62.0211046650303));
#49335=CARTESIAN_POINT('Ctrl Pts',(-4.06003353299557,6.79253661463927,62.0290150858732));
#49336=CARTESIAN_POINT('Ctrl Pts',(-4.22715170019501,6.68980186659931,62.036925506716));
#49337=CARTESIAN_POINT('Ctrl Pts',(-4.39004128030048,6.58114416779162,62.0448359275588));
#49338=CARTESIAN_POINT('Ctrl Pts',(-4.46072892405258,6.53399101840499,62.048268737749));
#49339=CARTESIAN_POINT('Ctrl Pts',(-4.53062065254584,6.48572296513387,62.0517015479392));
#49340=CARTESIAN_POINT('Ctrl Pts',(-4.59968007684202,6.43637042056333,62.0551343581294));
#49341=CARTESIAN_POINT('Ctrl Pts',(-4.76694906485711,6.31683351057001,62.0634489754668));
#49342=CARTESIAN_POINT('Ctrl Pts',(-4.9296995827341,6.19066978758528,62.0717635928043));
#49343=CARTESIAN_POINT('Ctrl Pts',(-5.08740474275343,6.05823687085689,62.0800782101417));
#49344=CARTESIAN_POINT('Ctrl Pts',(-5.244914987101,5.9259676345745,62.0883825510289));
#49345=CARTESIAN_POINT('Ctrl Pts',(-5.39739208704405,5.78744484600442,62.0966868919161));
#49346=CARTESIAN_POINT('Ctrl Pts',(-5.54433962944533,5.64306823220861,62.1049912328033));
#49347=CARTESIAN_POINT('Ctrl Pts',(-5.69111526575402,5.49886051691313,62.113285858885));
#49348=CARTESIAN_POINT('Ctrl Pts',(-5.83237403816444,5.34881283986969,62.1215804849667));
#49349=CARTESIAN_POINT('Ctrl Pts',(-5.96765339521192,5.19336441573434,62.1298751110484));
#49350=CARTESIAN_POINT('Ctrl Pts',(-6.10272906282565,5.03815004949357,62.1381572479542));
#49351=CARTESIAN_POINT('Ctrl Pts',(-6.23184309027495,4.87755138508124,62.14643938486));
#49352=CARTESIAN_POINT('Ctrl Pts',(-6.35457045289099,4.71204364997236,62.1547215217658));
#49353=CARTESIAN_POINT('Ctrl Pts',(-6.47718463692134,4.54668854530368,62.1629960209246));
#49354=CARTESIAN_POINT('Ctrl Pts',(-6.59342372711044,4.37643363246062,62.1712705200834));
#49355=CARTESIAN_POINT('Ctrl Pts',(-6.70290243281007,4.20178771194225,62.1795450192422));
#49356=CARTESIAN_POINT('Ctrl Pts',(-6.81225522067375,4.02734266186921,62.1878100014176));
#49357=CARTESIAN_POINT('Ctrl Pts',(-6.9148629842122,3.8485169296869,62.196074983593));
#49358=CARTESIAN_POINT('Ctrl Pts',(-7.01038313183886,3.66584906192675,62.2043399657683));
#49359=CARTESIAN_POINT('Ctrl Pts',(-7.04856092206612,3.5928397993797,62.2076433395964));
#49360=CARTESIAN_POINT('Ctrl Pts',(-7.08560696786961,3.51921710218892,62.2109467134245));
#49361=CARTESIAN_POINT('Ctrl Pts',(-7.12150134325963,3.44501663536641,62.2142500872526));
#49362=CARTESIAN_POINT('Ctrl Pts',(-7.20926811728443,3.26358610388664,62.2223272988251));
#49363=CARTESIAN_POINT('Ctrl Pts',(-7.29006283849697,3.07887174248909,62.2304045103976));
#49364=CARTESIAN_POINT('Ctrl Pts',(-7.36365968952011,2.89144202378961,62.2384817219701));
#49365=CARTESIAN_POINT('Ctrl Pts',(-7.43730034680104,2.70390074332546,62.2465637412539));
#49366=CARTESIAN_POINT('Ctrl Pts',(-7.503734470668,2.51364117971434,62.2546457605377));
#49367=CARTESIAN_POINT('Ctrl Pts',(-7.56278562785052,2.32124848889076,62.2627277798215));
#49368=CARTESIAN_POINT('Ctrl Pts',(-7.62191733429708,2.12859336308041,62.2708208234567));
#49369=CARTESIAN_POINT('Ctrl Pts',(-7.67364585089429,1.93379960118771,62.2789138670918));
#49370=CARTESIAN_POINT('Ctrl Pts',(-7.71784514141328,1.73746579050163,62.287006910727));
#49371=CARTESIAN_POINT('Ctrl Pts',(-7.7620756290831,1.54099340167475,62.2951056666689));
#49372=CARTESIAN_POINT('Ctrl Pts',(-7.79876622757874,1.34297910977914,62.3032044226107));
#49373=CARTESIAN_POINT('Ctrl Pts',(-7.82784252260321,1.14402903867208,62.3113031785526));
#49374=CARTESIAN_POINT('Ctrl Pts',(-7.85696518990773,0.944761672379959,
62.3194148507817));
#49375=CARTESIAN_POINT('Ctrl Pts',(-7.8784492406051,0.744555862049014,62.3275265230108));
#49376=CARTESIAN_POINT('Ctrl Pts',(-7.89227223078456,0.544022090715932,
62.3356381952399));
#49377=CARTESIAN_POINT('Ctrl Pts',(-7.90477176190875,0.362688089628877,
62.3429732289903));
#49378=CARTESIAN_POINT('Ctrl Pts',(-7.91100766955499,0.181086106885633,
62.3503082627406));
#49379=CARTESIAN_POINT('Ctrl Pts',(-7.91099999291779,-0.00033474584610353,
62.3576432964909));
#49380=CARTESIAN_POINT('',(-7.911,-7.32081062437828E-12,64.3576684917633));
#49381=CARTESIAN_POINT('Ctrl Pts',(-7.91099999260071,-0.000333258038948825,
62.3576819008605));
#49382=CARTESIAN_POINT('Ctrl Pts',(-7.91090223079165,-2.20189632652019,
62.4462648668942));
#49383=CARTESIAN_POINT('Ctrl Pts',(-6.94206342521017,-4.38617874871575,
62.5348478329279));
#49384=CARTESIAN_POINT('Ctrl Pts',(-3.67820201487601,-7.34180684107976,
62.7120182346942));
#49385=CARTESIAN_POINT('Ctrl Pts',(-1.40868175870985,-8.08992666571469,
62.800605670427));
#49386=CARTESIAN_POINT('Ctrl Pts',(2.97309270521997,-7.65454228024977,62.9777805418924));
#49387=CARTESIAN_POINT('Ctrl Pts',(5.05102072676217,-6.47444880833747,63.0663679776251));
#49388=CARTESIAN_POINT('Ctrl Pts',(7.66951518848153,-2.93425195366975,63.2435428490906));
#49389=CARTESIAN_POINT('Ctrl Pts',(8.1895687224713,-0.601881960091314,63.3321302848233));
#49390=CARTESIAN_POINT('Ctrl Pts',(7.32306689760985,3.71537198233157,63.5093051562888));
#49391=CARTESIAN_POINT('Ctrl Pts',(5.94329958849653,5.66643518937088,63.5978925920215));
#49392=CARTESIAN_POINT('Ctrl Pts',(2.16154501637074,7.92205913233209,63.775067463487));
#49393=CARTESIAN_POINT('Ctrl Pts',(-0.210816529308416,8.20894963712982,
63.8636548992197));
#49394=CARTESIAN_POINT('Ctrl Pts',(-4.42123908577121,6.91982244717395,64.0408297706851));
#49395=CARTESIAN_POINT('Ctrl Pts',(-6.22631625634719,5.35390358802904,64.1294172064179));
#49396=CARTESIAN_POINT('Ctrl Pts',(-7.65317280859711,2.31334857513774,64.2645592586882));
#49397=CARTESIAN_POINT('Ctrl Pts',(-7.91100000000107,1.15702837835769,64.3111138752258));
#49398=CARTESIAN_POINT('Ctrl Pts',(-7.911,-7.32081062437828E-12,64.3576684917633));
#49399=CARTESIAN_POINT('',(-7.9109999940852,0.000305915063436288,66.3576880390319));
#49400=CARTESIAN_POINT('Ctrl Pts',(-7.911,-7.32081062437828E-12,64.3576684917633));
#49401=CARTESIAN_POINT('Ctrl Pts',(-7.91099999999796,-2.20167589667412,
64.4462559274961));
#49402=CARTESIAN_POINT('Ctrl Pts',(-6.94214576671962,-4.38610418339331,
64.5348433632288));
#49403=CARTESIAN_POINT('Ctrl Pts',(-3.67820201487596,-7.34180684107979,
64.7120182346942));
#49404=CARTESIAN_POINT('Ctrl Pts',(-1.4086817587098,-8.0899266657147,64.800605670427));
#49405=CARTESIAN_POINT('Ctrl Pts',(2.97309270522002,-7.65454228024975,64.9777805418924));
#49406=CARTESIAN_POINT('Ctrl Pts',(5.05102072676222,-6.47444880833743,65.0663679776251));
#49407=CARTESIAN_POINT('Ctrl Pts',(7.66951518848155,-2.93425195366969,65.2435428490906));
#49408=CARTESIAN_POINT('Ctrl Pts',(8.1895687224713,-0.601881960091258,65.3321302848233));
#49409=CARTESIAN_POINT('Ctrl Pts',(7.32306689760982,3.71537198233162,65.5093051562888));
#49410=CARTESIAN_POINT('Ctrl Pts',(5.94329958849649,5.66643518937092,65.5978925920215));
#49411=CARTESIAN_POINT('Ctrl Pts',(2.16154501637069,7.92205913233211,65.775067463487));
#49412=CARTESIAN_POINT('Ctrl Pts',(-0.210816529308472,8.20894963712982,
65.8636548992197));
#49413=CARTESIAN_POINT('Ctrl Pts',(-4.42123908577125,6.91982244717392,66.0408297706851));
#49414=CARTESIAN_POINT('Ctrl Pts',(-6.22631625634723,5.353903588029,66.1294172064179));
#49415=CARTESIAN_POINT('Ctrl Pts',(-7.65312966182839,2.31344051859464,66.2645551721226));
#49416=CARTESIAN_POINT('Ctrl Pts',(-7.91095473404371,1.15723138115899,66.3111057020946));
#49417=CARTESIAN_POINT('Ctrl Pts',(-7.91099999404008,0.000304691929376763,
66.3576562320666));
#49418=CARTESIAN_POINT('',(-7.91099954886372,-0.00267168074885584,68.3574023474442));
#49419=CARTESIAN_POINT('Ctrl Pts',(-7.9109999940852,0.000305915063436288,
66.3576880390319));
#49420=CARTESIAN_POINT('Ctrl Pts',(-7.91100793685849,-0.2050951487285,66.3659089648299));
#49421=CARTESIAN_POINT('Ctrl Pts',(-7.90301201333921,-0.410360118679733,
66.3741298906278));
#49422=CARTESIAN_POINT('Ctrl Pts',(-7.88706988155102,-0.614857449764415,
66.3823508164258));
#49423=CARTESIAN_POINT('Ctrl Pts',(-7.8711114624684,-0.819563705746012,
66.3905801411405));
#49424=CARTESIAN_POINT('Ctrl Pts',(-7.84719065175379,-1.02350045984394,
66.3988094658553));
#49425=CARTESIAN_POINT('Ctrl Pts',(-7.81541669025749,-1.22604361979689,
66.40703879057));
#49426=CARTESIAN_POINT('Ctrl Pts',(-7.78216777393996,-1.43798888122569,
66.4156501224879));
#49427=CARTESIAN_POINT('Ctrl Pts',(-7.74031937245779,-1.64840771187476,
66.4242614544058));
#49428=CARTESIAN_POINT('Ctrl Pts',(-7.6900554697985,-1.85660116110655,66.4328727863237));
#49429=CARTESIAN_POINT('Ctrl Pts',(-7.64187765064024,-2.05615403735281,
66.4411267254311));
#49430=CARTESIAN_POINT('Ctrl Pts',(-7.58596885857615,-2.2536622577624,66.4493806645385));
#49431=CARTESIAN_POINT('Ctrl Pts',(-7.52254125280714,-2.44852896650516,
66.457634603646));
#49432=CARTESIAN_POINT('Ctrl Pts',(-7.45904666143902,-2.64360147307165,
66.4658972597001));
#49433=CARTESIAN_POINT('Ctrl Pts',(-7.38801750594898,-2.83602661913333,
66.4741599157542));
#49434=CARTESIAN_POINT('Ctrl Pts',(-7.30971382302372,-3.02522806173286,
66.4824225718082));
#49435=CARTESIAN_POINT('Ctrl Pts',(-7.23128197129088,-3.21473919248989,
66.4906987523191));
#49436=CARTESIAN_POINT('Ctrl Pts',(-7.14555191693428,-3.4010158024365,66.49897493283));
#49437=CARTESIAN_POINT('Ctrl Pts',(-7.05283007982976,-3.58350510883528,
66.5072511133408));
#49438=CARTESIAN_POINT('Ctrl Pts',(-7.04116481483934,-3.60646395201113,
66.5082923334221));
#49439=CARTESIAN_POINT('Ctrl Pts',(-7.02938894070794,-3.62936288698674,
66.5093335535034));
#49440=CARTESIAN_POINT('Ctrl Pts',(-7.01750311600732,-3.65220084563096,
66.5103747735847));
#49441=CARTESIAN_POINT('Ctrl Pts',(-6.92258938364662,-3.83457236372255,
66.518689390922));
#49442=CARTESIAN_POINT('Ctrl Pts',(-6.82048096715838,-4.01339878052998,
66.5270040082594));
#49443=CARTESIAN_POINT('Ctrl Pts',(-6.71145811088942,-4.18810828725531,
66.5353186255967));
#49444=CARTESIAN_POINT('Ctrl Pts',(-6.6025700014052,-4.36260186178899,66.5436229664839));
#49445=CARTESIAN_POINT('Ctrl Pts',(-6.48678465096934,-4.53298842694055,
66.551927307371));
#49446=CARTESIAN_POINT('Ctrl Pts',(-6.36442826724767,-4.69872044614902,
66.5602316482582));
#49447=CARTESIAN_POINT('Ctrl Pts',(-6.24221502173409,-4.86425858430666,
66.5685262743398));
#49448=CARTESIAN_POINT('Ctrl Pts',(-6.11344624863497,-5.02515280186179,
66.5768209004215));
#49449=CARTESIAN_POINT('Ctrl Pts',(-5.97849199928957,-5.18088355538229,
66.5851155265031));
#49450=CARTESIAN_POINT('Ctrl Pts',(-5.84374094986418,-5.33637982590716,
66.5933976634088));
#49451=CARTESIAN_POINT('Ctrl Pts',(-5.7028232020138,-5.48672792677824,66.6016798003146));
#49452=CARTESIAN_POINT('Ctrl Pts',(-5.55614972395224,-5.63144042364167,
66.6099619372203));
#49453=CARTESIAN_POINT('Ctrl Pts',(-5.40961150747035,-5.77601946733291,
66.618236436379));
#49454=CARTESIAN_POINT('Ctrl Pts',(-5.2573283535909,-5.91497306562621,66.6265109355377));
#49455=CARTESIAN_POINT('Ctrl Pts',(-5.09975004103882,-6.04784842063065,
66.6347854346964));
#49456=CARTESIAN_POINT('Ctrl Pts',(-4.94235296848039,-6.18057094795145,
66.6430504168718));
#49457=CARTESIAN_POINT('Ctrl Pts',(-4.77967311367969,-6.30722899337593,
66.6513153990472));
#49458=CARTESIAN_POINT('Ctrl Pts',(-4.61219569221497,-6.42740786761768,
66.6595803812226));
#49459=CARTESIAN_POINT('Ctrl Pts',(-4.54525779456572,-6.47544133453663,
66.6628837550511));
#49460=CARTESIAN_POINT('Ctrl Pts',(-4.47755389912394,-6.52244020255479,
66.6661871288795));
#49461=CARTESIAN_POINT('Ctrl Pts',(-4.40911652618476,-6.56837974378191,
66.669490502708));
#49462=CARTESIAN_POINT('Ctrl Pts',(-4.23786450353326,-6.68333505280314,
66.6777565922057));
#49463=CARTESIAN_POINT('Ctrl Pts',(-4.06221137484325,-6.79152428198379,
66.6860226817034));
#49464=CARTESIAN_POINT('Ctrl Pts',(-3.88271586641192,-6.89263654204348,
66.694288771201));
#49465=CARTESIAN_POINT('Ctrl Pts',(-3.70305893742194,-6.9938397324983,66.7025622944044));
#49466=CARTESIAN_POINT('Ctrl Pts',(-3.51955298617807,-7.08795310408813,
66.7108358176078));
#49467=CARTESIAN_POINT('Ctrl Pts',(-3.33277978190764,-7.17471253259026,
66.7191093408112));
#49468=CARTESIAN_POINT('Ctrl Pts',(-3.14582646382379,-7.26155562711706,
66.7273908425456));
#49469=CARTESIAN_POINT('Ctrl Pts',(-2.95559986852891,-7.34103049676887,
66.7356723442801));
#49470=CARTESIAN_POINT('Ctrl Pts',(-2.76270087022072,-7.41292148222829,
66.7439538460145));
#49471=CARTESIAN_POINT('Ctrl Pts',(-2.56948069923837,-7.48493216462887,
66.7522491362708));
#49472=CARTESIAN_POINT('Ctrl Pts',(-2.37357950522289,-7.54933361541845,
66.7605444265272));
#49473=CARTESIAN_POINT('Ctrl Pts',(-2.17561438137431,-7.60595970693753,
66.7688397167835));
#49474=CARTESIAN_POINT('Ctrl Pts',(-1.97746972180394,-7.66263715298824,
66.7771425300868));
#49475=CARTESIAN_POINT('Ctrl Pts',(-1.77725767987169,-7.7115250900311,66.7854453433901));
#49476=CARTESIAN_POINT('Ctrl Pts',(-1.57560590028026,-7.75250843579045,
66.7937481566934));
#49477=CARTESIAN_POINT('Ctrl Pts',(-1.37364488378663,-7.79355463030278,
66.8020637025214));
#49478=CARTESIAN_POINT('Ctrl Pts',(-1.17024000542739,-7.8266719515452,66.8103792483493));
#49479=CARTESIAN_POINT('Ctrl Pts',(-0.966026280522799,-7.85179687876217,
66.8186947941773));
#49480=CARTESIAN_POINT('Ctrl Pts',(-0.884891033184819,-7.86177915191765,
66.8219986067287));
#49481=CARTESIAN_POINT('Ctrl Pts',(-0.803628133299662,-7.87050038989894,
66.8253024192801));
#49482=CARTESIAN_POINT('Ctrl Pts',(-0.722277443167851,-7.8779588914319,
66.8286062318315));
#49483=CARTESIAN_POINT('Ctrl Pts',(-0.52751463616729,-7.89581539261491,
66.8365159349363));
#49484=CARTESIAN_POINT('Ctrl Pts',(-0.331842449390223,-7.90646769815302,
66.8444256380411));
#49485=CARTESIAN_POINT('Ctrl Pts',(-0.135835962244705,-7.90983372716273,
66.8523353411458));
#49486=CARTESIAN_POINT('Ctrl Pts',(0.0599716667651551,-7.91319634117193,
66.8602370194712));
#49487=CARTESIAN_POINT('Ctrl Pts',(0.256112578798345,-7.90928739768237,
66.8681386977966));
#49488=CARTESIAN_POINT('Ctrl Pts',(0.452005680182568,-7.89807646614558,
66.876040376122));
#49489=CARTESIAN_POINT('Ctrl Pts',(0.647736328092416,-7.88687483179571,
66.8839355016128));
#49490=CARTESIAN_POINT('Ctrl Pts',(0.843219232633905,-7.86838329254936,
66.8918306271036));
#49491=CARTESIAN_POINT('Ctrl Pts',(1.03787211072146,-7.84262344383476,66.8997257525944));
#49492=CARTESIAN_POINT('Ctrl Pts',(1.23239961387978,-7.81688018690777,66.907615792875));
#49493=CARTESIAN_POINT('Ctrl Pts',(1.42609781534182,-7.78387799302661,66.9155058331556));
#49494=CARTESIAN_POINT('Ctrl Pts',(1.61838808196957,-7.74369040032844,66.9233958734362));
#49495=CARTESIAN_POINT('Ctrl Pts',(1.81059010084316,-7.70352125091845,66.9312822927414));
#49496=CARTESIAN_POINT('Ctrl Pts',(2.00138513582339,-7.65617334422175,66.9391687120465));
#49497=CARTESIAN_POINT('Ctrl Pts',(2.190203013785,-7.60177161972176,66.9470551313516));
#49498=CARTESIAN_POINT('Ctrl Pts',(2.37896919496613,-7.54738478996604,66.9549393914201));
#49499=CARTESIAN_POINT('Ctrl Pts',(2.56575896727935,-7.4859480870699,66.9628236514886));
#49500=CARTESIAN_POINT('Ctrl Pts',(2.75001535489471,-7.41763685737198,66.9707079115571));
#49501=CARTESIAN_POINT('Ctrl Pts',(2.93429325434585,-7.34931765237414,66.9785930921087));
#49502=CARTESIAN_POINT('Ctrl Pts',(3.11603685255183,-7.27412243024097,66.9864782726603));
#49503=CARTESIAN_POINT('Ctrl Pts',(3.29470666243988,-7.19227564881062,66.994363453212));
#49504=CARTESIAN_POINT('Ctrl Pts',(3.47339875772641,-7.11041865867104,67.0022496172784));
#49505=CARTESIAN_POINT('Ctrl Pts',(3.64901598693531,-7.02190859902328,67.0101357813448));
#49506=CARTESIAN_POINT('Ctrl Pts',(3.82104112217347,-6.92701708837645,67.0180219454112));
#49507=CARTESIAN_POINT('Ctrl Pts',(3.99311657685187,-6.83209782081088,67.0259104162763));
#49508=CARTESIAN_POINT('Ctrl Pts',(4.16159754186321,-6.73079354888768,67.0337988871415));
#49509=CARTESIAN_POINT('Ctrl Pts',(4.3259933504383,-6.62342075758166,67.0416873580066));
#49510=CARTESIAN_POINT('Ctrl Pts',(4.49046483016038,-6.51599854273897,67.0495794599231));
#49511=CARTESIAN_POINT('Ctrl Pts',(4.6508471180396,-6.40250243043345,67.0574715618397));
#49512=CARTESIAN_POINT('Ctrl Pts',(4.80668016985543,-6.28329107591862,67.0653636637563));
#49513=CARTESIAN_POINT('Ctrl Pts',(4.96269387919311,-6.16394151947787,67.073264915));
#49514=CARTESIAN_POINT('Ctrl Pts',(5.11414754425515,-6.03886369579897,67.0811661662437));
#49515=CARTESIAN_POINT('Ctrl Pts',(5.26061485798518,-5.90845600101631,67.0890674174874));
#49516=CARTESIAN_POINT('Ctrl Pts',(5.40717922524051,-5.77796189428149,67.0969739043313));
#49517=CARTESIAN_POINT('Ctrl Pts',(5.54875040633782,-5.64213111356376,67.1048803911752));
#49518=CARTESIAN_POINT('Ctrl Pts',(5.68494020387709,-5.50139762954305,67.112786878019));
#49519=CARTESIAN_POINT('Ctrl Pts',(5.82131762546363,-5.3604702617929,67.1207042573606));
#49520=CARTESIAN_POINT('Ctrl Pts',(5.95229862564975,-5.21462695504968,67.1286216367022));
#49521=CARTESIAN_POINT('Ctrl Pts',(6.07753565096896,-5.06433425152817,67.1365390160438));
#49522=CARTESIAN_POINT('Ctrl Pts',(6.13183709109418,-4.99916893623319,67.1399719073886));
#49523=CARTESIAN_POINT('Ctrl Pts',(6.1850592202821,-4.93316750144315,67.1434047987334));
#49524=CARTESIAN_POINT('Ctrl Pts',(6.23717630797825,-4.86636956089391,67.1468376900782));
#49525=CARTESIAN_POINT('Ctrl Pts',(6.35622544274216,-4.71378549724167,67.1546793167385));
#49526=CARTESIAN_POINT('Ctrl Pts',(6.46985956898129,-4.55658989670021,67.1625209433989));
#49527=CARTESIAN_POINT('Ctrl Pts',(6.57769584434812,-4.39520629541385,67.1703625700592));
#49528=CARTESIAN_POINT('Ctrl Pts',(6.68540515062556,-4.23401271115865,67.178194963795));
#49529=CARTESIAN_POINT('Ctrl Pts',(6.78733000555567,-4.06864123376018,67.1860273575307));
#49530=CARTESIAN_POINT('Ctrl Pts',(6.88312687573189,-3.89954938583643,67.1938597512665));
#49531=CARTESIAN_POINT('Ctrl Pts',(6.97882960089393,-3.73062371405594,67.201684447665));
#49532=CARTESIAN_POINT('Ctrl Pts',(7.0684161621868,-3.55798525633578,67.2095091440634));
#49533=CARTESIAN_POINT('Ctrl Pts',(7.1515854191098,-3.38212167036849,67.2173338404619));
#49534=CARTESIAN_POINT('Ctrl Pts',(7.23468912153964,-3.20639670110487,67.2251523693891));
#49535=CARTESIAN_POINT('Ctrl Pts',(7.31138544418473,-3.02745198285435,67.2329708983163));
#49536=CARTESIAN_POINT('Ctrl Pts',(7.38141833725328,-2.84580117549717,67.2407894272434));
#49537=CARTESIAN_POINT('Ctrl Pts',(7.45140964932264,-2.66425822063245,67.2486033140341));
#49538=CARTESIAN_POINT('Ctrl Pts',(7.51474528652795,-2.48001270434945,67.2564172008249));
#49539=CARTESIAN_POINT('Ctrl Pts',(7.57121657576523,-2.29359991342385,67.2642310876156));
#49540=CARTESIAN_POINT('Ctrl Pts',(7.62766531494716,-2.10726156065625,67.2720418541733));
#49541=CARTESIAN_POINT('Ctrl Pts',(7.67725506553332,-1.91875799363098,67.2798526207311));
#49542=CARTESIAN_POINT('Ctrl Pts',(7.71982638358571,-1.72864154968404,67.2876633872888));
#49543=CARTESIAN_POINT('Ctrl Pts',(7.76239600963511,-1.53853266194172,67.2954738434065));
#49544=CARTESIAN_POINT('Ctrl Pts',(7.79794767318894,-1.34681136617057,67.3032842995243));
#49545=CARTESIAN_POINT('Ctrl Pts',(7.82637251123595,-1.15404259686128,67.311094755642));
#49546=CARTESIAN_POINT('Ctrl Pts',(7.85479813318496,-0.961268511362553,
67.318905427157));
#49547=CARTESIAN_POINT('Ctrl Pts',(7.87609648597023,-0.767447242884585,
67.326716098672));
#49548=CARTESIAN_POINT('Ctrl Pts',(7.89021030313044,-0.573151264828211,
67.334526770187));
#49549=CARTESIAN_POINT('Ctrl Pts',(7.90432699516657,-0.378815710176739,
67.3423390326756));
#49550=CARTESIAN_POINT('Ctrl Pts',(7.91125621081637,-0.184005604321285,
67.3501512951642));
#49551=CARTESIAN_POINT('Ctrl Pts',(7.91099275847185,0.0107039901909737,
67.3579635576529));
#49552=CARTESIAN_POINT('Ctrl Pts',(7.910729206063,0.205487539190638,67.3657787873906));
#49553=CARTESIAN_POINT('Ctrl Pts',(7.90326754433039,0.400170149202142,67.3735940171284));
#49554=CARTESIAN_POINT('Ctrl Pts',(7.8886546475695,0.594179140815355,67.3814092468662));
#49555=CARTESIAN_POINT('Ctrl Pts',(7.87402585857392,0.788399126626365,67.3892329760457));
#49556=CARTESIAN_POINT('Ctrl Pts',(7.85223032742534,0.981943679856485,67.3970567052252));
#49557=CARTESIAN_POINT('Ctrl Pts',(7.82336666886793,1.17424655181365,67.4048804344047));
#49558=CARTESIAN_POINT('Ctrl Pts',(7.79448549804766,1.36666609846189,67.4127089104254));
#49559=CARTESIAN_POINT('Ctrl Pts',(7.75852771829795,1.55784211773711,67.4205373864461));
#49560=CARTESIAN_POINT('Ctrl Pts',(7.71564258387514,1.7472207982658,67.4283658624667));
#49561=CARTESIAN_POINT('Ctrl Pts',(7.67269842748793,1.93686011693613,67.4362051126645));
#49562=CARTESIAN_POINT('Ctrl Pts',(7.6228079637375,2.12469681724964,67.4440443628623));
#49563=CARTESIAN_POINT('Ctrl Pts',(7.56616995667815,2.31019332235661,67.4518836130601));
#49564=CARTESIAN_POINT('Ctrl Pts',(7.53441511530983,2.41419437041388,67.4562787914818));
#49565=CARTESIAN_POINT('Ctrl Pts',(7.50054009812716,2.51746015525612,67.4606739699035));
#49566=CARTESIAN_POINT('Ctrl Pts',(7.46458638868163,2.61989905261806,67.4650691483252));
#49567=CARTESIAN_POINT('Ctrl Pts',(7.39988146754456,2.80425557319383,67.472979032383));
#49568=CARTESIAN_POINT('Ctrl Pts',(7.32825542580156,2.9864624671935,67.4808889164408));
#49569=CARTESIAN_POINT('Ctrl Pts',(7.24986915251191,3.16596245578753,67.4887988004985));
#49570=CARTESIAN_POINT('Ctrl Pts',(7.17156809824657,3.34526729779213,67.4967000851859));
#49571=CARTESIAN_POINT('Ctrl Pts',(7.08652158824193,3.5218707828198,67.5046013698732));
#49572=CARTESIAN_POINT('Ctrl Pts',(6.99494008734091,3.69523127483398,67.5125026545605));
#49573=CARTESIAN_POINT('Ctrl Pts',(6.90344113283932,3.86843550947874,67.5203968174754));
#49574=CARTESIAN_POINT('Ctrl Pts',(6.80541908140425,4.03840227095019,67.5282909803904));
#49575=CARTESIAN_POINT('Ctrl Pts',(6.70113234262546,4.20461012777868,67.5361851433054));
#49576=CARTESIAN_POINT('Ctrl Pts',(6.59692022909914,4.37069904999071,67.5440736573343));
#49577=CARTESIAN_POINT('Ctrl Pts',(6.48645254216465,4.53303413548696,67.5519621713632));
#49578=CARTESIAN_POINT('Ctrl Pts',(6.3700335793673,4.69111854441274,67.5598506853922));
#49579=CARTESIAN_POINT('Ctrl Pts',(6.25367630154217,4.84911919179195,67.5677350196659));
#49580=CARTESIAN_POINT('Ctrl Pts',(6.13137423526002,5.00287337334444,67.5756193539396));
#49581=CARTESIAN_POINT('Ctrl Pts',(6.00347510220884,5.15191301335325,67.5835036882133));
#49582=CARTESIAN_POINT('Ctrl Pts',(5.87561998684066,5.30090135997584,67.5913853090196));
#49583=CARTESIAN_POINT('Ctrl Pts',(5.7421718682063,5.44517813736502,67.5992669298259));
#49584=CARTESIAN_POINT('Ctrl Pts',(5.60351904371278,5.58430795414689,67.6071485506323));
#49585=CARTESIAN_POINT('Ctrl Pts',(5.46486440323129,5.72343959316408,67.6150302746671));
#49586=CARTESIAN_POINT('Ctrl Pts',(5.3210051581103,5.85742388651197,67.622911998702));
#49587=CARTESIAN_POINT('Ctrl Pts',(5.17236719654218,5.98586155738123,67.6307937227369));
#49588=CARTESIAN_POINT('Ctrl Pts',(5.02372028099649,6.1143069653589,67.6386759215682));
#49589=CARTESIAN_POINT('Ctrl Pts',(4.87029433616513,6.23720485891626,67.6465581203995));
#49590=CARTESIAN_POINT('Ctrl Pts',(4.71254915070054,6.35419558262347,67.6544403192309));
#49591=CARTESIAN_POINT('Ctrl Pts',(4.55476791880469,6.47121303993949,67.6623243192274));
#49592=CARTESIAN_POINT('Ctrl Pts',(4.392665756726,6.58232043204918,67.6702083192239));
#49593=CARTESIAN_POINT('Ctrl Pts',(4.22673249676059,6.68720071486029,67.6780923192205));
#49594=CARTESIAN_POINT('Ctrl Pts',(4.06073339729916,6.79212261238424,67.6859794474542));
#49595=CARTESIAN_POINT('Ctrl Pts',(3.89090046245507,6.89081229309079,67.6938665756878));
#49596=CARTESIAN_POINT('Ctrl Pts',(3.71774944231857,6.98299792955289,67.7017537039215));
#49597=CARTESIAN_POINT('Ctrl Pts',(3.54441368982391,7.07528191755805,67.70964924682));
#49598=CARTESIAN_POINT('Ctrl Pts',(3.36775308580008,7.16104783883787,67.7175447897185));
#49599=CARTESIAN_POINT('Ctrl Pts',(3.18830575535423,7.24007095340751,67.725440332617));
#49600=CARTESIAN_POINT('Ctrl Pts',(3.00874914770108,7.31914219031617,67.7333406836276));
#49601=CARTESIAN_POINT('Ctrl Pts',(2.82640275028521,7.39146230753328,67.7412410346381));
#49602=CARTESIAN_POINT('Ctrl Pts',(2.64182152784425,7.45685590681614,67.7491413856487));
#49603=CARTESIAN_POINT('Ctrl Pts',(2.45699997289216,7.5223346513143,67.7570520232484));
#49604=CARTESIAN_POINT('Ctrl Pts',(2.26993810896296,7.58086876098412,67.7649626608482));
#49605=CARTESIAN_POINT('Ctrl Pts',(2.08120392160856,7.63233327604876,67.7728732984479));
#49606=CARTESIAN_POINT('Ctrl Pts',(1.99827805121023,7.65494571190994,67.7763490678226));
#49607=CARTESIAN_POINT('Ctrl Pts',(1.91502944209998,7.67619400301762,67.7798248371972));
#49608=CARTESIAN_POINT('Ctrl Pts',(1.83150667409454,7.69607070541501,67.7833006065719));
#49609=CARTESIAN_POINT('Ctrl Pts',(1.64143253937006,7.7413044434673,67.7912104720154));
#49610=CARTESIAN_POINT('Ctrl Pts',(1.44942515025329,7.77955349249484,67.799120337459));
#49611=CARTESIAN_POINT('Ctrl Pts',(1.25604031289521,7.81065194029168,67.8070302029025));
#49612=CARTESIAN_POINT('Ctrl Pts',(1.06286564471425,7.84171659053089,67.8149314719642));
#49613=CARTESIAN_POINT('Ctrl Pts',(0.868316847569201,7.86564606426011,67.8228327410258));
#49614=CARTESIAN_POINT('Ctrl Pts',(0.672963367964798,7.88232461304262,67.8307340100875));
#49615=CARTESIAN_POINT('Ctrl Pts',(0.477785895686628,7.8989881349785,67.8386281603548));
#49616=CARTESIAN_POINT('Ctrl Pts',(0.281805526730041,7.90841371673059,67.8465223106221));
#49617=CARTESIAN_POINT('Ctrl Pts',(0.0856006284762027,7.91053686752072,
67.8544164608895));
#49618=CARTESIAN_POINT('Ctrl Pts',(-0.110463943530358,7.91265849982795,
67.8623049652403));
#49619=CARTESIAN_POINT('Ctrl Pts',(-0.306752381366858,7.90748810281787,
67.8701934695911));
#49620=CARTESIAN_POINT('Ctrl Pts',(-0.502682199417825,7.89501308462427,
67.8780819739418));
#49621=CARTESIAN_POINT('Ctrl Pts',(-0.698508276873272,7.88254467168264,
67.8859663015004));
#49622=CARTESIAN_POINT('Ctrl Pts',(-0.893975769459908,7.86277936616138,
67.893850629059));
#49623=CARTESIAN_POINT('Ctrl Pts',(-1.0885029155257,7.83575665796814,67.9017349566175));
#49624=CARTESIAN_POINT('Ctrl Pts',(-1.28296318618163,7.80874323976204,67.9096165736668));
#49625=CARTESIAN_POINT('Ctrl Pts',(-1.47648341333973,7.77447743884248,67.9174981907161));
#49626=CARTESIAN_POINT('Ctrl Pts',(-1.66848739715556,7.73305054978519,67.9253798077654));
#49627=CARTESIAN_POINT('Ctrl Pts',(-1.86049400352918,7.69162309488334,67.9332615324686));
#49628=CARTESIAN_POINT('Ctrl Pts',(-2.05098398619798,7.64303442079796,67.9411432571719));
#49629=CARTESIAN_POINT('Ctrl Pts',(-2.23939120623307,7.5874269700239,67.9490249818752));
#49630=CARTESIAN_POINT('Ctrl Pts',(-2.42780984186723,7.53181614999274,67.9569071841324));
#49631=CARTESIAN_POINT('Ctrl Pts',(-2.61414513217561,7.46918580299793,67.9647893863896));
#49632=CARTESIAN_POINT('Ctrl Pts',(-2.79784594470447,7.39972831053281,67.9726715886468));
#49633=CARTESIAN_POINT('Ctrl Pts',(-2.98158879906702,7.33025492200111,67.9805555948276));
#49634=CARTESIAN_POINT('Ctrl Pts',(-3.16269565143175,7.25395139659806,67.9884396010085));
#49635=CARTESIAN_POINT('Ctrl Pts',(-3.34063497619055,7.17105842647042,67.9963236071893));
#49636=CARTESIAN_POINT('Ctrl Pts',(-3.5186449665065,7.08813253681852,68.0042107443682));
#49637=CARTESIAN_POINT('Ctrl Pts',(-3.6934846101381,6.99861213367762,68.0120978815472));
#49638=CARTESIAN_POINT('Ctrl Pts',(-3.86464641054531,6.90278415724114,68.0199850187261));
#49639=CARTESIAN_POINT('Ctrl Pts',(-4.03599091049004,6.80685389322101,68.0278805747013));
#49640=CARTESIAN_POINT('Ctrl Pts',(-4.20364942462189,6.70460277635662,68.0357761306764));
#49641=CARTESIAN_POINT('Ctrl Pts',(-4.36714197427072,6.59636202588691,68.0436716866516));
#49642=CARTESIAN_POINT('Ctrl Pts',(-4.53073413426365,6.48805532807939,68.0515720531153));
#49643=CARTESIAN_POINT('Ctrl Pts',(-4.6901549899213,6.37375192188635,68.0594724195791));
#49644=CARTESIAN_POINT('Ctrl Pts',(-4.84495696967043,6.25382386720652,68.0673727860428));
#49645=CARTESIAN_POINT('Ctrl Pts',(-4.99996057685379,6.13373960789678,68.0752834426244));
#49646=CARTESIAN_POINT('Ctrl Pts',(-5.15033302757959,6.00801628741753,68.0831940992061));
#49647=CARTESIAN_POINT('Ctrl Pts',(-5.29566214425518,5.87706418664137,68.0911047557877));
#49648=CARTESIAN_POINT('Ctrl Pts',(-5.3595165831028,5.81952669448387,68.0945805254648));
#49649=CARTESIAN_POINT('Ctrl Pts',(-5.4223978937926,5.76098022411872,68.0980562951418));
#49650=CARTESIAN_POINT('Ctrl Pts',(-5.48427355201924,5.70146162020076,68.1015320648189));
#49651=CARTESIAN_POINT('Ctrl Pts',(-5.62176696829789,5.56920579586931,68.1092555454379));
#49652=CARTESIAN_POINT('Ctrl Pts',(-5.75470897477497,5.43174660576841,68.1169790260568));
#49653=CARTESIAN_POINT('Ctrl Pts',(-5.88266780366062,5.28943669134764,68.1247025066757));
#49654=CARTESIAN_POINT('Ctrl Pts',(-6.01048128585462,5.14728842482121,68.1324172142982));
#49655=CARTESIAN_POINT('Ctrl Pts',(-6.13332261708519,5.00030066704751,68.1401319219207));
#49656=CARTESIAN_POINT('Ctrl Pts',(-6.25079385755168,4.84886555293031,68.1478466295431));
#49657=CARTESIAN_POINT('Ctrl Pts',(-6.36815590208531,4.69757120602123,68.1555541659236));
#49658=CARTESIAN_POINT('Ctrl Pts',(-6.48015757249965,4.54183801652948,68.163261702304));
#49659=CARTESIAN_POINT('Ctrl Pts',(-6.58643847852492,4.38209415332514,68.1709692386845));
#49660=CARTESIAN_POINT('Ctrl Pts',(-6.6935537676721,4.22109618354351,68.1787372848828));
#49661=CARTESIAN_POINT('Ctrl Pts',(-6.79485781584916,4.05602455587056,68.1865053310811));
#49662=CARTESIAN_POINT('Ctrl Pts',(-6.89002303352795,3.8873517460418,68.1942733772794));
#49663=CARTESIAN_POINT('Ctrl Pts',(-6.98433017398566,3.72019981011489,68.2019713812537));
#49664=CARTESIAN_POINT('Ctrl Pts',(-7.07260854612563,3.54951168638046,68.209669385228));
#49665=CARTESIAN_POINT('Ctrl Pts',(-7.15458292517099,3.37577608363643,68.2173673892023));
#49666=CARTESIAN_POINT('Ctrl Pts',(-7.23653652760632,3.20208451461256,68.2250634420984));
#49667=CARTESIAN_POINT('Ctrl Pts',(-7.31218916276314,3.02534733151858,68.2327594949945));
#49668=CARTESIAN_POINT('Ctrl Pts',(-7.38131200158983,2.84607697281466,68.2404555478905));
#49669=CARTESIAN_POINT('Ctrl Pts',(-7.4504301815942,2.66681869678507,68.248151082079));
#49670=CARTESIAN_POINT('Ctrl Pts',(-7.51301931185719,2.48502792351462,68.2558466162675));
#49671=CARTESIAN_POINT('Ctrl Pts',(-7.56889907121512,2.30123615688587,68.2635421504559));
#49672=CARTESIAN_POINT('Ctrl Pts',(-7.62569483843707,2.11443158731187,68.2713638335383));
#49673=CARTESIAN_POINT('Ctrl Pts',(-7.6755592219986,1.92556021451917,68.2791855166206));
#49674=CARTESIAN_POINT('Ctrl Pts',(-7.71835601555024,1.73519492196681,68.287007199703));
#49675=CARTESIAN_POINT('Ctrl Pts',(-7.7604946658136,1.54775713003351,68.2947085983482));
#49676=CARTESIAN_POINT('Ctrl Pts',(-7.79578150902447,1.35887140329898,68.3024099969934));
#49677=CARTESIAN_POINT('Ctrl Pts',(-7.82413840397329,1.16909333907534,68.3101113956386));
#49678=CARTESIAN_POINT('Ctrl Pts',(-7.85315963795424,0.97486919654394,68.3179932209396));
#49679=CARTESIAN_POINT('Ctrl Pts',(-7.87492218388578,0.779710795304858,
68.3258750462405));
#49680=CARTESIAN_POINT('Ctrl Pts',(-7.88939866528744,0.584217168663089,
68.3337568715414));
#49681=CARTESIAN_POINT('Ctrl Pts',(-7.9038751466891,0.388723542021395,68.3416386968424));
#49682=CARTESIAN_POINT('Ctrl Pts',(-7.91106559513061,0.192895094132201,
68.3495205221433));
#49683=CARTESIAN_POINT('Ctrl Pts',(-7.91099954886372,-0.00267168074885584,
68.3574023474442));
#49684=CARTESIAN_POINT('',(-7.91835117330158,0.00158043531916788,70.357742247265));
#49685=CARTESIAN_POINT('Ctrl Pts',(-7.9109995297644,-0.00265674798181834,
68.3577753899841));
#49686=CARTESIAN_POINT('Ctrl Pts',(-7.91022048351088,-2.20343307818681,
68.4463271929765));
#49687=CARTESIAN_POINT('Ctrl Pts',(-6.94148933469359,-4.38669862313552,
68.5348789959691));
#49688=CARTESIAN_POINT('Ctrl Pts',(-3.67820201487734,-7.34180684107901,
68.7120182346942));
#49689=CARTESIAN_POINT('Ctrl Pts',(-1.40868175871169,-8.08992666571429,
68.8006056704269));
#49690=CARTESIAN_POINT('Ctrl Pts',(2.97309270521765,-7.65454228025058,68.9777805418923));
#49691=CARTESIAN_POINT('Ctrl Pts',(5.05102072675991,-6.47444880833913,69.066367977625));
#49692=CARTESIAN_POINT('Ctrl Pts',(7.66951518848024,-2.93425195367288,69.2435428490905));
#49693=CARTESIAN_POINT('Ctrl Pts',(8.18956872247094,-0.601881960095041,
69.3321302848232));
#49694=CARTESIAN_POINT('Ctrl Pts',(7.32306689761173,3.71537198232768,69.5093051562886));
#49695=CARTESIAN_POINT('Ctrl Pts',(5.94329958849969,5.66643518936744,69.5978925920213));
#49696=CARTESIAN_POINT('Ctrl Pts',(2.16154501637579,7.92205913233063,69.7750674634867));
#49697=CARTESIAN_POINT('Ctrl Pts',(-0.210816529302805,8.20894963712989,
69.8636548992195));
#49698=CARTESIAN_POINT('Ctrl Pts',(-4.42123908576595,6.91982244717722,70.0408297706849));
#49699=CARTESIAN_POINT('Ctrl Pts',(-6.22631625634286,5.35390358803395,70.1294172064176));
#49700=CARTESIAN_POINT('Ctrl Pts',(-7.65294264462806,2.31383904225023,70.2645374591378));
#49701=CARTESIAN_POINT('Ctrl Pts',(-7.91075848970524,1.15811126578363,70.3110702761253));
#49702=CARTESIAN_POINT('Ctrl Pts',(-7.91099983040495,0.00162536129911048,
70.3576030931128));
#49703=CARTESIAN_POINT('',(-7.90558067573546,0.00500151420475855,72.3576672233085));
#49704=CARTESIAN_POINT('Ctrl Pts',(-7.92187310646681,0.00155891186407059,
70.357808914217));
#49705=CARTESIAN_POINT('Ctrl Pts',(-7.90511105438765,-2.38948601125333,
70.4543338530758));
#49706=CARTESIAN_POINT('Ctrl Pts',(-5.47263506421283,-7.43816085005188,
70.6569359446836));
#49707=CARTESIAN_POINT('Ctrl Pts',(1.6316743039881,-8.57466520584624,70.9125766126657));
#49708=CARTESIAN_POINT('Ctrl Pts',(6.11859740475592,-5.49545041821264,71.1247309181634));
#49709=CARTESIAN_POINT('Ctrl Pts',(8.70002820540714,-0.704807661137227,
71.3368852236616));
#49710=CARTESIAN_POINT('Ctrl Pts',(6.73925246187953,6.4964979269881,71.6020781055336));
#49711=CARTESIAN_POINT('Ctrl Pts',(-1.83418328520544,9.17844853159298,71.9203095637806));
#49712=CARTESIAN_POINT('Ctrl Pts',(-7.27268681968312,4.62039446097428,72.1721722487799));
#49713=CARTESIAN_POINT('Ctrl Pts',(-7.90629361575619,0.994517640416839,
72.3179577810305));
#49714=CARTESIAN_POINT('Ctrl Pts',(-7.90104139764401,0.00502514377492854,
72.3576661605321));
#49715=CARTESIAN_POINT('',(-7.90643489614128,-0.00593696359886245,74.3576698040782));
#49716=CARTESIAN_POINT('Ctrl Pts',(-7.91099843674435,0.00497331162246579,
72.3576684917633));
#49717=CARTESIAN_POINT('Ctrl Pts',(-7.91112856116881,-0.202014345030353,
72.3659644912846));
#49718=CARTESIAN_POINT('Ctrl Pts',(-7.90312996393247,-0.409024146823264,
72.3742604908059));
#49719=CARTESIAN_POINT('Ctrl Pts',(-7.88702893860843,-0.615382418950373,
72.3825564903272));
#49720=CARTESIAN_POINT('Ctrl Pts',(-7.87157697295438,-0.813422038736245,
72.3905180640213));
#49721=CARTESIAN_POINT('Ctrl Pts',(-7.84866306220442,-1.01086127600091,
72.3984796377155));
#49722=CARTESIAN_POINT('Ctrl Pts',(-7.81836350731622,-1.20710938504594,
72.4064412114096));
#49723=CARTESIAN_POINT('Ctrl Pts',(-7.78805591091661,-1.40340957840095,
72.414404898108));
#49724=CARTESIAN_POINT('Ctrl Pts',(-7.75035881338431,-1.59851768184371,
72.4223685848063));
#49725=CARTESIAN_POINT('Ctrl Pts',(-7.70539985696176,-1.79185212680445,
72.4303322715046));
#49726=CARTESIAN_POINT('Ctrl Pts',(-7.66042202043323,-1.98526776081186,
72.438299302481));
#49727=CARTESIAN_POINT('Ctrl Pts',(-7.60817632116129,-2.17690792500901,
72.4462663334573));
#49728=CARTESIAN_POINT('Ctrl Pts',(-7.54884067694061,-2.36620485887569,
72.4542333644336));
#49729=CARTESIAN_POINT('Ctrl Pts',(-7.48947094380602,-2.5556105457013,72.462204972548));
#49730=CARTESIAN_POINT('Ctrl Pts',(-7.42300324516288,-2.74266999891853,
72.4701765806623));
#49731=CARTESIAN_POINT('Ctrl Pts',(-7.34966428105129,-2.92683377659868,
72.4781481887767));
#49732=CARTESIAN_POINT('Ctrl Pts',(-7.27623264649205,-3.11123026195236,
72.4861298697425));
#49733=CARTESIAN_POINT('Ctrl Pts',(-7.19591252544145,-3.29272345089769,
72.4941115507083));
#49734=CARTESIAN_POINT('Ctrl Pts',(-7.10897794312644,-3.47078573296334,
72.5020932316741));
#49735=CARTESIAN_POINT('Ctrl Pts',(-7.0219791373449,-3.64897955965377,72.5100808091567));
#49736=CARTESIAN_POINT('Ctrl Pts',(-6.92835628278054,-3.8237371302206,72.5180683866393));
#49737=CARTESIAN_POINT('Ctrl Pts',(-6.82842792612095,-3.99455793020598,
72.5260559641218));
#49738=CARTESIAN_POINT('Ctrl Pts',(-6.72836088398868,-4.16561580367263,
72.534054627156));
#49739=CARTESIAN_POINT('Ctrl Pts',(-6.62197103827709,-4.33272571100648,
72.5420532901902));
#49740=CARTESIAN_POINT('Ctrl Pts',(-6.50961926987508,-4.49541744015736,
72.5500519532245));
#49741=CARTESIAN_POINT('Ctrl Pts',(-6.47815304877411,-4.54098231193084,
72.5522921289077));
#49742=CARTESIAN_POINT('Ctrl Pts',(-6.44621941909069,-4.58620083614637,
72.554532304591));
#49743=CARTESIAN_POINT('Ctrl Pts',(-6.41382684745901,-4.63106317931574,
72.5567724802742));
#49744=CARTESIAN_POINT('Ctrl Pts',(-6.30047866556183,-4.78804562244238,
72.5646113096119));
#49745=CARTESIAN_POINT('Ctrl Pts',(-6.18119242386372,-4.94110127454116,
72.5724501389496));
#49746=CARTESIAN_POINT('Ctrl Pts',(-6.05627048094666,-5.08974546137762,
72.5802889682873));
#49747=CARTESIAN_POINT('Ctrl Pts',(-5.93148857345526,-5.23822302054653,
72.5881190104273));
#49748=CARTESIAN_POINT('Ctrl Pts',(-5.80108376814313,-5.38229869488082,
72.5959490525673));
#49749=CARTESIAN_POINT('Ctrl Pts',(-5.66540187578194,-5.52151633031059,
72.6037790947074));
#49750=CARTESIAN_POINT('Ctrl Pts',(-5.52984567315883,-5.6606050006454,72.6116018834407));
#49751=CARTESIAN_POINT('Ctrl Pts',(-5.38902236232815,-5.79484434408087,
72.619424672174));
#49752=CARTESIAN_POINT('Ctrl Pts',(-5.2433183435068,-5.92381074551214,72.6272474609074));
#49753=CARTESIAN_POINT('Ctrl Pts',(-5.09772095574409,-6.05268276503121,
72.6350645246631));
#49754=CARTESIAN_POINT('Ctrl Pts',(-4.94725023629629,-6.1762892963495,72.6428815884189));
#49755=CARTESIAN_POINT('Ctrl Pts',(-4.79232993588311,-6.29424298749569,
72.6506986521746));
#49756=CARTESIAN_POINT('Ctrl Pts',(-4.63749288684988,-6.41213329245212,
72.658511515181));
#49757=CARTESIAN_POINT('Ctrl Pts',(-4.47821129915083,-6.5243765959394,72.6663243781874));
#49758=CARTESIAN_POINT('Ctrl Pts',(-4.31494268944502,-6.63062520331265,
72.6741372411939));
#49759=CARTESIAN_POINT('Ctrl Pts',(-4.15173007737677,-6.73683736968835,
72.6819474245556));
#49760=CARTESIAN_POINT('Ctrl Pts',(-3.98453346235306,-6.83705874489097,
72.6897576079173));
#49761=CARTESIAN_POINT('Ctrl Pts',(-3.81384023064639,-6.93098432368037,
72.697567791279));
#49762=CARTESIAN_POINT('Ctrl Pts',(-3.64313930051956,-7.02491413859889,
72.705378326887));
#49763=CARTESIAN_POINT('Ctrl Pts',(-3.46894174238145,-7.1125474121264,72.7131888624951));
#49764=CARTESIAN_POINT('Ctrl Pts',(-3.29176094134949,-7.19362432331616,
72.7209993981032));
#49765=CARTESIAN_POINT('Ctrl Pts',(-3.11456593907785,-7.27470773291118,
72.7288105597344));
#49766=CARTESIAN_POINT('Ctrl Pts',(-2.93438753736343,-7.3492335861182,72.7366217213657));
#49767=CARTESIAN_POINT('Ctrl Pts',(-2.75176048389116,-7.4169896345684,72.7444328829969));
#49768=CARTESIAN_POINT('Ctrl Pts',(-2.56908662845072,-7.48476304691055,
72.7522460464003));
#49769=CARTESIAN_POINT('Ctrl Pts',(-2.38396320107523,-7.54576307590045,
72.7600592098036));
#49770=CARTESIAN_POINT('Ctrl Pts',(-2.19694168013937,-7.59982685684789,
72.767872373207));
#49771=CARTESIAN_POINT('Ctrl Pts',(-2.00983928999057,-7.65391401529429,
72.7756889150684));
#49772=CARTESIAN_POINT('Ctrl Pts',(-1.82083750901631,-7.70105885339732,
72.7835054569299));
#49773=CARTESIAN_POINT('Ctrl Pts',(-1.63049975986896,-7.74114923852184,
72.7913219987913));
#49774=CARTESIAN_POINT('Ctrl Pts',(-1.43993988328478,-7.78128640981742,
72.799147662692));
#49775=CARTESIAN_POINT('Ctrl Pts',(-1.24804126890946,-7.8143526125569,72.8069733265927));
#49776=CARTESIAN_POINT('Ctrl Pts',(-1.0553753461434,-7.84028723190373,72.8147989904933));
#49777=CARTESIAN_POINT('Ctrl Pts',(-0.862583837594134,-7.86623875626125,
72.8226297554109));
#49778=CARTESIAN_POINT('Ctrl Pts',(-0.669024372869679,-7.88504939954695,
72.8304605203284));
#49779=CARTESIAN_POINT('Ctrl Pts',(-0.475270250639864,-7.89671065627054,
72.838291285246));
#49780=CARTESIAN_POINT('Ctrl Pts',(-0.281236174430739,-7.90838876226261,
72.8461333647811));
#49781=CARTESIAN_POINT('Ctrl Pts',(-0.0870072292878414,-7.91289684099874,
72.8539754443163));
#49782=CARTESIAN_POINT('Ctrl Pts',(0.106845339014254,-7.91027844475344,
72.8618175238514));
#49783=CARTESIAN_POINT('Ctrl Pts',(0.215499356907363,-7.90881083834007,
72.866212995408));
#49784=CARTESIAN_POINT('Ctrl Pts',(0.324035244514684,-7.90510532434733,
72.8706084669645));
#49785=CARTESIAN_POINT('Ctrl Pts',(0.432353660334651,-7.8991766224332,72.875003938521));
#49786=CARTESIAN_POINT('Ctrl Pts',(0.627441848176251,-7.88849866242129,
72.8829204555249));
#49787=CARTESIAN_POINT('Ctrl Pts',(0.822409615450803,-7.8705741175999,72.8908369725288));
#49788=CARTESIAN_POINT('Ctrl Pts',(1.0166768073984,-7.84539924218635,72.8987534895327));
#49789=CARTESIAN_POINT('Ctrl Pts',(1.21072019175754,-7.82025336975628,72.9066608862288));
#49790=CARTESIAN_POINT('Ctrl Pts',(1.40406427008146,-7.78787384782983,72.9145682829249));
#49791=CARTESIAN_POINT('Ctrl Pts',(1.59612977651121,-7.74830889527091,72.922475679621));
#49792=CARTESIAN_POINT('Ctrl Pts',(1.78800960272789,-7.70878219231213,72.9303754318049));
#49793=CARTESIAN_POINT('Ctrl Pts',(1.97861298425648,-7.66208396562109,72.9382751839889));
#49794=CARTESIAN_POINT('Ctrl Pts',(2.16736637655079,-7.60831413585146,72.9461749361728));
#49795=CARTESIAN_POINT('Ctrl Pts',(2.35597225546501,-7.55458632794559,72.9540685145914));
#49796=CARTESIAN_POINT('Ctrl Pts',(2.54273069577453,-7.49379802149107,72.96196209301));
#49797=CARTESIAN_POINT('Ctrl Pts',(2.72707866063372,-7.42610011908782,72.9698556714287));
#49798=CARTESIAN_POINT('Ctrl Pts',(2.91131669508752,-7.35844258630765,72.9777445427474));
#49799=CARTESIAN_POINT('Ctrl Pts',(3.09314679574391,-7.28388378614634,72.9856334140662));
#49800=CARTESIAN_POINT('Ctrl Pts',(3.27202113046216,-7.20262443292784,72.993522285385));
#49801=CARTESIAN_POINT('Ctrl Pts',(3.45082191905448,-7.12139849037519,73.0014079131086));
#49802=CARTESIAN_POINT('Ctrl Pts',(3.62666905050166,-7.0334776276693,73.0092935408323));
#49803=CARTESIAN_POINT('Ctrl Pts',(3.79903446250772,-6.93911076094615,73.0171791685559));
#49804=CARTESIAN_POINT('Ctrl Pts',(3.97138454308658,-6.84475228789509,73.0250640948748));
#49805=CARTESIAN_POINT('Ctrl Pts',(4.14025321600823,-6.74394911287841,73.0329490211936));
#49806=CARTESIAN_POINT('Ctrl Pts',(4.30513637538387,-6.63699644337306,73.0408339475124));
#49807=CARTESIAN_POINT('Ctrl Pts',(4.47001896408724,-6.53004414403846,73.0487188465409));
#49808=CARTESIAN_POINT('Ctrl Pts',(4.63091577721423,-6.41694257974099,73.0566037455695));
#49809=CARTESIAN_POINT('Ctrl Pts',(4.78735101332433,-6.29803074581432,73.064488644598));
#49810=CARTESIAN_POINT('Ctrl Pts',(4.94381195425236,-6.17909937276644,73.0723748392419));
#49811=CARTESIAN_POINT('Ctrl Pts',(5.09580958298998,-6.05435603636255,73.0802610338858));
#49812=CARTESIAN_POINT('Ctrl Pts',(5.24290036559014,-5.92418068229648,73.0881472285297));
#49813=CARTESIAN_POINT('Ctrl Pts',(5.39003999613593,-5.79396209779472,73.0960360421305));
#49814=CARTESIAN_POINT('Ctrl Pts',(5.53226927578104,-5.65830812962327,73.1039248557311));
#49815=CARTESIAN_POINT('Ctrl Pts',(5.66918061027377,-5.51763646936765,73.1118136693318));
#49816=CARTESIAN_POINT('Ctrl Pts',(5.80622446450122,-5.37682864966863,73.1197101187027));
#49817=CARTESIAN_POINT('Ctrl Pts',(5.93793985156297,-5.23099368398513,73.1276065680736));
#49818=CARTESIAN_POINT('Ctrl Pts',(6.06395795657046,-5.0805841102127,73.1355030174445));
#49819=CARTESIAN_POINT('Ctrl Pts',(6.190045712928,-4.93009140370412,73.1434038312546));
#49820=CARTESIAN_POINT('Ctrl Pts',(6.31042969792822,-4.77501931958236,73.1513046450647));
#49821=CARTESIAN_POINT('Ctrl Pts',(6.4247835647362,-4.61585064167978,73.1592054588749));
#49822=CARTESIAN_POINT('Ctrl Pts',(6.53927638915582,-4.45648854924783,73.1671158733941));
#49823=CARTESIAN_POINT('Ctrl Pts',(6.64772426864196,-4.29302020600155,73.1750262879134));
#49824=CARTESIAN_POINT('Ctrl Pts',(6.74984549421544,-4.12595525959984,73.1829367024327));
#49825=CARTESIAN_POINT('Ctrl Pts',(6.79416324287183,-4.05345375697541,73.1863696005444));
#49826=CARTESIAN_POINT('Ctrl Pts',(6.83729008001318,-3.98027519227827,73.1898024986561));
#49827=CARTESIAN_POINT('Ctrl Pts',(6.87920577123963,-3.90646246071089,73.1932353967677));
#49828=CARTESIAN_POINT('Ctrl Pts',(6.98072775338417,-3.72768418944873,73.2015500543721));
#49829=CARTESIAN_POINT('Ctrl Pts',(7.07536409182775,-3.54479248452029,73.2098647119764));
#49830=CARTESIAN_POINT('Ctrl Pts',(7.16278704580388,-3.35833332718242,73.2181793695808));
#49831=CARTESIAN_POINT('Ctrl Pts',(7.25010194455162,-3.17210463433832,73.2264837502248));
#49832=CARTESIAN_POINT('Ctrl Pts',(7.33022111695024,-2.98231754762191,73.2347881308689));
#49833=CARTESIAN_POINT('Ctrl Pts',(7.40286217443645,-2.78954344405998,73.243092511513));
#49834=CARTESIAN_POINT('Ctrl Pts',(7.47541824782413,-2.59699487043909,73.2513871767106));
#49835=CARTESIAN_POINT('Ctrl Pts',(7.54051355296825,-2.40146652341505,73.2596818419082));
#49836=CARTESIAN_POINT('Ctrl Pts',(7.59791302528611,-2.20355137452878,73.2679765071058));
#49837=CARTESIAN_POINT('Ctrl Pts',(7.65522606353893,-2.00593425296159,73.2762586819163));
#49838=CARTESIAN_POINT('Ctrl Pts',(7.70486631435656,-1.8059377829597,73.2845408567268));
#49839=CARTESIAN_POINT('Ctrl Pts',(7.74664790199489,-1.60417183696703,73.2928230315373));
#49840=CARTESIAN_POINT('Ctrl Pts',(7.78839095501682,-1.40259197708958,73.3010975678054));
#49841=CARTESIAN_POINT('Ctrl Pts',(7.82228973910568,-1.19924618177941,73.3093721040735));
#49842=CARTESIAN_POINT('Ctrl Pts',(7.84820854440072,-0.994758082950565,
73.3176466403415));
#49843=CARTESIAN_POINT('Ctrl Pts',(7.87409753489035,-0.790505209966683,
73.3259116582817));
#49844=CARTESIAN_POINT('Ctrl Pts',(7.89202482691748,-0.585112945734738,
73.3341766762218));
#49845=CARTESIAN_POINT('Ctrl Pts',(7.9019059580874,-0.379213962747772,73.3424416941619));
#49846=CARTESIAN_POINT('Ctrl Pts',(7.90585498741587,-0.296925699538259,
73.3457448380717));
#49847=CARTESIAN_POINT('Ctrl Pts',(7.90851943387131,-0.214556603258294,
73.3490479819815));
#49848=CARTESIAN_POINT('Ctrl Pts',(7.90989621070171,-0.132147402270342,
73.3523511258913));
#49849=CARTESIAN_POINT('Ctrl Pts',(7.91334156146494,0.0740796326801837,
73.360617163741));
#49850=CARTESIAN_POINT('Ctrl Pts',(7.9087155022605,0.280324671188554,73.3688832015908));
#49851=CARTESIAN_POINT('Ctrl Pts',(7.89606065348131,0.485949746933029,73.3771492394405));
#49852=CARTESIAN_POINT('Ctrl Pts',(7.88339442547667,0.691759720508842,73.385422710102));
#49853=CARTESIAN_POINT('Ctrl Pts',(7.86268501313782,0.896948325257189,73.3936961807634));
#49854=CARTESIAN_POINT('Ctrl Pts',(7.8340268165024,1.10088366248269,73.4019696514249));
#49855=CARTESIAN_POINT('Ctrl Pts',(7.8053409857925,1.30501564726314,73.4102510998983));
#49856=CARTESIAN_POINT('Ctrl Pts',(7.76869110950227,1.50789166131395,73.4185325483718));
#49857=CARTESIAN_POINT('Ctrl Pts',(7.72422265443761,1.70889010315842,73.4268139968452));
#49858=CARTESIAN_POINT('Ctrl Pts',(7.6796801631823,1.91022319029111,73.4351092332251));
#49859=CARTESIAN_POINT('Ctrl Pts',(7.62729313179226,2.10967216826892,73.4434044696049));
#49860=CARTESIAN_POINT('Ctrl Pts',(7.56725742111864,2.30662873530287,73.4516997059848));
#49861=CARTESIAN_POINT('Ctrl Pts',(7.50716726540431,2.50376391783397,73.4600024651287));
#49862=CARTESIAN_POINT('Ctrl Pts',(7.43941467652915,2.69840189908309,73.4683052242726));
#49863=CARTESIAN_POINT('Ctrl Pts',(7.36424410043606,2.8899532572678,73.4766079834164));
#49864=CARTESIAN_POINT('Ctrl Pts',(7.28895824773573,3.08179836590421,73.4849234751207));
#49865=CARTESIAN_POINT('Ctrl Pts',(7.20623178261639,3.27054711904865,73.493238966825));
#49866=CARTESIAN_POINT('Ctrl Pts',(7.1163564409016,3.45563192571755,73.5015544585294));
#49867=CARTESIAN_POINT('Ctrl Pts',(7.08064478154718,3.52917474003488,73.5048585906911));
#49868=CARTESIAN_POINT('Ctrl Pts',(7.04380492569719,3.60213936756197,73.5081627228529));
#49869=CARTESIAN_POINT('Ctrl Pts',(7.00585711220989,3.67449141015436,73.5114668550147));
#49870=CARTESIAN_POINT('Ctrl Pts',(6.91501452263554,3.84769366625495,73.5193765576902));
#49871=CARTESIAN_POINT('Ctrl Pts',(6.81763001644092,4.01774461916287,73.5272862603657));
#49872=CARTESIAN_POINT('Ctrl Pts',(6.71394718237391,4.18411689993163,73.5351959630412));
#49873=CARTESIAN_POINT('Ctrl Pts',(6.61036954002703,4.35032038722022,73.5430976409049));
#49874=CARTESIAN_POINT('Ctrl Pts',(6.50050647898477,4.51285234657526,73.5509993187687));
#49875=CARTESIAN_POINT('Ctrl Pts',(6.3846482154567,4.67120842661357,73.5589009966324));
#49876=CARTESIAN_POINT('Ctrl Pts',(6.26888603325946,4.82943318185507,73.5667961216297));
#49877=CARTESIAN_POINT('Ctrl Pts',(6.14713875560896,4.9834886801912,73.574691246627));
#49878=CARTESIAN_POINT('Ctrl Pts',(6.01974091973089,5.1328978422834,73.5825863716243));
#49879=CARTESIAN_POINT('Ctrl Pts',(5.89242514065964,5.28221077009762,73.5904764113802));
#49880=CARTESIAN_POINT('Ctrl Pts',(5.75946627760064,5.4268830630797,73.5983664511361));
#49881=CARTESIAN_POINT('Ctrl Pts',(5.62124048922088,5.56646893122954,73.606256490892));
#49882=CARTESIAN_POINT('Ctrl Pts',(5.48307813732961,5.7059907387043,73.6141429096419));
#49883=CARTESIAN_POINT('Ctrl Pts',(5.33965391884534,5.84043052864044,73.6220293283918));
#49884=CARTESIAN_POINT('Ctrl Pts',(5.19138254565954,5.96937754415161,73.6299157471416));
#49885=CARTESIAN_POINT('Ctrl Pts',(5.04315176851963,6.09828925454051,73.637800006625));
#49886=CARTESIAN_POINT('Ctrl Pts',(4.89007674163458,6.22171096210383,73.6456842661083));
#49887=CARTESIAN_POINT('Ctrl Pts',(4.73260732106132,6.3392703795182,73.6535685255916));
#49888=CARTESIAN_POINT('Ctrl Pts',(4.57511951687059,6.45684352129474,73.6614537055153));
#49889=CARTESIAN_POINT('Ctrl Pts',(4.41323656598173,6.56855279372756,73.6693388854389));
#49890=CARTESIAN_POINT('Ctrl Pts',(4.24744004924162,6.67406727776236,73.6772240653626));
#49891=CARTESIAN_POINT('Ctrl Pts',(4.08162285334157,6.77959492221172,73.6851102287744));
#49892=CARTESIAN_POINT('Ctrl Pts',(3.91189140947407,6.87892605291088,73.6929963921861));
#49893=CARTESIAN_POINT('Ctrl Pts',(3.73875479338658,6.97177406367482,73.7008825555978));
#49894=CARTESIAN_POINT('Ctrl Pts',(3.56556753330826,7.06464923330274,73.7087710257821));
#49895=CARTESIAN_POINT('Ctrl Pts',(3.38897341986887,7.15103734103321,73.7166594959664));
#49896=CARTESIAN_POINT('Ctrl Pts',(3.20950476013447,7.23069845828701,73.7245479661506));
#49897=CARTESIAN_POINT('Ctrl Pts',(3.0299534918202,7.31039624317837,73.7324400673606));
#49898=CARTESIAN_POINT('Ctrl Pts',(2.84752535525844,7.38336072758949,73.7403321685706));
#49899=CARTESIAN_POINT('Ctrl Pts',(2.66277141849326,7.44940060493832,73.7482242697806));
#49900=CARTESIAN_POINT('Ctrl Pts',(2.47780329698364,7.51551704214022,73.7561255202824));
#49901=CARTESIAN_POINT('Ctrl Pts',(2.29050431416554,7.57469272137233,73.7640267707842));
#49902=CARTESIAN_POINT('Ctrl Pts',(2.10144056717119,7.62678625258682,73.771928021286));
#49903=CARTESIAN_POINT('Ctrl Pts',(1.9122515415065,7.67891430236145,73.7798345073666));
#49904=CARTESIAN_POINT('Ctrl Pts',(1.72129575480019,7.72395076983101,73.7877409934473));
#49905=CARTESIAN_POINT('Ctrl Pts',(1.52914845974499,7.7618055881386,73.7956474795279));
#49906=CARTESIAN_POINT('Ctrl Pts',(1.33673645052244,7.79971255761857,73.8035648580798));
#49907=CARTESIAN_POINT('Ctrl Pts',(1.14312999333838,7.83041806185964,73.8114822366316));
#49908=CARTESIAN_POINT('Ctrl Pts',(0.948909598373037,7.85388385285366,73.8193996151835));
#49909=CARTESIAN_POINT('Ctrl Pts',(0.864697498993089,7.86405839463426,73.8228325145428));
#49910=CARTESIAN_POINT('Ctrl Pts',(0.780369984610552,7.87287253021289,73.8262654139021));
#49911=CARTESIAN_POINT('Ctrl Pts',(0.695974292246004,7.88032618516091,73.8296983132614));
#49912=CARTESIAN_POINT('Ctrl Pts',(0.503191545222375,7.89735236310893,73.8375399903683));
#49913=CARTESIAN_POINT('Ctrl Pts',(0.309480002828726,7.90732678778585,73.8453816674753));
#49914=CARTESIAN_POINT('Ctrl Pts',(0.115403255200916,7.91015822146997,73.8532233445822));
#49915=CARTESIAN_POINT('Ctrl Pts',(-0.0784449856718756,7.91298632141252,
73.8610557888665));
#49916=CARTESIAN_POINT('Ctrl Pts',(-0.272657227937992,7.90868817129676,
73.8688882331508));
#49917=CARTESIAN_POINT('Ctrl Pts',(-0.46666271122103,7.89722400049257,73.8767206774351));
#49918=CARTESIAN_POINT('Ctrl Pts',(-0.660477537208162,7.88577109600811,
73.8845454244491));
#49919=CARTESIAN_POINT('Ctrl Pts',(-0.854085660550979,7.86716621558343,
73.8923701714631));
#49920=CARTESIAN_POINT('Ctrl Pts',(-1.0469140595466,7.84142155172923,73.9001949184771));
#49921=CARTESIAN_POINT('Ctrl Pts',(-1.23959047185993,7.81569717973072,73.9080134980523));
#49922=CARTESIAN_POINT('Ctrl Pts',(-1.43148803704333,7.78284427883069,73.9158320776276));
#49923=CARTESIAN_POINT('Ctrl Pts',(-1.62203640744121,7.74292702360904,73.9236506572028));
#49924=CARTESIAN_POINT('Ctrl Pts',(-1.81247164325526,7.70303346852217,73.9314645946405));
#49925=CARTESIAN_POINT('Ctrl Pts',(-2.00155893676101,7.65608398599158,73.9392785320782));
#49926=CARTESIAN_POINT('Ctrl Pts',(-2.18873552943269,7.60219427416841,73.9470924695159));
#49927=CARTESIAN_POINT('Ctrl Pts',(-2.37583737860299,7.54832608162654,73.9549032866861));
#49928=CARTESIAN_POINT('Ctrl Pts',(-2.56102970958169,7.48752327855418,73.9627141038562));
#49929=CARTESIAN_POINT('Ctrl Pts',(-2.74376220126369,7.41995215502881,73.9705249210264));
#49930=CARTESIAN_POINT('Ctrl Pts',(-2.9264874260422,7.35238371867105,73.9783354275761));
#49931=CARTESIAN_POINT('Ctrl Pts',(-3.10675267343504,7.27804761155472,73.9861459341258));
#49932=CARTESIAN_POINT('Ctrl Pts',(-3.28402453278888,7.1971594305004,73.9939564406755));
#49933=CARTESIAN_POINT('Ctrl Pts',(-3.46130127854716,7.11626901980642,74.0017671625176));
#49934=CARTESIAN_POINT('Ctrl Pts',(-3.63558415135138,7.02882632079456,74.0095778843597));
#49935=CARTESIAN_POINT('Ctrl Pts',(-3.80636144908283,6.93509434102637,74.0173886062018));
#49936=CARTESIAN_POINT('Ctrl Pts',(-3.97717352965858,6.84134327051895,74.0252009188826));
#49937=CARTESIAN_POINT('Ctrl Pts',(-4.14447830433175,6.74130053681446,74.0330132315634));
#49938=CARTESIAN_POINT('Ctrl Pts',(-4.30779019458443,6.63527427009934,74.0408255442442));
#49939=CARTESIAN_POINT('Ctrl Pts',(-4.47116411001637,6.52920773504742,74.0486408240089));
#49940=CARTESIAN_POINT('Ctrl Pts',(-4.63054182539353,6.41715333171838,74.0564561037737));
#49941=CARTESIAN_POINT('Ctrl Pts',(-4.78546805500666,6.29946160354286,74.0642713835384));
#49942=CARTESIAN_POINT('Ctrl Pts',(-4.94056276388966,6.18164188789561,74.0720951622683));
#49943=CARTESIAN_POINT('Ctrl Pts',(-5.09119603804208,6.05817281595878,74.0799189409983));
#49944=CARTESIAN_POINT('Ctrl Pts',(-5.23694610556563,5.9294448717735,74.0877427197282));
#49945=CARTESIAN_POINT('Ctrl Pts',(-5.38278459903386,5.8006388288932,74.0955712451113));
#49946=CARTESIAN_POINT('Ctrl Pts',(-5.52373372750108,5.66656779709337,74.1033997704944));
#49947=CARTESIAN_POINT('Ctrl Pts',(-5.65940967696242,5.52765801296572,74.1112282958776));
#49948=CARTESIAN_POINT('Ctrl Pts',(-5.79527234117178,5.38855706374621,74.1190675947334));
#49949=CARTESIAN_POINT('Ctrl Pts',(-5.92584709633149,5.24460432154438,74.1269068935893));
#49950=CARTESIAN_POINT('Ctrl Pts',(-6.05079066015617,5.09625876373707,74.1347461924452));
#49951=CARTESIAN_POINT('Ctrl Pts',(-6.12083108011365,5.01309973697655,74.1391407187995));
#49952=CARTESIAN_POINT('Ctrl Pts',(-6.18910269560798,4.92856081806555,74.1435352451539));
#49953=CARTESIAN_POINT('Ctrl Pts',(-6.25555115585064,4.84272658081537,74.1479297715083));
#49954=CARTESIAN_POINT('Ctrl Pts',(-6.37559513174575,4.68766078892482,74.1558688029596));
#49955=CARTESIAN_POINT('Ctrl Pts',(-6.49003378158572,4.52791714201392,74.1638078344109));
#49956=CARTESIAN_POINT('Ctrl Pts',(-6.5984834164448,4.3639360218618,74.1717468658621));
#49957=CARTESIAN_POINT('Ctrl Pts',(-6.70676445788647,4.20020982315291,74.1796735554697));
#49958=CARTESIAN_POINT('Ctrl Pts',(-6.80907485952521,4.03225956734306,74.1876002450773));
#49959=CARTESIAN_POINT('Ctrl Pts',(-6.90507137652646,3.86055828670867,74.1955269346849));
#49960=CARTESIAN_POINT('Ctrl Pts',(-7.00098019317911,3.68901386866302,74.2034463826397));
#49961=CARTESIAN_POINT('Ctrl Pts',(-7.09058644894565,3.51372554759673,74.2113658305945));
#49962=CARTESIAN_POINT('Ctrl Pts',(-7.17358974895407,3.33519581339703,74.2192852785494));
#49963=CARTESIAN_POINT('Ctrl Pts',(-7.25653085123015,3.15679985875332,74.2271987921413));
#49964=CARTESIAN_POINT('Ctrl Pts',(-7.33287871113123,2.97516763810119,74.2351123057332));
#49965=CARTESIAN_POINT('Ctrl Pts',(-7.40237837150453,2.79082701812241,74.2430258193252));
#49966=CARTESIAN_POINT('Ctrl Pts',(-7.47183736547843,2.60659426153802,74.2509347024757));
#49967=CARTESIAN_POINT('Ctrl Pts',(-7.53445602383177,2.41965658213687,74.2588435856262));
#49968=CARTESIAN_POINT('Ctrl Pts',(-7.59002701499753,2.23056291361793,74.2667524687767));
#49969=CARTESIAN_POINT('Ctrl Pts',(-7.64557659394122,2.04154210533663,74.2746583045322));
#49970=CARTESIAN_POINT('Ctrl Pts',(-7.6940838197897,1.85036729046182,74.2825641402877));
#49971=CARTESIAN_POINT('Ctrl Pts',(-7.73539073835603,1.65760403141272,74.2904699760432));
#49972=CARTESIAN_POINT('Ctrl Pts',(-7.77668764955054,1.46488747286015,74.2983738964625));
#49973=CARTESIAN_POINT('Ctrl Pts',(-7.81078765953284,1.27058357133946,74.3062778168818));
#49974=CARTESIAN_POINT('Ctrl Pts',(-7.83758354196369,1.07526983717572,74.314181737301));
#49975=CARTESIAN_POINT('Ctrl Pts',(-7.86438252247724,0.879933521255138,
74.3220865715547));
#49976=CARTESIAN_POINT('Ctrl Pts',(-7.88387563669531,0.68358747748106,74.3299914058084));
#49977=CARTESIAN_POINT('Ctrl Pts',(-7.89600724731406,0.486816752345093,
74.3378962400621));
#49978=CARTESIAN_POINT('Ctrl Pts',(-7.90612212347712,0.322756795278237,
74.3444869906292));
#49979=CARTESIAN_POINT('Ctrl Pts',(-7.91112049543788,0.158401844073439,
74.3510777411962));
#49980=CARTESIAN_POINT('Ctrl Pts',(-7.91099779416079,-0.00590768847896494,
74.3576684917633));
#49981=CARTESIAN_POINT('',(-7.91846474044373,-0.0010690628187093,76.3576290758486));
#49982=CARTESIAN_POINT('Ctrl Pts',(-7.90280119522295,-0.00596027707849772,
74.3576708491509));
#49983=CARTESIAN_POINT('Ctrl Pts',(-7.90869288684778,-0.90659764281454,
74.3938343093522));
#49984=CARTESIAN_POINT('Ctrl Pts',(-7.34860918258986,-4.44156078704885,
74.5360749223026));
#49985=CARTESIAN_POINT('Ctrl Pts',(-2.13974124634984,-9.11203122848944,
74.7843926880019));
#49986=CARTESIAN_POINT('Ctrl Pts',(6.51845747696313,-6.71804149910057,75.1026241462487));
#49987=CARTESIAN_POINT('Ctrl Pts',(8.71876257165608,0.413892218516685,75.3678170281211));
#49988=CARTESIAN_POINT('Ctrl Pts',(6.29868987220236,5.28787691418045,75.5799713336189));
#49989=CARTESIAN_POINT('Ctrl Pts',(1.91734040228322,8.51567395457576,75.792125639117));
#49990=CARTESIAN_POINT('Ctrl Pts',(-5.320841699348,7.60369065835455,76.0513265910671));
#49991=CARTESIAN_POINT('Ctrl Pts',(-7.91108836642875,2.47685045337626,76.2574889666432));
#49992=CARTESIAN_POINT('Ctrl Pts',(-7.92335669526798,-0.00104753037717561,
76.3575741894703));
#49993=CARTESIAN_POINT('',(-7.911,-5.90194559890733E-12,78.3576684917633));
#49994=CARTESIAN_POINT('Ctrl Pts',(-7.91099991910456,-0.00110191999642655,
76.3577128290767));
#49995=CARTESIAN_POINT('Ctrl Pts',(-7.9106767122703,-2.20240473643408,76.4462854857049));
#49996=CARTESIAN_POINT('Ctrl Pts',(-6.94187350370004,-4.38635073437256,
76.5348581423331));
#49997=CARTESIAN_POINT('Ctrl Pts',(-3.67820201487791,-7.34180684107874,
76.7120182346942));
#49998=CARTESIAN_POINT('Ctrl Pts',(-1.40868175871223,-8.08992666571422,
76.8006056704269));
#49999=CARTESIAN_POINT('Ctrl Pts',(2.97309270521729,-7.65454228025075,76.9777805418923));
#50000=CARTESIAN_POINT('Ctrl Pts',(5.05102072675967,-6.47444880833934,77.066367977625));
#50001=CARTESIAN_POINT('Ctrl Pts',(7.6695151884802,-2.93425195367305,77.2435428490905));
#50002=CARTESIAN_POINT('Ctrl Pts',(8.18956872247096,-0.601881960095122,
77.3321302848232));
#50003=CARTESIAN_POINT('Ctrl Pts',(7.32306689761172,3.71537198232775,77.5093051562886));
#50004=CARTESIAN_POINT('Ctrl Pts',(5.9432995884996,5.66643518936756,77.5978925920213));
#50005=CARTESIAN_POINT('Ctrl Pts',(2.16154501637551,7.92205913233073,77.7750674634868));
#50006=CARTESIAN_POINT('Ctrl Pts',(-0.210816529303192,8.2089496371299,77.8636548992195));
#50007=CARTESIAN_POINT('Ctrl Pts',(-4.42123908576641,6.91982244717695,78.0408297706849));
#50008=CARTESIAN_POINT('Ctrl Pts',(-6.22631625634328,5.35390358803349,78.1294172064176));
#50009=CARTESIAN_POINT('Ctrl Pts',(-7.65317280859601,2.31334857514211,78.264559258688));
#50010=CARTESIAN_POINT('Ctrl Pts',(-7.91100000000086,1.15702837836061,78.3111138752256));
#50011=CARTESIAN_POINT('Ctrl Pts',(-7.911,-5.90194559890733E-12,78.3576684917633));
#50012=CARTESIAN_POINT('',(-7.90317141111203,-0.000228506537956913,80.3576684917633));
#50013=CARTESIAN_POINT('Ctrl Pts',(-7.911,-5.90194559890733E-12,78.3576684917633));
#50014=CARTESIAN_POINT('Ctrl Pts',(-7.91099999999836,-2.20167589667262,
78.446255927496));
#50015=CARTESIAN_POINT('Ctrl Pts',(-6.94214576672048,-4.38610418339192,
78.5348433632287));
#50016=CARTESIAN_POINT('Ctrl Pts',(-3.67820201487754,-7.34180684107897,
78.7120182346942));
#50017=CARTESIAN_POINT('Ctrl Pts',(-1.40868175871163,-8.08992666571436,
78.8006056704269));
#50018=CARTESIAN_POINT('Ctrl Pts',(2.97309270521814,-7.65454228025046,78.9777805418923));
#50019=CARTESIAN_POINT('Ctrl Pts',(5.05102072676055,-6.47444880833871,79.0663679776251));
#50020=CARTESIAN_POINT('Ctrl Pts',(7.66951518848072,-2.93425195367178,79.2435428490905));
#50021=CARTESIAN_POINT('Ctrl Pts',(8.18956872247111,-0.601881960093584,
79.3321302848233));
#50022=CARTESIAN_POINT('Ctrl Pts',(7.32306689761092,3.7153719823294,79.5093051562887));
#50023=CARTESIAN_POINT('Ctrl Pts',(5.94329958849824,5.66643518936905,79.5978925920214));
#50024=CARTESIAN_POINT('Ctrl Pts',(2.1615450163733,7.92205913233138,79.7750674634869));
#50025=CARTESIAN_POINT('Ctrl Pts',(-0.210816529305671,8.20894963712987,
79.8636548992196));
#50026=CARTESIAN_POINT('Ctrl Pts',(-4.42123908576876,6.91982244717549,80.040829770685));
#50027=CARTESIAN_POINT('Ctrl Pts',(-6.22631625634523,5.35390358803129,80.1294172064178));
#50028=CARTESIAN_POINT('Ctrl Pts',(-7.65317280859644,2.31334857514018,80.2645592586881));
#50029=CARTESIAN_POINT('Ctrl Pts',(-7.91100000000084,1.15702837835973,80.3111138752257));
#50030=CARTESIAN_POINT('Ctrl Pts',(-7.911,-5.73152636462737E-12,80.3576684917633));
#50031=CARTESIAN_POINT('',(-7.91272987124828,-0.0069511639008941,82.3576684917633));
#50032=CARTESIAN_POINT('Ctrl Pts',(-7.8982622858675,-0.000371797647241044,
80.3576684917633));
#50033=CARTESIAN_POINT('Ctrl Pts',(-7.89966465680796,-1.28819607809109,
80.4092986399904));
#50034=CARTESIAN_POINT('Ctrl Pts',(-6.99340059655887,-5.22096879316791,
80.5670059409665));
#50035=CARTESIAN_POINT('Ctrl Pts',(-0.782238527603077,-9.32791637320139,
80.8307903946915));
#50036=CARTESIAN_POINT('Ctrl Pts',(6.03998710817404,-6.30125683006582,81.0959832765638));
#50037=CARTESIAN_POINT('Ctrl Pts',(8.12481793067604,-1.27457286690791,81.3081375820617));
#50038=CARTESIAN_POINT('Ctrl Pts',(7.67936794651516,4.14904204326629,81.5202918875595));
#50039=CARTESIAN_POINT('Ctrl Pts',(2.11166538450812,9.11936872126833,81.7854847694319));
#50040=CARTESIAN_POINT('Ctrl Pts',(-5.95633015797621,6.86030266448923,82.0822898296246));
#50041=CARTESIAN_POINT('Ctrl Pts',(-7.89397529231162,2.09439459744815,82.2730177370685));
#50042=CARTESIAN_POINT('Ctrl Pts',(-7.91272987124828,-0.0069511639008941,
82.3576684917633));
#50043=CARTESIAN_POINT('',(-7.91724620790701,0.00276230921017722,84.3576684917632));
#50044=CARTESIAN_POINT('Ctrl Pts',(-7.91272987124828,-0.0069511639008941,
82.3576684917633));
#50045=CARTESIAN_POINT('Ctrl Pts',(-7.91747694143191,-0.538833849344243,
82.3790948898174));
#50046=CARTESIAN_POINT('Ctrl Pts',(-7.62500664949156,-3.69864297510493,
82.5065984406204));
#50047=CARTESIAN_POINT('Ctrl Pts',(-3.380753567549,-8.72803821522355,82.7401791441724));
#50048=CARTESIAN_POINT('Ctrl Pts',(5.5255655561909,-7.5558013701102,83.058410602419));
#50049=CARTESIAN_POINT('Ctrl Pts',(8.6920369109565,-0.797332397813895,83.3236034842915));
#50050=CARTESIAN_POINT('Ctrl Pts',(6.97023541016857,4.36497741430031,83.5357577897894));
#50051=CARTESIAN_POINT('Ctrl Pts',(3.07771910783116,8.16791831007078,83.7479120952873));
#50052=CARTESIAN_POINT('Ctrl Pts',(-4.38505643770802,8.27002356725942,84.0131049771596));
#50053=CARTESIAN_POINT('Ctrl Pts',(-7.81686525122821,3.06263226942611,84.2340366347764));
#50054=CARTESIAN_POINT('Ctrl Pts',(-7.92391013983324,0.220078610135003,
84.3488911396443));
#50055=CARTESIAN_POINT('Ctrl Pts',(-7.92261405080686,0.00276418203836634,
84.3576684917632));
#50056=CARTESIAN_POINT('',(-7.91099839329515,0.0035651983779998,86.3576684917632));
#50057=CARTESIAN_POINT('Ctrl Pts',(-7.91099951849852,0.00276012975443844,
84.3576684917632));
#50058=CARTESIAN_POINT('Ctrl Pts',(-7.91106692192262,-0.190429503722451,
84.3654829140546));
#50059=CARTESIAN_POINT('Ctrl Pts',(-7.90405347510339,-0.383899768578029,
84.3732973363459));
#50060=CARTESIAN_POINT('Ctrl Pts',(-7.88992372170109,-0.57708289329906,
84.3811117586372));
#50061=CARTESIAN_POINT('Ctrl Pts',(-7.8758085715249,-0.770066361538518,
84.3889181046535));
#50062=CARTESIAN_POINT('Ctrl Pts',(-7.85459178483221,-0.962762930611376,
84.3967244506698));
#50063=CARTESIAN_POINT('Ctrl Pts',(-7.82628987288226,-1.1546028865461,84.404530796686));
#50064=CARTESIAN_POINT('Ctrl Pts',(-7.79801162681802,-1.34628242708271,
84.4123306150834));
#50065=CARTESIAN_POINT('Ctrl Pts',(-7.76266010513328,-1.53710643273618,
84.4201304334808));
#50066=CARTESIAN_POINT('Ctrl Pts',(-7.72030377557192,-1.72650821396538,
84.4279302518783));
#50067=CARTESIAN_POINT('Ctrl Pts',(-7.67797451163443,-1.91578896777265,
84.4357250862048));
#50068=CARTESIAN_POINT('Ctrl Pts',(-7.62864943192344,-2.10364896292528,
84.4435199205313));
#50069=CARTESIAN_POINT('Ctrl Pts',(-7.57244846598746,-2.28952947785438,
84.4513147548578));
#50070=CARTESIAN_POINT('Ctrl Pts',(-7.51627233435907,-2.47532785515815,
84.4591061447717));
#50071=CARTESIAN_POINT('Ctrl Pts',(-7.45322647154974,-2.65914815643696,
84.4668975346857));
#50072=CARTESIAN_POINT('Ctrl Pts',(-7.38348129528783,-2.84044450080171,
84.4746889245996));
#50073=CARTESIAN_POINT('Ctrl Pts',(-7.3137431265908,-3.02172262962868,84.4824795316828));
#50074=CARTESIAN_POINT('Ctrl Pts',(-7.23730710512835,-3.20047697360211,
84.4902701387659));
#50075=CARTESIAN_POINT('Ctrl Pts',(-7.15439279207838,-3.37617902023232,
84.4980607458491));
#50076=CARTESIAN_POINT('Ctrl Pts',(-7.07147906752829,-3.55187981978434,
84.505851297637));
#50077=CARTESIAN_POINT('Ctrl Pts',(-6.98208729351078,-3.72452804443674,
84.5136418494249));
#50078=CARTESIAN_POINT('Ctrl Pts',(-6.88648423743967,-3.8936173216554,84.5214324012127));
#50079=CARTESIAN_POINT('Ctrl Pts',(-6.7908647923431,-4.06273558548373,84.5292242885181));
#50080=CARTESIAN_POINT('Ctrl Pts',(-6.68903211880367,-4.22829337836133,
84.5370161758234));
#50081=CARTESIAN_POINT('Ctrl Pts',(-6.58129784696126,-4.38981088995678,
84.5448080631288));
#50082=CARTESIAN_POINT('Ctrl Pts',(-6.47352587108237,-4.55138492824558,
84.5526026773807));
#50083=CARTESIAN_POINT('Ctrl Pts',(-6.35984837987453,-4.70891557471506,
84.5603972916326));
#50084=CARTESIAN_POINT('Ctrl Pts',(-6.24061909826932,-4.86195375032674,
84.5681919058845));
#50085=CARTESIAN_POINT('Ctrl Pts',(-6.1212668145275,-5.01514980680737,84.5759945614011));
#50086=CARTESIAN_POINT('Ctrl Pts',(-5.99635151992537,-5.16384385726863,
84.5837972169177));
#50087=CARTESIAN_POINT('Ctrl Pts',(-5.86626647117264,-5.30762081249177,
84.5915998724342));
#50088=CARTESIAN_POINT('Ctrl Pts',(-5.73610523332489,-5.45148197597871,
84.5994070978631));
#50089=CARTESIAN_POINT('Ctrl Pts',(-5.60076845418176,-5.59042005269074,
84.6072143232919));
#50090=CARTESIAN_POINT('Ctrl Pts',(-5.4606847014455,-5.72405831481468,84.6150215487207));
#50091=CARTESIAN_POINT('Ctrl Pts',(-5.32041782530811,-5.85787127452206,
84.6228389800846));
#50092=CARTESIAN_POINT('Ctrl Pts',(-5.17539184732898,-5.98637035017073,
84.6306564114484));
#50093=CARTESIAN_POINT('Ctrl Pts',(-5.0260675072528,-6.10921978754551,84.6384738428122));
#50094=CARTESIAN_POINT('Ctrl Pts',(-4.95542999033655,-6.16733341594853,
84.6421718597593));
#50095=CARTESIAN_POINT('Ctrl Pts',(-4.88383102554381,-6.22418343540095,
84.6458698767063));
#50096=CARTESIAN_POINT('Ctrl Pts',(-4.81132146298963,-6.2797377954637,84.6495678936533));
#50097=CARTESIAN_POINT('Ctrl Pts',(-4.65622728924412,-6.39856567510311,
84.657477759093));
#50098=CARTESIAN_POINT('Ctrl Pts',(-4.4965190550354,-6.51180483402569,84.6653876245328));
#50099=CARTESIAN_POINT('Ctrl Pts',(-4.33263655781297,-6.61907708505518,
84.6732974899725));
#50100=CARTESIAN_POINT('Ctrl Pts',(-4.16893216684854,-6.72623275341391,
84.6811987590303));
#50101=CARTESIAN_POINT('Ctrl Pts',(-4.00106283495899,-6.82743424330512,
84.689100028088));
#50102=CARTESIAN_POINT('Ctrl Pts',(-3.82950127463175,-6.92234360513792,
84.6970012971458));
#50103=CARTESIAN_POINT('Ctrl Pts',(-3.65809428586274,-7.01716745662725,
84.7048954474093));
#50104=CARTESIAN_POINT('Ctrl Pts',(-3.48300199539357,-7.10571030720473,
84.7127895976726));
#50105=CARTESIAN_POINT('Ctrl Pts',(-3.30472616788266,-7.18767736861579,
84.7206837479361));
#50106=CARTESIAN_POINT('Ctrl Pts',(-3.12657784370117,-7.26958580697415,
84.7285722522829));
#50107=CARTESIAN_POINT('Ctrl Pts',(-2.94525083089561,-7.34492768260881,
84.7364607566299));
#50108=CARTESIAN_POINT('Ctrl Pts',(-2.76127182287398,-7.41345391300183,
84.7443492609768));
#50109=CARTESIAN_POINT('Ctrl Pts',(-2.57739022775557,-7.48194386023886,
84.7522335885313));
#50110=CARTESIAN_POINT('Ctrl Pts',(-2.39085975790355,-7.54362523295766,
84.7601179160859));
#50111=CARTESIAN_POINT('Ctrl Pts',(-2.20222768896848,-7.59829679638408,
84.7680022436404));
#50112=CARTESIAN_POINT('Ctrl Pts',(-2.01366046880723,-7.65294956457662,
84.7758838606857));
#50113=CARTESIAN_POINT('Ctrl Pts',(-1.8229934204459,-7.70059723046942,84.783765477731));
#50114=CARTESIAN_POINT('Ctrl Pts',(-1.63078987163276,-7.74108812729709,
84.7916470947762));
#50115=CARTESIAN_POINT('Ctrl Pts',(-1.43858369753527,-7.78157957718489,
84.7995288194755));
#50116=CARTESIAN_POINT('Ctrl Pts',(-1.24484131681875,-7.81491398321496,
84.8074105441748));
#50117=CARTESIAN_POINT('Ctrl Pts',(-1.05013773361246,-7.84099048210386,
84.8152922688741));
#50118=CARTESIAN_POINT('Ctrl Pts',(-0.85542235331027,-7.8670685609686,84.8231744711273));
#50119=CARTESIAN_POINT('Ctrl Pts',(-0.659745996512131,-7.88588780999542,
84.8310566733806));
#50120=CARTESIAN_POINT('Ctrl Pts',(-0.463690335164545,-7.8973990828041,
84.8389388756338));
#50121=CARTESIAN_POINT('Ctrl Pts',(-0.267589804447896,-7.9089129900868,
84.8468228818107));
#50122=CARTESIAN_POINT('Ctrl Pts',(-0.0711101407053061,-7.91311556819726,
84.8547068879876));
#50123=CARTESIAN_POINT('Ctrl Pts',(0.125165180769629,-7.91000977733422,
84.8625908941644));
#50124=CARTESIAN_POINT('Ctrl Pts',(0.321518449630203,-7.90690275305947,
84.8704780313395));
#50125=CARTESIAN_POINT('Ctrl Pts',(0.517666869767976,-7.89648158200195,
84.8783651685144));
#50126=CARTESIAN_POINT('Ctrl Pts',(0.713030041484756,-7.87880125145572,
84.8862523056895));
#50127=CARTESIAN_POINT('Ctrl Pts',(0.908601745483325,-7.86110204877694,
84.8941478616606));
#50128=CARTESIAN_POINT('Ctrl Pts',(1.10338618309347,-7.83612824070503,84.9020434176318));
#50129=CARTESIAN_POINT('Ctrl Pts',(1.29681001872961,-7.80398646688489,84.9099389736029));
#50130=CARTESIAN_POINT('Ctrl Pts',(1.49035170080613,-7.77182511019576,84.9178393400627));
#50131=CARTESIAN_POINT('Ctrl Pts',(1.68253079111909,-7.73248715020807,84.9257397065225));
#50132=CARTESIAN_POINT('Ctrl Pts',(1.87278688468571,-7.68612973378339,84.9336400729823));
#50133=CARTESIAN_POINT('Ctrl Pts',(2.06329078417946,-7.6397119374658,84.94155072956));
#50134=CARTESIAN_POINT('Ctrl Pts',(2.25186635304459,-7.58625651641438,84.9494613861377));
#50135=CARTESIAN_POINT('Ctrl Pts',(2.43796991255272,-7.52596995114169,84.9573720427154));
#50136=CARTESIAN_POINT('Ctrl Pts',(2.51973975202122,-7.49948135104461,84.9608478124436));
#50137=CARTESIAN_POINT('Ctrl Pts',(2.6010326365727,-7.47167459710296,84.9643235821718));
#50138=CARTESIAN_POINT('Ctrl Pts',(2.68180384210392,-7.44257006365924,84.9677993519));
#50139=CARTESIAN_POINT('Ctrl Pts',(2.86396539073789,-7.37693124039904,84.9756381800099));
#50140=CARTESIAN_POINT('Ctrl Pts',(3.0439908152153,-7.30450145393577,84.9834770081197));
#50141=CARTESIAN_POINT('Ctrl Pts',(3.22133083401293,-7.22543761012699,84.9913158362296));
#50142=CARTESIAN_POINT('Ctrl Pts',(3.39847205739639,-7.14646239566245,84.9991458771346));
#50143=CARTESIAN_POINT('Ctrl Pts',(3.57293355134956,-7.06086807350537,85.0069759180395));
#50144=CARTESIAN_POINT('Ctrl Pts',(3.74418145949518,-6.96886118374965,85.0148059589445));
#50145=CARTESIAN_POINT('Ctrl Pts',(3.91527073094477,-6.876939525219,85.0226287464363));
#50146=CARTESIAN_POINT('Ctrl Pts',(4.08315203739093,-6.7786172942189,85.0304515339282));
#50147=CARTESIAN_POINT('Ctrl Pts',(4.24731160023756,-6.67414902219657,85.0382743214201));
#50148=CARTESIAN_POINT('Ctrl Pts',(4.41135102551132,-6.56975720362249,85.046091383929));
#50149=CARTESIAN_POINT('Ctrl Pts',(4.57167383663879,-6.4592284904982,85.0539084464379));
#50150=CARTESIAN_POINT('Ctrl Pts',(4.72779080603319,-6.34286331985705,85.0617255089468));
#50151=CARTESIAN_POINT('Ctrl Pts',(4.88382388087507,-6.22656068184102,85.0695383707018));
#50152=CARTESIAN_POINT('Ctrl Pts',(5.03565533495399,-6.10442804376578,85.0773512324568));
#50153=CARTESIAN_POINT('Ctrl Pts',(5.18282474310586,-5.97680923923875,85.0851640942119));
#50154=CARTESIAN_POINT('Ctrl Pts',(5.32994367522474,-5.84923420529603,85.0929742763185));
#50155=CARTESIAN_POINT('Ctrl Pts',(5.47240348187388,-5.71617698412542,85.1007844584252));
#50156=CARTESIAN_POINT('Ctrl Pts',(5.60977652967726,-5.57802189732903,85.1085946405318));
#50157=CARTESIAN_POINT('Ctrl Pts',(5.74715577309297,-5.43986057964985,85.1164051748827));
#50158=CARTESIAN_POINT('Ctrl Pts',(5.87944754472689,-5.29660117992593,85.1242157092336));
#50159=CARTESIAN_POINT('Ctrl Pts',(6.00626046896467,-5.14866547553366,85.1320262435844));
#50160=CARTESIAN_POINT('Ctrl Pts',(6.13308355737754,-5.00071791395563,85.1398374039569));
#50161=CARTESIAN_POINT('Ctrl Pts',(6.25442669387939,-4.8480935678095,85.1476485643295));
#50162=CARTESIAN_POINT('Ctrl Pts',(6.36993833532186,-4.6912478728156,85.155459724702));
#50163=CARTESIAN_POINT('Ctrl Pts',(6.48547957901117,-4.5343619828689,85.1632728868459));
#50164=CARTESIAN_POINT('Ctrl Pts',(6.59518614180641,-4.37325287230649,85.1710860489898));
#50165=CARTESIAN_POINT('Ctrl Pts',(6.69874933173292,-4.20840568275062,85.1788992111337));
#50166=CARTESIAN_POINT('Ctrl Pts',(6.8023573030043,-4.04348721228066,85.1867157517358));
#50167=CARTESIAN_POINT('Ctrl Pts',(6.89981642268535,-3.87482774060308,85.1945322923379));
#50168=CARTESIAN_POINT('Ctrl Pts',(6.99086346655203,-3.70293788660142,85.20234883294));
#50169=CARTESIAN_POINT('Ctrl Pts',(7.082016763976,-3.53084743401166,85.2101744955873));
#50170=CARTESIAN_POINT('Ctrl Pts',(7.16674287510643,-3.35551938045594,85.2180001582345));
#50171=CARTESIAN_POINT('Ctrl Pts',(7.24482588504999,-3.17748625414961,85.2258258208818));
#50172=CARTESIAN_POINT('Ctrl Pts',(7.32295979200657,-2.99933708013512,85.2336565845472));
#50173=CARTESIAN_POINT('Ctrl Pts',(7.39444183966971,-2.81847964557318,85.2414873482126));
#50174=CARTESIAN_POINT('Ctrl Pts',(7.4591056843464,-2.63546265193633,85.2493181118781));
#50175=CARTESIAN_POINT('Ctrl Pts',(7.5238629614807,-2.45218121798378,85.2571601901738));
#50176=CARTESIAN_POINT('Ctrl Pts',(7.58178225433932,-2.26673432712953,85.2650022684695));
#50177=CARTESIAN_POINT('Ctrl Pts',(7.63274782294268,-2.07968306993249,85.2728443467652));
#50178=CARTESIAN_POINT('Ctrl Pts',(7.66131404305145,-1.97484077088352,85.2772398345591));
#50179=CARTESIAN_POINT('Ctrl Pts',(7.68769660438673,-1.86949459325518,85.281635322353));
#50180=CARTESIAN_POINT('Ctrl Pts',(7.71188224768466,-1.7637440851343,85.2860308101469));
#50181=CARTESIAN_POINT('Ctrl Pts',(7.75544196951926,-1.57328139365785,85.2939473341471));
#50182=CARTESIAN_POINT('Ctrl Pts',(7.7920031200178,-1.38093517548524,85.3018638581474));
#50183=CARTESIAN_POINT('Ctrl Pts',(7.82140203908545,-1.18726203636348,85.3097803821477));
#50184=CARTESIAN_POINT('Ctrl Pts',(7.85076708880784,-0.993812020493328,
85.3176877858301));
#50185=CARTESIAN_POINT('Ctrl Pts',(7.87298629100036,-0.799038465821142,
85.3255951895126));
#50186=CARTESIAN_POINT('Ctrl Pts',(7.88794617865336,-0.603511460262248,
85.333502593195));
#50187=CARTESIAN_POINT('Ctrl Pts',(7.90289160374776,-0.408173481575882,
85.3414023523489));
#50188=CARTESIAN_POINT('Ctrl Pts',(7.91059166837858,-0.212083844154115,
85.3493021115027));
#50189=CARTESIAN_POINT('Ctrl Pts',(7.91098417918274,-0.015821400708789,
85.3572018706566));
#50190=CARTESIAN_POINT('Ctrl Pts',(7.91137638323342,0.180287660496274,85.3650954560222));
#50191=CARTESIAN_POINT('Ctrl Pts',(7.90447241075511,0.376568915716337,85.3729890413879));
#50192=CARTESIAN_POINT('Ctrl Pts',(7.89026197064616,0.572439546655319,85.3808826267536));
#50193=CARTESIAN_POINT('Ctrl Pts',(7.87606000455408,0.768193375368819,85.3887715049902));
#50194=CARTESIAN_POINT('Ctrl Pts',(7.85456027743801,0.963536725033094,85.3966603832268));
#50195=CARTESIAN_POINT('Ctrl Pts',(7.82580457151532,1.15788764932089,85.4045492614634));
#50196=CARTESIAN_POINT('Ctrl Pts',(7.7970606889336,1.35215866330318,85.4124348960691));
#50197=CARTESIAN_POINT('Ctrl Pts',(7.76106682369745,1.5454377247974,85.4203205306747));
#50198=CARTESIAN_POINT('Ctrl Pts',(7.71791654339741,1.73714859155818,85.4282061652804));
#50199=CARTESIAN_POINT('Ctrl Pts',(7.67477010159794,1.92884240437944,85.4360910984071));
#50200=CARTESIAN_POINT('Ctrl Pts',(7.62446858240579,2.11896796295587,85.4439760315338));
#50201=CARTESIAN_POINT('Ctrl Pts',(7.56715665749851,2.30695928028128,85.4518609646605));
#50202=CARTESIAN_POINT('Ctrl Pts',(7.50984493129567,2.4949499458277,85.4597458704496));
#50203=CARTESIAN_POINT('Ctrl Pts',(7.44552294778714,2.68080605496448,85.4676307762388));
#50204=CARTESIAN_POINT('Ctrl Pts',(7.374385276009,2.86397674588702,85.4755156820279));
#50205=CARTESIAN_POINT('Ctrl Pts',(7.30323591565984,3.04717753343177,85.4834018833793));
#50206=CARTESIAN_POINT('Ctrl Pts',(7.22526876041979,3.22769170225382,85.4912880847306));
#50207=CARTESIAN_POINT('Ctrl Pts',(7.14072664268969,3.40498810781795,85.499174286082));
#50208=CARTESIAN_POINT('Ctrl Pts',(7.05615644969819,3.58234339105234,85.5070631063311));
#50209=CARTESIAN_POINT('Ctrl Pts',(6.96500709200787,3.7564784709895,85.5149519265802));
#50210=CARTESIAN_POINT('Ctrl Pts',(6.86756759842163,3.92688633412139,85.5228407468294));
#50211=CARTESIAN_POINT('Ctrl Pts',(6.7700337923989,4.09745913633679,85.5307372027284));
#50212=CARTESIAN_POINT('Ctrl Pts',(6.66619786074414,4.26429721646477,85.5386336586274));
#50213=CARTESIAN_POINT('Ctrl Pts',(6.55639302505851,4.4269212214545,85.5465301145265));
#50214=CARTESIAN_POINT('Ctrl Pts',(6.44652750012939,4.58963510889588,85.5544309348047));
#50215=CARTESIAN_POINT('Ctrl Pts',(6.33068669649665,4.74812999968534,85.5623317550828));
#50216=CARTESIAN_POINT('Ctrl Pts',(6.20924462442865,4.90195901594495,85.570232575361));
#50217=CARTESIAN_POINT('Ctrl Pts',(6.08765498379892,5.05597495528891,85.5781429962057));
#50218=CARTESIAN_POINT('Ctrl Pts',(5.96045070211805,5.20531343325787,85.5860534170503));
#50219=CARTESIAN_POINT('Ctrl Pts',(5.82804392610434,5.34956306583989,85.5939638378949));
#50220=CARTESIAN_POINT('Ctrl Pts',(5.77058461569455,5.41216170817954,85.5973966480612));
#50221=CARTESIAN_POINT('Ctrl Pts',(5.71214600837681,5.47380250434962,85.6008294582275));
#50222=CARTESIAN_POINT('Ctrl Pts',(5.65276374922151,5.53445417322135,85.6042622683938));
#50223=CARTESIAN_POINT('Ctrl Pts',(5.50893384386499,5.68135871874766,85.6125768857281));
#50224=CARTESIAN_POINT('Ctrl Pts',(5.35925051171007,5.8227797783906,85.6208915030624));
#50225=CARTESIAN_POINT('Ctrl Pts',(5.20414811838676,5.95825170346902,85.6292061203967));
#50226=CARTESIAN_POINT('Ctrl Pts',(5.04923742384508,6.09355619204035,85.6375104612809));
#50227=CARTESIAN_POINT('Ctrl Pts',(4.88892124611641,6.22292601884921,85.6458148021651));
#50228=CARTESIAN_POINT('Ctrl Pts',(4.72367087332647,6.34593212069647,85.6541191430492));
#50229=CARTESIAN_POINT('Ctrl Pts',(4.55861381813629,6.46879432426402,85.6624137691278));
#50230=CARTESIAN_POINT('Ctrl Pts',(4.38863431520403,6.58530747682992,85.6707083952064));
#50231=CARTESIAN_POINT('Ctrl Pts',(4.21423746538685,6.69508204470489,85.679003021285));
#50232=CARTESIAN_POINT('Ctrl Pts',(4.04010320400824,6.80469132557839,85.6872851581878));
#50233=CARTESIAN_POINT('Ctrl Pts',(3.86156511659703,6.90758211432676,85.6955672950906));
#50234=CARTESIAN_POINT('Ctrl Pts',(3.67915811983896,7.00340749415761,85.7038494319934));
#50235=CARTESIAN_POINT('Ctrl Pts',(3.49691933794007,7.09914450428193,85.7121239311492));
#50236=CARTESIAN_POINT('Ctrl Pts',(3.31081902033116,7.18782896284675,85.720398430305));
#50237=CARTESIAN_POINT('Ctrl Pts',(3.12141914942105,7.26915837588008,85.7286729294608));
#50238=CARTESIAN_POINT('Ctrl Pts',(2.93223711833086,7.35039424721984,85.7369379116333));
#50239=CARTESIAN_POINT('Ctrl Pts',(2.73976337548252,7.42429183793646,85.7452028938058));
#50240=CARTESIAN_POINT('Ctrl Pts',(2.54458273169738,7.49059541835945,85.7534678759783));
#50241=CARTESIAN_POINT('Ctrl Pts',(2.46657232338421,7.5170958401283,85.7567712498246));
#50242=CARTESIAN_POINT('Ctrl Pts',(2.38812975283229,7.5423836682559,85.7600746236709));
#50243=CARTESIAN_POINT('Ctrl Pts',(2.30929332429207,7.56644469631412,85.7633779975171));
#50244=CARTESIAN_POINT('Ctrl Pts',(2.11201956587983,7.62665302289864,85.7716440870161));
#50245=CARTESIAN_POINT('Ctrl Pts',(1.91250164971992,7.67910807102709,85.7799101765151));
#50246=CARTESIAN_POINT('Ctrl Pts',(1.71136454832781,7.72367479783598,85.7881762660141));
#50247=CARTESIAN_POINT('Ctrl Pts',(1.51004656406251,7.76828160356387,85.7964497892188));
#50248=CARTESIAN_POINT('Ctrl Pts',(1.30710677430522,7.80498586218106,85.8047233124235));
#50249=CARTESIAN_POINT('Ctrl Pts',(1.10317860488045,7.83370397485979,85.8129968356282));
#50250=CARTESIAN_POINT('Ctrl Pts',(0.899053778333808,7.86244978170848,85.8212783373641));
#50251=CARTESIAN_POINT('Ctrl Pts',(0.693938959777478,7.88319402637382,85.8295598391));
#50252=CARTESIAN_POINT('Ctrl Pts',(0.488471766304341,7.89590503574628,85.8378413408359));
#50253=CARTESIAN_POINT('Ctrl Pts',(0.282662474383059,7.90863720867535,85.8461366310937));
#50254=CARTESIAN_POINT('Ctrl Pts',(0.0764999282259149,7.91330938770227,
85.8544319213514));
#50255=CARTESIAN_POINT('Ctrl Pts',(-0.129377135245994,7.90994200717525,
85.8627272116092));
#50256=CARTESIAN_POINT('Ctrl Pts',(-0.335440909823312,7.90657157275125,
85.8710300249139));
#50257=CARTESIAN_POINT('Ctrl Pts',(-0.541218391845821,7.89514703645119,
85.8793328382187));
#50258=CARTESIAN_POINT('Ctrl Pts',(-0.74607558734896,7.8757407409057,85.8876356515234));
#50259=CARTESIAN_POINT('Ctrl Pts',(-0.951246935321723,7.85630468543083,
85.8959511973528));
#50260=CARTESIAN_POINT('Ctrl Pts',(-1.15549488415217,7.82886243844658,85.9042667431822));
#50261=CARTESIAN_POINT('Ctrl Pts',(-1.35819337639028,7.79353782003588,85.9125822890117));
#50262=CARTESIAN_POINT('Ctrl Pts',(-1.43872661315376,7.77950315294666,85.9158861015546));
#50263=CARTESIAN_POINT('Ctrl Pts',(-1.51901540936514,7.76422480033309,85.9191899140976));
#50264=CARTESIAN_POINT('Ctrl Pts',(-1.59902112962635,7.74771272228188,85.9224937266406));
#50265=CARTESIAN_POINT('Ctrl Pts',(-1.79056392623238,7.70818092883787,85.9304034297453));
#50266=CARTESIAN_POINT('Ctrl Pts',(-1.98088258563153,7.66149169908155,85.93831313285));
#50267=CARTESIAN_POINT('Ctrl Pts',(-2.16940300255316,7.60773367123964,85.9462228359547));
#50268=CARTESIAN_POINT('Ctrl Pts',(-2.35773215632278,7.5540301835373,85.9541245142801));
#50269=CARTESIAN_POINT('Ctrl Pts',(-2.54426637299649,7.49327227687575,85.9620261926054));
#50270=CARTESIAN_POINT('Ctrl Pts',(-2.72844080741549,7.42559975762429,85.9699278709308));
#50271=CARTESIAN_POINT('Ctrl Pts',(-2.91246250661091,7.35798335895976,85.9778229964216));
#50272=CARTESIAN_POINT('Ctrl Pts',(-3.09412800047449,7.28346388948508,85.9857181219123));
#50273=CARTESIAN_POINT('Ctrl Pts',(-3.27288642964673,7.20223128055704,85.9936132474031));
#50274=CARTESIAN_POINT('Ctrl Pts',(-3.45152972142404,7.1210509931392,86.0015032876837));
#50275=CARTESIAN_POINT('Ctrl Pts',(-3.62726936653998,7.03316632334309,86.0093933279643));
#50276=CARTESIAN_POINT('Ctrl Pts',(-3.79957309760087,6.93881584104865,86.0172833682449));
#50277=CARTESIAN_POINT('Ctrl Pts',(-3.97179775332592,6.84450865901259,86.02516978755));
#50278=CARTESIAN_POINT('Ctrl Pts',(-4.14058933554998,6.74374174275647,86.0330562068551));
#50279=CARTESIAN_POINT('Ctrl Pts',(-4.30543861381387,6.63680038442324,86.0409426261602));
#50280=CARTESIAN_POINT('Ctrl Pts',(-4.47024275770401,6.52988830575255,86.0488268862288));
#50281=CARTESIAN_POINT('Ctrl Pts',(-4.63110646018127,6.41680534183075,86.0567111462972));
#50282=CARTESIAN_POINT('Ctrl Pts',(-4.78754777132697,6.29788117840137,86.0645954063658));
#50283=CARTESIAN_POINT('Ctrl Pts',(-4.94400734691083,6.17894313064045,86.0724805869174));
#50284=CARTESIAN_POINT('Ctrl Pts',(-5.09604322096018,6.05416272383731,86.0803657674689));
#50285=CARTESIAN_POINT('Ctrl Pts',(-5.24320445367384,5.92391155040104,86.0882509480205));
#50286=CARTESIAN_POINT('Ctrl Pts',(-5.39038404173693,5.79364413079886,86.0961371120869));
#50287=CARTESIAN_POINT('Ctrl Pts',(-5.53268751823247,5.65790481287382,86.1040232761533));
#50288=CARTESIAN_POINT('Ctrl Pts',(-5.66969895078601,5.51710384236657,86.1119094402196));
#50289=CARTESIAN_POINT('Ctrl Pts',(-5.80675046084643,5.37626168586661,86.1197979110847));
#50290=CARTESIAN_POINT('Ctrl Pts',(-5.93850660177277,5.23035517330234,86.1276863819497));
#50291=CARTESIAN_POINT('Ctrl Pts',(-6.06458989786054,5.07982975804975,86.1355748528148));
#50292=CARTESIAN_POINT('Ctrl Pts',(-6.19073122990261,4.92923505617166,86.1434669547313));
#50293=CARTESIAN_POINT('Ctrl Pts',(-6.31119429257198,4.77401747886304,86.1513590566478));
#50294=CARTESIAN_POINT('Ctrl Pts',(-6.4256431690895,4.6146539267353,86.1592511585643));
#50295=CARTESIAN_POINT('Ctrl Pts',(-6.54022472638397,4.45510562417087,86.167152409808));
#50296=CARTESIAN_POINT('Ctrl Pts',(-6.64877796971867,4.29140202617195,86.1750536610516));
#50297=CARTESIAN_POINT('Ctrl Pts',(-6.75101081512904,4.12404825068897,86.1829549122953));
#50298=CARTESIAN_POINT('Ctrl Pts',(-6.85331140301262,3.95658358170001,86.1908613991391));
#50299=CARTESIAN_POINT('Ctrl Pts',(-6.9492830757254,3.7854642130014,86.1987678859829));
#50300=CARTESIAN_POINT('Ctrl Pts',(-7.03868055463757,3.61121822239629,86.2066743728267));
#50301=CARTESIAN_POINT('Ctrl Pts',(-7.12820119341234,3.4367321790232,86.2145917521682));
#50302=CARTESIAN_POINT('Ctrl Pts',(-7.21112940236688,3.25911122110945,86.2225091315097));
#50303=CARTESIAN_POINT('Ctrl Pts',(-7.28726826007096,3.07890277627637,86.2304265108512));
#50304=CARTESIAN_POINT('Ctrl Pts',(-7.32028125772858,3.00076631420494,86.2338594021966));
#50305=CARTESIAN_POINT('Ctrl Pts',(-7.35201849637787,2.92214359411228,86.2372922935419));
#50306=CARTESIAN_POINT('Ctrl Pts',(-7.38246687227592,2.84307999883024,86.2407251848872));
#50307=CARTESIAN_POINT('Ctrl Pts',(-7.46186561464569,2.6369097238164,86.2496769679453));
#50308=CARTESIAN_POINT('Ctrl Pts',(-7.53269619445423,2.42722379759038,86.2586287510035));
#50309=CARTESIAN_POINT('Ctrl Pts',(-7.59467025546627,2.2147019462528,86.2675805340616));
#50310=CARTESIAN_POINT('Ctrl Pts',(-7.65631623356132,2.00330515897866,86.2764849275014));
#50311=CARTESIAN_POINT('Ctrl Pts',(-7.7091991241833,1.78910254853394,86.2853893209411));
#50312=CARTESIAN_POINT('Ctrl Pts',(-7.7530808313697,1.57278689664167,86.2942937143809));
#50313=CARTESIAN_POINT('Ctrl Pts',(-7.79680836482911,1.35723124686413,86.3031668231782));
#50314=CARTESIAN_POINT('Ctrl Pts',(-7.83159774763029,1.13957753073449,86.3120399319754));
#50315=CARTESIAN_POINT('Ctrl Pts',(-7.85726037723687,0.920532652491735,
86.3209130407727));
#50316=CARTESIAN_POINT('Ctrl Pts',(-7.88277750392521,0.702729722930816,
86.3297358404923));
#50317=CARTESIAN_POINT('Ctrl Pts',(-7.89927099049118,0.483551527721885,
86.3385586402119));
#50318=CARTESIAN_POINT('Ctrl Pts',(-7.90660338426671,0.263711819799972,
86.3473814399316));
#50319=CARTESIAN_POINT('Ctrl Pts',(-7.90945314916429,0.178270216156082,
86.3508104572088));
#50320=CARTESIAN_POINT('Ctrl Pts',(-7.91091963434882,0.0927288781526532,
86.354239474486));
#50321=CARTESIAN_POINT('Ctrl Pts',(-7.9109967865903,0.00713039676099505,
86.3576684917632));
#50322=CARTESIAN_POINT('',(-7.91099856105006,-0.0033739488622614,88.3576684917632));
#50323=CARTESIAN_POINT('Ctrl Pts',(-7.911,-4.99544849930089E-12,86.3576684917632));
#50324=CARTESIAN_POINT('Ctrl Pts',(-7.91099999999861,-2.20167589667164,
86.4462559274959));
#50325=CARTESIAN_POINT('Ctrl Pts',(-6.94214576672105,-4.38610418339098,
86.5348433632287));
#50326=CARTESIAN_POINT('Ctrl Pts',(-3.67820201487865,-7.3418068410784,86.7120182346941));
#50327=CARTESIAN_POINT('Ctrl Pts',(-1.40868175871295,-8.08992666571411,
86.8006056704268));
#50328=CARTESIAN_POINT('Ctrl Pts',(2.97309270521675,-7.65454228025098,86.9777805418923));
#50329=CARTESIAN_POINT('Ctrl Pts',(5.0510207267593,-6.47444880833966,87.066367977625));
#50330=CARTESIAN_POINT('Ctrl Pts',(7.66951518848009,-2.93425195367338,87.2435428490904));
#50331=CARTESIAN_POINT('Ctrl Pts',(8.18956872247096,-0.601881960095381,
87.3321302848232));
#50332=CARTESIAN_POINT('Ctrl Pts',(7.32306689761179,3.71537198232766,87.5093051562886));
#50333=CARTESIAN_POINT('Ctrl Pts',(5.94329958849964,5.66643518936756,87.5978925920213));
#50334=CARTESIAN_POINT('Ctrl Pts',(2.1615450163754,7.92205913233078,87.7750674634868));
#50335=CARTESIAN_POINT('Ctrl Pts',(-0.210816529303402,8.20894963712991,
87.8636548992195));
#50336=CARTESIAN_POINT('Ctrl Pts',(-4.42123908576671,6.91982244717678,88.0408297706849));
#50337=CARTESIAN_POINT('Ctrl Pts',(-6.22631625634359,5.35390358803317,88.1294172064177));
#50338=CARTESIAN_POINT('Ctrl Pts',(-7.65317280859594,2.3133485751421,88.264559258688));
#50339=CARTESIAN_POINT('Ctrl Pts',(-7.9110000000007,1.15702837836116,88.3111138752256));
#50340=CARTESIAN_POINT('Ctrl Pts',(-7.911,-4.82447415350862E-12,88.3576684917632));
#50341=CARTESIAN_POINT('',(-7.91099998641113,-0.000451624858829035,90.3576866635156));
#50342=CARTESIAN_POINT('Ctrl Pts',(-7.91099712210012,-0.00674789771969833,
88.3576684917632));
#50343=CARTESIAN_POINT('Ctrl Pts',(-7.91079974958978,-0.238140462654705,
88.3669549096822));
#50344=CARTESIAN_POINT('Ctrl Pts',(-7.90044647194352,-0.469090082543646,
88.3762413276011));
#50345=CARTESIAN_POINT('Ctrl Pts',(-7.88007661870822,-0.698794306851447,
88.3855277455201));
#50346=CARTESIAN_POINT('Ctrl Pts',(-7.85957817621448,-0.929948590495647,
88.3948727860309));
#50347=CARTESIAN_POINT('Ctrl Pts',(-7.82893639447855,-1.15984165263072,
88.4042178265418));
#50348=CARTESIAN_POINT('Ctrl Pts',(-7.78834219788504,-1.38767676662948,
88.4135628670527));
#50349=CARTESIAN_POINT('Ctrl Pts',(-7.74741882746136,-1.6173593702552,88.4229836854588));
#50350=CARTESIAN_POINT('Ctrl Pts',(-7.69638104062731,-1.84495046201203,
88.432404503865));
#50351=CARTESIAN_POINT('Ctrl Pts',(-7.63547284515937,-2.06965587256285,
88.4418253222711));
#50352=CARTESIAN_POINT('Ctrl Pts',(-7.57831964966171,-2.28050815869487,
88.4506653457191));
#50353=CARTESIAN_POINT('Ctrl Pts',(-7.51247604239519,-2.4888197816889,88.4595053691671));
#50354=CARTESIAN_POINT('Ctrl Pts',(-7.43818125172721,-2.69395261028362,
88.4683453926152));
#50355=CARTESIAN_POINT('Ctrl Pts',(-7.37227735286866,-2.87591763187833,
88.4761870192755));
#50356=CARTESIAN_POINT('Ctrl Pts',(-7.29958832600452,-3.05574943342999,
88.4840286459358));
#50357=CARTESIAN_POINT('Ctrl Pts',(-7.22026924162715,-3.23289855677732,
88.4918702725962));
#50358=CARTESIAN_POINT('Ctrl Pts',(-7.14104354949535,-3.40983910037918,
88.4997026663319));
#50359=CARTESIAN_POINT('Ctrl Pts',(-7.05520348569415,-3.5841029378101,88.5075350600677));
#50360=CARTESIAN_POINT('Ctrl Pts',(-6.96295380772239,-3.75515582519878,
88.5153674538035));
#50361=CARTESIAN_POINT('Ctrl Pts',(-6.87079478873815,-3.92604060921923,
88.5231921502019));
#50362=CARTESIAN_POINT('Ctrl Pts',(-6.77223886523992,-4.09372042014354,
88.5310168466004));
#50363=CARTESIAN_POINT('Ctrl Pts',(-6.66753886026993,-4.25768088832293,
88.5388415429989));
#50364=CARTESIAN_POINT('Ctrl Pts',(-6.56292138045455,-4.42151212190496,
88.546660071926));
#50365=CARTESIAN_POINT('Ctrl Pts',(-6.45216965273698,-4.58162955663426,
88.5544786008531));
#50366=CARTESIAN_POINT('Ctrl Pts',(-6.33558250049089,-4.73754317969489,
88.5622971297803));
#50367=CARTESIAN_POINT('Ctrl Pts',(-6.21906457014911,-4.89336423133845,
88.570111016571));
#50368=CARTESIAN_POINT('Ctrl Pts',(-6.09671832684766,-5.04498616234068,
88.5779249033618));
#50369=CARTESIAN_POINT('Ctrl Pts',(-5.96888610478008,-5.19194757948916,
88.5857387901525));
#50370=CARTESIAN_POINT('Ctrl Pts',(-5.8411049285406,-5.33885031215952,88.5935495567102));
#50371=CARTESIAN_POINT('Ctrl Pts',(-5.70784236861505,-5.48109597383794,
88.6013603232679));
#50372=CARTESIAN_POINT('Ctrl Pts',(-5.56948137970588,-5.61825579349227,
88.6091710898256));
#50373=CARTESIAN_POINT('Ctrl Pts',(-5.43112588997301,-5.75541016171094,
88.6169815459433));
#50374=CARTESIAN_POINT('Ctrl Pts',(-5.28767261831783,-5.88747883659304,
88.6247920020611));
#50375=CARTESIAN_POINT('Ctrl Pts',(-5.13954208745199,-6.01406918245123,
88.6326024581788));
#50376=CARTESIAN_POINT('Ctrl Pts',(-4.99140747143296,-6.14066301942602,
88.6404131296938));
#50377=CARTESIAN_POINT('Ctrl Pts',(-4.83859560631866,-6.26177799713768,
88.6482238012088));
#50378=CARTESIAN_POINT('Ctrl Pts',(-4.68156083935325,-6.37706116541421,
88.6560344727238));
#50379=CARTESIAN_POINT('Ctrl Pts',(-4.52449408561535,-6.49236781598418,
88.6638467352124));
#50380=CARTESIAN_POINT('Ctrl Pts',(-4.36320300018651,-6.60184008248953,
88.671658997701));
#50381=CARTESIAN_POINT('Ctrl Pts',(-4.1981718174763,-6.705167737719,88.6794712601896));
#50382=CARTESIAN_POINT('Ctrl Pts',(-4.03307795271457,-6.80853463880069,
88.6872864899274));
#50383=CARTESIAN_POINT('Ctrl Pts',(-3.86424145900895,-6.9057520931507,88.6951017196652));
#50384=CARTESIAN_POINT('Ctrl Pts',(-3.69217224236431,-6.99655523330693,
88.702916949403));
#50385=CARTESIAN_POINT('Ctrl Pts',(-3.51991589209342,-7.08745712628613,
88.7107406785825));
#50386=CARTESIAN_POINT('Ctrl Pts',(-3.34442010821241,-7.17193060794182,
88.718564407762));
#50387=CARTESIAN_POINT('Ctrl Pts',(-3.16621686751772,-7.2497580475383,88.7263881369415));
#50388=CARTESIAN_POINT('Ctrl Pts',(-2.98790550671005,-7.32763270687965,
88.7342166129622));
#50389=CARTESIAN_POINT('Ctrl Pts',(-2.80688374181482,-7.39885315973558,
88.7420450889829));
#50390=CARTESIAN_POINT('Ctrl Pts',(-2.62369994818983,-7.46325127420139,
88.7498735650036));
#50391=CARTESIAN_POINT('Ctrl Pts',(-2.44026404232468,-7.52773801852129,
88.7577128152014));
#50392=CARTESIAN_POINT('Ctrl Pts',(-2.25466049935241,-7.58538356643291,
88.7655520653991));
#50393=CARTESIAN_POINT('Ctrl Pts',(-2.06745027669823,-7.63607034759243,
88.7733913155969));
#50394=CARTESIAN_POINT('Ctrl Pts',(-1.96248841042801,-7.66448855611922,
88.7777864940185));
#50395=CARTESIAN_POINT('Ctrl Pts',(-1.85702165132031,-7.69072025127963,
88.7821816724401));
#50396=CARTESIAN_POINT('Ctrl Pts',(-1.75114965382108,-7.71475183592592,
88.7865768508617));
#50397=CARTESIAN_POINT('Ctrl Pts',(-1.56061467552175,-7.75800083062928,
88.7944867349195));
#50398=CARTESIAN_POINT('Ctrl Pts',(-1.36821932111949,-7.79424541203708,
88.8023966189773));
#50399=CARTESIAN_POINT('Ctrl Pts',(-1.17452109004874,-7.82332545718448,
88.8103065030351));
#50400=CARTESIAN_POINT('Ctrl Pts',(-0.981033441438009,-7.85237388744613,
88.8182077877225));
#50401=CARTESIAN_POINT('Ctrl Pts',(-0.786246075529237,-7.87427324520897,
88.8261090724098));
#50402=CARTESIAN_POINT('Ctrl Pts',(-0.590729610027844,-7.88891371025418,
88.8340103570972));
#50403=CARTESIAN_POINT('Ctrl Pts',(-0.395389372041236,-7.90354097920993,
88.8419045200121));
#50404=CARTESIAN_POINT('Ctrl Pts',(-0.199321685415827,-7.91092236349717,
88.8497986829271));
#50405=CARTESIAN_POINT('Ctrl Pts',(-0.00310555553988154,-7.91099939043891,
88.8576928458421));
#50406=CARTESIAN_POINT('Ctrl Pts',(0.192970166471871,-7.9110763622619,88.865581359871));
#50407=CARTESIAN_POINT('Ctrl Pts',(0.38919377655344,-7.90385939016733,88.8734698738999));
#50408=CARTESIAN_POINT('Ctrl Pts',(0.584982690679458,-7.88934194033985,
88.8813583879289));
#50409=CARTESIAN_POINT('Ctrl Pts',(0.780667865402883,-7.87483218263111,
88.8892427222026));
#50410=CARTESIAN_POINT('Ctrl Pts',(0.975918459923912,-7.85302968045513,
88.8971270564763));
#50411=CARTESIAN_POINT('Ctrl Pts',(1.17015315541674,-7.82397997139999,88.9050113907501));
#50412=CARTESIAN_POINT('Ctrl Pts',(1.36432100322448,-7.79494026007363,88.9128930115565));
#50413=CARTESIAN_POINT('Ctrl Pts',(1.55747330806565,-7.75865836381019,88.9207746323629));
#50414=CARTESIAN_POINT('Ctrl Pts',(1.74903485101827,-7.71523156424507,88.9286562531694));
#50415=CARTESIAN_POINT('Ctrl Pts',(1.94059890292189,-7.67180419590341,88.9365379772043));
#50416=CARTESIAN_POINT('Ctrl Pts',(2.13057181301397,-7.62123180519448,88.9444197012391));
#50417=CARTESIAN_POINT('Ctrl Pts',(2.3183889546336,-7.56366271425643,88.952301425274));
#50418=CARTESIAN_POINT('Ctrl Pts',(2.5062174103923,-7.50609015534577,88.9601836241054));
#50419=CARTESIAN_POINT('Ctrl Pts',(2.69188950870627,-7.4415201569228,88.9680658229368));
#50420=CARTESIAN_POINT('Ctrl Pts',(2.87485614753901,-7.37015082145252,88.9759480217682));
#50421=CARTESIAN_POINT('Ctrl Pts',(3.05786459616895,-7.29876517734005,88.9838320217647));
#50422=CARTESIAN_POINT('Ctrl Pts',(3.23816603190562,-7.22057722556154,88.9917160217612));
#50423=CARTESIAN_POINT('Ctrl Pts',(3.41523146054028,-7.13583317286327,88.9996000217578));
#50424=CARTESIAN_POINT('Ctrl Pts',(3.59236714572668,-7.05105549516566,89.0074871499915));
#50425=CARTESIAN_POINT('Ctrl Pts',(3.76626395433527,-6.95971668199355,89.0153742782252));
#50426=CARTESIAN_POINT('Ctrl Pts',(3.93641740053939,-6.86210893594169,89.0232614064589));
#50427=CARTESIAN_POINT('Ctrl Pts',(4.10675238103278,-6.7643970535752,89.0311569493574));
#50428=CARTESIAN_POINT('Ctrl Pts',(4.27333572252414,-6.66040305084007,89.0390524922559));
#50429=CARTESIAN_POINT('Ctrl Pts',(4.43569091597372,-6.55046312087536,89.0469480351545));
#50430=CARTESIAN_POINT('Ctrl Pts',(4.59814497811076,-6.44045624130255,89.054848386165));
#50431=CARTESIAN_POINT('Ctrl Pts',(4.75636548145493,-6.32449641926763,89.0627487371756));
#50432=CARTESIAN_POINT('Ctrl Pts',(4.90990874665963,-6.20296034966171,89.0706490881862));
#50433=CARTESIAN_POINT('Ctrl Pts',(5.0636519316507,-6.08126603498369,89.0785597257859));
#50434=CARTESIAN_POINT('Ctrl Pts',(5.2127054525779,-5.95398119365958,89.0864703633857));
#50435=CARTESIAN_POINT('Ctrl Pts',(5.35666141948419,-5.82152037160479,89.0943810009854));
#50436=CARTESIAN_POINT('Ctrl Pts',(5.41991267258949,-5.76331984569136,89.0978567703599));
#50437=CARTESIAN_POINT('Ctrl Pts',(5.48218033033942,-5.70412052482345,89.1013325397343));
#50438=CARTESIAN_POINT('Ctrl Pts',(5.54343225297704,-5.64395959027471,89.1048083091088));
#50439=CARTESIAN_POINT('Ctrl Pts',(5.68282425918286,-5.50705036357862,89.1127181745523));
#50440=CARTESIAN_POINT('Ctrl Pts',(5.8173293829207,-5.36478933970217,89.1206280399957));
#50441=CARTESIAN_POINT('Ctrl Pts',(5.94651153067353,-5.21755897097165,89.1285379054392));
#50442=CARTESIAN_POINT('Ctrl Pts',(6.07555328424637,-5.07048861109102,89.1364391745007));
#50443=CARTESIAN_POINT('Ctrl Pts',(6.19928335909494,-4.91845992050672,89.1443404435623));
#50444=CARTESIAN_POINT('Ctrl Pts',(6.31730088897865,-4.76189358114076,89.1522417126239));
#50445=CARTESIAN_POINT('Ctrl Pts',(6.43521208878854,-4.60546830311069,89.1601358628912));
#50446=CARTESIAN_POINT('Ctrl Pts',(6.54742079014679,-4.44451379417601,89.1680300131584));
#50447=CARTESIAN_POINT('Ctrl Pts',(6.65356479037635,-4.27948555088857,89.1759241634256));
#50448=CARTESIAN_POINT('Ctrl Pts',(6.75963287614463,-4.11457533622413,89.1838126677764));
#50449=CARTESIAN_POINT('Ctrl Pts',(6.85964471663764,-3.94559748088743,89.1917011721271));
#50450=CARTESIAN_POINT('Ctrl Pts',(6.95327986994004,-3.7730385699442,89.1995896764778));
#50451=CARTESIAN_POINT('Ctrl Pts',(7.04686544545525,-3.60057102520975,89.2074740040362));
#50452=CARTESIAN_POINT('Ctrl Pts',(7.13408089736744,-3.42452650553766,89.2153583315946));
#50453=CARTESIAN_POINT('Ctrl Pts',(7.21465027456597,-3.24541868111113,89.223242659153));
#50454=CARTESIAN_POINT('Ctrl Pts',(7.2951919532653,-3.06637243116992,89.2311242762021));
#50455=CARTESIAN_POINT('Ctrl Pts',(7.36909196958923,-2.88426528957942,89.2390058932513));
#50456=CARTESIAN_POINT('Ctrl Pts',(7.43612120143288,-2.69963376731,89.2468875103004));
#50457=CARTESIAN_POINT('Ctrl Pts',(7.50315134882047,-2.51499972318162,89.2547692350036));
#50458=CARTESIAN_POINT('Ctrl Pts',(7.56331039846575,-2.32784155079379,89.2626509597068));
#50459=CARTESIAN_POINT('Ctrl Pts',(7.61641789382016,-2.13871444253227,89.27053268441));
#50460=CARTESIAN_POINT('Ctrl Pts',(7.66952860695933,-1.9495758750535,89.2784148866671));
#50461=CARTESIAN_POINT('Ctrl Pts',(7.71558682054423,-1.75846846614513,89.2862970889242));
#50462=CARTESIAN_POINT('Ctrl Pts',(7.75446234995561,-1.56596125849935,89.2941792911814));
#50463=CARTESIAN_POINT('Ctrl Pts',(7.79334677643459,-1.37340999358505,89.3020632973621));
#50464=CARTESIAN_POINT('Ctrl Pts',(7.82504517484067,-1.17945862983582,89.3099473035429));
#50465=CARTESIAN_POINT('Ctrl Pts',(7.84947870008574,-0.984685298407717,
89.3178313097236));
#50466=CARTESIAN_POINT('Ctrl Pts',(7.87392192868729,-0.789834616083665,
89.3257184469025));
#50467=CARTESIAN_POINT('Ctrl Pts',(7.89109449236527,-0.594161657757231,
89.3336055840815));
#50468=CARTESIAN_POINT('Ctrl Pts',(7.90096949066409,-0.398248801122208,
89.3414927212604));
#50469=CARTESIAN_POINT('Ctrl Pts',(7.91085502961861,-0.202126825466925,
89.3493882772354));
#50470=CARTESIAN_POINT('Ctrl Pts',(7.91342742691867,-0.00576478475610737,
89.3572838332104));
#50471=CARTESIAN_POINT('Ctrl Pts',(7.90871191469999,0.190254698450245,89.3651793891855));
#50472=CARTESIAN_POINT('Ctrl Pts',(7.90399352948313,0.38639360953459,89.3730797556492));
#50473=CARTESIAN_POINT('Ctrl Pts',(7.89197840357576,0.582189203546922,89.3809801221129));
#50474=CARTESIAN_POINT('Ctrl Pts',(7.87274359008219,0.777064582142223,89.3888804885765));
#50475=CARTESIAN_POINT('Ctrl Pts',(7.85348372351049,0.972193783218559,89.3967911451581));
#50476=CARTESIAN_POINT('Ctrl Pts',(7.82698543281866,1.16640003399136,89.4047018017396));
#50477=CARTESIAN_POINT('Ctrl Pts',(7.79337696207088,1.35911608299763,89.4126124583212));
#50478=CARTESIAN_POINT('Ctrl Pts',(7.77861013426741,1.44379130467012,89.4160882279993));
#50479=CARTESIAN_POINT('Ctrl Pts',(7.76247131623399,1.52817902287073,89.4195639976774));
#50480=CARTESIAN_POINT('Ctrl Pts',(7.74497441297671,1.61223209940011,89.4230397673555));
#50481=CARTESIAN_POINT('Ctrl Pts',(7.70551402583924,1.80179518328834,89.4308785954659));
#50482=CARTESIAN_POINT('Ctrl Pts',(7.65903031854054,1.99019500384961,89.4387174235763));
#50483=CARTESIAN_POINT('Ctrl Pts',(7.60560166455082,2.17686571018558,89.4465562516867));
#50484=CARTESIAN_POINT('Ctrl Pts',(7.55223290325468,2.36332716155107,89.4543862925922));
#50485=CARTESIAN_POINT('Ctrl Pts',(7.49193479291027,2.54806302366974,89.4622163334977));
#50486=CARTESIAN_POINT('Ctrl Pts',(7.42483701321142,2.73051576213097,89.4700463744032));
#50487=CARTESIAN_POINT('Ctrl Pts',(7.35780139000911,2.91279948422447,89.4778691618957));
#50488=CARTESIAN_POINT('Ctrl Pts',(7.28397876196211,3.09280396682753,89.4856919493881));
#50489=CARTESIAN_POINT('Ctrl Pts',(7.20354914040319,3.26998482898566,89.4935147368806));
#50490=CARTESIAN_POINT('Ctrl Pts',(7.12317837998744,3.44703602413938,89.5013317993901));
#50491=CARTESIAN_POINT('Ctrl Pts',(7.03621040116478,3.62126739576317,89.5091488618996));
#50492=CARTESIAN_POINT('Ctrl Pts',(6.94287410866501,3.79215243776263,89.516965924409));
#50493=CARTESIAN_POINT('Ctrl Pts',(6.84958797347095,3.96294564910262,89.5247787861646));
#50494=CARTESIAN_POINT('Ctrl Pts',(6.74994050990455,4.1303958050917,89.5325916479202));
#50495=CARTESIAN_POINT('Ctrl Pts',(6.64420762769525,4.29399883559326,89.5404045096758));
#50496=CARTESIAN_POINT('Ctrl Pts',(6.53851100965514,4.45754575367403,89.5482146917831));
#50497=CARTESIAN_POINT('Ctrl Pts',(6.42673332223231,4.61724788019711,89.5560248738904));
#50498=CARTESIAN_POINT('Ctrl Pts',(6.30919515940801,4.77262793862066,89.5638350559977));
#50499=CARTESIAN_POINT('Ctrl Pts',(6.1916516955372,4.92801500478449,89.5716455903491));
#50500=CARTESIAN_POINT('Ctrl Pts',(6.0683474420616,5.07907932728141,89.5794561247006));
#50501=CARTESIAN_POINT('Ctrl Pts',(5.93964516069064,5.22537427990419,89.5872666590521));
#50502=CARTESIAN_POINT('Ctrl Pts',(5.81093256371075,5.37168095820506,89.5950778194253));
#50503=CARTESIAN_POINT('Ctrl Pts',(5.67682130887087,5.51321724027827,89.6028889797984));
#50504=CARTESIAN_POINT('Ctrl Pts',(5.53771306666677,5.64957122189535,89.6107001401716));
#50505=CARTESIAN_POINT('Ctrl Pts',(5.39856917509871,5.78596014704015,89.6185133023162));
#50506=CARTESIAN_POINT('Ctrl Pts',(5.25442599636751,5.91716387967365,89.6263264644607));
#50507=CARTESIAN_POINT('Ctrl Pts',(5.10572061940688,6.04280878040696,89.6341396266053));
#50508=CARTESIAN_POINT('Ctrl Pts',(4.95695094134949,6.16850801074881,89.641956167208));
#50509=CARTESIAN_POINT('Ctrl Pts',(4.80361540382972,6.28864339410337,89.6497727078107));
#50510=CARTESIAN_POINT('Ctrl Pts',(4.64618269403846,6.40288273933058,89.6575892484134));
#50511=CARTESIAN_POINT('Ctrl Pts',(4.48856625740856,6.51725540395358,89.6654149110613));
#50512=CARTESIAN_POINT('Ctrl Pts',(4.32684338332908,6.62571808083098,89.6732405737092));
#50513=CARTESIAN_POINT('Ctrl Pts',(4.16151108263852,6.7279823505325,89.6810662363572));
#50514=CARTESIAN_POINT('Ctrl Pts',(3.99607101304628,6.83031327936826,89.6888970000232));
#50515=CARTESIAN_POINT('Ctrl Pts',(3.8270171330316,6.92643757614659,89.6967277636893));
#50516=CARTESIAN_POINT('Ctrl Pts',(3.65486941463108,7.01611363662207,89.7045585273554));
#50517=CARTESIAN_POINT('Ctrl Pts',(3.48247296087428,7.10591926957787,89.7124006056518));
#50518=CARTESIAN_POINT('Ctrl Pts',(3.30697405670186,7.18925790678759,89.7202426839482));
#50519=CARTESIAN_POINT('Ctrl Pts',(3.12891203323844,7.2659363118772,89.7280847622445));
#50520=CARTESIAN_POINT('Ctrl Pts',(3.02910820322112,7.30891458629368,89.7324802500305));
#50521=CARTESIAN_POINT('Ctrl Pts',(2.92849942072416,7.34980137541722,89.7368757378164));
#50522=CARTESIAN_POINT('Ctrl Pts',(2.82718239294255,7.388569598849,89.7412712256024));
#50523=CARTESIAN_POINT('Ctrl Pts',(2.64470465191667,7.45839337862535,89.7491877496008));
#50524=CARTESIAN_POINT('Ctrl Pts',(2.45938110114356,7.52155164713901,89.7571042735993));
#50525=CARTESIAN_POINT('Ctrl Pts',(2.27173991503261,7.57780434944369,89.7650207975978));
#50526=CARTESIAN_POINT('Ctrl Pts',(2.08431490299651,7.63399224520918,89.7729282012784));
#50527=CARTESIAN_POINT('Ctrl Pts',(1.89457790064729,7.68329032293475,89.7808356049591));
#50528=CARTESIAN_POINT('Ctrl Pts',(1.70307746622446,7.72550633577104,89.7887430086398));
#50529=CARTESIAN_POINT('Ctrl Pts',(1.51176216596351,7.7676815360307,89.7966427677918));
#50530=CARTESIAN_POINT('Ctrl Pts',(1.31868716380311,7.80278823657131,89.8045425269438));
#50531=CARTESIAN_POINT('Ctrl Pts',(1.12441688244685,7.83068372969235,89.8124422860958));
#50532=CARTESIAN_POINT('Ctrl Pts',(0.93029842642419,7.85855742203913,89.8203358714597));
#50533=CARTESIAN_POINT('Ctrl Pts',(0.734986891740987,7.87923108619266,89.8282294568235));
#50534=CARTESIAN_POINT('Ctrl Pts',(0.539057901824469,7.89261284863768,89.8361230421874));
#50535=CARTESIAN_POINT('Ctrl Pts',(0.343245748935179,7.90598663122559,89.8440119204221));
#50536=CARTESIAN_POINT('Ctrl Pts',(0.146817217275051,7.91207715313049,89.8519007986569));
#50537=CARTESIAN_POINT('Ctrl Pts',(-0.0496456348362537,7.91084422239129,
89.8597896768916));
#50538=CARTESIAN_POINT('Ctrl Pts',(-0.246027708291441,7.90961179859011,
89.8676753114954));
#50539=CARTESIAN_POINT('Ctrl Pts',(-0.442443730037354,7.90106192539069,
89.8755609460992));
#50540=CARTESIAN_POINT('Ctrl Pts',(-0.638310031637585,7.88520648451966,
89.8834465807031));
#50541=CARTESIAN_POINT('Ctrl Pts',(-0.8341589096448,7.86935245409415,89.8913315138279));
#50542=CARTESIAN_POINT('Ctrl Pts',(-1.02945782110312,7.84619417212444,89.8992164469528));
#50543=CARTESIAN_POINT('Ctrl Pts',(-1.22362608918042,7.81579555732345,89.9071013800777));
#50544=CARTESIAN_POINT('Ctrl Pts',(-1.41779368406282,7.78539704791658,89.914986285865));
#50545=CARTESIAN_POINT('Ctrl Pts',(-1.61083030271615,7.74775830845246,89.9228711916522));
#50546=CARTESIAN_POINT('Ctrl Pts',(-1.80216325093471,7.70299478235449,89.9307560974395));
#50547=CARTESIAN_POINT('Ctrl Pts',(-1.99352763690808,7.65822390119942,89.938642298789));
#50548=CARTESIAN_POINT('Ctrl Pts',(-2.18318745903772,7.60632597932667,89.9465285001384));
#50549=CARTESIAN_POINT('Ctrl Pts',(-2.37058278149718,7.54746701059826,89.9544147014879));
#50550=CARTESIAN_POINT('Ctrl Pts',(-2.55804033533732,7.48858849562483,89.9623035217351));
#50551=CARTESIAN_POINT('Ctrl Pts',(-2.7432315625057,7.42274443108365,89.9701923419824));
#50552=CARTESIAN_POINT('Ctrl Pts',(-2.92561394544023,7.35014993331739,89.9780811622297));
#50553=CARTESIAN_POINT('Ctrl Pts',(-3.10817285768912,7.27748517077714,89.9859776181269));
#50554=CARTESIAN_POINT('Ctrl Pts',(-3.28791717490341,7.19805705172566,89.9938740740241));
#50555=CARTESIAN_POINT('Ctrl Pts',(-3.46432557319129,7.11212832582012,90.0017705299213));
#50556=CARTESIAN_POINT('Ctrl Pts',(-3.64083147257813,7.02615210702144,90.0096713501976));
#50557=CARTESIAN_POINT('Ctrl Pts',(-3.81399747353355,6.93366827984826,90.0175721704739));
#50558=CARTESIAN_POINT('Ctrl Pts',(-3.98332869013005,6.83498453153969,90.0254729907502));
#50559=CARTESIAN_POINT('Ctrl Pts',(-4.15286566708425,6.73618086911392,90.033383411593));
#50560=CARTESIAN_POINT('Ctrl Pts',(-4.31855826141697,6.63116242099108,90.0412938324358));
#50561=CARTESIAN_POINT('Ctrl Pts',(-4.47994138578039,6.52027960903304,90.0492042532786));
#50562=CARTESIAN_POINT('Ctrl Pts',(-4.5499752872436,6.47216084842989,90.0526370634688));
#50563=CARTESIAN_POINT('Ctrl Pts',(-4.61919804849276,6.42293821132822,90.0560698736589));
#50564=CARTESIAN_POINT('Ctrl Pts',(-4.68757370137022,6.37264260681723,90.0595026838491));
#50565=CARTESIAN_POINT('Ctrl Pts',(-4.85318652508569,6.25082150920415,90.0678173011866));
#50566=CARTESIAN_POINT('Ctrl Pts',(-5.01419036393472,6.12243622989692,90.076131918524));
#50567=CARTESIAN_POINT('Ctrl Pts',(-5.17006328744622,5.98785158498445,90.0844465358615));
#50568=CARTESIAN_POINT('Ctrl Pts',(-5.32574355983871,5.85343327994589,90.0927508767487));
#50569=CARTESIAN_POINT('Ctrl Pts',(-5.47630534384549,5.7128310816791,90.101055217636));
#50570=CARTESIAN_POINT('Ctrl Pts',(-5.62125775855654,5.56645149191726,90.1093595585233));
#50571=CARTESIAN_POINT('Ctrl Pts',(-5.76604060116759,5.42024314383142,90.117654184605));
#50572=CARTESIAN_POINT('Ctrl Pts',(-5.90522695718064,5.26827109222717,90.1259488106867));
#50573=CARTESIAN_POINT('Ctrl Pts',(-6.03836034606067,5.11098085802735,90.1342434367684));
#50574=CARTESIAN_POINT('Ctrl Pts',(-6.1712932766807,4.9539274549255,90.1425255736742));
#50575=CARTESIAN_POINT('Ctrl Pts',(-6.29819123942203,4.7915720726692,90.15080771058));
#50576=CARTESIAN_POINT('Ctrl Pts',(-6.41863577121813,4.62439572662625,90.1590898474858));
#50577=CARTESIAN_POINT('Ctrl Pts',(-6.53896922964461,4.4573735498079,90.1673643466447));
#50578=CARTESIAN_POINT('Ctrl Pts',(-6.65286095413846,4.28553951206331,90.1756388458036));
#50579=CARTESIAN_POINT('Ctrl Pts',(-6.75993267263712,4.1094076533502,90.1839133449624));
#50580=CARTESIAN_POINT('Ctrl Pts',(-6.86688124171569,3.933478374147,90.1921783271379));
#50581=CARTESIAN_POINT('Ctrl Pts',(-6.96702530521538,3.75326138778045,90.2004433093133));
#50582=CARTESIAN_POINT('Ctrl Pts',(-7.06002969432137,3.5692998914774,90.2087082914887));
#50583=CARTESIAN_POINT('Ctrl Pts',(-7.09720197834301,3.49577358744641,90.2120116653167));
#50584=CARTESIAN_POINT('Ctrl Pts',(-7.13323420630645,3.42164943754332,90.2153150391446));
#50585=CARTESIAN_POINT('Ctrl Pts',(-7.16810694353174,3.34696337686747,90.2186184129726));
#50586=CARTESIAN_POINT('Ctrl Pts',(-7.25289334992292,3.16537847140652,90.2266499361086));
#50587=CARTESIAN_POINT('Ctrl Pts',(-7.33074559233991,2.98063483199827,90.2346814592445));
#50588=CARTESIAN_POINT('Ctrl Pts',(-7.40144652869959,2.79329738531379,90.2427129823805));
#50589=CARTESIAN_POINT('Ctrl Pts',(-7.47218534022186,2.60585958018117,90.2507488080797));
#50590=CARTESIAN_POINT('Ctrl Pts',(-7.53576509030279,2.41582550177319,90.2587846337788));
#50591=CARTESIAN_POINT('Ctrl Pts',(-7.5920182070502,2.22377619013655,90.266820459478));
#50592=CARTESIAN_POINT('Ctrl Pts',(-7.64834272464466,2.03148311452171,90.2748664848744));
#50593=CARTESIAN_POINT('Ctrl Pts',(-7.69732193257746,1.83717000750674,90.2829125102708));
#50594=CARTESIAN_POINT('Ctrl Pts',(-7.7388388401238,1.6414305975555,90.2909585356672));
#50595=CARTESIAN_POINT('Ctrl Pts',(-7.78038381628874,1.44555885272749,90.2990100007949));
#50596=CARTESIAN_POINT('Ctrl Pts',(-7.81445637095806,1.24825920224464,90.3070614659225));
#50597=CARTESIAN_POINT('Ctrl Pts',(-7.84099122394232,1.05013219456386,90.3151129310502));
#50598=CARTESIAN_POINT('Ctrl Pts',(-7.86756582474199,0.851708403036846,
90.3231764568495));
#50599=CARTESIAN_POINT('Ctrl Pts',(-7.88658012332793,0.652455101885583,
90.3312399826488));
#50600=CARTESIAN_POINT('Ctrl Pts',(-7.89802086058761,0.452976252934894,
90.3393035084481));
#50601=CARTESIAN_POINT('Ctrl Pts',(-7.90668697854369,0.301875218490092,
90.3454114597219));
#50602=CARTESIAN_POINT('Ctrl Pts',(-7.91100865671468,0.150644818809502,
90.3515194109957));
#50603=CARTESIAN_POINT('Ctrl Pts',(-7.91099998697758,-0.000453917034045954,
90.3576273622695));
#50604=CARTESIAN_POINT('',(-7.91348203759552,0.000837024955133735,92.3578223768916));
#50605=CARTESIAN_POINT('Ctrl Pts',(-7.91099998641113,-0.000451624858829035,
90.3576866635156));
#50606=CARTESIAN_POINT('Ctrl Pts',(-7.91086750422562,-2.20197461812199,
90.4462680419976));
#50607=CARTESIAN_POINT('Ctrl Pts',(-6.94203417908043,-4.38620523289174,
90.5348494204795));
#50608=CARTESIAN_POINT('Ctrl Pts',(-3.67820201487802,-7.34180684107875,
90.7120182346941));
#50609=CARTESIAN_POINT('Ctrl Pts',(-1.40868175871207,-8.08992666571431,
90.8006056704269));
#50610=CARTESIAN_POINT('Ctrl Pts',(2.97309270521788,-7.65454228025058,90.9777805418923));
#50611=CARTESIAN_POINT('Ctrl Pts',(5.0510207267604,-6.47444880833885,91.066367977625));
#50612=CARTESIAN_POINT('Ctrl Pts',(7.66951518848072,-2.93425195367184,91.2435428490905));
#50613=CARTESIAN_POINT('Ctrl Pts',(8.18956872247113,-0.601881960093553,
91.3321302848232));
#50614=CARTESIAN_POINT('Ctrl Pts',(7.32306689761086,3.71537198232957,91.5093051562887));
#50615=CARTESIAN_POINT('Ctrl Pts',(5.94329958849807,5.66643518936925,91.5978925920214));
#50616=CARTESIAN_POINT('Ctrl Pts',(2.16154501637291,7.9220591323315,91.7750674634869));
#50617=CARTESIAN_POINT('Ctrl Pts',(-0.210816529306171,8.20894963712988,
91.8636548992196));
#50618=CARTESIAN_POINT('Ctrl Pts',(-4.42123908576931,6.91982244717516,92.040829770685));
#50619=CARTESIAN_POINT('Ctrl Pts',(-6.22631625634573,5.35390358803074,92.1294172064178));
#50620=CARTESIAN_POINT('Ctrl Pts',(-7.65305292437075,2.31360404201413,92.2645479040777));
#50621=CARTESIAN_POINT('Ctrl Pts',(-7.91087421866498,1.15759242186707,92.3110911660047));
#50622=CARTESIAN_POINT('Ctrl Pts',(-7.91099995398858,0.00084659301766466,
92.3576344279319));
#50623=CARTESIAN_POINT('',(-7.89534346295974,0.00069161415478913,94.3576955927382));
#50624=CARTESIAN_POINT('Ctrl Pts',(-7.9137082678045,0.000836152871381276,
92.3578395075525));
#50625=CARTESIAN_POINT('Ctrl Pts',(-7.90855828367506,-0.731198149654099,
92.3873058786017));
#50626=CARTESIAN_POINT('Ctrl Pts',(-7.60962963928138,-2.78494886841547,
92.4698108260254));
#50627=CARTESIAN_POINT('Ctrl Pts',(-5.22373353997936,-6.99284294143041,
92.6583929261981));
#50628=CARTESIAN_POINT('Ctrl Pts',(1.91752129298265,-9.16215704951927,92.9235858080707));
#50629=CARTESIAN_POINT('Ctrl Pts',(8.74828639842495,-3.32800690420377,93.2418172663172));
#50630=CARTESIAN_POINT('Ctrl Pts',(7.52558118799366,5.55410540008025,93.560048724564));
#50631=CARTESIAN_POINT('Ctrl Pts',(-0.601507980866756,9.34057455472231,
93.8782801828113));
#50632=CARTESIAN_POINT('Ctrl Pts',(-6.94138208571764,5.32395168258709,94.1441534385439));
#50633=CARTESIAN_POINT('Ctrl Pts',(-7.89629725284548,1.34085654164704,94.3039495415281));
#50634=CARTESIAN_POINT('Ctrl Pts',(-7.89534399850304,0.00136738064416724,
94.3576684917632));
#50635=CARTESIAN_POINT('',(-7.91175229129129,-4.45848290299239E-5,96.3563650965844));
#50636=CARTESIAN_POINT('Ctrl Pts',(-7.89534292741644,1.58476654102983E-5,
94.3577226937131));
#50637=CARTESIAN_POINT('Ctrl Pts',(-7.89534100553285,-0.00218476492922217,
94.3578109471868));
#50638=CARTESIAN_POINT('Ctrl Pts',(-7.89533858281069,-0.00411872059818796,
94.3578885065983));
#50639=CARTESIAN_POINT('Ctrl Pts',(-7.89533499935064,-0.00631604597571947,
94.357976628182));
#50640=CARTESIAN_POINT('Ctrl Pts',(-7.89494973591493,-0.242553959490402,
94.3674507184937));
#50641=CARTESIAN_POINT('Ctrl Pts',(-7.8841455758433,-0.479166263720991,
94.376708057421));
#50642=CARTESIAN_POINT('Ctrl Pts',(-7.86299604179089,-0.71502109617178,
94.3858293751233));
#50643=CARTESIAN_POINT('Ctrl Pts',(-7.8417777960691,-0.951642185658164,
94.3949803266211));
#50644=CARTESIAN_POINT('Ctrl Pts',(-7.81014756052766,-1.18750036699406,
94.403994371633));
#50645=CARTESIAN_POINT('Ctrl Pts',(-7.76821154680769,-1.42149411747968,
94.4129530297179));
#50646=CARTESIAN_POINT('Ctrl Pts',(-7.72630123746556,-1.65534444317972,
94.4219061966579));
#50647=CARTESIAN_POINT('Ctrl Pts',(-7.67409852972891,-1.88733229461253,
94.4308040445481));
#50648=CARTESIAN_POINT('Ctrl Pts',(-7.61173028829981,-2.1164056968663,94.4397279431391));
#50649=CARTESIAN_POINT('Ctrl Pts',(-7.54951510244527,-2.34491693862951,
94.4486299419236));
#50650=CARTESIAN_POINT('Ctrl Pts',(-7.47718496765697,-2.57052786406193,
94.4575578637056));
#50651=CARTESIAN_POINT('Ctrl Pts',(-7.39487531212015,-2.79224511439129,
94.466592480645));
#50652=CARTESIAN_POINT('Ctrl Pts',(-7.31283718645635,-3.01323094558839,
94.4755972934457));
#50653=CARTESIAN_POINT('Ctrl Pts',(-7.22088601136339,-3.23034875908435,
94.4847080986156));
#50654=CARTESIAN_POINT('Ctrl Pts',(-7.11915418516265,-3.44266666809989,
94.4940048715749));
#50655=CARTESIAN_POINT('Ctrl Pts',(-7.0699761682239,-3.54530292379201,94.4984990094976));
#50656=CARTESIAN_POINT('Ctrl Pts',(-7.01851247856327,-3.64681829260696,
94.5030366050537));
#50657=CARTESIAN_POINT('Ctrl Pts',(-6.96477715111767,-3.74711178296017,
94.5076266926376));
#50658=CARTESIAN_POINT('Ctrl Pts',(-6.85450764867543,-3.95292263040759,
94.5170459461921));
#50659=CARTESIAN_POINT('Ctrl Pts',(-6.73467378089451,-4.15358522068934,
94.5266862466224));
#50660=CARTESIAN_POINT('Ctrl Pts',(-6.60615843297703,-4.34865370677128,
94.5366256641826));
#50661=CARTESIAN_POINT('Ctrl Pts',(-6.48405065385526,-4.53399639150189,
94.5460695183502));
#50662=CARTESIAN_POINT('Ctrl Pts',(-6.3541058958454,-4.71428950597768,94.5557834062116));
#50663=CARTESIAN_POINT('Ctrl Pts',(-6.21705650342287,-4.88918645561241,
94.5658342931876));
#50664=CARTESIAN_POINT('Ctrl Pts',(-6.10664964088334,-5.03008327489469,
94.5739312783484));
#50665=CARTESIAN_POINT('Ctrl Pts',(-5.99137346960744,-5.1670881326108,94.5819830907967));
#50666=CARTESIAN_POINT('Ctrl Pts',(-5.87141429726191,-5.29988137000902,
94.589879209913));
#50667=CARTESIAN_POINT('Ctrl Pts',(-5.75157619366024,-5.43254058588864,
94.5977673598745));
#50668=CARTESIAN_POINT('Ctrl Pts',(-5.62706391422946,-5.56099639982551,
94.6055001306122));
#50669=CARTESIAN_POINT('Ctrl Pts',(-5.49808382191283,-5.68488255749942,
94.612967335798));
#50670=CARTESIAN_POINT('Ctrl Pts',(-5.43572154205482,-5.74478190395382,
94.6165777529655));
#50671=CARTESIAN_POINT('Ctrl Pts',(-5.37231516452397,-5.80361229321,94.6201260874695));
#50672=CARTESIAN_POINT('Ctrl Pts',(-5.30789038223661,-5.86132864337651,
94.6235998848297));
#50673=CARTESIAN_POINT('Ctrl Pts',(-5.08342662142632,-6.06241941246647,
94.6357030164522));
#50674=CARTESIAN_POINT('Ctrl Pts',(-4.84723506706229,-6.25108700614638,
94.6476322608195));
#50675=CARTESIAN_POINT('Ctrl Pts',(-4.60109727133566,-6.42610935418111,
94.6594544706515));
#50676=CARTESIAN_POINT('Ctrl Pts',(-4.50680645297714,-6.49315716525988,
94.6639833396803));
#50677=CARTESIAN_POINT('Ctrl Pts',(-4.41105590223857,-6.55820305847355,
94.6684965012432));
#50678=CARTESIAN_POINT('Ctrl Pts',(-4.31394518764209,-6.62118026040317,
94.6729977136483));
#50679=CARTESIAN_POINT('Ctrl Pts',(-4.05854234315178,-6.78681138131193,
94.6848359794534));
#50680=CARTESIAN_POINT('Ctrl Pts',(-3.79373341421565,-6.93813033637002,
94.6965915930514));
#50681=CARTESIAN_POINT('Ctrl Pts',(-3.5214291932744,-7.07413416149846,94.7083329248413));
#50682=CARTESIAN_POINT('Ctrl Pts',(-3.24875448172607,-7.21032303017695,
94.7200902316062));
#50683=CARTESIAN_POINT('Ctrl Pts',(-2.96856483070124,-7.33115582289544,
94.7318332176736));
#50684=CARTESIAN_POINT('Ctrl Pts',(-2.68274243446052,-7.43566256934059,
94.7436305328917));
#50685=CARTESIAN_POINT('Ctrl Pts',(-2.39793828801589,-7.53979700775578,
94.7553858198644));
#50686=CARTESIAN_POINT('Ctrl Pts',(-2.10754195593512,-7.62772242160117,
94.7671950495793));
#50687=CARTESIAN_POINT('Ctrl Pts',(-1.81337008770093,-7.69850348437741,
94.7791261407947));
#50688=CARTESIAN_POINT('Ctrl Pts',(-1.52167118980876,-7.76868952265293,
94.7909569327025));
#50689=CARTESIAN_POINT('Ctrl Pts',(-1.22626018781794,-7.82201924741345,
94.8029075458534));
#50690=CARTESIAN_POINT('Ctrl Pts',(-0.928858225085867,-7.85759046373914,
94.8150442004776));
#50691=CARTESIAN_POINT('Ctrl Pts',(-0.824197036538944,-7.87010862516789,
94.8193153111532));
#50692=CARTESIAN_POINT('Ctrl Pts',(-0.719288805131689,-7.88042747494532,
94.8236094624102));
#50693=CARTESIAN_POINT('Ctrl Pts',(-0.614207000587532,-7.88850761447765,
94.8279295403805));
#50694=CARTESIAN_POINT('Ctrl Pts',(-0.321228819834413,-7.91103582086582,
94.8399743333869));
#50695=CARTESIAN_POINT('Ctrl Pts',(-0.0269049073670538,-7.91616263996339,
94.8522206671931));
#50696=CARTESIAN_POINT('Ctrl Pts',(0.267116403962486,-7.90475530100067,
94.8647310935471));
#50697=CARTESIAN_POINT('Ctrl Pts',(0.438879687916884,-7.898091287455,94.872039515867));
#50698=CARTESIAN_POINT('Ctrl Pts',(0.610540626108601,-7.88578434077762,
94.8794380660752));
#50699=CARTESIAN_POINT('Ctrl Pts',(0.781778134030084,-7.86800393038236,
94.8869392149633));
#50700=CARTESIAN_POINT('Ctrl Pts',(0.990272335153488,-7.84635497913328,
94.8960724128468));
#50701=CARTESIAN_POINT('Ctrl Pts',(1.19769759054455,-7.81605049268673,94.9050024100971));
#50702=CARTESIAN_POINT('Ctrl Pts',(1.4035102551961,-7.77751410296379,94.9137855452439));
#50703=CARTESIAN_POINT('Ctrl Pts',(1.61153801110222,-7.73856295927029,94.9226632102676));
#50704=CARTESIAN_POINT('Ctrl Pts',(1.81791877285403,-7.69120199890053,94.931390834923));
#50705=CARTESIAN_POINT('Ctrl Pts',(2.02212431683724,-7.63582626547788,94.9400265964449));
#50706=CARTESIAN_POINT('Ctrl Pts',(2.22898882802423,-7.5797294827821,94.9487748045058));
#50707=CARTESIAN_POINT('Ctrl Pts',(2.43362168331101,-7.5154080927409,94.9574287415523));
#50708=CARTESIAN_POINT('Ctrl Pts',(2.63549947541872,-7.44322580125453,94.9660488871222));
#50709=CARTESIAN_POINT('Ctrl Pts',(2.75827799668934,-7.39932580156614,94.9712915079928));
#50710=CARTESIAN_POINT('Ctrl Pts',(2.88003792388024,-7.35251723702134,94.9765216298747));
#50711=CARTESIAN_POINT('Ctrl Pts',(3.00066460806138,-7.30287304158761,94.9817528581273));
#50712=CARTESIAN_POINT('Ctrl Pts',(3.25249594460139,-7.19923126305081,94.9926740503292));
#50713=CARTESIAN_POINT('Ctrl Pts',(3.499365700582,-7.08278886020871,95.0033667402724));
#50714=CARTESIAN_POINT('Ctrl Pts',(3.73986399801828,-6.95426081533967,95.0139265904244));
#50715=CARTESIAN_POINT('Ctrl Pts',(3.98899794096346,-6.82111767487423,95.0248656163275));
#50716=CARTESIAN_POINT('Ctrl Pts',(4.23129481725793,-6.6750066424291,95.035662091327));
#50717=CARTESIAN_POINT('Ctrl Pts',(4.46524258947272,-6.51670421475433,95.046422357286));
#50718=CARTESIAN_POINT('Ctrl Pts',(4.691060121441,-6.36390317209562,95.0568086784686));
#50719=CARTESIAN_POINT('Ctrl Pts',(4.90909972038032,-6.1997441618502,95.0671612635803));
#50720=CARTESIAN_POINT('Ctrl Pts',(5.11804272480831,-6.02489396212108,95.0775757484205));
#50721=CARTESIAN_POINT('Ctrl Pts',(5.32415330391685,-5.85241402663785,95.0878490548056));
#50722=CARTESIAN_POINT('Ctrl Pts',(5.52141317268533,-5.66953150135819,95.0981825940724));
#50723=CARTESIAN_POINT('Ctrl Pts',(5.7085837663623,-5.47684411697809,95.108668165197));
#50724=CARTESIAN_POINT('Ctrl Pts',(5.88994050679585,-5.29014194722298,95.1188280357375));
#50725=CARTESIAN_POINT('Ctrl Pts',(6.06182604291708,-5.09423494806226,95.1291306400588));
#50726=CARTESIAN_POINT('Ctrl Pts',(6.22312501876962,-4.88961927936072,95.1396594857775));
#50727=CARTESIAN_POINT('Ctrl Pts',(6.25109883642619,-4.85413311848659,95.1414854862758));
#50728=CARTESIAN_POINT('Ctrl Pts',(6.27875424423695,-4.81838489689965,95.1433182915265));
#50729=CARTESIAN_POINT('Ctrl Pts',(6.30608542407995,-4.78237703912036,95.1451583371284));
#50730=CARTESIAN_POINT('Ctrl Pts',(6.32526741042165,-4.75710545406317,95.1464497460542));
#50731=CARTESIAN_POINT('Ctrl Pts',(6.34428969055677,-4.73170597803243,95.1477447213798));
#50732=CARTESIAN_POINT('Ctrl Pts',(6.36315210291656,-4.70618089701231,95.1490434136937));
#50733=CARTESIAN_POINT('Ctrl Pts',(6.50744063091238,-4.5109261068446,95.1589777952948));
#50734=CARTESIAN_POINT('Ctrl Pts',(6.64197303335215,-4.30883982975102,95.1690924217835));
#50735=CARTESIAN_POINT('Ctrl Pts',(6.76661025656409,-4.100890200801,95.1793029581414));
#50736=CARTESIAN_POINT('Ctrl Pts',(6.89623385261474,-3.8846211119425,95.1899219883654));
#50737=CARTESIAN_POINT('Ctrl Pts',(7.01515418370291,-3.66200912270891,95.2006447561186));
#50738=CARTESIAN_POINT('Ctrl Pts',(7.12316187524308,-3.43416186488374,95.2113763940341));
#50739=CARTESIAN_POINT('Ctrl Pts',(7.23238618389855,-3.20374809656665,95.222228914955));
#50740=CARTESIAN_POINT('Ctrl Pts',(7.33044977485948,-2.9679796290668,95.2330905069936));
#50741=CARTESIAN_POINT('Ctrl Pts',(7.41709369809658,-2.72803464773274,95.2438630607299));
#50742=CARTESIAN_POINT('Ctrl Pts',(7.5040678757603,-2.48717508532628,95.2546766754365));
#50743=CARTESIAN_POINT('Ctrl Pts',(7.57953421124156,-2.24210651772726,95.2654005717852));
#50744=CARTESIAN_POINT('Ctrl Pts',(7.64320198233374,-1.99406408260649,95.2759355142046));
#50745=CARTESIAN_POINT('Ctrl Pts',(7.66664902386801,-1.90271706073385,95.2798152358947));
#50746=CARTESIAN_POINT('Ctrl Pts',(7.68849568765391,-1.81096717658473,95.2836693308816));
#50747=CARTESIAN_POINT('Ctrl Pts',(7.70872687526107,-1.71887781026362,95.2874928426938));
#50748=CARTESIAN_POINT('Ctrl Pts',(7.75898361138552,-1.49011659896288,95.2969909121075));
#50749=CARTESIAN_POINT('Ctrl Pts',(7.79954659050739,-1.25928664176328,95.3064578422713));
#50750=CARTESIAN_POINT('Ctrl Pts',(7.83026459247564,-1.02719205262028,95.3158665627013));
#50751=CARTESIAN_POINT('Ctrl Pts',(7.86070706604573,-0.797179260673331,
95.3251908906089));
#50752=CARTESIAN_POINT('Ctrl Pts',(7.88148014767695,-0.565923622146464,
95.3344580483361));
#50753=CARTESIAN_POINT('Ctrl Pts',(7.89238767747411,-0.334220330441234,
95.3436416873198));
#50754=CARTESIAN_POINT('Ctrl Pts',(7.9031503468454,-0.105594237527625,95.3527033604799));
#50755=CARTESIAN_POINT('Ctrl Pts',(7.90430751752217,0.123468375233821,95.3616837185523));
#50756=CARTESIAN_POINT('Ctrl Pts',(7.89562647892617,0.352180447046821,95.3705574488811));
#50757=CARTESIAN_POINT('Ctrl Pts',(7.88717230511806,0.574915501814209,95.3791992787378));
#50758=CARTESIAN_POINT('Ctrl Pts',(7.8693871037499,0.797318582573102,95.3877399811137));
#50759=CARTESIAN_POINT('Ctrl Pts',(7.84201791527239,1.01863228290947,95.3961561764574));
#50760=CARTESIAN_POINT('Ctrl Pts',(7.81972748646366,1.19887793709816,95.403010621678));
#50761=CARTESIAN_POINT('Ctrl Pts',(7.79107922300819,1.37840056851073,95.409782480812));
#50762=CARTESIAN_POINT('Ctrl Pts',(7.75591905237436,1.55677219662619,95.4164591237919));
#50763=CARTESIAN_POINT('Ctrl Pts',(7.70399925959459,1.8201673338681,95.4263182886859));
#50764=CARTESIAN_POINT('Ctrl Pts',(7.63898456107242,2.08058599369728,95.4365195678523));
#50765=CARTESIAN_POINT('Ctrl Pts',(7.56051601014418,2.33664673504757,95.4469859602393));
#50766=CARTESIAN_POINT('Ctrl Pts',(7.52068164815656,2.46663532463033,95.4522991979393));
#50767=CARTESIAN_POINT('Ctrl Pts',(7.47738015587361,2.59549999938065,95.4576807568967));
#50768=CARTESIAN_POINT('Ctrl Pts',(7.43056524834723,2.72305495898814,95.463120563543));
#50769=CARTESIAN_POINT('Ctrl Pts',(7.33699259977474,2.97800911867122,95.4739935341951));
#50770=CARTESIAN_POINT('Ctrl Pts',(7.22938209043632,3.22773380596663,95.4850992111801));
#50771=CARTESIAN_POINT('Ctrl Pts',(7.10875465450052,3.47122856406998,95.4963571534699));
#50772=CARTESIAN_POINT('Ctrl Pts',(6.98745956561423,3.71607102547493,95.5076774066124));
#50773=CARTESIAN_POINT('Ctrl Pts',(6.85300226629674,3.95461386141648,95.5191516152508));
#50774=CARTESIAN_POINT('Ctrl Pts',(6.70644811440811,4.18579495424151,95.530697995267));
#50775=CARTESIAN_POINT('Ctrl Pts',(6.5591113642813,4.41821055263064,95.542306032879));
#50776=CARTESIAN_POINT('Ctrl Pts',(6.39954757251653,4.64318485801121,95.5539870147162));
#50777=CARTESIAN_POINT('Ctrl Pts',(6.22887775388047,4.85960282968115,95.5656578394716));
#50778=CARTESIAN_POINT('Ctrl Pts',(6.05843496404739,5.07573291733362,95.5773131394353));
#50779=CARTESIAN_POINT('Ctrl Pts',(5.8769152431992,5.2833285187262,95.5889583093217));
#50780=CARTESIAN_POINT('Ctrl Pts',(5.68548149276933,5.48125562332238,95.6005105790124));
#50781=CARTESIAN_POINT('Ctrl Pts',(5.49590911641781,5.67725821679619,95.6119505221394));
#50782=CARTESIAN_POINT('Ctrl Pts',(5.29661439405186,5.86377840795389,95.6232993628868));
#50783=CARTESIAN_POINT('Ctrl Pts',(5.08877650123915,6.03970626308767,95.6344767221404));
#50784=CARTESIAN_POINT('Ctrl Pts',(4.9435858722972,6.16260529554803,95.6422849605611));
#50785=CARTESIAN_POINT('Ctrl Pts',(4.79422715432221,6.28033496272848,95.6500095144926));
#50786=CARTESIAN_POINT('Ctrl Pts',(4.64111741998645,6.39251848315742,95.6576229817758));
#50787=CARTESIAN_POINT('Ctrl Pts',(4.50985051667586,6.48869775871474,95.664150302054));
#50788=CARTESIAN_POINT('Ctrl Pts',(4.37573012004144,6.5810382843292,95.6706810766281));
#50789=CARTESIAN_POINT('Ctrl Pts',(4.2388122776661,6.6692204070492,95.6771207269103));
#50790=CARTESIAN_POINT('Ctrl Pts',(4.17603526051647,6.70965203038073,95.6800733153326));
#50791=CARTESIAN_POINT('Ctrl Pts',(4.11267048510002,6.74920882288298,95.6830067472875));
#50792=CARTESIAN_POINT('Ctrl Pts',(4.04872521441862,6.78785680626155,95.6859119065566));
#50793=CARTESIAN_POINT('Ctrl Pts',(3.8594739302814,6.90223868948401,95.6945099641839));
#50794=CARTESIAN_POINT('Ctrl Pts',(3.66522601748946,7.00886792686582,95.7029934026401));
#50795=CARTESIAN_POINT('Ctrl Pts',(3.46675775369528,7.10714538394219,95.7114238857058));
#50796=CARTESIAN_POINT('Ctrl Pts',(3.2690302159716,7.20505604849865,95.7198229044031));
#50797=CARTESIAN_POINT('Ctrl Pts',(3.06711452315287,7.29467719512274,95.728169362254));
#50798=CARTESIAN_POINT('Ctrl Pts',(2.86177508594341,7.37546778374205,95.7365242351857));
#50799=CARTESIAN_POINT('Ctrl Pts',(2.65822634073895,7.45555382644906,95.7448062482501));
#50800=CARTESIAN_POINT('Ctrl Pts',(2.4513139447209,7.52696280965348,95.7530965302653));
#50801=CARTESIAN_POINT('Ctrl Pts',(2.24176898568361,7.5892168383936,95.7614544757817));
#50802=CARTESIAN_POINT('Ctrl Pts',(2.07152115430481,7.63979602405519,95.7682450094481));
#50803=CARTESIAN_POINT('Ctrl Pts',(1.89953544225083,7.68433299485283,95.7750802076896));
#50804=CARTESIAN_POINT('Ctrl Pts',(1.72619315043018,7.72259443194149,95.7819919241935));
#50805=CARTESIAN_POINT('Ctrl Pts',(1.51152103309105,7.76997850437985,95.7905515942011));
#50806=CARTESIAN_POINT('Ctrl Pts',(1.29476966977163,7.80773694119226,95.7992286207526));
#50807=CARTESIAN_POINT('Ctrl Pts',(1.07680296937618,7.83621616594034,95.808083506307));
#50808=CARTESIAN_POINT('Ctrl Pts',(0.858510041804163,7.86473801507583,95.816951644823));
#50809=CARTESIAN_POINT('Ctrl Pts',(0.638998681851458,7.88395354531904,95.8259981751378));
#50810=CARTESIAN_POINT('Ctrl Pts',(0.419097366059129,7.89424503100409,95.8352838717764));
#50811=CARTESIAN_POINT('Ctrl Pts',(0.200450360998181,7.9044778143531,95.8445166030705));
#50812=CARTESIAN_POINT('Ctrl Pts',(-0.0185817889182326,7.90588874189786,
95.8539857800743));
#50813=CARTESIAN_POINT('Ctrl Pts',(-0.237230341947614,7.89887720199766,
95.8637511432652));
#50814=CARTESIAN_POINT('Ctrl Pts',(-0.274561099084255,7.89768009326064,
95.8654184234579));
#50815=CARTESIAN_POINT('Ctrl Pts',(-0.311880789818695,7.8962375108515,95.8670943375142));
#50816=CARTESIAN_POINT('Ctrl Pts',(-0.349185733300582,7.89455149027729,
95.8687791827576));
#50817=CARTESIAN_POINT('Ctrl Pts',(-0.538494228772429,7.88599557279161,
95.8773291358834));
#50818=CARTESIAN_POINT('Ctrl Pts',(-0.72735735993748,7.87030059175063,95.8856029470287));
#50819=CARTESIAN_POINT('Ctrl Pts',(-0.915345549147819,7.84777852947421,
95.8936804113027));
#50820=CARTESIAN_POINT('Ctrl Pts',(-1.10475219890014,7.8250865274968,95.9018188238969));
#50821=CARTESIAN_POINT('Ctrl Pts',(-1.29327105689764,7.79546439524873,95.9097579153795));
#50822=CARTESIAN_POINT('Ctrl Pts',(-1.4805043442638,7.7591980005021,95.9175793007997));
#50823=CARTESIAN_POINT('Ctrl Pts',(-1.66924469039254,7.72263969405132,95.9254636413045));
#50824=CARTESIAN_POINT('Ctrl Pts',(-1.85667916095413,7.67933010587731,95.933228373266));
#50825=CARTESIAN_POINT('Ctrl Pts',(-2.04243577504038,7.62952283008212,95.9409570984214));
#50826=CARTESIAN_POINT('Ctrl Pts',(-2.13273456251568,7.60531084369404,95.9447141356267));
#50827=CARTESIAN_POINT('Ctrl Pts',(-2.22263734885794,7.57956279034144,95.9484626641976));
#50828=CARTESIAN_POINT('Ctrl Pts',(-2.31210385396676,7.55230409462123,95.9522122876043));
#50829=CARTESIAN_POINT('Ctrl Pts',(-2.52277369089802,7.4881171122936,95.9610416539766));
#50830=CARTESIAN_POINT('Ctrl Pts',(-2.73113406439668,7.41506052231833,95.9696350598388));
#50831=CARTESIAN_POINT('Ctrl Pts',(-2.93628257126045,7.33347201603543,95.9780772240315));
#50832=CARTESIAN_POINT('Ctrl Pts',(-3.14175621895565,7.25175419974598,95.9865327682499));
#50833=CARTESIAN_POINT('Ctrl Pts',(-3.34400753884291,7.16147815677355,95.9948365910117));
#50834=CARTESIAN_POINT('Ctrl Pts',(-3.5421783994591,7.06300229683345,96.0030738146103));
#50835=CARTESIAN_POINT('Ctrl Pts',(-3.7400392144396,6.96468050601582,96.0112981507681));
#50836=CARTESIAN_POINT('Ctrl Pts',(-3.93383221393402,6.85818527569541,96.0194560959933));
#50837=CARTESIAN_POINT('Ctrl Pts',(-4.12275452664767,6.74388114006049,96.0276323736732));
#50838=CARTESIAN_POINT('Ctrl Pts',(-4.31122247602586,6.62985190900183,96.0357889871814));
#50839=CARTESIAN_POINT('Ctrl Pts',(-4.49484316467593,6.508051989285,96.0439638450702));
#50840=CARTESIAN_POINT('Ctrl Pts',(-4.67287117856765,6.3788402829317,96.0522410609095));
#50841=CARTESIAN_POINT('Ctrl Pts',(-4.85040866823104,6.24998459623601,96.0604954703667));
#50842=CARTESIAN_POINT('Ctrl Pts',(-5.02238441735062,6.11375856238643,96.0688516744936));
#50843=CARTESIAN_POINT('Ctrl Pts',(-5.18810922960627,5.97050501405808,96.0773930934946));
#50844=CARTESIAN_POINT('Ctrl Pts',(-5.31644066140156,5.85957453408643,96.0840072662008));
#50845=CARTESIAN_POINT('Ctrl Pts',(-5.44102482967134,5.7444298897345,96.0907325012597));
#50846=CARTESIAN_POINT('Ctrl Pts',(-5.56156121099912,5.62522120200396,96.0976075340458));
#50847=CARTESIAN_POINT('Ctrl Pts',(-5.71925048114818,5.46926886000907,96.1066016559065));
#50848=CARTESIAN_POINT('Ctrl Pts',(-5.87001100066274,5.30636278252122,96.1158521513142));
#50849=CARTESIAN_POINT('Ctrl Pts',(-6.01376735822492,5.13738654839755,96.1254457483515));
#50850=CARTESIAN_POINT('Ctrl Pts',(-6.15752371578701,4.96841031427398,96.1350393453888));
#50851=CARTESIAN_POINT('Ctrl Pts',(-6.29427647074201,4.79336454690273,96.1449760440555));
#50852=CARTESIAN_POINT('Ctrl Pts',(-6.4239862901908,4.61308959593157,96.155342572434));
#50853=CARTESIAN_POINT('Ctrl Pts',(-6.55088879474878,4.43671634304658,96.1654847376177));
#50854=CARTESIAN_POINT('Ctrl Pts',(-6.66981469275507,4.25476027087685,96.1752518688182));
#50855=CARTESIAN_POINT('Ctrl Pts',(-6.78067563690051,4.06803364556051,96.1846930936941));
#50856=CARTESIAN_POINT('Ctrl Pts',(-6.89419944722437,3.87682186977934,96.1943610956247));
#50857=CARTESIAN_POINT('Ctrl Pts',(-6.99926676695183,3.68060738080236,96.2036873467384));
#50858=CARTESIAN_POINT('Ctrl Pts',(-7.09577185797243,3.48020914404722,96.2127246005285));
#50859=CARTESIAN_POINT('Ctrl Pts',(-7.11542939169053,3.43938917222604,96.2145654373095));
#50860=CARTESIAN_POINT('Ctrl Pts',(-7.13473161541277,3.39839544573362,96.2163942832001));
#50861=CARTESIAN_POINT('Ctrl Pts',(-7.15367754904318,3.3572346392387,96.2182115840493));
#50862=CARTESIAN_POINT('Ctrl Pts',(-7.25200300283662,3.14361861713775,96.2276429973625));
#50863=CARTESIAN_POINT('Ctrl Pts',(-7.34116641750469,2.9258357364677,96.2370648513991));
#50864=CARTESIAN_POINT('Ctrl Pts',(-7.4209725176741,2.7046873025448,96.2464754577597));
#50865=CARTESIAN_POINT('Ctrl Pts',(-7.50120798246339,2.48234906843032,96.2559366941024));
#50866=CARTESIAN_POINT('Ctrl Pts',(-7.57198539139196,2.25660814656931,96.2653865614164));
#50867=CARTESIAN_POINT('Ctrl Pts',(-7.63305716512908,2.0282612805973,96.2748233439042));
#50868=CARTESIAN_POINT('Ctrl Pts',(-7.69358059489057,1.8019646682965,96.2841753965322));
#50869=CARTESIAN_POINT('Ctrl Pts',(-7.74457199343469,1.57310788518565,96.2935145982482));
#50870=CARTESIAN_POINT('Ctrl Pts',(-7.78574009386206,1.34246146366351,96.3028392790578));
#50871=CARTESIAN_POINT('Ctrl Pts',(-7.82577159118107,1.1181829201079,96.3119065163351));
#50872=CARTESIAN_POINT('Ctrl Pts',(-7.8565146589521,0.892211509128002,96.320960023448));
#50873=CARTESIAN_POINT('Ctrl Pts',(-7.87765371442561,0.66526191660585,96.3299982649382));
#50874=CARTESIAN_POINT('Ctrl Pts',(-7.89824468402497,0.44419659199532,96.3388021661338));
#50875=CARTESIAN_POINT('Ctrl Pts',(-7.90972315218024,0.222202594470807,
96.3475915830478));
#50876=CARTESIAN_POINT('Ctrl Pts',(-7.91175229129129,-4.45848290304383E-5,
96.3563650965844));
#50877=CARTESIAN_POINT('',(-7.91868362782468,0.00154658286907643,98.357726602302));
#50878=CARTESIAN_POINT('Ctrl Pts',(-7.911,-4.14168699336415E-12,96.3576684917632));
#50879=CARTESIAN_POINT('Ctrl Pts',(-7.91099999999885,-2.20167589667079,
96.4462559274959));
#50880=CARTESIAN_POINT('Ctrl Pts',(-6.94214576672153,-4.38610418339023,
96.5348433632286));
#50881=CARTESIAN_POINT('Ctrl Pts',(-3.67820201487944,-7.341806841078,96.7120182346941));
#50882=CARTESIAN_POINT('Ctrl Pts',(-1.40868175871382,-8.08992666571396,
96.8006056704268));
#50883=CARTESIAN_POINT('Ctrl Pts',(2.97309270521593,-7.6545422802513,96.9777805418923));
#50884=CARTESIAN_POINT('Ctrl Pts',(5.0510207267586,-6.47444880834021,97.066367977625));
#50885=CARTESIAN_POINT('Ctrl Pts',(7.66951518847978,-2.9342519536742,97.2435428490904));
#50886=CARTESIAN_POINT('Ctrl Pts',(8.1895687224709,-0.601881960096264,97.3321302848231));
#50887=CARTESIAN_POINT('Ctrl Pts',(7.32306689761219,3.71537198232687,97.5093051562886));
#50888=CARTESIAN_POINT('Ctrl Pts',(5.94329958850025,5.66643518936691,97.5978925920213));
#50889=CARTESIAN_POINT('Ctrl Pts',(2.16154501637625,7.92205913233055,97.7750674634867));
#50890=CARTESIAN_POINT('Ctrl Pts',(-0.210816529302517,8.20894963712994,
97.8636548992195));
#50891=CARTESIAN_POINT('Ctrl Pts',(-4.42123908576597,6.91982244717725,98.0408297706849));
#50892=CARTESIAN_POINT('Ctrl Pts',(-6.22631625634301,5.35390358803384,98.1294172064176));
#50893=CARTESIAN_POINT('Ctrl Pts',(-7.65294787893378,2.31382788822453,98.2645379548953));
#50894=CARTESIAN_POINT('Ctrl Pts',(-7.91076398318387,1.15808663968023,98.3110712676403));
#50895=CARTESIAN_POINT('Ctrl Pts',(-7.91099983803092,0.00158839793129274,
98.3576045803853));
#50896=CARTESIAN_POINT('',(-7.90591968225023,0.00541017765921074,100.357667186137));
#50897=CARTESIAN_POINT('Ctrl Pts',(-7.92261381100118,0.00152519487455055,
98.3577890153166));
#50898=CARTESIAN_POINT('Ctrl Pts',(-7.90753284617846,-2.42511318705542,
98.4557766957155));
#50899=CARTESIAN_POINT('Ctrl Pts',(-5.41078064749634,-7.50661730602548,
98.6598415288631));
#50900=CARTESIAN_POINT('Ctrl Pts',(1.74919137803737,-8.55146619143505,98.9169449383855));
#50901=CARTESIAN_POINT('Ctrl Pts',(6.19343569208429,-5.41096699287904,99.1290992438833));
#50902=CARTESIAN_POINT('Ctrl Pts',(8.70888107749104,-0.585350218599905,
99.3412535493814));
#50903=CARTESIAN_POINT('Ctrl Pts',(6.64946598043916,6.58836944045884,99.6064464312537));
#50904=CARTESIAN_POINT('Ctrl Pts',(-1.95996707955373,9.15241355656713,99.9246778895003));
#50905=CARTESIAN_POINT('Ctrl Pts',(-7.30433020370274,4.54693693773015,100.175084447898));
#50906=CARTESIAN_POINT('Ctrl Pts',(-7.90728284534243,0.958428727150744,
100.319413853548));
#50907=CARTESIAN_POINT('Ctrl Pts',(-7.90172002473078,0.00543421965308875,
100.357666106448));
#50908=CARTESIAN_POINT('',(-7.90607670224956,-0.00557672470292666,102.357669804003));
#50909=CARTESIAN_POINT('Ctrl Pts',(-7.91099816987171,0.00538110458176591,
100.357668491763));
#50910=CARTESIAN_POINT('Ctrl Pts',(-7.91113279599411,-0.192538670395385,
100.365603511931));
#50911=CARTESIAN_POINT('Ctrl Pts',(-7.90383567542204,-0.390497577918663,
100.3735385321));
#50912=CARTESIAN_POINT('Ctrl Pts',(-7.88912477896871,-0.587904092401064,
100.381473552268));
#50913=CARTESIAN_POINT('Ctrl Pts',(-7.8744106177791,-0.78535441660042,100.389410333427));
#50914=CARTESIAN_POINT('Ctrl Pts',(-7.85227941295536,-0.982251765136944,
100.397347114585));
#50915=CARTESIAN_POINT('Ctrl Pts',(-7.8228011557655,-1.17800809732108,100.405283895744));
#50916=CARTESIAN_POINT('Ctrl Pts',(-7.79331752937729,-1.37380008475337,
100.413222122516));
#50917=CARTESIAN_POINT('Ctrl Pts',(-7.75648423295182,-1.56845030693343,
100.421160349288));
#50918=CARTESIAN_POINT('Ctrl Pts',(-7.71242270003436,-1.76137931632989,
100.429098576059));
#50919=CARTESIAN_POINT('Ctrl Pts',(-7.66834613799111,-1.95437413265946,
100.437039510513));
#50920=CARTESIAN_POINT('Ctrl Pts',(-7.61703649998356,-2.1456462362215,100.444980444966));
#50921=CARTESIAN_POINT('Ctrl Pts',(-7.5586656439331,-2.33462945308789,100.45292137942));
#50922=CARTESIAN_POINT('Ctrl Pts',(-7.50026559888049,-2.52370717313441,
100.460866284827));
#50923=CARTESIAN_POINT('Ctrl Pts',(-7.43479739679541,-2.71049340213586,
100.468811190233));
#50924=CARTESIAN_POINT('Ctrl Pts',(-7.36248186594788,-2.89443980306875,
100.47675609564));
#50925=CARTESIAN_POINT('Ctrl Pts',(-7.29007834870731,-3.07861001180806,
100.484710667623));
#50926=CARTESIAN_POINT('Ctrl Pts',(-7.2108109822883,-3.25993317470558,100.492665239606));
#50927=CARTESIAN_POINT('Ctrl Pts',(-7.12494814906543,-3.4378823239211,100.500619811589));
#50928=CARTESIAN_POINT('Ctrl Pts',(-7.03902685184802,-3.61595263869448,
100.508579799839));
#50929=CARTESIAN_POINT('Ctrl Pts',(-6.94650129016071,-3.79064406045562,
100.516539788089));
#50930=CARTESIAN_POINT('Ctrl Pts',(-6.84768462299399,-3.96145633624955,
100.524499776339));
#50931=CARTESIAN_POINT('Ctrl Pts',(-6.74872617033783,-4.13251369926226,
100.532471185849));
#50932=CARTESIAN_POINT('Ctrl Pts',(-6.64345875685786,-4.29968051032878,
100.540442595359));
#50933=CARTESIAN_POINT('Ctrl Pts',(-6.53223824768452,-4.46248635577606,
100.548414004869));
#50934=CARTESIAN_POINT('Ctrl Pts',(-6.47304832652731,-4.54912923511173,
100.55265627191));
#50935=CARTESIAN_POINT('Ctrl Pts',(-6.41217304298212,-4.63453756222787,
100.556898538952));
#50936=CARTESIAN_POINT('Ctrl Pts',(-6.34967046958094,-4.71864450109687,
100.561140805994));
#50937=CARTESIAN_POINT('Ctrl Pts',(-6.23417869960183,-4.87405664989205,
100.568979634104));
#50938=CARTESIAN_POINT('Ctrl Pts',(-6.11280331819254,-5.02546089097958,
100.576818462214));
#50939=CARTESIAN_POINT('Ctrl Pts',(-5.98585330647374,-5.17237674511219,
100.584657290325));
#50940=CARTESIAN_POINT('Ctrl Pts',(-5.85904560375187,-5.31912790884777,
100.59248733123));
#50941=CARTESIAN_POINT('Ctrl Pts',(-5.72667594144932,-5.4614004408611,100.600317372136));
#50942=CARTESIAN_POINT('Ctrl Pts',(-5.58909635740859,-5.59874297566891,
100.608147413041));
#50943=CARTESIAN_POINT('Ctrl Pts',(-5.4516442211758,-5.73595828226101,100.615970200534));
#50944=CARTESIAN_POINT('Ctrl Pts',(-5.30899202155895,-5.86825243977816,
100.623792988026));
#50945=CARTESIAN_POINT('Ctrl Pts',(-5.16153193549735,-5.99520717563964,
100.631615775518));
#50946=CARTESIAN_POINT('Ctrl Pts',(-5.01417976576146,-6.12206900169079,
100.639432838028));
#50947=CARTESIAN_POINT('Ctrl Pts',(-4.86202698290902,-6.24359896041867,
100.647249900537));
#50948=CARTESIAN_POINT('Ctrl Pts',(-4.70550261323149,-6.35941555151664,
100.655066963047));
#50949=CARTESIAN_POINT('Ctrl Pts',(-4.54906235703669,-6.47516990478636,
100.662879824802));
#50950=CARTESIAN_POINT('Ctrl Pts',(-4.38825547572164,-6.58521679778036,
100.670692686558));
#50951=CARTESIAN_POINT('Ctrl Pts',(-4.22354421412487,-6.68921484715003,
100.678505548314));
#50952=CARTESIAN_POINT('Ctrl Pts',(-4.058889445049,-6.79317722736192,100.686315730421));
#50953=CARTESIAN_POINT('Ctrl Pts',(-3.89033326087425,-6.89109470995801,
100.694125912528));
#50954=CARTESIAN_POINT('Ctrl Pts',(-3.71836718741699,-6.98266900687271,
100.701936094636));
#50955=CARTESIAN_POINT('Ctrl Pts',(-3.54639335817967,-7.07424743384685,
100.709746628987));
#50956=CARTESIAN_POINT('Ctrl Pts',(-3.37100963855793,-7.15948193008002,
100.717557163339));
#50957=CARTESIAN_POINT('Ctrl Pts',(-3.19273293070338,-7.23811974432602,
100.72536769769));
#50958=CARTESIAN_POINT('Ctrl Pts',(-3.01444193380339,-7.31676386146663,
100.733178858063));
#50959=CARTESIAN_POINT('Ctrl Pts',(-2.83325780852366,-7.38881010053658,
100.740990018436));
#50960=CARTESIAN_POINT('Ctrl Pts',(-2.64971816473443,-7.45405357154592,
100.74880117881));
#50961=CARTESIAN_POINT('Ctrl Pts',(-2.46613148511572,-7.51931376254399,
100.756614340954));
#50962=CARTESIAN_POINT('Ctrl Pts',(-2.28018841600672,-7.57776759459709,
100.764427503099));
#50963=CARTESIAN_POINT('Ctrl Pts',(-2.0924426186994,-7.62925978633907,100.772240665243));
#50964=CARTESIAN_POINT('Ctrl Pts',(-1.90461563898359,-7.6807742436135,100.780057205846));
#50965=CARTESIAN_POINT('Ctrl Pts',(-1.714984717257,-7.7253209710461,100.787873746449));
#50966=CARTESIAN_POINT('Ctrl Pts',(-1.5241147617666,-7.76279557846045,100.795690287051));
#50967=CARTESIAN_POINT('Ctrl Pts',(-1.33302205756247,-7.80031391942405,
100.803515949699));
#50968=CARTESIAN_POINT('Ctrl Pts',(-1.14068777687912,-7.83074358833103,
100.811341612347));
#50969=CARTESIAN_POINT('Ctrl Pts',(-0.94768412697614,-7.85403181782946,
100.819167274995));
#50970=CARTESIAN_POINT('Ctrl Pts',(-0.754554671097795,-7.87733522734353,
100.826998038661));
#50971=CARTESIAN_POINT('Ctrl Pts',(-0.560755325868441,-7.893487891755,100.834828802327));
#50972=CARTESIAN_POINT('Ctrl Pts',(-0.366859452539099,-7.90248917380358,
100.842659565993));
#50973=CARTESIAN_POINT('Ctrl Pts',(-0.172683420055691,-7.91150346175847,
100.85050164429));
#50974=CARTESIAN_POINT('Ctrl Pts',(0.0215890686840955,-7.91334572567888,
100.858343722586));
#50975=CARTESIAN_POINT('Ctrl Pts',(0.215387419524853,-7.90806735299532,
100.866185800883));
#50976=CARTESIAN_POINT('Ctrl Pts',(0.324011466864043,-7.90510882315353,
100.870581288669));
#50977=CARTESIAN_POINT('Ctrl Pts',(0.432486683125326,-7.89991420106491,
100.874976776455));
#50978=CARTESIAN_POINT('Ctrl Pts',(0.540713937046143,-7.89249956846905,
100.879372264241));
#50979=CARTESIAN_POINT('Ctrl Pts',(0.735637389148293,-7.87914539260949,
100.88728878824));
#50980=CARTESIAN_POINT('Ctrl Pts',(0.930340983616197,-7.85854695445958,
100.895205312238));
#50981=CARTESIAN_POINT('Ctrl Pts',(1.12424456805213,-7.83070847057948,100.903121836237));
#50982=CARTESIAN_POINT('Ctrl Pts',(1.31792476374908,-7.80290205832833,100.911029239917));
#50983=CARTESIAN_POINT('Ctrl Pts',(1.51080644751213,-7.76787226248475,100.918936643598));
#50984=CARTESIAN_POINT('Ctrl Pts',(1.7023110689238,-7.72567524716251,100.926844047279));
#50985=CARTESIAN_POINT('Ctrl Pts',(1.89363055212579,-7.68351902605094,100.934743806431));
#50986=CARTESIAN_POINT('Ctrl Pts',(2.08357529084069,-7.63420946189932,100.942643565583));
#50987=CARTESIAN_POINT('Ctrl Pts',(2.27157316497154,-7.57785433722378,100.950543324735));
#50988=CARTESIAN_POINT('Ctrl Pts',(2.45942411575497,-7.5215432549801,100.958436910099));
#50989=CARTESIAN_POINT('Ctrl Pts',(2.64533090474981,-7.45819768074241,100.966330495463));
#50990=CARTESIAN_POINT('Ctrl Pts',(2.82873261822868,-7.3879762299678,100.974224080826));
#50991=CARTESIAN_POINT('Ctrl Pts',(3.01202496498791,-7.31779665388221,100.982112959061));
#50992=CARTESIAN_POINT('Ctrl Pts',(3.19281489196223,-7.24074949421967,100.990001837296));
#50993=CARTESIAN_POINT('Ctrl Pts',(3.37055737228734,-7.15704296480882,100.997890715531));
#50994=CARTESIAN_POINT('Ctrl Pts',(3.54822677111899,-7.07337085259622,101.005776350135));
#50995=CARTESIAN_POINT('Ctrl Pts',(3.72285090922833,-6.98304497413313,101.013661984738));
#50996=CARTESIAN_POINT('Ctrl Pts',(3.89390518922201,-6.88632146921344,101.021547619342));
#50997=CARTESIAN_POINT('Ctrl Pts',(4.06494425281458,-6.78960656848446,101.029432552467));
#50998=CARTESIAN_POINT('Ctrl Pts',(4.23241378798273,-6.68649533906992,101.037317485592));
#50999=CARTESIAN_POINT('Ctrl Pts',(4.39581378675215,-6.57728987898509,101.045202418717));
#51000=CARTESIAN_POINT('Ctrl Pts',(4.55921321900226,-6.46808479752328,101.053087324504));
#51001=CARTESIAN_POINT('Ctrl Pts',(4.71854285604712,-6.35278571856391,101.060972230292));
#51002=CARTESIAN_POINT('Ctrl Pts',(4.87333159259317,-6.23173813543487,101.068857136079));
#51003=CARTESIAN_POINT('Ctrl Pts',(5.02814576234542,-6.11067066307997,101.076743337428));
#51004=CARTESIAN_POINT('Ctrl Pts',(5.17841727340561,-5.98385301687583,101.084629538778));
#51005=CARTESIAN_POINT('Ctrl Pts',(5.3237078468869,-5.85167119385521,101.092515740127));
#51006=CARTESIAN_POINT('Ctrl Pts',(5.46904666934658,-5.71944547508988,101.100404560374));
#51007=CARTESIAN_POINT('Ctrl Pts',(5.6094010036736,-5.58185226199119,101.108293380622));
#51008=CARTESIAN_POINT('Ctrl Pts',(5.74436902526336,-5.4393148007442,101.116182200869));
#51009=CARTESIAN_POINT('Ctrl Pts',(5.87946768344214,-5.29663937638916,101.124078656766));
#51010=CARTESIAN_POINT('Ctrl Pts',(6.00916937827817,-5.14901039541447,101.131975112663));
#51011=CARTESIAN_POINT('Ctrl Pts',(6.13311153906114,-4.99688541487946,101.13987156856));
#51012=CARTESIAN_POINT('Ctrl Pts',(6.25712220280107,-4.84467635471466,101.147772388837));
#51013=CARTESIAN_POINT('Ctrl Pts',(6.37536677842443,-4.68796661503222,101.155673209113));
#51014=CARTESIAN_POINT('Ctrl Pts',(6.48752557431558,-4.52724341322635,101.163574029389));
#51015=CARTESIAN_POINT('Ctrl Pts',(6.599820658331,-4.36632491096699,101.171484450232));
#51016=CARTESIAN_POINT('Ctrl Pts',(6.70601500494907,-4.20138349406655,101.179394871075));
#51017=CARTESIAN_POINT('Ctrl Pts',(6.80583392484042,-4.03293262868241,101.187305291918));
#51018=CARTESIAN_POINT('Ctrl Pts',(6.8491513933011,-3.95983160678803,101.190738102108));
#51019=CARTESIAN_POINT('Ctrl Pts',(6.89126883213213,-3.88606996347512,101.194170912298));
#51020=CARTESIAN_POINT('Ctrl Pts',(6.93216659895858,-3.81169086420752,101.197603722488));
#51021=CARTESIAN_POINT('Ctrl Pts',(7.03122517263022,-3.63153707938851,101.205918339825));
#51022=CARTESIAN_POINT('Ctrl Pts',(7.12334236935668,-3.44736477383205,101.214232957163));
#51023=CARTESIAN_POINT('Ctrl Pts',(7.2081979740973,-3.25972436966987,101.2225475745));
#51024=CARTESIAN_POINT('Ctrl Pts',(7.29294870156444,-3.07231587964045,101.230851915388));
#51025=CARTESIAN_POINT('Ctrl Pts',(7.37045561683469,-2.88144810591812,101.239156256275));
#51026=CARTESIAN_POINT('Ctrl Pts',(7.4404442012699,-2.68769624172621,101.247460597162));
#51027=CARTESIAN_POINT('Ctrl Pts',(7.5103509097929,-2.49417103750678,101.255755223244));
#51028=CARTESIAN_POINT('Ctrl Pts',(7.57275673067613,-2.29776874706939,101.264049849326));
#51029=CARTESIAN_POINT('Ctrl Pts',(7.62743476114083,-2.09908550672442,101.272344475407));
#51030=CARTESIAN_POINT('Ctrl Pts',(7.68203046317551,-1.90070142271537,101.280626612313));
#51031=CARTESIAN_POINT('Ctrl Pts',(7.72892151793529,-1.70004352459353,101.288908749219));
#51032=CARTESIAN_POINT('Ctrl Pts',(7.76793043876415,-1.49772417304435,101.297190886125));
#51033=CARTESIAN_POINT('Ctrl Pts',(7.8069033857533,-1.29559139943092,101.305465385283));
#51034=CARTESIAN_POINT('Ctrl Pts',(7.83800863871172,-1.09180051476274,101.313739884442));
#51035=CARTESIAN_POINT('Ctrl Pts',(7.86111906100353,-0.886976949377467,
101.322014383601));
#51036=CARTESIAN_POINT('Ctrl Pts',(7.88420290265242,-0.682388963506358,
101.330279365776));
#51037=CARTESIAN_POINT('Ctrl Pts',(7.89931022953192,-0.476770957721406,
101.338544347952));
#51038=CARTESIAN_POINT('Ctrl Pts',(7.90636527173355,-0.27075669876413,101.346809330127));
#51039=CARTESIAN_POINT('Ctrl Pts',(7.90918505298297,-0.188416277839943,
101.350112703955));
#51040=CARTESIAN_POINT('Ctrl Pts',(7.91071908446983,-0.106012650500569,
101.353416077783));
#51041=CARTESIAN_POINT('Ctrl Pts',(7.91096483829011,-0.0235865923251115,
101.356719451611));
#51042=CARTESIAN_POINT('Ctrl Pts',(7.91157979232759,0.18266955949944,101.364985541109));
#51043=CARTESIAN_POINT('Ctrl Pts',(7.90412375114978,0.388832937379216,101.373251630607));
#51044=CARTESIAN_POINT('Ctrl Pts',(7.88864808877916,0.594266212568875,101.381517720104));
#51045=CARTESIAN_POINT('Ctrl Pts',(7.87315850912396,0.799884234187099,101.389791243308));
#51046=CARTESIAN_POINT('Ctrl Pts',(7.84963493235122,1.00477054946824,101.398064766511));
#51047=CARTESIAN_POINT('Ctrl Pts',(7.81818042396406,1.20829460743029,101.406338289714));
#51048=CARTESIAN_POINT('Ctrl Pts',(7.78669558257738,1.41201493281061,101.414619791449));
#51049=CARTESIAN_POINT('Ctrl Pts',(7.74726458536066,1.61437008822508,101.422901293183));
#51050=CARTESIAN_POINT('Ctrl Pts',(7.7000414184488,1.81474051979148,101.431182794918));
#51051=CARTESIAN_POINT('Ctrl Pts',(7.6527396259826,2.01544456380459,101.439478085174));
#51052=CARTESIAN_POINT('Ctrl Pts',(7.59761979330777,2.21415699101003,101.44777337543));
#51053=CARTESIAN_POINT('Ctrl Pts',(7.53488611335355,2.41027223748517,101.456068665686));
#51054=CARTESIAN_POINT('Ctrl Pts',(7.47209553986051,2.60656534201677,101.46437147899));
#51055=CARTESIAN_POINT('Ctrl Pts',(7.40167743164466,2.80025628697147,101.472674292293));
#51056=CARTESIAN_POINT('Ctrl Pts',(7.32388430308222,2.99075905332841,101.480977105596));
#51057=CARTESIAN_POINT('Ctrl Pts',(7.24597187725304,3.18155395936084,101.489292651424));
#51058=CARTESIAN_POINT('Ctrl Pts',(7.16066194149775,3.36915064474596,101.497608197252));
#51059=CARTESIAN_POINT('Ctrl Pts',(7.06825399608287,3.55298556806223,101.50592374308));
#51060=CARTESIAN_POINT('Ctrl Pts',(7.03153980602914,3.62602420432716,101.509227555631));
#51061=CARTESIAN_POINT('Ctrl Pts',(6.99370567780142,3.69846933964838,101.512531368183));
#51062=CARTESIAN_POINT('Ctrl Pts',(6.95477231411373,3.77028686691572,101.515835180734));
#51063=CARTESIAN_POINT('Ctrl Pts',(6.86156141221415,3.94222619747257,101.523744883839));
#51064=CARTESIAN_POINT('Ctrl Pts',(6.76185245423408,4.11092474515443,101.531654586944));
#51065=CARTESIAN_POINT('Ctrl Pts',(6.65589624332205,4.27585853345635,101.539564290049));
#51066=CARTESIAN_POINT('Ctrl Pts',(6.55004753015076,4.44062498839043,101.547465968374));
#51067=CARTESIAN_POINT('Ctrl Pts',(6.43796437391843,4.60163400460239,101.5553676467));
#51068=CARTESIAN_POINT('Ctrl Pts',(6.31994388496384,4.75838526087455,101.563269325025));
#51069=CARTESIAN_POINT('Ctrl Pts',(6.20202126999436,4.91500652386962,101.571164450516));
#51070=CARTESIAN_POINT('Ctrl Pts',(6.07817133745655,5.06737678737977,101.579059576007));
#51071=CARTESIAN_POINT('Ctrl Pts',(5.94873514026518,5.21502360790191,101.586954701498));
#51072=CARTESIAN_POINT('Ctrl Pts',(5.81938231227119,5.36257532985664,101.594844741778));
#51073=CARTESIAN_POINT('Ctrl Pts',(5.68445061487505,5.50540941223202,101.602734782059));
#51074=CARTESIAN_POINT('Ctrl Pts',(5.54432228911601,5.64308526910691,101.610624822339));
#51075=CARTESIAN_POINT('Ctrl Pts',(5.40425827243544,5.78069794241462,101.618511241644));
#51076=CARTESIAN_POINT('Ctrl Pts',(5.25900262512153,5.9131568664827,101.62639766095));
#51077=CARTESIAN_POINT('Ctrl Pts',(5.1089756570331,6.04005701428747,101.634284080255));
#51078=CARTESIAN_POINT('Ctrl Pts',(4.95898976509124,6.16692241787832,101.642168340323));
#51079=CARTESIAN_POINT('Ctrl Pts',(4.80423541898661,6.28823185636755,101.650052600392));
#51080=CARTESIAN_POINT('Ctrl Pts',(4.64516754150017,6.40361925096998,101.657936860461));
#51081=CARTESIAN_POINT('Ctrl Pts',(4.48608109292573,6.51902011698783,101.665822041012));
#51082=CARTESIAN_POINT('Ctrl Pts',(4.32268038165523,6.62849734967503,101.673707221564));
#51083=CARTESIAN_POINT('Ctrl Pts',(4.15545148456132,6.73172666999018,101.681592402116));
#51084=CARTESIAN_POINT('Ctrl Pts',(3.98820172908867,6.83496886604808,101.689478566182));
#51085=CARTESIAN_POINT('Ctrl Pts',(3.81712312939198,6.93196141514126,101.697364730249));
#51086=CARTESIAN_POINT('Ctrl Pts',(3.64272864653235,7.02242472424822,101.705250894315));
#51087=CARTESIAN_POINT('Ctrl Pts',(3.46828315116926,7.11291449497134,101.71313936518));
#51088=CARTESIAN_POINT('Ctrl Pts',(3.29052014573448,7.19687106100321,101.721027836045));
#51089=CARTESIAN_POINT('Ctrl Pts',(3.10997517984555,7.2740618213447,101.72891630691));
#51090=CARTESIAN_POINT('Ctrl Pts',(2.92934710937687,7.35128811247858,101.736808408827));
#51091=CARTESIAN_POINT('Ctrl Pts',(2.74593484329511,7.42174225660399,101.744700510744));
#51092=CARTESIAN_POINT('Ctrl Pts',(2.5602920231717,7.48524052760387,101.75259261266));
#51093=CARTESIAN_POINT('Ctrl Pts',(2.37443398701087,7.54881241225742,101.760493863904));
#51094=CARTESIAN_POINT('Ctrl Pts',(2.18634055780104,7.60541220488174,101.768395115148));
#51095=CARTESIAN_POINT('Ctrl Pts',(1.99657971976665,7.65490629744196,101.776296366391));
#51096=CARTESIAN_POINT('Ctrl Pts',(1.80669314065104,7.70443318623546,101.784202853235));
#51097=CARTESIAN_POINT('Ctrl Pts',(1.61513728549257,7.7468449141241,101.792109340079));
#51098=CARTESIAN_POINT('Ctrl Pts',(1.42248858888792,7.78205931707563,101.800015826923));
#51099=CARTESIAN_POINT('Ctrl Pts',(1.22957448673385,7.81732223371103,101.807933206265));
#51100=CARTESIAN_POINT('Ctrl Pts',(1.0355648757293,7.84536797080917,101.815850585606));
#51101=CARTESIAN_POINT('Ctrl Pts',(0.841040736337092,7.86616625045654,101.823767964948));
#51102=CARTESIAN_POINT('Ctrl Pts',(0.756697141615612,7.87518416296326,101.827200856293));
#51103=CARTESIAN_POINT('Ctrl Pts',(0.67225681227205,7.88284021999969,101.830633747637));
#51104=CARTESIAN_POINT('Ctrl Pts',(0.587766981559898,7.88913499538371,101.834066638982));
#51105=CARTESIAN_POINT('Ctrl Pts',(0.394769987910758,7.90351391784779,101.841908265642));
#51106=CARTESIAN_POINT('Ctrl Pts',(0.200941043716103,7.91082909852056,101.849749892303));
#51107=CARTESIAN_POINT('Ctrl Pts',(0.00684493132486958,7.91099703873761,
101.857591518963));
#51108=CARTESIAN_POINT('Ctrl Pts',(-0.187022647517414,7.9111647812177,101.865423912699));
#51109=CARTESIAN_POINT('Ctrl Pts',(-0.381156420501285,7.90420203919917,
101.873256306434));
#51110=CARTESIAN_POINT('Ctrl Pts',(-0.574985141527442,7.89007687459525,
101.88108870017));
#51111=CARTESIAN_POINT('Ctrl Pts',(-0.768623376083116,7.8759655915912,101.888913396569));
#51112=CARTESIAN_POINT('Ctrl Pts',(-0.961956807702577,7.85470592869529,
101.896738092967));
#51113=CARTESIAN_POINT('Ctrl Pts',(-1.15441264185323,7.82631793708443,101.904562789365));
#51114=CARTESIAN_POINT('Ctrl Pts',(-1.34671678119287,7.79795232105413,101.912381318293));
#51115=CARTESIAN_POINT('Ctrl Pts',(-1.53814435460433,7.76246961773916,101.92019984722));
#51116=CARTESIAN_POINT('Ctrl Pts',(-1.72812595435393,7.71994181881498,101.928018376147));
#51117=CARTESIAN_POINT('Ctrl Pts',(-1.91799475532786,7.6774392701448,101.935832262938));
#51118=CARTESIAN_POINT('Ctrl Pts',(-2.10641895060174,7.62790003471959,101.943646149728));
#51119=CARTESIAN_POINT('Ctrl Pts',(-2.2928374276349,7.57144751883262,101.951460036519));
#51120=CARTESIAN_POINT('Ctrl Pts',(-2.47918146423998,7.51501754550427,101.959270803077));
#51121=CARTESIAN_POINT('Ctrl Pts',(-2.6635210421948,7.45167989363244,101.967081569635));
#51122=CARTESIAN_POINT('Ctrl Pts',(-2.84530817926851,7.38160838604892,101.974892336192));
#51123=CARTESIAN_POINT('Ctrl Pts',(-3.02708809118582,7.31153966346773,101.98270279231));
#51124=CARTESIAN_POINT('Ctrl Pts',(-3.20631543293658,7.23473773639045,101.990513248428));
#51125=CARTESIAN_POINT('Ctrl Pts',(-3.38245980761755,7.15142549774882,101.998323704546));
#51126=CARTESIAN_POINT('Ctrl Pts',(-3.55860904001995,7.06811096151665,102.006134376061));
#51127=CARTESIAN_POINT('Ctrl Pts',(-3.73167481745588,6.9782859058432,102.013945047576));
#51128=CARTESIAN_POINT('Ctrl Pts',(-3.90114910004849,6.88222033207241,102.021755719091));
#51129=CARTESIAN_POINT('Ctrl Pts',(-4.07065790324607,6.78613519048477,102.029567981579));
#51130=CARTESIAN_POINT('Ctrl Pts',(-4.23657344812533,6.68380717213187,102.037380244068));
#51131=CARTESIAN_POINT('Ctrl Pts',(-4.39841443514638,6.57555103825496,102.045192506556));
#51132=CARTESIAN_POINT('Ctrl Pts',(-4.56031689252224,6.46725378659275,102.053007736294));
#51133=CARTESIAN_POINT('Ctrl Pts',(-4.71814141707677,6.35302412981759,102.060822966032));
#51134=CARTESIAN_POINT('Ctrl Pts',(-4.87143758129479,6.23321882269095,102.06863819577));
#51135=CARTESIAN_POINT('Ctrl Pts',(-5.02490046253155,6.11328322147813,102.076461924949));
#51136=CARTESIAN_POINT('Ctrl Pts',(-5.17382486982215,5.98776007550052,102.084285654129));
#51137=CARTESIAN_POINT('Ctrl Pts',(-5.31779443444756,5.85704561643142,102.092109383308));
#51138=CARTESIAN_POINT('Ctrl Pts',(-5.46185134880608,5.72625184981463,102.099937859329));
#51139=CARTESIAN_POINT('Ctrl Pts',(-5.60094717857692,5.59026073830054,102.10776633535));
#51140=CARTESIAN_POINT('Ctrl Pts',(-5.73470400011519,5.44950374172391,102.11559481137));
#51141=CARTESIAN_POINT('Ctrl Pts',(-5.86864490852806,5.30855302406986,102.123434061568));
#51142=CARTESIAN_POINT('Ctrl Pts',(-5.997231900249,5.16282358326201,102.131273311766));
#51143=CARTESIAN_POINT('Ctrl Pts',(-6.12012802892761,5.0127790605147,102.139112561964));
#51144=CARTESIAN_POINT('Ctrl Pts',(-6.18903135503916,4.9286546312648,102.143507740385));
#51145=CARTESIAN_POINT('Ctrl Pts',(-6.2561465794987,4.84317430749099,102.147902918807));
#51146=CARTESIAN_POINT('Ctrl Pts',(-6.3214204938421,4.75642343994236,102.152298097228));
#51147=CARTESIAN_POINT('Ctrl Pts',(-6.43967391169762,4.5992613225368,102.160260617565));
#51148=CARTESIAN_POINT('Ctrl Pts',(-6.55222125606194,4.43747613818277,102.168223137902));
#51149=CARTESIAN_POINT('Ctrl Pts',(-6.65868367227015,4.27151644649098,102.176185658238));
#51150=CARTESIAN_POINT('Ctrl Pts',(-6.76497769988389,4.10581924855255,102.184135584482));
#51151=CARTESIAN_POINT('Ctrl Pts',(-6.86520580707316,3.93596099116097,102.192085510725));
#51152=CARTESIAN_POINT('Ctrl Pts',(-6.95903009909599,3.76242223572476,102.200035436969));
#51153=CARTESIAN_POINT('Ctrl Pts',(-7.05276659930876,3.58904586127887,102.207977924431));
#51154=CARTESIAN_POINT('Ctrl Pts',(-7.14011106066552,3.41199614529247,102.215920411892));
#51155=CARTESIAN_POINT('Ctrl Pts',(-7.22076887284424,3.23178246250637,102.223862899354));
#51156=CARTESIAN_POINT('Ctrl Pts',(-7.30136417999953,3.05170843464222,102.231799231859));
#51157=CARTESIAN_POINT('Ctrl Pts',(-7.37528302387227,2.86847563305343,102.239735564364));
#51158=CARTESIAN_POINT('Ctrl Pts',(-7.44227658919542,2.68261815581602,102.247671896869));
#51159=CARTESIAN_POINT('Ctrl Pts',(-7.50922900592288,2.49687483542564,102.255603354742));
#51160=CARTESIAN_POINT('Ctrl Pts',(-7.5692645055819,2.30851037000006,102.263534812616));
#51161=CARTESIAN_POINT('Ctrl Pts',(-7.62218218110039,2.1180792709707,102.271466270489));
#51162=CARTESIAN_POINT('Ctrl Pts',(-7.67507592790131,1.9277342825261,102.279394141856));
#51163=CARTESIAN_POINT('Ctrl Pts',(-7.72085817505793,1.73532484938847,102.287322013222));
#51164=CARTESIAN_POINT('Ctrl Pts',(-7.7593776195998,1.54142140780961,102.295249884589));
#51165=CARTESIAN_POINT('Ctrl Pts',(-7.79788659221713,1.34757068096308,102.303175600678));
#51166=CARTESIAN_POINT('Ctrl Pts',(-7.82913663230724,1.15222708782594,102.311101316768));
#51167=CARTESIAN_POINT('Ctrl Pts',(-7.85302730058534,0.955972393043547,
102.319027032857));
#51168=CARTESIAN_POINT('Ctrl Pts',(-7.87691833251812,0.759714710946676,
102.326952869589));
#51169=CARTESIAN_POINT('Ctrl Pts',(-7.89344972305619,0.562546235659305,
102.334878706321));
#51170=CARTESIAN_POINT('Ctrl Pts',(-7.90257271029148,0.365055555438395,
102.342804543052));
#51171=CARTESIAN_POINT('Ctrl Pts',(-7.90827573021412,0.241598922781995,
102.347759192623));
#51172=CARTESIAN_POINT('Ctrl Pts',(-7.91108470261973,0.11801649464083,102.352713842193));
#51173=CARTESIAN_POINT('Ctrl Pts',(-7.91099805494791,-0.00554748685628613,
102.357668491763));
#51174=CARTESIAN_POINT('',(-7.91810557688692,-0.00176888807660425,104.357636950005));
#51175=CARTESIAN_POINT('Ctrl Pts',(-7.90203417854292,-0.00560074141040939,
102.35767088191));
#51176=CARTESIAN_POINT('Ctrl Pts',(-7.90771100978507,-0.942735975233794,
102.395290439766));
#51177=CARTESIAN_POINT('Ctrl Pts',(-7.317879724775,-4.51501751106402,102.538987150367));
#51178=CARTESIAN_POINT('Ctrl Pts',(-2.01450770818587,-9.14056363453498,
102.788761013724));
#51179=CARTESIAN_POINT('Ctrl Pts',(6.61006158010275,-6.62790280679132,103.106992471968));
#51180=CARTESIAN_POINT('Ctrl Pts',(8.71221666557344,0.533409104126239,103.372185353842));
#51181=CARTESIAN_POINT('Ctrl Pts',(6.22559096011058,5.37393958538891,103.584339659338));
#51182=CARTESIAN_POINT('Ctrl Pts',(1.80015232899122,8.54088380044195,103.796493964838));
#51183=CARTESIAN_POINT('Ctrl Pts',(-5.38372996403238,7.53625788284238,104.054236257431));
#51184=CARTESIAN_POINT('Ctrl Pts',(-7.90872346788403,2.44045610435053,104.258939973652));
#51185=CARTESIAN_POINT('Ctrl Pts',(-7.92290895871525,-0.0017445537039696,
104.357566537123));
#51186=CARTESIAN_POINT('',(-7.911,-3.28903571045203E-12,106.357668491763));
#51187=CARTESIAN_POINT('Ctrl Pts',(-7.91099978297005,-0.00180488667992536,
104.357741113999));
#51188=CARTESIAN_POINT('Ctrl Pts',(-7.91047045206602,-2.20286967811119,
104.44630434232));
#51189=CARTESIAN_POINT('Ctrl Pts',(-6.94169981391732,-4.38650802119732,
104.534867570641));
#51190=CARTESIAN_POINT('Ctrl Pts',(-3.6782020148806,-7.34180684107737,104.712018234694));
#51191=CARTESIAN_POINT('Ctrl Pts',(-1.40868175871529,-8.08992666571367,
104.800605670427));
#51192=CARTESIAN_POINT('Ctrl Pts',(2.97309270521425,-7.65454228025191,104.977780541892));
#51193=CARTESIAN_POINT('Ctrl Pts',(5.05102072675703,-6.47444880834138,105.066367977625));
#51194=CARTESIAN_POINT('Ctrl Pts',(7.66951518847893,-2.93425195367629,105.24354284909));
#51195=CARTESIAN_POINT('Ctrl Pts',(8.18956872247068,-0.601881960098685,
105.332130284823));
#51196=CARTESIAN_POINT('Ctrl Pts',(7.32306689761338,3.71537198232442,105.509305156288));
#51197=CARTESIAN_POINT('Ctrl Pts',(5.94329958850222,5.66643518936479,105.597892592021));
#51198=CARTESIAN_POINT('Ctrl Pts',(2.16154501637932,7.92205913232967,105.775067463487));
#51199=CARTESIAN_POINT('Ctrl Pts',(-0.210816529299153,8.20894963712998,
105.863654899219));
#51200=CARTESIAN_POINT('Ctrl Pts',(-4.42123908576287,6.91982244717918,106.040829770685));
#51201=CARTESIAN_POINT('Ctrl Pts',(-6.22631625634048,5.35390358803672,106.129417206417));
#51202=CARTESIAN_POINT('Ctrl Pts',(-7.65317280859501,2.31334857514568,106.264559258688));
#51203=CARTESIAN_POINT('Ctrl Pts',(-7.91100000000048,1.15702837836374,106.311113875226));
#51204=CARTESIAN_POINT('Ctrl Pts',(-7.911,-3.28903571045203E-12,106.357668491763));
#51205=CARTESIAN_POINT('',(-7.91099991715881,-0.000809541038039417,108.357668491763));
#51206=CARTESIAN_POINT('Ctrl Pts',(-7.911,-3.28903571045203E-12,106.357668491763));
#51207=CARTESIAN_POINT('Ctrl Pts',(-7.91099999999908,-2.20167589667009,
106.446255927496));
#51208=CARTESIAN_POINT('Ctrl Pts',(-6.94214576672186,-4.38610418338977,
106.534843363229));
#51209=CARTESIAN_POINT('Ctrl Pts',(-3.6782020148797,-7.34180684107791,106.712018234694));
#51210=CARTESIAN_POINT('Ctrl Pts',(-1.40868175871392,-8.08992666571399,
106.800605670427));
#51211=CARTESIAN_POINT('Ctrl Pts',(2.97309270521612,-7.65454228025126,106.977780541892));
#51212=CARTESIAN_POINT('Ctrl Pts',(5.05102072675892,-6.47444880834001,107.066367977625));
#51213=CARTESIAN_POINT('Ctrl Pts',(7.66951518848005,-2.9342519536736,107.24354284909));
#51214=CARTESIAN_POINT('Ctrl Pts',(8.18956872247099,-0.601881960095431,
107.332130284823));
#51215=CARTESIAN_POINT('Ctrl Pts',(7.32306689761171,3.71537198232789,107.509305156289));
#51216=CARTESIAN_POINT('Ctrl Pts',(5.94329958849938,5.66643518936789,107.597892592021));
#51217=CARTESIAN_POINT('Ctrl Pts',(2.16154501637473,7.92205913233101,107.775067463487));
#51218=CARTESIAN_POINT('Ctrl Pts',(-0.210816529304289,8.20894963712993,
107.86365489922));
#51219=CARTESIAN_POINT('Ctrl Pts',(-4.42123908576773,6.91982244717618,108.040829770685));
#51220=CARTESIAN_POINT('Ctrl Pts',(-6.2263162563445,5.35390358803217,108.129417206418));
#51221=CARTESIAN_POINT('Ctrl Pts',(-7.65317280859598,2.31334857514152,108.264559258688));
#51222=CARTESIAN_POINT('Ctrl Pts',(-7.91100000000052,1.15702837836152,108.311113875226));
#51223=CARTESIAN_POINT('Ctrl Pts',(-7.911,-3.56825680114525E-12,108.357668491763));
#51224=CARTESIAN_POINT('',(-7.91099996833566,-0.000689401199207026,110.357696230784));
#51225=CARTESIAN_POINT('Ctrl Pts',(-7.91099983431761,-0.00161908207251058,
108.357668491763));
#51226=CARTESIAN_POINT('Ctrl Pts',(-7.91095706826763,-0.210578356008037,
108.366032203258));
#51227=CARTESIAN_POINT('Ctrl Pts',(-7.90263095137406,-0.419335154028208,
108.374395914752));
#51228=CARTESIAN_POINT('Ctrl Pts',(-7.88609496611805,-0.627237742301582,
108.382759626247));
#51229=CARTESIAN_POINT('Ctrl Pts',(-7.86953193721219,-0.835480343263119,
108.391137016109));
#51230=CARTESIAN_POINT('Ctrl Pts',(-7.84473223822582,-1.04286566971612,
108.399514405971));
#51231=CARTESIAN_POINT('Ctrl Pts',(-7.81182074813354,-1.24875041502709,
108.407891795833));
#51232=CARTESIAN_POINT('Ctrl Pts',(-7.7788550691014,-1.45497415064365,108.416282979111));
#51233=CARTESIAN_POINT('Ctrl Pts',(-7.73775095957343,-1.65969209823175,
108.424674162389));
#51234=CARTESIAN_POINT('Ctrl Pts',(-7.68868381084718,-1.86227341086545,
108.433065345667));
#51235=CARTESIAN_POINT('Ctrl Pts',(-7.63949205421211,-2.06536918652358,
108.441477838677));
#51236=CARTESIAN_POINT('Ctrl Pts',(-7.58229687058085,-2.26631720498226,
108.449890331688));
#51237=CARTESIAN_POINT('Ctrl Pts',(-7.51732357991094,-2.46450140899026,
108.458302824698));
#51238=CARTESIAN_POINT('Ctrl Pts',(-7.45226006582057,-2.66296081618687,
108.466726999491));
#51239=CARTESIAN_POINT('Ctrl Pts',(-7.37939696543437,-2.85864848567774,
108.475151174285));
#51240=CARTESIAN_POINT('Ctrl Pts',(-7.29900733791689,-3.05096917077759,
108.483575349078));
#51241=CARTESIAN_POINT('Ctrl Pts',(-7.21844862570473,-3.24369436682402,
108.492017242564));
#51242=CARTESIAN_POINT('Ctrl Pts',(-7.13033184281655,-3.43303816640151,
108.500459136049));
#51243=CARTESIAN_POINT('Ctrl Pts',(-7.03497657739299,-3.61842860307233,
108.508901029534));
#51244=CARTESIAN_POINT('Ctrl Pts',(-7.00475651897568,-3.6771826718835,108.511576440411));
#51245=CARTESIAN_POINT('Ctrl Pts',(-6.97380976383304,-3.73553988732904,
108.514251851287));
#51246=CARTESIAN_POINT('Ctrl Pts',(-6.94214738164216,-3.79348266525088,
108.516927262164));
#51247=CARTESIAN_POINT('Ctrl Pts',(-6.84934497044179,-3.96331289060716,
108.524768888825));
#51248=CARTESIAN_POINT('Ctrl Pts',(-6.75016062405178,-4.13000313299525,
108.532610515485));
#51249=CARTESIAN_POINT('Ctrl Pts',(-6.64483114589177,-4.29303389720914,
108.540452142145));
#51250=CARTESIAN_POINT('Ctrl Pts',(-6.53962568525626,-4.4558727049817,108.548284535881));
#51251=CARTESIAN_POINT('Ctrl Pts',(-6.42828968841049,-4.61506032195092,
108.556116929617));
#51252=CARTESIAN_POINT('Ctrl Pts',(-6.31110675512517,-4.77009984438623,
108.563949323353));
#51253=CARTESIAN_POINT('Ctrl Pts',(-6.19403898415056,-4.92498700069487,
108.571774019751));
#51254=CARTESIAN_POINT('Ctrl Pts',(-6.07113592995873,-5.07573390221857,
108.57959871615));
#51255=CARTESIAN_POINT('Ctrl Pts',(-5.9427256775954,-5.2218705959501,108.587423412548));
#51256=CARTESIAN_POINT('Ctrl Pts',(-5.81441663894217,-5.36789210388703,
108.595241941475));
#51257=CARTESIAN_POINT('Ctrl Pts',(-5.68060927852424,-5.50931037850196,
108.603060470402));
#51258=CARTESIAN_POINT('Ctrl Pts',(-5.5416734439547,-5.64568653403351,108.61087899933));
#51259=CARTESIAN_POINT('Ctrl Pts',(-5.40282010049028,-5.78198171823165,
108.61869288612));
#51260=CARTESIAN_POINT('Ctrl Pts',(-5.2588445985855,-5.91324050103304,108.626506772911));
#51261=CARTESIAN_POINT('Ctrl Pts',(-5.11015543976854,-6.03905889865333,
108.634320659702));
#51262=CARTESIAN_POINT('Ctrl Pts',(-4.96152565534921,-6.16482705460416,
108.64213142626));
#51263=CARTESIAN_POINT('Ctrl Pts',(-4.80818623225492,-6.28515892681596,
108.649942192818));
#51264=CARTESIAN_POINT('Ctrl Pts',(-4.65058086069437,-6.39968895010869,
108.657752959375));
#51265=CARTESIAN_POINT('Ctrl Pts',(-4.49298175318107,-6.51421442138982,
108.665563415493));
#51266=CARTESIAN_POINT('Ctrl Pts',(-4.3311173141357,-6.6229382890854,108.673373871611));
#51267=CARTESIAN_POINT('Ctrl Pts',(-4.16546287131606,-6.72553641486591,
108.681184327729));
#51268=CARTESIAN_POINT('Ctrl Pts',(-3.99980386006779,-6.82813737010397,
108.688994999244));
#51269=CARTESIAN_POINT('Ctrl Pts',(-3.83035493565669,-6.92461206088938,
108.696805670759));
#51270=CARTESIAN_POINT('Ctrl Pts',(-3.65761882368748,-7.01468071551422,
108.704616342274));
#51271=CARTESIAN_POINT('Ctrl Pts',(-3.48484752670273,-7.10476771643026,
108.712428604763));
#51272=CARTESIAN_POINT('Ctrl Pts',(-3.30878802036883,-7.18844591910283,
108.720240867251));
#51273=CARTESIAN_POINT('Ctrl Pts',(-3.12996607474961,-7.26548232197399,
108.72805312974));
#51274=CARTESIAN_POINT('Ctrl Pts',(-2.9510762090793,-7.34254798476848,108.735868359478));
#51275=CARTESIAN_POINT('Ctrl Pts',(-2.76942213703738,-7.41296668362044,
108.743683589216));
#51276=CARTESIAN_POINT('Ctrl Pts',(-2.58554810570294,-7.47655415235494,
108.751498818953));
#51277=CARTESIAN_POINT('Ctrl Pts',(-2.40147410243307,-7.54021077554862,
108.759322548133));
#51278=CARTESIAN_POINT('Ctrl Pts',(-2.21517565043103,-7.59702121512676,
108.767146277312));
#51279=CARTESIAN_POINT('Ctrl Pts',(-2.02721162948329,-7.64685124801625,
108.774970006492));
#51280=CARTESIAN_POINT('Ctrl Pts',(-1.83913356632677,-7.69671151396303,
108.782798482513));
#51281=CARTESIAN_POINT('Ctrl Pts',(-1.64938826247017,-7.73958285562081,
108.790626958534));
#51282=CARTESIAN_POINT('Ctrl Pts',(-1.45854328020047,-7.77538246646312,
108.798455434554));
#51283=CARTESIAN_POINT('Ctrl Pts',(-1.267435641748,-7.81123134760332,108.806294684752));
#51284=CARTESIAN_POINT('Ctrl Pts',(-1.0752256487331,-7.83998900646917,108.81413393495));
#51285=CARTESIAN_POINT('Ctrl Pts',(-0.882485612244638,-7.86162452322554,
108.821973185148));
#51286=CARTESIAN_POINT('Ctrl Pts',(-0.774423383347515,-7.873754759406,108.826368363569));
#51287=CARTESIAN_POINT('Ctrl Pts',(-0.666194552038647,-7.88364713922093,
108.83076354199));
#51288=CARTESIAN_POINT('Ctrl Pts',(-0.557899681538563,-7.89130337430637,
108.835158720411));
#51289=CARTESIAN_POINT('Ctrl Pts',(-0.363004324027375,-7.90508209408578,
108.843068604469));
#51290=CARTESIAN_POINT('Ctrl Pts',(-0.167335115482649,-7.9116549857076,
108.850978488527));
#51291=CARTESIAN_POINT('Ctrl Pts',(0.0285325814148896,-7.91094854564216,
108.858888372584));
#51292=CARTESIAN_POINT('Ctrl Pts',(0.224187337279239,-7.91024287359554,
108.866789657272));
#51293=CARTESIAN_POINT('Ctrl Pts',(0.420039809847823,-7.90227363419173,
108.874690941959));
#51294=CARTESIAN_POINT('Ctrl Pts',(0.615509318319252,-7.88701903630657,
108.882592226646));
#51295=CARTESIAN_POINT('Ctrl Pts',(0.810802641600462,-7.87177818805556,
108.890486389561));
#51296=CARTESIAN_POINT('Ctrl Pts',(1.00571334666963,-7.8492650891588,108.898380552476));
#51297=CARTESIAN_POINT('Ctrl Pts',(1.19966026904507,-7.8195099743446,108.906274715391));
#51298=CARTESIAN_POINT('Ctrl Pts',(1.39346840735018,-7.78977615162361,108.91416322942));
#51299=CARTESIAN_POINT('Ctrl Pts',(1.58631379741495,-7.75281068976761,108.922051743449));
#51300=CARTESIAN_POINT('Ctrl Pts',(1.77761963412016,-7.70869570267179,108.929940257478));
#51301=CARTESIAN_POINT('Ctrl Pts',(1.9688241067963,-7.6646040900475,108.937824591752));
#51302=CARTESIAN_POINT('Ctrl Pts',(2.15849031622885,-7.61337057795531,108.945708926025));
#51303=CARTESIAN_POINT('Ctrl Pts',(2.34605062434113,-7.55512855403723,108.953593260299));
#51304=CARTESIAN_POINT('Ctrl Pts',(2.53354638182123,-7.49690657465576,108.961474881106));
#51305=CARTESIAN_POINT('Ctrl Pts',(2.7189373534025,-7.43168099287984,108.969356501912));
#51306=CARTESIAN_POINT('Ctrl Pts',(2.90166979678511,-7.35963541151497,108.977238122718));
#51307=CARTESIAN_POINT('Ctrl Pts',(3.08440463348052,-7.2875888865431,108.985119846753));
#51308=CARTESIAN_POINT('Ctrl Pts',(3.26448054836888,-7.20872230206148,108.993001570788));
#51309=CARTESIAN_POINT('Ctrl Pts',(3.44136202810132,-7.1232680976882,109.000883294823));
#51310=CARTESIAN_POINT('Ctrl Pts',(3.61825416320654,-7.03780874553796,109.008765493654));
#51311=CARTESIAN_POINT('Ctrl Pts',(3.79195116863494,-6.94576113234965,109.016647692486));
#51312=CARTESIAN_POINT('Ctrl Pts',(3.96194044342778,-6.84740453914703,109.024529891317));
#51313=CARTESIAN_POINT('Ctrl Pts',(4.13196856255395,-6.7490254704306,109.032413891314));
#51314=CARTESIAN_POINT('Ctrl Pts',(4.29828696405931,-6.64433472178238,109.04029789131));
#51315=CARTESIAN_POINT('Ctrl Pts',(4.46041023448753,-6.53365606227316,109.048181891307));
#51316=CARTESIAN_POINT('Ctrl Pts',(4.62259783267329,-6.42293348735345,109.05606901954));
#51317=CARTESIAN_POINT('Ctrl Pts',(4.78058669824597,-6.3062184617961,109.063956147774));
#51318=CARTESIAN_POINT('Ctrl Pts',(4.93392263410113,-6.18387648976794,109.071843276008));
#51319=CARTESIAN_POINT('Ctrl Pts',(5.08742216188307,-6.0614039928317,109.079738818906));
#51320=CARTESIAN_POINT('Ctrl Pts',(5.23625857463332,-5.93329277354653,109.087634361805));
#51321=CARTESIAN_POINT('Ctrl Pts',(5.38001201481399,-5.79994756187132,109.095529904703));
#51322=CARTESIAN_POINT('Ctrl Pts',(5.5238529958589,-5.6665211475824,109.103430255714));
#51323=CARTESIAN_POINT('Ctrl Pts',(5.66260458993656,-5.52785462983011,109.111330606724));
#51324=CARTESIAN_POINT('Ctrl Pts',(5.79588554515911,-5.38438777832872,109.119230957735));
#51325=CARTESIAN_POINT('Ctrl Pts',(5.92934003778859,-5.24073412695522,109.127141595335));
#51326=CARTESIAN_POINT('Ctrl Pts',(6.05730943919919,-5.09226791789037,109.135052232934));
#51327=CARTESIAN_POINT('Ctrl Pts',(6.17945362544743,-4.93946089071921,109.142962870534));
#51328=CARTESIAN_POINT('Ctrl Pts',(6.23312123649674,-4.87232066610667,109.146438639909));
#51329=CARTESIAN_POINT('Ctrl Pts',(6.28566483662988,-4.80434279559942,109.149914409283));
#51330=CARTESIAN_POINT('Ctrl Pts',(6.33705831246445,-4.73556891454715,109.153390178658));
#51331=CARTESIAN_POINT('Ctrl Pts',(6.45401528938204,-4.57905906406232,109.161300044101));
#51332=CARTESIAN_POINT('Ctrl Pts',(6.56532854390461,-4.41800259386137,109.169209909545));
#51333=CARTESIAN_POINT('Ctrl Pts',(6.67062519711001,-4.25284381087304,109.177119774988));
#51334=CARTESIAN_POINT('Ctrl Pts',(6.77580741471002,-4.08786452119945,109.18502104405));
#51335=CARTESIAN_POINT('Ctrl Pts',(6.87498587143819,-3.91879208730285,109.192922313111));
#51336=CARTESIAN_POINT('Ctrl Pts',(6.96782831829315,-3.74610324561298,109.200823582173));
#51337=CARTESIAN_POINT('Ctrl Pts',(7.06058711703034,-3.57356999112546,109.20871773244));
#51338=CARTESIAN_POINT('Ctrl Pts',(7.14702111541331,-3.3974271214705,109.216611882707));
#51339=CARTESIAN_POINT('Ctrl Pts',(7.2268415715172,-3.21817990488269,109.224506032975));
#51340=CARTESIAN_POINT('Ctrl Pts',(7.30660493982616,-3.03906088636392,109.232394537325));
#51341=CARTESIAN_POINT('Ctrl Pts',(7.37976404985226,-2.85684225819138,109.240283041676));
#51342=CARTESIAN_POINT('Ctrl Pts',(7.44607616145086,-2.67205366672774,109.248171546027));
#51343=CARTESIAN_POINT('Ctrl Pts',(7.51235316222157,-2.4873629168239,109.256055873585));
#51344=CARTESIAN_POINT('Ctrl Pts',(7.57179027224848,-2.30010523898282,109.263940201144));
#51345=CARTESIAN_POINT('Ctrl Pts',(7.62419284282803,-2.1108302857809,109.271824528702));
#51346=CARTESIAN_POINT('Ctrl Pts',(7.67657739821851,-1.92162040236524,109.279706145751));
#51347=CARTESIAN_POINT('Ctrl Pts',(7.7219321420792,-1.73039495782352,109.2875877628));
#51348=CARTESIAN_POINT('Ctrl Pts',(7.76011218289167,-1.53771906047116,109.29546937985));
#51349=CARTESIAN_POINT('Ctrl Pts',(7.79829274520056,-1.3450405313827,109.303351104553));
#51350=CARTESIAN_POINT('Ctrl Pts',(7.8292983332167,-1.15091184659485,109.311232829256));
#51351=CARTESIAN_POINT('Ctrl Pts',(7.85303499544822,-0.955909179925386,
109.319114553959));
#51352=CARTESIAN_POINT('Ctrl Pts',(7.87677309588481,-0.760894698038554,
109.326996756216));
#51353=CARTESIAN_POINT('Ctrl Pts',(7.89324135062022,-0.565006471327188,
109.334878958473));
#51354=CARTESIAN_POINT('Ctrl Pts',(7.90239760140287,-0.368826719940726,
109.34276116073));
#51355=CARTESIAN_POINT('Ctrl Pts',(7.91155594768836,-0.172602070785931,
109.350645166911));
#51356=CARTESIAN_POINT('Ctrl Pts',(7.91339893936832,0.0239138912713034,
109.358529173092));
#51357=CARTESIAN_POINT('Ctrl Pts',(7.90793654266766,0.220137768548511,109.366413179273));
#51358=CARTESIAN_POINT('Ctrl Pts',(7.90247197666961,0.416439572780986,109.374300316452));
#51359=CARTESIAN_POINT('Ctrl Pts',(7.88969625097962,0.612448716436179,109.382187453631));
#51360=CARTESIAN_POINT('Ctrl Pts',(7.86967131823589,0.807585501934868,109.390074590809));
#51361=CARTESIAN_POINT('Ctrl Pts',(7.84962501071162,1.002930578069,109.397970146784));
#51362=CARTESIAN_POINT('Ctrl Pts',(7.82231407557405,1.19740109275375,109.405865702759));
#51363=CARTESIAN_POINT('Ctrl Pts',(7.78785202926404,1.39042503224301,109.413761258735));
#51364=CARTESIAN_POINT('Ctrl Pts',(7.75336898642348,1.58356657452943,109.421661625198));
#51365=CARTESIAN_POINT('Ctrl Pts',(7.71172621937584,1.77525944825649,109.429561991662));
#51366=CARTESIAN_POINT('Ctrl Pts',(7.66308759286952,1.96494517582788,109.437462358126));
#51367=CARTESIAN_POINT('Ctrl Pts',(7.614385615226,2.15487796643159,109.445373014707));
#51368=CARTESIAN_POINT('Ctrl Pts',(7.55866967518494,2.34279805922108,109.453283671289));
#51369=CARTESIAN_POINT('Ctrl Pts',(7.49615276674389,2.52816429403588,109.46119432787));
#51370=CARTESIAN_POINT('Ctrl Pts',(7.46868420297819,2.60961016792806,109.464670097548));
#51371=CARTESIAN_POINT('Ctrl Pts',(7.4399033076061,2.69056329321023,109.468145867227));
#51372=CARTESIAN_POINT('Ctrl Pts',(7.40983099053721,2.77097919365599,109.471621636905));
#51373=CARTESIAN_POINT('Ctrl Pts',(7.34200954487035,2.9523394330529,109.479460465015));
#51374=CARTESIAN_POINT('Ctrl Pts',(7.26742327569606,3.13148215794732,109.487299293126));
#51375=CARTESIAN_POINT('Ctrl Pts',(7.18623567320809,3.30786001050701,109.495138121236));
#51376=CARTESIAN_POINT('Ctrl Pts',(7.10513908076501,3.48404014622587,109.502968162142));
#51377=CARTESIAN_POINT('Ctrl Pts',(7.01745603542431,3.6574612649623,109.510798203047));
#51378=CARTESIAN_POINT('Ctrl Pts',(6.92339947281602,3.82759202891464,109.518628243953));
#51379=CARTESIAN_POINT('Ctrl Pts',(6.82943004016098,3.99756519104635,109.526451031445));
#51380=CARTESIAN_POINT('Ctrl Pts',(6.7290990170093,4.1642537628276,109.534273818938));
#51381=CARTESIAN_POINT('Ctrl Pts',(6.6226670857949,4.32714705905969,109.54209660643));
#51382=CARTESIAN_POINT('Ctrl Pts',(6.51631304510166,4.48992114441593,109.54991366894));
#51383=CARTESIAN_POINT('Ctrl Pts',(6.40386718056499,4.64890519313521,109.557730731449));
#51384=CARTESIAN_POINT('Ctrl Pts',(6.28563578209234,4.80361362048203,109.565547793959));
#51385=CARTESIAN_POINT('Ctrl Pts',(6.167467919124,4.95823891020145,109.573360655714));
#51386=CARTESIAN_POINT('Ctrl Pts',(6.04352092852737,5.10859287675396,109.58117351747));
#51387=CARTESIAN_POINT('Ctrl Pts',(5.91414414780228,5.25421925684644,109.588986379226));
#51388=CARTESIAN_POINT('Ctrl Pts',(5.78481174060952,5.39979569013358,109.596796561333));
#51389=CARTESIAN_POINT('Ctrl Pts',(5.65005348715701,5.54064750498899,109.60460674344));
#51390=CARTESIAN_POINT('Ctrl Pts',(5.51025881626388,5.67635171371421,109.612416925548));
#51391=CARTESIAN_POINT('Ctrl Pts',(5.37045784054122,5.81206204278647,109.620227459899));
#51392=CARTESIAN_POINT('Ctrl Pts',(5.22562023953531,5.94262405024515,109.628037994251));
#51393=CARTESIAN_POINT('Ctrl Pts',(5.07617245976413,6.06765145329989,109.635848528602));
#51394=CARTESIAN_POINT('Ctrl Pts',(4.92671270161279,6.1926888774186,109.643659688975));
#51395=CARTESIAN_POINT('Ctrl Pts',(4.77264229809379,6.31219058693558,109.651470849348));
#51396=CARTESIAN_POINT('Ctrl Pts',(4.61442087334313,6.42581053281648,109.659282009722));
#51397=CARTESIAN_POINT('Ctrl Pts',(4.45615890108023,6.53945959615827,109.667095171866));
#51398=CARTESIAN_POINT('Ctrl Pts',(4.29374407420746,6.64722368778318,109.674908334011));
#51399=CARTESIAN_POINT('Ctrl Pts',(4.12766520607387,6.74879996344292,109.682721496155));
#51400=CARTESIAN_POINT('Ctrl Pts',(3.96151452444149,6.85042016129356,109.690538036758));
#51401=CARTESIAN_POINT('Ctrl Pts',(3.79169694533208,6.94584702976316,109.698354577361));
#51402=CARTESIAN_POINT('Ctrl Pts',(3.61872621155272,7.03482349500123,109.706171117964));
#51403=CARTESIAN_POINT('Ctrl Pts',(3.44555361777809,7.12390379739405,109.713996780612));
#51404=CARTESIAN_POINT('Ctrl Pts',(3.26922083265525,7.20651850048568,109.721822443259));
#51405=CARTESIAN_POINT('Ctrl Pts',(3.09026293866372,7.28245809942779,109.729648105907));
#51406=CARTESIAN_POINT('Ctrl Pts',(2.91118839417133,7.35844719823859,109.737478869574));
#51407=CARTESIAN_POINT('Ctrl Pts',(2.72948565840863,7.42775239714644,109.74530963324));
#51408=CARTESIAN_POINT('Ctrl Pts',(2.54570539070657,7.49021395313428,109.753140396906));
#51409=CARTESIAN_POINT('Ctrl Pts',(2.36165957983734,7.55276575950434,109.760982475202));
#51410=CARTESIAN_POINT('Ctrl Pts',(2.1755305771564,7.60845407227149,109.768824553498));
#51411=CARTESIAN_POINT('Ctrl Pts',(1.98788082254989,7.65716989724914,109.776666631795));
#51412=CARTESIAN_POINT('Ctrl Pts',(1.88270306568575,7.68447513516794,109.781062119581));
#51413=CARTESIAN_POINT('Ctrl Pts',(1.7770476874526,7.70959082129426,109.785457607366));
#51414=CARTESIAN_POINT('Ctrl Pts',(1.67101438797397,7.7325048926712,109.789853095152));
#51415=CARTESIAN_POINT('Ctrl Pts',(1.48004237283508,7.77377444108104,109.797769619151));
#51416=CARTESIAN_POINT('Ctrl Pts',(1.28727100405664,7.80802330576419,109.805686143149));
#51417=CARTESIAN_POINT('Ctrl Pts',(1.0932588124498,7.83509452202083,109.813602667147));
#51418=CARTESIAN_POINT('Ctrl Pts',(0.899470134704176,7.86213455058755,109.821510070828));
#51419=CARTESIAN_POINT('Ctrl Pts',(0.704443819299248,7.88201335405967,109.829417474509));
#51420=CARTESIAN_POINT('Ctrl Pts',(0.508751275535268,7.89462431909469,109.837324878189));
#51421=CARTESIAN_POINT('Ctrl Pts',(0.313247918679629,7.90722309240568,109.845224637341));
#51422=CARTESIAN_POINT('Ctrl Pts',(0.117079957929666,7.91256800186929,109.853124396493));
#51423=CARTESIAN_POINT('Ctrl Pts',(-0.0791730489321256,7.91060380933863,
109.861024155646));
#51424=CARTESIAN_POINT('Ctrl Pts',(-0.275272680928759,7.90864115185586,
109.868917741009));
#51425=CARTESIAN_POINT('Ctrl Pts',(-0.4714568836888,7.89938077620507,109.876811326373));
#51426=CARTESIAN_POINT('Ctrl Pts',(-0.667142757361975,7.88281939037674,
109.884704911737));
#51427=CARTESIAN_POINT('Ctrl Pts',(-0.862711938983061,7.86626788048917,
109.892593789972));
#51428=CARTESIAN_POINT('Ctrl Pts',(-1.05778304128565,7.84242406465922,109.900482668206));
#51429=CARTESIAN_POINT('Ctrl Pts',(-1.25177466161008,7.81133670997167,109.908371546441));
#51430=CARTESIAN_POINT('Ctrl Pts',(-1.44568651936325,7.78026213731737,109.916257181045));
#51431=CARTESIAN_POINT('Ctrl Pts',(-1.63851943999301,7.74195001584696,109.924142815649));
#51432=CARTESIAN_POINT('Ctrl Pts',(-1.82969834633736,7.69650082579157,109.932028450253));
#51433=CARTESIAN_POINT('Ctrl Pts',(-2.02086024606327,7.65105567873993,109.939913383378));
#51434=CARTESIAN_POINT('Ctrl Pts',(-2.21036808805915,7.59847480139269,109.947798316502));
#51435=CARTESIAN_POINT('Ctrl Pts',(-2.39765766330912,7.53890965124102,109.955683249627));
#51436=CARTESIAN_POINT('Ctrl Pts',(-2.58494658921295,7.47934470760593,109.963568155415));
#51437=CARTESIAN_POINT('Ctrl Pts',(-2.77001693501704,7.41279564334951,109.971453061202));
#51438=CARTESIAN_POINT('Ctrl Pts',(-2.95232021497289,7.33946362810406,109.979337966989));
#51439=CARTESIAN_POINT('Ctrl Pts',(-3.13465344902654,7.26611956373719,109.987224168339));
#51440=CARTESIAN_POINT('Ctrl Pts',(-3.31421839151424,7.18599045632738,109.995110369688));
#51441=CARTESIAN_POINT('Ctrl Pts',(-3.49048685207083,7.09932549863159,110.002996571037));
#51442=CARTESIAN_POINT('Ctrl Pts',(-3.666813848932,7.01263176070851,110.010885391285));
#51443=CARTESIAN_POINT('Ctrl Pts',(-3.8398418735395,6.91939799989301,110.018774211532));
#51444=CARTESIAN_POINT('Ctrl Pts',(-4.00906741953157,6.81991931225366,110.026663031779));
#51445=CARTESIAN_POINT('Ctrl Pts',(-4.17845676023396,6.72034433842579,110.034559487676));
#51446=CARTESIAN_POINT('Ctrl Pts',(-4.3440359736098,6.61451253902403,110.042455943574));
#51447=CARTESIAN_POINT('Ctrl Pts',(-4.5053297424175,6.50276286758853,110.050352399471));
#51448=CARTESIAN_POINT('Ctrl Pts',(-4.66671265845338,6.39095143199729,110.058253219747));
#51449=CARTESIAN_POINT('Ctrl Pts',(-4.82380513221666,6.27321580925561,110.066154040023));
#51450=CARTESIAN_POINT('Ctrl Pts',(-4.97616480907838,6.14993534867562,110.0740548603));
#51451=CARTESIAN_POINT('Ctrl Pts',(-5.12870962357899,6.02650508564224,110.081965281142));
#51452=CARTESIAN_POINT('Ctrl Pts',(-5.27650989459288,5.89751675225094,110.089875701985));
#51453=CARTESIAN_POINT('Ctrl Pts',(-5.41915921673199,5.76338740531198,110.097786122828));
#51454=CARTESIAN_POINT('Ctrl Pts',(-5.48106338800262,5.70518056674579,110.101218933018));
#51455=CARTESIAN_POINT('Ctrl Pts',(-5.54199802297115,5.64600600346155,110.104651743209));
#51456=CARTESIAN_POINT('Ctrl Pts',(-5.60193227078134,5.58589973357727,110.108084553399));
#51457=CARTESIAN_POINT('Ctrl Pts',(-5.74709914815854,5.44031620114478,110.116399170736));
#51458=CARTESIAN_POINT('Ctrl Pts',(-5.88671264835898,5.28894550837697,110.124713788074));
#51459=CARTESIAN_POINT('Ctrl Pts',(-6.02031237203694,5.13222758099239,110.133028405411));
#51460=CARTESIAN_POINT('Ctrl Pts',(-6.15374697315395,4.97570334910959,110.141332746299));
#51461=CARTESIAN_POINT('Ctrl Pts',(-6.28118243254853,4.81384528582643,110.149637087186));
#51462=CARTESIAN_POINT('Ctrl Pts',(-6.40219537707625,4.64712979738499,110.157941428073));
#51463=CARTESIAN_POINT('Ctrl Pts',(-6.52306675501411,4.48060934050211,110.166236054155));
#51464=CARTESIAN_POINT('Ctrl Pts',(-6.63753043204616,4.3092430287315,110.174530680237));
#51465=CARTESIAN_POINT('Ctrl Pts',(-6.7452029677036,4.13354060394749,110.182825306319));
#51466=CARTESIAN_POINT('Ctrl Pts',(-6.85271338137667,3.95810273340278,110.191107443224));
#51467=CARTESIAN_POINT('Ctrl Pts',(-6.95345290714794,3.77834202845535,110.19938958013));
#51468=CARTESIAN_POINT('Ctrl Pts',(-7.04708107639469,3.59479753292447,110.207671717036));
#51469=CARTESIAN_POINT('Ctrl Pts',(-7.1406229021927,3.41142230124729,110.215946216195));
#51470=CARTESIAN_POINT('Ctrl Pts',(-7.22706631643813,3.22427049770358,110.224220715354));
#51471=CARTESIAN_POINT('Ctrl Pts',(-7.30611559512506,3.03390769646514,110.232495214513));
#51472=CARTESIAN_POINT('Ctrl Pts',(-7.38507395463228,2.84376384257224,110.240760196688));
#51473=CARTESIAN_POINT('Ctrl Pts',(-7.45665503644043,2.65041663065321,110.249025178864));
#51474=CARTESIAN_POINT('Ctrl Pts',(-7.52061015159196,2.45445390011138,110.257290161039));
#51475=CARTESIAN_POINT('Ctrl Pts',(-7.54617193128604,2.37613090539093,110.260593534867));
#51476=CARTESIAN_POINT('Ctrl Pts',(-7.57051601546906,2.29739034014392,110.263896908695));
#51477=CARTESIAN_POINT('Ctrl Pts',(-7.59362865868611,2.21827067644617,110.267200282522));
#51478=CARTESIAN_POINT('Ctrl Pts',(-7.64735406795353,2.03435677818093,110.274878985005));
#51479=CARTESIAN_POINT('Ctrl Pts',(-7.69438959007227,1.84850444935335,110.282557687488));
#51480=CARTESIAN_POINT('Ctrl Pts',(-7.7346069444322,1.66125748008586,110.290236389971));
#51481=CARTESIAN_POINT('Ctrl Pts',(-7.77483067255035,1.4739808353977,110.297916309397));
#51482=CARTESIAN_POINT('Ctrl Pts',(-7.80823401252635,1.28530946842787,110.305596228822));
#51483=CARTESIAN_POINT('Ctrl Pts',(-7.83474004329294,1.09579626483312,110.313276148247));
#51484=CARTESIAN_POINT('Ctrl Pts',(-7.86126910490242,0.906118394983401,
110.320962740682));
#51485=CARTESIAN_POINT('Ctrl Pts',(-7.88088884210709,0.715597589647698,
110.328649333118));
#51486=CARTESIAN_POINT('Ctrl Pts',(-7.89357427237069,0.524791583933543,
110.336335925553));
#51487=CARTESIAN_POINT('Ctrl Pts',(-7.90521327432692,0.349725273401021,
110.343388446637));
#51488=CARTESIAN_POINT('Ctrl Pts',(-7.91101540931456,0.174419123218421,
110.350440967722));
#51489=CARTESIAN_POINT('Ctrl Pts',(-7.91099996925002,-0.000697514249990952,
110.357493488806));
#51490=CARTESIAN_POINT('',(-7.91099998544305,0.000479916693955615,112.357717318707));
#51491=CARTESIAN_POINT('Ctrl Pts',(-7.91099996833566,-0.000689401199207026,
110.357696230784));
#51492=CARTESIAN_POINT('Ctrl Pts',(-7.9107977438684,-2.20213188969668,110.446274420177));
#51493=CARTESIAN_POINT('Ctrl Pts',(-6.9419754291647,-4.38625843456785,110.534852609569));
#51494=CARTESIAN_POINT('Ctrl Pts',(-3.67820201488108,-7.34180684107713,
110.712018234694));
#51495=CARTESIAN_POINT('Ctrl Pts',(-1.40868175871581,-8.08992666571357,
110.800605670427));
#51496=CARTESIAN_POINT('Ctrl Pts',(2.97309270521375,-7.6545422802521,110.977780541892));
#51497=CARTESIAN_POINT('Ctrl Pts',(5.05102072675661,-6.47444880834171,111.066367977625));
#51498=CARTESIAN_POINT('Ctrl Pts',(7.66951518847874,-2.93425195367679,111.24354284909));
#51499=CARTESIAN_POINT('Ctrl Pts',(8.18956872247064,-0.601881960099215,
111.332130284823));
#51500=CARTESIAN_POINT('Ctrl Pts',(7.32306689761362,3.71537198232395,111.509305156288));
#51501=CARTESIAN_POINT('Ctrl Pts',(5.94329958850258,5.66643518936441,111.597892592021));
#51502=CARTESIAN_POINT('Ctrl Pts',(2.16154501637983,7.92205913232953,111.775067463487));
#51503=CARTESIAN_POINT('Ctrl Pts',(-0.210816529298622,8.20894963713,111.863654899219));
#51504=CARTESIAN_POINT('Ctrl Pts',(-4.42123908576242,6.91982244717947,112.040829770685));
#51505=CARTESIAN_POINT('Ctrl Pts',(-6.22631625634013,5.35390358803712,112.129417206417));
#51506=CARTESIAN_POINT('Ctrl Pts',(-7.65310523772621,2.31349256505397,112.264552858839));
#51507=CARTESIAN_POINT('Ctrl Pts',(-7.91092910873721,1.15734629425771,112.311101075528));
#51508=CARTESIAN_POINT('Ctrl Pts',(-7.91099998538287,0.000477168944170301,
112.357649292217));
#51509=CARTESIAN_POINT('',(-7.91099861424721,0.00331099508029248,114.357668491763));
#51510=CARTESIAN_POINT('Ctrl Pts',(-7.91099998544305,0.000479916693955615,
112.357717318707));
#51511=CARTESIAN_POINT('Ctrl Pts',(-7.91101205913391,-0.198544141936758,
112.365761839543));
#51512=CARTESIAN_POINT('Ctrl Pts',(-7.90350929980243,-0.397800859065147,
112.373806360379));
#51513=CARTESIAN_POINT('Ctrl Pts',(-7.88846502048386,-0.596691394778329,
112.381850881216));
#51514=CARTESIAN_POINT('Ctrl Pts',(-7.87343761463156,-0.795358857476649,
112.389886379423));
#51515=CARTESIAN_POINT('Ctrl Pts',(-7.85088556931378,-0.993660631931276,
112.39792187763));
#51516=CARTESIAN_POINT('Ctrl Pts',(-7.82083419264467,-1.19099686446272,
112.405957375838));
#51517=CARTESIAN_POINT('Ctrl Pts',(-7.79082085321744,-1.38808332054989,
112.41398270319));
#51518=CARTESIAN_POINT('Ctrl Pts',(-7.75332716275793,-1.58420634900734,
112.422008030543));
#51519=CARTESIAN_POINT('Ctrl Pts',(-7.70843027685618,-1.77877026814792,
112.430033357895));
#51520=CARTESIAN_POINT('Ctrl Pts',(-7.66356643316235,-1.97319099647826,
112.438052778946));
#51521=CARTESIAN_POINT('Ctrl Pts',(-7.61131032372251,-2.16605458308518,
112.446072199997));
#51522=CARTESIAN_POINT('Ctrl Pts',(-7.55179050507049,-2.35677346546655,
112.454091621048));
#51523=CARTESIAN_POINT('Ctrl Pts',(-7.49231445891098,-2.54735208799767,
112.462105144399));
#51524=CARTESIAN_POINT('Ctrl Pts',(-7.42558545338359,-2.73578883877218,
112.47011866775));
#51525=CARTESIAN_POINT('Ctrl Pts',(-7.35178247536766,-2.92150910230946,
112.478132191101));
#51526=CARTESIAN_POINT('Ctrl Pts',(-7.30055048825237,-3.05043097517122,
112.483694957484));
#51527=CARTESIAN_POINT('Ctrl Pts',(-7.24591078874864,-3.17804408040484,
112.489257723867));
#51528=CARTESIAN_POINT('Ctrl Pts',(-7.18793731267412,-3.30416073898761,
112.49482049025));
#51529=CARTESIAN_POINT('Ctrl Pts',(-7.10179061717378,-3.49156598221443,
112.503086579748));
#51530=CARTESIAN_POINT('Ctrl Pts',(-7.00835969554944,-3.67549421227672,
112.511352669245));
#51531=CARTESIAN_POINT('Ctrl Pts',(-6.90795907835648,-3.85538874456938,
112.519618758743));
#51532=CARTESIAN_POINT('Ctrl Pts',(-6.80746817074922,-4.03544505626445,
112.527892281946));
#51533=CARTESIAN_POINT('Ctrl Pts',(-6.69999519769422,-4.21146017185755,
112.53616580515));
#51534=CARTESIAN_POINT('Ctrl Pts',(-6.58589874287142,-4.38290528629637,
112.544439328353));
#51535=CARTESIAN_POINT('Ctrl Pts',(-6.4716922596982,-4.55451573298111,112.552720830088));
#51536=CARTESIAN_POINT('Ctrl Pts',(-6.3508497054498,-4.72154713585784,112.561002331822));
#51537=CARTESIAN_POINT('Ctrl Pts',(-6.22377124380185,-4.88350207380167,
112.569283833557));
#51538=CARTESIAN_POINT('Ctrl Pts',(-6.09648119925438,-5.04572666322629,
112.577579123813));
#51539=CARTESIAN_POINT('Ctrl Pts',(-5.96293467128937,-5.20285765809875,
112.58587441407));
#51540=CARTESIAN_POINT('Ctrl Pts',(-5.82357149775722,-5.3544314367176,112.594169704326));
#51541=CARTESIAN_POINT('Ctrl Pts',(-5.68408193495291,-5.50614267847735,
112.602472517629));
#51542=CARTESIAN_POINT('Ctrl Pts',(-5.53876540024198,-5.65228643257972,
112.610775330933));
#51543=CARTESIAN_POINT('Ctrl Pts',(-5.38809735982587,-5.79243712447857,
112.619078144236));
#51544=CARTESIAN_POINT('Ctrl Pts',(-5.23719826705766,-5.93280274017227,
112.627393690064));
#51545=CARTESIAN_POINT('Ctrl Pts',(-5.08093148405528,-6.0671567279693,112.635709235892));
#51546=CARTESIAN_POINT('Ctrl Pts',(-4.91980566072326,-6.19511366003202,
112.64402478172));
#51547=CARTESIAN_POINT('Ctrl Pts',(-4.8557894760444,-6.24595165995329,112.647328594271));
#51548=CARTESIAN_POINT('Ctrl Pts',(-4.79100660653029,-6.29578035355523,
112.650632406822));
#51549=CARTESIAN_POINT('Ctrl Pts',(-4.7254901745442,-6.34457749659394,112.653936219373));
#51550=CARTESIAN_POINT('Ctrl Pts',(-4.5686363829092,-6.46140340842323,112.661845922478));
#51551=CARTESIAN_POINT('Ctrl Pts',(-4.40724891346103,-6.57255718027244,
112.669755625583));
#51552=CARTESIAN_POINT('Ctrl Pts',(-4.24177559867099,-6.67766881258118,
112.677665328688));
#51553=CARTESIAN_POINT('Ctrl Pts',(-4.07647016462471,-6.78267380401534,
112.685567007013));
#51554=CARTESIAN_POINT('Ctrl Pts',(-3.90708743087371,-6.88164868324912,
112.693468685339));
#51555=CARTESIAN_POINT('Ctrl Pts',(-3.73410730270417,-6.97426438069933,
112.701370363664));
#51556=CARTESIAN_POINT('Ctrl Pts',(-3.56127062635837,-7.06680327227104,
112.709265489155));
#51557=CARTESIAN_POINT('Ctrl Pts',(-3.38484280093639,-7.15299332627278,
112.717160614646));
#51558=CARTESIAN_POINT('Ctrl Pts',(-3.20533188400639,-7.23254924030055,
112.725055740136));
#51559=CARTESIAN_POINT('Ctrl Pts',(-3.02593658914555,-7.31205391276847,
112.732945780417));
#51560=CARTESIAN_POINT('Ctrl Pts',(-2.84346247326496,-7.38493281976084,
112.740835820698));
#51561=CARTESIAN_POINT('Ctrl Pts',(-2.65844157392847,-7.45094687929049,
112.748725860978));
#51562=CARTESIAN_POINT('Ctrl Pts',(-2.47350558621744,-7.51693064299347,
112.756612280283));
#51563=CARTESIAN_POINT('Ctrl Pts',(-2.28602546804307,-7.57605572168821,
112.764498699588));
#51564=CARTESIAN_POINT('Ctrl Pts',(-2.09655285072453,-7.62813130092284,
112.772385118893));
#51565=CARTESIAN_POINT('Ctrl Pts',(-1.9071321094482,-7.68019262229276,112.780269378962));
#51566=CARTESIAN_POINT('Ctrl Pts',(-1.71572028831223,-7.72520819996158,
112.78815363903));
#51567=CARTESIAN_POINT('Ctrl Pts',(-1.52288405188894,-7.76303710956623,
112.796037899099));
#51568=CARTESIAN_POINT('Ctrl Pts',(-1.33002530193706,-7.80087043567606,
112.80392307965));
#51569=CARTESIAN_POINT('Ctrl Pts',(-1.13574214129956,-7.83151534411266,
112.811808260202));
#51570=CARTESIAN_POINT('Ctrl Pts',(-0.940611930730435,-7.85488193391648,
112.819693440754));
#51571=CARTESIAN_POINT('Ctrl Pts',(-0.745457381665204,-7.87825143822367,
112.82757960482));
#51572=CARTESIAN_POINT('Ctrl Pts',(-0.549455914445102,-7.89434077323925,
112.835465768886));
#51573=CARTESIAN_POINT('Ctrl Pts',(-0.353190498390034,-7.90311188531752,
112.843351932953));
#51574=CARTESIAN_POINT('Ctrl Pts',(-0.156867672318178,-7.91188556305255,
112.851240403818));
#51575=CARTESIAN_POINT('Ctrl Pts',(0.0397189121080171,-7.91333673656131,
112.859128874683));
#51576=CARTESIAN_POINT('Ctrl Pts',(0.2359855440319,-7.90747948609467,112.867017345548));
#51577=CARTESIAN_POINT('Ctrl Pts',(0.432342517195068,-7.90161953954433,
112.874909447465));
#51578=CARTESIAN_POINT('Ctrl Pts',(0.628378900205937,-7.8884444756149,112.882801549381));
#51579=CARTESIAN_POINT('Ctrl Pts',(0.823515112172881,-7.86802032661475,
112.890693651298));
#51580=CARTESIAN_POINT('Ctrl Pts',(1.01887754588227,-7.84757249986393,112.898594902541));
#51581=CARTESIAN_POINT('Ctrl Pts',(1.21333738122448,-7.81985883761164,112.906496153785));
#51582=CARTESIAN_POINT('Ctrl Pts',(1.40632309181363,-7.784996876135,112.914397405029));
#51583=CARTESIAN_POINT('Ctrl Pts',(1.59943668037931,-7.750111814103,112.922303891873));
#51584=CARTESIAN_POINT('Ctrl Pts',(1.79107386132513,-7.70806908361338,112.930210378716));
#51585=CARTESIAN_POINT('Ctrl Pts',(1.98067706652023,-7.65903645102704,112.93811686556));
#51586=CARTESIAN_POINT('Ctrl Pts',(2.17054148159449,-7.6099362678525,112.946034244902));
#51587=CARTESIAN_POINT('Ctrl Pts',(2.35836599483712,-7.5538270461825,112.953951624243));
#51588=CARTESIAN_POINT('Ctrl Pts',(2.54361072498379,-7.49092554226428,112.961869003585));
#51589=CARTESIAN_POINT('Ctrl Pts',(2.62393086671046,-7.46365212020509,112.96530189493));
#51590=CARTESIAN_POINT('Ctrl Pts',(2.70376629238775,-7.43510235247908,112.968734786275));
#51591=CARTESIAN_POINT('Ctrl Pts',(2.78307438609223,-7.40529661536102,112.97216767762));
#51592=CARTESIAN_POINT('Ctrl Pts',(2.96423492963485,-7.33721247306506,112.98000930428));
#51593=CARTESIAN_POINT('Ctrl Pts',(3.14318093264782,-7.2623693071675,112.987850930941));
#51594=CARTESIAN_POINT('Ctrl Pts',(3.31936483863494,-7.18092877475011,112.995692557601));
#51595=CARTESIAN_POINT('Ctrl Pts',(3.4953413013473,-7.09958413242352,113.003524951337));
#51596=CARTESIAN_POINT('Ctrl Pts',(3.66856182698873,-7.01165773657921,113.011357345072));
#51597=CARTESIAN_POINT('Ctrl Pts',(3.83849466888646,-6.91736074503349,113.019189738808));
#51598=CARTESIAN_POINT('Ctrl Pts',(4.00826050814803,-6.82315642448646,113.027014435207));
#51599=CARTESIAN_POINT('Ctrl Pts',(4.17474479279578,-6.72259414520845,113.034839131605));
#51600=CARTESIAN_POINT('Ctrl Pts',(4.3374362261068,-6.61593288844864,113.042663828004));
#51601=CARTESIAN_POINT('Ctrl Pts',(4.49999942508129,-6.50935570271345,113.050482356931));
#51602=CARTESIAN_POINT('Ctrl Pts',(4.65877543429084,-6.39668930578726,113.058300885858));
#51603=CARTESIAN_POINT('Ctrl Pts',(4.81327786445093,-6.27823838346289,113.066119414785));
#51604=CARTESIAN_POINT('Ctrl Pts',(4.96768856106883,-6.15985778962894,113.073933301576));
#51605=CARTESIAN_POINT('Ctrl Pts',(5.11783045472054,-6.03569972512417,113.081747188367));
#51606=CARTESIAN_POINT('Ctrl Pts',(5.26324629612979,-5.90611203976661,113.089561075157));
#51607=CARTESIAN_POINT('Ctrl Pts',(5.40860407023905,-5.77657610122649,113.097371841715));
#51608=CARTESIAN_POINT('Ctrl Pts',(5.54923928989609,-5.6416150952412,113.105182608273));
#51609=CARTESIAN_POINT('Ctrl Pts',(5.68472781341491,-5.50161709748933,113.112993374831));
#51610=CARTESIAN_POINT('Ctrl Pts',(5.82021095192375,-5.36162466397712,113.120803830948));
#51611=CARTESIAN_POINT('Ctrl Pts',(5.95054755074093,-5.2165958839276,113.128614287066));
#51612=CARTESIAN_POINT('Ctrl Pts',(6.0753500520282,-5.06695596441502,113.136424743184));
#51613=CARTESIAN_POINT('Ctrl Pts',(6.20015599512677,-4.91731191812324,113.144235414699));
#51614=CARTESIAN_POINT('Ctrl Pts',(6.31942731061589,-4.76305674885004,113.152046086214));
#51615=CARTESIAN_POINT('Ctrl Pts',(6.43281652946883,-4.6046490092289,113.159856757729));
#51616=CARTESIAN_POINT('Ctrl Pts',(6.54622884483228,-4.4462090031713,113.167669020218));
#51617=CARTESIAN_POINT('Ctrl Pts',(6.65375647194648,-4.28361502794457,113.175481282706));
#51618=CARTESIAN_POINT('Ctrl Pts',(6.75509502054357,-4.11735500818516,113.183293545195));
#51619=CARTESIAN_POINT('Ctrl Pts',(6.85647205949167,-3.95103183963779,113.191108774933));
#51620=CARTESIAN_POINT('Ctrl Pts',(6.95165515441584,-3.78104015314079,113.198924004671));
#51621=CARTESIAN_POINT('Ctrl Pts',(7.04038557978585,-3.6078929984055,113.206739234409));
#51622=CARTESIAN_POINT('Ctrl Pts',(7.12921250380062,-3.4345575377345,113.214562963588));
#51623=CARTESIAN_POINT('Ctrl Pts',(7.21157258156766,-3.25806006791309,113.222386692768));
#51624=CARTESIAN_POINT('Ctrl Pts',(7.28725458589867,-3.07893514064504,113.230210421947));
#51625=CARTESIAN_POINT('Ctrl Pts',(7.36298250828826,-2.89970153405514,113.238038897968));
#51626=CARTESIAN_POINT('Ctrl Pts',(7.43202415801405,-2.71783762099379,113.245867373989));
#51627=CARTESIAN_POINT('Ctrl Pts',(7.49421800006026,-2.53389375617306,113.253695850009));
#51628=CARTESIAN_POINT('Ctrl Pts',(7.55649743826388,-2.34969673304131,113.261535100207));
#51629=CARTESIAN_POINT('Ctrl Pts',(7.61191014478525,-2.16341437661997,113.269374350405));
#51630=CARTESIAN_POINT('Ctrl Pts',(7.6603452936068,-1.97560901564964,113.277213600603));
#51631=CARTESIAN_POINT('Ctrl Pts',(7.68750109493618,-1.8703134772816,113.281608779024));
#51632=CARTESIAN_POINT('Ctrl Pts',(7.71246447789895,-1.76453933763496,113.286003957446));
#51633=CARTESIAN_POINT('Ctrl Pts',(7.73522304295573,-1.65838640724249,113.290399135867));
#51634=CARTESIAN_POINT('Ctrl Pts',(7.77618101864123,-1.46734584158682,113.298309019925));
#51635=CARTESIAN_POINT('Ctrl Pts',(7.81011274704514,-1.274529141365,113.306218903983));
#51636=CARTESIAN_POINT('Ctrl Pts',(7.836864811074,-1.08049568853837,113.31412878804));
#51637=CARTESIAN_POINT('Ctrl Pts',(7.86358779112303,-0.886673182613733,
113.322030072728));
#51638=CARTESIAN_POINT('Ctrl Pts',(7.88314660738071,-0.691636897541618,
113.329931357415));
#51639=CARTESIAN_POINT('Ctrl Pts',(7.8954382993942,-0.495958728584598,113.337832642102));
#51640=CARTESIAN_POINT('Ctrl Pts',(7.90771891236974,-0.300456932893186,
113.345726805017));
#51641=CARTESIAN_POINT('Ctrl Pts',(7.91274542803671,-0.104314747953952,
113.353620967932));
#51642=CARTESIAN_POINT('Ctrl Pts',(7.91046633049954,0.0918881604620854,
113.361515130847));
#51643=CARTESIAN_POINT('Ctrl Pts',(7.90818886383349,0.28795067047491,113.369403644876));
#51644=CARTESIAN_POINT('Ctrl Pts',(7.89861620330697,0.484073473865925,113.377292158905));
#51645=CARTESIAN_POINT('Ctrl Pts',(7.88174881111296,0.679673950155128,113.385180672934));
#51646=CARTESIAN_POINT('Ctrl Pts',(7.86489035616241,0.875170786885998,113.393065007208));
#51647=CARTESIAN_POINT('Ctrl Pts',(7.84074490086257,1.07014550511917,113.400949341482));
#51648=CARTESIAN_POINT('Ctrl Pts',(7.80936495986349,1.26401737474461,113.408833675755));
#51649=CARTESIAN_POINT('Ctrl Pts',(7.77799581856399,1.45782252155666,113.416715296562));
#51650=CARTESIAN_POINT('Ctrl Pts',(7.73939720886962,1.65052523609926,113.424596917368));
#51651=CARTESIAN_POINT('Ctrl Pts',(7.69367331250093,1.84155150905725,113.432478538175));
#51652=CARTESIAN_POINT('Ctrl Pts',(7.6479488172701,2.0325802839543,113.44036026221));
#51653=CARTESIAN_POINT('Ctrl Pts',(7.59509892087008,2.22193223594145,113.448241986244));
#51654=CARTESIAN_POINT('Ctrl Pts',(7.53527871465488,2.40904456008376,113.456123710279));
#51655=CARTESIAN_POINT('Ctrl Pts',(7.47545490485943,2.59616815590695,113.464005909111));
#51656=CARTESIAN_POINT('Ctrl Pts',(7.40866005309115,2.78105152607834,113.471888107942));
#51657=CARTESIAN_POINT('Ctrl Pts',(7.33509884102577,2.96314798691905,113.479770306774));
#51658=CARTESIAN_POINT('Ctrl Pts',(7.26152081945135,3.14528605871231,113.48765430677));
#51659=CARTESIAN_POINT('Ctrl Pts',(7.18117348582827,3.3246356322043,113.495538306767));
#51660=CARTESIAN_POINT('Ctrl Pts',(7.09430938119519,3.50067070771959,113.503422306763));
#51661=CARTESIAN_POINT('Ctrl Pts',(7.00741081036265,3.67677563095908,113.511309434997));
#51662=CARTESIAN_POINT('Ctrl Pts',(6.91399046878444,3.84956312649917,113.51919656323));
#51663=CARTESIAN_POINT('Ctrl Pts',(6.81434659574041,4.01853225358726,113.527083691464));
#51664=CARTESIAN_POINT('Ctrl Pts',(6.7145964140664,4.1876816514322,113.534979234363));
#51665=CARTESIAN_POINT('Ctrl Pts',(6.60860961377191,4.35300424647187,113.542874777261));
#51666=CARTESIAN_POINT('Ctrl Pts',(6.49672808557066,4.5140276009521,113.55077032016));
#51667=CARTESIAN_POINT('Ctrl Pts',(6.38477842539586,4.67514901307513,113.55867067117));
#51668=CARTESIAN_POINT('Ctrl Pts',(6.26692708755868,4.83196569004043,113.566571022181));
#51669=CARTESIAN_POINT('Ctrl Pts',(6.14355606739335,4.98403850775597,113.574471373191));
#51670=CARTESIAN_POINT('Ctrl Pts',(6.02002441297259,5.13630933067413,113.582382010791));
#51671=CARTESIAN_POINT('Ctrl Pts',(5.89095894738568,5.28382369785403,113.590292648391));
#51672=CARTESIAN_POINT('Ctrl Pts',(5.75677908451137,5.42617872651947,113.598203285991));
#51673=CARTESIAN_POINT('Ctrl Pts',(5.6978232478711,5.48872656071111,113.601679055365));
#51674=CARTESIAN_POINT('Ctrl Pts',(5.63788049907605,5.55027887715659,113.60515482474));
#51675=CARTESIAN_POINT('Ctrl Pts',(5.57698840264617,5.61080398488043,113.608630594114));
#51676=CARTESIAN_POINT('Ctrl Pts',(5.4384152588507,5.748541966451,113.616540459557));
#51677=CARTESIAN_POINT('Ctrl Pts',(5.29454938429741,5.88132915470733,113.624450325001));
#51678=CARTESIAN_POINT('Ctrl Pts',(5.14577844025169,6.00873407997399,113.632360190444));
#51679=CARTESIAN_POINT('Ctrl Pts',(4.99716917934169,6.1360005425324,113.640261459506));
#51680=CARTESIAN_POINT('Ctrl Pts',(4.84366572664063,6.25789617080285,113.648162728567));
#51681=CARTESIAN_POINT('Ctrl Pts',(4.68569354725228,6.37402517889899,113.656063997629));
#51682=CARTESIAN_POINT('Ctrl Pts',(4.52786369581773,6.49004955841963,113.663958147896));
#51683=CARTESIAN_POINT('Ctrl Pts',(4.36557341432979,6.60031746463485,113.671852298163));
#51684=CARTESIAN_POINT('Ctrl Pts',(4.19928251574874,6.70447219048054,113.679746448431));
#51685=CARTESIAN_POINT('Ctrl Pts',(4.0331105488446,6.80855242459933,113.687634952781));
#51686=CARTESIAN_POINT('Ctrl Pts',(3.8629439565525,6.9065280067639,113.695523457132));
#51687=CARTESIAN_POINT('Ctrl Pts',(3.68927313665149,6.99808436096491,113.703411961483));
#51688=CARTESIAN_POINT('Ctrl Pts',(3.51569427168885,7.08959223805898,113.711296289041));
#51689=CARTESIAN_POINT('Ctrl Pts',(3.33861518067781,7.17468749930346,113.7191806166));
#51690=CARTESIAN_POINT('Ctrl Pts',(3.15855281032658,7.2531003815181,113.727064944158));
#51691=CARTESIAN_POINT('Ctrl Pts',(2.9785523426212,7.3314863066019,113.734946561207));
#51692=CARTESIAN_POINT('Ctrl Pts',(2.79557095552454,7.40319429365219,113.742828178256));
#51693=CARTESIAN_POINT('Ctrl Pts',(2.61014787257316,7.46800167938531,113.750709795306));
#51694=CARTESIAN_POINT('Ctrl Pts',(2.42472225695041,7.53280995031464,113.758591520009));
#51695=CARTESIAN_POINT('Ctrl Pts',(2.23685520163579,7.5907173097183,113.766473244712));
#51696=CARTESIAN_POINT('Ctrl Pts',(2.04710402586936,7.64154998068255,113.774354969415));
#51697=CARTESIAN_POINT('Ctrl Pts',(1.85734135307399,7.69238573159973,113.782237171672));
#51698=CARTESIAN_POINT('Ctrl Pts',(1.6656946656146,7.73614585001636,113.790119373929));
#51699=CARTESIAN_POINT('Ctrl Pts',(1.47273452838523,7.77270699363497,113.798001576186));
#51700=CARTESIAN_POINT('Ctrl Pts',(1.27973023022795,7.80927650465034,113.805885582367));
#51701=CARTESIAN_POINT('Ctrl Pts',(1.08541222237756,7.83864369360576,113.813769588548));
#51702=CARTESIAN_POINT('Ctrl Pts',(0.890359541063216,7.86073666316572,113.821653594729));
#51703=CARTESIAN_POINT('Ctrl Pts',(0.695229397916131,7.88283840657027,113.829540731908));
#51704=CARTESIAN_POINT('Ctrl Pts',(0.499364342549996,7.89766013553226,113.837427869086));
#51705=CARTESIAN_POINT('Ctrl Pts',(0.303347033686154,7.90518194459519,113.845315006265));
#51706=CARTESIAN_POINT('Ctrl Pts',(0.107120494307821,7.91271178250001,113.85321056224));
#51707=CARTESIAN_POINT('Ctrl Pts',(-0.0892582782667623,7.91292612335113,
113.861106118215));
#51708=CARTESIAN_POINT('Ctrl Pts',(-0.28520700646409,7.9058571934651,113.86900167419));
#51709=CARTESIAN_POINT('Ctrl Pts',(-0.481275119430983,7.89878395672505,
113.876902040654));
#51710=CARTESIAN_POINT('Ctrl Pts',(-0.676912322465104,7.88441862783349,
113.884802407118));
#51711=CARTESIAN_POINT('Ctrl Pts',(-0.871542684049729,7.86284518160439,
113.892702773581));
#51712=CARTESIAN_POINT('Ctrl Pts',(-1.06642654898368,7.84124363626049,113.900613430163));
#51713=CARTESIAN_POINT('Ctrl Pts',(-1.26030061279475,7.81241527123588,113.908524086744));
#51714=CARTESIAN_POINT('Ctrl Pts',(-1.45259920484215,7.7764951327762,113.916434743326));
#51715=CARTESIAN_POINT('Ctrl Pts',(-1.53709100505145,7.76071260868223,113.919910513004));
#51716=CARTESIAN_POINT('Ctrl Pts',(-1.62127884796818,7.74356164554976,113.923386282682));
#51717=CARTESIAN_POINT('Ctrl Pts',(-1.70511576575961,7.72505671340723,113.926862052361));
#51718=CARTESIAN_POINT('Ctrl Pts',(-1.89419135151687,7.68332294054891,113.934700880471));
#51719=CARTESIAN_POINT('Ctrl Pts',(-2.08201942337306,7.63458032208507,113.942539708582));
#51720=CARTESIAN_POINT('Ctrl Pts',(-2.26803511231633,7.57891402044516,113.950378536692));
#51721=CARTESIAN_POINT('Ctrl Pts',(-2.45384228055332,7.52331011986722,113.958208577597));
#51722=CARTESIAN_POINT('Ctrl Pts',(-2.6378407778947,7.46079809030432,113.966038618503));
#51723=CARTESIAN_POINT('Ctrl Pts',(-2.8194746672902,7.39151429684803,113.973868659408));
#51724=CARTESIAN_POINT('Ctrl Pts',(-3.00094029886425,7.32229468491749,113.981691446901));
#51725=CARTESIAN_POINT('Ctrl Pts',(-3.18004535845198,7.24631592605009,113.989514234393));
#51726=CARTESIAN_POINT('Ctrl Pts',(-3.35624766588196,7.16376455540394,113.997337021886));
#51727=CARTESIAN_POINT('Ctrl Pts',(-3.5323210224481,7.08127359866901,114.005154084395));
#51728=CARTESIAN_POINT('Ctrl Pts',(-3.70549554087494,6.99221975896303,114.012971146905));
#51729=CARTESIAN_POINT('Ctrl Pts',(-3.87524750166329,6.89683824667887,114.020788209414));
#51730=CARTESIAN_POINT('Ctrl Pts',(-4.04490824068853,6.80150799076711,114.02860107117));
#51731=CARTESIAN_POINT('Ctrl Pts',(-4.21114977999066,6.69985700776171,114.036413932925));
#51732=CARTESIAN_POINT('Ctrl Pts',(-4.37347139883613,6.5921672402604,114.044226794681));
#51733=CARTESIAN_POINT('Ctrl Pts',(-4.53573734475922,6.48451440809837,114.052036976788));
#51734=CARTESIAN_POINT('Ctrl Pts',(-4.69408575621211,6.37082711236166,114.059847158895));
#51735=CARTESIAN_POINT('Ctrl Pts',(-4.84804324068267,6.25143165494682,114.067657341003));
#51736=CARTESIAN_POINT('Ctrl Pts',(-5.00200766873462,6.13203081272019,114.075467875354));
#51737=CARTESIAN_POINT('Ctrl Pts',(-5.15158049051273,6.00692150274678,114.083278409706));
#51738=CARTESIAN_POINT('Ctrl Pts',(-5.29631946797021,5.87647182356895,114.091088944057));
#51739=CARTESIAN_POINT('Ctrl Pts',(-5.44107004639379,5.7460116887258,114.09890010443));
#51740=CARTESIAN_POINT('Ctrl Pts',(-5.58098574665272,5.61021056708316,114.106711264803));
#51741=CARTESIAN_POINT('Ctrl Pts',(-5.71565951738365,5.46947504623083,114.114522425177));
#51742=CARTESIAN_POINT('Ctrl Pts',(-5.85036780105318,5.32870345899106,114.122335587321));
#51743=CARTESIAN_POINT('Ctrl Pts',(-5.97983123573259,5.18299520763568,114.130148749466));
#51744=CARTESIAN_POINT('Ctrl Pts',(-6.10368145743595,5.03279183616336,114.13796191161));
#51745=CARTESIAN_POINT('Ctrl Pts',(-6.22758523271817,4.88252351585212,114.145778452213));
#51746=CARTESIAN_POINT('Ctrl Pts',(-6.34587073633552,4.72775647467498,114.153594992816));
#51747=CARTESIAN_POINT('Ctrl Pts',(-6.45821142898739,4.56896335490849,114.161411533419));
#51748=CARTESIAN_POINT('Ctrl Pts',(-6.57068322527232,4.40998492068102,114.169237196066));
#51749=CARTESIAN_POINT('Ctrl Pts',(-6.67719615072514,4.24697131085798,114.177062858714));
#51750=CARTESIAN_POINT('Ctrl Pts',(-6.77746777470318,4.08042296372079,114.184888521362));
#51751=CARTESIAN_POINT('Ctrl Pts',(-6.8778047589454,3.91376605502315,114.192719285028));
#51752=CARTESIAN_POINT('Ctrl Pts',(-6.97189216478442,3.74357012427854,114.200550048695));
#51753=CARTESIAN_POINT('Ctrl Pts',(-7.05949464910017,3.57035800716483,114.208380812361));
#51754=CARTESIAN_POINT('Ctrl Pts',(-7.14722370979633,3.39689561675125,114.216222890657));
#51755=CARTESIAN_POINT('Ctrl Pts',(-7.2284489874672,3.22040865381887,114.224064968953));
#51756=CARTESIAN_POINT('Ctrl Pts',(-7.30298373583653,3.04143873094743,114.23190704725));
#51757=CARTESIAN_POINT('Ctrl Pts',(-7.3447604898661,2.94112602298145,114.236302535035));
#51758=CARTESIAN_POINT('Ctrl Pts',(-7.38443624370311,2.84003353465224,114.240698022821));
#51759=CARTESIAN_POINT('Ctrl Pts',(-7.42198508013926,2.73825829135789,114.245093510607));
#51760=CARTESIAN_POINT('Ctrl Pts',(-7.50212521020549,2.52104034243423,114.254474759037));
#51761=CARTESIAN_POINT('Ctrl Pts',(-7.57277029602603,2.30018099658234,114.263856007466));
#51762=CARTESIAN_POINT('Ctrl Pts',(-7.63362932991678,2.07644510002896,114.273237255896));
#51763=CARTESIAN_POINT('Ctrl Pts',(-7.69410323020584,1.85412506906133,114.282559137067));
#51764=CARTESIAN_POINT('Ctrl Pts',(-7.74491449709366,1.62896484033121,114.291881018238));
#51765=CARTESIAN_POINT('Ctrl Pts',(-7.78582391605684,1.40173711806362,114.301202899409));
#51766=CARTESIAN_POINT('Ctrl Pts',(-7.82712413812168,1.17233871479164,114.310613831468));
#51767=CARTESIAN_POINT('Ctrl Pts',(-7.8583322206228,0.940833134487127,114.320024763527));
#51768=CARTESIAN_POINT('Ctrl Pts',(-7.87925145285519,0.708037811617052,
114.329435695586));
#51769=CARTESIAN_POINT('Ctrl Pts',(-7.90017068508755,0.475242488747126,
114.338846627645));
#51770=CARTESIAN_POINT('Ctrl Pts',(-7.91080090790091,0.241157474615384,
114.348257559704));
#51771=CARTESIAN_POINT('Ctrl Pts',(-7.91099722849441,0.0066219901636414,
114.357668491763));
#51772=CARTESIAN_POINT('',(-7.91099829967312,-0.00366759908724605,116.357668491763));
#51773=CARTESIAN_POINT('Ctrl Pts',(-7.911,-3.05644398679306E-12,114.357668491763));
#51774=CARTESIAN_POINT('Ctrl Pts',(-7.91099999999915,-2.20167589667,114.446255927496));
#51775=CARTESIAN_POINT('Ctrl Pts',(-6.94214576672185,-4.38610418338986,
114.534843363229));
#51776=CARTESIAN_POINT('Ctrl Pts',(-3.67820201487939,-7.34180684107811,
114.712018234694));
#51777=CARTESIAN_POINT('Ctrl Pts',(-1.40868175871339,-8.08992666571412,
114.800605670427));
#51778=CARTESIAN_POINT('Ctrl Pts',(2.97309270521692,-7.654542280251,114.977780541892));
#51779=CARTESIAN_POINT('Ctrl Pts',(5.05102072675974,-6.47444880833942,115.066367977625));
#51780=CARTESIAN_POINT('Ctrl Pts',(7.66951518848055,-2.9342519536724,115.24354284909));
#51781=CARTESIAN_POINT('Ctrl Pts',(8.18956872247114,-0.601881960093957,
115.332130284823));
#51782=CARTESIAN_POINT('Ctrl Pts',(7.32306689761095,3.71537198232949,115.509305156289));
#51783=CARTESIAN_POINT('Ctrl Pts',(5.94329958849806,5.66643518936933,115.597892592021));
#51784=CARTESIAN_POINT('Ctrl Pts',(2.16154501637258,7.92205913233164,115.775067463487));
#51785=CARTESIAN_POINT('Ctrl Pts',(-0.210816529306704,8.20894963712991,
115.86365489922));
#51786=CARTESIAN_POINT('Ctrl Pts',(-4.42123908577003,6.91982244717475,116.040829770685));
#51787=CARTESIAN_POINT('Ctrl Pts',(-6.22631625634641,5.35390358803001,116.129417206418));
#51788=CARTESIAN_POINT('Ctrl Pts',(-7.65317280859632,2.31334857513979,116.264559258688));
#51789=CARTESIAN_POINT('Ctrl Pts',(-7.91100000000042,1.157028378361,116.311113875226));
#51790=CARTESIAN_POINT('Ctrl Pts',(-7.911,-2.88657986402541E-12,116.357668491763));
#51791=CARTESIAN_POINT('',(-7.91739038802327,-0.00251068180719704,118.357668491763));
#51792=CARTESIAN_POINT('Ctrl Pts',(-7.91099659934624,-0.00733519817160553,
116.357668491763));
#51793=CARTESIAN_POINT('Ctrl Pts',(-7.91079165791022,-0.228364128203642,
116.366524152405));
#51794=CARTESIAN_POINT('Ctrl Pts',(-7.9013198004979,-0.449004782483658,
116.375379813047));
#51795=CARTESIAN_POINT('Ctrl Pts',(-7.88270168216785,-0.668532115868853,
116.384235473689));
#51796=CARTESIAN_POINT('Ctrl Pts',(-7.86395074028927,-0.889625579563492,
116.393154311514));
#51797=CARTESIAN_POINT('Ctrl Pts',(-7.83592265161949,-1.1095896151356,116.402073149339));
#51798=CARTESIAN_POINT('Ctrl Pts',(-7.79879015635228,-1.32770218693152,
116.410991987165));
#51799=CARTESIAN_POINT('Ctrl Pts',(-7.76152078889647,-1.546618732305,116.419943700261));
#51800=CARTESIAN_POINT('Ctrl Pts',(-7.71507987912638,-1.76366999155661,
116.428895413357));
#51801=CARTESIAN_POINT('Ctrl Pts',(-7.65969030410487,-1.9781469725988,116.437847126454));
#51802=CARTESIAN_POINT('Ctrl Pts',(-7.60404426163348,-2.19361703517964,
116.446840288199));
#51803=CARTESIAN_POINT('Ctrl Pts',(-7.53936658935755,-2.40648877887871,
116.455833449944));
#51804=CARTESIAN_POINT('Ctrl Pts',(-7.46593033294524,-2.6160667544251,116.464826611689));
#51805=CARTESIAN_POINT('Ctrl Pts',(-7.44446218479463,-2.67733418890422,
116.467455647238));
#51806=CARTESIAN_POINT('Ctrl Pts',(-7.42224581913866,-2.73832029444676,
116.470084682787));
#51807=CARTESIAN_POINT('Ctrl Pts',(-7.39928879407273,-2.79900809965062,
116.472713718336));
#51808=CARTESIAN_POINT('Ctrl Pts',(-7.33016084335,-2.98175057588845,116.480630242334));
#51809=CARTESIAN_POINT('Ctrl Pts',(-7.25416142372823,-3.16218858067247,
116.488546766333));
#51810=CARTESIAN_POINT('Ctrl Pts',(-7.17146226843079,-3.33976794590186,
116.496463290331));
#51811=CARTESIAN_POINT('Ctrl Pts',(-7.08885838759699,-3.51714272888714,
116.504370694012));
#51812=CARTESIAN_POINT('Ctrl Pts',(-6.99957028891942,-3.69166512275979,
116.512278097693));
#51813=CARTESIAN_POINT('Ctrl Pts',(-6.90381897258189,-3.86279750877758,
116.520185501374));
#51814=CARTESIAN_POINT('Ctrl Pts',(-6.80816022438812,-4.03376445156269,
116.528085260526));
#51815=CARTESIAN_POINT('Ctrl Pts',(-6.70605087262423,-4.20134761648342,
116.535985019678));
#51816=CARTESIAN_POINT('Ctrl Pts',(-6.59775947367232,-4.36503046124162,
116.54388477883));
#51817=CARTESIAN_POINT('Ctrl Pts',(-6.48955270618156,-4.52858538523739,
116.551778364194));
#51818=CARTESIAN_POINT('Ctrl Pts',(-6.37517370628077,-4.68824577591688,
116.559671949558));
#51819=CARTESIAN_POINT('Ctrl Pts',(-6.25493645407182,-4.84352051255318,
116.567565534922));
#51820=CARTESIAN_POINT('Ctrl Pts',(-6.13477090214157,-4.99870265524137,
116.575454413156));
#51821=CARTESIAN_POINT('Ctrl Pts',(-6.00875426919875,-5.1495040833816,116.583343291391));
#51822=CARTESIAN_POINT('Ctrl Pts',(-5.87724342427105,-5.2954632216514,116.591232169626));
#51823=CARTESIAN_POINT('Ctrl Pts',(-5.74578665200444,-5.44136234662708,
116.59911780423));
#51824=CARTESIAN_POINT('Ctrl Pts',(-5.60884040019354,-5.58242289407251,
116.607003438833));
#51825=CARTESIAN_POINT('Ctrl Pts',(-5.46680151270793,-5.7182166993438,116.614889073437));
#51826=CARTESIAN_POINT('Ctrl Pts',(-5.32477526051347,-5.85399842486498,
116.622774006562));
#51827=CARTESIAN_POINT('Ctrl Pts',(-5.17765751971691,-5.98451409895819,
116.630658939687));
#51828=CARTESIAN_POINT('Ctrl Pts',(-5.02588202282583,-6.10937238123821,
116.638543872812));
#51829=CARTESIAN_POINT('Ctrl Pts',(-4.87410705215107,-6.23423023062577,
116.646428778599));
#51830=CARTESIAN_POINT('Ctrl Pts',(-4.71767462341049,-6.35343050784156,
116.654313684386));
#51831=CARTESIAN_POINT('Ctrl Pts',(-4.55705165747088,-6.46662208507208,
116.662198590174));
#51832=CARTESIAN_POINT('Ctrl Pts',(-4.39640229970778,-6.57983226071478,
116.670084791523));
#51833=CARTESIAN_POINT('Ctrl Pts',(-4.23156131455783,-6.68703157060123,
116.677970992873));
#51834=CARTESIAN_POINT('Ctrl Pts',(-4.06302490889848,-6.78791201988288,
116.685857194222));
#51835=CARTESIAN_POINT('Ctrl Pts',(-3.89443253464182,-6.8888259701593,116.693746014469));
#51836=CARTESIAN_POINT('Ctrl Pts',(-3.72214259028624,-6.98341670189376,
116.701634834717));
#51837=CARTESIAN_POINT('Ctrl Pts',(-3.54667640443721,-7.07142188546323,
116.709523654964));
#51838=CARTESIAN_POINT('Ctrl Pts',(-3.37104038351512,-7.15951224992786,
116.717420110861));
#51839=CARTESIAN_POINT('Ctrl Pts',(-3.19222228861093,-7.24100417960231,
116.725316566758));
#51840=CARTESIAN_POINT('Ctrl Pts',(-3.01076494796376,-7.31568284086405,
116.733213022655));
#51841=CARTESIAN_POINT('Ctrl Pts',(-2.82920731566157,-7.39040277709713,
116.741113842932));
#51842=CARTESIAN_POINT('Ctrl Pts',(-2.64500785192931,-7.45830181786224,
116.749014663208));
#51843=CARTESIAN_POINT('Ctrl Pts',(-2.45872538473524,-7.51921475171833,
116.756915483484));
#51844=CARTESIAN_POINT('Ctrl Pts',(-2.27221655911886,-7.58020170303733,
116.764825904327));
#51845=CARTESIAN_POINT('Ctrl Pts',(-2.08362000463707,-7.63418549598408,
116.77273632517));
#51846=CARTESIAN_POINT('Ctrl Pts',(-1.89350666932651,-7.68105158772001,
116.780646746013));
#51847=CARTESIAN_POINT('Ctrl Pts',(-1.81100499114681,-7.70138962035523,
116.784079556203));
#51848=CARTESIAN_POINT('Ctrl Pts',(-1.72821776810303,-7.72038789334774,
116.787512366392));
#51849=CARTESIAN_POINT('Ctrl Pts',(-1.6451920007676,-7.7380400800597,116.790945176582));
#51850=CARTESIAN_POINT('Ctrl Pts',(-1.44409510160924,-7.78079548148584,
116.799259793919));
#51851=CARTESIAN_POINT('Ctrl Pts',(-1.24115767201284,-7.8157442401945,116.807574411257));
#51852=CARTESIAN_POINT('Ctrl Pts',(-1.03699919790736,-7.84273891338603,
116.815889028594));
#51853=CARTESIAN_POINT('Ctrl Pts',(-0.833093053441164,-7.86970022251477,
116.824193369481));
#51854=CARTESIAN_POINT('Ctrl Pts',(-0.627969163730191,-7.88872701493928,
116.832497710369));
#51855=CARTESIAN_POINT('Ctrl Pts',(-0.422257519540355,-7.89972275381811,
116.840802051256));
#51856=CARTESIAN_POINT('Ctrl Pts',(-0.216786526432214,-7.91070562936845,
116.849096677337));
#51857=CARTESIAN_POINT('Ctrl Pts',(-0.0107294420360976,-7.91367617457794,
116.857391303419));
#51858=CARTESIAN_POINT('Ctrl Pts',(0.195277457471319,-7.9085894895742,116.865685929501));
#51859=CARTESIAN_POINT('Ctrl Pts',(0.400974173447822,-7.90351046356596,
116.873968066407));
#51860=CARTESIAN_POINT('Ctrl Pts',(0.606620563022363,-7.89039842520223,
116.882250203312));
#51861=CARTESIAN_POINT('Ctrl Pts',(0.811579102264985,-7.86926047102056,
116.890532340218));
#51862=CARTESIAN_POINT('Ctrl Pts',(1.01634862972473,-7.84814201015896,116.898806839377));
#51863=CARTESIAN_POINT('Ctrl Pts',(1.22043128110172,-7.81901242310457,116.907081338536));
#51864=CARTESIAN_POINT('Ctrl Pts',(1.42319157471596,-7.7819307849439,116.915355837695));
#51865=CARTESIAN_POINT('Ctrl Pts',(1.6257186619076,-7.74489179653493,116.92362081987));
#51866=CARTESIAN_POINT('Ctrl Pts',(1.82692613844127,-7.69991906017166,116.931885802045));
#51867=CARTESIAN_POINT('Ctrl Pts',(2.02618538996855,-7.64712323462085,116.940150784221));
#51868=CARTESIAN_POINT('Ctrl Pts',(2.10582594847745,-7.62602163456174,116.943454158049));
#51869=CARTESIAN_POINT('Ctrl Pts',(2.18515536128749,-7.60367090045974,116.946757531877));
#51870=CARTESIAN_POINT('Ctrl Pts',(2.26413386273611,-7.58008039875645,116.950060905705));
#51871=CARTESIAN_POINT('Ctrl Pts',(2.46176313369386,-7.52104947809277,116.958326995203));
#51872=CARTESIAN_POINT('Ctrl Pts',(2.65697061966016,-7.45431891274739,116.966593084701));
#51873=CARTESIAN_POINT('Ctrl Pts',(2.84916104808126,-7.38012210753294,116.974859174198));
#51874=CARTESIAN_POINT('Ctrl Pts',(3.04152431362093,-7.30585857702876,116.983132697402));
#51875=CARTESIAN_POINT('Ctrl Pts',(3.23086483097424,-7.22411550795258,116.991406220605));
#51876=CARTESIAN_POINT('Ctrl Pts',(3.41660875776642,-7.13517383084349,116.999679743808));
#51877=CARTESIAN_POINT('Ctrl Pts',(3.60253180579428,-7.04614638326868,117.007961245543));
#51878=CARTESIAN_POINT('Ctrl Pts',(3.7848510742948,-6.94990659525351,117.016242747277));
#51879=CARTESIAN_POINT('Ctrl Pts',(3.96301796747552,-6.84678096549512,117.024524249011));
#51880=CARTESIAN_POINT('Ctrl Pts',(4.14148150469202,-6.74348363378661,117.032819539268));
#51881=CARTESIAN_POINT('Ctrl Pts',(4.31577858984202,-6.6332776866314,117.041114829524));
#51882=CARTESIAN_POINT('Ctrl Pts',(4.48538853247721,-6.51653364241465,117.04941011978));
#51883=CARTESIAN_POINT('Ctrl Pts',(4.65515229535517,-6.39968372234567,117.057712933083));
#51884=CARTESIAN_POINT('Ctrl Pts',(4.82022019296743,-6.2762840412262,117.066015746387));
#51885=CARTESIAN_POINT('Ctrl Pts',(4.98010421305185,-6.14674572657298,117.07431855969));
#51886=CARTESIAN_POINT('Ctrl Pts',(5.14023341837178,-6.01700876241016,117.082634105518));
#51887=CARTESIAN_POINT('Ctrl Pts',(5.29516263203528,-5.88111453788343,117.090949651346));
#51888=CARTESIAN_POINT('Ctrl Pts',(5.44443894142245,-5.73951266338204,117.099265197174));
#51889=CARTESIAN_POINT('Ctrl Pts',(5.5037472483953,-5.683253452022,117.102569009725));
#51890=CARTESIAN_POINT('Ctrl Pts',(5.56216366462417,-5.62609366540991,117.105872822277));
#51891=CARTESIAN_POINT('Ctrl Pts',(5.61966152320723,-5.5680629813773,117.109176634828));
#51892=CARTESIAN_POINT('Ctrl Pts',(5.75731793786419,-5.42913092197752,117.117086337933));
#51893=CARTESIAN_POINT('Ctrl Pts',(5.88999360825696,-5.28491496316134,117.124996041038));
#51894=CARTESIAN_POINT('Ctrl Pts',(6.01725942153507,-5.13580666049136,117.132905744143));
#51895=CARTESIAN_POINT('Ctrl Pts',(6.14439611744201,-4.98684963546276,117.140807422468));
#51896=CARTESIAN_POINT('Ctrl Pts',(6.26613366716165,-4.83301041354343,117.148709100794));
#51897=CARTESIAN_POINT('Ctrl Pts',(6.38207898871818,-4.6747180430227,117.156610779119));
#51898=CARTESIAN_POINT('Ctrl Pts',(6.49792815721914,-4.5165569438193,117.16450590461));
#51899=CARTESIAN_POINT('Ctrl Pts',(6.60799446436491,-4.35395032949121,117.172401030101));
#51900=CARTESIAN_POINT('Ctrl Pts',(6.71192421772876,-4.18736125686167,117.180296155592));
#51901=CARTESIAN_POINT('Ctrl Pts',(6.81578703046658,-4.02087948340731,117.188186195872));
#51902=CARTESIAN_POINT('Ctrl Pts',(6.91352098273932,-3.85042065370394,117.196076236153));
#51903=CARTESIAN_POINT('Ctrl Pts',(7.00481478545324,-3.6764780458335,117.203966276433));
#51904=CARTESIAN_POINT('Ctrl Pts',(7.09606669071054,-3.50261526542835,117.211852695739));
#51905=CARTESIAN_POINT('Ctrl Pts',(7.18088417621274,-3.32527219735225,117.219739115044));
#51906=CARTESIAN_POINT('Ctrl Pts',(7.25900099785885,-3.14496828490913,117.227625534349));
#51907=CARTESIAN_POINT('Ctrl Pts',(7.33709643176276,-2.96471373819178,117.235509794417));
#51908=CARTESIAN_POINT('Ctrl Pts',(7.40849472158182,-2.78150027876586,117.243394054486));
#51909=CARTESIAN_POINT('Ctrl Pts',(7.47297691391634,-2.59586922707469,117.251278314554));
#51910=CARTESIAN_POINT('Ctrl Pts',(7.53746663451241,-2.4102165030573,117.259163495106));
#51911=CARTESIAN_POINT('Ctrl Pts',(7.595038524639,-2.22214594611724,117.267048675658));
#51912=CARTESIAN_POINT('Ctrl Pts',(7.64552265158189,-2.03221661841157,117.27493385621));
#51913=CARTESIAN_POINT('Ctrl Pts',(7.69601307538542,-1.84226360091309,117.282820020276));
#51914=CARTESIAN_POINT('Ctrl Pts',(7.73941388514382,-1.65045168374889,117.290706184342));
#51915=CARTESIAN_POINT('Ctrl Pts',(7.77560569765339,-1.45735274886356,117.298592348409));
#51916=CARTESIAN_POINT('Ctrl Pts',(7.81180809670744,-1.26419733019577,117.306480819274));
#51917=CARTESIAN_POINT('Ctrl Pts',(7.84079723278438,-1.06975448237004,117.314369290139));
#51918=CARTESIAN_POINT('Ctrl Pts',(7.86250523807596,-0.874604128293515,
117.322257761004));
#51919=CARTESIAN_POINT('Ctrl Pts',(7.8842232355301,-0.67936394679919,117.330149862921));
#51920=CARTESIAN_POINT('Ctrl Pts',(7.89865338549164,-0.483415952306765,
117.338041964837));
#51921=CARTESIAN_POINT('Ctrl Pts',(7.90577983826125,-0.287343259781535,
117.345934066754));
#51922=CARTESIAN_POINT('Ctrl Pts',(7.91291455273971,-0.0910432598497572,
117.353835317998));
#51923=CARTESIAN_POINT('Ctrl Pts',(7.9127286447279,0.105381382380236,117.361736569241));
#51924=CARTESIAN_POINT('Ctrl Pts',(7.90525838900726,0.301348308490955,117.369637820485));
#51925=CARTESIAN_POINT('Ctrl Pts',(7.89778318327669,0.497445088018359,117.377544307329));
#51926=CARTESIAN_POINT('Ctrl Pts',(7.88301403312867,0.693083204222326,117.385450794173));
#51927=CARTESIAN_POINT('Ctrl Pts',(7.86103890394467,0.887687079250537,117.393357281017));
#51928=CARTESIAN_POINT('Ctrl Pts',(7.83903350037349,1.08255905341074,117.401274660359));
#51929=CARTESIAN_POINT('Ctrl Pts',(7.80980233968711,1.27639360083801,117.4091920397));
#51930=CARTESIAN_POINT('Ctrl Pts',(7.77348437248839,1.46862578987253,117.417109419042));
#51931=CARTESIAN_POINT('Ctrl Pts',(7.75773728877846,1.55197561933596,117.420542310386));
#51932=CARTESIAN_POINT('Ctrl Pts',(7.7406585225722,1.63502440123127,117.423975201731));
#51933=CARTESIAN_POINT('Ctrl Pts',(7.72226227625815,1.7177270844579,117.427408093076));
#51934=CARTESIAN_POINT('Ctrl Pts',(7.68024041157919,1.90664176323575,117.435249719736));
#51935=CARTESIAN_POINT('Ctrl Pts',(7.6312158607668,2.0943110598549,117.443091346397));
#51936=CARTESIAN_POINT('Ctrl Pts',(7.57527194338821,2.28017016551734,117.450932973057));
#51937=CARTESIAN_POINT('Ctrl Pts',(7.5193938957573,2.46581043608624,117.458765366793));
#51938=CARTESIAN_POINT('Ctrl Pts',(7.45661280379767,2.6496444266374,117.466597760528));
#51939=CARTESIAN_POINT('Ctrl Pts',(7.38706321502987,2.83111604445183,117.474430154264));
#51940=CARTESIAN_POINT('Ctrl Pts',(7.31758197658512,3.01240931982136,117.482254850663));
#51941=CARTESIAN_POINT('Ctrl Pts',(7.24134561259178,3.1913445199734,117.490079547061));
#51942=CARTESIAN_POINT('Ctrl Pts',(7.15853888810705,3.36737909767508,117.49790424346));
#51943=CARTESIAN_POINT('Ctrl Pts',(7.07579743236562,3.54327492389571,117.505722772387));
#51944=CARTESIAN_POINT('Ctrl Pts',(6.9864960795171,3.71627436457766,117.513541301314));
#51945=CARTESIAN_POINT('Ctrl Pts',(6.89086833891235,3.88585312843593,117.521359830241));
#51946=CARTESIAN_POINT('Ctrl Pts',(6.79529737586998,4.05533120740108,117.529173717032));
#51947=CARTESIAN_POINT('Ctrl Pts',(6.69340767955163,4.22139234974059,117.536987603822));
#51948=CARTESIAN_POINT('Ctrl Pts',(6.58547958136801,4.38353506697334,117.544801490613));
#51949=CARTESIAN_POINT('Ctrl Pts',(6.47759458091849,4.54561303754762,117.552612257171));
#51950=CARTESIAN_POINT('Ctrl Pts',(6.3636761772956,4.70377540810573,117.560423023729));
#51951=CARTESIAN_POINT('Ctrl Pts',(6.24404917087586,4.85754783318543,117.568233790286));
#51952=CARTESIAN_POINT('Ctrl Pts',(6.12442691904792,5.01131414655898,117.576044246404));
#51953=CARTESIAN_POINT('Ctrl Pts',(5.99909672521037,5.16069057892542,117.583854702522));
#51954=CARTESIAN_POINT('Ctrl Pts',(5.86842528199299,5.30523380348741,117.59166515864));
#51955=CARTESIAN_POINT('Ctrl Pts',(5.73775023511026,5.44978101427163,117.599475830154));
#51956=CARTESIAN_POINT('Ctrl Pts',(5.60173388087419,5.58949449009391,117.607286501669));
#51957=CARTESIAN_POINT('Ctrl Pts',(5.46078154693117,5.72396592378885,117.615097173184));
#51958=CARTESIAN_POINT('Ctrl Pts',(5.31980050208339,5.8584647482791,117.622909435673));
#51959=CARTESIAN_POINT('Ctrl Pts',(5.17388172929063,5.98771916065832,117.630721698162));
#51960=CARTESIAN_POINT('Ctrl Pts',(5.02346567593081,6.11135939073665,117.63853396065));
#51961=CARTESIAN_POINT('Ctrl Pts',(4.87299249162997,6.23504658177781,117.646349190388));
#51962=CARTESIAN_POINT('Ctrl Pts',(4.71801889584076,6.35311511969274,117.654164420126));
#51963=CARTESIAN_POINT('Ctrl Pts',(4.55901661309642,6.46523692694327,117.661979649864));
#51964=CARTESIAN_POINT('Ctrl Pts',(4.39984140765079,6.57748067210216,117.669803379043));
#51965=CARTESIAN_POINT('Ctrl Pts',(4.23662905198565,6.68376456656124,117.677627108223));
#51966=CARTESIAN_POINT('Ctrl Pts',(4.06987921745359,6.78380454872775,117.685450837402));
#51967=CARTESIAN_POINT('Ctrl Pts',(3.90302821186046,6.88390522751309,117.693279313423));
#51968=CARTESIAN_POINT('Ctrl Pts',(3.73263575734608,6.97775427500677,117.701107789443));
#51969=CARTESIAN_POINT('Ctrl Pts',(3.55922413682134,7.06511461647073,117.708936265464));
#51970=CARTESIAN_POINT('Ctrl Pts',(3.38557385330543,7.15259519024866,117.716775515662));
#51971=CARTESIAN_POINT('Ctrl Pts',(3.2088964231017,7.23356907501793,117.72461476586));
#51972=CARTESIAN_POINT('Ctrl Pts',(3.02973309200395,7.30784772632929,117.732454016057));
#51973=CARTESIAN_POINT('Ctrl Pts',(2.92928282100942,7.34949302622195,117.736849194479));
#51974=CARTESIAN_POINT('Ctrl Pts',(2.82805139765376,7.3890346249793,117.7412443729));
#51975=CARTESIAN_POINT('Ctrl Pts',(2.72613590948133,7.42644625665845,117.745639551322));
#51976=CARTESIAN_POINT('Ctrl Pts',(2.54272135429595,7.49377496111977,117.75354943538));
#51977=CARTESIAN_POINT('Ctrl Pts',(2.3565634426319,7.55439570016004,117.761459319437));
#51978=CARTESIAN_POINT('Ctrl Pts',(2.16819453330328,7.60807817163794,117.769369203495));
#51979=CARTESIAN_POINT('Ctrl Pts',(1.98003041256838,7.66170228126686,117.777270488182));
#51980=CARTESIAN_POINT('Ctrl Pts',(1.78966041073773,7.70840305418294,117.78517177287));
#51981=CARTESIAN_POINT('Ctrl Pts',(1.59763634808956,7.74799839308599,117.793073057557));
#51982=CARTESIAN_POINT('Ctrl Pts',(1.40578536510107,7.78755804298378,117.800967220472));
#51983=CARTESIAN_POINT('Ctrl Pts',(1.2122836269496,7.82002494774707,117.808861383387));
#51984=CARTESIAN_POINT('Ctrl Pts',(1.01769785785694,7.84526685780117,117.816755546302));
#51985=CARTESIAN_POINT('Ctrl Pts',(0.823251329979141,7.87049070531021,117.824644060331));
#51986=CARTESIAN_POINT('Ctrl Pts',(0.627722657320462,7.88849981433292,117.83253257436));
#51987=CARTESIAN_POINT('Ctrl Pts',(0.431688774556004,7.89921298623618,117.840421088389));
#51988=CARTESIAN_POINT('Ctrl Pts',(0.235758760990982,7.90992048172997,117.848305422662));
#51989=CARTESIAN_POINT('Ctrl Pts',(0.039324414345863,7.91333972434937,117.856189756936));
#51990=CARTESIAN_POINT('Ctrl Pts',(-0.157031907085009,7.90944131909184,
117.86407409121));
#51991=CARTESIAN_POINT('Ctrl Pts',(-0.3533206506534,7.9055442555069,117.871955712016));
#51992=CARTESIAN_POINT('Ctrl Pts',(-0.549531078044028,7.89433457017896,
117.879837332823));
#51993=CARTESIAN_POINT('Ctrl Pts',(-0.745080244104152,7.875834967154,117.887718953629));
#51994=CARTESIAN_POINT('Ctrl Pts',(-0.940631971342325,7.85733512183306,
117.895600677664));
#51995=CARTESIAN_POINT('Ctrl Pts',(-1.13552207573532,7.83154519200619,117.903482401699));
#51996=CARTESIAN_POINT('Ctrl Pts',(-1.32917157076089,7.79853985919679,117.911364125734));
#51997=CARTESIAN_POINT('Ctrl Pts',(-1.52283273126742,7.7655325381401,117.919246324565));
#51998=CARTESIAN_POINT('Ctrl Pts',(-1.71525279311446,7.7253090053851,117.927128523397));
#51999=CARTESIAN_POINT('Ctrl Pts',(-1.90586178166159,7.67799530275981,117.935010722228));
#52000=CARTESIAN_POINT('Ctrl Pts',(-2.09651432636319,7.63067078845688,117.942894722225));
#52001=CARTESIAN_POINT('Ctrl Pts',(-2.2853546381759,7.5762529589668,117.950778722221));
#52002=CARTESIAN_POINT('Ctrl Pts',(-2.47182651465308,7.51491814203308,117.958662722218));
#52003=CARTESIAN_POINT('Ctrl Pts',(-2.65837238000031,7.45355898848688,117.966549850451));
#52004=CARTESIAN_POINT('Ctrl Pts',(-2.84254760993641,7.38527748649901,117.974436978685));
#52005=CARTESIAN_POINT('Ctrl Pts',(-3.02381440883524,7.31029872309746,117.982324106919));
#52006=CARTESIAN_POINT('Ctrl Pts',(-3.20527459870139,7.23523996592061,117.990219649817));
#52007=CARTESIAN_POINT('Ctrl Pts',(-3.38381984063555,7.15346980724472,117.998115192716));
#52008=CARTESIAN_POINT('Ctrl Pts',(-3.558934442781,7.06526054947637,118.006010735614));
#52009=CARTESIAN_POINT('Ctrl Pts',(-3.73415568365131,6.97699757532655,118.013911086625));
#52010=CARTESIAN_POINT('Ctrl Pts',(-3.90594181839956,6.88228785083727,118.021811437636));
#52011=CARTESIAN_POINT('Ctrl Pts',(-4.07380451921806,6.78144805621915,118.029711788646));
#52012=CARTESIAN_POINT('Ctrl Pts',(-4.24188578433035,6.68047696394891,118.037622426246));
#52013=CARTESIAN_POINT('Ctrl Pts',(-4.40603312355957,6.5733600467252,118.045533063846));
#52014=CARTESIAN_POINT('Ctrl Pts',(-4.56578884836695,6.46045611331955,118.053443701445));
#52015=CARTESIAN_POINT('Ctrl Pts',(-4.63598218597049,6.41084847688671,118.05691947082));
#52016=CARTESIAN_POINT('Ctrl Pts',(-4.7053281509237,6.36012414408697,118.060395240194));
#52017=CARTESIAN_POINT('Ctrl Pts',(-4.77379010025081,6.30831586707161,118.063871009569));
#52018=CARTESIAN_POINT('Ctrl Pts',(-4.92785616684936,6.19172705335163,118.071692845219));
#52019=CARTESIAN_POINT('Ctrl Pts',(-5.07788000157877,6.06931558110785,118.07951468087));
#52020=CARTESIAN_POINT('Ctrl Pts',(-5.22338588974355,5.94139384713958,118.08733651652));
#52021=CARTESIAN_POINT('Ctrl Pts',(-5.3687326525521,5.81361200848237,118.095149798205));
#52022=CARTESIAN_POINT('Ctrl Pts',(-5.50957104373117,5.68033213790914,118.102963079889));
#52023=CARTESIAN_POINT('Ctrl Pts',(-5.64545491891002,5.54190939645847,118.110776361574));
#52024=CARTESIAN_POINT('Ctrl Pts',(-5.78121693991536,5.40361078591541,118.118582636681));
#52025=CARTESIAN_POINT('Ctrl Pts',(-5.91203304661729,5.2601787392757,118.126388911787));
#52026=CARTESIAN_POINT('Ctrl Pts',(-6.03749063183514,5.11200820328987,118.134195186894));
#52027=CARTESIAN_POINT('Ctrl Pts',(-6.16286039290777,4.96394139120919,118.141995997369));
#52028=CARTESIAN_POINT('Ctrl Pts',(-6.282878876065,4.81114296519533,118.149796807844));
#52029=CARTESIAN_POINT('Ctrl Pts',(-6.39717067080784,4.65404430668167,118.15759761832));
#52030=CARTESIAN_POINT('Ctrl Pts',(-6.51140493154762,4.49702473096408,118.1653945019));
#52031=CARTESIAN_POINT('Ctrl Pts',(-6.61991803901518,4.33570952033906,118.173191385481));
#52032=CARTESIAN_POINT('Ctrl Pts',(-6.72237509636622,4.17056279940193,118.180988269061));
#52033=CARTESIAN_POINT('Ctrl Pts',(-6.82481259867789,4.00544759850562,118.188783664522));
#52034=CARTESIAN_POINT('Ctrl Pts',(-6.921196162118,3.83650264120311,118.196579059983));
#52035=CARTESIAN_POINT('Ctrl Pts',(-7.01123424735637,3.6642209715978,118.204374455444));
#52036=CARTESIAN_POINT('Ctrl Pts',(-7.10126646972894,3.49195052018206,118.212169343304));
#52037=CARTESIAN_POINT('Ctrl Pts',(-7.18495387231422,3.31634410237102,118.219964231165));
#52038=CARTESIAN_POINT('Ctrl Pts',(-7.26205090181683,3.13791932646799,118.227759119025));
#52039=CARTESIAN_POINT('Ctrl Pts',(-7.33915663979812,2.9594743966321,118.235554887356));
#52040=CARTESIAN_POINT('Ctrl Pts',(-7.40967038173992,2.77821079944886,118.243350655686));
#52041=CARTESIAN_POINT('Ctrl Pts',(-7.47339470106483,2.59466619088009,118.251146424017));
#52042=CARTESIAN_POINT('Ctrl Pts',(-7.5371375666491,2.41106816368006,118.258944461219));
#52043=CARTESIAN_POINT('Ctrl Pts',(-7.59408695844901,2.22518813702575,118.266742498422));
#52044=CARTESIAN_POINT('Ctrl Pts',(-7.64409526188591,2.03757910943684,118.274540535625));
#52045=CARTESIAN_POINT('Ctrl Pts',(-7.69415138836612,1.84979067094942,118.282346030106));
#52046=CARTESIAN_POINT('Ctrl Pts',(-7.73725307824949,1.66027027122004,118.290151524588));
#52047=CARTESIAN_POINT('Ctrl Pts',(-7.77330361370663,1.46958222945686,118.29795701907));
#52048=CARTESIAN_POINT('Ctrl Pts',(-7.80937339613195,1.27879238153119,118.305766680816));
#52049=CARTESIAN_POINT('Ctrl Pts',(-7.83838446918683,1.08683399817102,118.313576342562));
#52050=CARTESIAN_POINT('Ctrl Pts',(-7.8602919833563,0.894276767217355,118.321386004308));
#52051=CARTESIAN_POINT('Ctrl Pts',(-7.88222718161888,0.701476205492797,
118.329205534969));
#52052=CARTESIAN_POINT('Ctrl Pts',(-7.89704086536167,0.508075636413814,
118.33702506563));
#52053=CARTESIAN_POINT('Ctrl Pts',(-7.90474027759045,0.31464606121696,118.344844596291));
#52054=CARTESIAN_POINT('Ctrl Pts',(-7.90894924536154,0.208905671718469,
118.349119228115));
#52055=CARTESIAN_POINT('Ctrl Pts',(-7.91103310971454,0.103156567800752,
118.353393859939));
#52056=CARTESIAN_POINT('Ctrl Pts',(-7.91099960224048,-0.00250865522661604,
118.357668491763));
#52057=CARTESIAN_POINT('',(-7.9122673030836,0.00701237838125787,120.357668491763));
#52058=CARTESIAN_POINT('Ctrl Pts',(-7.92290232931793,-0.00251242969760849,
118.357668491763));
#52059=CARTESIAN_POINT('Ctrl Pts',(-7.92403808898173,-0.204144684807022,
118.365813150447));
#52060=CARTESIAN_POINT('Ctrl Pts',(-7.91699393318657,-0.405710916029759,
118.373957809132));
#52061=CARTESIAN_POINT('Ctrl Pts',(-7.69988300863637,-3.2236589545846,118.488179620565));
#52062=CARTESIAN_POINT('Ctrl Pts',(-4.43429229470843,-8.24372861963162,
118.700333926063));
#52063=CARTESIAN_POINT('Ctrl Pts',(3.02895942017901,-8.18612541628597,118.965526807936));
#52064=CARTESIAN_POINT('Ctrl Pts',(6.94408330637767,-4.40646303786943,119.177681113432));
#52065=CARTESIAN_POINT('Ctrl Pts',(8.69663683459128,0.745487939167516,119.389835418932));
#52066=CARTESIAN_POINT('Ctrl Pts',(5.57052227007294,7.52271834829018,119.655028300802));
#52067=CARTESIAN_POINT('Ctrl Pts',(-3.32864853973696,8.74804228169172,119.973259759051));
#52068=CARTESIAN_POINT('Ctrl Pts',(-7.61439352537567,3.73049070384629,120.207473156037));
#52069=CARTESIAN_POINT('Ctrl Pts',(-7.91716285885491,0.554684267022833,
120.335609400274));
#52070=CARTESIAN_POINT('Ctrl Pts',(-7.9122673030836,0.00701237838125787,
120.357668491763));
#52071=CARTESIAN_POINT('',(-7.90352584329644,7.42828143361043E-5,122.357668491763));
#52072=CARTESIAN_POINT('Ctrl Pts',(-7.9122673030836,0.00701237838125787,
120.357668491763));
#52073=CARTESIAN_POINT('Ctrl Pts',(-7.89362124484021,-2.07894525562691,
120.441686553023));
#52074=CARTESIAN_POINT('Ctrl Pts',(-5.97996265754411,-6.82958157585722,
120.631781767032));
#52075=CARTESIAN_POINT('Ctrl Pts',(2.05724953842661,-9.13179796347452,120.92795413379));
#52076=CARTESIAN_POINT('Ctrl Pts',(7.65449062796197,-4.19476074725102,121.193147015663));
#52077=CARTESIAN_POINT('Ctrl Pts',(8.13227400217734,1.22610318632951,121.40530132116));
#52078=CARTESIAN_POINT('Ctrl Pts',(6.07745315432454,6.26512630816728,121.61745562666));
#52079=CARTESIAN_POINT('Ctrl Pts',(-0.726601117103637,9.33241986440786,
121.88264850853));
#52080=CARTESIAN_POINT('Ctrl Pts',(-6.97710178777028,5.25280976497826,122.147065655691));
#52081=CARTESIAN_POINT('Ctrl Pts',(-7.89925698168475,1.30374424487291,122.305405650101));
#52082=CARTESIAN_POINT('Ctrl Pts',(-7.89821528668816,0.000127062427985106,
122.357668491763));
#52083=CARTESIAN_POINT('',(-7.911,-2.20379270388094E-12,124.357668491763));
#52084=CARTESIAN_POINT('Ctrl Pts',(-7.911,-2.37476704967321E-12,122.357668491763));
#52085=CARTESIAN_POINT('Ctrl Pts',(-7.91099999999934,-2.20167589666902,
122.446255927496));
#52086=CARTESIAN_POINT('Ctrl Pts',(-6.94214576672251,-4.38610418338868,
122.534843363229));
#52087=CARTESIAN_POINT('Ctrl Pts',(-3.67820201488108,-7.34180684107718,
122.712018234694));
#52088=CARTESIAN_POINT('Ctrl Pts',(-1.40868175871563,-8.08992666571365,
122.800605670427));
#52089=CARTESIAN_POINT('Ctrl Pts',(2.97309270521422,-7.65454228025196,122.977780541892));
#52090=CARTESIAN_POINT('Ctrl Pts',(5.05102072675715,-6.47444880834133,123.066367977625));
#52091=CARTESIAN_POINT('Ctrl Pts',(7.66951518847912,-2.93425195367592,123.24354284909));
#52092=CARTESIAN_POINT('Ctrl Pts',(8.18956872247076,-0.601881960098094,
123.332130284823));
#52093=CARTESIAN_POINT('Ctrl Pts',(7.32306689761302,3.71537198232523,123.509305156288));
#52094=CARTESIAN_POINT('Ctrl Pts',(5.94329958850151,5.66643518936559,123.597892592021));
#52095=CARTESIAN_POINT('Ctrl Pts',(2.16154501637802,7.92205913233007,123.775067463487));
#52096=CARTESIAN_POINT('Ctrl Pts',(-0.210816529300683,8.20894963712998,
123.863654899219));
#52097=CARTESIAN_POINT('Ctrl Pts',(-4.42123908576442,6.91982244717824,124.040829770685));
#52098=CARTESIAN_POINT('Ctrl Pts',(-6.22631625634181,5.35390358803523,124.129417206418));
#52099=CARTESIAN_POINT('Ctrl Pts',(-7.65317280859517,2.31334857514464,124.264559258688));
#52100=CARTESIAN_POINT('Ctrl Pts',(-7.91100000000032,1.15702837836378,124.311113875226));
#52101=CARTESIAN_POINT('Ctrl Pts',(-7.911,-2.20379270388094E-12,124.357668491763));
#52102=CARTESIAN_POINT('',(-7.91840974246489,0.00164577101414091,126.357721590925));
#52103=CARTESIAN_POINT('Ctrl Pts',(-7.911,-2.20379270388094E-12,124.357668491763));
#52104=CARTESIAN_POINT('Ctrl Pts',(-7.91099999999939,-2.20167589666915,
124.446255927496));
#52105=CARTESIAN_POINT('Ctrl Pts',(-6.94214576672232,-4.38610418338912,
124.534843363229));
#52106=CARTESIAN_POINT('Ctrl Pts',(-3.67820201488018,-7.34180684107772,
124.712018234694));
#52107=CARTESIAN_POINT('Ctrl Pts',(-1.40868175871426,-8.08992666571397,
124.800605670427));
#52108=CARTESIAN_POINT('Ctrl Pts',(2.97309270521609,-7.65454228025132,124.977780541892));
#52109=CARTESIAN_POINT('Ctrl Pts',(5.05102072675904,-6.47444880833996,125.066367977625));
#52110=CARTESIAN_POINT('Ctrl Pts',(7.66951518848024,-2.93425195367323,125.24354284909));
#52111=CARTESIAN_POINT('Ctrl Pts',(8.18956872247108,-0.60188196009484,125.332130284823));
#52112=CARTESIAN_POINT('Ctrl Pts',(7.32306689761135,3.7153719823287,125.509305156289));
#52113=CARTESIAN_POINT('Ctrl Pts',(5.94329958849867,5.66643518936869,125.597892592021));
#52114=CARTESIAN_POINT('Ctrl Pts',(2.16154501637343,7.9220591323314,125.775067463487));
#52115=CARTESIAN_POINT('Ctrl Pts',(-0.210816529305819,8.20894963712993,
125.86365489922));
#52116=CARTESIAN_POINT('Ctrl Pts',(-4.42123908576928,6.91982244717523,126.040829770685));
#52117=CARTESIAN_POINT('Ctrl Pts',(-6.22631625634583,5.35390358803068,126.129417206418));
#52118=CARTESIAN_POINT('Ctrl Pts',(-7.65293518925909,2.31385492924122,126.264536753016));
#52119=CARTESIAN_POINT('Ctrl Pts',(-7.91075066509672,1.15814634139517,126.311068863883));
#52120=CARTESIAN_POINT('Ctrl Pts',(-7.9109998192402,0.00167800926889546,
126.357600974748));
#52121=CARTESIAN_POINT('',(-7.90392088591637,0.0024881653853563,128.357668491763));
#52122=CARTESIAN_POINT('Ctrl Pts',(-7.92352486655139,0.00162351671157913,
126.357804853153));
#52123=CARTESIAN_POINT('Ctrl Pts',(-7.91094766732972,-2.45855671784116,
126.457243362846));
#52124=CARTESIAN_POINT('Ctrl Pts',(-5.34962893444157,-7.57264949493443,
126.662759025289));
#52125=CARTESIAN_POINT('Ctrl Pts',(3.35234681176765,-8.73179419511677,126.97435184048));
#52126=CARTESIAN_POINT('Ctrl Pts',(9.16409439033137,-1.90460464885401,127.292583298727));
#52127=CARTESIAN_POINT('Ctrl Pts',(6.54805283706349,6.68917138008194,127.610814756974));
#52128=CARTESIAN_POINT('Ctrl Pts',(-0.637984975502353,8.70518349440442,
127.876007638845));
#52129=CARTESIAN_POINT('Ctrl Pts',(-5.4483076350138,6.16061306886672,128.088161944344));
#52130=CARTESIAN_POINT('Ctrl Pts',(-7.54512756758505,3.15493213566288,128.231036036525));
#52131=CARTESIAN_POINT('Ctrl Pts',(-7.90452149261816,0.920835889764306,
128.320871552331));
#52132=CARTESIAN_POINT('Ctrl Pts',(-7.89890066374168,0.00425267191875162,
128.357668491763));
#52133=CARTESIAN_POINT('',(-7.9109995580894,-0.00186974719043329,130.357668491763));
#52134=CARTESIAN_POINT('Ctrl Pts',(-7.911,-1.86295423532101E-12,128.357668491763));
#52135=CARTESIAN_POINT('Ctrl Pts',(-7.91099999999948,-2.20167589666851,
128.446255927496));
#52136=CARTESIAN_POINT('Ctrl Pts',(-6.94214576672279,-4.38610418338823,
128.534843363229));
#52137=CARTESIAN_POINT('Ctrl Pts',(-3.67820201488156,-7.34180684107694,
128.712018234694));
#52138=CARTESIAN_POINT('Ctrl Pts',(-1.40868175871615,-8.08992666571356,
128.800605670427));
#52139=CARTESIAN_POINT('Ctrl Pts',(2.97309270521372,-7.65454228025215,128.977780541892));
#52140=CARTESIAN_POINT('Ctrl Pts',(5.05102072675673,-6.47444880834166,129.066367977625));
#52141=CARTESIAN_POINT('Ctrl Pts',(7.66951518847893,-2.93425195367641,129.24354284909));
#52142=CARTESIAN_POINT('Ctrl Pts',(8.18956872247072,-0.601881960098624,
129.332130284823));
#52143=CARTESIAN_POINT('Ctrl Pts',(7.32306689761326,3.71537198232476,129.509305156288));
#52144=CARTESIAN_POINT('Ctrl Pts',(5.94329958850188,5.6664351893652,129.597892592021));
#52145=CARTESIAN_POINT('Ctrl Pts',(2.16154501637854,7.92205913232993,129.775067463487));
#52146=CARTESIAN_POINT('Ctrl Pts',(-0.210816529300152,8.20894963713,129.863654899219));
#52147=CARTESIAN_POINT('Ctrl Pts',(-4.42123908576398,6.91982244717853,130.040829770685));
#52148=CARTESIAN_POINT('Ctrl Pts',(-6.22631625634147,5.35390358803564,130.129417206418));
#52149=CARTESIAN_POINT('Ctrl Pts',(-7.65317280859502,2.31334857514513,130.264559258688));
#52150=CARTESIAN_POINT('Ctrl Pts',(-7.91100000000025,1.15702837836429,130.311113875225));
#52151=CARTESIAN_POINT('Ctrl Pts',(-7.911,-1.69197988952874E-12,130.357668491763));
#52152=CARTESIAN_POINT('',(-7.91099991273041,-0.00117506573469943,132.357550177074));
#52153=CARTESIAN_POINT('Ctrl Pts',(-7.9109991161788,-0.00373949437917459,
130.357668491763));
#52154=CARTESIAN_POINT('Ctrl Pts',(-7.91089584571042,-0.222210897528256,
130.366434366415));
#52155=CARTESIAN_POINT('Ctrl Pts',(-7.90173845183842,-0.440413092802176,
130.375200241067));
#52156=CARTESIAN_POINT('Ctrl Pts',(-7.88361836605496,-0.657633985132213,
130.38396611572));
#52157=CARTESIAN_POINT('Ctrl Pts',(-7.86541916559622,-0.875803292418298,
130.392770263332));
#52158=CARTESIAN_POINT('Ctrl Pts',(-7.83817890181611,-1.0929825126435,130.401574410945));
#52159=CARTESIAN_POINT('Ctrl Pts',(-7.80204093071744,-1.30846410551064,
130.410378558558));
#52160=CARTESIAN_POINT('Ctrl Pts',(-7.76582530704639,-1.52440872105108,
130.419201624352));
#52161=CARTESIAN_POINT('Ctrl Pts',(-7.72067378382519,-1.7386482197866,130.428024690147));
#52162=CARTESIAN_POINT('Ctrl Pts',(-7.66678030483148,-1.95048731281392,
130.436847755941));
#52163=CARTESIAN_POINT('Ctrl Pts',(-7.6127392364279,-2.16290653552136,130.445694984048));
#52164=CARTESIAN_POINT('Ctrl Pts',(-7.54990835301261,-2.37291200415262,
130.454542212155));
#52165=CARTESIAN_POINT('Ctrl Pts',(-7.47853177456327,-2.57982237699567,
130.463389440262));
#52166=CARTESIAN_POINT('Ctrl Pts',(-7.4475829799364,-2.66953845437577,130.46722558724));
#52167=CARTESIAN_POINT('Ctrl Pts',(-7.41502813651028,-2.75867289557034,
130.471061734217));
#52168=CARTESIAN_POINT('Ctrl Pts',(-7.38088990741013,-2.84717143401856,
130.474897881195));
#52169=CARTESIAN_POINT('Ctrl Pts',(-7.31050072308688,-3.02964545506092,
130.4828075843));
#52170=CARTESIAN_POINT('Ctrl Pts',(-7.23325150427447,-3.20973885994879,
130.490717287405));
#52171=CARTESIAN_POINT('Ctrl Pts',(-7.14932378069951,-3.38689983299247,
130.498626990509));
#52172=CARTESIAN_POINT('Ctrl Pts',(-7.065481205891,-3.56388106759366,130.506528668835));
#52173=CARTESIAN_POINT('Ctrl Pts',(-6.97497376930275,-3.73793548763144,
130.51443034716));
#52174=CARTESIAN_POINT('Ctrl Pts',(-6.87803195930351,-3.90852879825639,
130.522332025486));
#52175=CARTESIAN_POINT('Ctrl Pts',(-6.78117054281328,-4.07898063643663,
130.530227150976));
#52176=CARTESIAN_POINT('Ctrl Pts',(-6.67788555241016,-4.24597678534226,
130.538122276467));
#52177=CARTESIAN_POINT('Ctrl Pts',(-6.56845463156288,-4.40900496179128,
130.546017401958));
#52178=CARTESIAN_POINT('Ctrl Pts',(-6.45909419461557,-4.57192813262039,
130.553907442239));
#52179=CARTESIAN_POINT('Ctrl Pts',(-6.34359590571145,-4.73088813800196,
130.561797482519));
#52180=CARTESIAN_POINT('Ctrl Pts',(-6.22228234214997,-4.8853990066901,130.5696875228));
#52181=CARTESIAN_POINT('Ctrl Pts',(-6.10102445301144,-5.03983896571901,
130.577573942105));
#52182=CARTESIAN_POINT('Ctrl Pts',(-5.97395681976943,-5.18983358636831,
130.58546036141));
#52183=CARTESIAN_POINT('Ctrl Pts',(-5.84144433471934,-5.33492728013938,
130.593346780715));
#52184=CARTESIAN_POINT('Ctrl Pts',(-5.70896813049634,-5.47998124845201,
130.601231040784));
#52185=CARTESIAN_POINT('Ctrl Pts',(-5.57105027794571,-5.62013671017715,
130.609115300852));
#52186=CARTESIAN_POINT('Ctrl Pts',(-5.42809499169923,-5.754972264146,130.616999560921));
#52187=CARTESIAN_POINT('Ctrl Pts',(-5.28512301549902,-5.88982356009414,
130.624884741472));
#52188=CARTESIAN_POINT('Ctrl Pts',(-5.13711267647559,-6.01935346576271,
130.632769922024));
#52189=CARTESIAN_POINT('Ctrl Pts',(-4.9845044470491,-6.14317803887758,130.640655102576));
#52190=CARTESIAN_POINT('Ctrl Pts',(-4.83187718287227,-6.26701805657131,
130.648541266642));
#52191=CARTESIAN_POINT('Ctrl Pts',(-4.67465115286065,-6.38515110588662,
130.656427430708));
#52192=CARTESIAN_POINT('Ctrl Pts',(-4.51329922275996,-6.49723411351587,
130.664313594775));
#52193=CARTESIAN_POINT('Ctrl Pts',(-4.35190009526084,-6.60934990678559,
130.67220206564));
#52194=CARTESIAN_POINT('Ctrl Pts',(-4.1863729457104,-6.71541193506504,130.680090536505));
#52195=CARTESIAN_POINT('Ctrl Pts',(-4.01721906877824,-6.81512083190346,
130.68797900737));
#52196=CARTESIAN_POINT('Ctrl Pts',(-3.84798733056831,-6.91487562459868,
130.695871109287));
#52197=CARTESIAN_POINT('Ctrl Pts',(-3.67512583497725,-7.00827128357385,
130.703763211203));
#52198=CARTESIAN_POINT('Ctrl Pts',(-3.49916008761638,-7.09505459325244,
130.71165531312));
#52199=CARTESIAN_POINT('Ctrl Pts',(-3.32299034286489,-7.18193851096975,
130.719556564363));
#52200=CARTESIAN_POINT('Ctrl Pts',(-3.14370946715935,-7.26219461505559,
130.727457815607));
#52201=CARTESIAN_POINT('Ctrl Pts',(-2.96186361816154,-7.33561755460377,
130.735359066851));
#52202=CARTESIAN_POINT('Ctrl Pts',(-2.7798972727856,-7.40908914633916,130.743265553695));
#52203=CARTESIAN_POINT('Ctrl Pts',(-2.59536288892839,-7.47571843030834,
130.751172040539));
#52204=CARTESIAN_POINT('Ctrl Pts',(-2.40882160273842,-7.53534999095468,
130.759078527382));
#52205=CARTESIAN_POINT('Ctrl Pts',(-2.22202332497055,-7.59506370397155,
130.766995906724));
#52206=CARTESIAN_POINT('Ctrl Pts',(-2.03321295306132,-7.64776034514328,
130.774913286066));
#52207=CARTESIAN_POINT('Ctrl Pts',(-1.84296278608913,-7.69333537349637,
130.782830665407));
#52208=CARTESIAN_POINT('Ctrl Pts',(-1.76047234027415,-7.71309622031564,
130.786263556752));
#52209=CARTESIAN_POINT('Ctrl Pts',(-1.67771129521446,-7.73151886537192,
130.789696448097));
#52210=CARTESIAN_POINT('Ctrl Pts',(-1.5947265676748,-7.74859781988665,130.793129339442));
#52211=CARTESIAN_POINT('Ctrl Pts',(-1.40516762552119,-7.78761064365418,
130.800970966102));
#52212=CARTESIAN_POINT('Ctrl Pts',(-1.21387764991051,-7.81972476370473,
130.808812592763));
#52213=CARTESIAN_POINT('Ctrl Pts',(-1.0214060498034,-7.84478493532009,130.816654219423));
#52214=CARTESIAN_POINT('Ctrl Pts',(-0.829161070503838,-7.86981560047151,
130.824486613159));
#52215=CARTESIAN_POINT('Ctrl Pts',(-0.635737581738321,-7.88780880983657,
130.832319006895));
#52216=CARTESIAN_POINT('Ctrl Pts',(-0.441698015690497,-7.89865962445117,
130.84015140063));
#52217=CARTESIAN_POINT('Ctrl Pts',(-0.24784914332251,-7.90949977535522,
130.847976097029));
#52218=CARTESIAN_POINT('Ctrl Pts',(-0.0533857477400354,-7.9132114901666,
130.855800793427));
#52219=CARTESIAN_POINT('Ctrl Pts',(0.141121535392811,-7.90974119123049,
130.863625489826));
#52220=CARTESIAN_POINT('Ctrl Pts',(0.335475506750435,-7.90627362760425,
130.871444018753));
#52221=CARTESIAN_POINT('Ctrl Pts',(0.529872946920586,-7.89563533112102,
130.87926254768));
#52222=CARTESIAN_POINT('Ctrl Pts',(0.723739917486823,-7.87782467003653,
130.887081076607));
#52223=CARTESIAN_POINT('Ctrl Pts',(0.91749178239512,-7.8600245837697,130.894894963398));
#52224=CARTESIAN_POINT('Ctrl Pts',(1.11071345589391,-7.83506064775668,130.902708850189));
#52225=CARTESIAN_POINT('Ctrl Pts',(1.30283263211802,-7.8029832841477,130.910522736979));
#52226=CARTESIAN_POINT('Ctrl Pts',(1.49487509151544,-7.7709187296377,130.918333503537));
#52227=CARTESIAN_POINT('Ctrl Pts',(1.68581558435728,-7.73174646473343,130.926144270095));
#52228=CARTESIAN_POINT('Ctrl Pts',(1.87508836052272,-7.6855685957665,130.933955036653));
#52229=CARTESIAN_POINT('Ctrl Pts',(2.06435361401569,-7.63939256214531,130.94176549277));
#52230=CARTESIAN_POINT('Ctrl Pts',(2.25195093909346,-7.58621155371739,130.949575948888));
#52231=CARTESIAN_POINT('Ctrl Pts',(2.43732573229109,-7.52617859705121,130.957386405006));
#52232=CARTESIAN_POINT('Ctrl Pts',(2.62270563776668,-7.46614398479229,130.965197076521));
#52233=CARTESIAN_POINT('Ctrl Pts',(2.80586255415591,-7.39925715556025,130.973007748036));
#52234=CARTESIAN_POINT('Ctrl Pts',(2.98625800853511,-7.3257207226634,130.980818419551));
#52235=CARTESIAN_POINT('Ctrl Pts',(3.16669020807862,-7.25216931096168,130.98863068204));
#52236=CARTESIAN_POINT('Ctrl Pts',(3.34435949920978,-7.17196573023374,130.996442944528));
#52237=CARTESIAN_POINT('Ctrl Pts',(3.51874818786322,-7.08536041358584,131.004255207017));
#52238=CARTESIAN_POINT('Ctrl Pts',(3.69320311273072,-6.99872220255507,131.012070436755));
#52239=CARTESIAN_POINT('Ctrl Pts',(3.8643746381874,-6.90567756858897,131.019885666492));
#52240=CARTESIAN_POINT('Ctrl Pts',(4.03177030139072,-6.80652255096711,131.02770089623));
#52241=CARTESIAN_POINT('Ctrl Pts',(4.19934801550418,-6.70725969744999,131.03552462541));
#52242=CARTESIAN_POINT('Ctrl Pts',(4.36314136278643,-6.60187336698383,131.043348354589));
#52243=CARTESIAN_POINT('Ctrl Pts',(4.52268659483622,-6.49070311791325,131.051172083769));
#52244=CARTESIAN_POINT('Ctrl Pts',(4.68232862674443,-6.37946541922833,131.059000559789));
#52245=CARTESIAN_POINT('Ctrl Pts',(4.83771712665129,-6.26243701939575,131.06682903581));
#52246=CARTESIAN_POINT('Ctrl Pts',(4.98842195556946,-6.13999734472195,131.074657511831));
#52247=CARTESIAN_POINT('Ctrl Pts',(5.13933419656986,-6.01738915873996,131.082496762028));
#52248=CARTESIAN_POINT('Ctrl Pts',(5.28554962778369,-5.88935505378018,131.090336012226));
#52249=CARTESIAN_POINT('Ctrl Pts',(5.42667462170755,-5.75631162725883,131.098175262424));
#52250=CARTESIAN_POINT('Ctrl Pts',(5.50579820016106,-5.68171908554531,131.102570440846));
#52251=CARTESIAN_POINT('Ctrl Pts',(5.58332234328611,-5.60555251584328,131.106965619267));
#52252=CARTESIAN_POINT('Ctrl Pts',(5.65918333546722,-5.52788973981665,131.111360797689));
#52253=CARTESIAN_POINT('Ctrl Pts',(5.79570831695938,-5.38812213653572,131.119270681746));
#52254=CARTESIAN_POINT('Ctrl Pts',(5.92723666008975,-5.24310511329249,131.127180565804));
#52255=CARTESIAN_POINT('Ctrl Pts',(6.05334027917667,-5.09323006200361,131.135090449862));
#52256=CARTESIAN_POINT('Ctrl Pts',(6.17930680248239,-4.94351795002915,131.142991734549));
#52257=CARTESIAN_POINT('Ctrl Pts',(6.29986012868711,-4.78895859143482,131.150893019237));
#52258=CARTESIAN_POINT('Ctrl Pts',(6.41460818253311,-4.62998087086537,131.158794303924));
#52259=CARTESIAN_POINT('Ctrl Pts',(6.52925280895531,-4.47114644384671,131.166688466839));
#52260=CARTESIAN_POINT('Ctrl Pts',(6.63810238601186,-4.3079018661502,131.174582629754));
#52261=CARTESIAN_POINT('Ctrl Pts',(6.7408042137958,-4.14071002984668,131.182476792669));
#52262=CARTESIAN_POINT('Ctrl Pts',(6.84343255045384,-3.97363783227359,131.190365306698));
#52263=CARTESIAN_POINT('Ctrl Pts',(6.9399217226487,-3.80262429629234,131.198253820727));
#52264=CARTESIAN_POINT('Ctrl Pts',(7.02996142529944,-3.62816253202662,131.206142334756));
#52265=CARTESIAN_POINT('Ctrl Pts',(7.11995342011652,-3.45379320690259,131.214026669029));
#52266=CARTESIAN_POINT('Ctrl Pts',(7.20350259688611,-3.27597959993413,131.221911003303));
#52267=CARTESIAN_POINT('Ctrl Pts',(7.2803436920171,-3.09524098029651,131.229795337577));
#52268=CARTESIAN_POINT('Ctrl Pts',(7.35715834156725,-2.91456456354353,131.237676958383));
#52269=CARTESIAN_POINT('Ctrl Pts',(7.42726937585404,-2.73096545751856,131.24555857919));
#52270=CARTESIAN_POINT('Ctrl Pts',(7.4904588226988,-2.54498479866848,131.253440199996));
#52271=CARTESIAN_POINT('Ctrl Pts',(7.55364909715867,-2.35900170396226,131.261321924031));
#52272=CARTESIAN_POINT('Ctrl Pts',(7.60991748396962,-2.17063731795321,131.269203648066));
#52273=CARTESIAN_POINT('Ctrl Pts',(7.65909505259427,-1.98045044758155,131.2770853721));
#52274=CARTESIAN_POINT('Ctrl Pts',(7.70827558368472,-1.79025212031777,131.284967570932));
#52275=CARTESIAN_POINT('Ctrl Pts',(7.7503643584307,-1.59823142396163,131.292849769763));
#52276=CARTESIAN_POINT('Ctrl Pts',(7.78524299391339,-1.40495997299656,131.300731968595));
#52277=CARTESIAN_POINT('Ctrl Pts',(7.82012959953032,-1.2116443574767,131.308615968591));
#52278=CARTESIAN_POINT('Ctrl Pts',(7.84780272151483,-1.01707775743535,131.316499968588));
#52279=CARTESIAN_POINT('Ctrl Pts',(7.86819549346673,-0.821839812001022,
131.324383968584));
#52280=CARTESIAN_POINT('Ctrl Pts',(7.88859635692385,-0.626524399469087,
131.332271096818));
#52281=CARTESIAN_POINT('Ctrl Pts',(7.90171107851393,-0.430537453695613,
131.340158225052));
#52282=CARTESIAN_POINT('Ctrl Pts',(7.90752481319848,-0.23446178505328,131.348045353285));
#52283=CARTESIAN_POINT('Ctrl Pts',(7.91334475047378,-0.0381769260717599,
131.355940896184));
#52284=CARTESIAN_POINT('Ctrl Pts',(7.91184813204109,0.158196499830445,131.363836439082));
#52285=CARTESIAN_POINT('Ctrl Pts',(7.90307223937577,0.354076516035831,131.371731981981));
#52286=CARTESIAN_POINT('Ctrl Pts',(7.89429100249589,0.550075816384149,131.379632332991));
#52287=CARTESIAN_POINT('Ctrl Pts',(7.87822168216327,0.745580765039928,131.387532684002));
#52288=CARTESIAN_POINT('Ctrl Pts',(7.85495325136521,0.940016180109228,131.395433035012));
#52289=CARTESIAN_POINT('Ctrl Pts',(7.83165452409203,1.13470475826316,131.403343672612));
#52290=CARTESIAN_POINT('Ctrl Pts',(7.80113801678985,1.32832068145589,131.411254310212));
#52291=CARTESIAN_POINT('Ctrl Pts',(7.76354368293116,1.52029947155803,131.419164947812));
#52292=CARTESIAN_POINT('Ctrl Pts',(7.74702551576303,1.60465095280951,131.422640717186));
#52293=CARTESIAN_POINT('Ctrl Pts',(7.72914159403645,1.68868657702022,131.42611648656));
#52294=CARTESIAN_POINT('Ctrl Pts',(7.70990679523191,1.77235950327152,131.429592255935));
#52295=CARTESIAN_POINT('Ctrl Pts',(7.66613384772448,1.96277535559263,131.437502121378));
#52296=CARTESIAN_POINT('Ctrl Pts',(7.61524342536188,2.15182559266713,131.445411986822));
#52297=CARTESIAN_POINT('Ctrl Pts',(7.55733337608319,2.33893848630933,131.453321852265));
#52298=CARTESIAN_POINT('Ctrl Pts',(7.49948626300756,2.52584802707557,131.461223121327));
#52299=CARTESIAN_POINT('Ctrl Pts',(7.43463481955377,2.71082409164834,131.469124390388));
#52300=CARTESIAN_POINT('Ctrl Pts',(7.36292790276842,2.89330497850368,131.47702565945));
#52301=CARTESIAN_POINT('Ctrl Pts',(7.29128559165454,3.07562145583268,131.484919809717));
#52302=CARTESIAN_POINT('Ctrl Pts',(7.2128002367439,3.25544691474066,131.492813959985));
#52303=CARTESIAN_POINT('Ctrl Pts',(7.12767059110865,3.4322343953531,131.500708110252));
#52304=CARTESIAN_POINT('Ctrl Pts',(7.04260183041424,3.60889543710611,131.508596614603));
#52305=CARTESIAN_POINT('Ctrl Pts',(6.95089839561357,3.78252251989815,131.516485118953));
#52306=CARTESIAN_POINT('Ctrl Pts',(6.8528073801641,3.95258801424693,131.524373623304));
#52307=CARTESIAN_POINT('Ctrl Pts',(6.75476830178432,4.12256346259718,131.532257950862));
#52308=CARTESIAN_POINT('Ctrl Pts',(6.65034855391276,4.28898078204876,131.540142278421));
#52309=CARTESIAN_POINT('Ctrl Pts',(6.53984158637937,4.45133609437245,131.548026605979));
#52310=CARTESIAN_POINT('Ctrl Pts',(6.42937260942353,4.61363559146366,131.555908223028));
#52311=CARTESIAN_POINT('Ctrl Pts',(6.3128207774534,4.77187557975789,131.563789840078));
#52312=CARTESIAN_POINT('Ctrl Pts',(6.1905235023506,4.92558014520573,131.571671457127));
#52313=CARTESIAN_POINT('Ctrl Pts',(6.06822455680444,5.07928681008522,131.57955318183));
#52314=CARTESIAN_POINT('Ctrl Pts',(5.94018021939878,5.22845765309482,131.587434906533));
#52315=CARTESIAN_POINT('Ctrl Pts',(5.80676927975302,5.37264846530243,131.595316631236));
#52316=CARTESIAN_POINT('Ctrl Pts',(5.67335025673447,5.51684801403565,131.603198833494));
#52317=CARTESIAN_POINT('Ctrl Pts',(5.53456421752344,5.65606667693122,131.611081035751));
#52318=CARTESIAN_POINT('Ctrl Pts',(5.39082805225096,5.78989584630537,131.618963238008));
#52319=CARTESIAN_POINT('Ctrl Pts',(5.24705899146809,5.92375564387126,131.626847244189));
#52320=CARTESIAN_POINT('Ctrl Pts',(5.09833779973761,6.05222325493353,131.634731250369));
#52321=CARTESIAN_POINT('Ctrl Pts',(4.94511596769183,6.17492907376913,131.64261525655));
#52322=CARTESIAN_POINT('Ctrl Pts',(4.79183328621712,6.29768362312115,131.650502393729));
#52323=CARTESIAN_POINT('Ctrl Pts',(4.63404667210869,6.4146716052893,131.658389530908));
#52324=CARTESIAN_POINT('Ctrl Pts',(4.47223840631225,6.52556546493142,131.666276668087));
#52325=CARTESIAN_POINT('Ctrl Pts',(4.31025742502092,6.6365776936059,131.674172224062));
#52326=CARTESIAN_POINT('Ctrl Pts',(4.14424650233152,6.7414826115451,131.682067780037));
#52327=CARTESIAN_POINT('Ctrl Pts',(3.9747153972542,6.83999696716529,131.689963336012));
#52328=CARTESIAN_POINT('Ctrl Pts',(3.80508100274972,6.93857134416831,131.697863702476));
#52329=CARTESIAN_POINT('Ctrl Pts',(3.6319224538412,7.03074723486181,131.70576406894));
#52330=CARTESIAN_POINT('Ctrl Pts',(3.45577173724022,7.11628854811915,131.713664435403));
#52331=CARTESIAN_POINT('Ctrl Pts',(3.27939158677093,7.20194127775207,131.721575091985));
#52332=CARTESIAN_POINT('Ctrl Pts',(3.10001179885957,7.28094203051928,131.729485748566));
#52333=CARTESIAN_POINT('Ctrl Pts',(2.91818291514442,7.35310339066161,131.737396405148));
#52334=CARTESIAN_POINT('Ctrl Pts',(2.83829127605092,7.38480951580077,131.740872174826));
#52335=CARTESIAN_POINT('Ctrl Pts',(2.75792701517316,7.41519592730195,131.744347944504));
#52336=CARTESIAN_POINT('Ctrl Pts',(2.67713758109783,7.44424981928157,131.747823714182));
#52337=CARTESIAN_POINT('Ctrl Pts',(2.49493491938076,7.50977443289615,131.755662542292));
#52338=CARTESIAN_POINT('Ctrl Pts',(2.31004995145518,7.56870469733447,131.763501370403));
#52339=CARTESIAN_POINT('Ctrl Pts',(2.12300593910925,7.62081142546559,131.771340198513));
#52340=CARTESIAN_POINT('Ctrl Pts',(1.93617160020406,7.67285974276154,131.779170239419));
#52341=CARTESIAN_POINT('Ctrl Pts',(1.74718337136202,7.71809966122804,131.787000280324));
#52342=CARTESIAN_POINT('Ctrl Pts',(1.55658426346542,7.75635007144029,131.79483032123));
#52343=CARTESIAN_POINT('Ctrl Pts',(1.36616171838287,7.79456504811804,131.802653108722));
#52344=CARTESIAN_POINT('Ctrl Pts',(1.17413160834321,7.82580334203642,131.810475896215));
#52345=CARTESIAN_POINT('Ctrl Pts',(0.981052061062631,7.84993362096042,131.818298683707));
#52346=CARTESIAN_POINT('Ctrl Pts',(0.788113815986769,7.87404624052246,131.826115746217));
#52347=CARTESIAN_POINT('Ctrl Pts',(0.594128010749377,7.89106116234817,131.833932808726));
#52348=CARTESIAN_POINT('Ctrl Pts',(0.399663113605735,7.90089807525847,131.841749871236));
#52349=CARTESIAN_POINT('Ctrl Pts',(0.205302718527595,7.91072970198225,131.849562732991));
#52350=CARTESIAN_POINT('Ctrl Pts',(0.010464094781512,7.91339098596106,131.857375594747));
#52351=CARTESIAN_POINT('Ctrl Pts',(-0.184278823972296,7.90885341342444,
131.865188456502));
#52352=CARTESIAN_POINT('Ctrl Pts',(-0.378954949974643,7.90431739718038,
131.87299863861));
#52353=CARTESIAN_POINT('Ctrl Pts',(-0.573535085160128,7.8925874520569,131.880808820717));
#52354=CARTESIAN_POINT('Ctrl Pts',(-0.76744475834389,7.87368716313332,131.888619002824));
#52355=CARTESIAN_POINT('Ctrl Pts',(-0.961363176978565,7.85478602179457,
131.896429537175));
#52356=CARTESIAN_POINT('Ctrl Pts',(-1.15461072218794,7.82871391549095,131.904240071527));
#52357=CARTESIAN_POINT('Ctrl Pts',(-1.34661698864132,7.79554640072796,131.912050605879));
#52358=CARTESIAN_POINT('Ctrl Pts',(-1.5386386445773,7.76237622755751,131.919861766252));
#52359=CARTESIAN_POINT('Ctrl Pts',(-1.72941847653137,7.72210957215602,131.927672926625));
#52360=CARTESIAN_POINT('Ctrl Pts',(-1.91839531990764,7.67487331469103,131.935484086998));
#52361=CARTESIAN_POINT('Ctrl Pts',(-2.10742059250838,7.62762495195814,131.943297249142));
#52362=CARTESIAN_POINT('Ctrl Pts',(-2.29464161464747,7.57340351430882,131.951110411287));
#52363=CARTESIAN_POINT('Ctrl Pts',(-2.47951130771365,7.51238608398957,131.958923573432));
#52364=CARTESIAN_POINT('Ctrl Pts',(-2.66446093954404,7.45134226936744,131.966740114034));
#52365=CARTESIAN_POINT('Ctrl Pts',(-2.84705688312377,7.38349671838267,131.974556654637));
#52366=CARTESIAN_POINT('Ctrl Pts',(-3.02677085724862,7.30907512464542,131.98237319524));
#52367=CARTESIAN_POINT('Ctrl Pts',(-3.20669456085284,7.23456667955348,131.990198857888));
#52368=CARTESIAN_POINT('Ctrl Pts',(-3.38372925235048,7.1534669984069,131.998024520535));
#52369=CARTESIAN_POINT('Ctrl Pts',(-3.55736914106945,7.06604881062725,132.005850183183));
#52370=CARTESIAN_POINT('Ctrl Pts',(-3.73112221384284,6.97857364086612,132.013680946849));
#52371=CARTESIAN_POINT('Ctrl Pts',(-3.90147576696341,6.88477192596603,132.021511710515));
#52372=CARTESIAN_POINT('Ctrl Pts',(-4.06795189917533,6.78496045279527,132.029342474182));
#52373=CARTESIAN_POINT('Ctrl Pts',(-4.23466857189771,6.68500476253833,132.037184552478));
#52374=CARTESIAN_POINT('Ctrl Pts',(-4.39749634006955,6.57902216146759,132.045026630774));
#52375=CARTESIAN_POINT('Ctrl Pts',(-4.55598839936478,6.46737123604743,132.052868709071));
#52376=CARTESIAN_POINT('Ctrl Pts',(-4.64482325723005,6.40479085104686,132.057264196857));
#52377=CARTESIAN_POINT('Ctrl Pts',(-4.73229662514873,6.34043040864525,132.061659684643));
#52378=CARTESIAN_POINT('Ctrl Pts',(-4.81833483756805,6.27435816582685,132.066055172429));
#52379=CARTESIAN_POINT('Ctrl Pts',(-4.97183518733137,6.15647900380008,132.073897140475));
#52380=CARTESIAN_POINT('Ctrl Pts',(-5.12124346991903,6.03278191119074,132.081739108521));
#52381=CARTESIAN_POINT('Ctrl Pts',(-5.26608374474064,5.90358221704233,132.089581076568));
#52382=CARTESIAN_POINT('Ctrl Pts',(-5.41075677738981,5.77453170541622,132.097413989758));
#52383=CARTESIAN_POINT('Ctrl Pts',(-5.5508720452749,5.63999147576539,132.105246902949));
#52384=CARTESIAN_POINT('Ctrl Pts',(-5.68598331006465,5.50031951777952,132.113079816139));
#52385=CARTESIAN_POINT('Ctrl Pts',(-5.82096490632567,5.3607816052955,132.120905211953));
#52386=CARTESIAN_POINT('Ctrl Pts',(-5.95095182064843,5.21612202379973,132.128730607766));
#52387=CARTESIAN_POINT('Ctrl Pts',(-6.07553145825877,5.06673844792763,132.13655600358));
#52388=CARTESIAN_POINT('Ctrl Pts',(-6.20001580688461,4.91746913317812,132.144375413873));
#52389=CARTESIAN_POINT('Ctrl Pts',(-6.31910089240349,4.76348329009855,132.152194824165));
#52390=CARTESIAN_POINT('Ctrl Pts',(-6.43241139925501,4.60521493426032,132.160014234458));
#52391=CARTESIAN_POINT('Ctrl Pts',(-6.54565730415862,4.44703681227915,132.167829186654));
#52392=CARTESIAN_POINT('Ctrl Pts',(-6.65313498475536,4.28458132700701,132.175644138851));
#52393=CARTESIAN_POINT('Ctrl Pts',(-6.75450970018044,4.1183151543038,132.183459091047));
#52394=CARTESIAN_POINT('Ctrl Pts',(-6.85585384782215,3.95209911627498,132.191271686781));
#52395=CARTESIAN_POINT('Ctrl Pts',(-6.9510985106699,3.78207497844818,132.199084282514));
#52396=CARTESIAN_POINT('Ctrl Pts',(-7.03995238370444,3.60873820540839,132.206896878248));
#52397=CARTESIAN_POINT('Ctrl Pts',(-7.12879453234187,3.43542430440661,132.214708443098));
#52398=CARTESIAN_POINT('Ctrl Pts',(-7.21124740971074,3.25879895178036,132.222520007948));
#52399=CARTESIAN_POINT('Ctrl Pts',(-7.28706571365825,3.07938212712005,132.230331572798));
#52400=CARTESIAN_POINT('Ctrl Pts',(-7.36288738445613,2.89995733512769,132.238143484535));
#52401=CARTESIAN_POINT('Ctrl Pts',(-7.43207375820792,2.71774114864288,132.245955396272));
#52402=CARTESIAN_POINT('Ctrl Pts',(-7.49442766561047,2.53327356693516,132.253767308009));
#52403=CARTESIAN_POINT('Ctrl Pts',(-7.55679533896533,2.34876526008225,132.261580944392));
#52404=CARTESIAN_POINT('Ctrl Pts',(-7.61232742948562,2.1620049016543,132.269394580775));
#52405=CARTESIAN_POINT('Ctrl Pts',(-7.66087657969628,1.9735478283186,132.277208217158));
#52406=CARTESIAN_POINT('Ctrl Pts',(-7.70946566857206,1.78493572191003,132.285028281381));
#52407=CARTESIAN_POINT('Ctrl Pts',(-7.75106025658121,1.59462445409737,132.292848345605));
#52408=CARTESIAN_POINT('Ctrl Pts',(-7.78556389772135,1.40318059938765,132.300668409828));
#52409=CARTESIAN_POINT('Ctrl Pts',(-7.82008381387908,1.21164644255335,132.308492162697));
#52410=CARTESIAN_POINT('Ctrl Pts',(-7.84750606669332,1.01897898190208,132.316315915566));
#52411=CARTESIAN_POINT('Ctrl Pts',(-7.86778606549067,0.82575022111459,132.324139668434));
#52412=CARTESIAN_POINT('Ctrl Pts',(-7.88808855803473,0.63230713887447,132.33197209909));
#52413=CARTESIAN_POINT('Ctrl Pts',(-7.90123295178609,0.43830186352041,132.339804529746));
#52414=CARTESIAN_POINT('Ctrl Pts',(-7.90722674356102,0.244307646039636,
132.347636960401));
#52415=CARTESIAN_POINT('Ctrl Pts',(-7.90975545013015,0.162463886606973,
132.350941365959));
#52416=CARTESIAN_POINT('Ctrl Pts',(-7.91101206252141,0.080622056533713,
132.354245771516));
#52417=CARTESIAN_POINT('Ctrl Pts',(-7.91099991273041,-0.00117506573469943,
132.357550177074));
#52418=CARTESIAN_POINT('',(-7.911,-1.35114142096882E-12,134.357668491763));
#52419=CARTESIAN_POINT('Ctrl Pts',(-7.91099990902224,-0.00116857302219743,
132.357715510959));
#52420=CARTESIAN_POINT('Ctrl Pts',(-7.91065715600478,-2.20244882135127,
132.446287273627));
#52421=CARTESIAN_POINT('Ctrl Pts',(-6.94185703501063,-4.38636564778651,
132.534859036294));
#52422=CARTESIAN_POINT('Ctrl Pts',(-3.67820201488134,-7.34180684107709,
132.712018234694));
#52423=CARTESIAN_POINT('Ctrl Pts',(-1.40868175871573,-8.08992666571367,
132.800605670427));
#52424=CARTESIAN_POINT('Ctrl Pts',(2.97309270521441,-7.65454228025193,132.977780541892));
#52425=CARTESIAN_POINT('Ctrl Pts',(5.05102072675747,-6.47444880834114,133.066367977625));
#52426=CARTESIAN_POINT('Ctrl Pts',(7.6695151884794,-2.93425195367532,133.24354284909));
#52427=CARTESIAN_POINT('Ctrl Pts',(8.18956872247086,-0.601881960097262,
133.332130284823));
#52428=CARTESIAN_POINT('Ctrl Pts',(7.32306689761255,3.71537198232625,133.509305156289));
#52429=CARTESIAN_POINT('Ctrl Pts',(5.94329958850064,5.66643518936656,133.597892592021));
#52430=CARTESIAN_POINT('Ctrl Pts',(2.1615450163765,7.92205913233052,133.775067463487));
#52431=CARTESIAN_POINT('Ctrl Pts',(-0.210816529302454,8.20894963712998,
133.863654899219));
#52432=CARTESIAN_POINT('Ctrl Pts',(-4.42123908576618,6.91982244717717,134.040829770685));
#52433=CARTESIAN_POINT('Ctrl Pts',(-6.2263162563433,5.35390358803356,134.129417206418));
#52434=CARTESIAN_POINT('Ctrl Pts',(-7.6531728085954,2.31334857514337,134.264559258688));
#52435=CARTESIAN_POINT('Ctrl Pts',(-7.9110000000002,1.15702837836358,134.311113875226));
#52436=CARTESIAN_POINT('Ctrl Pts',(-7.911,-1.35114142096882E-12,134.357668491763));
#52437=CARTESIAN_POINT('',(-7.911,-1.18072218668885E-12,136.357668491763));
#52438=CARTESIAN_POINT('Ctrl Pts',(-7.911,-1.35114142096882E-12,134.357668491763));
#52439=CARTESIAN_POINT('Ctrl Pts',(-7.91099999999962,-2.20167589666815,
134.446255927496));
#52440=CARTESIAN_POINT('Ctrl Pts',(-6.94214576672294,-4.38610418338807,
134.534843363229));
#52441=CARTESIAN_POINT('Ctrl Pts',(-3.6782020148815,-7.34180684107701,134.712018234694));
#52442=CARTESIAN_POINT('Ctrl Pts',(-1.4086817587159,-8.08992666571364,134.800605670427));
#52443=CARTESIAN_POINT('Ctrl Pts',(2.97309270521425,-7.65454228025199,134.977780541892));
#52444=CARTESIAN_POINT('Ctrl Pts',(5.05102072675733,-6.47444880834125,135.066367977625));
#52445=CARTESIAN_POINT('Ctrl Pts',(7.66951518847933,-2.93425195367548,135.24354284909));
#52446=CARTESIAN_POINT('Ctrl Pts',(8.18956872247085,-0.601881960097438,
135.332130284823));
#52447=CARTESIAN_POINT('Ctrl Pts',(7.32306689761262,3.7153719823261,135.509305156289));
#52448=CARTESIAN_POINT('Ctrl Pts',(5.94329958850076,5.66643518936643,135.597892592021));
#52449=CARTESIAN_POINT('Ctrl Pts',(2.16154501637667,7.92205913233048,135.775067463487));
#52450=CARTESIAN_POINT('Ctrl Pts',(-0.210816529302277,8.20894963712998,
135.863654899219));
#52451=CARTESIAN_POINT('Ctrl Pts',(-4.42123908576603,6.91982244717726,136.040829770685));
#52452=CARTESIAN_POINT('Ctrl Pts',(-6.22631625634319,5.3539035880337,136.129417206418));
#52453=CARTESIAN_POINT('Ctrl Pts',(-7.65317280859534,2.31334857514353,136.264559258688));
#52454=CARTESIAN_POINT('Ctrl Pts',(-7.91100000000017,1.15702837836375,136.311113875225));
#52455=CARTESIAN_POINT('Ctrl Pts',(-7.911,-1.18072218668885E-12,136.357668491763));
#52456=CARTESIAN_POINT('',(-7.91172576763303,-0.00412227042729108,138.357668491763));
#52457=CARTESIAN_POINT('Ctrl Pts',(-7.911,-1.18072218668885E-12,136.357668491763));
#52458=CARTESIAN_POINT('Ctrl Pts',(-7.91099999999967,-2.20167589666783,
136.446255927496));
#52459=CARTESIAN_POINT('Ctrl Pts',(-6.94214576672317,-4.38610418338763,
136.534843363229));
#52460=CARTESIAN_POINT('Ctrl Pts',(-3.67820201488219,-7.34180684107662,
136.712018234694));
#52461=CARTESIAN_POINT('Ctrl Pts',(-1.40868175871685,-8.08992666571343,
136.800605670427));
#52462=CARTESIAN_POINT('Ctrl Pts',(2.97309270521306,-7.65454228025241,136.977780541892));
#52463=CARTESIAN_POINT('Ctrl Pts',(5.05102072675617,-6.4744488083421,137.066367977625));
#52464=CARTESIAN_POINT('Ctrl Pts',(7.66951518847868,-2.93425195367707,137.24354284909));
#52465=CARTESIAN_POINT('Ctrl Pts',(8.18956872247067,-0.601881960099329,
137.332130284823));
#52466=CARTESIAN_POINT('Ctrl Pts',(7.32306689761358,3.71537198232413,137.509305156288));
#52467=CARTESIAN_POINT('Ctrl Pts',(5.94329958850237,5.66643518936469,137.597892592021));
#52468=CARTESIAN_POINT('Ctrl Pts',(2.16154501637922,7.92205913232974,137.775067463487));
#52469=CARTESIAN_POINT('Ctrl Pts',(-0.210816529299444,8.20894963713002,
137.863654899219));
#52470=CARTESIAN_POINT('Ctrl Pts',(-4.42123908576338,6.91982244717891,138.040829770685));
#52471=CARTESIAN_POINT('Ctrl Pts',(-6.226316256341,5.35390358803617,138.129417206417));
#52472=CARTESIAN_POINT('Ctrl Pts',(-7.65317280859482,2.31334857514579,138.264559258688));
#52473=CARTESIAN_POINT('Ctrl Pts',(-7.91100000000015,1.15702837836497,138.311113875225));
#52474=CARTESIAN_POINT('Ctrl Pts',(-7.911,-1.00974784089658E-12,138.357668491763));
#52475=CARTESIAN_POINT('',(-7.91692124670087,0.00260438373366838,140.357668491763));
#52476=CARTESIAN_POINT('Ctrl Pts',(-7.9121326383558,-0.00643324582964995,
138.357668491763));
#52477=CARTESIAN_POINT('Ctrl Pts',(-7.91784775911465,-0.610979849499266,
138.382007106964));
#52478=CARTESIAN_POINT('Ctrl Pts',(-7.57810911672367,-3.84456081973681,
138.512422874915));
#52479=CARTESIAN_POINT('Ctrl Pts',(-3.12943036986337,-8.82205618148566,
138.748915795611));
#52480=CARTESIAN_POINT('Ctrl Pts',(4.23830707040841,-7.63046510228338,139.014108677485));
#52481=CARTESIAN_POINT('Ctrl Pts',(7.53328766571923,-3.29951305733849,139.226262982982));
#52482=CARTESIAN_POINT('Ctrl Pts',(8.48220415360649,2.05899421969992,139.438417288479));
#52483=CARTESIAN_POINT('Ctrl Pts',(4.36206927714242,8.28217129323548,139.703610170354));
#52484=CARTESIAN_POINT('Ctrl Pts',(-4.61994212435092,8.14028744154645,140.021841628598));
#52485=CARTESIAN_POINT('Ctrl Pts',(-7.85289975606266,2.91743073677501,140.239861069069));
#52486=CARTESIAN_POINT('Ctrl Pts',(-7.92258005546765,0.147753258561319,
140.351803356791));
#52487=CARTESIAN_POINT('Ctrl Pts',(-7.92196407697051,0.00260604264433853,
140.357668491763));
#52488=CARTESIAN_POINT('',(-7.91099906863223,0.00271441514469461,142.357668491763));
#52489=CARTESIAN_POINT('Ctrl Pts',(-7.91099957194591,0.00260243571461738,
140.357668491763));
#52490=CARTESIAN_POINT('Ctrl Pts',(-7.91106335204651,-0.191279144422676,
140.365513763889));
#52491=CARTESIAN_POINT('Ctrl Pts',(-7.90399549224218,-0.385438385360763,
140.373359036015));
#52492=CARTESIAN_POINT('Ctrl Pts',(-7.88976095331893,-0.579303978481056,
140.381204308142));
#52493=CARTESIAN_POINT('Ctrl Pts',(-7.87554147399741,-0.772964469164422,
140.389041280268));
#52494=CARTESIAN_POINT('Ctrl Pts',(-7.85417043973893,-0.966331583624417,
140.396878252394));
#52495=CARTESIAN_POINT('Ctrl Pts',(-7.82566477298294,-1.15883211074506,
140.40471522452));
#52496=CARTESIAN_POINT('Ctrl Pts',(-7.79718373514862,-1.35116631723747,
140.412545425495));
#52497=CARTESIAN_POINT('Ctrl Pts',(-7.7615803929866,-1.54263508229892,140.420375626471));
#52498=CARTESIAN_POINT('Ctrl Pts',(-7.71892361913266,-1.7326682204034,140.428205827446));
#52499=CARTESIAN_POINT('Ctrl Pts',(-7.6762954307552,-1.92257401207944,140.436030781188));
#52500=CARTESIAN_POINT('Ctrl Pts',(-7.6266233024895,-2.1110457517298,140.44385573493));
#52501=CARTESIAN_POINT('Ctrl Pts',(-7.57002756976397,-2.29752118445368,
140.451680688673));
#52502=CARTESIAN_POINT('Ctrl Pts',(-7.51345879436308,-2.48390779636834,
140.459501915282));
#52503=CARTESIAN_POINT('Ctrl Pts',(-7.44997308640442,-2.66829966033515,
140.467323141892));
#52504=CARTESIAN_POINT('Ctrl Pts',(-7.37974128529881,-2.85014728778291,
140.475144368501));
#52505=CARTESIAN_POINT('Ctrl Pts',(-7.30951976620366,-3.0319682925444,140.482964450074));
#52506=CARTESIAN_POINT('Ctrl Pts',(-7.23255424131079,-3.21124547284067,
140.490784531648));
#52507=CARTESIAN_POINT('Ctrl Pts',(-7.14906472596667,-3.38744661123082,
140.498604613221));
#52508=CARTESIAN_POINT('Ctrl Pts',(-7.0655789087473,-3.56363994488298,140.506424348409));
#52509=CARTESIAN_POINT('Ctrl Pts',(-6.97556982626458,-3.73675719005832,
140.514244083596));
#52510=CARTESIAN_POINT('Ctrl Pts',(-6.87930476865276,-3.90628812301288,
140.522063818783));
#52511=CARTESIAN_POINT('Ctrl Pts',(-6.78302707565235,-4.07584130795863,
140.529884580359));
#52512=CARTESIAN_POINT('Ctrl Pts',(-6.68049194516839,-4.24180693729539,
140.537705341935));
#52513=CARTESIAN_POINT('Ctrl Pts',(-6.57201163539827,-4.40370117789455,
140.545526103511));
#52514=CARTESIAN_POINT('Ctrl Pts',(-6.46349804212243,-4.56564509025344,
140.553349264622));
#52515=CARTESIAN_POINT('Ctrl Pts',(-6.349035831643,-4.7235148338636,140.561172425734));
#52516=CARTESIAN_POINT('Ctrl Pts',(-6.22897950457071,-4.87685711618026,
140.568995586845));
#52517=CARTESIAN_POINT('Ctrl Pts',(-6.10880037454934,-5.03035624890994,
140.576826750095));
#52518=CARTESIAN_POINT('Ctrl Pts',(-5.98301591407282,-5.17931839233316,
140.584657913344));
#52519=CARTESIAN_POINT('Ctrl Pts',(-5.8520203963911,-5.32332398790666,140.592489076593));
#52520=CARTESIAN_POINT('Ctrl Pts',(-5.72095393456939,-5.46740757357718,
140.600324481019));
#52521=CARTESIAN_POINT('Ctrl Pts',(-5.58467103587247,-5.60652901054929,
140.608159885445));
#52522=CARTESIAN_POINT('Ctrl Pts',(-5.44360154106573,-5.74030689616042,
140.615995289871));
#52523=CARTESIAN_POINT('Ctrl Pts',(-5.30233550066011,-5.87427116830877,
140.623841611003));
#52524=CARTESIAN_POINT('Ctrl Pts',(-5.15626980297759,-6.00287678243778,
140.631687932136));
#52525=CARTESIAN_POINT('Ctrl Pts',(-5.00586695910596,-6.12578296936247,
140.639534253268));
#52526=CARTESIAN_POINT('Ctrl Pts',(-4.88593367134506,-6.22379004625401,
140.64579101721));
#52527=CARTESIAN_POINT('Ctrl Pts',(-4.76324318593414,-6.3181738247826,140.652047781151));
#52528=CARTESIAN_POINT('Ctrl Pts',(-4.63804215597438,-6.40878194038497,
140.658304545093));
#52529=CARTESIAN_POINT('Ctrl Pts',(-4.48118321702758,-6.52230091764837,
140.666143373203));
#52530=CARTESIAN_POINT('Ctrl Pts',(-4.31991715194024,-6.63022905894237,
140.673982201313));
#52531=CARTESIAN_POINT('Ctrl Pts',(-4.15468305701145,-6.73220095479792,
140.681821029424));
#52532=CARTESIAN_POINT('Ctrl Pts',(-3.98963418694379,-6.83405854173763,
140.689651070329));
#52533=CARTESIAN_POINT('Ctrl Pts',(-3.8206264402778,-6.92997299544976,140.697481111235));
#52534=CARTESIAN_POINT('Ctrl Pts',(-3.64813123004012,-7.01961961422455,
140.70531115214));
#52535=CARTESIAN_POINT('Ctrl Pts',(-3.47579581194466,-7.1091831882282,140.713133939633));
#52536=CARTESIAN_POINT('Ctrl Pts',(-3.29997967376778,-7.1924903291321,140.720956727125));
#52537=CARTESIAN_POINT('Ctrl Pts',(-3.12118256666135,-7.26925996134196,
140.728779514618));
#52538=CARTESIAN_POINT('Ctrl Pts',(-2.94251630938244,-7.34597341091388,
140.736596577127));
#52539=CARTESIAN_POINT('Ctrl Pts',(-2.76087374996427,-7.41615874276132,
140.744413639637));
#52540=CARTESIAN_POINT('Ctrl Pts',(-2.57677873425341,-7.47958102801884,
140.752230702146));
#52541=CARTESIAN_POINT('Ctrl Pts',(-2.39278264801264,-7.54296923123972,
140.760043563902));
#52542=CARTESIAN_POINT('Ctrl Pts',(-2.2063370624747,-7.59960151328478,140.767856425658));
#52543=CARTESIAN_POINT('Ctrl Pts',(-2.01798545004014,-7.64929119091608,
140.775669287413));
#52544=CARTESIAN_POINT('Ctrl Pts',(-1.82969843827413,-7.69896382602592,
140.783479469521));
#52545=CARTESIAN_POINT('Ctrl Pts',(-1.63950704182425,-7.74169851144335,
140.791289651628));
#52546=CARTESIAN_POINT('Ctrl Pts',(-1.44796970902329,-7.77735846684149,
140.799099833735));
#52547=CARTESIAN_POINT('Ctrl Pts',(-1.2564237377643,-7.81302003052676,140.806910368087));
#52548=CARTESIAN_POINT('Ctrl Pts',(-1.06353205301641,-7.84160615324437,
140.814720902438));
#52549=CARTESIAN_POINT('Ctrl Pts',(-0.869863621148918,-7.86303111278352,
140.82253143679));
#52550=CARTESIAN_POINT('Ctrl Pts',(-0.676179666574861,-7.88445778955329,
140.830342597163));
#52551=CARTESIAN_POINT('Ctrl Pts',(-0.481719190672601,-7.89872212023501,
140.838153757536));
#52552=CARTESIAN_POINT('Ctrl Pts',(-0.287056526486923,-7.90579025465521,
140.845964917909));
#52553=CARTESIAN_POINT('Ctrl Pts',(-0.0923439759677483,-7.91286020043103,
140.853778080054));
#52554=CARTESIAN_POINT('Ctrl Pts',(0.102570514381587,-7.91273026330336,
140.861591242198));
#52555=CARTESIAN_POINT('Ctrl Pts',(0.297112211024626,-7.90541873236706,
140.869404404343));
#52556=CARTESIAN_POINT('Ctrl Pts',(0.49173802866483,-7.89810403988091,140.877220944946));
#52557=CARTESIAN_POINT('Ctrl Pts',(0.685990380209172,-7.88360158077329,
140.885037485549));
#52558=CARTESIAN_POINT('Ctrl Pts',(0.879299099446526,-7.86198156279398,
140.892854026152));
#52559=CARTESIAN_POINT('Ctrl Pts',(1.07283341347798,-7.84033631386015,140.900679688799));
#52560=CARTESIAN_POINT('Ctrl Pts',(1.26542154598018,-7.81155695501726,140.908505351447));
#52561=CARTESIAN_POINT('Ctrl Pts',(1.45650188338359,-7.77576512400549,140.916331014095));
#52562=CARTESIAN_POINT('Ctrl Pts',(1.64770677308509,-7.73994996272925,140.924161777761));
#52563=CARTESIAN_POINT('Ctrl Pts',(1.83740156712912,-7.69711329745667,140.931992541428));
#52564=CARTESIAN_POINT('Ctrl Pts',(2.02503921798722,-7.64742683296896,140.939823305094));
#52565=CARTESIAN_POINT('Ctrl Pts',(2.21294798552638,-7.5976685767631,140.94766538339));
#52566=CARTESIAN_POINT('Ctrl Pts',(2.39879333790389,-7.5410408554811,140.955507461686));
#52567=CARTESIAN_POINT('Ctrl Pts',(2.58204650177999,-7.47776416201031,140.963349539983));
#52568=CARTESIAN_POINT('Ctrl Pts',(2.68475996791432,-7.44229755191511,140.967745027769));
#52569=CARTESIAN_POINT('Ctrl Pts',(2.78665946903391,-7.40474294752419,140.972140515554));
#52570=CARTESIAN_POINT('Ctrl Pts',(2.8876552895524,-7.36514547912803,140.97653600334));
#52571=CARTESIAN_POINT('Ctrl Pts',(3.0695545179995,-7.29382818190976,140.984452527339));
#52572=CARTESIAN_POINT('Ctrl Pts',(3.24906693009082,-7.21566758276959,140.992369051337));
#52573=CARTESIAN_POINT('Ctrl Pts',(3.42564045981255,-7.13084205687486,141.000285575336));
#52574=CARTESIAN_POINT('Ctrl Pts',(3.60201056607367,-7.04611425515234,141.008192979016));
#52575=CARTESIAN_POINT('Ctrl Pts',(3.77544822629118,-6.95473696833451,141.016100382697));
#52576=CARTESIAN_POINT('Ctrl Pts',(3.94541851420322,-6.8569376362763,141.024007786378));
#52577=CARTESIAN_POINT('Ctrl Pts',(4.11522448234757,-6.75923285229307,141.03190754553));
#52578=CARTESIAN_POINT('Ctrl Pts',(4.28156945919491,-6.65511856144155,141.039807304682));
#52579=CARTESIAN_POINT('Ctrl Pts',(4.44394016445202,-6.54486950326515,141.047707063834));
#52580=CARTESIAN_POINT('Ctrl Pts',(4.60618397440471,-6.43470660649191,141.055600649197));
#52581=CARTESIAN_POINT('Ctrl Pts',(4.76445941704984,-6.31841868697704,141.063494234561));
#52582=CARTESIAN_POINT('Ctrl Pts',(4.91827917727038,-6.19632559945236,141.071387819925));
#52583=CARTESIAN_POINT('Ctrl Pts',(5.07200721117977,-6.07430531888381,141.07927669816));
#52584=CARTESIAN_POINT('Ctrl Pts',(5.22128458791495,-5.94648698177163,141.087165576395));
#52585=CARTESIAN_POINT('Ctrl Pts',(5.36565405063375,-5.81323297390683,141.095054454629));
#52586=CARTESIAN_POINT('Ctrl Pts',(5.50996415367775,-5.68003375543047,141.102940089233));
#52587=CARTESIAN_POINT('Ctrl Pts',(5.64937011160394,-5.54140355372392,141.110825723837));
#52588=CARTESIAN_POINT('Ctrl Pts',(5.78344855584883,-5.39774432535018,141.118711358441));
#52589=CARTESIAN_POINT('Ctrl Pts',(5.91751507293542,-5.25409787640842,141.126596291566));
#52590=CARTESIAN_POINT('Ctrl Pts',(6.04625478081094,-5.10542353949511,141.134481224691));
#52591=CARTESIAN_POINT('Ctrl Pts',(6.16928157546607,-4.95215971497436,141.142366157815));
#52592=CARTESIAN_POINT('Ctrl Pts',(6.29230794357874,-4.79889642182996,141.150251063603));
#52593=CARTESIAN_POINT('Ctrl Pts',(6.40962122170412,-4.64104394125102,141.15813596939));
#52594=CARTESIAN_POINT('Ctrl Pts',(6.5208759140238,-4.47907337670464,141.166020875177));
#52595=CARTESIAN_POINT('Ctrl Pts',(6.63214888650748,-4.31707619891236,141.173907076527));
#52596=CARTESIAN_POINT('Ctrl Pts',(6.73736109447993,-4.15095987304952,141.181793277876));
#52597=CARTESIAN_POINT('Ctrl Pts',(6.83621052363777,-3.98122426855159,141.189679479225));
#52598=CARTESIAN_POINT('Ctrl Pts',(6.9350927793172,-3.81143229721845,141.197568299473));
#52599=CARTESIAN_POINT('Ctrl Pts',(7.02760787274722,-3.63801895014476,141.20545711972));
#52600=CARTESIAN_POINT('Ctrl Pts',(7.11349975321371,-3.46150866834513,141.213345939967));
#52601=CARTESIAN_POINT('Ctrl Pts',(7.19947476909308,-3.28482754088378,141.221242395864));
#52602=CARTESIAN_POINT('Ctrl Pts',(7.2788136162776,-3.10504380136803,141.229138851762));
#52603=CARTESIAN_POINT('Ctrl Pts',(7.35130799479212,-2.92270281857486,141.237035307659));
#52604=CARTESIAN_POINT('Ctrl Pts',(7.42384244102232,-2.74026105573773,141.244936127935));
#52605=CARTESIAN_POINT('Ctrl Pts',(7.48952476102888,-2.55525955570648,141.252836948211));
#52606=CARTESIAN_POINT('Ctrl Pts',(7.54819646556174,-2.36825908998178,141.260737768488));
#52607=CARTESIAN_POINT('Ctrl Pts',(7.60693946416074,-2.1810313933682,141.268648189331));
#52608=CARTESIAN_POINT('Ctrl Pts',(7.65865474031047,-1.99180021074833,141.276558610173));
#52609=CARTESIAN_POINT('Ctrl Pts',(7.70323461524538,-1.8011378244003,141.284469031016));
#52610=CARTESIAN_POINT('Ctrl Pts',(7.72258052009646,-1.71839787974242,141.287901841206));
#52611=CARTESIAN_POINT('Ctrl Pts',(7.74058333313737,-1.63538849833788,141.291334651397));
#52612=CARTESIAN_POINT('Ctrl Pts',(7.75723729255867,-1.55215675333939,141.294767461587));
#52613=CARTESIAN_POINT('Ctrl Pts',(7.79757488539591,-1.35056095525013,141.303082078924));
#52614=CARTESIAN_POINT('Ctrl Pts',(7.83008429766918,-1.14721849981829,141.311396696262));
#52615=CARTESIAN_POINT('Ctrl Pts',(7.85462553585582,-0.942750598770242,
141.319711313599));
#52616=CARTESIAN_POINT('Ctrl Pts',(7.87913644230235,-0.738535409797657,
141.328015654487));
#52617=CARTESIAN_POINT('Ctrl Pts',(7.89569878168113,-0.533197839257424,
141.336319995374));
#52618=CARTESIAN_POINT('Ctrl Pts',(7.90422358889733,-0.327368991688265,
141.344624336261));
#52619=CARTESIAN_POINT('Ctrl Pts',(7.91273842339619,-0.12178093231108,141.352918962343));
#52620=CARTESIAN_POINT('Ctrl Pts',(7.91323446755868,0.0842969658480649,
141.361213588425));
#52621=CARTESIAN_POINT('Ctrl Pts',(7.90567446500996,0.290227933337863,141.369508214507));
#52622=CARTESIAN_POINT('Ctrl Pts',(7.89812584551826,0.495848831627049,141.377790351412));
#52623=CARTESIAN_POINT('Ctrl Pts',(7.88254539712639,0.701322948546397,141.386072488318));
#52624=CARTESIAN_POINT('Ctrl Pts',(7.85894787110344,0.906012891342435,141.394354625224));
#52625=CARTESIAN_POINT('Ctrl Pts',(7.83537210660609,1.11051407005261,141.402629124383));
#52626=CARTESIAN_POINT('Ctrl Pts',(7.80379404133808,1.3142322264089,141.410903623542));
#52627=CARTESIAN_POINT('Ctrl Pts',(7.7642803768472,1.51653263390719,141.419178122701));
#52628=CARTESIAN_POINT('Ctrl Pts',(7.72481215932269,1.71860036392706,141.427443104876));
#52629=CARTESIAN_POINT('Ctrl Pts',(7.67742661142091,1.91925331177573,141.435708087052));
#52630=CARTESIAN_POINT('Ctrl Pts',(7.62224193218953,2.11786423719078,141.443973069227));
#52631=CARTESIAN_POINT('Ctrl Pts',(7.60018554765108,2.19724567068834,141.447276443055));
#52632=CARTESIAN_POINT('Ctrl Pts',(7.57688385529471,2.27630098160028,141.450579816883));
#52633=CARTESIAN_POINT('Ctrl Pts',(7.55234669838382,2.3549905196011,141.45388319071));
#52634=CARTESIAN_POINT('Ctrl Pts',(7.49094694600511,2.55189671234343,141.462149280208));
#52635=CARTESIAN_POINT('Ctrl Pts',(7.42187718430449,2.74628883910267,141.470415369705));
#52636=CARTESIAN_POINT('Ctrl Pts',(7.34537794916531,2.93757447291402,141.478681459203));
#52637=CARTESIAN_POINT('Ctrl Pts',(7.2688099181583,3.12903213016004,141.486954982406));
#52638=CARTESIAN_POINT('Ctrl Pts',(7.18479918430057,3.3173774445395,141.495228505609));
#52639=CARTESIAN_POINT('Ctrl Pts',(7.09363354844675,3.50203998839974,141.503502028812));
#52640=CARTESIAN_POINT('Ctrl Pts',(7.00237999746393,3.6868806106687,141.511783530547));
#52641=CARTESIAN_POINT('Ctrl Pts',(6.90395789939115,3.86803110907492,141.520065032281));
#52642=CARTESIAN_POINT('Ctrl Pts',(6.79870031680055,4.0449468479,141.528346534015));
#52643=CARTESIAN_POINT('Ctrl Pts',(6.69326748260403,4.22215714761635,141.536641824271));
#52644=CARTESIAN_POINT('Ctrl Pts',(6.58097656085844,4.39511833855824,141.544937114527));
#52645=CARTESIAN_POINT('Ctrl Pts',(6.46220429556927,4.56331421691802,141.553232404783));
#52646=CARTESIAN_POINT('Ctrl Pts',(6.3433243150223,4.73166263309758,141.561535218087));
#52647=CARTESIAN_POINT('Ctrl Pts',(6.21795143252452,4.89523687451447,141.56983803139));
#52648=CARTESIAN_POINT('Ctrl Pts',(6.08650260589297,5.05355390081654,141.578140844693));
#52649=CARTESIAN_POINT('Ctrl Pts',(5.95485219994399,5.21211370933978,141.58645639052));
#52650=CARTESIAN_POINT('Ctrl Pts',(5.81710741786874,5.36539996611454,141.594771936348));
#52651=CARTESIAN_POINT('Ctrl Pts',(5.67372327611372,5.51296518999399,141.603087482176));
#52652=CARTESIAN_POINT('Ctrl Pts',(5.6167559600581,5.57159367320464,141.606391294729));
#52653=CARTESIAN_POINT('Ctrl Pts',(5.5588988433002,5.62931951606852,141.609695107281));
#52654=CARTESIAN_POINT('Ctrl Pts',(5.50018192174204,5.68611640997105,141.612998919833));
#52655=CARTESIAN_POINT('Ctrl Pts',(5.35960693167085,5.82209463540498,141.620908622938));
#52656=CARTESIAN_POINT('Ctrl Pts',(5.21380823078182,5.9530290277964,141.628818326043));
#52657=CARTESIAN_POINT('Ctrl Pts',(5.06318249909811,6.0784952069428,141.636728029148));
#52658=CARTESIAN_POINT('Ctrl Pts',(4.91270958456158,6.20383409453449,141.644629707473));
#52659=CARTESIAN_POINT('Ctrl Pts',(4.75741965684749,6.32371560087875,141.652531385799));
#52660=CARTESIAN_POINT('Ctrl Pts',(4.59774645335204,6.43775182425424,141.660433064124));
#52661=CARTESIAN_POINT('Ctrl Pts',(4.43820566629358,6.55169347778295,141.668328189615));
#52662=CARTESIAN_POINT('Ctrl Pts',(4.2742891239056,6.65979930613653,141.676223315106));
#52663=CARTESIAN_POINT('Ctrl Pts',(4.10646409668552,6.76172120266969,141.684118440597));
#52664=CARTESIAN_POINT('Ctrl Pts',(3.93874716471385,6.86357745182648,141.692008480877));
#52665=CARTESIAN_POINT('Ctrl Pts',(3.7671270571935,6.95925752679173,141.699898521158));
#52666=CARTESIAN_POINT('Ctrl Pts',(3.59210075453213,7.04845608408606,141.707788561438));
#52667=CARTESIAN_POINT('Ctrl Pts',(3.41715477667467,7.13761370549523,141.715674980744));
#52668=CARTESIAN_POINT('Ctrl Pts',(3.23880602511844,7.22029558053709,141.723561400049));
#52669=CARTESIAN_POINT('Ctrl Pts',(3.05757710271658,7.29624172166351,141.731447819354));
#52670=CARTESIAN_POINT('Ctrl Pts',(2.87639779930157,7.37216706936177,141.739332079422));
#52671=CARTESIAN_POINT('Ctrl Pts',(2.69234021429555,7.44136022585706,141.747216339491));
#52672=CARTESIAN_POINT('Ctrl Pts',(2.50594825825776,7.50360875358883,141.755100599559));
#52673=CARTESIAN_POINT('Ctrl Pts',(2.319534541058,7.56586454880319,141.762985780111));
#52674=CARTESIAN_POINT('Ctrl Pts',(2.13078623299568,7.62117397950423,141.770870960663));
#52675=CARTESIAN_POINT('Ctrl Pts',(1.94026439643537,7.66937383832118,141.778756141215));
#52676=CARTESIAN_POINT('Ctrl Pts',(1.74971879617863,7.71757970908317,141.786642305281));
#52677=CARTESIAN_POINT('Ctrl Pts',(1.55739956075781,7.75867415568526,141.794528469347));
#52678=CARTESIAN_POINT('Ctrl Pts',(1.36387996441368,7.79254467055986,141.802414633414));
#52679=CARTESIAN_POINT('Ctrl Pts',(1.17030376123954,7.82642509297104,141.810303104279));
#52680=CARTESIAN_POINT('Ctrl Pts',(0.975526836956832,7.85307731329363,141.818191575144));
#52681=CARTESIAN_POINT('Ctrl Pts',(0.780129887603958,7.87244043219554,141.826080046009));
#52682=CARTESIAN_POINT('Ctrl Pts',(0.584642997325844,7.89181246391229,141.833972147926));
#52683=CARTESIAN_POINT('Ctrl Pts',(0.38853585590506,7.903888674302,141.841864249842));
#52684=CARTESIAN_POINT('Ctrl Pts',(0.192391726586302,7.90866021672073,141.849756351759));
#52685=CARTESIAN_POINT('Ctrl Pts',(-0.00397979295669995,7.91343729079674,
141.857657603003));
#52686=CARTESIAN_POINT('Ctrl Pts',(-0.200388041431948,7.91089277349285,
141.865558854246));
#52687=CARTESIAN_POINT('Ctrl Pts',(-0.396251137986991,7.90106992980343,
141.87346010549));
#52688=CARTESIAN_POINT('Ctrl Pts',(-0.592244019158217,7.8912405772105,141.881366592334));
#52689=CARTESIAN_POINT('Ctrl Pts',(-0.787690686038262,7.87412331358912,
141.889273079178));
#52690=CARTESIAN_POINT('Ctrl Pts',(-0.982016658540009,7.84981300938754,
141.897179566022));
#52691=CARTESIAN_POINT('Ctrl Pts',(-1.1766103473169,7.82546921370768,141.905096945364));
#52692=CARTESIAN_POINT('Ctrl Pts',(-1.37007991889728,7.79391263904577,141.913014324705));
#52693=CARTESIAN_POINT('Ctrl Pts',(-1.56186215083803,7.75528900955855,141.920931704047));
#52694=CARTESIAN_POINT('Ctrl Pts',(-1.64501688368922,7.73854221524266,141.924364595391));
#52695=CARTESIAN_POINT('Ctrl Pts',(-1.72785460013434,7.72046744935075,141.927797486736));
#52696=CARTESIAN_POINT('Ctrl Pts',(-1.81033042285988,7.70107945421082,141.93123037808));
#52697=CARTESIAN_POINT('Ctrl Pts',(-1.99872689261025,7.65679217438513,141.93907200474));
#52698=CARTESIAN_POINT('Ctrl Pts',(-2.18579398331701,7.60551766755849,141.946913631401));
#52699=CARTESIAN_POINT('Ctrl Pts',(-2.37096792738509,7.5473460293875,141.954755258061));
#52700=CARTESIAN_POINT('Ctrl Pts',(-2.55592384308579,7.48924288393756,141.962587651797));
#52701=CARTESIAN_POINT('Ctrl Pts',(-2.73899071879854,7.42425888124231,141.970420045533));
#52702=CARTESIAN_POINT('Ctrl Pts',(-2.91961411751259,7.35253523655761,141.978252439268));
#52703=CARTESIAN_POINT('Ctrl Pts',(-3.10006000737474,7.28088207876393,141.986077135667));
#52704=CARTESIAN_POINT('Ctrl Pts',(-3.27806687800664,7.20250259767271,141.993901832065));
#52705=CARTESIAN_POINT('Ctrl Pts',(-3.45309443990792,7.11758805980488,142.001726528464));
#52706=CARTESIAN_POINT('Ctrl Pts',(-3.6279840440632,7.03274045207147,142.009545057391));
#52707=CARTESIAN_POINT('Ctrl Pts',(-3.79989870173604,6.94136819931556,142.017363586318));
#52708=CARTESIAN_POINT('Ctrl Pts',(-3.96831696336821,6.84371108962412,142.025182115245));
#52709=CARTESIAN_POINT('Ctrl Pts',(-4.13663522913849,6.74611196240298,142.032996002036));
#52710=CARTESIAN_POINT('Ctrl Pts',(-4.30146093070975,6.64223558726326,142.040809888827));
#52711=CARTESIAN_POINT('Ctrl Pts',(-4.46229598191233,6.53236829716521,142.048623775617));
#52712=CARTESIAN_POINT('Ctrl Pts',(-4.62306680863312,6.42254487915673,142.056434542175));
#52713=CARTESIAN_POINT('Ctrl Pts',(-4.77984986989528,6.30673551059833,142.064245308733));
#52714=CARTESIAN_POINT('Ctrl Pts',(-4.93217475456442,6.1852706642828,142.072056075291));
#52715=CARTESIAN_POINT('Ctrl Pts',(-5.08449358505963,6.06381064560464,142.079866531408));
#52716=CARTESIAN_POINT('Ctrl Pts',(-5.23235431136309,5.93669580913485,142.087676987526));
#52717=CARTESIAN_POINT('Ctrl Pts',(-5.3753180418017,5.8042981444341,142.095487443644));
#52718=CARTESIAN_POINT('Ctrl Pts',(-5.51828571490337,5.67189682846195,142.103298115159));
#52719=CARTESIAN_POINT('Ctrl Pts',(-5.65635586432456,5.53421263261948,142.111108786674));
#52720=CARTESIAN_POINT('Ctrl Pts',(-5.7891250794199,5.39165575819076,142.118919458189));
#52721=CARTESIAN_POINT('Ctrl Pts',(-5.92192133858203,5.2490698460244,142.126731720678));
#52722=CARTESIAN_POINT('Ctrl Pts',(-6.04941427261299,5.10160953561801,142.134543983166));
#52723=CARTESIAN_POINT('Ctrl Pts',(-6.17123942677439,4.94971968271187,142.142356245655));
#52724=CARTESIAN_POINT('Ctrl Pts',(-6.2931108524963,4.79777213908851,142.150171475393));
#52725=CARTESIAN_POINT('Ctrl Pts',(-6.40930999025035,4.64139197595457,142.157986705131));
#52726=CARTESIAN_POINT('Ctrl Pts',(-6.51951445051296,4.48105482331479,142.165801934868));
#52727=CARTESIAN_POINT('Ctrl Pts',(-6.62983876347712,4.32054329623628,142.173625664048));
#52728=CARTESIAN_POINT('Ctrl Pts',(-6.73415517823525,4.15606647454006,142.181449393227));
#52729=CARTESIAN_POINT('Ctrl Pts',(-6.83218565361493,3.98812740450181,142.189273122407));
#52730=CARTESIAN_POINT('Ctrl Pts',(-6.930275606398,3.82008644186562,142.197101598428));
#52731=CARTESIAN_POINT('Ctrl Pts',(-7.02207185368854,3.6485793538073,142.204930074448));
#52732=CARTESIAN_POINT('Ctrl Pts',(-7.10734360929572,3.47413123232317,142.212758550469));
#52733=CARTESIAN_POINT('Ctrl Pts',(-7.19273272273763,3.29944302133152,142.220597800667));
#52734=CARTESIAN_POINT('Ctrl Pts',(-7.2715792669835,3.12180601274751,142.228437050865));
#52735=CARTESIAN_POINT('Ctrl Pts',(-7.34370121033454,2.94176367734239,142.236276301063));
#52736=CARTESIAN_POINT('Ctrl Pts',(-7.38413732362819,2.84082058105531,142.240671479484));
#52737=CARTESIAN_POINT('Ctrl Pts',(-7.4224605075538,2.73912164949256,142.245066657906));
#52738=CARTESIAN_POINT('Ctrl Pts',(-7.45864566386742,2.63676427859446,142.249461836327));
#52739=CARTESIAN_POINT('Ctrl Pts',(-7.53540491871628,2.41963448508658,142.25878528978));
#52740=CARTESIAN_POINT('Ctrl Pts',(-7.60272127187402,2.19903128111711,142.268108743232));
#52741=CARTESIAN_POINT('Ctrl Pts',(-7.66031837808705,1.97571337656599,142.277432196685));
#52742=CARTESIAN_POINT('Ctrl Pts',(-7.71768456206012,1.75329081336332,142.286718269913));
#52743=CARTESIAN_POINT('Ctrl Pts',(-7.76540921234219,1.5281753369818,142.296004343141));
#52744=CARTESIAN_POINT('Ctrl Pts',(-7.80326604226389,1.30113799177921,142.30529041637));
#52745=CARTESIAN_POINT('Ctrl Pts',(-7.840801781141,1.0760263138468,142.314497727721));
#52746=CARTESIAN_POINT('Ctrl Pts',(-7.86863633167718,0.849025309717781,
142.323705039073));
#52747=CARTESIAN_POINT('Ctrl Pts',(-7.88659597041506,0.620906594773285,
142.332912350425));
#52748=CARTESIAN_POINT('Ctrl Pts',(-7.90269228554174,0.416455337393836,
142.341164397538));
#52749=CARTESIAN_POINT('Ctrl Pts',(-7.91085699332149,0.211106556477672,
142.34941644465));
#52750=CARTESIAN_POINT('Ctrl Pts',(-7.91099813726446,0.00542883029005868,
142.357668491763));
#52751=CARTESIAN_POINT('',(-7.90415356074214,-0.00309866779400792,144.357668491763));
#52752=CARTESIAN_POINT('Ctrl Pts',(-7.911,-6.69464483848969E-13,142.357668491763));
#52753=CARTESIAN_POINT('Ctrl Pts',(-7.91099999999981,-2.20167589666747,
142.446255927496));
#52754=CARTESIAN_POINT('Ctrl Pts',(-6.94214576672331,-4.38610418338747,
142.534843363229));
#52755=CARTESIAN_POINT('Ctrl Pts',(-3.67820201488214,-7.34180684107669,
142.712018234694));
#52756=CARTESIAN_POINT('Ctrl Pts',(-1.4086817587166,-8.08992666571352,142.800605670427));
#52757=CARTESIAN_POINT('Ctrl Pts',(2.97309270521359,-7.65454228025225,142.977780541892));
#52758=CARTESIAN_POINT('Ctrl Pts',(5.05102072675677,-6.47444880834168,143.066367977625));
#52759=CARTESIAN_POINT('Ctrl Pts',(7.66951518847908,-2.93425195367614,143.24354284909));
#52760=CARTESIAN_POINT('Ctrl Pts',(8.1895687224708,-0.601881960098144,143.332130284823));
#52761=CARTESIAN_POINT('Ctrl Pts',(7.32306689761295,3.71537198232546,143.509305156288));
#52762=CARTESIAN_POINT('Ctrl Pts',(5.94329958850125,5.66643518936592,143.597892592021));
#52763=CARTESIAN_POINT('Ctrl Pts',(2.16154501637735,7.92205913233029,143.775067463487));
#52764=CARTESIAN_POINT('Ctrl Pts',(-0.210816529301569,8.20894963713,143.863654899219));
#52765=CARTESIAN_POINT('Ctrl Pts',(-4.42123908576543,6.91982244717764,144.040829770685));
#52766=CARTESIAN_POINT('Ctrl Pts',(-6.22631625634273,5.35390358803423,144.129417206418));
#52767=CARTESIAN_POINT('Ctrl Pts',(-7.65317280859508,2.31334857514433,144.264559258688));
#52768=CARTESIAN_POINT('Ctrl Pts',(-7.91100000000001,1.15702837836474,144.311113875225));
#52769=CARTESIAN_POINT('Ctrl Pts',(-7.911,-4.82947015711943E-14,144.357668491763));
#52770=CARTESIAN_POINT('',(-7.91789235578852,-0.0010059796957165,146.357631904486));
#52771=CARTESIAN_POINT('Ctrl Pts',(-7.90105610939419,-0.00450056042370127,
144.357668491763));
#52772=CARTESIAN_POINT('Ctrl Pts',(-7.90689325060477,-0.997333501851549,
144.397473009194));
#52773=CARTESIAN_POINT('Ctrl Pts',(-7.27322451497355,-4.62900481828023,
144.543354679371));
#52774=CARTESIAN_POINT('Ctrl Pts',(-1.82054063441708,-9.17431691246998,
144.795313502303));
#52775=CARTESIAN_POINT('Ctrl Pts',(6.73662521562475,-6.49815555119431,145.113544960548));
#52776=CARTESIAN_POINT('Ctrl Pts',(9.10643661084831,2.16675378454077,145.431776418795));
#52777=CARTESIAN_POINT('Ctrl Pts',(4.10254492915994,7.70430850903412,145.696969300668));
#52778=CARTESIAN_POINT('Ctrl Pts',(-1.32366529678204,8.11696492869233,145.909123606165));
#52779=CARTESIAN_POINT('Ctrl Pts',(-6.11008896738171,6.09778331381346,146.111649179355));
#52780=CARTESIAN_POINT('Ctrl Pts',(-7.9048743251548,2.38505523999662,146.261136176172));
#52781=CARTESIAN_POINT('Ctrl Pts',(-7.92202559494964,-0.000978787874874063,
146.357584596613));
#52782=CARTESIAN_POINT('',(-7.91099987608327,0.00138933783038613,148.357612589845));
#52783=CARTESIAN_POINT('Ctrl Pts',(-7.91099992636282,-0.00105132372223101,
146.357710793261));
#52784=CARTESIAN_POINT('Ctrl Pts',(-7.91069155732802,-2.20237127150424,
146.446284128495));
#52785=CARTESIAN_POINT('Ctrl Pts',(-6.94188600507358,-4.3863394136048,146.534857463728));
#52786=CARTESIAN_POINT('Ctrl Pts',(-3.67820201488245,-7.34180684107653,
146.712018234694));
#52787=CARTESIAN_POINT('Ctrl Pts',(-1.40868175871695,-8.08992666571346,
146.800605670427));
#52788=CARTESIAN_POINT('Ctrl Pts',(2.97309270521326,-7.65454228025238,146.977780541892));
#52789=CARTESIAN_POINT('Ctrl Pts',(5.05102072675649,-6.4744488083419,147.066367977625));
#52790=CARTESIAN_POINT('Ctrl Pts',(7.66951518847895,-2.93425195367647,147.24354284909));
#52791=CARTESIAN_POINT('Ctrl Pts',(8.18956872247077,-0.601881960098497,
147.332130284823));
#52792=CARTESIAN_POINT('Ctrl Pts',(7.32306689761311,3.71537198232515,147.509305156288));
#52793=CARTESIAN_POINT('Ctrl Pts',(5.9432995885015,5.66643518936566,147.597892592021));
#52794=CARTESIAN_POINT('Ctrl Pts',(2.16154501637769,7.9220591323302,147.775067463487));
#52795=CARTESIAN_POINT('Ctrl Pts',(-0.210816529301215,8.20894963713001,
147.863654899219));
#52796=CARTESIAN_POINT('Ctrl Pts',(-4.42123908576514,6.91982244717783,148.040829770685));
#52797=CARTESIAN_POINT('Ctrl Pts',(-6.22631625634249,5.3539035880345,148.129417206418));
#52798=CARTESIAN_POINT('Ctrl Pts',(-7.65297606741948,2.31376782006909,148.264540624715));
#52799=CARTESIAN_POINT('Ctrl Pts',(-7.91079356649125,1.1579540194574,148.311076607279));
#52800=CARTESIAN_POINT('Ctrl Pts',(-7.91099987608327,0.00138933783038613,
148.357612589845));
#52801=CARTESIAN_POINT('',(-7.911,1.33226762955019E-14,150.357668491763));
#52802=CARTESIAN_POINT('Ctrl Pts',(-7.9109998762523,0.00139926271889242,
148.357864421896));
#52803=CARTESIAN_POINT('Ctrl Pts',(-7.91103419945879,-0.192653561413069,
148.365678114097));
#52804=CARTESIAN_POINT('Ctrl Pts',(-7.90392420100454,-0.386895670116855,
148.373491806299));
#52805=CARTESIAN_POINT('Ctrl Pts',(-7.88965428496979,-0.580754908423348,
148.381305498501));
#52806=CARTESIAN_POINT('Ctrl Pts',(-7.87539373648693,-0.774486886942986,
148.389114061368));
#52807=CARTESIAN_POINT('Ctrl Pts',(-7.85398265784157,-0.96783614515552,
148.396922624236));
#52808=CARTESIAN_POINT('Ctrl Pts',(-7.82545752325939,-1.16023081826982,
148.404731187104));
#52809=CARTESIAN_POINT('Ctrl Pts',(-7.79694553304693,-1.3525368360016,148.412536151789));
#52810=CARTESIAN_POINT('Ctrl Pts',(-7.76132606900809,-1.54388879662352,
148.420341116474));
#52811=CARTESIAN_POINT('Ctrl Pts',(-7.71868743478577,-1.73372007085349,
148.428146081159));
#52812=CARTESIAN_POINT('Ctrl Pts',(-7.67605352254792,-1.92353032235738,
148.435950181489));
#52813=CARTESIAN_POINT('Ctrl Pts',(-7.62640205757169,-2.11181987705395,
148.443754281819));
#52814=CARTESIAN_POINT('Ctrl Pts',(-7.56987252230388,-2.29803198325627,
148.451558382149));
#52815=CARTESIAN_POINT('Ctrl Pts',(-7.51334441660939,-2.48423938034751,
148.459362285122));
#52816=CARTESIAN_POINT('Ctrl Pts',(-7.44993868850091,-2.66836909545884,
148.467166188094));
#52817=CARTESIAN_POINT('Ctrl Pts',(-7.37984479689068,-2.84987925600464,
148.474970091067));
#52818=CARTESIAN_POINT('Ctrl Pts',(-7.30974025646079,-3.0314169919771,148.482775179626));
#52819=CARTESIAN_POINT('Ctrl Pts',(-7.23294565545322,-3.21033405121888,
148.490580268184));
#52820=CARTESIAN_POINT('Ctrl Pts',(-7.14969877825737,-3.38610814655779,
148.498385356743));
#52821=CARTESIAN_POINT('Ctrl Pts',(-7.06642450048534,-3.56194009765841,
148.506193014334));
#52822=CARTESIAN_POINT('Ctrl Pts',(-6.97669386727089,-3.73462670542988,
148.514000671925));
#52823=CARTESIAN_POINT('Ctrl Pts',(-6.88079088311935,-3.90366978915758,
148.521808329517));
#52824=CARTESIAN_POINT('Ctrl Pts',(-6.7847833043722,-4.07289723620974,148.529624502367));
#52825=CARTESIAN_POINT('Ctrl Pts',(-6.68259010082437,-4.23847291350021,
148.537440675218));
#52826=CARTESIAN_POINT('Ctrl Pts',(-6.57453954467923,-4.39992622386434,
148.545256848068));
#52827=CARTESIAN_POINT('Ctrl Pts',(-6.46642820732519,-4.56147035585617,
148.553077417717));
#52828=CARTESIAN_POINT('Ctrl Pts',(-6.35245315740072,-4.71888721416122,
148.560897987365));
#52829=CARTESIAN_POINT('Ctrl Pts',(-6.23298335758991,-4.8717388542498,148.568718557013));
#52830=CARTESIAN_POINT('Ctrl Pts',(-6.11333400357754,-5.02482021895698,
148.576550880394));
#52831=CARTESIAN_POINT('Ctrl Pts',(-5.98817362538431,-5.17332238601346,
148.584383203776));
#52832=CARTESIAN_POINT('Ctrl Pts',(-5.85790945201707,-5.31684284627345,
148.592215527157));
#52833=CARTESIAN_POINT('Ctrl Pts',(-5.73663464364711,-5.45045914203059,
148.599507351859));
#52834=CARTESIAN_POINT('Ctrl Pts',(-5.61093668500354,-5.57975779986694,
148.606799176561));
#52835=CARTESIAN_POINT('Ctrl Pts',(-5.48116956406796,-5.70444574081786,
148.614091001264));
#52836=CARTESIAN_POINT('Ctrl Pts',(-5.34161801288141,-5.83853514226644,
148.621932628949));
#52837=CARTESIAN_POINT('Ctrl Pts',(-5.19692320930869,-5.96771174700591,
148.629774256634));
#52838=CARTESIAN_POINT('Ctrl Pts',(-5.04746713421435,-6.09155124159898,
148.637615884319));
#52839=CARTESIAN_POINT('Ctrl Pts',(-4.89818703230537,-6.21524492458603,
148.645448279083));
#52840=CARTESIAN_POINT('Ctrl Pts',(-4.74415708910208,-6.33361378810063,
148.653280673847));
#52841=CARTESIAN_POINT('Ctrl Pts',(-4.58579712909097,-6.44626912956798,
148.661113068611));
#52842=CARTESIAN_POINT('Ctrl Pts',(-4.42759279831991,-6.55881375829469,
148.668937766039));
#52843=CARTESIAN_POINT('Ctrl Pts',(-4.26506720917366,-6.66565584445674,
148.676762463468));
#52844=CARTESIAN_POINT('Ctrl Pts',(-4.09867451543366,-6.76644575952062,
148.684587160897));
#52845=CARTESIAN_POINT('Ctrl Pts',(-3.93241297333208,-6.86715623141787,
148.692405690856));
#52846=CARTESIAN_POINT('Ctrl Pts',(-3.76229069666347,-6.96182385190315,
148.700224220816));
#52847=CARTESIAN_POINT('Ctrl Pts',(-3.58879233452092,-7.05014117445061,
148.708042750775));
#52848=CARTESIAN_POINT('Ctrl Pts',(-3.41539698444037,-7.13840605990649,
148.715856638599));
#52849=CARTESIAN_POINT('Ctrl Pts',(-3.23862985429503,-7.22032799885895,
148.723670526422));
#52850=CARTESIAN_POINT('Ctrl Pts',(-3.05900197109044,-7.29564445000336,
148.731484414246));
#52851=CARTESIAN_POINT('Ctrl Pts',(-2.87944581668535,-7.37093082586921,
148.739295181837));
#52852=CARTESIAN_POINT('Ctrl Pts',(-2.69703150909478,-7.43961683337175,
148.747105949429));
#52853=CARTESIAN_POINT('Ctrl Pts',(-2.5122920913392,-7.50148714907881,148.75491671702));
#52854=CARTESIAN_POINT('Ctrl Pts',(-2.32756001612867,-7.56335500572442,
148.762727174169));
#52855=CARTESIAN_POINT('Ctrl Pts',(-2.14050334543881,-7.61840758997842,
148.770537631317));
#52856=CARTESIAN_POINT('Ctrl Pts',(-1.95167284726542,-7.66647859823837,
148.778348088466));
#52857=CARTESIAN_POINT('Ctrl Pts',(-1.76283714154313,-7.71455093219584,
148.786158761011));
#52858=CARTESIAN_POINT('Ctrl Pts',(-1.57222785179897,-7.75564121901117,
148.793969433556));
#52859=CARTESIAN_POINT('Ctrl Pts',(-1.38040854380454,-7.78963370462254,
148.801780106101));
#52860=CARTESIAN_POINT('Ctrl Pts',(-1.18855016374411,-7.82363311423261,
148.809592369618));
#52861=CARTESIAN_POINT('Ctrl Pts',(-0.99548162096845,-7.85053178116441,
148.817404633135));
#52862=CARTESIAN_POINT('Ctrl Pts',(-0.801774404552212,-7.87026548498873,
148.825216896651));
#52863=CARTESIAN_POINT('Ctrl Pts',(-0.607993614441421,-7.89000668405007,
148.833032127415));
#52864=CARTESIAN_POINT('Ctrl Pts',(-0.413574017275125,-7.9025774635303,
148.840847358178));
#52865=CARTESIAN_POINT('Ctrl Pts',(-0.219090078518901,-7.90796563836077,
148.848662588941));
#52866=CARTESIAN_POINT('Ctrl Pts',(-0.024394629273337,-7.91335967308641,
148.856486319138));
#52867=CARTESIAN_POINT('Ctrl Pts',(0.170364949480691,-7.91155549173148,
148.864310049335));
#52868=CARTESIAN_POINT('Ctrl Pts',(0.364615275489833,-7.90259303652159,
148.872133779532));
#52869=CARTESIAN_POINT('Ctrl Pts',(0.558983457666191,-7.89362514358275,
148.879962256567));
#52870=CARTESIAN_POINT('Ctrl Pts',(0.752841421771199,-7.87749035052994,
148.887790733602));
#52871=CARTESIAN_POINT('Ctrl Pts',(0.945622956665146,-7.85428024861781,
148.895619210637));
#52872=CARTESIAN_POINT('Ctrl Pts',(1.13866981262137,-7.83103820314377,148.903458461835));
#52873=CARTESIAN_POINT('Ctrl Pts',(1.33063693402655,-7.80070145415603,148.911297713034));
#52874=CARTESIAN_POINT('Ctrl Pts',(1.52096917400047,-7.76341250815261,148.919136964233));
#52875=CARTESIAN_POINT('Ctrl Pts',(1.62768110296808,-7.74250603766847,148.923532129325));
#52876=CARTESIAN_POINT('Ctrl Pts',(1.73387939145228,-7.71941510618414,148.927927294418));
#52877=CARTESIAN_POINT('Ctrl Pts',(1.83946864032763,-7.694171568223,148.93232245951));
#52878=CARTESIAN_POINT('Ctrl Pts',(2.02949528431883,-7.64874132932735,148.940232341256));
#52879=CARTESIAN_POINT('Ctrl Pts',(2.21809443601166,-7.59620580985692,148.948142223003));
#52880=CARTESIAN_POINT('Ctrl Pts',(2.40469524067325,-7.53666781804024,148.956052104749));
#52881=CARTESIAN_POINT('Ctrl Pts',(2.59109317887584,-7.47719455403434,148.963953387123));
#52882=CARTESIAN_POINT('Ctrl Pts',(2.77549677173073,-7.41073408516476,148.971854669498));
#52883=CARTESIAN_POINT('Ctrl Pts',(2.95734563337055,-7.33744013977519,148.979755951872));
#52884=CARTESIAN_POINT('Ctrl Pts',(3.13903058666945,-7.26421225742764,148.987650112475));
#52885=CARTESIAN_POINT('Ctrl Pts',(3.31816507795086,-7.1841632964965,148.995544273078));
#52886=CARTESIAN_POINT('Ctrl Pts',(3.49420389537122,-7.09749675150138,149.003438433681));
#52887=CARTESIAN_POINT('Ctrl Pts',(3.67011674338177,-7.01089222313237,149.0113269454));
#52888=CARTESIAN_POINT('Ctrl Pts',(3.84293802269998,-6.91767969689486,149.019215457119));
#52889=CARTESIAN_POINT('Ctrl Pts',(4.01214227058525,-6.81811083809753,149.027103968839));
#52890=CARTESIAN_POINT('Ctrl Pts',(4.18125686511461,-6.71859473614554,149.034988300808));
#52891=CARTESIAN_POINT('Ctrl Pts',(4.34675795045919,-6.61272918715504,149.042872632776));
#52892=CARTESIAN_POINT('Ctrl Pts',(4.50814421646872,-6.50081200493597,149.050756964745));
#52893=CARTESIAN_POINT('Ctrl Pts',(4.66947494000625,-6.38893333997808,149.058638583253));
#52894=CARTESIAN_POINT('Ctrl Pts',(4.8266933834927,-6.27100738904184,149.066520201762));
#52895=CARTESIAN_POINT('Ctrl Pts',(4.97932658136968,-6.1473756836609,149.07440182027));
#52896=CARTESIAN_POINT('Ctrl Pts',(5.13196177866581,-6.02374235876598,149.082283542023));
#52897=CARTESIAN_POINT('Ctrl Pts',(5.28001133691194,-5.89440334054266,149.090165263777));
#52898=CARTESIAN_POINT('Ctrl Pts',(5.4230343537672,-5.75974126136416,149.09804698553));
#52899=CARTESIAN_POINT('Ctrl Pts',(5.56606598655101,-5.62507106993297,149.105929182091));
#52900=CARTESIAN_POINT('Ctrl Pts',(5.70407022283161,-5.48507741474963,149.113811378651));
#52901=CARTESIAN_POINT('Ctrl Pts',(5.83664209074272,-5.34018071834375,149.121693575212));
#52902=CARTESIAN_POINT('Ctrl Pts',(5.9692442529349,-5.19525091128389,149.12957757295));
#52903=CARTESIAN_POINT('Ctrl Pts',(6.09641134020214,-5.04541608503013,149.137461570688));
#52904=CARTESIAN_POINT('Ctrl Pts',(6.21777768138167,-4.89113092289626,149.145345568426));
#52905=CARTESIAN_POINT('Ctrl Pts',(6.33919217889602,-4.7367845427356,149.153232694416));
#52906=CARTESIAN_POINT('Ctrl Pts',(6.45480113091654,-4.57798457913831,149.161119820406));
#52907=CARTESIAN_POINT('Ctrl Pts',(6.56428118224404,-4.41521613971919,149.169006946395));
#52908=CARTESIAN_POINT('Ctrl Pts',(6.67387803675808,-4.25227404425806,149.176902487082));
#52909=CARTESIAN_POINT('Ctrl Pts',(6.77733273705257,-4.08535530243727,149.184798027768));
#52910=CARTESIAN_POINT('Ctrl Pts',(6.87436646860418,-3.91497211424685,149.192693568455));
#52911=CARTESIAN_POINT('Ctrl Pts',(6.97145929053952,-3.74448516824141,149.200593917269));
#52912=CARTESIAN_POINT('Ctrl Pts',(7.0621231892713,-3.57052987500456,149.208494266083));
#52913=CARTESIAN_POINT('Ctrl Pts',(7.14612670179428,-3.39364025228114,149.216394614896));
#52914=CARTESIAN_POINT('Ctrl Pts',(7.23023959088703,-3.21652031085342,149.22430525034));
#52915=CARTESIAN_POINT('Ctrl Pts',(7.30767463577674,-3.03645872443077,149.232215885784));
#52916=CARTESIAN_POINT('Ctrl Pts',(7.37824920807456,-2.85400764251731,149.240126521228));
#52917=CARTESIAN_POINT('Ctrl Pts',(7.40925847635465,-2.77384173625897,149.243602320071));
#52918=CARTESIAN_POINT('Ctrl Pts',(7.43894393371744,-2.69321469837884,149.247078118914));
#52919=CARTESIAN_POINT('Ctrl Pts',(7.4672931863409,-2.61217408861408,149.250553917757));
#52920=CARTESIAN_POINT('Ctrl Pts',(7.53180750577824,-2.42775018667901,149.258463784018));
#52921=CARTESIAN_POINT('Ctrl Pts',(7.58957260064992,-2.24068595604946,149.26637365028));
#52922=CARTESIAN_POINT('Ctrl Pts',(7.64036635717733,-2.05151722588741,149.274283516541));
#52923=CARTESIAN_POINT('Ctrl Pts',(7.69110491135422,-1.86255408316886,149.282184786407));
#52924=CARTESIAN_POINT('Ctrl Pts',(7.73488712950447,-1.67149132670043,149.290086056273));
#52925=CARTESIAN_POINT('Ctrl Pts',(7.77153939559275,-1.47888350546954,149.29798732614));
#52926=CARTESIAN_POINT('Ctrl Pts',(7.80815863908356,-1.28644921813513,149.305881477197));
#52927=CARTESIAN_POINT('Ctrl Pts',(7.83766066325707,-1.09247297585826,149.313775628255));
#52928=CARTESIAN_POINT('Ctrl Pts',(7.85992192259556,-0.897523465265205,
149.321669779313));
#52929=CARTESIAN_POINT('Ctrl Pts',(7.88216726058491,-0.702713383406976,
149.32955828444));
#52930=CARTESIAN_POINT('Ctrl Pts',(7.89718211228078,-0.506931761396544,
149.337446789567));
#52931=CARTESIAN_POINT('Ctrl Pts',(7.90489413375551,-0.31075671210399,149.345335294693));
#52932=CARTESIAN_POINT('Ctrl Pts',(7.91260207186756,-0.114685533616116,
149.353219623013));
#52933=CARTESIAN_POINT('Ctrl Pts',(7.91301487111404,0.0817783131925406,
149.361103951332));
#52934=CARTESIAN_POINT('Ctrl Pts',(7.90611206832419,0.278052087024499,149.368988279652));
#52935=CARTESIAN_POINT('Ctrl Pts',(7.89921163862408,0.474258384601366,149.376869897447));
#52936=CARTESIAN_POINT('Ctrl Pts',(7.88500063145307,0.670274395096636,149.384751515241));
#52937=CARTESIAN_POINT('Ctrl Pts',(7.86351068558139,0.865517589507741,149.392633133036));
#52938=CARTESIAN_POINT('Ctrl Pts',(7.84202044625025,1.06076345009417,149.400514858459));
#52939=CARTESIAN_POINT('Ctrl Pts',(7.81325109885063,1.25523612970774,149.408396583882));
#52940=CARTESIAN_POINT('Ctrl Pts',(7.77728619285518,1.44835785440759,149.416278309306));
#52941=CARTESIAN_POINT('Ctrl Pts',(7.74131910781728,1.64149127997037,149.424160512267));
#52942=CARTESIAN_POINT('Ctrl Pts',(7.6981556580643,1.8332732480634,149.432042715229));
#52943=CARTESIAN_POINT('Ctrl Pts',(7.64793060912958,2.0231357833667,149.43992491819));
#52944=CARTESIAN_POINT('Ctrl Pts',(7.59769406577727,2.21304177028056,149.447808925059));
#52945=CARTESIAN_POINT('Ctrl Pts',(7.54039279115692,2.40102711545622,149.455692931928));
#52946=CARTESIAN_POINT('Ctrl Pts',(7.47621161956474,2.58653838546526,149.463576938796));
#52947=CARTESIAN_POINT('Ctrl Pts',(7.41200495965826,2.77212332769681,149.471464076646));
#52948=CARTESIAN_POINT('Ctrl Pts',(7.34091307133737,2.95523191113743,149.479351214496));
#52949=CARTESIAN_POINT('Ctrl Pts',(7.26316926010277,3.1353298549113,149.487238352346));
#52950=CARTESIAN_POINT('Ctrl Pts',(7.18534246476197,3.31562003606917,149.495133908964));
#52951=CARTESIAN_POINT('Ctrl Pts',(7.1008497010102,3.49289284179275,149.503029465582));
#52952=CARTESIAN_POINT('Ctrl Pts',(7.00997114524581,3.6666368163238,149.5109250222));
#52953=CARTESIAN_POINT('Ctrl Pts',(6.91903722050739,3.84048664669217,149.518825389291));
#52954=CARTESIAN_POINT('Ctrl Pts',(6.82170991802717,4.01080306080901,149.526725756382));
#52955=CARTESIAN_POINT('Ctrl Pts',(6.71831336699858,4.17710264451427,149.534626123473));
#52956=CARTESIAN_POINT('Ctrl Pts',(6.61478214377821,4.34361883050665,149.542536780653));
#52957=CARTESIAN_POINT('Ctrl Pts',(6.50516607441492,4.50610745061167,149.550447437833));
#52958=CARTESIAN_POINT('Ctrl Pts',(6.389830941801,4.66411637239065,149.558358095014));
#52959=CARTESIAN_POINT('Ctrl Pts',(6.33915534438178,4.73354184862885,149.561833855344));
#52960=CARTESIAN_POINT('Ctrl Pts',(6.28737617348114,4.80210296382564,149.565309615674));
#52961=CARTESIAN_POINT('Ctrl Pts',(6.23452673857495,4.86976358214585,149.568785376004));
#52962=CARTESIAN_POINT('Ctrl Pts',(6.11533612381838,5.0223576582549,149.576624211201));
#52963=CARTESIAN_POINT('Ctrl Pts',(5.99035983087738,5.17080368396709,149.584463046398));
#52964=CARTESIAN_POINT('Ctrl Pts',(5.85991829096024,5.31462873804649,149.592301881595));
#52965=CARTESIAN_POINT('Ctrl Pts',(5.72962297355157,5.45829256695022,149.600131929605));
#52966=CARTESIAN_POINT('Ctrl Pts',(5.59387484196166,5.59734548090741,149.607961977615));
#52967=CARTESIAN_POINT('Ctrl Pts',(5.45303667253296,5.73134469806264,149.615792025626));
#52968=CARTESIAN_POINT('Ctrl Pts',(5.31232896916856,5.86521978444739,149.623614820236));
#52969=CARTESIAN_POINT('Ctrl Pts',(5.1665408709855,5.99405025634176,149.631437614847));
#52970=CARTESIAN_POINT('Ctrl Pts',(5.01607448712298,6.11742737918759,149.639260409458));
#52971=CARTESIAN_POINT('Ctrl Pts',(4.86571821943737,6.24071421065578,149.647077479094));
#52972=CARTESIAN_POINT('Ctrl Pts',(4.71069075588652,6.35855541988836,149.654894548729));
#52973=CARTESIAN_POINT('Ctrl Pts',(4.55143016125698,6.47057991892537,149.662711618365));
#52974=CARTESIAN_POINT('Ctrl Pts',(4.39225515036246,6.58254421804248,149.670524487251));
#52975=CARTESIAN_POINT('Ctrl Pts',(4.22885182680198,6.68869783176658,149.678337356136));
#52976=CARTESIAN_POINT('Ctrl Pts',(4.06169050093677,6.78871057525654,149.686150225022));
#52977=CARTESIAN_POINT('Ctrl Pts',(3.89458650789091,6.88868901647876,149.693960414258));
#52978=CARTESIAN_POINT('Ctrl Pts',(3.72372738211049,6.98253060354984,149.701770603493));
#52979=CARTESIAN_POINT('Ctrl Pts',(3.54961167158209,7.06994893764928,149.709580792729));
#52980=CARTESIAN_POINT('Ctrl Pts',(3.3754881087995,7.15737121413266,149.717391334188));
#52981=CARTESIAN_POINT('Ctrl Pts',(3.19810797807609,7.23836949280769,149.725201875647));
#52982=CARTESIAN_POINT('Ctrl Pts',(3.01799410288058,7.3127035079359,149.733012417106));
#52983=CARTESIAN_POINT('Ctrl Pts',(2.83786579167468,7.38704348088726,149.740823584575));
#52984=CARTESIAN_POINT('Ctrl Pts',(2.65500362462042,7.45471799120727,149.748634752044));
#52985=CARTESIAN_POINT('Ctrl Pts',(2.46994997758998,7.5155351178877,149.756445919512));
#52986=CARTESIAN_POINT('Ctrl Pts',(2.28484890716228,7.5763678300743,149.764259088736));
#52987=CARTESIAN_POINT('Ctrl Pts',(2.09755557226844,7.63033954788241,149.77207225796));
#52988=CARTESIAN_POINT('Ctrl Pts',(1.90862720427759,7.67730833007842,149.779885427184));
#52989=CARTESIAN_POINT('Ctrl Pts',(1.71961714309979,7.72429742171523,149.787701974846));
#52990=CARTESIAN_POINT('Ctrl Pts',(1.5289709816044,7.76427746084871,149.795518522507));
#52991=CARTESIAN_POINT('Ctrl Pts',(1.33725597278598,7.79715765284044,149.803335070169));
#52992=CARTESIAN_POINT('Ctrl Pts',(1.14531723083956,7.83007621630996,149.811160739811));
#52993=CARTESIAN_POINT('Ctrl Pts',(0.952307497086017,7.85587832441459,149.818986409454));
#52994=CARTESIAN_POINT('Ctrl Pts',(0.758800081773679,7.8745249657297,149.826812079096));
#52995=CARTESIAN_POINT('Ctrl Pts',(0.565166532832405,7.89318376145518,149.834642849732));
#52996=CARTESIAN_POINT('Ctrl Pts',(0.37103500582103,7.90467777492654,149.842473620369));
#52997=CARTESIAN_POINT('Ctrl Pts',(0.176978712829425,7.90902013748892,149.850304391005));
#52998=CARTESIAN_POINT('Ctrl Pts',(-0.0173579684307403,7.91336877424886,
149.858146476173));
#52999=CARTESIAN_POINT('Ctrl Pts',(-0.211618848159001,7.91054512626607,
149.865988561342));
#53000=CARTESIAN_POINT('Ctrl Pts',(-0.40523472985427,7.90061426812624,149.873830646511));
#53001=CARTESIAN_POINT('Ctrl Pts',(-0.513754139792657,7.89504813968636,
149.878226042424));
#53002=CARTESIAN_POINT('Ctrl Pts',(-0.622071072280622,7.88725023103341,
149.882621438338));
#53003=CARTESIAN_POINT('Ctrl Pts',(-0.730086817096597,7.87723899850079,
149.887016834251));
#53004=CARTESIAN_POINT('Ctrl Pts',(-0.924632870215468,7.85920786998898,
149.894933336871));
#53005=CARTESIAN_POINT('Ctrl Pts',(-1.11878517603069,7.83393988467338,149.902849839492));
#53006=CARTESIAN_POINT('Ctrl Pts',(-1.31196385325694,7.80145318820457,149.910766342112));
#53007=CARTESIAN_POINT('Ctrl Pts',(-1.50491997773897,7.76900391824449,149.918673724474));
#53008=CARTESIAN_POINT('Ctrl Pts',(-1.69690437138156,7.72935255834266,149.926581106836));
#53009=CARTESIAN_POINT('Ctrl Pts',(-1.88734000174799,7.68256914826036,149.934488489198));
#53010=CARTESIAN_POINT('Ctrl Pts',(-2.0775915287638,7.63583096596728,149.942388227111));
#53011=CARTESIAN_POINT('Ctrl Pts',(-2.26629694287303,7.58197455009893,149.950287965023));
#53012=CARTESIAN_POINT('Ctrl Pts',(-2.4528868795594,7.52112138953264,149.958187702936));
#53013=CARTESIAN_POINT('Ctrl Pts',(-2.63933099515242,7.46031578605632,149.966081267158));
#53014=CARTESIAN_POINT('Ctrl Pts',(-2.82366260106464,7.39252443812066,149.973974831381));
#53015=CARTESIAN_POINT('Ctrl Pts',(-3.00532475653873,7.31791938379588,149.981868395604));
#53016=CARTESIAN_POINT('Ctrl Pts',(-3.18687858504193,7.24335881721554,149.989757252814));
#53017=CARTESIAN_POINT('Ctrl Pts',(-3.36576581712271,7.16199277082344,149.997646110025));
#53018=CARTESIAN_POINT('Ctrl Pts',(-3.54144658530784,7.07404248527046,150.005534967236));
#53019=CARTESIAN_POINT('Ctrl Pts',(-3.71705512255395,6.98612836037284,150.013420580953));
#53020=CARTESIAN_POINT('Ctrl Pts',(-3.8894595156393,6.89163554546707,150.021306194669));
#53021=CARTESIAN_POINT('Ctrl Pts',(-4.05814147153863,6.79083270276763,150.029191808386));
#53022=CARTESIAN_POINT('Ctrl Pts',(-4.22680842775133,6.69003882374805,150.037076720891));
#53023=CARTESIAN_POINT('Ctrl Pts',(-4.3917533072821,6.58293620598582,150.044961633396));
#53024=CARTESIAN_POINT('Ctrl Pts',(-4.5524835030535,6.46983886618714,150.052846545901));
#53025=CARTESIAN_POINT('Ctrl Pts',(-4.7132131450218,6.35674191607042,150.060731431238));
#53026=CARTESIAN_POINT('Ctrl Pts',(-4.86972784991524,6.23765048298116,150.068616316575));
#53027=CARTESIAN_POINT('Ctrl Pts',(-5.02156494712211,6.11292127234063,150.076501201912));
#53028=CARTESIAN_POINT('Ctrl Pts',(-5.1734269962266,5.98817156453206,150.084387382999));
#53029=CARTESIAN_POINT('Ctrl Pts',(-5.32060963964438,5.85778245193239,150.092273564086));
#53030=CARTESIAN_POINT('Ctrl Pts',(-5.46268399640442,5.72215034365815,150.100159745172));
#53031=CARTESIAN_POINT('Ctrl Pts',(-5.60480553789616,5.58647319020626,150.108048545362));
#53032=CARTESIAN_POINT('Ctrl Pts',(-5.74181516327823,5.4455498095179,150.115937345551));
#53033=CARTESIAN_POINT('Ctrl Pts',(-5.87332132991007,5.29981297364571,150.123826145741));
#53034=CARTESIAN_POINT('Ctrl Pts',(-6.00495478942234,5.15393507015595,150.131722581984));
#53035=CARTESIAN_POINT('Ctrl Pts',(-6.13107391858747,5.00323466098418,150.139619018227));
#53036=CARTESIAN_POINT('Ctrl Pts',(-6.25132724132941,4.84817787646172,150.147515454469));
#53037=CARTESIAN_POINT('Ctrl Pts',(-6.37164703148385,4.69303538766912,150.155416255296));
#53038=CARTESIAN_POINT('Ctrl Pts',(-6.48609435037436,4.53353200209237,150.163317056122));
#53039=CARTESIAN_POINT('Ctrl Pts',(-6.59436130100118,4.3701624720207,150.171217856949));
#53040=CARTESIAN_POINT('Ctrl Pts',(-6.70275981733189,4.20659441574048,150.179128258807));
#53041=CARTESIAN_POINT('Ctrl Pts',(-6.80496278437607,4.03915112393029,150.187038660665));
#53042=CARTESIAN_POINT('Ctrl Pts',(-6.90070792484196,3.86835250927618,150.194949062523));
#53043=CARTESIAN_POINT('Ctrl Pts',(-6.94226085891219,3.79422672556044,150.198382139181));
#53044=CARTESIAN_POINT('Ctrl Pts',(-6.9825980577417,3.71946922999763,150.20181521584));
#53045=CARTESIAN_POINT('Ctrl Pts',(-7.02170091700514,3.64412365763418,150.205248292498));
#53046=CARTESIAN_POINT('Ctrl Pts',(-7.11711963402917,3.4602655463916,150.213625679123));
#53047=CARTESIAN_POINT('Ctrl Pts',(-7.20539118102205,3.27250754448863,150.222003065747));
#53048=CARTESIAN_POINT('Ctrl Pts',(-7.28620562234504,3.08141665941292,150.230380452372));
#53049=CARTESIAN_POINT('Ctrl Pts',(-7.36691453401297,2.89057530591668,150.238746899582));
#53050=CARTESIAN_POINT('Ctrl Pts',(-7.440185654043,2.69641001091652,150.247113346791));
#53051=CARTESIAN_POINT('Ctrl Pts',(-7.50575542314802,2.49951125780305,150.255479794001));
#53052=CARTESIAN_POINT('Ctrl Pts',(-7.57249511513446,2.29909935587516,150.263995518814));
#53053=CARTESIAN_POINT('Ctrl Pts',(-7.63125588850341,2.09585578156161,150.272511243628));
#53054=CARTESIAN_POINT('Ctrl Pts',(-7.68181022303012,1.89042659136765,150.281026968441));
#53055=CARTESIAN_POINT('Ctrl Pts',(-7.73133129727984,1.68919608807067,150.289368643685));
#53056=CARTESIAN_POINT('Ctrl Pts',(-7.77297801270694,1.48586872873715,150.297710318929));
#53057=CARTESIAN_POINT('Ctrl Pts',(-7.80658574964955,1.28106983937982,150.306051994172));
#53058=CARTESIAN_POINT('Ctrl Pts',(-7.84124532785696,1.06986123778334,150.314654743771));
#53059=CARTESIAN_POINT('Ctrl Pts',(-7.86735446370792,0.857087777498576,
150.323257493369));
#53060=CARTESIAN_POINT('Ctrl Pts',(-7.88478865212675,0.643450783893536,
150.331860242968));
#53061=CARTESIAN_POINT('Ctrl Pts',(-7.90222284054558,0.429813790288495,
150.340462992566));
#53062=CARTESIAN_POINT('Ctrl Pts',(-7.91098199912815,0.21531358928186,150.349065742165));
#53063=CARTESIAN_POINT('Ctrl Pts',(-7.9109999722679,0.000662402618438335,
150.357668491763));
#53064=CARTESIAN_POINT('',(-7.90811390162807,-0.00405051921047928,152.357668491763));
#53065=CARTESIAN_POINT('Ctrl Pts',(-7.911,1.33226762955019E-14,150.357668491763));
#53066=CARTESIAN_POINT('Ctrl Pts',(-7.911,-2.20167589666678,150.446255927496));
#53067=CARTESIAN_POINT('Ctrl Pts',(-6.94214576672369,-4.38610418338688,
150.534843363228));
#53068=CARTESIAN_POINT('Ctrl Pts',(-3.67820201488277,-7.34180684107638,
150.712018234694));
#53069=CARTESIAN_POINT('Ctrl Pts',(-1.4086817587173,-8.0899266657134,150.800605670427));
#53070=CARTESIAN_POINT('Ctrl Pts',(2.97309270521293,-7.6545422802525,150.977780541892));
#53071=CARTESIAN_POINT('Ctrl Pts',(5.05102072675621,-6.47444880834212,151.066367977625));
#53072=CARTESIAN_POINT('Ctrl Pts',(7.66951518847883,-2.9342519536768,151.24354284909));
#53073=CARTESIAN_POINT('Ctrl Pts',(8.18956872247074,-0.60188196009885,151.332130284823));
#53074=CARTESIAN_POINT('Ctrl Pts',(7.32306689761327,3.71537198232483,151.509305156288));
#53075=CARTESIAN_POINT('Ctrl Pts',(5.94329958850174,5.66643518936541,151.597892592021));
#53076=CARTESIAN_POINT('Ctrl Pts',(2.16154501637804,7.92205913233011,151.775067463487));
#53077=CARTESIAN_POINT('Ctrl Pts',(-0.210816529300861,8.20894963713002,
151.863654899219));
#53078=CARTESIAN_POINT('Ctrl Pts',(-4.42123908576484,6.91982244717802,152.040829770685));
#53079=CARTESIAN_POINT('Ctrl Pts',(-6.22631625634226,5.35390358803477,152.129417206418));
#53080=CARTESIAN_POINT('Ctrl Pts',(-7.65317280859495,2.31334857514485,152.264559258688));
#53081=CARTESIAN_POINT('Ctrl Pts',(-7.91099999999997,1.15702837836512,152.311113875225));
#53082=CARTESIAN_POINT('Ctrl Pts',(-7.911,1.84297022087776E-13,152.357668491763));
#53083=CARTESIAN_POINT('',(5.2614341371596,-5.92453136998931,153.089));
#53084=CARTESIAN_POINT('Ctrl Pts',(-7.90647091379303,-0.00635638440671541,
152.357668491763));
#53085=CARTESIAN_POINT('Ctrl Pts',(-7.91213139978848,-0.629379302256461,
152.38273516125));
#53086=CARTESIAN_POINT('Ctrl Pts',(-7.70330066450379,-2.56750138527614,
152.460840407114));
#53087=CARTESIAN_POINT('Ctrl Pts',(-6.0944015489518,-5.52158318776385,152.591984229347));
#53088=CARTESIAN_POINT('Ctrl Pts',(-1.59537475001636,-8.5823965927603,152.804138534849));
#53089=CARTESIAN_POINT('Ctrl Pts',(3.00709256577575,-7.82448181932476,152.969810458397));
#53090=CARTESIAN_POINT('Ctrl Pts',(5.1407390732733,-6.03284475623591,153.082443805573));
#53091=CARTESIAN_POINT('Ctrl Pts',(5.2614341371596,-5.92453136998931,153.089));
#53092=CARTESIAN_POINT('',(-1.31895459586133,-7.80015452554508,153.089118084603));
#53093=CARTESIAN_POINT('Origin',(0.,0.,153.089));
#53094=CARTESIAN_POINT('',(-7.9024637590362,0.00270873549297636,152.642331508237));
#53095=CARTESIAN_POINT('Ctrl Pts',(-1.31926283107568,-7.80022221366431,
153.089));
#53096=CARTESIAN_POINT('Ctrl Pts',(-3.4855731451168,-7.43383102638713,153.00059764804));
#53097=CARTESIAN_POINT('Ctrl Pts',(-5.47418924799311,-6.11917608473493,
152.91219529608));
#53098=CARTESIAN_POINT('Ctrl Pts',(-7.47127099337646,-3.00398534954474,
152.763305798825));
#53099=CARTESIAN_POINT('Ctrl Pts',(-7.91100000000169,-1.50329545889063,
152.702818653531));
#53100=CARTESIAN_POINT('Ctrl Pts',(-7.911,8.90509888051838E-12,152.642331508237));
#53101=CARTESIAN_POINT('',(-7.92179161750093,0.00222580852156247,150.642443359737));
#53102=CARTESIAN_POINT('Ctrl Pts',(-7.89956579123653,0.00362832389775192,
152.642331508237));
#53103=CARTESIAN_POINT('Ctrl Pts',(-7.90553504434981,1.01558807491038,152.601762501006));
#53104=CARTESIAN_POINT('Ctrl Pts',(-7.25780544737249,4.66357791674521,152.455259113975));
#53105=CARTESIAN_POINT('Ctrl Pts',(-1.76836855728288,9.18370799003887,152.202821347136));
#53106=CARTESIAN_POINT('Ctrl Pts',(6.76945915019856,6.45863669117592,151.88501820773));
#53107=CARTESIAN_POINT('Ctrl Pts',(8.69546239001067,-0.742159892978413,
151.620182258224));
#53108=CARTESIAN_POINT('Ctrl Pts',(6.0989790094406,-5.51533468420419,151.408313498619));
#53109=CARTESIAN_POINT('Ctrl Pts',(1.60954184334504,-8.57675766711039,151.196444739013));
#53110=CARTESIAN_POINT('Ctrl Pts',(-5.48070072932496,-7.42723891679903,
150.941154692719));
#53111=CARTESIAN_POINT('Ctrl Pts',(-7.90535662791195,-2.38546751608027,
150.738831836327));
#53112=CARTESIAN_POINT('Ctrl Pts',(-7.92179161750093,0.00222580852156247,
150.642443359737));
#53113=CARTESIAN_POINT('',(-7.91099986105201,0.00147982984735487,146.642308865166));
#53114=CARTESIAN_POINT('Ctrl Pts',(-7.91099961209329,0.00247738972013287,
150.648656354446));
#53115=CARTESIAN_POINT('Ctrl Pts',(-7.91092915531688,0.22746562077841,150.640490528989));
#53116=CARTESIAN_POINT('Ctrl Pts',(-7.90126072315176,0.452335888079179,
150.632016437377));
#53117=CARTESIAN_POINT('Ctrl Pts',(-7.88142029371198,0.683509341423131,
150.622712655205));
#53118=CARTESIAN_POINT('Ctrl Pts',(-7.88080703590663,0.690544226057316,
150.622428961552));
#53119=CARTESIAN_POINT('Ctrl Pts',(-7.87979645475322,0.701960243835202,
150.621967655276));
#53120=CARTESIAN_POINT('Ctrl Pts',(-7.8794048931755,0.706341901386491,150.621790374355));
#53121=CARTESIAN_POINT('Ctrl Pts',(-7.87870958632744,0.714050006509404,
150.621478108927));
#53122=CARTESIAN_POINT('Ctrl Pts',(-7.87840738927717,0.7173765859027,150.62134321488));
#53123=CARTESIAN_POINT('Ctrl Pts',(-7.87781270219561,0.72387719203348,150.621079360247));
#53124=CARTESIAN_POINT('Ctrl Pts',(-7.87752040051,0.727051235824467,150.620950410523));
#53125=CARTESIAN_POINT('Ctrl Pts',(-7.87693567713893,0.733358877483924,
150.620693921517));
#53126=CARTESIAN_POINT('Ctrl Pts',(-7.87664330364484,0.736492479298589,
150.620566385013));
#53127=CARTESIAN_POINT('Ctrl Pts',(-7.87595355558775,0.743837674280561,
150.62026717187));
#53128=CARTESIAN_POINT('Ctrl Pts',(-7.87555467300646,0.74804912125201,150.62009540955));
#53129=CARTESIAN_POINT('Ctrl Pts',(-7.87416074740549,0.762641646552916,
150.619499552508));
#53130=CARTESIAN_POINT('Ctrl Pts',(-7.87314855891915,0.77302103741235,150.619074491792));
#53131=CARTESIAN_POINT('Ctrl Pts',(-7.86220563995538,0.882982879789421,
150.614558392151));
#53132=CARTESIAN_POINT('Ctrl Pts',(-7.85040703174,0.98236661591551,150.610364643893));
#53133=CARTESIAN_POINT('Ctrl Pts',(-7.83230316470806,1.11355072941246,150.604705042791));
#53134=CARTESIAN_POINT('Ctrl Pts',(-7.82768288061923,1.14557791759272,150.603313487368));
#53135=CARTESIAN_POINT('Ctrl Pts',(-7.81770376236306,1.21187116827608,150.600413997071));
#53136=CARTESIAN_POINT('Ctrl Pts',(-7.81231581911655,1.24613214977066,150.598904911465));
#53137=CARTESIAN_POINT('Ctrl Pts',(-7.79915336916526,1.32638742096287,150.595346780335));
#53138=CARTESIAN_POINT('Ctrl Pts',(-7.79119703413402,1.37235036631787,150.593291132861));
#53139=CARTESIAN_POINT('Ctrl Pts',(-7.77883640223423,1.44018146708135,150.590233600891));
#53140=CARTESIAN_POINT('Ctrl Pts',(-7.77474526793858,1.46210616521036,150.58924163456));
#53141=CARTESIAN_POINT('Ctrl Pts',(-7.63817637445548,2.17720561654808,150.556772906631));
#53142=CARTESIAN_POINT('Ctrl Pts',(-7.41363400925527,2.84959123214577,150.523084960769));
#53143=CARTESIAN_POINT('Ctrl Pts',(-6.96836842988337,3.75752981011897,150.478479563164));
#53144=CARTESIAN_POINT('Ctrl Pts',(-6.81812488277147,4.02372822725777,150.465467174321));
#53145=CARTESIAN_POINT('Ctrl Pts',(-6.62877818709735,4.31800882587217,150.451191974965));
#53146=CARTESIAN_POINT('Ctrl Pts',(-6.60438877748413,4.35522093971914,150.449388648229));
#53147=CARTESIAN_POINT('Ctrl Pts',(-6.57321429408625,4.40192125513837,150.447127481806));
#53148=CARTESIAN_POINT('Ctrl Pts',(-6.56672066965125,4.41160249123715,150.446658836459));
#53149=CARTESIAN_POINT('Ctrl Pts',(-6.55634520189289,4.42699743703263,150.445913766547));
#53150=CARTESIAN_POINT('Ctrl Pts',(-6.55247724495641,4.43272045909914,150.445636825025));
#53151=CARTESIAN_POINT('Ctrl Pts',(-6.54517393652263,4.44349597386237,150.445115454841));
#53152=CARTESIAN_POINT('Ctrl Pts',(-6.54174021929269,4.44854956503452,150.444870965467));
#53153=CARTESIAN_POINT('Ctrl Pts',(-6.53400412025852,4.45990688284943,150.444321565301));
#53154=CARTESIAN_POINT('Ctrl Pts',(-6.52969846117015,4.46620837555204,150.444016777363));
#53155=CARTESIAN_POINT('Ctrl Pts',(-6.51871961956967,4.48222650759002,150.443242119683));
#53156=CARTESIAN_POINT('Ctrl Pts',(-6.51203381647745,4.49193449623709,150.442772723128));
#53157=CARTESIAN_POINT('Ctrl Pts',(-6.47485440910975,4.54566265914021,150.440175369299));
#53158=CARTESIAN_POINT('Ctrl Pts',(-6.44393581119019,4.58938776216048,150.438063420303));
#53159=CARTESIAN_POINT('Ctrl Pts',(-5.86439432450722,5.39157143238999,150.399338193375));
#53160=CARTESIAN_POINT('Ctrl Pts',(-5.18602585089256,6.0468999811995,150.369205450616));
#53161=CARTESIAN_POINT('Ctrl Pts',(-4.29766747739003,6.64318696381936,150.330642404276));
#53162=CARTESIAN_POINT('Ctrl Pts',(-4.18452541402164,6.7150296796407,150.325723539682));
#53163=CARTESIAN_POINT('Ctrl Pts',(-3.99123665528837,6.83098128384793,150.317219859528));
#53164=CARTESIAN_POINT('Ctrl Pts',(-3.91204945372838,6.87663750790894,150.313708624991));
#53165=CARTESIAN_POINT('Ctrl Pts',(-3.80531660668065,6.935735231399,150.30891689159));
#53166=CARTESIAN_POINT('Ctrl Pts',(-3.77845627990965,6.95040472016694,150.307706087798));
#53167=CARTESIAN_POINT('Ctrl Pts',(-3.74017508790437,6.9710241084333,150.305972568751));
#53168=CARTESIAN_POINT('Ctrl Pts',(-3.72882351830667,6.97710269197855,150.305457546377));
#53169=CARTESIAN_POINT('Ctrl Pts',(-3.70886608630795,6.98772696074326,150.304550271655));
#53170=CARTESIAN_POINT('Ctrl Pts',(-3.70026655700388,6.99228454295532,150.304158746885));
#53171=CARTESIAN_POINT('Ctrl Pts',(-3.68764993785024,6.99894131132883,150.303583440944));
#53172=CARTESIAN_POINT('Ctrl Pts',(-3.68363939239396,7.00105294725003,150.303400432494));
#53173=CARTESIAN_POINT('Ctrl Pts',(-3.67671920949135,7.00468897556172,150.303084421928));
#53174=CARTESIAN_POINT('Ctrl Pts',(-3.67381042798319,7.00621500733765,150.302951522165));
#53175=CARTESIAN_POINT('Ctrl Pts',(-3.66801538494513,7.0092506550434,150.302686610709));
#53176=CARTESIAN_POINT('Ctrl Pts',(-3.66512914652523,7.01076029747543,150.302554601436));
#53177=CARTESIAN_POINT('Ctrl Pts',(-3.6582729623709,7.01434102269576,150.302240853811));
#53178=CARTESIAN_POINT('Ctrl Pts',(-3.65430219280813,7.01641051631357,150.302059016685));
#53179=CARTESIAN_POINT('Ctrl Pts',(-3.64240530506515,7.02259812148763,150.301513828318));
#53180=CARTESIAN_POINT('Ctrl Pts',(-3.63447399238149,7.02670616859194,150.301149858019));
#53181=CARTESIAN_POINT('Ctrl Pts',(-3.55935828942507,7.06545136890281,150.297698092285));
#53182=CARTESIAN_POINT('Ctrl Pts',(-3.49168957346997,7.0991364073923,150.294553136003));
#53183=CARTESIAN_POINT('Ctrl Pts',(-3.16059923639091,7.25807205917222,150.279033846659));
#53184=CARTESIAN_POINT('Ctrl Pts',(-2.89088412413446,7.36965155334711,150.265997445874));
#53185=CARTESIAN_POINT('Ctrl Pts',(-2.47660163127544,7.51479018988298,150.246023640053));
#53186=CARTESIAN_POINT('Ctrl Pts',(-2.33622482441889,7.55960845750603,150.239262669616));
#53187=CARTESIAN_POINT('Ctrl Pts',(-2.15189696983936,7.61283412606556,150.230450982739));
#53188=CARTESIAN_POINT('Ctrl Pts',(-2.10901043563407,7.6248264887977,150.228405361108));
#53189=CARTESIAN_POINT('Ctrl Pts',(-2.01687265776054,7.64975414414357,150.22402252869));
#53190=CARTESIAN_POINT('Ctrl Pts',(-1.96759304643228,7.66257733451901,150.221685688397));
#53191=CARTESIAN_POINT('Ctrl Pts',(-1.86076081896549,7.6892779027404,150.216638647553));
#53192=CARTESIAN_POINT('Ctrl Pts',(-1.80316910481317,7.7029868707906,150.213929678311));
#53193=CARTESIAN_POINT('Ctrl Pts',(-1.67665362859226,7.73160563237193,150.20800913758));
#53194=CARTESIAN_POINT('Ctrl Pts',(-1.6076731120852,7.74624298387695,150.204800723056));
#53195=CARTESIAN_POINT('Ctrl Pts',(-1.30429137802051,7.80639209773261,150.190789500558));
#53196=CARTESIAN_POINT('Ctrl Pts',(-1.06808583121151,7.84220226626713,150.180145587103));
#53197=CARTESIAN_POINT('Ctrl Pts',(-0.644322659858789,7.88694234952294,
150.161657657725));
#53198=CARTESIAN_POINT('Ctrl Pts',(-0.457387220624849,7.89998825052059,
150.153709218142));
#53199=CARTESIAN_POINT('Ctrl Pts',(-0.1826563605207,7.90937562606933,150.142342655629));
#53200=CARTESIAN_POINT('Ctrl Pts',(-0.0951113524039408,7.91091275458935,
150.138767041912));
#53201=CARTESIAN_POINT('Ctrl Pts',(0.00677694519215901,7.91101008302992,
150.134658277288));
#53202=CARTESIAN_POINT('Ctrl Pts',(0.0211109007411958,7.91098481817794,
150.134081454107));
#53203=CARTESIAN_POINT('Ctrl Pts',(0.0429375071318609,7.91088702440545,
150.133204944196));
#53204=CARTESIAN_POINT('Ctrl Pts',(0.0504302184334194,7.91084280818981,
150.132904381373));
#53205=CARTESIAN_POINT('Ctrl Pts',(0.0634380765365338,7.91074756452198,
150.132383151844));
#53206=CARTESIAN_POINT('Ctrl Pts',(0.0689532474881799,7.91070141447408,
150.132162334252));
#53207=CARTESIAN_POINT('Ctrl Pts',(0.0804269928389719,7.91059340423459,
150.131703313708));
#53208=CARTESIAN_POINT('Ctrl Pts',(0.0863855553656897,7.91053057919053,
150.131465140801));
#53209=CARTESIAN_POINT('Ctrl Pts',(0.100924328230168,7.91036085846773,150.130884505442));
#53210=CARTESIAN_POINT('Ctrl Pts',(0.109504455761332,7.91024673483588,150.13054226708));
#53211=CARTESIAN_POINT('Ctrl Pts',(0.142072888911172,7.9097605444271,150.129244809737));
#53212=CARTESIAN_POINT('Ctrl Pts',(0.166059757534419,7.90929331518965,150.128292540732));
#53213=CARTESIAN_POINT('Ctrl Pts',(0.229241307182391,7.9077750801567,150.125792859797));
#53214=CARTESIAN_POINT('Ctrl Pts',(0.26843114365175,7.90654178965083,150.124251098044));
#53215=CARTESIAN_POINT('Ctrl Pts',(1.17057048911248,7.87143654261414,150.088954905694));
#53216=CARTESIAN_POINT('Ctrl Pts',(2.02208939794266,7.69680456498812,150.060606833125));
#53217=CARTESIAN_POINT('Ctrl Pts',(3.05347760895975,7.30193122630002,150.021909974678));
#53218=CARTESIAN_POINT('Ctrl Pts',(3.27433704111667,7.20559715699836,150.01328328766));
#53219=CARTESIAN_POINT('Ctrl Pts',(3.57069949098794,7.05988835973848,150.000823008299));
#53220=CARTESIAN_POINT('Ctrl Pts',(3.65027582538324,7.01907429375369,149.997386108494));
#53221=CARTESIAN_POINT('Ctrl Pts',(3.75486174685292,6.96317347458829,149.992725813978));
#53222=CARTESIAN_POINT('Ctrl Pts',(3.78050628824733,6.94928368544182,149.991571512775));
#53223=CARTESIAN_POINT('Ctrl Pts',(3.81690770495389,6.92930655366915,149.989915674117));
#53224=CARTESIAN_POINT('Ctrl Pts',(3.82772826294864,6.92333518506525,149.98942126979));
#53225=CARTESIAN_POINT('Ctrl Pts',(3.84673886240101,6.91278591874854,149.988548710246));
#53226=CARTESIAN_POINT('Ctrl Pts',(3.85493485810317,6.90821874815308,149.988171232345));
#53227=CARTESIAN_POINT('Ctrl Pts',(3.86696640198103,6.90148616215294,149.987615173184));
#53228=CARTESIAN_POINT('Ctrl Pts',(3.87080832298895,6.89933209281672,149.987437322277));
#53229=CARTESIAN_POINT('Ctrl Pts',(3.87744847555632,6.89560183261177,149.987129430601));
#53230=CARTESIAN_POINT('Ctrl Pts',(3.88024755340246,6.89402714230009,149.986999487304));
#53231=CARTESIAN_POINT('Ctrl Pts',(3.88580670322695,6.89089524721308,149.986741101565));
#53232=CARTESIAN_POINT('Ctrl Pts',(3.88856679997324,6.88933808758115,149.986612662081));
#53233=CARTESIAN_POINT('Ctrl Pts',(3.89508532224324,6.88565537739181,149.986308965672));
#53234=CARTESIAN_POINT('Ctrl Pts',(3.89884294200569,6.88352840898737,149.986133615303));
#53235=CARTESIAN_POINT('Ctrl Pts',(3.91208808982789,6.87601678189935,149.985514520991));
#53236=CARTESIAN_POINT('Ctrl Pts',(3.92156616709638,6.8706156057767,149.985069685711));
#53237=CARTESIAN_POINT('Ctrl Pts',(4.04493159692747,6.79997615786413,149.979256375689));
#53238=CARTESIAN_POINT('Ctrl Pts',(4.15718397927057,6.73193621906005,149.973706780942));
#53239=CARTESIAN_POINT('Ctrl Pts',(4.57667742043928,6.46317344511306,149.952131008886));
#53240=CARTESIAN_POINT('Ctrl Pts',(4.87150381807986,6.24395776364467,149.935236049072));
#53241=CARTESIAN_POINT('Ctrl Pts',(5.6057130212541,5.6142915080586,149.890493496174));
#53242=CARTESIAN_POINT('Ctrl Pts',(6.01549453998622,5.17284191857809,149.862812196008));
#53243=CARTESIAN_POINT('Ctrl Pts',(6.46386527732439,4.56362718872494,149.830728989147));
#53244=CARTESIAN_POINT('Ctrl Pts',(6.55258410245583,4.43530075497591,149.824255795098));
#53245=CARTESIAN_POINT('Ctrl Pts',(6.6533305152101,4.27994922851812,149.816747317899));
#53246=CARTESIAN_POINT('Ctrl Pts',(6.66907090493354,4.25538078586971,149.815569314261));
#53247=CARTESIAN_POINT('Ctrl Pts',(6.68988708159433,4.22249059395434,149.81400476241));
#53248=CARTESIAN_POINT('Ctrl Pts',(6.69508382794791,4.21424590148369,149.81361360942));
#53249=CARTESIAN_POINT('Ctrl Pts',(6.70362328881433,4.20064229524931,149.812969917956));
#53250=CARTESIAN_POINT('Ctrl Pts',(6.70697483738707,4.19528895570661,149.81271704406));
#53251=CARTESIAN_POINT('Ctrl Pts',(6.71347920027869,4.18487199418691,149.812225822908));
#53252=CARTESIAN_POINT('Ctrl Pts',(6.71663270509428,4.17980880966691,149.811987449555));
#53253=CARTESIAN_POINT('Ctrl Pts',(6.72393195790878,4.1680597300926,149.811435198014));
#53254=CARTESIAN_POINT('Ctrl Pts',(6.72807346878722,4.1613712027745,149.811121480302));
#53255=CARTESIAN_POINT('Ctrl Pts',(6.74142747226627,4.13973248093241,149.810108694158));
#53256=CARTESIAN_POINT('Ctrl Pts',(6.75060019497805,4.1247577371651,149.809411127749));
#53257=CARTESIAN_POINT('Ctrl Pts',(6.8355855099744,3.98497384785066,149.802930231968));
#53258=CARTESIAN_POINT('Ctrl Pts',(6.90798067081007,3.85811504668108,149.797276358375));
#53259=CARTESIAN_POINT('Ctrl Pts',(6.98057463752772,3.7223060041083,149.791441284305));
#53260=CARTESIAN_POINT('Ctrl Pts',(6.98431342346669,3.71528602687971,149.791140269718));
#53261=CARTESIAN_POINT('Ctrl Pts',(6.9986925448824,3.68818925162454,149.78998066874));
#53262=CARTESIAN_POINT('Ctrl Pts',(7.00925699401844,3.6680722041987,149.789124629275));
#53263=CARTESIAN_POINT('Ctrl Pts',(7.03127382170546,3.62570484967388,149.787331786412));
#53264=CARTESIAN_POINT('Ctrl Pts',(7.04270760100052,3.60344513934872,149.78639559728));
#53265=CARTESIAN_POINT('Ctrl Pts',(7.40076418251151,2.89815299162774,149.756910516542));
#53266=CARTESIAN_POINT('Ctrl Pts',(7.64643153588114,2.16853727568436,149.732186654909));
#53267=CARTESIAN_POINT('Ctrl Pts',(7.81762026450783,1.22690391307422,149.698291697599));
#53268=CARTESIAN_POINT('Ctrl Pts',(7.84498757865914,1.03761404069944,149.691353038888));
#53269=CARTESIAN_POINT('Ctrl Pts',(7.87666113311587,0.743668332854099,149.680142740212));
#53270=CARTESIAN_POINT('Ctrl Pts',(7.88579372141803,0.639600569253509,149.676089960124));
#53271=CARTESIAN_POINT('Ctrl Pts',(7.8936674117543,0.523523799019757,149.671446505456));
#53272=CARTESIAN_POINT('Ctrl Pts',(7.89444534213445,0.511659176303168,149.670970452013));
#53273=CARTESIAN_POINT('Ctrl Pts',(7.89576727185624,0.490776737161409,149.670129985119));
#53274=CARTESIAN_POINT('Ctrl Pts',(7.89632257898012,0.481759633472731,149.669766221055));
#53275=CARTESIAN_POINT('Ctrl Pts',(7.89711690924771,0.468490827856677,149.669229663842));
#53276=CARTESIAN_POINT('Ctrl Pts',(7.89736794882502,0.464239824707906,149.669057571748));
#53277=CARTESIAN_POINT('Ctrl Pts',(7.897796524426,0.456881544265296,149.668759352879));
#53278=CARTESIAN_POINT('Ctrl Pts',(7.89797565957893,0.453774357329536,149.668633320134));
#53279=CARTESIAN_POINT('Ctrl Pts',(7.89832832302281,0.447593764138455,149.668382417317));
#53280=CARTESIAN_POINT('Ctrl Pts',(7.89850189054344,0.444520371820042,149.668257549902));
#53281=CARTESIAN_POINT('Ctrl Pts',(7.89891079728028,0.437203928901474,149.667960050495));
#53282=CARTESIAN_POINT('Ctrl Pts',(7.89914451096828,0.432960799074963,149.667787323018));
#53283=CARTESIAN_POINT('Ctrl Pts',(7.89996148959228,0.417907481939246,149.6671738548));
#53284=CARTESIAN_POINT('Ctrl Pts',(7.90052598089328,0.407096331918799,149.666732015811));
#53285=CARTESIAN_POINT('Ctrl Pts',(7.90761760016446,0.265704419743534,149.660937439552));
#53286=CARTESIAN_POINT('Ctrl Pts',(7.91092847763104,0.134988999559838,149.655401499155));
#53287=CARTESIAN_POINT('Ctrl Pts',(7.91100386771795,-0.00505529020108679,
149.649323498358));
#53288=CARTESIAN_POINT('Ctrl Pts',(7.91099243291304,-0.0143692827151416,
149.648918568706));
#53289=CARTESIAN_POINT('Ctrl Pts',(7.9089385233884,-0.70044224624324,149.619040988456));
#53290=CARTESIAN_POINT('Ctrl Pts',(7.82008407366501,-1.37413713735386,149.586362036858));
#53291=CARTESIAN_POINT('Ctrl Pts',(7.63563525924089,-2.06949538491413,149.553463641788));
#53292=CARTESIAN_POINT('Ctrl Pts',(7.62437669984048,-2.1105963495069,149.551521125052));
#53293=CARTESIAN_POINT('Ctrl Pts',(7.59963202440341,-2.19814771870425,149.547388760209));
#53294=CARTESIAN_POINT('Ctrl Pts',(7.58605086525964,-2.24456959187779,149.545201004147));
#53295=CARTESIAN_POINT('Ctrl Pts',(7.55573789075456,-2.34476373549494,149.540487782271));
#53296=CARTESIAN_POINT('Ctrl Pts',(7.53885585049072,-2.39848799449484,149.537966012219));
#53297=CARTESIAN_POINT('Ctrl Pts',(7.5001815210725,-2.51711843053026,149.532411726644));
#53298=CARTESIAN_POINT('Ctrl Pts',(7.47811726366694,-2.58193154771427,149.529386638262));
#53299=CARTESIAN_POINT('Ctrl Pts',(7.36654419751321,-2.89623967871215,149.514768690928));
#53300=CARTESIAN_POINT('Ctrl Pts',(7.26537203284612,-3.14142728292245,149.5035344786));
#53301=CARTESIAN_POINT('Ctrl Pts',(7.13462767580495,-3.41799283883676,149.491065139604));
#53302=CARTESIAN_POINT('Ctrl Pts',(7.11689686531971,-3.45475993291284,149.489411501405));
#53303=CARTESIAN_POINT('Ctrl Pts',(7.0939890648529,-3.50133732567146,149.487321549054));
#53304=CARTESIAN_POINT('Ctrl Pts',(7.08907510291591,-3.51127585172964,149.486875887958));
#53305=CARTESIAN_POINT('Ctrl Pts',(7.08118086248714,-3.52715789256235,149.486164159051));
#53306=CARTESIAN_POINT('Ctrl Pts',(7.0782139645453,-3.53310801967908,149.485897614621));
#53307=CARTESIAN_POINT('Ctrl Pts',(7.07258642472409,-3.5443585368482,149.485393821232));
#53308=CARTESIAN_POINT('Ctrl Pts',(7.06992731782188,-3.54965968704581,149.485156517745));
#53309=CARTESIAN_POINT('Ctrl Pts',(7.06390335035979,-3.56163534460087,149.484620611652));
#53310=CARTESIAN_POINT('Ctrl Pts',(7.06053498418739,-3.56830808768019,149.484322134515));
#53311=CARTESIAN_POINT('Ctrl Pts',(7.05188302436484,-3.58538743008752,149.483558479371));
#53312=CARTESIAN_POINT('Ctrl Pts',(7.04658584102068,-3.5957871460654,149.483093787532));
#53313=CARTESIAN_POINT('Ctrl Pts',(7.01618411311258,-3.65514827928551,149.480443038039));
#53314=CARTESIAN_POINT('Ctrl Pts',(6.99059202867877,-3.70385902782594,149.478274479522));
#53315=CARTESIAN_POINT('Ctrl Pts',(6.54989969593821,-4.52181050347926,149.441958188016));
#53316=CARTESIAN_POINT('Ctrl Pts',(6.01072134227546,-5.21718858489354,149.413430129067));
#53317=CARTESIAN_POINT('Ctrl Pts',(5.12109578670382,-6.03920780721774,149.370729971823));
#53318=CARTESIAN_POINT('Ctrl Pts',(4.8590239118827,-6.25200273239228,149.35842271667));
#53319=CARTESIAN_POINT('Ctrl Pts',(4.56763310984833,-6.45918421800138,149.344166651783));
#53320=CARTESIAN_POINT('Ctrl Pts',(4.55104567371395,-6.47088218500881,149.343353632332));
#53321=CARTESIAN_POINT('Ctrl Pts',(4.52866614015609,-6.48653630109342,149.342254904525));
#53322=CARTESIAN_POINT('Ctrl Pts',(4.52291342823913,-6.49054884540434,149.341972313433));
#53323=CARTESIAN_POINT('Ctrl Pts',(4.51343185646688,-6.49714356075586,149.341506294557));
#53324=CARTESIAN_POINT('Ctrl Pts',(4.50970609046465,-6.49973019051875,149.341323108709));
#53325=CARTESIAN_POINT('Ctrl Pts',(4.5024482631929,-6.50475972504361,149.340966138286));
#53326=CARTESIAN_POINT('Ctrl Pts',(4.49891643243196,-6.50720296111665,149.340792371565));
#53327=CARTESIAN_POINT('Ctrl Pts',(4.49070664082053,-6.51287241990594,149.340388320285));
#53328=CARTESIAN_POINT('Ctrl Pts',(4.48602719351208,-6.51609647800787,149.340157921213));
#53329=CARTESIAN_POINT('Ctrl Pts',(4.47150811876265,-6.52607681609769,149.339442765104));
#53330=CARTESIAN_POINT('Ctrl Pts',(4.46165670107198,-6.53281585117169,149.338957109161));
#53331=CARTESIAN_POINT('Ctrl Pts',(4.37845518211635,-6.58945532760305,149.334852206526));
#53332=CARTESIAN_POINT('Ctrl Pts',(4.3042875199556,-6.63813975639834,149.33117194482));
#53333=CARTESIAN_POINT('Ctrl Pts',(3.55990156228777,-7.10904168312127,149.294138814529));
#53334=CARTESIAN_POINT('Ctrl Pts',(2.83065900917638,-7.42959847810138,149.25764977628));
#53335=CARTESIAN_POINT('Ctrl Pts',(1.79917464852797,-7.70864753382524,149.21190284172));
#53336=CARTESIAN_POINT('Ctrl Pts',(1.52883155996935,-7.76678594866081,149.200354022928));
#53337=CARTESIAN_POINT('Ctrl Pts',(1.20689325086633,-7.81855499691087,149.187087081397));
#53338=CARTESIAN_POINT('Ctrl Pts',(1.15772539519168,-7.82598655418925,149.185073798849));
#53339=CARTESIAN_POINT('Ctrl Pts',(1.0927245790804,-7.8351852263697,149.182428498573));
#53340=CARTESIAN_POINT('Ctrl Pts',(1.07695207409938,-7.83736874019975,149.181787877185));
#53341=CARTESIAN_POINT('Ctrl Pts',(1.05110633813079,-7.84086727737101,149.180740152587));
#53342=CARTESIAN_POINT('Ctrl Pts',(1.04103700037219,-7.84221054039673,149.180332470934));
#53343=CARTESIAN_POINT('Ctrl Pts',(1.02159242672985,-7.84476636223987,149.179546174594));
#53344=CARTESIAN_POINT('Ctrl Pts',(1.01221754634572,-7.84598151947403,149.179167506845));
#53345=CARTESIAN_POINT('Ctrl Pts',(0.990768093654178,-7.84872268001833,
149.178302111037));
#53346=CARTESIAN_POINT('Ctrl Pts',(0.978692121403351,-7.85023763053391,
149.177815609775));
#53347=CARTESIAN_POINT('Ctrl Pts',(0.946739072639208,-7.85417131685011,
149.176530207551));
#53348=CARTESIAN_POINT('Ctrl Pts',(0.926856189083176,-7.856542468275,149.175732286614));
#53349=CARTESIAN_POINT('Ctrl Pts',(0.796108832971649,-7.87163162050543,
149.170497814899));
#53350=CARTESIAN_POINT('Ctrl Pts',(0.684993217024253,-7.88207832916265,
149.166108857532));
#53351=CARTESIAN_POINT('Ctrl Pts',(-0.110773817093137,-7.93993829575988,
149.135071931437));
#53352=CARTESIAN_POINT('Ctrl Pts',(-0.798778168017218,-7.90043385837942,
149.110659956625));
#53353=CARTESIAN_POINT('Ctrl Pts',(-1.67121591648593,-7.73509120590145,
149.078380193435));
#53354=CARTESIAN_POINT('Ctrl Pts',(-1.8678623735826,-7.68997300234885,149.070987374967));
#53355=CARTESIAN_POINT('Ctrl Pts',(-2.19260125175708,-7.60227358415099,
149.058337034674));
#53356=CARTESIAN_POINT('Ctrl Pts',(-2.32171639331088,-7.56384126512282,
149.053187411601));
#53357=CARTESIAN_POINT('Ctrl Pts',(-2.51035481665794,-7.50240613140274,
149.045414714383));
#53358=CARTESIAN_POINT('Ctrl Pts',(-2.57068481570564,-7.48194883268298,
149.042890687503));
#53359=CARTESIAN_POINT('Ctrl Pts',(-2.64038896335427,-7.45737027158181,
149.039923838663));
#53360=CARTESIAN_POINT('Ctrl Pts',(-2.65001132706484,-7.45395634614931,
149.039513151579));
#53361=CARTESIAN_POINT('Ctrl Pts',(-2.66463067652972,-7.44873765040983,
149.038887443896));
#53362=CARTESIAN_POINT('Ctrl Pts',(-2.66963252130659,-7.4469464499161,149.038673053767));
#53363=CARTESIAN_POINT('Ctrl Pts',(-2.67830287152923,-7.44383167046296,
149.038300877909));
#53364=CARTESIAN_POINT('Ctrl Pts',(-2.68197221377194,-7.4425104134495,149.038143201375));
#53365=CARTESIAN_POINT('Ctrl Pts',(-2.68959428536389,-7.43975948859834,
149.037815315808));
#53366=CARTESIAN_POINT('Ctrl Pts',(-2.69354685440106,-7.43832938307341,
149.037645086052));
#53367=CARTESIAN_POINT('Ctrl Pts',(-2.70435080962519,-7.4344105908674,149.037179232755));
#53368=CARTESIAN_POINT('Ctrl Pts',(-2.71119988716017,-7.43191558795201,
149.036883306929));
#53369=CARTESIAN_POINT('Ctrl Pts',(-2.73724493449828,-7.42238702341264,
149.035755664892));
#53370=CARTESIAN_POINT('Ctrl Pts',(-2.75641693850311,-7.41528857196749,
149.034920793306));
#53371=CARTESIAN_POINT('Ctrl Pts',(-3.04508196158709,-7.30713591792976,
149.022275242403));
#53372=CARTESIAN_POINT('Ctrl Pts',(-3.30884578878543,-7.19153976667503,
149.009660128665));
#53373=CARTESIAN_POINT('Ctrl Pts',(-3.86645566951851,-6.9099904760934,148.981486276701));
#53374=CARTESIAN_POINT('Ctrl Pts',(-4.15721345301412,-6.73906663907074,
148.965839381709));
#53375=CARTESIAN_POINT('Ctrl Pts',(-4.73443380443059,-6.34813456049918,
148.933790807392));
#53376=CARTESIAN_POINT('Ctrl Pts',(-5.01855674891759,-6.12599355001103,
148.917455432688));
#53377=CARTESIAN_POINT('Ctrl Pts',(-5.48732525513993,-5.70491086492572,
148.890052053284));
#53378=CARTESIAN_POINT('Ctrl Pts',(-5.67873585817106,-5.51441062791798,
148.87870231674));
#53379=CARTESIAN_POINT('Ctrl Pts',(-5.87258067753897,-5.30066648576751,
148.867040919445));
#53380=CARTESIAN_POINT('Ctrl Pts',(-5.88506392404763,-5.28680353557291,
148.866289113506));
#53381=CARTESIAN_POINT('Ctrl Pts',(-5.9029580740366,-5.26678973192563,148.865210207601));
#53382=CARTESIAN_POINT('Ctrl Pts',(-5.90840859524454,-5.26067447922086,
148.864881409969));
#53383=CARTESIAN_POINT('Ctrl Pts',(-5.9178574563556,-5.25004005084794,148.864311126344));
#53384=CARTESIAN_POINT('Ctrl Pts',(-5.9218601373108,-5.24552475197567,148.864069454827));
#53385=CARTESIAN_POINT('Ctrl Pts',(-5.92955015569906,-5.2368298632195,148.863604975457));
#53386=CARTESIAN_POINT('Ctrl Pts',(-5.93323824865338,-5.23265094862386,
148.863382135414));
#53387=CARTESIAN_POINT('Ctrl Pts',(-5.94192081028687,-5.22279190593248,
148.862857336532));
#53388=CARTESIAN_POINT('Ctrl Pts',(-5.94691155969522,-5.21710850088318,
148.86255553614));
#53389=CARTESIAN_POINT('Ctrl Pts',(-5.96415669192368,-5.19741305464539,
148.861512181106));
#53390=CARTESIAN_POINT('Ctrl Pts',(-5.97636980931023,-5.18336487380359,
148.860772379657));
#53391=CARTESIAN_POINT('Ctrl Pts',(-6.11258035280688,-5.02556681007315,
148.852511257575));
#53392=CARTESIAN_POINT('Ctrl Pts',(-6.23141876092967,-4.87743648363437,
148.845210307832));
#53393=CARTESIAN_POINT('Ctrl Pts',(-6.82841010841845,-4.07581369218198,
148.80781868917));
#53394=CARTESIAN_POINT('Ctrl Pts',(-7.20939802013467,-3.35617009044395,
148.781955481912));
#53395=CARTESIAN_POINT('Ctrl Pts',(-7.52538137031228,-2.44471253632168,
148.748089365807));
#53396=CARTESIAN_POINT('Ctrl Pts',(-7.57186897398844,-2.29668917125152,
148.742536570122));
#53397=CARTESIAN_POINT('Ctrl Pts',(-7.65651502922844,-1.99656218909036,
148.731010833574));
#53398=CARTESIAN_POINT('Ctrl Pts',(-7.6945625978662,-1.84450104108649,148.725036573261));
#53399=CARTESIAN_POINT('Ctrl Pts',(-7.73296796118194,-1.66902753348587,
148.717890519831));
#53400=CARTESIAN_POINT('Ctrl Pts',(-7.73777133156448,-1.6466150721659,148.71697311198));
#53401=CARTESIAN_POINT('Ctrl Pts',(-7.74373287222399,-1.61819640680624,
148.715803593481));
#53402=CARTESIAN_POINT('Ctrl Pts',(-7.74498161522343,-1.61220910145263,
148.715556845351));
#53403=CARTESIAN_POINT('Ctrl Pts',(-7.74696355560872,-1.60265091548136,
148.715162365469));
#53404=CARTESIAN_POINT('Ctrl Pts',(-7.74770123292901,-1.59908095295293,
148.715014901369));
#53405=CARTESIAN_POINT('Ctrl Pts',(-7.74909482285481,-1.59231312339752,
148.714735101477));
#53406=CARTESIAN_POINT('Ctrl Pts',(-7.74975122237288,-1.58911536642455,
148.714602795706));
#53407=CARTESIAN_POINT('Ctrl Pts',(-7.75123785439433,-1.58185016926167,
148.714301971123));
#53408=CARTESIAN_POINT('Ctrl Pts',(-7.75206686439499,-1.57778248286342,
148.714133379559));
#53409=CARTESIAN_POINT('Ctrl Pts',(-7.75419679564904,-1.56728939020988,
148.713698058049));
#53410=CARTESIAN_POINT('Ctrl Pts',(-7.75549292983254,-1.56086302830029,
148.713431045785));
#53411=CARTESIAN_POINT('Ctrl Pts',(-7.76309063535863,-1.52294974451091,
148.711853411207));
#53412=CARTESIAN_POINT('Ctrl Pts',(-7.76920835339804,-1.49142671345929,
148.710532105867));
#53413=CARTESIAN_POINT('Ctrl Pts',(-7.86559670462253,-0.978070393359079,
148.68886949681));
#53414=CARTESIAN_POINT('Ctrl Pts',(-7.91107393500614,-0.488943892504856,
148.666215133163));
#53415=CARTESIAN_POINT('Ctrl Pts',(-7.91093589495348,0.425052308809872,
148.623880575233));
#53416=CARTESIAN_POINT('Ctrl Pts',(-7.87680757959934,0.848248594413475,
148.604279788228));
#53417=CARTESIAN_POINT('Ctrl Pts',(-7.7569377716937,1.58722450434003,148.571244463978));
#53418=CARTESIAN_POINT('Ctrl Pts',(-7.68525539490773,1.90427112437255,148.557459048505));
#53419=CARTESIAN_POINT('Ctrl Pts',(-7.58820368100426,2.23686305051484,148.543448480544));
#53420=CARTESIAN_POINT('Ctrl Pts',(-7.58204250288556,2.25765872214134,148.542574280886));
#53421=CARTESIAN_POINT('Ctrl Pts',(-7.57348107557444,2.28612554211239,148.541380070242));
#53422=CARTESIAN_POINT('Ctrl Pts',(-7.57115457153753,2.29381866126426,148.541057583723));
#53423=CARTESIAN_POINT('Ctrl Pts',(-7.56716680123419,2.30693297498313,148.540508266147));
#53424=CARTESIAN_POINT('Ctrl Pts',(-7.56551142538087,2.31235594608302,148.540281237192));
#53425=CARTESIAN_POINT('Ctrl Pts',(-7.56229197485612,2.32286232356471,148.53984163091));
#53426=CARTESIAN_POINT('Ctrl Pts',(-7.5607286013615,2.32794594093536,148.539629030122));
#53427=CARTESIAN_POINT('Ctrl Pts',(-7.55699694123851,2.34003675874718,148.53912363663));
#53428=CARTESIAN_POINT('Ctrl Pts',(-7.55482403161433,2.34704253346622,148.538830999776));
#53429=CARTESIAN_POINT('Ctrl Pts',(-7.5483529058202,2.36780428034962,148.537964362653));
#53430=CARTESIAN_POINT('Ctrl Pts',(-7.54402682916036,2.38155157505634,148.537391301631));
#53431=CARTESIAN_POINT('Ctrl Pts',(-7.50920547116318,2.49115902882886,148.532828401821));
#53432=CARTESIAN_POINT('Ctrl Pts',(-7.47692126107482,2.58644341140148,148.528899384002));
#53433=CARTESIAN_POINT('Ctrl Pts',(-7.33268651360203,2.98684584932947,148.512527032226));
#53434=CARTESIAN_POINT('Ctrl Pts',(-7.20380449674291,3.28553850822161,148.500673940781));
#53435=CARTESIAN_POINT('Ctrl Pts',(-6.70204633541516,4.27585771948024,148.461510065733));
#53436=CARTESIAN_POINT('Ctrl Pts',(-6.24497034089314,4.91938564427989,148.436653689384));
#53437=CARTESIAN_POINT('Ctrl Pts',(-5.65356205128053,5.53405737612092,148.403595439074));
#53438=CARTESIAN_POINT('Ctrl Pts',(-5.60573459863632,5.5824989044821,148.400913884116));
#53439=CARTESIAN_POINT('Ctrl Pts',(-5.55067177066127,5.63684755417532,148.397809194485));
#53440=CARTESIAN_POINT('Ctrl Pts',(-5.54404276132924,5.64336755084235,148.397435138008));
#53441=CARTESIAN_POINT('Ctrl Pts',(-5.53431024558022,5.65290631890934,148.396885517534));
#53442=CARTESIAN_POINT('Ctrl Pts',(-5.53121571243371,5.65593427181423,148.396710696015));
#53443=CARTESIAN_POINT('Ctrl Pts',(-5.52569713149072,5.66132525748214,148.396398817837));
#53444=CARTESIAN_POINT('Ctrl Pts',(-5.52327404732735,5.66368927979123,148.396261840331));
#53445=CARTESIAN_POINT('Ctrl Pts',(-5.51820917972769,5.66862435147306,148.395975442637));
#53446=CARTESIAN_POINT('Ctrl Pts',(-5.51556711573298,5.67119511047733,148.395825999512));
#53447=CARTESIAN_POINT('Ctrl Pts',(-5.50868893813668,5.67787830440986,148.395436834124));
#53448=CARTESIAN_POINT('Ctrl Pts',(-5.50445002258888,5.68198783924278,148.395196884271));
#53449=CARTESIAN_POINT('Ctrl Pts',(-5.4862551480414,5.69958789862072,148.394166469421));
#53450=CARTESIAN_POINT('Ctrl Pts',(-5.47225426820697,5.71303167987043,148.393372390894));
#53451=CARTESIAN_POINT('Ctrl Pts',(-5.37372892377484,5.80694220330205,148.38777712729));
#53452=CARTESIAN_POINT('Ctrl Pts',(-5.28748588964605,5.88557821216553,148.382842150047));
#53453=CARTESIAN_POINT('Ctrl Pts',(-5.02569905531426,6.11387547205516,148.367840939935));
#53454=CARTESIAN_POINT('Ctrl Pts',(-4.84532029472162,6.25779389824532,148.357479564097));
#53455=CARTESIAN_POINT('Ctrl Pts',(-4.51317490384423,6.49982270225128,148.338721787915));
#53456=CARTESIAN_POINT('Ctrl Pts',(-4.3638394159758,6.60101105854147,148.330394439908));
#53457=CARTESIAN_POINT('Ctrl Pts',(-3.99678933189694,6.83181768334312,148.310369481882));
#53458=CARTESIAN_POINT('Ctrl Pts',(-3.77604505833299,6.95625960055671,148.298685325143));
#53459=CARTESIAN_POINT('Ctrl Pts',(-3.13138256934769,7.27993647787237,148.266008709818));
#53460=CARTESIAN_POINT('Ctrl Pts',(-2.69520571836805,7.45244887556802,148.245652454536));
#53461=CARTESIAN_POINT('Ctrl Pts',(-2.21544924007381,7.5945203667391,148.225323931461));
#53462=CARTESIAN_POINT('Ctrl Pts',(-2.18456222137497,7.60346255785421,148.224023610946));
#53463=CARTESIAN_POINT('Ctrl Pts',(-2.14326201593034,7.61514706591514,148.222296023244));
#53464=CARTESIAN_POINT('Ctrl Pts',(-2.13289673298962,7.61805673594162,148.221863375489));
#53465=CARTESIAN_POINT('Ctrl Pts',(-2.1167084924406,7.62256535692265,148.221189124472));
#53466=CARTESIAN_POINT('Ctrl Pts',(-2.11088960744574,7.62417881006936,148.220947055588));
#53467=CARTESIAN_POINT('Ctrl Pts',(-2.09976769885941,7.62724897028517,148.22048493337));
#53468=CARTESIAN_POINT('Ctrl Pts',(-2.09446499397367,7.62870681262968,148.220264843717));
#53469=CARTESIAN_POINT('Ctrl Pts',(-2.0820826234574,7.63209714332255,148.21975147245));
#53470=CARTESIAN_POINT('Ctrl Pts',(-2.07500177507332,7.63402531367505,148.219458329397));
#53471=CARTESIAN_POINT('Ctrl Pts',(-2.05478149625032,7.6395012424466,148.218622438149));
#53472=CARTESIAN_POINT('Ctrl Pts',(-2.041635550892,7.64302495811424,148.218080459983));
#53473=CARTESIAN_POINT('Ctrl Pts',(-1.95842877204707,7.66509819500693,148.214659227505));
#53474=CARTESIAN_POINT('Ctrl Pts',(-1.8881238719227,7.68271841106502,148.211809741363));
#53475=CARTESIAN_POINT('Ctrl Pts',(-1.68022062607629,7.73179800094543,148.203498978231));
#53476=CARTESIAN_POINT('Ctrl Pts',(-1.54200906600314,7.76054456982866,148.198122883539));
#53477=CARTESIAN_POINT('Ctrl Pts',(-1.23306479534329,7.81622175431553,148.186389871754));
#53478=CARTESIAN_POINT('Ctrl Pts',(-1.06206930170562,7.84128709913149,148.180086778253));
#53479=CARTESIAN_POINT('Ctrl Pts',(-0.476144606609255,7.90765478760128,
148.158954792078));
#53480=CARTESIAN_POINT('Ctrl Pts',(-0.0588370628559313,7.92175856032181,
148.144730754861));
#53481=CARTESIAN_POINT('Ctrl Pts',(0.735032008694882,7.8858337137424,148.117062605254));
#53482=CARTESIAN_POINT('Ctrl Pts',(1.11069911345139,7.84174395717142,148.103689703025));
#53483=CARTESIAN_POINT('Ctrl Pts',(1.55427855291734,7.7571638969136,148.086202855121));
#53484=CARTESIAN_POINT('Ctrl Pts',(1.62661389690692,7.74231878523468,148.083295804598));
#53485=CARTESIAN_POINT('Ctrl Pts',(1.70823157896408,7.72437444331806,148.079942501642));
#53486=CARTESIAN_POINT('Ctrl Pts',(1.71773046271818,7.72226765425011,148.079551108575));
#53487=CARTESIAN_POINT('Ctrl Pts',(1.73168680785101,7.71914520526742,148.078974362287));
#53488=CARTESIAN_POINT('Ctrl Pts',(1.73614734377517,7.71814318997965,148.078789776964));
#53489=CARTESIAN_POINT('Ctrl Pts',(1.74400705435517,7.71637042545534,148.078464076634));
#53490=CARTESIAN_POINT('Ctrl Pts',(1.74740659828806,7.71560129404987,148.078323053398));
#53491=CARTESIAN_POINT('Ctrl Pts',(1.75445713929826,7.71400124232155,148.078030265659));
#53492=CARTESIAN_POINT('Ctrl Pts',(1.75810804766525,7.71316997821378,148.07787848205));
#53493=CARTESIAN_POINT('Ctrl Pts',(1.76753288105133,7.71101702757333,148.077486209544));
#53494=CARTESIAN_POINT('Ctrl Pts',(1.77330590570613,7.7096914496989,148.077245500539));
#53495=CARTESIAN_POINT('Ctrl Pts',(1.79745332059851,7.70411826370192,148.076236883664));
#53496=CARTESIAN_POINT('Ctrl Pts',(1.81581385241687,7.69981147191977,148.07546566866));
#53497=CARTESIAN_POINT('Ctrl Pts',(1.94134500849951,7.6698919241853,148.070164204104));
#53498=CARTESIAN_POINT('Ctrl Pts',(2.04798171734216,7.6421091002705,148.065517679895));
#53499=CARTESIAN_POINT('Ctrl Pts',(2.37634494483499,7.54919214675338,148.050840980337));
#53500=CARTESIAN_POINT('Ctrl Pts',(2.59581708914995,7.47656606828914,148.040506954937));
#53501=CARTESIAN_POINT('Ctrl Pts',(3.00309594389115,7.32169573966932,148.020715655174));
#53502=CARTESIAN_POINT('Ctrl Pts',(3.19151137379599,7.24155144687217,148.011300062701));
#53503=CARTESIAN_POINT('Ctrl Pts',(3.97025895759536,6.87400152092731,147.971759281154));
#53504=CARTESIAN_POINT('Ctrl Pts',(4.52682266400117,6.52096542962951,147.942234803954));
#53505=CARTESIAN_POINT('Ctrl Pts',(5.06692873406214,6.07552805960929,147.913677337722));
#53506=CARTESIAN_POINT('Ctrl Pts',(5.10021357258826,6.04761354511706,147.911916459809));
#53507=CARTESIAN_POINT('Ctrl Pts',(5.14230412986137,6.01171941248033,147.909688236262));
#53508=CARTESIAN_POINT('Ctrl Pts',(5.15132376493752,6.00399246574771,147.909210658862));
#53509=CARTESIAN_POINT('Ctrl Pts',(5.16558309384168,5.99172098869538,147.908455498405));
#53510=CARTESIAN_POINT('Ctrl Pts',(5.17083425372177,5.98718984387565,147.908177369966));
#53511=CARTESIAN_POINT('Ctrl Pts',(5.18023445451904,5.97905696435531,147.907679427706));
#53512=CARTESIAN_POINT('Ctrl Pts',(5.18438571180846,5.97545780490032,147.907459508813));
#53513=CARTESIAN_POINT('Ctrl Pts',(5.19389305945674,5.9671975248454,147.906955794362));
#53514=CARTESIAN_POINT('Ctrl Pts',(5.19924663440435,5.96253350921946,147.906672117775));
#53515=CARTESIAN_POINT('Ctrl Pts',(5.21402073154748,5.94962734041811,147.905889162303));
#53516=CARTESIAN_POINT('Ctrl Pts',(5.22342800055496,5.9413700106717,147.905390507995));
#53517=CARTESIAN_POINT('Ctrl Pts',(5.27408649890585,5.89669066699126,147.902704578308));
#53518=CARTESIAN_POINT('Ctrl Pts',(5.31497691309309,5.85986090164036,147.900534211307));
#53519=CARTESIAN_POINT('Ctrl Pts',(5.50949302237821,5.68095011801749,147.890195000266));
#53520=CARTESIAN_POINT('Ctrl Pts',(5.65782993461925,5.53323372354095,147.882268622808));
#53521=CARTESIAN_POINT('Ctrl Pts',(5.93530290248307,5.23408096556415,147.867232290146));
#53522=CARTESIAN_POINT('Ctrl Pts',(6.06492732134635,5.0833143860368,147.860106424396));
#53523=CARTESIAN_POINT('Ctrl Pts',(6.67884158402428,4.31231332320873,147.825399965357));
#53524=CARTESIAN_POINT('Ctrl Pts',(7.07429577031348,3.62724800941383,147.800275370008));
#53525=CARTESIAN_POINT('Ctrl Pts',(7.37841773920854,2.85391773125621,147.767636923401));
#53526=CARTESIAN_POINT('Ctrl Pts',(7.39432821852242,2.81243752069445,147.765873028821));
#53527=CARTESIAN_POINT('Ctrl Pts',(7.41250649815316,2.76382421632936,147.763788098943));
#53528=CARTESIAN_POINT('Ctrl Pts',(7.41511487590344,2.7568185033495,147.763487209687));
#53529=CARTESIAN_POINT('Ctrl Pts',(7.41926068415732,2.7456350300021,147.763006191873));
#53530=CARTESIAN_POINT('Ctrl Pts',(7.42080452973278,2.74145963836216,147.762826447147));
#53531=CARTESIAN_POINT('Ctrl Pts',(7.42352272867965,2.73408904120906,147.762508876492));
#53532=CARTESIAN_POINT('Ctrl Pts',(7.4246985467434,2.73089437335107,147.762371138848));
#53533=CARTESIAN_POINT('Ctrl Pts',(7.42712466168525,2.72428953166578,147.762086180699));
#53534=CARTESIAN_POINT('Ctrl Pts',(7.42837467252755,2.72087925439996,147.761938942919));
#53535=CARTESIAN_POINT('Ctrl Pts',(7.43157261749131,2.7121359969833,147.761561182414));
#53536=CARTESIAN_POINT('Ctrl Pts',(7.43351714388872,2.70680182250626,147.761330453496));
#53537=CARTESIAN_POINT('Ctrl Pts',(7.44166003651497,2.6843894991263,147.760359916198));
#53538=CARTESIAN_POINT('Ctrl Pts',(7.44780524813394,2.66729227073327,147.759616881641));
#53539=CARTESIAN_POINT('Ctrl Pts',(7.48959725703416,2.54974788335504,147.754491039096));
#53540=CARTESIAN_POINT('Ctrl Pts',(7.52326840734035,2.44861428859249,147.74999360827));
#53541=CARTESIAN_POINT('Ctrl Pts',(7.60155984612015,2.19658012052913,147.738628709491));
#53542=CARTESIAN_POINT('Ctrl Pts',(7.64374011171562,2.0449716652365,147.731655458579));
#53543=CARTESIAN_POINT('Ctrl Pts',(7.76157322352243,1.56663259911239,147.709447980611));
#53544=CARTESIAN_POINT('Ctrl Pts',(7.82099366487555,1.23628781987725,147.693828965333));
#53545=CARTESIAN_POINT('Ctrl Pts',(7.89522874391354,0.59030802259276,147.663789306108));
#53546=CARTESIAN_POINT('Ctrl Pts',(7.91247045273205,0.275557006149398,147.649380083742));
#53547=CARTESIAN_POINT('Ctrl Pts',(7.9092144286864,-0.378229125280889,147.620444312156));
#53548=CARTESIAN_POINT('Ctrl Pts',(7.88576056627405,-0.716623088197248,
147.606025698784));
#53549=CARTESIAN_POINT('Ctrl Pts',(7.83768124596388,-1.07479278363729,147.591407139106));
#53550=CARTESIAN_POINT('Ctrl Pts',(7.83459392930034,-1.09707101651083,147.59050043064));
#53551=CARTESIAN_POINT('Ctrl Pts',(7.8301540947938,-1.12813423125074,147.589239721103));
#53552=CARTESIAN_POINT('Ctrl Pts',(7.82888173003655,-1.1369304506973,147.588883120565));
#53553=CARTESIAN_POINT('Ctrl Pts',(7.82671450949683,-1.15173691008189,147.588283527779));
#53554=CARTESIAN_POINT('Ctrl Pts',(7.82582754914811,-1.157748286295,147.588040279396));
#53555=CARTESIAN_POINT('Ctrl Pts',(7.82414827562132,-1.16903946253727,147.587583730715));
#53556=CARTESIAN_POINT('Ctrl Pts',(7.82335754226196,-1.17431949228743,147.587370379235));
#53557=CARTESIAN_POINT('Ctrl Pts',(7.8213904782326,-1.18736416498312,147.586843629098));
#53558=CARTESIAN_POINT('Ctrl Pts',(7.82020792834831,-1.19512787229747,147.58653043271));
#53559=CARTESIAN_POINT('Ctrl Pts',(7.81642429181523,-1.21972223316322,147.585539233222));
#53560=CARTESIAN_POINT('Ctrl Pts',(7.8137804082903,-1.23654630788361,147.584862621857));
#53561=CARTESIAN_POINT('Ctrl Pts',(7.77114370386214,-1.50226272561509,147.574198662081));
#53562=CARTESIAN_POINT('Ctrl Pts',(7.71932980497701,-1.74912225790972,147.564608268771));
#53563=CARTESIAN_POINT('Ctrl Pts',(7.60590931723317,-2.18478797513713,147.548059670667));
#53564=CARTESIAN_POINT('Ctrl Pts',(7.54882322874031,-2.37453730989995,147.540982091399));
#53565=CARTESIAN_POINT('Ctrl Pts',(7.23103272131675,-3.30295453489013,147.506561783295));
#53566=CARTESIAN_POINT('Ctrl Pts',(6.86881183373858,-4.00204502466144,147.481725711336));
#53567=CARTESIAN_POINT('Ctrl Pts',(6.38391620959262,-4.67241978700235,147.449232658954));
#53568=CARTESIAN_POINT('Ctrl Pts',(6.35758932760608,-4.70817912079544,147.447469099326));
#53569=CARTESIAN_POINT('Ctrl Pts',(6.32657649121231,-4.74956886688329,147.445389947481));
#53570=CARTESIAN_POINT('Ctrl Pts',(6.3221815948993,-4.75541737399408,147.445095267313));
#53571=CARTESIAN_POINT('Ctrl Pts',(6.31517026032976,-4.76472080665741,147.444625076769));
#53572=CARTESIAN_POINT('Ctrl Pts',(6.3125590766239,-4.7681797036503,147.444449950009));
#53573=CARTESIAN_POINT('Ctrl Pts',(6.30795409088466,-4.77426927215136,147.444141069909));
#53574=CARTESIAN_POINT('Ctrl Pts',(6.30596148009766,-4.77690084753458,147.444007404356));
#53575=CARTESIAN_POINT('Ctrl Pts',(6.30184049943086,-4.78233621894065,147.443730942207));
#53576=CARTESIAN_POINT('Ctrl Pts',(6.29971191243885,-4.78513983195751,147.443588129163));
#53577=CARTESIAN_POINT('Ctrl Pts',(6.29422240281678,-4.79236018547139,147.443219788102));
#53578=CARTESIAN_POINT('Ctrl Pts',(6.29085870929139,-4.79677480218072,147.442994054876));
#53579=CARTESIAN_POINT('Ctrl Pts',(6.276840136198,-4.81513310906028,147.442053164647));
#53580=CARTESIAN_POINT('Ctrl Pts',(6.26614359551777,-4.82904476932111,147.441334949204));
#53581=CARTESIAN_POINT('Ctrl Pts',(6.193410077902,-4.92299165604127,147.43645001041));
#53582=CARTESIAN_POINT('Ctrl Pts',(6.12988999094503,-5.00186188030843,147.432177682796));
#53583=CARTESIAN_POINT('Ctrl Pts',(5.91657821073534,-5.25655479407876,147.417874033677));
#53584=CARTESIAN_POINT('Ctrl Pts',(5.76060524623282,-5.42703237305624,147.407484983798));
#53585=CARTESIAN_POINT('Ctrl Pts',(5.54919254572091,-5.63870895343066,147.393762502684));
#53586=CARTESIAN_POINT('Ctrl Pts',(5.50035341283223,-5.68635988328701,147.390615354296));
#53587=CARTESIAN_POINT('Ctrl Pts',(5.32411781332532,-5.85391282173301,147.379356838872));
#53588=CARTESIAN_POINT('Ctrl Pts',(5.19336853283439,-5.97021341680011,147.371183686555));
#53589=CARTESIAN_POINT('Ctrl Pts',(5.00465278059966,-6.12718084850084,147.359731545663));
#53590=CARTESIAN_POINT('Ctrl Pts',(4.94983235730225,-6.17155201717955,147.356443402943));
#53591=CARTESIAN_POINT('Ctrl Pts',(4.8736582885577,-6.23153870574493,147.351932371006));
#53592=CARTESIAN_POINT('Ctrl Pts',(4.85280886932392,-6.24778887592645,147.350703517767));
#53593=CARTESIAN_POINT('Ctrl Pts',(4.81198468946208,-6.27927986264132,147.34830910058));
#53594=CARTESIAN_POINT('Ctrl Pts',(4.79201798958187,-6.29453062890741,147.347143430159));
#53595=CARTESIAN_POINT('Ctrl Pts',(4.75288503744982,-6.32412665342139,147.344869660389));
#53596=CARTESIAN_POINT('Ctrl Pts',(4.73372564642155,-6.33848054488581,147.343761450202));
#53597=CARTESIAN_POINT('Ctrl Pts',(4.48495464062853,-6.52309850461027,147.329438551072));
#53598=CARTESIAN_POINT('Ctrl Pts',(4.24633270470723,-6.68089129609932,147.316440460884));
#53599=CARTESIAN_POINT('Ctrl Pts',(3.73613054745982,-6.97986812395028,147.29042433546));
#53600=CARTESIAN_POINT('Ctrl Pts',(3.46384239562063,-7.11892229455873,147.277490153354));
#53601=CARTESIAN_POINT('Ctrl Pts',(3.16487452184701,-7.25037478776653,147.264274917261));
#53602=CARTESIAN_POINT('Ctrl Pts',(3.14554492703048,-7.25878174512276,147.263424697256));
#53603=CARTESIAN_POINT('Ctrl Pts',(3.11885391029224,-7.27026374504147,147.262256423046));
#53604=CARTESIAN_POINT('Ctrl Pts',(3.11152118116277,-7.27340501937474,147.261936062603));
#53605=CARTESIAN_POINT('Ctrl Pts',(3.09895698223819,-7.27876493043158,147.261388159598));
#53606=CARTESIAN_POINT('Ctrl Pts',(3.09372785711837,-7.2809890287324,147.26116042728));
#53607=CARTESIAN_POINT('Ctrl Pts',(3.08310830553083,-7.28549232568808,147.260698546738));
#53608=CARTESIAN_POINT('Ctrl Pts',(3.07771773660136,-7.28777118090987,147.260464410526));
#53609=CARTESIAN_POINT('Ctrl Pts',(3.06533775182537,-7.29298861607669,147.259927421016));
#53610=CARTESIAN_POINT('Ctrl Pts',(3.05834662524347,-7.29592313605843,147.259624708525));
#53611=CARTESIAN_POINT('Ctrl Pts',(3.04367927068535,-7.30205496035293,147.258990729963));
#53612=CARTESIAN_POINT('Ctrl Pts',(3.03600219619126,-7.30525022241433,147.258659534704));
#53613=CARTESIAN_POINT('Ctrl Pts',(3.01571643378002,-7.31365582434048,147.257786064805));
#53614=CARTESIAN_POINT('Ctrl Pts',(3.00309925598472,-7.31884567312467,147.257244496669));
#53615=CARTESIAN_POINT('Ctrl Pts',(2.96527250767284,-7.33429073886641,147.255625925291));
#53616=CARTESIAN_POINT('Ctrl Pts',(2.94002326199174,-7.34444857868534,147.254552262836));
#53617=CARTESIAN_POINT('Ctrl Pts',(2.6600979644896,-7.45538842083882,147.242722330809));
#53618=CARTESIAN_POINT('Ctrl Pts',(2.40039556468224,-7.54301364581422,147.232425205799));
#53619=CARTESIAN_POINT('Ctrl Pts',(1.42740195179222,-7.81594948556875,147.195696820419));
#53620=CARTESIAN_POINT('Ctrl Pts',(0.693926166972634,-7.91484995316757,
147.171898875596));
#53621=CARTESIAN_POINT('Ctrl Pts',(-0.264972799758299,-7.90968828836991,
147.136974349162));
#53622=CARTESIAN_POINT('Ctrl Pts',(-0.487210570889519,-7.89911433551051,
147.128575362273));
#53623=CARTESIAN_POINT('Ctrl Pts',(-0.724442810736541,-7.87777589374369,
147.119054345134));
#53624=CARTESIAN_POINT('Ctrl Pts',(-0.74016792610319,-7.87631397633031,
147.118420850828));
#53625=CARTESIAN_POINT('Ctrl Pts',(-0.761746669491083,-7.87424267128036,
147.117548353959));
#53626=CARTESIAN_POINT('Ctrl Pts',(-0.767604227070623,-7.87367381753953,
147.117311191943));
#53627=CARTESIAN_POINT('Ctrl Pts',(-0.777603765633786,-7.87269145278235,
147.116905783793));
#53628=CARTESIAN_POINT('Ctrl Pts',(-0.781746070554488,-7.87228120738246,
147.116737683986));
#53629=CARTESIAN_POINT('Ctrl Pts',(-0.789781156683354,-7.87147902442379,
147.116411302963));
#53630=CARTESIAN_POINT('Ctrl Pts',(-0.793673975944867,-7.87108746789276,
147.116253038673));
#53631=CARTESIAN_POINT('Ctrl Pts',(-0.802947350066434,-7.87014776252027,
147.115875694367));
#53632=CARTESIAN_POINT('Ctrl Pts',(-0.808327632158715,-7.86959698394783,
147.115656498815));
#53633=CARTESIAN_POINT('Ctrl Pts',(-0.824319029222221,-7.86794337487276,
147.115004218826));
#53634=CARTESIAN_POINT('Ctrl Pts',(-0.834928455343997,-7.86682459986257,
147.114570442701));
#53635=CARTESIAN_POINT('Ctrl Pts',(-0.921199569797452,-7.8575507349788,
147.111035004269));
#53636=CARTESIAN_POINT('Ctrl Pts',(-0.996740622014635,-7.84832592380449,
147.107888225247));
#53637=CARTESIAN_POINT('Ctrl Pts',(-1.43099667393972,-7.78892552127458,
147.089544810863));
#53638=CARTESIAN_POINT('Ctrl Pts',(-1.78604880867886,-7.71525236003017,
147.07356676));
#53639=CARTESIAN_POINT('Ctrl Pts',(-2.66287500766157,-7.46952472933315,
147.033189570492));
#53640=CARTESIAN_POINT('Ctrl Pts',(-3.17418813919936,-7.2670020763461,147.008886879855));
#53641=CARTESIAN_POINT('Ctrl Pts',(-3.84058693153651,-6.91918351647105,
146.977280065042));
#53642=CARTESIAN_POINT('Ctrl Pts',(-4.01703621966544,-6.81825740125398,
146.968900633639));
#53643=CARTESIAN_POINT('Ctrl Pts',(-4.19558481845984,-6.70679073930889,
146.960388728017));
#53644=CARTESIAN_POINT('Ctrl Pts',(-4.20175438767153,-6.70292727513101,
146.960094562339));
#53645=CARTESIAN_POINT('Ctrl Pts',(-4.21498684211986,-6.69461549249407,
146.959463536559));
#53646=CARTESIAN_POINT('Ctrl Pts',(-4.2220480396606,-6.69016449893049,146.959126742113));
#53647=CARTESIAN_POINT('Ctrl Pts',(-4.23708962740804,-6.68064980496048,
146.958409172855));
#53648=CARTESIAN_POINT('Ctrl Pts',(-4.24506801686404,-6.67558296030649,
146.958028475205));
#53649=CARTESIAN_POINT('Ctrl Pts',(-4.26377629368547,-6.66365477235136,
146.957135584038));
#53650=CARTESIAN_POINT('Ctrl Pts',(-4.27449873902532,-6.65678178544482,
146.956623674359));
#53651=CARTESIAN_POINT('Ctrl Pts',(-4.29318247822905,-6.64474192768985,
146.955731381361));
#53652=CARTESIAN_POINT('Ctrl Pts',(-4.30115114796233,-6.63958657446708,
146.955350721343));
#53653=CARTESIAN_POINT('Ctrl Pts',(-4.31738675145416,-6.62904141108799,
146.954574951285));
#53654=CARTESIAN_POINT('Ctrl Pts',(-4.32565291784011,-6.62365044567749,
146.954179870141));
#53655=CARTESIAN_POINT('Ctrl Pts',(-4.34611076008194,-6.61025377639325,
146.953201820104));
#53656=CARTESIAN_POINT('Ctrl Pts',(-4.35829043946903,-6.6022297880615,146.95261929647));
#53657=CARTESIAN_POINT('Ctrl Pts',(-4.40346132160714,-6.5722916878667,146.95045798881));
#53658=CARTESIAN_POINT('Ctrl Pts',(-4.43631017106618,-6.550163490004,146.948884477606));
#53659=CARTESIAN_POINT('Ctrl Pts',(-4.62718926098445,-6.41948570479533,
146.939729903226));
#53660=CARTESIAN_POINT('Ctrl Pts',(-4.78140126280387,-6.30546455737791,
146.932291023522));
#53661=CARTESIAN_POINT('Ctrl Pts',(-5.06869271538402,-6.07644120466206,
146.918290195343));
#53662=CARTESIAN_POINT('Ctrl Pts',(-5.20237889813908,-5.96238542035076,
146.911710599816));
#53663=CARTESIAN_POINT('Ctrl Pts',(-5.88333562283849,-5.34106642573863,
146.877621751639));
#53664=CARTESIAN_POINT('Ctrl Pts',(-6.36052460095868,-4.76278422421943,
146.852072947798));
#53665=CARTESIAN_POINT('Ctrl Pts',(-6.78023025731822,-4.07625361827561,
146.820500614373));
#53666=CARTESIAN_POINT('Ctrl Pts',(-6.81028555485571,-4.02583858606354,
146.81817346005));
#53667=CARTESIAN_POINT('Ctrl Pts',(-6.84463846831642,-3.96672898766845,
146.815430105813));
#53668=CARTESIAN_POINT('Ctrl Pts',(-6.84948503047238,-3.95835438531086,
146.81504108488));
#53669=CARTESIAN_POINT('Ctrl Pts',(-6.85718233882849,-3.94499737935321,
146.814420040561));
#53670=CARTESIAN_POINT('Ctrl Pts',(-6.86004305727132,-3.94002071100837,
146.814188518869));
#53671=CARTESIAN_POINT('Ctrl Pts',(-6.86507621408844,-3.93124264640356,
146.813779919009));
#53672=CARTESIAN_POINT('Ctrl Pts',(-6.86725092026755,-3.92744254803497,
146.813602956217));
#53673=CARTESIAN_POINT('Ctrl Pts',(-6.87173428210063,-3.91959317821807,
146.813237265763));
#53674=CARTESIAN_POINT('Ctrl Pts',(-6.87404251554839,-3.9155436686142,146.813048516586));
#53675=CARTESIAN_POINT('Ctrl Pts',(-6.87992867086586,-3.90519589183057,
146.812565971342));
#53676=CARTESIAN_POINT('Ctrl Pts',(-6.88350151840562,-3.8988947556134,146.812271913319));
#53677=CARTESIAN_POINT('Ctrl Pts',(-6.89792215031076,-3.87338067076191,
146.811080319352));
#53678=CARTESIAN_POINT('Ctrl Pts',(-6.90869811204368,-3.85412742309881,
146.810179027823));
#53679=CARTESIAN_POINT('Ctrl Pts',(-6.97608728616633,-3.73253343833869,
146.804472300182));
#53680=CARTESIAN_POINT('Ctrl Pts',(-7.03049932969253,-3.62900455969918,
146.799539917991));
#53681=CARTESIAN_POINT('Ctrl Pts',(-7.15093558249259,-3.3869713512484,146.787888806798));
#53682=CARTESIAN_POINT('Ctrl Pts',(-7.21526556239071,-3.24767512257988,
146.781099554338));
#53683=CARTESIAN_POINT('Ctrl Pts',(-7.65056755156856,-2.22822051914534,
146.731257767539));
#53684=CARTESIAN_POINT('Ctrl Pts',(-7.8635908985282,-1.28879029546252,146.68576265606));
#53685=CARTESIAN_POINT('Ctrl Pts',(-7.90557380768858,-0.295490631218893,
146.645226367397));
#53686=CARTESIAN_POINT('Ctrl Pts',(-7.90692190982321,-0.256900584353839,
146.643660990879));
#53687=CARTESIAN_POINT('Ctrl Pts',(-7.90831138068428,-0.206566981904476,
146.641631442917));
#53688=CARTESIAN_POINT('Ctrl Pts',(-7.90860920427075,-0.194831382413272,
146.641159104917));
#53689=CARTESIAN_POINT('Ctrl Pts',(-7.90905439448839,-0.175601179965185,
146.640386530699));
#53690=CARTESIAN_POINT('Ctrl Pts',(-7.90921723276855,-0.168106973880743,
146.640085801187));
#53691=CARTESIAN_POINT('Ctrl Pts',(-7.9094843670096,-0.15495193955771,146.639558525692));
#53692=CARTESIAN_POINT('Ctrl Pts',(-7.90959323787568,-0.149291215646896,
146.639331833835));
#53693=CARTESIAN_POINT('Ctrl Pts',(-7.90979661746725,-0.138091141967158,
146.638883704002));
#53694=CARTESIAN_POINT('Ctrl Pts',(-7.90989138443403,-0.132551800467134,
146.638662257907));
#53695=CARTESIAN_POINT('Ctrl Pts',(-7.91008347407537,-0.120588985773937,
146.638184430707));
#53696=CARTESIAN_POINT('Ctrl Pts',(-7.91017879149016,-0.114165481847901,
146.637928113781));
#53697=CARTESIAN_POINT('Ctrl Pts',(-7.91039063560605,-0.0986121640945126,
146.637308106009));
#53698=CARTESIAN_POINT('Ctrl Pts',(-7.91049918122022,-0.0894822409103802,
146.636944670265));
#53699=CARTESIAN_POINT('Ctrl Pts',(-7.91086278010519,-0.0536862713631455,
146.635521741244));
#53700=CARTESIAN_POINT('Ctrl Pts',(-7.910998807096,-0.0270190770009432,
146.634466053238));
#53701=CARTESIAN_POINT('Ctrl Pts',(-7.91099999218839,-0.000351561277017258,
146.633414644735));
#53702=CARTESIAN_POINT('',(-7.91099997917165,0.000559131365739208,144.642309010809));
#53703=CARTESIAN_POINT('Ctrl Pts',(-7.91099986071816,0.0014844922367362,
146.642331508237));
#53704=CARTESIAN_POINT('Ctrl Pts',(-7.91096070114018,0.210169595666695,
146.63397861785));
#53705=CARTESIAN_POINT('Ctrl Pts',(-7.90265989499709,0.418657654408056,
146.625625727462));
#53706=CARTESIAN_POINT('Ctrl Pts',(-7.88616961499353,0.626298493972929,
146.617272837075));
#53707=CARTESIAN_POINT('Ctrl Pts',(-7.8696532919512,0.834267259954797,146.608906754998));
#53708=CARTESIAN_POINT('Ctrl Pts',(-7.84492168017966,1.04138585805498,146.600540672921));
#53709=CARTESIAN_POINT('Ctrl Pts',(-7.81209836721751,1.24701247023335,146.592174590845));
#53710=CARTESIAN_POINT('Ctrl Pts',(-7.77922265175918,1.45296736578069,146.583795152298));
#53711=CARTESIAN_POINT('Ctrl Pts',(-7.73822947183251,1.65742524414367,146.575415713752));
#53712=CARTESIAN_POINT('Ctrl Pts',(-7.68929294810761,1.85975669327539,146.567036275206));
#53713=CARTESIAN_POINT('Ctrl Pts',(-7.64023459965335,2.06259183519428,146.558635976518));
#53714=CARTESIAN_POINT('Ctrl Pts',(-7.58319341738956,2.26328968901699,146.550235677829));
#53715=CARTESIAN_POINT('Ctrl Pts',(-7.51839346328524,2.46123561066994,146.541835379141));
#53716=CARTESIAN_POINT('Ctrl Pts',(-7.45350555941553,2.65945019450961,146.533423679144));
#53717=CARTESIAN_POINT('Ctrl Pts',(-7.38083794575107,2.85490512674468,146.525011979146));
#53718=CARTESIAN_POINT('Ctrl Pts',(-7.30066244530874,3.04700654079683,146.516600279149));
#53719=CARTESIAN_POINT('Ctrl Pts',(-7.22031945268051,3.23950926803784,146.508171006527));
#53720=CARTESIAN_POINT('Ctrl Pts',(-7.13243732293407,3.42864421540676,146.499741733904));
#53721=CARTESIAN_POINT('Ctrl Pts',(-7.03733443343984,3.61384076460515,146.491312461282));
#53722=CARTESIAN_POINT('Ctrl Pts',(-7.00368404685071,3.6793691150963,146.488329920121));
#53723=CARTESIAN_POINT('Ctrl Pts',(-6.96913004297996,3.74440465389762,146.485347378961));
#53724=CARTESIAN_POINT('Ctrl Pts',(-6.93368780882427,3.8089229934145,146.4823648378));
#53725=CARTESIAN_POINT('Ctrl Pts',(-6.84048602586118,3.97858566903415,146.474521704867));
#53726=CARTESIAN_POINT('Ctrl Pts',(-6.7409070111708,4.1450914995612,146.466678571934));
#53727=CARTESIAN_POINT('Ctrl Pts',(-6.63518906266479,4.30792143645791,146.458835439));
#53728=CARTESIAN_POINT('Ctrl Pts',(-6.52959526863741,4.47056014692423,146.451001516992));
#53729=CARTESIAN_POINT('Ctrl Pts',(-6.41787708549216,4.6295312680319,146.443167594984));
#53730=CARTESIAN_POINT('Ctrl Pts',(-6.30031954512722,4.7843384735288,146.435333672975));
#53731=CARTESIAN_POINT('Ctrl Pts',(-6.18287720066292,4.93899398177679,146.427507427512));
#53732=CARTESIAN_POINT('Ctrl Pts',(-6.05960710492921,5.089493422178,146.419681182048));
#53733=CARTESIAN_POINT('Ctrl Pts',(-5.93083870144767,5.23536754176921,146.411854936584));
#53734=CARTESIAN_POINT('Ctrl Pts',(-5.8021714510098,5.38112707105105,146.404034838968));
#53735=CARTESIAN_POINT('Ctrl Pts',(-5.66801472669524,5.52226825387506,146.396214741352));
#53736=CARTESIAN_POINT('Ctrl Pts',(-5.52873965068755,5.65835301787679,146.388394643737));
#53737=CARTESIAN_POINT('Ctrl Pts',(-5.38954692141156,5.79435732142665,146.380579169773));
#53738=CARTESIAN_POINT('Ctrl Pts',(-5.2452421193869,5.92531091647335,146.372763695809));
#53739=CARTESIAN_POINT('Ctrl Pts',(-5.09623492766473,6.05081073593035,146.364948221845));
#53740=CARTESIAN_POINT('Ctrl Pts',(-4.94728689410474,6.17626073001594,146.357135850745));
#53741=CARTESIAN_POINT('Ctrl Pts',(-4.79364045898952,6.29626103633434,146.349323479645));
#53742=CARTESIAN_POINT('Ctrl Pts',(-4.63574039303495,6.41044709894592,146.341511108546));
#53743=CARTESIAN_POINT('Ctrl Pts',(-4.47784630416448,6.52462883920529,146.333699033172));
#53744=CARTESIAN_POINT('Ctrl Pts',(-4.31569918478182,6.6329965609269,146.325886957799));
#53745=CARTESIAN_POINT('Ctrl Pts',(-4.14977533552394,6.73522721700443,146.318074882425));
#53746=CARTESIAN_POINT('Ctrl Pts',(-3.98384663351259,6.83746086300879,146.310262578573));
#53747=CARTESIAN_POINT('Ctrl Pts',(-3.81414128072488,6.93355690060145,146.302450274721));
#53748=CARTESIAN_POINT('Ctrl Pts',(-3.64116286195743,7.02323671911335,146.294637970868));
#53749=CARTESIAN_POINT('Ctrl Pts',(-3.46814894800641,7.11293493993024,146.286824063931));
#53750=CARTESIAN_POINT('Ctrl Pts',(-3.29186094242496,7.19621415697964,146.279010156993));
#53751=CARTESIAN_POINT('Ctrl Pts',(-3.11282535646868,7.27284258733308,146.271196250056));
#53752=CARTESIAN_POINT('Ctrl Pts',(-2.93372152828843,7.3495002258156,146.263379364725));
#53753=CARTESIAN_POINT('Ctrl Pts',(-2.7518683566932,7.41950188962338,146.255562479394));
#53754=CARTESIAN_POINT('Ctrl Pts',(-2.56781070895024,7.48266457640595,146.247745594063));
#53755=CARTESIAN_POINT('Ctrl Pts',(-2.38355339760369,7.54589578133928,146.239920229066));
#53756=CARTESIAN_POINT('Ctrl Pts',(-2.19708716662012,7.60227307761764,146.232094864069));
#53757=CARTESIAN_POINT('Ctrl Pts',(-2.00897138739168,7.65166354230514,146.224269499071));
#53758=CARTESIAN_POINT('Ctrl Pts',(-1.82074127972997,7.70108402432807,146.216439378164));
#53759=CARTESIAN_POINT('Ctrl Pts',(-1.63085996805879,7.74350913581897,146.208609257256));
#53760=CARTESIAN_POINT('Ctrl Pts',(-1.43989538263479,7.77885738955709,146.200779136349));
#53761=CARTESIAN_POINT('Ctrl Pts',(-1.24866976128388,7.81425396201442,146.192938312185));
#53762=CARTESIAN_POINT('Ctrl Pts',(-1.05635825535513,7.84255430455995,146.185097488022));
#53763=CARTESIAN_POINT('Ctrl Pts',(-0.863533404153835,7.86372882670241,
146.177256663858));
#53764=CARTESIAN_POINT('Ctrl Pts',(-0.759466757756689,7.87515661463898,
146.173025008703));
#53765=CARTESIAN_POINT('Ctrl Pts',(-0.655250596235465,7.88450975841976,
146.168793353547));
#53766=CARTESIAN_POINT('Ctrl Pts',(-0.550974645430076,7.89178990724495,
146.164561698391));
#53767=CARTESIAN_POINT('Ctrl Pts',(-0.35602841327858,7.90540030899158,146.156650524032));
#53768=CARTESIAN_POINT('Ctrl Pts',(-0.160315528008974,7.91180125141527,
146.148739349672));
#53769=CARTESIAN_POINT('Ctrl Pts',(0.0355883609934201,7.91091995083769,
146.140828175313));
#53770=CARTESIAN_POINT('Ctrl Pts',(0.231279864754714,7.91003960570432,146.132925577693));
#53771=CARTESIAN_POINT('Ctrl Pts',(0.427161618077138,7.90189274456782,146.125022980073));
#53772=CARTESIAN_POINT('Ctrl Pts',(0.622652724432515,7.88645830425526,146.117120382454));
#53773=CARTESIAN_POINT('Ctrl Pts',(0.817968181673127,7.87103773181541,146.109224885332));
#53774=CARTESIAN_POINT('Ctrl Pts',(1.01289334956661,7.84834265117043,146.101329388211));
#53775=CARTESIAN_POINT('Ctrl Pts',(1.20684691750255,7.81840402625207,146.093433891089));
#53776=CARTESIAN_POINT('Ctrl Pts',(1.4006622098253,7.78848674552327,146.085544022917));
#53777=CARTESIAN_POINT('Ctrl Pts',(1.59350694285165,7.751336261671,146.077654154744));
#53778=CARTESIAN_POINT('Ctrl Pts',(1.78480423289768,7.70703541254551,146.069764286572));
#53779=CARTESIAN_POINT('Ctrl Pts',(1.97600063222358,7.66275792781044,146.061878579537));
#53780=CARTESIAN_POINT('Ctrl Pts',(2.16565087967339,7.61133766989136,146.053992872503));
#53781=CARTESIAN_POINT('Ctrl Pts',(2.35318732353836,7.55290873904474,146.046107165469));
#53782=CARTESIAN_POINT('Ctrl Pts',(2.54065964789161,7.49449978529931,146.038224154591));
#53783=CARTESIAN_POINT('Ctrl Pts',(2.72601928024173,7.42908703698421,146.030341143714));
#53784=CARTESIAN_POINT('Ctrl Pts',(2.90871252642285,7.35685479254762,146.022458132837));
#53785=CARTESIAN_POINT('Ctrl Pts',(3.09140849903498,7.28462147014981,146.014575004317));
#53786=CARTESIAN_POINT('Ctrl Pts',(3.2714376822132,7.20556856719058,146.006691875797));
#53787=CARTESIAN_POINT('Ctrl Pts',(3.44826466930564,7.11992919700881,145.998808747277));
#53788=CARTESIAN_POINT('Ctrl Pts',(3.62510258979157,7.03428453165718,145.990925131335));
#53789=CARTESIAN_POINT('Ctrl Pts',(3.79873760886763,6.94205273744811,145.983041515394));
#53790=CARTESIAN_POINT('Ctrl Pts',(3.9686572868143,6.8435137422099,145.975157899452));
#53791=CARTESIAN_POINT('Ctrl Pts',(4.13861603366217,6.74495209032407,145.967272470864));
#53792=CARTESIAN_POINT('Ctrl Pts',(4.30485743874423,6.64008052073081,145.959387042277));
#53793=CARTESIAN_POINT('Ctrl Pts',(4.46689629992931,6.52922341826943,145.951501613689));
#53794=CARTESIAN_POINT('Ctrl Pts',(4.62899965623215,6.41832219218346,145.943613046523));
#53795=CARTESIAN_POINT('Ctrl Pts',(4.78689685115993,6.30143088072875,145.935724479357));
#53796=CARTESIAN_POINT('Ctrl Pts',(4.94013394429008,6.17891556929474,145.927835912191));
#53797=CARTESIAN_POINT('Ctrl Pts',(5.09353411499974,6.05626987493559,145.919938949875));
#53798=CARTESIAN_POINT('Ctrl Pts',(5.24226400858081,5.92798844126273,145.912041987559));
#53799=CARTESIAN_POINT('Ctrl Pts',(5.38590406968878,5.79447653823103,145.904145025243));
#53800=CARTESIAN_POINT('Ctrl Pts',(5.52963173212614,5.66088321069906,145.89624324683));
#53801=CARTESIAN_POINT('Ctrl Pts',(5.66826313053842,5.52205329771764,145.888341468417));
#53802=CARTESIAN_POINT('Ctrl Pts',(5.80141734995539,5.37842706854305,145.880439690004));
#53803=CARTESIAN_POINT('Ctrl Pts',(5.93474378375484,5.23461508106149,145.872527691863));
#53804=CARTESIAN_POINT('Ctrl Pts',(6.06257866500054,5.08599464756745,145.864615693723));
#53805=CARTESIAN_POINT('Ctrl Pts',(6.18458224618046,4.93303795244163,145.856703695582));
#53806=CARTESIAN_POINT('Ctrl Pts',(6.23570048705311,4.86895067640507,145.85338865005));
#53807=CARTESIAN_POINT('Ctrl Pts',(6.28579556031459,4.80410249859803,145.850073604517));
#53808=CARTESIAN_POINT('Ctrl Pts',(6.33484481640776,4.7385295347852,145.846758558985));
#53809=CARTESIAN_POINT('Ctrl Pts',(6.45189805716921,4.58204341181436,145.838847392664));
#53810=CARTESIAN_POINT('Ctrl Pts',(6.56330678818272,4.42100714550051,145.830936226343));
#53811=CARTESIAN_POINT('Ctrl Pts',(6.66869797636449,4.25586516469122,145.823025060023));
#53812=CARTESIAN_POINT('Ctrl Pts',(6.77397492383228,4.0909021925649,145.815122469156));
#53813=CARTESIAN_POINT('Ctrl Pts',(6.87324713713644,3.92184265866409,145.80721987829));
#53814=CARTESIAN_POINT('Ctrl Pts',(6.96618221402821,3.74916342147912,145.799317287423));
#53815=CARTESIAN_POINT('Ctrl Pts',(7.05903380358072,3.57663930903866,145.791421795774));
#53816=CARTESIAN_POINT('Ctrl Pts',(7.14555943509989,3.40050227277601,145.783526304125));
#53817=CARTESIAN_POINT('Ctrl Pts',(7.22547021314931,3.22125770451419,145.775630812475));
#53818=CARTESIAN_POINT('Ctrl Pts',(7.30532403317756,3.04214089643896,145.767740948497));
#53819=CARTESIAN_POINT('Ctrl Pts',(7.3785722535376,2.85992128298122,145.759851084519));
#53820=CARTESIAN_POINT('Ctrl Pts',(7.44497197941793,2.67512863722137,145.75196122054));
#53821=CARTESIAN_POINT('Ctrl Pts',(7.51133669660912,2.49043342180787,145.744075516425));
#53822=CARTESIAN_POINT('Ctrl Pts',(7.57085999802765,2.30316820106481,145.736189812311));
#53823=CARTESIAN_POINT('Ctrl Pts',(7.62334707857467,2.11388275918677,145.728304108196));
#53824=CARTESIAN_POINT('Ctrl Pts',(7.67581622202991,1.92466200428138,145.720421098965));
#53825=CARTESIAN_POINT('Ctrl Pts',(7.72125384500339,1.73342273611908,145.712538089734));
#53826=CARTESIAN_POINT('Ctrl Pts',(7.75951489762185,1.54073020142549,145.704655080504));
#53827=CARTESIAN_POINT('Ctrl Pts',(7.79777653046566,1.3480347445673,145.696771951728));
#53828=CARTESIAN_POINT('Ctrl Pts',(7.82886130005154,1.1538863136922,145.688888822952));
#53829=CARTESIAN_POINT('Ctrl Pts',(7.85267509470553,0.958861229267025,145.681005694176));
#53830=CARTESIAN_POINT('Ctrl Pts',(7.87649036537527,0.763824056886142,145.673122076792));
#53831=CARTESIAN_POINT('Ctrl Pts',(7.89303372069079,0.567910465103365,145.665238459408));
#53832=CARTESIAN_POINT('Ctrl Pts',(7.90226284082103,0.37170283100762,145.657354842023));
#53833=CARTESIAN_POINT('Ctrl Pts',(7.91149408435247,0.175450054198505,145.649469410806));
#53834=CARTESIAN_POINT('Ctrl Pts',(7.91340772318329,-0.0210965551616383,
145.641583979589));
#53835=CARTESIAN_POINT('Ctrl Pts',(7.90801356134308,-0.217353430186908,
145.633698548371));
#53836=CARTESIAN_POINT('Ctrl Pts',(7.90261725169281,-0.413688449417042,
145.625809977388));
#53837=CARTESIAN_POINT('Ctrl Pts',(7.8899073528546,-0.609733159915272,145.617921406404));
#53838=CARTESIAN_POINT('Ctrl Pts',(7.86994565581487,-0.804907680743947,
145.61003283542));
#53839=CARTESIAN_POINT('Ctrl Pts',(7.84996271070972,-1.00028995349764,145.602135867511));
#53840=CARTESIAN_POINT('Ctrl Pts',(7.82271258430308,-1.19479984322531,145.594238899603));
#53841=CARTESIAN_POINT('Ctrl Pts',(7.78830863181515,-1.38786514315824,145.586341931694));
#53842=CARTESIAN_POINT('Ctrl Pts',(7.75388369305167,-1.58104821216395,145.578440146666));
#53843=CARTESIAN_POINT('Ctrl Pts',(7.71229630126433,-1.77278459843256,145.570538361638));
#53844=CARTESIAN_POINT('Ctrl Pts',(7.66371016324732,-1.96251561362953,145.56263657661));
#53845=CARTESIAN_POINT('Ctrl Pts',(7.61506117733343,-2.15249205264011,145.554724570342));
#53846=CARTESIAN_POINT('Ctrl Pts',(7.55939546008387,-2.34045760962865,145.546812564074));
#53847=CARTESIAN_POINT('Ctrl Pts',(7.49692584652523,-2.52587090954824,145.538900557806));
#53848=CARTESIAN_POINT('Ctrl Pts',(7.4707517460105,-2.60355710084037,145.535585511729));
#53849=CARTESIAN_POINT('Ctrl Pts',(7.44338378020625,-2.68079550062831,145.532270465653));
#53850=CARTESIAN_POINT('Ctrl Pts',(7.41484003564203,-2.75754750563615,145.528955419576));
#53851=CARTESIAN_POINT('Ctrl Pts',(7.34733185913206,-2.93907196854973,145.521115077705));
#53852=CARTESIAN_POINT('Ctrl Pts',(7.27305221069926,-3.11838892380742,145.513274735834));
#53853=CARTESIAN_POINT('Ctrl Pts',(7.19216390375891,-3.29495058862305,145.505434393962));
#53854=CARTESIAN_POINT('Ctrl Pts',(7.11136603235314,-3.47131485224254,145.497602817826));
#53855=CARTESIAN_POINT('Ctrl Pts',(7.02397435983904,-3.64492964307849,145.489771241691));
#53856=CARTESIAN_POINT('Ctrl Pts',(6.93020116613366,-3.81526313599988,145.481939665555));
#53857=CARTESIAN_POINT('Ctrl Pts',(6.83651458008369,-3.98543931120736,145.474115322557));
#53858=CARTESIAN_POINT('Ctrl Pts',(6.73645837867059,-4.15233991798948,145.466290979559));
#53859=CARTESIAN_POINT('Ctrl Pts',(6.63029261615817,-4.31545372169816,145.458466636561));
#53860=CARTESIAN_POINT('Ctrl Pts',(6.52420427454969,-4.47844857540045,145.45064799943));
#53861=CARTESIAN_POINT('Ctrl Pts',(6.41201543666426,-4.63766183289461,145.442829362299));
#53862=CARTESIAN_POINT('Ctrl Pts',(6.29403179840267,-4.7926072988193,145.435010725168));
#53863=CARTESIAN_POINT('Ctrl Pts',(6.1761112783406,-4.94746987292123,145.427196270806));
#53864=CARTESIAN_POINT('Ctrl Pts',(6.05240234581321,-5.09806892458549,145.419381816444));
#53865=CARTESIAN_POINT('Ctrl Pts',(5.92325378516453,-5.2439475203833,145.411567362082));
#53866=CARTESIAN_POINT('Ctrl Pts',(5.79414923184489,-5.38977640809814,145.403755570493));
#53867=CARTESIAN_POINT('Ctrl Pts',(5.6596089763201,-5.53088778187332,145.395943778904));
#53868=CARTESIAN_POINT('Ctrl Pts',(5.52002194177641,-5.66685792677979,145.388131987314));
#53869=CARTESIAN_POINT('Ctrl Pts',(5.38042837433479,-5.80283443530795,145.380319830121));
#53870=CARTESIAN_POINT('Ctrl Pts',(5.23578780148227,-5.93366898234449,145.372507672927));
#53871=CARTESIAN_POINT('Ctrl Pts',(5.08652621748585,-6.0589745038933,145.364695515733));
#53872=CARTESIAN_POINT('Ctrl Pts',(4.93725243122015,-6.18429026928164,145.356882719889));
#53873=CARTESIAN_POINT('Ctrl Pts',(4.7833571502544,-6.3040758819019,145.349069924044));
#53874=CARTESIAN_POINT('Ctrl Pts',(4.62529960652721,-6.41798446164053,145.341257128199));
#53875=CARTESIAN_POINT('Ctrl Pts',(4.46720132987094,-6.53192239670121,145.333442318923));
#53876=CARTESIAN_POINT('Ctrl Pts',(4.30493893892572,-6.63998007596844,145.325627509647));
#53877=CARTESIAN_POINT('Ctrl Pts',(4.13900092100807,-6.74185377888711,145.31781270037));
#53878=CARTESIAN_POINT('Ctrl Pts',(3.9729909385748,-6.84377166271005,145.309994501943));
#53879=CARTESIAN_POINT('Ctrl Pts',(3.8033024531629,-6.93950004389283,145.302176303516));
#53880=CARTESIAN_POINT('Ctrl Pts',(3.63044895345303,-7.02878093244994,145.294358105089));
#53881=CARTESIAN_POINT('Ctrl Pts',(3.45739425320743,-7.11816574347688,145.286530806322));
#53882=CARTESIAN_POINT('Ctrl Pts',(3.28116749311361,-7.20108791123106,145.278703507554));
#53883=CARTESIAN_POINT('Ctrl Pts',(3.10230357176408,-7.27733698193369,145.270876208787));
#53884=CARTESIAN_POINT('Ctrl Pts',(2.92332288731849,-7.35363582834012,145.263043800326));
#53885=CARTESIAN_POINT('Ctrl Pts',(2.74170193806947,-7.42325277108259,145.255211391866));
#53886=CARTESIAN_POINT('Ctrl Pts',(2.55799128137919,-7.48602709081313,145.247378983406));
#53887=CARTESIAN_POINT('Ctrl Pts',(2.3740169740096,-7.54889150053811,145.239535334336));
#53888=CARTESIAN_POINT('Ctrl Pts',(2.18794730468875,-7.60489357274815,145.231691685266));
#53889=CARTESIAN_POINT('Ctrl Pts',(2.00034467952648,-7.653923318344,145.223848036197));
#53890=CARTESIAN_POINT('Ctrl Pts',(1.89912660538616,-7.68037655384915,145.219616117521));
#53891=CARTESIAN_POINT('Ctrl Pts',(1.79746242346425,-7.70480105338649,145.215384198845));
#53892=CARTESIAN_POINT('Ctrl Pts',(1.69544106047893,-7.72718581441149,145.211152280169));
#53893=CARTESIAN_POINT('Ctrl Pts',(1.50456310870687,-7.76906682060793,145.203234527011));
#53894=CARTESIAN_POINT('Ctrl Pts',(1.31186409198688,-7.8039298644076,145.195316773853));
#53895=CARTESIAN_POINT('Ctrl Pts',(1.11790229142303,-7.83161640192056,145.187399020695));
#53896=CARTESIAN_POINT('Ctrl Pts',(0.924163339010726,-7.85927112959421,
145.179490364466));
#53897=CARTESIAN_POINT('Ctrl Pts',(0.729164830202006,-7.87976572598927,
145.171581708237));
#53898=CARTESIAN_POINT('Ctrl Pts',(0.533478058350739,-7.89299196510793,
145.163673052008));
#53899=CARTESIAN_POINT('Ctrl Pts',(0.337979892166719,-7.90620545659101,
145.155772018253));
#53900=CARTESIAN_POINT('Ctrl Pts',(0.141795125631044,-7.91216452283891,
145.147870984498));
#53901=CARTESIAN_POINT('Ctrl Pts',(-0.054496661243007,-7.91081229166218,
145.139969950743));
#53902=CARTESIAN_POINT('Ctrl Pts',(-0.250635582957945,-7.90946111355566,
145.132075070036));
#53903=CARTESIAN_POINT('Ctrl Pts',(-0.446881016145848,-7.90080998421351,
145.124180189329));
#53904=CARTESIAN_POINT('Ctrl Pts',(-0.642649897258296,-7.88485396881603,
145.116285308623));
#53905=CARTESIAN_POINT('Ctrl Pts',(-0.838302538104702,-7.86890742750588,
145.108395115602));
#53906=CARTESIAN_POINT('Ctrl Pts',(-1.03347884837812,-7.84566467070511,
145.100504922581));
#53907=CARTESIAN_POINT('Ctrl Pts',(-1.22759711815532,-7.81517282697553,
145.09261472956));
#53908=CARTESIAN_POINT('Ctrl Pts',(-1.42163603338515,-7.78469344815439,
145.084727762009));
#53909=CARTESIAN_POINT('Ctrl Pts',(-1.61461743037493,-7.74697094173008,
145.076840794458));
#53910=CARTESIAN_POINT('Ctrl Pts',(-1.80596578028313,-7.7021041670732,145.068953826907));
#53911=CARTESIAN_POINT('Ctrl Pts',(-1.99729751289319,-7.65724128878947,
145.061067544286));
#53912=CARTESIAN_POINT('Ctrl Pts',(-2.18699614429357,-7.60523545070669,
145.053181261665));
#53913=CARTESIAN_POINT('Ctrl Pts',(-2.37449686967172,-7.54623652000911,
145.045294979043));
#53914=CARTESIAN_POINT('Ctrl Pts',(-2.56199726549072,-7.48723769301052,
145.037408710283));
#53915=CARTESIAN_POINT('Ctrl Pts',(-2.74729943412486,-7.42124590078946,
145.029522441523));
#53916=CARTESIAN_POINT('Ctrl Pts',(-2.92985415210936,-7.34846076721973,
145.021636172763));
#53917=CARTESIAN_POINT('Ctrl Pts',(-3.11243914634898,-7.27566356241296,
145.013748596084));
#53918=CARTESIAN_POINT('Ctrl Pts',(-3.29227546195785,-7.19607089894714,
145.005861019405));
#53919=CARTESIAN_POINT('Ctrl Pts',(-3.46883403197991,-7.10993048197927,
144.997973442727));
#53920=CARTESIAN_POINT('Ctrl Pts',(-3.6454514760663,-7.02376134119217,144.990083235908));
#53921=CARTESIAN_POINT('Ctrl Pts',(-3.81878868736588,-6.93104024755936,
144.98219302909));
#53922=CARTESIAN_POINT('Ctrl Pts',(-3.98834114846013,-6.83206088113241,
144.974302822272));
#53923=CARTESIAN_POINT('Ctrl Pts',(-4.15805733980565,-6.73298593416105,
144.966404996186));
#53924=CARTESIAN_POINT('Ctrl Pts',(-4.32398118316231,-6.62764081706805,
144.9585071701));
#53925=CARTESIAN_POINT('Ctrl Pts',(-4.48563622476486,-6.51636314665453,
144.950609344015));
#53926=CARTESIAN_POINT('Ctrl Pts',(-4.64738077781904,-6.40502385969187,
144.942707144753));
#53927=CARTESIAN_POINT('Ctrl Pts',(-4.80485154056625,-6.28774567512402,
144.934804945492));
#53928=CARTESIAN_POINT('Ctrl Pts',(-4.95760490001591,-6.16490670289002,
144.926902746231));
#53929=CARTESIAN_POINT('Ctrl Pts',(-5.1105426443513,-6.04191945470359,144.918991008416));
#53930=CARTESIAN_POINT('Ctrl Pts',(-5.25875135179053,-5.91335823652702,
144.911079270601));
#53931=CARTESIAN_POINT('Ctrl Pts',(-5.40182325383769,-5.77963896227943,
144.903167532786));
#53932=CARTESIAN_POINT('Ctrl Pts',(-5.46100688095171,-5.72432417613491,
144.899894735444));
#53933=CARTESIAN_POINT('Ctrl Pts',(-5.51931197328507,-5.66812716490685,
144.896621938103));
#53934=CARTESIAN_POINT('Ctrl Pts',(-5.57671167798816,-5.61107902818971,
144.893349140761));
#53935=CARTESIAN_POINT('Ctrl Pts',(-5.72254114542075,-5.46614275302046,
144.885034284513));
#53936=CARTESIAN_POINT('Ctrl Pts',(-5.86284221960547,-5.31539421925882,
144.876719428264));
#53937=CARTESIAN_POINT('Ctrl Pts',(-5.99715259149553,-5.15927144026348,
144.868404572015));
#53938=CARTESIAN_POINT('Ctrl Pts',(-6.13129756483191,-5.00334092104287,
144.860099955223));
#53939=CARTESIAN_POINT('Ctrl Pts',(-6.25946635928404,-4.8420495774869,144.851795338431));
#53940=CARTESIAN_POINT('Ctrl Pts',(-6.38123353964414,-4.67587205904104,
144.843490721638));
#53941=CARTESIAN_POINT('Ctrl Pts',(-6.50285879985164,-4.5098882211806,144.835195783911));
#53942=CARTESIAN_POINT('Ctrl Pts',(-6.61809715472091,-4.33902980270076,
144.826900846184));
#53943=CARTESIAN_POINT('Ctrl Pts',(-6.72656296210199,-4.16380495663254,
144.818605908457));
#53944=CARTESIAN_POINT('Ctrl Pts',(-6.83486619940837,-3.98884274002332,
144.810323403299));
#53945=CARTESIAN_POINT('Ctrl Pts',(-6.93641699278435,-3.80952740488747,
144.802040898141));
#53946=CARTESIAN_POINT('Ctrl Pts',(-7.03087254620634,-3.62639659152194,
144.793758392983));
#53947=CARTESIAN_POINT('Ctrl Pts',(-7.12524132875031,-3.44343400988967,
144.785483496486));
#53948=CARTESIAN_POINT('Ctrl Pts',(-7.21252773529438,-3.25666319938354,
144.777208599989));
#53949=CARTESIAN_POINT('Ctrl Pts',(-7.29243360353874,-3.06664851881969,
144.768933703491));
#53950=CARTESIAN_POINT('Ctrl Pts',(-7.37224806995356,-2.87685119012029,
144.76066827239));
#53951=CARTESIAN_POINT('Ctrl Pts',(-7.44469873091024,-2.68381766523571,
144.752402841288));
#53952=CARTESIAN_POINT('Ctrl Pts',(-7.50953436370736,-2.48813477132939,
144.744137410187));
#53953=CARTESIAN_POINT('Ctrl Pts',(-7.53487068490354,-2.41166625488684,
144.74090746381));
#53954=CARTESIAN_POINT('Ctrl Pts',(-7.55904464307123,-2.33479340311073,
144.737677517434));
#53955=CARTESIAN_POINT('Ctrl Pts',(-7.58204322356163,-2.25755211590856,
144.734447571058));
#53956=CARTESIAN_POINT('Ctrl Pts',(-7.6367944674298,-2.07366874301679,144.726758245109));
#53957=CARTESIAN_POINT('Ctrl Pts',(-7.68484746179367,-1.88780794319174,
144.719068919161));
#53958=CARTESIAN_POINT('Ctrl Pts',(-7.72607096885417,-1.70051415290459,
144.711379593213));
#53959=CARTESIAN_POINT('Ctrl Pts',(-7.76730118200993,-1.51318989432178,
144.703689016393));
#53960=CARTESIAN_POINT('Ctrl Pts',(-7.80169962506568,-1.32443253807318,
144.695998439572));
#53961=CARTESIAN_POINT('Ctrl Pts',(-7.82918637756967,-1.13479586943093,
144.688307862751));
#53962=CARTESIAN_POINT('Ctrl Pts',(-7.85669790838933,-0.944988250173958,
144.680610353153));
#53963=CARTESIAN_POINT('Ctrl Pts',(-7.87728525577776,-0.754300096158211,
144.672912843555));
#53964=CARTESIAN_POINT('Ctrl Pts',(-7.89092041321999,-0.563290362271563,
144.665215333957));
#53965=CARTESIAN_POINT('Ctrl Pts',(-7.90432776465935,-0.375471876023305,
144.657646428587));
#53966=CARTESIAN_POINT('Ctrl Pts',(-7.91101345033552,-0.187342803459868,
144.650077523217));
#53967=CARTESIAN_POINT('Ctrl Pts',(-7.91099997967269,0.000567114363191055,
144.642508617847));
#53968=CARTESIAN_POINT('',(-7.91099998020127,-0.000555341303987942,142.642353853155));
#53969=CARTESIAN_POINT('Ctrl Pts',(-7.91099997917165,0.000559131365739208,
144.642309010808));
#53970=CARTESIAN_POINT('Ctrl Pts',(-7.91083596349065,2.2020457259927,144.553729074218));
#53971=CARTESIAN_POINT('Ctrl Pts',(-6.94200761631339,4.38622928711889,144.465149137628));
#53972=CARTESIAN_POINT('Ctrl Pts',(-3.67820201487554,7.34180684108,144.287981765306));
#53973=CARTESIAN_POINT('Ctrl Pts',(-1.40868175870934,8.08992666571478,144.199394329573));
#53974=CARTESIAN_POINT('Ctrl Pts',(2.97309270522046,7.65454228024958,144.022219458108));
#53975=CARTESIAN_POINT('Ctrl Pts',(5.05102072676259,6.47444880833715,143.933632022375));
#53976=CARTESIAN_POINT('Ctrl Pts',(7.66951518848171,2.93425195366926,143.756457150909));
#53977=CARTESIAN_POINT('Ctrl Pts',(8.18956872247134,0.60188196009079,143.667869715177));
#53978=CARTESIAN_POINT('Ctrl Pts',(7.32306689760961,-3.71537198233204,143.490694843711));
#53979=CARTESIAN_POINT('Ctrl Pts',(5.94329958849617,-5.66643518937126,143.402107407979));
#53980=CARTESIAN_POINT('Ctrl Pts',(2.16154501637024,-7.92205913233223,143.224932536513));
#53981=CARTESIAN_POINT('Ctrl Pts',(-0.21081652930894,-8.20894963712981,
143.13634510078));
#53982=CARTESIAN_POINT('Ctrl Pts',(-4.42123908577165,-6.91982244717367,
142.959170229315));
#53983=CARTESIAN_POINT('Ctrl Pts',(-6.22631625634753,-5.35390358802864,
142.870582793582));
#53984=CARTESIAN_POINT('Ctrl Pts',(-7.653094167907,-2.31351615424296,142.735448189618));
#53985=CARTESIAN_POINT('Ctrl Pts',(-7.91091749410943,-1.15739837654274,
142.688901021386));
#53986=CARTESIAN_POINT('Ctrl Pts',(-7.91099998020127,-0.000555341303987942,
142.642353853155));
#53987=CARTESIAN_POINT('',(-7.91156134791759,-0.0007562664353129,140.64330292144));
#53988=CARTESIAN_POINT('Ctrl Pts',(-7.91099998025987,-0.000558863451393805,
142.642266634146));
#53989=CARTESIAN_POINT('Ctrl Pts',(-7.91101396606582,0.197417422812076,
142.634266600749));
#53990=CARTESIAN_POINT('Ctrl Pts',(-7.90359199240421,0.39563115781575,142.626266567353));
#53991=CARTESIAN_POINT('Ctrl Pts',(-7.88870658119376,0.593489238175604,
142.618266533957));
#53992=CARTESIAN_POINT('Ctrl Pts',(-7.87383727106835,0.791133301621042,
142.610275153947));
#53993=CARTESIAN_POINT('Ctrl Pts',(-7.85152063367933,0.988422146600453,
142.602283773937));
#53994=CARTESIAN_POINT('Ctrl Pts',(-7.82178119339689,1.18476156361639,142.594292393928));
#53995=CARTESIAN_POINT('Ctrl Pts',(-7.79207685683757,1.38086922628637,142.586310446751));
#53996=CARTESIAN_POINT('Ctrl Pts',(-7.75496723908072,1.57602936757451,142.578328499575));
#53997=CARTESIAN_POINT('Ctrl Pts',(-7.71052873213815,1.76965185018752,142.570346552399));
#53998=CARTESIAN_POINT('Ctrl Pts',(-7.66612070386264,1.9631415345679,142.562370079734));
#53999=CARTESIAN_POINT('Ctrl Pts',(-7.61439387511261,2.15509533749356,142.55439360707));
#54000=CARTESIAN_POINT('Ctrl Pts',(-7.5554760441043,2.34493128832511,142.546417134405));
#54001=CARTESIAN_POINT('Ctrl Pts',(-7.49659622615169,2.53464475934965,142.538445808062));
#54002=CARTESIAN_POINT('Ctrl Pts',(-7.43053475480413,2.72224278470734,142.530474481718));
#54003=CARTESIAN_POINT('Ctrl Pts',(-7.35746985812211,2.90715639187586,142.522503155375));
#54004=CARTESIAN_POINT('Ctrl Pts',(-7.3187358346882,3.00518497083198,142.518277301985));
#54005=CARTESIAN_POINT('Ctrl Pts',(-7.2780344182534,3.10245935149916,142.514051448594));
#54006=CARTESIAN_POINT('Ctrl Pts',(-7.2353978186162,3.19889659200856,142.509825595203));
#54007=CARTESIAN_POINT('Ctrl Pts',(-7.1519925489431,3.38754611189657,142.501559025058));
#54008=CARTESIAN_POINT('Ctrl Pts',(-7.06125235358972,3.57282549477544,142.493292454913));
#54009=CARTESIAN_POINT('Ctrl Pts',(-6.96348352833377,3.75417343107965,142.485025884768));
#54010=CARTESIAN_POINT('Ctrl Pts',(-6.86562710107853,3.93568385723422,142.476751907681));
#54011=CARTESIAN_POINT('Ctrl Pts',(-6.76072961063135,4.11325554586154,142.468477930593));
#54012=CARTESIAN_POINT('Ctrl Pts',(-6.64914181382372,4.2863544113455,142.460203953506));
#54013=CARTESIAN_POINT('Ctrl Pts',(-6.5374467900207,4.45961961106836,142.451922025785));
#54014=CARTESIAN_POINT('Ctrl Pts',(-6.41904878404736,4.62840316036439,142.443640098063));
#54015=CARTESIAN_POINT('Ctrl Pts',(-6.29434059322681,4.79220173787135,142.435358170342));
#54016=CARTESIAN_POINT('Ctrl Pts',(-6.16942568390501,4.95627183079542,142.427062514351));
#54017=CARTESIAN_POINT('Ctrl Pts',(-6.038179856008,5.11534019772091,142.41876685836));
#54018=CARTESIAN_POINT('Ctrl Pts',(-5.90103607306085,5.26893672997073,142.410471202369));
#54019=CARTESIAN_POINT('Ctrl Pts',(-5.76376833867507,5.42267208376047,142.402168048711));
#54020=CARTESIAN_POINT('Ctrl Pts',(-5.62059220905539,5.57092551696632,142.393864895052));
#54021=CARTESIAN_POINT('Ctrl Pts',(-5.471976837168,5.71326443406018,142.385561741394));
#54022=CARTESIAN_POINT('Ctrl Pts',(-5.32313488081947,5.85582036630137,142.377245928442));
#54023=CARTESIAN_POINT('Ctrl Pts',(-5.16883732252925,5.99244355951086,142.36893011549));
#54024=CARTESIAN_POINT('Ctrl Pts',(-5.0095870836539,6.12274107335007,142.360614302538));
#54025=CARTESIAN_POINT('Ctrl Pts',(-4.94772987490577,6.17335224084241,142.357384210192));
#54026=CARTESIAN_POINT('Ctrl Pts',(-4.88512574290236,6.22300947232399,142.354154117846));
#54027=CARTESIAN_POINT('Ctrl Pts',(-4.82180532302,6.27169151241481,142.3509240255));
#54028=CARTESIAN_POINT('Ctrl Pts',(-4.66672440730128,6.39092090745619,142.343013059657));
#54029=CARTESIAN_POINT('Ctrl Pts',(-4.50702284465997,6.50454530354762,142.335102093814));
#54030=CARTESIAN_POINT('Ctrl Pts',(-4.34314304490546,6.61218795040563,142.32719112797));
#54031=CARTESIAN_POINT('Ctrl Pts',(-4.17942907636278,6.71972167285319,142.319288167294));
#54032=CARTESIAN_POINT('Ctrl Pts',(-4.01154557821584,6.82128551566821,142.311385206617));
#54033=CARTESIAN_POINT('Ctrl Pts',(-3.83996763692179,6.9165431790305,142.30348224594));
#54034=CARTESIAN_POINT('Ctrl Pts',(-3.66853156416113,7.01172207897545,142.295585819794));
#54035=CARTESIAN_POINT('Ctrl Pts',(-3.49340743333372,7.10060502088164,142.287689393649));
#54036=CARTESIAN_POINT('Ctrl Pts',(-3.3150991308719,7.182899049304,142.279792967503));
#54037=CARTESIAN_POINT('Ctrl Pts',(-3.13690527287704,7.26514025855819,142.271901609559));
#54038=CARTESIAN_POINT('Ctrl Pts',(-2.95553162687625,7.34080083646944,142.264010251614));
#54039=CARTESIAN_POINT('Ctrl Pts',(-2.77150674539036,7.40963368596962,142.256118893669));
#54040=CARTESIAN_POINT('Ctrl Pts',(-2.58756593752473,7.47843508848935,142.248231140971));
#54041=CARTESIAN_POINT('Ctrl Pts',(-2.40097662985685,7.5404148581255,142.240343388273));
#54042=CARTESIAN_POINT('Ctrl Pts',(-2.21228768731736,7.59537386759493,142.232455635574));
#54043=CARTESIAN_POINT('Ctrl Pts',(-2.02365005161559,7.65031793303563,142.224570027653));
#54044=CARTESIAN_POINT('Ctrl Pts',(-1.83291424938462,7.6982449471224,142.216684419731));
#54045=CARTESIAN_POINT('Ctrl Pts',(-1.64064492386193,7.73900544216155,142.208798811809));
#54046=CARTESIAN_POINT('Ctrl Pts',(-1.44835292184097,7.77977074454733,142.200912273849));
#54047=CARTESIAN_POINT('Ctrl Pts',(-1.25452737076121,7.81336776091123,142.193025735888));
#54048=CARTESIAN_POINT('Ctrl Pts',(-1.05974437350371,7.83969788083873,142.185139197927));
#54049=CARTESIAN_POINT('Ctrl Pts',(-0.864936837270453,7.86603131786363,
142.177251666412));
#54050=CARTESIAN_POINT('Ctrl Pts',(-0.669171956001874,7.88509598734318,
142.169364134897));
#54051=CARTESIAN_POINT('Ctrl Pts',(-0.473032219651286,7.89684503578307,
142.161476603381));
#54052=CARTESIAN_POINT('Ctrl Pts',(-0.276834898113549,7.90859753365736,
142.153586756144));
#54053=CARTESIAN_POINT('Ctrl Pts',(-0.0802628461053111,7.91303010974445,
142.145696908908));
#54054=CARTESIAN_POINT('Ctrl Pts',(0.11609991967804,7.91014802697464,142.137807061671));
#54055=CARTESIAN_POINT('Ctrl Pts',(0.312553249532429,7.9072646149653,142.129913575574));
#54056=CARTESIAN_POINT('Ctrl Pts',(0.508796756665151,7.89705982647217,142.122020089477));
#54057=CARTESIAN_POINT('Ctrl Pts',(0.704249769468778,7.87959093241541,142.11412660338));
#54058=CARTESIAN_POINT('Ctrl Pts',(0.899928725686014,7.86210184434119,142.106223992423));
#54059=CARTESIAN_POINT('Ctrl Pts',(1.09481501909843,7.83733190836066,142.098321381467));
#54060=CARTESIAN_POINT('Ctrl Pts',(1.28833525885604,7.80539001336822,142.090418770511));
#54061=CARTESIAN_POINT('Ctrl Pts',(1.48198385178215,7.77342693277042,142.082510918113));
#54062=CARTESIAN_POINT('Ctrl Pts',(1.67426424830275,7.73428247856622,142.074603065714));
#54063=CARTESIAN_POINT('Ctrl Pts',(1.86461625191157,7.68811597422329,142.066695213316));
#54064=CARTESIAN_POINT('Ctrl Pts',(2.05522871105117,7.64188630100814,142.058776540732));
#54065=CARTESIAN_POINT('Ctrl Pts',(2.24390717669586,7.58861547974743,142.050857868149));
#54066=CARTESIAN_POINT('Ctrl Pts',(2.4301084074716,7.52851207928471,142.042939195566));
#54067=CARTESIAN_POINT('Ctrl Pts',(2.50706496337553,7.50367147711224,142.039666425741));
#54068=CARTESIAN_POINT('Ctrl Pts',(2.58359862466643,7.47766432900829,142.036393655917));
#54069=CARTESIAN_POINT('Ctrl Pts',(2.65967219190864,7.45050768951941,142.033120886092));
#54070=CARTESIAN_POINT('Ctrl Pts',(2.84198110194762,7.3854273005615,142.025277753173));
#54071=CARTESIAN_POINT('Ctrl Pts',(3.02218579136077,7.31354933772559,142.017434620255));
#54072=CARTESIAN_POINT('Ctrl Pts',(3.19973595932908,7.23502666135906,142.009591487336));
#54073=CARTESIAN_POINT('Ctrl Pts',(3.37707761352304,7.15659620151819,142.001757565342));
#54074=CARTESIAN_POINT('Ctrl Pts',(3.55177063578898,7.07153670688227,141.993923643347));
#54075=CARTESIAN_POINT('Ctrl Pts',(3.72327973891718,6.98005078676143,141.986089721353));
#54076=CARTESIAN_POINT('Ctrl Pts',(3.89462077842683,6.88865451467968,141.978263475904));
#54077=CARTESIAN_POINT('Ctrl Pts',(4.06278380421339,6.79084452189787,141.970437230454));
#54078=CARTESIAN_POINT('Ctrl Pts',(4.22725320722755,6.68687156463951,141.962610985005));
#54079=CARTESIAN_POINT('Ctrl Pts',(4.39159341254989,6.58298028254895,141.954790887403));
#54080=CARTESIAN_POINT('Ctrl Pts',(4.55224547833337,6.47293586517373,141.946970789801));
#54081=CARTESIAN_POINT('Ctrl Pts',(4.70871796283319,6.35703516951826,141.9391506922));
#54082=CARTESIAN_POINT('Ctrl Pts',(4.86509793259174,6.24120300043414,141.93133521825));
#54083=CARTESIAN_POINT('Ctrl Pts',(5.01730296197389,6.11952165904375,141.9235197443));
#54084=CARTESIAN_POINT('Ctrl Pts',(5.1648700477419,5.99233163217279,141.91570427035));
#54085=CARTESIAN_POINT('Ctrl Pts',(5.31237854709233,5.86519210171156,141.907891899265));
#54086=CARTESIAN_POINT('Ctrl Pts',(5.45525250555584,5.73254847238278,141.900079528179));
#54087=CARTESIAN_POINT('Ctrl Pts',(5.59306137127033,5.5947819883534,141.892267157093));
#54088=CARTESIAN_POINT('Ctrl Pts',(5.73086502042888,5.45702071927568,141.884455081734));
#54089=CARTESIAN_POINT('Ctrl Pts',(5.86360370383074,5.3141372239608,141.876643006374));
#54090=CARTESIAN_POINT('Ctrl Pts',(5.99088284554568,5.16655046727955,141.868830931014));
#54091=CARTESIAN_POINT('Ctrl Pts',(6.11816570977847,5.01895939414605,141.861018627176));
#54092=CARTESIAN_POINT('Ctrl Pts',(6.23998848388287,4.86666505156086,141.853206323338));
#54093=CARTESIAN_POINT('Ctrl Pts',(6.35599613246674,4.71012039804376,141.845394019499));
#54094=CARTESIAN_POINT('Ctrl Pts',(6.47202758583008,4.55354362155027,141.837580112575));
#54095=CARTESIAN_POINT('Ctrl Pts',(6.58224132716533,4.39271507933296,141.829766205651));
#54096=CARTESIAN_POINT('Ctrl Pts',(6.68632491450132,4.22811780083277,141.821952298727));
#54097=CARTESIAN_POINT('Ctrl Pts',(6.79044817493164,4.06345778349426,141.81413541341));
#54098=CARTESIAN_POINT('Ctrl Pts',(6.88843643913402,3.89502646545144,141.806318528093));
#54099=CARTESIAN_POINT('Ctrl Pts',(6.98002251231746,3.7233327446713,141.798501642776));
#54100=CARTESIAN_POINT('Ctrl Pts',(7.0717079370148,3.55145277252679,141.790676277792));
#54101=CARTESIAN_POINT('Ctrl Pts',(7.15697713402299,3.37630363968181,141.782850912808));
#54102=CARTESIAN_POINT('Ctrl Pts',(7.23561004969321,3.19841651583696,141.775025547823));
#54103=CARTESIAN_POINT('Ctrl Pts',(7.31429075496577,3.02042128007946,141.767195426929));
#54104=CARTESIAN_POINT('Ctrl Pts',(7.38632701118634,2.8396850627496,141.759365306035));
#54105=CARTESIAN_POINT('Ctrl Pts',(7.45154818893114,2.6567556507961,141.751535185141));
#54106=CARTESIAN_POINT('Ctrl Pts',(7.51685851970399,2.47357618645844,141.74369436099));
#54107=CARTESIAN_POINT('Ctrl Pts',(7.57533506014372,2.288197873882,141.735853536839));
#54108=CARTESIAN_POINT('Ctrl Pts',(7.62685768736909,2.10118129075504,141.728012712689));
#54109=CARTESIAN_POINT('Ctrl Pts',(7.65466420313479,2.00024933430764,141.723781057354));
#54110=CARTESIAN_POINT('Ctrl Pts',(7.6804461335336,1.89884034749855,141.719549402019));
#54111=CARTESIAN_POINT('Ctrl Pts',(7.70419086017597,1.79704317977644,141.715317746684));
#54112=CARTESIAN_POINT('Ctrl Pts',(7.74858215794803,1.60673109689738,141.707406572348));
#54113=CARTESIAN_POINT('Ctrl Pts',(7.78597718486723,1.41451736889222,141.699495398012));
#54114=CARTESIAN_POINT('Ctrl Pts',(7.8162126789919,1.22095878585896,141.691584223675));
#54115=CARTESIAN_POINT('Ctrl Pts',(7.84641539391533,1.02761004546037,141.683681626079));
#54116=CARTESIAN_POINT('Ctrl Pts',(7.86947398378279,0.832919691770439,141.675779028483));
#54117=CARTESIAN_POINT('Ctrl Pts',(7.88527541788998,0.637457907645663,141.667876430887));
#54118=CARTESIAN_POINT('Ctrl Pts',(7.90106265437923,0.442171746297559,141.659980933789));
#54119=CARTESIAN_POINT('Ctrl Pts',(7.9096056970441,0.246115876839994,141.652085436692));
#54120=CARTESIAN_POINT('Ctrl Pts',(7.91084281652067,0.0498691518213697,
141.644189939594));
#54121=CARTESIAN_POINT('Ctrl Pts',(7.91207905401571,-0.146237662711553,
141.636300071446));
#54122=CARTESIAN_POINT('Ctrl Pts',(7.90601974352117,-0.342534718297289,
141.628410203298));
#54123=CARTESIAN_POINT('Ctrl Pts',(7.89265507442595,-0.538439296614054,
141.620520335149));
#54124=CARTESIAN_POINT('Ctrl Pts',(7.87929745389464,-0.734240554307788,
141.612634628139));
#54125=CARTESIAN_POINT('Ctrl Pts',(7.85864217554049,-0.92964940398611,141.60474892113));
#54126=CARTESIAN_POINT('Ctrl Pts',(7.83073150669614,-1.12408410274164,141.59686321412));
#54127=CARTESIAN_POINT('Ctrl Pts',(7.80283038062938,-1.31845232343824,141.588980203267));
#54128=CARTESIAN_POINT('Ctrl Pts',(7.76767885704064,-1.51184671610671,141.581097192414));
#54129=CARTESIAN_POINT('Ctrl Pts',(7.72537098081794,-1.70369134784916,141.573214181561));
#54130=CARTESIAN_POINT('Ctrl Pts',(7.683062473214,-1.89553884258334,141.565331053067));
#54131=CARTESIAN_POINT('Ctrl Pts',(7.63359746557776,-2.08583619164996,141.557447924572));
#54132=CARTESIAN_POINT('Ctrl Pts',(7.57712110211298,-2.27401776684226,141.549564796077));
#54133=CARTESIAN_POINT('Ctrl Pts',(7.52064124665819,-2.46221097748943,141.541681180161));
#54134=CARTESIAN_POINT('Ctrl Pts',(7.45714927014244,-2.64828782294039,141.533797564244));
#54135=CARTESIAN_POINT('Ctrl Pts',(7.38684018405892,-2.83169791735848,141.525913948328));
#54136=CARTESIAN_POINT('Ctrl Pts',(7.316514932111,-3.01515018246717,141.518028519765));
#54137=CARTESIAN_POINT('Ctrl Pts',(7.23936957072014,-3.19593415264087,141.510143091203));
#54138=CARTESIAN_POINT('Ctrl Pts',(7.15564732919218,-3.3735192752117,141.502257662641));
#54139=CARTESIAN_POINT('Ctrl Pts',(7.07189176432692,-3.55117508065998,141.494369095501));
#54140=CARTESIAN_POINT('Ctrl Pts',(6.98155425019417,-3.72562918976471,141.48648052836));
#54141=CARTESIAN_POINT('Ctrl Pts',(6.88492415136977,-3.89637529376794,141.47859196122));
#54142=CARTESIAN_POINT('Ctrl Pts',(6.7881912171149,-4.0673031087424,141.470694998929));
#54143=CARTESIAN_POINT('Ctrl Pts',(6.68515249212069,-4.2345147363401,141.462798036639));
#54144=CARTESIAN_POINT('Ctrl Pts',(6.57614148809467,-4.39753159494733,141.454901074348));
#54145=CARTESIAN_POINT('Ctrl Pts',(6.46706400185862,-4.56064787215115,141.446999295961));
#54146=CARTESIAN_POINT('Ctrl Pts',(6.35200717688742,-4.71956400151608,141.439097517574));
#54147=CARTESIAN_POINT('Ctrl Pts',(6.23134521550626,-4.87383399442239,141.431195739187));
#54148=CARTESIAN_POINT('Ctrl Pts',(6.11052719654456,-5.02830351169883,141.423283741072));
#54149=CARTESIAN_POINT('Ctrl Pts',(5.98408978299929,-5.1781146272737,141.415371742957));
#54150=CARTESIAN_POINT('Ctrl Pts',(5.8524452240126,-5.32285693025203,141.407459744842));
#54151=CARTESIAN_POINT('Ctrl Pts',(5.79728750742877,-5.38350246689117,141.404144698987));
#54152=CARTESIAN_POINT('Ctrl Pts',(5.74121608317219,-5.44325863162316,141.400829653132));
#54153=CARTESIAN_POINT('Ctrl Pts',(5.68426301255612,-5.5020973277548,141.397514607277));
#54154=CARTESIAN_POINT('Ctrl Pts',(5.54834778401845,-5.64251249317228,141.38960344094));
#54155=CARTESIAN_POINT('Ctrl Pts',(5.4070439001594,-5.77807722674997,141.381692274603));
#54156=CARTESIAN_POINT('Ctrl Pts',(5.26073092161834,-5.90835266130321,141.373781108266));
#54157=CARTESIAN_POINT('Ctrl Pts',(5.11457654171377,-6.03848688140989,141.365878517384));
#54158=CARTESIAN_POINT('Ctrl Pts',(4.96342413749641,-6.16334299540037,141.357975926501));
#54159=CARTESIAN_POINT('Ctrl Pts',(4.80769173920856,-6.28251710230428,141.350073335618));
#54160=CARTESIAN_POINT('Ctrl Pts',(4.65209924163074,-6.40158415028945,141.342177843952));
#54161=CARTESIAN_POINT('Ctrl Pts',(4.49193521834265,-6.51497915131509,141.334282352286));
#54162=CARTESIAN_POINT('Ctrl Pts',(4.32765277895553,-6.62233662877375,141.32638686062));
#54163=CARTESIAN_POINT('Ctrl Pts',(4.16348743519291,-6.72961758502348,141.318496996625));
#54164=CARTESIAN_POINT('Ctrl Pts',(3.9952098113043,-6.83086940362176,141.31060713263));
#54165=CARTESIAN_POINT('Ctrl Pts',(3.82330439283543,-6.92576815376643,141.302717268635));
#54166=CARTESIAN_POINT('Ctrl Pts',(3.65148961002931,-7.02061686935612,141.294831564504));
#54167=CARTESIAN_POINT('Ctrl Pts',(3.47605114517209,-7.10911902477591,141.286945860372));
#54168=CARTESIAN_POINT('Ctrl Pts',(3.29750087674578,-7.19099499150575,141.279060156241));
#54169=CARTESIAN_POINT('Ctrl Pts',(3.11901162661846,-7.27284297769956,141.271177146993));
#54170=CARTESIAN_POINT('Ctrl Pts',(2.9374130054616,-7.34806914478693,141.263294137746));
#54171=CARTESIAN_POINT('Ctrl Pts',(2.75324005826381,-7.41644053313795,141.255411128498));
#54172=CARTESIAN_POINT('Ctrl Pts',(2.56906431809793,-7.48481295833564,141.247527999705));
#54173=CARTESIAN_POINT('Ctrl Pts',(2.38231449418747,-7.54633026916426,141.239644870913));
#54174=CARTESIAN_POINT('Ctrl Pts',(2.19354465274656,-7.60080803970255,141.23176174212));
#54175=CARTESIAN_POINT('Ctrl Pts',(2.0047631110577,-7.65528918685767,141.223878124718));
#54176=CARTESIAN_POINT('Ctrl Pts',(1.81396163369587,-7.70272982805217,141.215994507317));
#54177=CARTESIAN_POINT('Ctrl Pts',(1.62170849017035,-7.74299571050568,141.208110889916));
#54178=CARTESIAN_POINT('Ctrl Pts',(1.42941111376424,-7.78327085718207,141.200225458681));
#54179=CARTESIAN_POINT('Ctrl Pts',(1.23566174328376,-7.81636788504171,141.192340027447));
#54180=CARTESIAN_POINT('Ctrl Pts',(1.04103809916656,-7.8422038150053,141.184454596212));
#54181=CARTESIAN_POINT('Ctrl Pts',(0.84633696115265,-7.86805003214081,141.176566025212));
#54182=CARTESIAN_POINT('Ctrl Pts',(0.650761197511675,-7.88662934509372,
141.168677454211));
#54183=CARTESIAN_POINT('Ctrl Pts',(0.454893143980661,-7.89791068748941,
141.16078888321));
#54184=CARTESIAN_POINT('Ctrl Pts',(0.258816600300158,-7.90920403821784,
141.152891915284));
#54185=CARTESIAN_POINT('Ctrl Pts',(0.0624474897329449,-7.91318388217811,
141.144994947358));
#54186=CARTESIAN_POINT('Ctrl Pts',(-0.133631241430665,-7.90987128158946,
141.137097979432));
#54187=CARTESIAN_POINT('Ctrl Pts',(-0.329829579847529,-7.90655666032751,
141.129196194387));
#54188=CARTESIAN_POINT('Ctrl Pts',(-0.525736842255237,-7.8959407446982,
141.121294409342));
#54189=CARTESIAN_POINT('Ctrl Pts',(-0.720775434481017,-7.87809645619097,
141.113392624297));
#54190=CARTESIAN_POINT('Ctrl Pts',(-0.916066316057366,-7.86022908546238,
141.105480618012));
#54191=CARTESIAN_POINT('Ctrl Pts',(-1.11048594208799,-7.8351147098806,141.097568611727));
#54192=CARTESIAN_POINT('Ctrl Pts',(-1.30346601147186,-7.80287750492968,
141.089656605442));
#54193=CARTESIAN_POINT('Ctrl Pts',(-1.38432259279204,-7.78937046147192,
141.086341559584));
#54194=CARTESIAN_POINT('Ctrl Pts',(-1.46492662522691,-7.77461359795081,
141.083026513727));
#54195=CARTESIAN_POINT('Ctrl Pts',(-1.5452371234515,-7.75861864202046,141.079711467869));
#54196=CARTESIAN_POINT('Ctrl Pts',(-1.73517771216056,-7.72078932439762,
141.071871126));
#54197=CARTESIAN_POINT('Ctrl Pts',(-1.92401397181497,-7.67592392978999,
141.064030784131));
#54198=CARTESIAN_POINT('Ctrl Pts',(-2.11117921729541,-7.6240962292235,141.056190442262));
#54199=CARTESIAN_POINT('Ctrl Pts',(-2.29813520646132,-7.57232647356865,
141.048358866128));
#54200=CARTESIAN_POINT('Ctrl Pts',(-2.48342356625144,-7.5136100046007,141.040527289995));
#54201=CARTESIAN_POINT('Ctrl Pts',(-2.66648551247275,-7.44807196607101,
141.032695713861));
#54202=CARTESIAN_POINT('Ctrl Pts',(-2.84937838515238,-7.38259445758877,
141.024871370865));
#54203=CARTESIAN_POINT('Ctrl Pts',(-3.03004861066099,-7.31030804406366,
141.01704702787));
#54204=CARTESIAN_POINT('Ctrl Pts',(-3.20795014846785,-7.23138830688445,
141.009222684874));
#54205=CARTESIAN_POINT('Ctrl Pts',(-3.38572195238176,-7.15252612156713,
141.001404047745));
#54206=CARTESIAN_POINT('Ctrl Pts',(-3.56072877009257,-7.06704038916747,
140.993585410616));
#54207=CARTESIAN_POINT('Ctrl Pts',(-3.73244203572983,-6.97515572943837,
140.985766773487));
#54208=CARTESIAN_POINT('Ctrl Pts',(-3.90406343920261,-6.8833202256303,140.977952319127));
#54209=CARTESIAN_POINT('Ctrl Pts',(-4.07239449130314,-6.7850927792193,140.970137864768));
#54210=CARTESIAN_POINT('Ctrl Pts',(-4.2369286752944,-6.68074519799012,140.962323410408));
#54211=CARTESIAN_POINT('Ctrl Pts',(-4.40140679431659,-6.57643317316492,
140.954511618821));
#54212=CARTESIAN_POINT('Ctrl Pts',(-4.56209032647814,-6.4660053567526,140.946699827233));
#54213=CARTESIAN_POINT('Ctrl Pts',(-4.71849917888739,-6.34977846061097,
140.938888035646));
#54214=CARTESIAN_POINT('Ctrl Pts',(-4.87491535148405,-6.23354612486251,
140.931075878455));
#54215=CARTESIAN_POINT('Ctrl Pts',(-5.02705615694601,-6.11151436953882,
140.923263721263));
#54216=CARTESIAN_POINT('Ctrl Pts',(-5.17447180221511,-5.9840423267287,140.915451564072));
#54217=CARTESIAN_POINT('Ctrl Pts',(-5.32189949884725,-5.85655986296319,
140.907638768229));
#54218=CARTESIAN_POINT('Ctrl Pts',(-5.46460099908586,-5.72363645529987,
140.899825972386));
#54219=CARTESIAN_POINT('Ctrl Pts',(-5.60216090650573,-5.58567043224168,
140.892013176544));
#54220=CARTESIAN_POINT('Ctrl Pts',(-5.73975626441959,-5.44766885402963,
140.88419836727));
#54221=CARTESIAN_POINT('Ctrl Pts',(-5.87220714147425,-5.3046223206498,140.876383557995));
#54222=CARTESIAN_POINT('Ctrl Pts',(-5.99913610811226,-5.15696489772266,
140.868568748721));
#54223=CARTESIAN_POINT('Ctrl Pts',(-6.12612012169816,-5.00924343826642,
140.860750550296));
#54224=CARTESIAN_POINT('Ctrl Pts',(-6.24757722533467,-4.85690737227738,
140.852932351871));
#54225=CARTESIAN_POINT('Ctrl Pts',(-6.36317117017967,-4.70042271067127,
140.845114153446));
#54226=CARTESIAN_POINT('Ctrl Pts',(-6.47889966575044,-4.54375590176654,
140.837286854681));
#54227=CARTESIAN_POINT('Ctrl Pts',(-6.58875116277602,-4.38293113545497,
140.829459555915));
#54228=CARTESIAN_POINT('Ctrl Pts',(-6.69243294611102,-4.21844310875563,
140.82163225715));
#54229=CARTESIAN_POINT('Ctrl Pts',(-6.79618241333639,-4.05384770360262,
140.813799848692));
#54230=CARTESIAN_POINT('Ctrl Pts',(-6.89375396476075,-3.88558457557204,
140.805967440234));
#54231=CARTESIAN_POINT('Ctrl Pts',(-6.98490150243916,-3.71417177863695,
140.798135031776));
#54232=CARTESIAN_POINT('Ctrl Pts',(-7.07617984967847,-3.54251298018309,
140.790291382708));
#54233=CARTESIAN_POINT('Ctrl Pts',(-7.16101561659004,-3.36769579977956,
140.78244773364));
#54234=CARTESIAN_POINT('Ctrl Pts',(-7.23921091056943,-3.19025804478142,
140.774604084572));
#54235=CARTESIAN_POINT('Ctrl Pts',(-7.28139996368055,-3.09452426735603,
140.770372165868));
#54236=CARTESIAN_POINT('Ctrl Pts',(-7.32165685034114,-2.99802791882006,
140.766140247165));
#54237=CARTESIAN_POINT('Ctrl Pts',(-7.35995658780249,-2.90085505078464,
140.761908328462));
#54238=CARTESIAN_POINT('Ctrl Pts',(-7.44302986567066,-2.69008418908618,
140.752729170022));
#54239=CARTESIAN_POINT('Ctrl Pts',(-7.51709701138963,-2.47561178123072,
140.743550011582));
#54240=CARTESIAN_POINT('Ctrl Pts',(-7.58186242813559,-2.25815923283232,
140.734370853142));
#54241=CARTESIAN_POINT('Ctrl Pts',(-7.64626385011824,-2.04192881181091,
140.725243283432));
#54242=CARTESIAN_POINT('Ctrl Pts',(-7.70146774048433,-1.82275176528591,
140.716115713722));
#54243=CARTESIAN_POINT('Ctrl Pts',(-7.74722959436371,-1.6013602381148,140.706988144012));
#54244=CARTESIAN_POINT('Ctrl Pts',(-7.79280697487484,-1.38086117567706,
140.697897368999));
#54245=CARTESIAN_POINT('Ctrl Pts',(-7.82901820197523,-1.15816555753905,
140.688806593986));
#54246=CARTESIAN_POINT('Ctrl Pts',(-7.8556687641481,-0.934017809245542,
140.679715818973));
#54247=CARTESIAN_POINT('Ctrl Pts',(-7.88213558553228,-0.711415434884059,
140.670687719792));
#54248=CARTESIAN_POINT('Ctrl Pts',(-7.89917304269829,-0.487381005202657,
140.661659620611));
#54249=CARTESIAN_POINT('Ctrl Pts',(-7.9066383030024,-0.262662798080353,
140.65263152143));
#54250=CARTESIAN_POINT('Ctrl Pts',(-7.90947730148492,-0.177203668321175,
140.649198183699));
#54251=CARTESIAN_POINT('Ctrl Pts',(-7.9109324306235,-0.0916458368497545,
140.645764845968));
#54252=CARTESIAN_POINT('Ctrl Pts',(-7.91099770101101,-0.00603113576254674,
140.642331508237));
#54253=CARTESIAN_POINT('',(-7.90671737907022,0.00501511144919005,138.642331508237));
#54254=CARTESIAN_POINT('Ctrl Pts',(-7.911,7.88147325181399E-12,140.642331508237));
#54255=CARTESIAN_POINT('Ctrl Pts',(-7.91099999999781,2.20167589667468,140.553744072504));
#54256=CARTESIAN_POINT('Ctrl Pts',(-6.94214576671932,4.3861041833938,140.465156636771));
#54257=CARTESIAN_POINT('Ctrl Pts',(-3.67820201487544,7.34180684108005,140.287981765306));
#54258=CARTESIAN_POINT('Ctrl Pts',(-1.40868175870923,8.0899266657148,140.199394329573));
#54259=CARTESIAN_POINT('Ctrl Pts',(2.97309270522057,7.65454228024954,140.022219458108));
#54260=CARTESIAN_POINT('Ctrl Pts',(5.05102072676267,6.47444880833708,139.933632022375));
#54261=CARTESIAN_POINT('Ctrl Pts',(7.66951518848175,2.93425195366915,139.756457150909));
#54262=CARTESIAN_POINT('Ctrl Pts',(8.18956872247135,0.601881960090677,139.667869715177));
#54263=CARTESIAN_POINT('Ctrl Pts',(7.32306689760956,-3.71537198233214,139.490694843711));
#54264=CARTESIAN_POINT('Ctrl Pts',(5.94329958849609,-5.66643518937134,139.402107407979));
#54265=CARTESIAN_POINT('Ctrl Pts',(2.16154501637013,-7.92205913233226,139.224932536513));
#54266=CARTESIAN_POINT('Ctrl Pts',(-0.210816529309054,-8.20894963712981,
139.13634510078));
#54267=CARTESIAN_POINT('Ctrl Pts',(-4.42123908577174,-6.91982244717361,
138.959170229315));
#54268=CARTESIAN_POINT('Ctrl Pts',(-6.22631625634761,-5.35390358802856,
138.870582793582));
#54269=CARTESIAN_POINT('Ctrl Pts',(-7.65317280859725,-2.31334857513722,
138.735440741312));
#54270=CARTESIAN_POINT('Ctrl Pts',(-7.91100000000113,-1.15702837835722,
138.688886124774));
#54271=CARTESIAN_POINT('Ctrl Pts',(-7.911,7.71105401753402E-12,138.642331508237));
#54272=CARTESIAN_POINT('',(-7.92070690004078,0.000688450382506796,136.642332689193));
#54273=CARTESIAN_POINT('Ctrl Pts',(-7.90399247642154,0.00820607573821075,
138.642331508237));
#54274=CARTESIAN_POINT('Ctrl Pts',(-7.91040497386928,0.880579291061528,
138.60731645636));
#54275=CARTESIAN_POINT('Ctrl Pts',(-7.37502394767783,4.3833748071562,138.466367024682));
#54276=CARTESIAN_POINT('Ctrl Pts',(-3.34421556203096,8.05994887033659,138.272450403101));
#54277=CARTESIAN_POINT('Ctrl Pts',(2.08882747359352,7.95366654480699,138.060581643496));
#54278=CARTESIAN_POINT('Ctrl Pts',(6.87299752086058,5.37665868323933,137.848712883892));
#54279=CARTESIAN_POINT('Ctrl Pts',(9.20038080623976,-1.70147935996806,137.583876934383));
#54280=CARTESIAN_POINT('Ctrl Pts',(3.54223654011048,-8.65913268958539,137.266073794978));
#54281=CARTESIAN_POINT('Ctrl Pts',(-5.24241200874194,-7.67706431858937,
136.952225856877));
#54282=CARTESIAN_POINT('Ctrl Pts',(-7.91663072399812,-2.52296611631306,
136.744312298581));
#54283=CARTESIAN_POINT('Ctrl Pts',(-7.92424864988173,0.000678108123123556,
136.642333120087));
#54284=CARTESIAN_POINT('',(-7.90858822339541,-0.00709720147611503,134.642331508237));
#54285=CARTESIAN_POINT('Ctrl Pts',(-7.91099996752649,0.000716795584281833,
136.642331508237));
#54286=CARTESIAN_POINT('Ctrl Pts',(-7.91099111508014,0.0984178756964286,
136.638376844212));
#54287=CARTESIAN_POINT('Ctrl Pts',(-7.90917241970919,0.196100735934578,
136.634422180187));
#54288=CARTESIAN_POINT('Ctrl Pts',(-7.90554545851632,0.293720961682897,
136.630467516162));
#54289=CARTESIAN_POINT('Ctrl Pts',(-7.89835480577871,0.487258500740033,
136.622627174293));
#54290=CARTESIAN_POINT('Ctrl Pts',(-7.88404199044287,0.680822908395119,
136.614786832423));
#54291=CARTESIAN_POINT('Ctrl Pts',(-7.862589869426,0.873842975138913,136.606946490554));
#54292=CARTESIAN_POINT('Ctrl Pts',(-7.84116173251893,1.06664723970303,136.599114914421));
#54293=CARTESIAN_POINT('Ctrl Pts',(-7.81261022220641,1.25890802941457,136.591283338287));
#54294=CARTESIAN_POINT('Ctrl Pts',(-7.77697017092517,1.45005377849934,136.583451762153));
#54295=CARTESIAN_POINT('Ctrl Pts',(-7.74136303631394,1.64102298795184,136.575627419158));
#54296=CARTESIAN_POINT('Ctrl Pts',(-7.69868046261918,1.8308788645228,136.567803076162));
#54297=CARTESIAN_POINT('Ctrl Pts',(-7.64900910350115,2.01905441594737,136.559978733166));
#54298=CARTESIAN_POINT('Ctrl Pts',(-7.59937396699795,2.20709274119893,136.552160096037));
#54299=CARTESIAN_POINT('Ctrl Pts',(-7.54276028534159,2.39345284352173,136.544341458909));
#54300=CARTESIAN_POINT('Ctrl Pts',(-7.47930590308153,2.57757719731723,136.53652282178));
#54301=CARTESIAN_POINT('Ctrl Pts',(-7.41588546727722,2.76160304933861,136.52870836742));
#54302=CARTESIAN_POINT('Ctrl Pts',(-7.34563173519456,2.94339520389513,136.52089391306));
#54303=CARTESIAN_POINT('Ctrl Pts',(-7.26873264174794,3.12241041229177,136.5130794587));
#54304=CARTESIAN_POINT('Ctrl Pts',(-7.19185975164176,3.30136462131586,136.505267667113));
#54305=CARTESIAN_POINT('Ctrl Pts',(-7.10834615052097,3.47754344687064,136.497455875526));
#54306=CARTESIAN_POINT('Ctrl Pts',(-7.01842830329717,3.65042259902566,136.489644083939));
#54307=CARTESIAN_POINT('Ctrl Pts',(-6.92850624777322,3.82330984220358,136.481831926747));
#54308=CARTESIAN_POINT('Ctrl Pts',(-6.83217950146916,3.99289678728025,136.474019769556));
#54309=CARTESIAN_POINT('Ctrl Pts',(-6.72973122239094,4.15868232429173,136.466207612364));
#54310=CARTESIAN_POINT('Ctrl Pts',(-6.62727456807317,4.32448141442095,136.458394816522));
#54311=CARTESIAN_POINT('Ctrl Pts',(-6.51869556836926,4.48647817765456,136.450582020679));
#54312=CARTESIAN_POINT('Ctrl Pts',(-6.40432154194982,4.6441992406999,136.442769224837));
#54313=CARTESIAN_POINT('Ctrl Pts',(-6.2899180402582,4.80196094996018,136.434954415562));
#54314=CARTESIAN_POINT('Ctrl Pts',(-6.16971674319755,4.95544447913854,136.427139606288));
#54315=CARTESIAN_POINT('Ctrl Pts',(-6.044086281573,5.10420826582351,136.419324797014));
#54316=CARTESIAN_POINT('Ctrl Pts',(-5.91840133613917,5.25303656885011,136.411506598589));
#54317=CARTESIAN_POINT('Ctrl Pts',(-5.78728276248387,5.39714078345749,136.403688400164));
#54318=CARTESIAN_POINT('Ctrl Pts',(-5.65113727012219,5.53611493325743,136.395870201739));
#54319=CARTESIAN_POINT('Ctrl Pts',(-5.51483330514526,5.67525084821456,136.388042902974));
#54320=CARTESIAN_POINT('Ctrl Pts',(-5.37349098096021,5.80924452064656,136.380215604208));
#54321=CARTESIAN_POINT('Ctrl Pts',(-5.22755224155258,5.93772840081446,136.372388305443));
#54322=CARTESIAN_POINT('Ctrl Pts',(-5.08151823274156,6.06629615578254,136.364555896985));
#54323=CARTESIAN_POINT('Ctrl Pts',(-4.93088210049844,6.18934672898214,136.356723488527));
#54324=CARTESIAN_POINT('Ctrl Pts',(-4.7761162513342,6.30655488787193,136.348891080069));
#54325=CARTESIAN_POINT('Ctrl Pts',(-4.62112829136721,6.42393125698639,136.341047431001));
#54326=CARTESIAN_POINT('Ctrl Pts',(-4.4619990639663,6.53544826420216,136.333203781933));
#54327=CARTESIAN_POINT('Ctrl Pts',(-4.29922813247562,6.64082513434364,136.325360132865));
#54328=CARTESIAN_POINT('Ctrl Pts',(-4.2114076112622,6.69767958356815,136.321128214161));
#54329=CARTESIAN_POINT('Ctrl Pts',(-4.12252740358087,6.75274745884198,136.316896295458));
#54330=CARTESIAN_POINT('Ctrl Pts',(-4.03266850263118,6.80599043107514,136.312664376754));
#54331=CARTESIAN_POINT('Ctrl Pts',(-3.86454603947509,6.90560593430282,136.304746623602));
#54332=CARTESIAN_POINT('Ctrl Pts',(-3.6924939819573,6.99912829698076,136.296828870449));
#54333=CARTESIAN_POINT('Ctrl Pts',(-3.51699275295656,7.0862319306985,136.288911117296));
#54334=CARTESIAN_POINT('Ctrl Pts',(-3.34169316224011,7.17323548860847,136.281002461072));
#54335=CARTESIAN_POINT('Ctrl Pts',(-3.16295259883223,7.2538348549971,136.273093804848));
#54336=CARTESIAN_POINT('Ctrl Pts',(-2.981279617994,7.32774814246052,136.265185148623));
#54337=CARTESIAN_POINT('Ctrl Pts',(-2.79978173613478,7.40159019125592,136.257284114873));
#54338=CARTESIAN_POINT('Ctrl Pts',(-2.6153573838318,7.468758869378,136.249383081124));
#54339=CARTESIAN_POINT('Ctrl Pts',(-2.4285390862048,7.52901845573349,136.241482047374));
#54340=CARTESIAN_POINT('Ctrl Pts',(-2.24186627611685,7.58923111403626,136.233587166672));
#54341=CARTESIAN_POINT('Ctrl Pts',(-2.05280356129854,7.64254529511686,136.22569228597));
#54342=CARTESIAN_POINT('Ctrl Pts',(-1.86190305875275,7.68877350425978,136.217797405268));
#54343=CARTESIAN_POINT('Ctrl Pts',(-1.67111590581146,7.7349742648148,136.209907212252));
#54344=CARTESIAN_POINT('Ctrl Pts',(-1.47849347330298,7.77409735625623,136.202017019236));
#54345=CARTESIAN_POINT('Ctrl Pts',(-1.28460291636169,7.8060051465058,136.19412682622));
#54346=CARTESIAN_POINT('Ctrl Pts',(-1.09079162088131,7.83789989301508,136.186239858675));
#54347=CARTESIAN_POINT('Ctrl Pts',(-0.895713573480848,7.86258516091987,
136.178352891129));
#54348=CARTESIAN_POINT('Ctrl Pts',(-0.699946279108443,7.87997437853463,
136.170465923584));
#54349=CARTESIAN_POINT('Ctrl Pts',(-0.504195985789498,7.89736208601452,
136.162579640967));
#54350=CARTESIAN_POINT('Ctrl Pts',(-0.307756907132425,7.90745496869302,
136.154693358351));
#54351=CARTESIAN_POINT('Ctrl Pts',(-0.111212357335414,7.91021825309365,
136.146807075735));
#54352=CARTESIAN_POINT('Ctrl Pts',(0.0853318470066554,7.91298153263741,
136.138920806979));
#54353=CARTESIAN_POINT('Ctrl Pts',(0.281981177578248,7.90841523417769,136.131034538224));
#54354=CARTESIAN_POINT('Ctrl Pts',(0.478151515600098,7.89653671732927,136.123148269469));
#54355=CARTESIAN_POINT('Ctrl Pts',(0.674354387994053,7.88465623045781,136.115260692796));
#54356=CARTESIAN_POINT('Ctrl Pts',(0.870077765617847,7.86546112963606,136.107373116122));
#54357=CARTESIAN_POINT('Ctrl Pts',(1.06474159487503,7.83902075109787,136.099485539449));
#54358=CARTESIAN_POINT('Ctrl Pts',(1.25947033545747,7.81257155592426,136.091595332636));
#54359=CARTESIAN_POINT('Ctrl Pts',(1.45313848250933,7.7788723156153,136.083705125822));
#54360=CARTESIAN_POINT('Ctrl Pts',(1.64517487955874,7.73804372019627,136.075814919009));
#54361=CARTESIAN_POINT('Ctrl Pts',(1.83739671872727,7.69717569818222,136.067917092929));
#54362=CARTESIAN_POINT('Ctrl Pts',(2.02798332339201,7.64916464147595,136.060019266848));
#54363=CARTESIAN_POINT('Ctrl Pts',(2.21637641015455,7.59418176030245,136.052121440767));
#54364=CARTESIAN_POINT('Ctrl Pts',(2.40487381372971,7.53916843406851,136.044219241511));
#54365=CARTESIAN_POINT('Ctrl Pts',(2.59117495151574,7.47717569490734,136.036317042255));
#54366=CARTESIAN_POINT('Ctrl Pts',(2.77474002911661,7.40842350104379,136.028414842999));
#54367=CARTESIAN_POINT('Ctrl Pts',(2.95852668368397,7.33958831806949,136.020503105189));
#54368=CARTESIAN_POINT('Ctrl Pts',(3.13957036413097,7.26397751525178,136.012591367379));
#54369=CARTESIAN_POINT('Ctrl Pts',(3.31735346046525,7.18185818701116,136.004679629569));
#54370=CARTESIAN_POINT('Ctrl Pts',(3.39089584404692,7.14788841563545,136.001406832162));
#54371=CARTESIAN_POINT('Ctrl Pts',(3.46388059569693,7.11280545460241,135.998134034754));
#54372=CARTESIAN_POINT('Ctrl Pts',(3.53627246584339,7.07663041618806,135.994861237346));
#54373=CARTESIAN_POINT('Ctrl Pts',(3.72019096729623,6.98472425543122,135.986546381085));
#54374=CARTESIAN_POINT('Ctrl Pts',(3.90068215448687,6.88556557792565,135.978231524823));
#54375=CARTESIAN_POINT('Ctrl Pts',(4.07716969805466,6.77942536305732,135.969916668562));
#54376=CARTESIAN_POINT('Ctrl Pts',(4.25343990334744,6.67341585617406,135.961612051757));
#54377=CARTESIAN_POINT('Ctrl Pts',(4.42571604825334,6.5604421096607,135.953307434951));
#54378=CARTESIAN_POINT('Ctrl Pts',(4.59344533142924,6.44082145282501,135.945002818146));
#54379=CARTESIAN_POINT('Ctrl Pts',(4.76097912543036,6.3213402143607,135.936707880407));
#54380=CARTESIAN_POINT('Ctrl Pts',(4.92397638964062,6.19522768689238,135.928412942667));
#54381=CARTESIAN_POINT('Ctrl Pts',(5.08191160489734,6.06284549036257,135.920118004927));
#54382=CARTESIAN_POINT('Ctrl Pts',(5.23961010463231,5.93066171013067,135.911835499756));
#54383=CARTESIAN_POINT('Ctrl Pts',(5.39226147249852,5.79222720192398,135.903552994586));
#54384=CARTESIAN_POINT('Ctrl Pts',(5.53937162988225,5.64794501974441,135.895270489416));
#54385=CARTESIAN_POINT('Ctrl Pts',(5.68634664563341,5.50379538129939,135.886995592906));
#54386=CARTESIAN_POINT('Ctrl Pts',(5.82779039332744,5.3538089859626,135.878720696396));
#54387=CARTESIAN_POINT('Ctrl Pts',(5.96324280045138,5.19842825312274,135.870445799886));
#54388=CARTESIAN_POINT('Ctrl Pts',(6.09854026778757,5.04322525546144,135.862180368773));
#54389=CARTESIAN_POINT('Ctrl Pts',(6.22785987768987,4.88264045350778,135.853914937659));
#54390=CARTESIAN_POINT('Ctrl Pts',(6.35077908591578,4.71715231913225,135.845649506546));
#54391=CARTESIAN_POINT('Ctrl Pts',(6.39881317348746,4.6524832437827,135.842419560245));
#54392=CARTESIAN_POINT('Ctrl Pts',(6.44587027874722,4.58706578330995,135.839189613944));
#54393=CARTESIAN_POINT('Ctrl Pts',(6.49192678752703,4.52092994696766,135.835959667643));
#54394=CARTESIAN_POINT('Ctrl Pts',(6.60980161422419,4.35166504926146,135.827693097498));
#54395=CARTESIAN_POINT('Ctrl Pts',(6.72098648933855,4.17788312753284,135.819426527353));
#54396=CARTESIAN_POINT('Ctrl Pts',(6.82516088355226,4.00013748684069,135.811159957208));
#54397=CARTESIAN_POINT('Ctrl Pts',(6.9294286192295,3.82223258399623,135.80288598012));
#54398=CARTESIAN_POINT('Ctrl Pts',(7.02667318534892,3.64035712532824,135.794612003032));
#54399=CARTESIAN_POINT('Ctrl Pts',(7.11662041098348,3.45508826601772,135.786338025945));
#54400=CARTESIAN_POINT('Ctrl Pts',(7.20665406874608,3.26964137807256,135.778056098223));
#54401=CARTESIAN_POINT('Ctrl Pts',(7.28937625859859,3.08079484345056,135.769774170502));
#54402=CARTESIAN_POINT('Ctrl Pts',(7.36456093580272,2.88914576005582,135.76149224278));
#54403=CARTESIAN_POINT('Ctrl Pts',(7.43987024045673,2.69717899575291,135.753196586789));
#54404=CARTESIAN_POINT('Ctrl Pts',(7.5076169457623,2.50240066888266,135.744900930798));
#54405=CARTESIAN_POINT('Ctrl Pts',(7.56762425173167,2.30542494664274,135.736605274807));
#54406=CARTESIAN_POINT('Ctrl Pts',(7.62768579269254,2.10827119647023,135.728302121148));
#54407=CARTESIAN_POINT('Ctrl Pts',(7.67999389271445,1.90891636903003,135.719998967489));
#54408=CARTESIAN_POINT('Ctrl Pts',(7.72442260553246,1.70798606877784,135.711695813831));
#54409=CARTESIAN_POINT('Ctrl Pts',(7.76891905599974,1.50674942280136,135.703380000879));
#54410=CARTESIAN_POINT('Ctrl Pts',(7.8055120496907,1.30393279076379,135.695064187926));
#54411=CARTESIAN_POINT('Ctrl Pts',(7.83412706679606,1.10017003290101,135.686748374974));
#54412=CARTESIAN_POINT('Ctrl Pts',(7.84524193292429,1.02102292747637,135.683518282629));
#54413=CARTESIAN_POINT('Ctrl Pts',(7.85515366939065,0.941733108081712,135.680288190284));
#54414=CARTESIAN_POINT('Ctrl Pts',(7.86386002732667,0.862337793798822,135.677058097939));
#54415=CARTESIAN_POINT('Ctrl Pts',(7.8851831639089,0.667887124198026,135.669147132095));
#54416=CARTESIAN_POINT('Ctrl Pts',(7.89931662002861,0.472399687478545,135.661236166252));
#54417=CARTESIAN_POINT('Ctrl Pts',(7.90616827704328,0.276449226937729,135.653325200409));
#54418=CARTESIAN_POINT('Ctrl Pts',(7.91301300081428,0.0806970501535383,
135.645422239732));
#54419=CARTESIAN_POINT('Ctrl Pts',(7.91259059119092,-0.115516875670679,
135.637519279055));
#54420=CARTESIAN_POINT('Ctrl Pts',(7.90486046843095,-0.311611897458337,
135.629616318378));
#54421=CARTESIAN_POINT('Ctrl Pts',(7.89713673729206,-0.507544778861777,
135.621719892233));
#54422=CARTESIAN_POINT('Ctrl Pts',(7.8821173439548,-0.703358609790985,135.613823466087));
#54423=CARTESIAN_POINT('Ctrl Pts',(7.85981370664763,-0.89847064325665,135.605927039942));
#54424=CARTESIAN_POINT('Ctrl Pts',(7.83752438459008,-1.09345744703786,135.598035681997));
#54425=CARTESIAN_POINT('Ctrl Pts',(7.80796017272988,-1.28774300978114,135.590144324053));
#54426=CARTESIAN_POINT('Ctrl Pts',(7.77118448809304,-1.48074732889246,135.582252966108));
#54427=CARTESIAN_POINT('Ctrl Pts',(7.73442560479834,-1.67366347203555,135.57436521341));
#54428=CARTESIAN_POINT('Ctrl Pts',(7.69046187840374,-1.86529920028309,135.566477460711));
#54429=CARTESIAN_POINT('Ctrl Pts',(7.63940826737231,-2.05508207242525,135.558589708013));
#54430=CARTESIAN_POINT('Ctrl Pts',(7.58836853844377,-2.24481334027724,135.550704100091));
#54431=CARTESIAN_POINT('Ctrl Pts',(7.53024285678663,-2.43269242390119,135.54281849217));
#54432=CARTESIAN_POINT('Ctrl Pts',(7.46519681095899,-2.61815919562729,135.534932884248));
#54433=CARTESIAN_POINT('Ctrl Pts',(7.40014309351457,-2.80364784155004,135.527046346287));
#54434=CARTESIAN_POINT('Ctrl Pts',(7.32816748864173,-2.98672327972482,135.519159808327));
#54435=CARTESIAN_POINT('Ctrl Pts',(7.24948499505314,-3.16684200845248,135.511273270366));
#54436=CARTESIAN_POINT('Ctrl Pts',(7.17079258895755,-3.34698342873552,135.503385738851));
#54437=CARTESIAN_POINT('Ctrl Pts',(7.0853917478297,-3.5241670811841,135.495498207335));
#54438=CARTESIAN_POINT('Ctrl Pts',(6.99354501429168,-3.69787089188846,135.48761067582));
#54439=CARTESIAN_POINT('Ctrl Pts',(6.90167131522661,-3.87162570075711,135.479720828583));
#54440=CARTESIAN_POINT('Ctrl Pts',(6.80334811350886,-4.04189832734603,135.471830981346));
#54441=CARTESIAN_POINT('Ctrl Pts',(6.69888327813029,-4.20819246541629,135.46394113411));
#54442=CARTESIAN_POINT('Ctrl Pts',(6.59437026273732,-4.37456329966796,135.456047648012));
#54443=CARTESIAN_POINT('Ctrl Pts',(6.48371015218338,-4.5369516974449,135.448154161915));
#54444=CARTESIAN_POINT('Ctrl Pts',(6.36725351846449,-4.69489122681257,135.440260675818));
#54445=CARTESIAN_POINT('Ctrl Pts',(6.2506622610382,-4.85301333405757,135.432358064862));
#54446=CARTESIAN_POINT('Ctrl Pts',(6.12826130060803,-5.00667602300382,135.424455453906));
#54447=CARTESIAN_POINT('Ctrl Pts',(6.00044153449429,-5.15544589643959,135.41655284295));
#54448=CARTESIAN_POINT('Ctrl Pts',(5.87253699134649,-5.30431444216221,135.408644990551));
#54449=CARTESIAN_POINT('Ctrl Pts',(5.73920671084679,-5.44828345092031,135.400737138153));
#54450=CARTESIAN_POINT('Ctrl Pts',(5.60087783257149,-5.58695699863613,135.392829285755));
#54451=CARTESIAN_POINT('Ctrl Pts',(5.46235968115648,-5.72582029109722,135.384910613171));
#54452=CARTESIAN_POINT('Ctrl Pts',(5.31882952213985,-5.85937341628803,135.376991940588));
#54453=CARTESIAN_POINT('Ctrl Pts',(5.17074776761939,-5.98726051910714,135.369073268005));
#54454=CARTESIAN_POINT('Ctrl Pts',(5.10954590674255,-6.04011597520315,135.36580049818));
#54455=CARTESIAN_POINT('Ctrl Pts',(5.04756691244677,-6.09200409841252,135.362527728355));
#54456=CARTESIAN_POINT('Ctrl Pts',(4.98484468130388,-6.14290196106664,135.35925495853));
#54457=CARTESIAN_POINT('Ctrl Pts',(4.83453200360936,-6.26487775633198,135.351411825612));
#54458=CARTESIAN_POINT('Ctrl Pts',(4.67950387729446,-6.38152445229471,135.343568692693));
#54459=CARTESIAN_POINT('Ctrl Pts',(4.52017677883435,-6.49245122338911,135.335725559774));
#54460=CARTESIAN_POINT('Ctrl Pts',(4.36103679309332,-6.60324772279741,135.32789163778));
#54461=CARTESIAN_POINT('Ctrl Pts',(4.19760817327514,-6.70833747434412,135.320057715786));
#54462=CARTESIAN_POINT('Ctrl Pts',(4.03034210722823,-6.80736832400768,135.312223793792));
#54463=CARTESIAN_POINT('Ctrl Pts',(3.86323994700134,-6.90630213227483,135.304397548342));
#54464=CARTESIAN_POINT('Ctrl Pts',(3.6923081291256,-6.99918868440921,135.296571302893));
#54465=CARTESIAN_POINT('Ctrl Pts',(3.51802876084143,-7.0857176515786,135.288745057443));
#54466=CARTESIAN_POINT('Ctrl Pts',(3.34388629639326,-7.17217864657407,135.280924959842));
#54467=CARTESIAN_POINT('Ctrl Pts',(3.16640183223815,-7.25229184785456,135.27310486224));
#54468=CARTESIAN_POINT('Ctrl Pts',(2.98608431467643,-7.32579152485541,135.265284764638));
#54469=CARTESIAN_POINT('Ctrl Pts',(2.80587341029001,-7.39924774499165,135.257469290689));
#54470=CARTESIAN_POINT('Ctrl Pts',(2.6228331137715,-7.46609809773762,135.249653816739));
#54471=CARTESIAN_POINT('Ctrl Pts',(2.43749488034718,-7.52612381696457,135.241838342789));
#54472=CARTESIAN_POINT('Ctrl Pts',(2.25223022907008,-7.58612570505194,135.234025971703));
#54473=CARTESIAN_POINT('Ctrl Pts',(2.06466979255896,-7.63930824978848,135.226213600618));
#54474=CARTESIAN_POINT('Ctrl Pts',(1.87536299592791,-7.68550158633152,135.218401229532));
#54475=CARTESIAN_POINT('Ctrl Pts',(1.68606336523435,-7.73169317429201,135.210589154172));
#54476=CARTESIAN_POINT('Ctrl Pts',(1.49501784547347,-7.77089598903363,135.202777078813));
#54477=CARTESIAN_POINT('Ctrl Pts',(1.30278940599468,-7.80299050131602,135.194965003453));
#54478=CARTESIAN_POINT('Ctrl Pts',(1.11055534443338,-7.83508595226283,135.187152699615));
#54479=CARTESIAN_POINT('Ctrl Pts',(0.917138641137321,-7.8600726279092,135.179340395776));
#54480=CARTESIAN_POINT('Ctrl Pts',(0.723110773275259,-7.87788244451345,
135.171528091938));
#54481=CARTESIAN_POINT('Ctrl Pts',(0.529043090878745,-7.89569591569354,
135.163714185014));
#54482=CARTESIAN_POINT('Ctrl Pts',(0.3343643443826,-7.9063295619679,135.15590027809));
#54483=CARTESIAN_POINT('Ctrl Pts',(0.139649580975725,-7.90976731608037,
135.148086371167));
#54484=CARTESIAN_POINT('Ctrl Pts',(-0.0551394010230107,-7.91320638054685,
135.140269485849));
#54485=CARTESIAN_POINT('Ctrl Pts',(-0.249964075889232,-7.90944408307697,
135.132452600532));
#54486=CARTESIAN_POINT('Ctrl Pts',(-0.444250795860102,-7.89851645756199,
135.124635715215));
#54487=CARTESIAN_POINT('Ctrl Pts',(-0.638748275819347,-7.88757697788516,
135.116810350231));
#54488=CARTESIAN_POINT('Ctrl Pts',(-0.832706284084506,-7.86945666540598,
135.108984985247));
#54489=CARTESIAN_POINT('Ctrl Pts',(-1.02555662959735,-7.84424340516591,
135.101159620263));
#54490=CARTESIAN_POINT('Ctrl Pts',(-1.21852418100588,-7.81901482142336,
135.093329499369));
#54491=CARTESIAN_POINT('Ctrl Pts',(-1.41038238231514,-7.78668475716327,
135.085499378474));
#54492=CARTESIAN_POINT('Ctrl Pts',(-1.60057451687288,-7.74739196219845,
135.07766925758));
#54493=CARTESIAN_POINT('Ctrl Pts',(-1.79102663147558,-7.70804545658663,
135.06982843343));
#54494=CARTESIAN_POINT('Ctrl Pts',(-1.97980779030585,-7.66171729424447,
135.061987609279));
#54495=CARTESIAN_POINT('Ctrl Pts',(-2.16637658307278,-7.60859602688393,
135.054146785128));
#54496=CARTESIAN_POINT('Ctrl Pts',(-2.26706686920622,-7.57992673267359,
135.049915129793));
#54497=CARTESIAN_POINT('Ctrl Pts',(-2.36711309001969,-7.54927964076426,
135.045683474458));
#54498=CARTESIAN_POINT('Ctrl Pts',(-2.466432769271,-7.51669012229892,135.041451819124));
#54499=CARTESIAN_POINT('Ctrl Pts',(-2.65211313201021,-7.45576328830433,
135.033540644787));
#54500=CARTESIAN_POINT('Ctrl Pts',(-2.83578417829544,-7.38787034295405,
135.025629470451));
#54501=CARTESIAN_POINT('Ctrl Pts',(-3.01688532541028,-7.31316100830032,
135.017718296115));
#54502=CARTESIAN_POINT('Ctrl Pts',(-3.19779013536897,-7.238532668265,135.009815698519));
#54503=CARTESIAN_POINT('Ctrl Pts',(-3.37613027977014,-7.15710278872621,
135.001913100922));
#54504=CARTESIAN_POINT('Ctrl Pts',(-3.55135982482645,-7.06907097111131,
134.994010503326));
#54505=CARTESIAN_POINT('Ctrl Pts',(-3.72643192580988,-6.98111825024865,
134.986115006229));
#54506=CARTESIAN_POINT('Ctrl Pts',(-3.89839868890227,-6.88657556191102,
134.978219509131));
#54507=CARTESIAN_POINT('Ctrl Pts',(-4.06673342096132,-6.78569084786776,
134.970324012034));
#54508=CARTESIAN_POINT('Ctrl Pts',(-4.234948141876,-6.68487805772181,134.962434143885));
#54509=CARTESIAN_POINT('Ctrl Pts',(-4.39953569613678,-6.57773242665006,
134.954544275737));
#54510=CARTESIAN_POINT('Ctrl Pts',(-4.55999305689652,-6.46454826890909,
134.946654407588));
#54511=CARTESIAN_POINT('Ctrl Pts',(-4.72036579199413,-6.35142380481038,
134.938768700579));
#54512=CARTESIAN_POINT('Ctrl Pts',(-4.87661239299423,-6.23226735835444,
134.930882993569));
#54513=CARTESIAN_POINT('Ctrl Pts',(-5.02825771881472,-6.10741723752194,
134.922997286559));
#54514=CARTESIAN_POINT('Ctrl Pts',(-5.17985119644617,-5.98260980348268,
134.915114275706));
#54515=CARTESIAN_POINT('Ctrl Pts',(-5.326846268445,-5.85211279380975,134.907231264854));
#54516=CARTESIAN_POINT('Ctrl Pts',(-5.46879965459889,-5.71630574216067,
134.899348254001));
#54517=CARTESIAN_POINT('Ctrl Pts',(-5.61075515919423,-5.58049666379497,
134.891465125506));
#54518=CARTESIAN_POINT('Ctrl Pts',(-5.74766857261715,-5.43937761735855,
134.883581997011));
#54519=CARTESIAN_POINT('Ctrl Pts',(-5.87913196389727,-5.29336644783652,
134.875698868517));
#54520=CARTESIAN_POINT('Ctrl Pts',(-6.01060348369017,-5.14734625029805,
134.8678152526));
#54521=CARTESIAN_POINT('Ctrl Pts',(-6.13662407855223,-4.99643358295228,
134.859931636684));
#54522=CARTESIAN_POINT('Ctrl Pts',(-6.25682474599815,-4.84108098443573,
134.852048020767));
#54523=CARTESIAN_POINT('Ctrl Pts',(-6.37705305066459,-4.68569266636691,
134.844162592205));
#54524=CARTESIAN_POINT('Ctrl Pts',(-6.49145855034864,-4.52586265573655,
134.836277163643));
#54525=CARTESIAN_POINT('Ctrl Pts',(-6.59971423703762,-4.36207439063606,
134.82839173508));
#54526=CARTESIAN_POINT('Ctrl Pts',(-6.70801301192683,-4.19822093411906,
134.82050316794));
#54527=CARTESIAN_POINT('Ctrl Pts',(-6.81015690638498,-4.03040637137842,
134.8126146008));
#54528=CARTESIAN_POINT('Ctrl Pts',(-6.90586359404163,-3.85914096924308,
134.804726033659));
#54529=CARTESIAN_POINT('Ctrl Pts',(-7.00167213441906,-3.6876933034895,134.796829071369));
#54530=CARTESIAN_POINT('Ctrl Pts',(-7.09102961629076,-3.51278776416627,
134.788932109078));
#54531=CARTESIAN_POINT('Ctrl Pts',(-7.17370033858609,-3.33495793859081,
134.781035146788));
#54532=CARTESIAN_POINT('Ctrl Pts',(-7.25642147902373,-3.15701966047971,
134.773133368401));
#54533=CARTESIAN_POINT('Ctrl Pts',(-7.33244759646324,-2.97615385770899,
134.765231590014));
#54534=CARTESIAN_POINT('Ctrl Pts',(-7.40159197747227,-2.79291195690414,
134.757329811627));
#54535=CARTESIAN_POINT('Ctrl Pts',(-7.47082578604139,-2.60943306104842,
134.749417813512));
#54536=CARTESIAN_POINT('Ctrl Pts',(-7.53315997106042,-2.42357225487405,
134.741505815397));
#54537=CARTESIAN_POINT('Ctrl Pts',(-7.58845798383476,-2.23589499475592,
134.733593817282));
#54538=CARTESIAN_POINT('Ctrl Pts',(-7.61162728258782,-2.15726015254958,
134.730278771426));
#54539=CARTESIAN_POINT('Ctrl Pts',(-7.63356198405403,-2.07830654139874,
134.726963725571));
#54540=CARTESIAN_POINT('Ctrl Pts',(-7.65425473420167,-1.99907615261434,
134.723648679716));
#54541=CARTESIAN_POINT('Ctrl Pts',(-7.71759372002424,-1.7565577615776,134.713501568242));
#54542=CARTESIAN_POINT('Ctrl Pts',(-7.76943036390135,-1.51092178810988,
134.703354456769));
#54543=CARTESIAN_POINT('Ctrl Pts',(-7.80951006415253,-1.26312056348565,
134.693207345296));
#54544=CARTESIAN_POINT('Ctrl Pts',(-7.84891124105464,-1.01951445299105,
134.683232017844));
#54545=CARTESIAN_POINT('Ctrl Pts',(-7.87695022360203,-0.773815615821124,
134.673256690391));
#54546=CARTESIAN_POINT('Ctrl Pts',(-7.89343050424911,-0.526949593974311,
134.663281362939));
#54547=CARTESIAN_POINT('Ctrl Pts',(-7.90496760305664,-0.35412986187993,
134.656298087537));
#54548=CARTESIAN_POINT('Ctrl Pts',(-7.91084097439085,-0.180738545498725,
134.649314812135));
#54549=CARTESIAN_POINT('Ctrl Pts',(-7.91099681386514,-0.00710007152402601,
134.642331536734));
#54550=CARTESIAN_POINT('',(-7.89859990304224,0.000673465603601259,132.642392143699));
#54551=CARTESIAN_POINT('Ctrl Pts',(-7.90858822339541,-0.00709720147611503,
134.642331508237));
#54552=CARTESIAN_POINT('Ctrl Pts',(-7.89174604813805,1.95238971443055,134.56350285226));
#54553=CARTESIAN_POINT('Ctrl Pts',(-6.16908709444098,6.57245961758447,134.378739816482));
#54554=CARTESIAN_POINT('Ctrl Pts',(1.59515389369185,9.21941012471406,134.0880424009));
#54555=CARTESIAN_POINT('Ctrl Pts',(7.42670583543603,4.5815492960006,133.823206451394));
#54556=CARTESIAN_POINT('Ctrl Pts',(8.18443024418726,-0.799445619444897,
133.611337691789));
#54557=CARTESIAN_POINT('Ctrl Pts',(6.39974472309062,-5.93210089235586,133.399468932183));
#54558=CARTESIAN_POINT('Ctrl Pts',(-0.219058148002564,-9.35382555535514,
133.134632982678));
#54559=CARTESIAN_POINT('Ctrl Pts',(-6.81879397155213,-5.54610506984683,
132.864618323215));
#54560=CARTESIAN_POINT('Ctrl Pts',(-7.89554591951126,-1.44945742194562,
132.700538043555));
#54561=CARTESIAN_POINT('Ctrl Pts',(-7.89859990304224,0.000673465603601259,
132.642392143699));
#54562=CARTESIAN_POINT('',(-7.91099958186279,-0.00257211328256086,128.642116733665));
#54563=CARTESIAN_POINT('Ctrl Pts',(-7.9109999900693,0.000396388217883126,
132.635232504311));
#54564=CARTESIAN_POINT('Ctrl Pts',(-7.91094795170318,1.03896286230102,132.594969264453));
#54565=CARTESIAN_POINT('Ctrl Pts',(-7.70642795972031,2.06713172426845,132.562880167328));
#54566=CARTESIAN_POINT('Ctrl Pts',(-7.26277582939789,3.1385874062988,132.519128789588));
#54567=CARTESIAN_POINT('Ctrl Pts',(-7.21378524248674,3.24960670015131,132.514440493338));
#54568=CARTESIAN_POINT('Ctrl Pts',(-7.15375931622026,3.37758044291283,132.508807127237));
#54569=CARTESIAN_POINT('Ctrl Pts',(-7.1451868268163,3.39567772316477,132.508005074824));
#54570=CARTESIAN_POINT('Ctrl Pts',(-7.13393196830758,3.41920639359231,132.506955005739));
#54571=CARTESIAN_POINT('Ctrl Pts',(-7.13131187994195,3.42466765702155,132.506710759162));
#54572=CARTESIAN_POINT('Ctrl Pts',(-7.1270490433218,3.43352693002828,132.506313698973));
#54573=CARTESIAN_POINT('Ctrl Pts',(-7.1254101270074,3.43692679104352,132.506161120237));
#54574=CARTESIAN_POINT('Ctrl Pts',(-7.1222576605826,3.44345449956403,132.505867780234));
#54575=CARTESIAN_POINT('Ctrl Pts',(-7.12074448532198,3.44658251735062,132.505727042026));
#54576=CARTESIAN_POINT('Ctrl Pts',(-7.11726503482431,3.45376312358334,132.505403571937));
#54577=CARTESIAN_POINT('Ctrl Pts',(-7.115297359392,3.45781502933073,132.505220753944));
#54578=CARTESIAN_POINT('Ctrl Pts',(-7.11005202093613,3.46859297733137,132.504733699352));
#54579=CARTESIAN_POINT('Ctrl Pts',(-7.10676828187674,3.47531603883496,132.504429092044));
#54580=CARTESIAN_POINT('Ctrl Pts',(-7.0847362246594,3.52026222537289,132.50238742415));
#54581=CARTESIAN_POINT('Ctrl Pts',(-7.06568946305138,3.55833750450519,132.500632423061));
#54582=CARTESIAN_POINT('Ctrl Pts',(-6.69321051406074,4.28815531483912,132.466529263544));
#54583=CARTESIAN_POINT('Ctrl Pts',(-6.24011065199555,4.9242715280125,132.429196272166));
#54584=CARTESIAN_POINT('Ctrl Pts',(-5.47240228657801,5.72241320228477,132.379576049925));
#54585=CARTESIAN_POINT('Ctrl Pts',(-5.22851662524904,5.9460781776067,132.365197900984));
#54586=CARTESIAN_POINT('Ctrl Pts',(-4.91685151743975,6.1978542360538,132.348540362587));
#54587=CARTESIAN_POINT('Ctrl Pts',(-4.86178908113642,6.24114037931201,132.345656815579));
#54588=CARTESIAN_POINT('Ctrl Pts',(-4.78407932283109,6.30057764708837,132.341668796865));
#54589=CARTESIAN_POINT('Ctrl Pts',(-4.76191150434184,6.31734853394899,132.340540252326));
#54590=CARTESIAN_POINT('Ctrl Pts',(-4.72846890179672,6.34237321974727,132.338851261044));
#54591=CARTESIAN_POINT('Ctrl Pts',(-4.71726000541295,6.35071446828932,132.338287432713));
#54592=CARTESIAN_POINT('Ctrl Pts',(-4.69916748147276,6.36410393121257,132.337380979926));
#54593=CARTESIAN_POINT('Ctrl Pts',(-4.69229770223487,6.36917075767319,132.337037637922));
#54594=CARTESIAN_POINT('Ctrl Pts',(-4.67914146613145,6.37884134098802,132.336381710035));
#54595=CARTESIAN_POINT('Ctrl Pts',(-4.6728563845281,6.38344694687672,132.336069053155));
#54596=CARTESIAN_POINT('Ctrl Pts',(-4.66169209213125,6.39160263530104,132.335514908935));
#54597=CARTESIAN_POINT('Ctrl Pts',(-4.65681560966391,6.39515643180208,132.335273279085));
#54598=CARTESIAN_POINT('Ctrl Pts',(-4.64718383090292,6.40215885053305,132.334796843789));
#54599=CARTESIAN_POINT('Ctrl Pts',(-4.64242875028248,6.40560776229773,132.334562027312));
#54600=CARTESIAN_POINT('Ctrl Pts',(-4.62961550578364,6.41487958645215,132.333930336976));
#54601=CARTESIAN_POINT('Ctrl Pts',(-4.62155018750916,6.42069261881666,132.333533841232));
#54602=CARTESIAN_POINT('Ctrl Pts',(-4.59194489407692,6.44194578181686,132.332082525674));
#54603=CARTESIAN_POINT('Ctrl Pts',(-4.57033821705598,6.45729292855071,132.331031253419));
#54604=CARTESIAN_POINT('Ctrl Pts',(-4.22535730263465,6.69973270689204,132.31437085995));
#54605=CARTESIAN_POINT('Ctrl Pts',(-3.88548028124914,6.90240161556681,132.299733877187));
#54606=CARTESIAN_POINT('Ctrl Pts',(-3.34715800890321,7.17098716448073,132.278355786895));
#54607=CARTESIAN_POINT('Ctrl Pts',(-3.15892726184116,7.25587383091731,132.271183081488));
#54608=CARTESIAN_POINT('Ctrl Pts',(-2.61412396807595,7.47634098188474,132.25091564276));
#54609=CARTESIAN_POINT('Ctrl Pts',(-2.25079216990757,7.5936311732605,132.23799617387));
#54610=CARTESIAN_POINT('Ctrl Pts',(-1.72073573494283,7.72334257308298,132.218493191774));
#54611=CARTESIAN_POINT('Ctrl Pts',(-1.55986348048593,7.75743344346827,132.212486692338));
#54612=CARTESIAN_POINT('Ctrl Pts',(-1.28977901677055,7.80592673992084,132.202096264893));
#54613=CARTESIAN_POINT('Ctrl Pts',(-1.18111550855892,7.82310593368083,132.197834040615));
#54614=CARTESIAN_POINT('Ctrl Pts',(-1.05359868904454,7.84054849938519,132.192701881381));
#54615=CARTESIAN_POINT('Ctrl Pts',(-1.0350550412092,7.84301804279016,132.191952340923));
#54616=CARTESIAN_POINT('Ctrl Pts',(-1.01072785409723,7.84617002853083,132.190964618979));
#54617=CARTESIAN_POINT('Ctrl Pts',(-1.0049519447476,7.84691190851998,132.19072978234));
#54618=CARTESIAN_POINT('Ctrl Pts',(-0.995536243046376,7.84811073097967,
132.190346421189));
#54619=CARTESIAN_POINT('Ctrl Pts',(-0.991896934104965,7.84857152155503,
132.190198115428));
#54620=CARTESIAN_POINT('Ctrl Pts',(-0.984893002831329,7.84945337402424,
132.189912443526));
#54621=CARTESIAN_POINT('Ctrl Pts',(-0.981528426883154,7.84987480442578,
132.189775098502));
#54622=CARTESIAN_POINT('Ctrl Pts',(-0.973829634070222,7.85083409062804,
132.189460566666));
#54623=CARTESIAN_POINT('Ctrl Pts',(-0.969495243439694,7.85137052033414,
132.18928329783));
#54624=CARTESIAN_POINT('Ctrl Pts',(-0.957943699437552,7.85279044268084,
132.188810352685));
#54625=CARTESIAN_POINT('Ctrl Pts',(-0.950725783858959,7.85366757325387,
132.188514307789));
#54626=CARTESIAN_POINT('Ctrl Pts',(-0.90078313612652,7.85966681113154,132.186462296839));
#54627=CARTESIAN_POINT('Ctrl Pts',(-0.85801918780058,7.86445011294794,132.184687024655));
#54628=CARTESIAN_POINT('Ctrl Pts',(0.0186333393416185,7.95527161920517,
132.147953451114));
#54629=CARTESIAN_POINT('Ctrl Pts',(0.86092998641323,7.90858411738611,132.106983843917));
#54630=CARTESIAN_POINT('Ctrl Pts',(1.85443983819299,7.6926427696871,132.061545989791));
#54631=CARTESIAN_POINT('Ctrl Pts',(2.02731538522306,7.64890170177291,132.053719070985));
#54632=CARTESIAN_POINT('Ctrl Pts',(2.31672561877076,7.5651723044627,132.04078890563));
#54633=CARTESIAN_POINT('Ctrl Pts',(2.43406849349038,7.52823764126726,132.035594997805));
#54634=CARTESIAN_POINT('Ctrl Pts',(2.61187809791459,7.46767816836738,132.027801359881));
#54635=CARTESIAN_POINT('Ctrl Pts',(2.6729916807331,7.44602176805093,132.025136644212));
#54636=CARTESIAN_POINT('Ctrl Pts',(2.7582244420919,7.41463381056795,132.02143938825));
#54637=CARTESIAN_POINT('Ctrl Pts',(2.7825714613354,7.40553122319316,132.02038545397));
#54638=CARTESIAN_POINT('Ctrl Pts',(2.81917980552136,7.39163848444385,132.018804006081));
#54639=CARTESIAN_POINT('Ctrl Pts',(2.83147464019921,7.38693749971669,132.018273435129));
#54640=CARTESIAN_POINT('Ctrl Pts',(2.85131051991028,7.37929636407066,132.017418324722));
#54641=CARTESIAN_POINT('Ctrl Pts',(2.85885886034996,7.37637529731627,132.017093128996));
#54642=CARTESIAN_POINT('Ctrl Pts',(2.87330900930542,7.37075784719751,132.016470986355));
#54643=CARTESIAN_POINT('Ctrl Pts',(2.88021153591049,7.36806334213986,132.016173975111));
#54644=CARTESIAN_POINT('Ctrl Pts',(2.89250007835589,7.36324641786719,132.015645513019));
#54645=CARTESIAN_POINT('Ctrl Pts',(2.89788756427784,7.3611277789828,132.015413932));
#54646=CARTESIAN_POINT('Ctrl Pts',(2.90855290091077,7.35692009214983,132.014955689146));
#54647=CARTESIAN_POINT('Ctrl Pts',(2.91383083769874,7.35483127400743,132.014729019584));
#54648=CARTESIAN_POINT('Ctrl Pts',(2.92659786310087,7.34976264332575,132.014180960208));
#54649=CARTESIAN_POINT('Ctrl Pts',(2.93408466238265,7.34677705936597,132.013859770034));
#54650=CARTESIAN_POINT('Ctrl Pts',(2.96183600284105,7.33566120020737,132.012669952706));
#54651=CARTESIAN_POINT('Ctrl Pts',(2.98207151011635,7.32745844549907,132.01180383477));
#54652=CARTESIAN_POINT('Ctrl Pts',(3.32003177746828,7.18882951898955,131.997362332769));
#54653=CARTESIAN_POINT('Ctrl Pts',(3.62897825334765,7.03792785898434,131.984538251107));
#54654=CARTESIAN_POINT('Ctrl Pts',(4.09283314236616,6.77267007839567,131.965391487316));
#54655=CARTESIAN_POINT('Ctrl Pts',(4.2550238055422,6.67196512140592,131.958713375773));
#54656=CARTESIAN_POINT('Ctrl Pts',(4.66916527709572,6.3935732931529,131.941463400556));
#54657=CARTESIAN_POINT('Ctrl Pts',(4.91464688839365,6.20686131123768,131.931043404374));
#54658=CARTESIAN_POINT('Ctrl Pts',(5.33638453856187,5.84534760120043,131.911836957138));
#54659=CARTESIAN_POINT('Ctrl Pts',(5.5164997941389,5.67567683911407,131.903140796033));
#54660=CARTESIAN_POINT('Ctrl Pts',(5.79912937379087,5.38325391866127,131.888111139432));
#54661=CARTESIAN_POINT('Ctrl Pts',(5.90640090886794,5.26533446712871,131.882039253812));
#54662=CARTESIAN_POINT('Ctrl Pts',(6.02509285689291,5.12666690078153,131.874778676996));
#54663=CARTESIAN_POINT('Ctrl Pts',(6.0400763906773,5.10900524752315,131.873851754122));
#54664=CARTESIAN_POINT('Ctrl Pts',(6.05894947626649,5.08655976557817,131.872670662167));
#54665=CARTESIAN_POINT('Ctrl Pts',(6.06291142525821,5.08183668114252,131.872421958219));
#54666=CARTESIAN_POINT('Ctrl Pts',(6.06922349211669,5.07429410611729,131.872024503519));
#54667=CARTESIAN_POINT('Ctrl Pts',(6.07157718244386,5.07147759436793,131.871876024749));
#54668=CARTESIAN_POINT('Ctrl Pts',(6.07601603174254,5.06615838613592,131.871595489335));
#54669=CARTESIAN_POINT('Ctrl Pts',(6.07810160936931,5.0636560346834,131.87146346451));
#54670=CARTESIAN_POINT('Ctrl Pts',(6.08282208055239,5.0579851244103,131.871164149244));
#54671=CARTESIAN_POINT('Ctrl Pts',(6.08545603929925,5.05481580040668,131.870996787837));
#54672=CARTESIAN_POINT('Ctrl Pts',(6.09323888713325,5.04543614999178,131.870501241705));
#54673=CARTESIAN_POINT('Ctrl Pts',(6.09838074083817,5.03922002081146,131.870172522504));
#54674=CARTESIAN_POINT('Ctrl Pts',(6.13259273654294,4.99773114220861,131.867976535246));
#54675=CARTESIAN_POINT('Ctrl Pts',(6.16136566898044,4.96221555058488,131.866087157071));
#54676=CARTESIAN_POINT('Ctrl Pts',(6.66638880892651,4.32768062494586,131.832194411121));
#54677=CARTESIAN_POINT('Ctrl Pts',(7.0535396805134,3.66294428229163,131.794938896219));
#54678=CARTESIAN_POINT('Ctrl Pts',(7.4576447239246,2.65859771345574,131.745354575948));
#54679=CARTESIAN_POINT('Ctrl Pts',(7.55827724914286,2.35734591467176,131.731183309549));
#54680=CARTESIAN_POINT('Ctrl Pts',(7.67660025608047,1.91652548443221,131.711633354972));
#54681=CARTESIAN_POINT('Ctrl Pts',(7.70910570283183,1.7812785755044,131.705788320328));
#54682=CARTESIAN_POINT('Ctrl Pts',(7.7478294659085,1.59914974625125,131.698119186125));
#54683=CARTESIAN_POINT('Ctrl Pts',(7.75721717900618,1.55297233888448,131.696191887625));
#54684=CARTESIAN_POINT('Ctrl Pts',(7.770101227033,1.48656289536027,131.693444391243));
#54685=CARTESIAN_POINT('Ctrl Pts',(7.77393216493602,1.46639729394148,131.692613293131));
#54686=CARTESIAN_POINT('Ctrl Pts',(7.77971464450336,1.43529939845721,131.691336513389));
#54687=CARTESIAN_POINT('Ctrl Pts',(7.78172171020141,1.42437759721175,131.690889025046));
#54688=CARTESIAN_POINT('Ctrl Pts',(7.78541675798574,1.40402941884346,131.690057033618));
#54689=CARTESIAN_POINT('Ctrl Pts',(7.78711063207951,1.39460414064827,131.68967233954));
#54690=CARTESIAN_POINT('Ctrl Pts',(7.78988219011802,1.37901978197349,131.689037387381));
#54691=CARTESIAN_POINT('Ctrl Pts',(7.7909696913176,1.37286247097084,131.688786810826));
#54692=CARTESIAN_POINT('Ctrl Pts',(7.7930877055696,1.36078694157827,131.688295954902));
#54693=CARTESIAN_POINT('Ctrl Pts',(7.79411877955699,1.35486882665335,131.688055657487));
#54694=CARTESIAN_POINT('Ctrl Pts',(7.79648925002074,1.34117064444636,131.687500076104));
#54695=CARTESIAN_POINT('Ctrl Pts',(7.79782374473194,1.33338972914269,131.687184951107));
#54696=CARTESIAN_POINT('Ctrl Pts',(7.80138162582009,1.31245709975048,131.6863384149));
#54697=CARTESIAN_POINT('Ctrl Pts',(7.80358340596412,1.29930171200063,131.685807702898));
#54698=CARTESIAN_POINT('Ctrl Pts',(7.81900233569048,1.20572226688222,131.682041741535));
#54699=CARTESIAN_POINT('Ctrl Pts',(7.83100943927282,1.125102384467,131.678845690526));
#54700=CARTESIAN_POINT('Ctrl Pts',(7.91896026888329,0.464675656566267,131.653035159888));
#54701=CARTESIAN_POINT('Ctrl Pts',(7.9316514265255,-0.121759544513063,131.632629427665));
#54702=CARTESIAN_POINT('Ctrl Pts',(7.84316226858836,-1.11183984236711,131.598400623501));
#54703=CARTESIAN_POINT('Ctrl Pts',(7.77516385517507,-1.51597293921305,131.584434331657));
#54704=CARTESIAN_POINT('Ctrl Pts',(7.63598187411996,-2.07446096873227,131.563252345613));
#54705=CARTESIAN_POINT('Ctrl Pts',(7.59066262230468,-2.23460197419843,131.55694914809));
#54706=CARTESIAN_POINT('Ctrl Pts',(7.52914742851288,-2.42842050066906,131.548915818308));
#54707=CARTESIAN_POINT('Ctrl Pts',(7.51771953247,-2.46357059711809,131.547442850672));
#54708=CARTESIAN_POINT('Ctrl Pts',(7.50329665156053,-2.50689770949118,131.545608370049));
#54709=CARTESIAN_POINT('Ctrl Pts',(7.50053379095651,-2.5151520067348,131.545258032619));
#54710=CARTESIAN_POINT('Ctrl Pts',(7.49616650419597,-2.52812848061597,131.5447059537));
#54711=CARTESIAN_POINT('Ctrl Pts',(7.49457122037041,-2.53285374543423,131.544504643964));
#54712=CARTESIAN_POINT('Ctrl Pts',(7.49172801176544,-2.54124918598517,131.544146488653));
#54713=CARTESIAN_POINT('Ctrl Pts',(7.4904818545929,-2.54491996209606,131.543989725659));
#54714=CARTESIAN_POINT('Ctrl Pts',(7.48759928362759,-2.55339062515391,131.54362760119));
#54715=CARTESIAN_POINT('Ctrl Pts',(7.48596095272213,-2.55818985435979,131.543422150995));
#54716=CARTESIAN_POINT('Ctrl Pts',(7.48145326778402,-2.57135298824682,131.542857884869));
#54717=CARTESIAN_POINT('Ctrl Pts',(7.47857450918445,-2.57971364648603,131.542498638606));
#54718=CARTESIAN_POINT('Ctrl Pts',(7.46438476031598,-2.62070097284575,131.540733359138));
#54719=CARTESIAN_POINT('Ctrl Pts',(7.45287435907547,-2.65325784178718,131.539318388305));
#54720=CARTESIAN_POINT('Ctrl Pts',(7.29297855637333,-3.09626787658655,131.519898925119));
#54721=CARTESIAN_POINT('Ctrl Pts',(7.11109337842901,-3.49381222573771,131.500570918388));
#54722=CARTESIAN_POINT('Ctrl Pts',(6.70528432356826,-4.21626843459996,131.463806649159));
#54723=CARTESIAN_POINT('Ctrl Pts',(6.4880263442299,-4.54348941593306,131.446426747615));
#54724=CARTESIAN_POINT('Ctrl Pts',(6.06606946027511,-5.08665661225072,131.416878620206));
#54725=CARTESIAN_POINT('Ctrl Pts',(5.8718072473367,-5.30972415006333,131.40449583932));
#54726=CARTESIAN_POINT('Ctrl Pts',(5.62930591405306,-5.55855433409347,131.390351730688));
#54727=CARTESIAN_POINT('Ctrl Pts',(5.59273992746962,-5.59534373847565,131.388251003892));
#54728=CARTESIAN_POINT('Ctrl Pts',(5.54429746231643,-5.64313285138328,131.385508756135));
#54729=CARTESIAN_POINT('Ctrl Pts',(5.5327456039383,-5.65445919728429,131.384857818466));
#54730=CARTESIAN_POINT('Ctrl Pts',(5.51384237877515,-5.67288000859969,131.383797472318));
#54731=CARTESIAN_POINT('Ctrl Pts',(5.50651188801334,-5.67999579205593,131.383387458373));
#54732=CARTESIAN_POINT('Ctrl Pts',(5.4925265928464,-5.69351894409775,131.382607452013));
#54733=CARTESIAN_POINT('Ctrl Pts',(5.48587430704625,-5.6999288967277,131.382237386594));
#54734=CARTESIAN_POINT('Ctrl Pts',(5.47167526625449,-5.71356280433379,131.381449524467));
#54735=CARTESIAN_POINT('Ctrl Pts',(5.46412539406275,-5.72078349678331,131.381031819927));
#54736=CARTESIAN_POINT('Ctrl Pts',(5.44114928664589,-5.74267085236367,131.379764322483));
#54737=CARTESIAN_POINT('Ctrl Pts',(5.4256781032117,-5.75729026577929,131.378915860604));
#54738=CARTESIAN_POINT('Ctrl Pts',(5.37373696486679,-5.80597645639405,131.376084006294));
#54739=CARTESIAN_POINT('Ctrl Pts',(5.33700347100113,-5.83976074913527,131.374108585878));
#54740=CARTESIAN_POINT('Ctrl Pts',(5.09255342306083,-6.06035167687583,131.361139427583));
#54741=CARTESIAN_POINT('Ctrl Pts',(4.87538086881165,-6.23639607301965,131.350459051153));
#54742=CARTESIAN_POINT('Ctrl Pts',(4.49149460519032,-6.51524821110713,131.332735679711));
#54743=CARTESIAN_POINT('Ctrl Pts',(4.32945852145937,-6.62403007630357,131.325570973267));
#54744=CARTESIAN_POINT('Ctrl Pts',(3.60891623936488,-7.0700167587946,131.294717704627));
#54745=CARTESIAN_POINT('Ctrl Pts',(3.01400059395305,-7.34336654465063,131.271963906837));
#54746=CARTESIAN_POINT('Ctrl Pts',(2.3670767210127,-7.54861400357023,131.244958244254));
#54747=CARTESIAN_POINT('Ctrl Pts',(2.34173565613689,-7.556513724665,131.243896633074));
#54748=CARTESIAN_POINT('Ctrl Pts',(2.30893497647872,-7.56655803536547,131.24251717119));
#54749=CARTESIAN_POINT('Ctrl Pts',(2.301511101712,-7.56881945063003,131.242204600444));
#54750=CARTESIAN_POINT('Ctrl Pts',(2.28951274441062,-7.5724550317202,131.241698842399));
#54751=CARTESIAN_POINT('Ctrl Pts',(2.28494031214915,-7.57383598871878,131.241505966682));
#54752=CARTESIAN_POINT('Ctrl Pts',(2.27621020899762,-7.57646401205051,131.241137444508));
#54753=CARTESIAN_POINT('Ctrl Pts',(2.27205275564896,-7.57771179953933,131.240961831523));
#54754=CARTESIAN_POINT('Ctrl Pts',(2.26263461859717,-7.5805300424112,131.240563739826));
#54755=CARTESIAN_POINT('Ctrl Pts',(2.2573733266131,-7.58209844338886,131.240341165324));
#54756=CARTESIAN_POINT('Ctrl Pts',(2.2436528585288,-7.58617299361049,131.239760236373));
#54757=CARTESIAN_POINT('Ctrl Pts',(2.23519113137637,-7.58867046615007,131.239401472826));
#54758=CARTESIAN_POINT('Ctrl Pts',(2.18420495671738,-7.60362632226738,131.23723669737));
#54759=CARTESIAN_POINT('Ctrl Pts',(2.14158123999707,-7.61574121246456,131.235414232346));
#54760=CARTESIAN_POINT('Ctrl Pts',(1.37911887385481,-7.82554800652509,131.202554128601));
#54761=CARTESIAN_POINT('Ctrl Pts',(0.634987577964584,-7.92073081713082,
131.166722058371));
#54762=CARTESIAN_POINT('Ctrl Pts',(-0.397712696560308,-7.90618200270992,
131.119963531086));
#54763=CARTESIAN_POINT('Ctrl Pts',(-0.683569875026899,-7.88661151090959,
131.107286691559));
#54764=CARTESIAN_POINT('Ctrl Pts',(-1.10081546267506,-7.83518350010563,
131.089340236663));
#54765=CARTESIAN_POINT('Ctrl Pts',(-1.233441738958,-7.8154026753967,131.083717454687));
#54766=CARTESIAN_POINT('Ctrl Pts',(-1.43349669254303,-7.78034529779056,
131.075361766605));
#54767=CARTESIAN_POINT('Ctrl Pts',(-1.5013298142648,-7.76754110587916,131.072550574063));
#54768=CARTESIAN_POINT('Ctrl Pts',(-1.58185370165547,-7.75124713669702,
131.069239008941));
#54769=CARTESIAN_POINT('Ctrl Pts',(-1.59471308578156,-7.74861171332221,
131.068710940988));
#54770=CARTESIAN_POINT('Ctrl Pts',(-1.614516634146,-7.7445017549083,131.067898901919));
#54771=CARTESIAN_POINT('Ctrl Pts',(-1.62146544308083,-7.74304986494043,
131.067614193809));
#54772=CARTESIAN_POINT('Ctrl Pts',(-1.63413641041717,-7.74038457748103,
131.067095446513));
#54773=CARTESIAN_POINT('Ctrl Pts',(-1.63985919138712,-7.73917418383735,
131.066861309592));
#54774=CARTESIAN_POINT('Ctrl Pts',(-1.6523363781673,-7.73652074240015,131.066351160731));
#54775=CARTESIAN_POINT('Ctrl Pts',(-1.6590902503675,-7.7350751932775,131.066075230638));
#54776=CARTESIAN_POINT('Ctrl Pts',(-1.67749774714395,-7.73111017012517,
131.0653237668));
#54777=CARTESIAN_POINT('Ctrl Pts',(-1.68914760465236,-7.72857318821637,
131.06484880544));
#54778=CARTESIAN_POINT('Ctrl Pts',(-1.74492752582118,-7.71629388370907,
131.062577667096));
#54779=CARTESIAN_POINT('Ctrl Pts',(-1.78897972468597,-7.7061997769764,131.060793023287));
#54780=CARTESIAN_POINT('Ctrl Pts',(-1.84706304523951,-7.69236568150757,
131.058451378223));
#54781=CARTESIAN_POINT('Ctrl Pts',(-1.86117336115243,-7.68896386997159,
131.057883410271));
#54782=CARTESIAN_POINT('Ctrl Pts',(-2.71240001714543,-7.48126383329723,
131.023673000603));
#54783=CARTESIAN_POINT('Ctrl Pts',(-3.51042653431377,-7.14165685064727,
130.995560409281));
#54784=CARTESIAN_POINT('Ctrl Pts',(-4.40954899709344,-6.57123057393559,
130.958885717486));
#54785=CARTESIAN_POINT('Ctrl Pts',(-4.57683320094183,-6.4558334586399,130.951772417187));
#54786=CARTESIAN_POINT('Ctrl Pts',(-4.89572206163713,-6.21722635110868,
130.937284777857));
#54787=CARTESIAN_POINT('Ctrl Pts',(-5.04757169919715,-6.09458844169352,
130.92993623124));
#54788=CARTESIAN_POINT('Ctrl Pts',(-5.21396155370323,-5.94972071977245,
130.921173455877));
#54789=CARTESIAN_POINT('Ctrl Pts',(-5.23311934502349,-5.93287734738094,
130.920153436527));
#54790=CARTESIAN_POINT('Ctrl Pts',(-5.25694017960767,-5.9117291218545,130.918870767154));
#54791=CARTESIAN_POINT('Ctrl Pts',(-5.26168014864321,-5.90751075116037,
130.918614820894));
#54792=CARTESIAN_POINT('Ctrl Pts',(-5.26917320794426,-5.90082607495836,
130.918209072388));
#54793=CARTESIAN_POINT('Ctrl Pts',(-5.27192966505674,-5.89836352464966,
130.918059565217));
#54794=CARTESIAN_POINT('Ctrl Pts',(-5.27711113120327,-5.89372799774494,
130.917778064739));
#54795=CARTESIAN_POINT('Ctrl Pts',(-5.27953652128446,-5.89155545869114,
130.91764610613));
#54796=CARTESIAN_POINT('Ctrl Pts',(-5.28499159555949,-5.88666301156981,
130.917348882059));
#54797=CARTESIAN_POINT('Ctrl Pts',(-5.28802052075513,-5.88394226253862,
130.917183550488));
#54798=CARTESIAN_POINT('Ctrl Pts',(-5.29572919494782,-5.87700714265529,
130.916762021924));
#54799=CARTESIAN_POINT('Ctrl Pts',(-5.30040600605356,-5.87278952726674,
130.916505571665));
#54800=CARTESIAN_POINT('Ctrl Pts',(-5.32636533793939,-5.84932276106918,
130.915078178322));
#54801=CARTESIAN_POINT('Ctrl Pts',(-5.34754778819162,-5.82996372960949,
130.91389875151));
#54802=CARTESIAN_POINT('Ctrl Pts',(-5.6946911491533,-5.50921931710964,130.894334496078));
#54803=CARTESIAN_POINT('Ctrl Pts',(-5.99479350416303,-5.18106042245828,
130.8740210156));
#54804=CARTESIAN_POINT('Ctrl Pts',(-6.5200741493786,-4.49956539958774,130.834228668107));
#54805=CARTESIAN_POINT('Ctrl Pts',(-6.74794193065218,-4.15003275107279,
130.814844099563));
#54806=CARTESIAN_POINT('Ctrl Pts',(-7.03508379043539,-3.62287872985283,
130.788037293962));
#54807=CARTESIAN_POINT('Ctrl Pts',(-7.11729875571675,-3.45857170326395,
130.779987059471));
#54808=CARTESIAN_POINT('Ctrl Pts',(-7.25185074359103,-3.16450617368557,
130.766146800626));
#54809=CARTESIAN_POINT('Ctrl Pts',(-7.30660454619088,-3.03594651390896,
130.760279047811));
#54810=CARTESIAN_POINT('Ctrl Pts',(-7.38440199271126,-2.83896508320385,
130.751563044479));
#54811=CARTESIAN_POINT('Ctrl Pts',(-7.40996021439371,-2.77157094916318,
130.748628567891));
#54812=CARTESIAN_POINT('Ctrl Pts',(-7.43910990870253,-2.69141957275958,
130.745193644116));
#54813=CARTESIAN_POINT('Ctrl Pts',(-7.4435943489459,-2.67899210917003,130.744662612598));
#54814=CARTESIAN_POINT('Ctrl Pts',(-7.4504348339017,-2.65988570112069,130.74384855905));
#54815=CARTESIAN_POINT('Ctrl Pts',(-7.45281306624921,-2.6532147589541,130.743564778228));
#54816=CARTESIAN_POINT('Ctrl Pts',(-7.45695171924324,-2.64155636517062,
130.74306960412));
#54817=CARTESIAN_POINT('Ctrl Pts',(-7.45871610049223,-2.63657033016418,
130.742858075597));
#54818=CARTESIAN_POINT('Ctrl Pts',(-7.4624012307939,-2.62612307113866,130.742415373882));
#54819=CARTESIAN_POINT('Ctrl Pts',(-7.46432098856182,-2.62066149932168,
130.742184234618));
#54820=CARTESIAN_POINT('Ctrl Pts',(-7.46963049808029,-2.60550316436887,
130.741543532976));
#54821=CARTESIAN_POINT('Ctrl Pts',(-7.47300736680033,-2.59580188269205,
130.741134410099));
#54822=CARTESIAN_POINT('Ctrl Pts',(-7.48628578863159,-2.5574141320149,130.739519155188));
#54823=CARTESIAN_POINT('Ctrl Pts',(-7.49604119900371,-2.52867718805475,
130.738317999717));
#54824=CARTESIAN_POINT('Ctrl Pts',(-7.64727756504756,-2.07460648163473,
130.719462981015));
#54825=CARTESIAN_POINT('Ctrl Pts',(-7.75253102546044,-1.63803713484436,
130.703121639252));
#54826=CARTESIAN_POINT('Ctrl Pts',(-7.88062165178306,-0.799703456417926,
130.673462881414));
#54827=CARTESIAN_POINT('Ctrl Pts',(-7.91095997801479,-0.400537241286116,
130.660034885164));
#54828=CARTESIAN_POINT('Ctrl Pts',(-7.91103291491228,0.328689150824926,
130.634747395728));
#54829=CARTESIAN_POINT('Ctrl Pts',(-7.89048220500111,0.657826822631501,
130.623038747333));
#54830=CARTESIAN_POINT('Ctrl Pts',(-7.83991796357951,1.06089848483932,130.6073645755));
#54831=CARTESIAN_POINT('Ctrl Pts',(-7.82924963479842,1.13695589894975,130.604347262515));
#54832=CARTESIAN_POINT('Ctrl Pts',(-7.81600004916629,1.22235711517645,130.600880103638));
#54833=CARTESIAN_POINT('Ctrl Pts',(-7.81450671352799,1.23186789399559,130.600492872467));
#54834=CARTESIAN_POINT('Ctrl Pts',(-7.81230726535053,1.24571082433252,130.599927613742));
#54835=CARTESIAN_POINT('Ctrl Pts',(-7.81161489773633,1.2500451813399,130.599750390828));
#54836=CARTESIAN_POINT('Ctrl Pts',(-7.81038073212566,1.25773023339407,130.599435751197));
#54837=CARTESIAN_POINT('Ctrl Pts',(-7.8098403834645,1.26108116530687,130.599298418585));
#54838=CARTESIAN_POINT('Ctrl Pts',(-7.80871313508163,1.26804320058586,130.599012802242));
#54839=CARTESIAN_POINT('Ctrl Pts',(-7.80812588674762,1.27165424591941,130.598864498432));
#54840=CARTESIAN_POINT('Ctrl Pts',(-7.80660454369678,1.28096834298144,130.598481559491));
#54841=CARTESIAN_POINT('Ctrl Pts',(-7.80566670570576,1.28667077237749,130.59824671014));
#54842=CARTESIAN_POINT('Ctrl Pts',(-7.80172808803881,1.31045635015706,130.597265468251));
#54843=CARTESIAN_POINT('Ctrl Pts',(-7.79867073197085,1.32852994290822,130.596515875738));
#54844=CARTESIAN_POINT('Ctrl Pts',(-7.77742721374019,1.45151065805286,130.591388921731));
#54845=CARTESIAN_POINT('Ctrl Pts',(-7.75718827594154,1.55604803244397,130.586900046625));
#54846=CARTESIAN_POINT('Ctrl Pts',(-7.70222767587984,1.81211778496722,130.575636306599));
#54847=CARTESIAN_POINT('Ctrl Pts',(-7.66513785409964,1.96309440088421,130.568762424454));
#54848=CARTESIAN_POINT('Ctrl Pts',(-7.48713718941258,2.6053527430499,130.538793985833));
#54849=CARTESIAN_POINT('Ctrl Pts',(-7.3032496197308,3.08344847744397,130.51472866198));
#54850=CARTESIAN_POINT('Ctrl Pts',(-6.86133372848045,3.96647821342088,130.469937158483));
#54851=CARTESIAN_POINT('Ctrl Pts',(-6.61007948701673,4.37239069874427,130.449186903871));
#54852=CARTESIAN_POINT('Ctrl Pts',(-6.30555883645787,4.77752756079774,130.428587305544));
#54853=CARTESIAN_POINT('Ctrl Pts',(-6.28718655365735,4.80167961241627,130.427359353216));
#54854=CARTESIAN_POINT('Ctrl Pts',(-6.26117714035271,4.83546615375253,130.425641564277));
#54855=CARTESIAN_POINT('Ctrl Pts',(-6.25365594172405,4.84518931222048,130.425147215988));
#54856=CARTESIAN_POINT('Ctrl Pts',(-6.24174007671733,4.86051978374536,130.424367769685));
#54857=CARTESIAN_POINT('Ctrl Pts',(-6.23736046119012,4.866138739391,130.424082083511));
#54858=CARTESIAN_POINT('Ctrl Pts',(-6.22925650876816,4.87650702598924,130.423554919828));
#54859=CARTESIAN_POINT('Ctrl Pts',(-6.22553431762297,4.881258022975,130.423313358516));
#54860=CARTESIAN_POINT('Ctrl Pts',(-6.21728122239431,4.89176746076434,130.422779006194));
#54861=CARTESIAN_POINT('Ctrl Pts',(-6.2127477451879,4.89752387881474,130.42248631656));
#54862=CARTESIAN_POINT('Ctrl Pts',(-6.1998036349346,4.91391286838042,130.421652988074));
#54863=CARTESIAN_POINT('Ctrl Pts',(-6.19137364097122,4.92453015322171,130.421113111792));
#54864=CARTESIAN_POINT('Ctrl Pts',(-6.13831449288885,4.99100470561949,130.417732766416));
#54865=CARTESIAN_POINT('Ctrl Pts',(-6.09295647148239,5.04627729650937,130.41492124437));
#54866=CARTESIAN_POINT('Ctrl Pts',(-5.95725269975102,5.20714624530884,130.406730687115));
#54867=CARTESIAN_POINT('Ctrl Pts',(-5.86486542671557,5.31098742954592,130.401434120583));
#54868=CARTESIAN_POINT('Ctrl Pts',(-5.50603241222408,5.69351859760438,130.381813610588));
#54869=CARTESIAN_POINT('Ctrl Pts',(-5.22206775622077,5.95504643575549,130.368202391086));
#54870=CARTESIAN_POINT('Ctrl Pts',(-4.80019551598562,6.29011228114838,130.349482684246));
#54871=CARTESIAN_POINT('Ctrl Pts',(-4.67749188618746,6.38188523948141,130.344192836534));
#54872=CARTESIAN_POINT('Ctrl Pts',(-4.41120547188366,6.56923954120295,130.332904058251));
#54873=CARTESIAN_POINT('Ctrl Pts',(-4.26700664810291,6.66380479476013,130.326902525107));
#54874=CARTESIAN_POINT('Ctrl Pts',(-4.10284402528909,6.76394767028824,130.320080444955));
#54875=CARTESIAN_POINT('Ctrl Pts',(-4.08581278607769,6.77424911373059,130.319372789222));
#54876=CARTESIAN_POINT('Ctrl Pts',(-3.81139426529799,6.93882140184577,130.307969700936));
#54877=CARTESIAN_POINT('Ctrl Pts',(-3.5454922719141,7.07837721351181,130.296912953092));
#54878=CARTESIAN_POINT('Ctrl Pts',(-3.25463932061844,7.21052158760868,130.284179645582));
#54879=CARTESIAN_POINT('Ctrl Pts',(-3.23691660724795,7.21849496352832,130.283401292647));
#54880=CARTESIAN_POINT('Ctrl Pts',(-3.21347062439935,7.22893950760221,130.28236811055));
#54881=CARTESIAN_POINT('Ctrl Pts',(-3.2077734325387,7.23146938481679,130.282116785247));
#54882=CARTESIAN_POINT('Ctrl Pts',(-3.19893421058472,7.23538200102203,130.281726425675));
#54883=CARTESIAN_POINT('Ctrl Pts',(-3.1957942504147,7.23676943762263,130.281587674613));
#54884=CARTESIAN_POINT('Ctrl Pts',(-3.18953558221783,7.23953005254834,130.281310943462));
#54885=CARTESIAN_POINT('Ctrl Pts',(-3.18641689944599,7.2409032554512,130.281172965483));
#54886=CARTESIAN_POINT('Ctrl Pts',(-3.17938646988891,7.24399343765884,130.280861735138));
#54887=CARTESIAN_POINT('Ctrl Pts',(-3.17547422640833,7.24570926045485,130.280688413514));
#54888=CARTESIAN_POINT('Ctrl Pts',(-3.16392437808449,7.25076361555622,130.280176347699));
#54889=CARTESIAN_POINT('Ctrl Pts',(-3.15628290402593,7.25409323814436,130.279837070396));
#54890=CARTESIAN_POINT('Ctrl Pts',(-3.0973794629864,7.27964856541783,130.277218099187));
#54891=CARTESIAN_POINT('Ctrl Pts',(-3.04588968978225,7.30134223921569,130.274907249107));
#54892=CARTESIAN_POINT('Ctrl Pts',(-2.87136915736464,7.37270392794885,130.267013586535));
#54893=CARTESIAN_POINT('Ctrl Pts',(-2.74732391538786,7.41982023551406,130.261301297803));
#54894=CARTESIAN_POINT('Ctrl Pts',(-2.27203882899092,7.58679602875068,130.239191723613));
#54895=CARTESIAN_POINT('Ctrl Pts',(-1.9137103059457,7.68500675676215,130.222089342572));
#54896=CARTESIAN_POINT('Ctrl Pts',(-0.906523780322296,7.88622173017763,
130.174927234953));
#54897=CARTESIAN_POINT('Ctrl Pts',(-0.249631199968885,7.93424366056588,
130.145415133292));
#54898=CARTESIAN_POINT('Ctrl Pts',(0.450221938594702,7.89830405165142,130.116818826349));
#54899=CARTESIAN_POINT('Ctrl Pts',(0.49470468697603,7.89564272514561,130.115012083063));
#54900=CARTESIAN_POINT('Ctrl Pts',(0.55122710415142,7.89178154158142,130.112729866365));
#54901=CARTESIAN_POINT('Ctrl Pts',(0.563289279236045,7.89092975573633,130.112243613629));
#54902=CARTESIAN_POINT('Ctrl Pts',(0.582408222969144,7.88953558534941,130.111474122293));
#54903=CARTESIAN_POINT('Ctrl Pts',(0.58946627508628,7.88901138302808,130.111190319687));
#54904=CARTESIAN_POINT('Ctrl Pts',(0.602602291767799,7.88801804253934,130.110662618495));
#54905=CARTESIAN_POINT('Ctrl Pts',(0.608680432799848,7.8875513495894,130.110418644177));
#54906=CARTESIAN_POINT('Ctrl Pts',(0.622142988460595,7.8865020110791,130.109878697659));
#54907=CARTESIAN_POINT('Ctrl Pts',(0.629527140494808,7.88591601835874,130.109582829671));
#54908=CARTESIAN_POINT('Ctrl Pts',(0.650795692714577,7.88419812178436,130.108731474332));
#54909=CARTESIAN_POINT('Ctrl Pts',(0.664677971958839,7.88303991194524,130.108176805025));
#54910=CARTESIAN_POINT('Ctrl Pts',(0.756990123922037,7.87509265190044,130.104495190106));
#54911=CARTESIAN_POINT('Ctrl Pts',(0.835319224920858,7.86716979354909,130.101403665925));
#54912=CARTESIAN_POINT('Ctrl Pts',(1.05408590595373,7.84173769891461,130.092853915453));
#54913=CARTESIAN_POINT('Ctrl Pts',(1.19419307205132,7.82162722728017,130.087476680529));
#54914=CARTESIAN_POINT('Ctrl Pts',(1.49027988480946,7.77098607757518,130.076281392198));
#54915=CARTESIAN_POINT('Ctrl Pts',(1.64603128935182,7.73949238604636,130.070492881113));
#54916=CARTESIAN_POINT('Ctrl Pts',(2.06726376488785,7.64102493061572,130.055004966588));
#54917=CARTESIAN_POINT('Ctrl Pts',(2.33038643058641,7.56492872936868,130.045519425484));
#54918=CARTESIAN_POINT('Ctrl Pts',(2.8478452158403,7.38571008781671,130.026672806573));
#54919=CARTESIAN_POINT('Ctrl Pts',(3.1018167686513,7.28269619177499,130.017323336003));
#54920=CARTESIAN_POINT('Ctrl Pts',(3.66125196792386,7.02120026050839,129.995643578202));
#54921=CARTESIAN_POINT('Ctrl Pts',(3.96273547279232,6.85556009797179,129.98318309493));
#54922=CARTESIAN_POINT('Ctrl Pts',(4.27192873229387,6.65845917864147,129.968605280587));
#54923=CARTESIAN_POINT('Ctrl Pts',(4.29133686943987,6.64596731711211,129.96768228304));
#54924=CARTESIAN_POINT('Ctrl Pts',(4.31614169682477,6.62984797163986,129.966492066511));
#54925=CARTESIAN_POINT('Ctrl Pts',(4.32158913210057,6.62629841215792,129.966230024657));
#54926=CARTESIAN_POINT('Ctrl Pts',(4.32993920728474,6.62084281036624,129.965827338139));
#54927=CARTESIAN_POINT('Ctrl Pts',(4.33284498851648,6.61894155917422,129.965687016161));
#54928=CARTESIAN_POINT('Ctrl Pts',(4.33827209714199,6.61538549947473,129.965424582212));
#54929=CARTESIAN_POINT('Ctrl Pts',(4.34079373370236,6.61373116001208,129.965302502059));
#54930=CARTESIAN_POINT('Ctrl Pts',(4.3464254523047,6.61003181854868,129.965029531019));
#54931=CARTESIAN_POINT('Ctrl Pts',(4.34953503656226,6.60798606386961,129.964878588751));
#54932=CARTESIAN_POINT('Ctrl Pts',(4.35791601134747,6.60246385158004,129.964471171882));
#54933=CARTESIAN_POINT('Ctrl Pts',(4.36318464149177,6.5989833047822,129.964214414518));
#54934=CARTESIAN_POINT('Ctrl Pts',(4.37481178386018,6.59128220451629,129.963646381333));
#54935=CARTESIAN_POINT('Ctrl Pts',(4.38116835252576,6.58705876016172,129.963334908169));
#54936=CARTESIAN_POINT('Ctrl Pts',(4.40028359449438,6.57431826218581,129.962395484877));
#54937=CARTESIAN_POINT('Ctrl Pts',(4.41302355311181,6.56577333129612,129.961765651342));
#54938=CARTESIAN_POINT('Ctrl Pts',(4.5586595980414,6.46747712409643,129.954523808993));
#54939=CARTESIAN_POINT('Ctrl Pts',(4.68881475888441,6.37374677186225,129.947651275249));
#54940=CARTESIAN_POINT('Ctrl Pts',(5.1233848425342,6.04027707809516,129.923574407558));
#54941=CARTESIAN_POINT('Ctrl Pts',(5.41299301948203,5.7821711650125,129.905577592736));
#54942=CARTESIAN_POINT('Ctrl Pts',(6.14848771365607,5.02280815117252,129.856663723811));
#54943=CARTESIAN_POINT('Ctrl Pts',(6.55155729124435,4.48440551749035,129.826341119464));
#54944=CARTESIAN_POINT('Ctrl Pts',(6.90486569511002,3.86120498475101,129.797100233172));
#54945=CARTESIAN_POINT('Ctrl Pts',(6.92739532360677,3.82063716295443,129.795219334459));
#54946=CARTESIAN_POINT('Ctrl Pts',(6.95529007101208,3.76935067364485,129.792869415242));
#54947=CARTESIAN_POINT('Ctrl Pts',(6.96098927351625,3.75881534642264,129.792388164429));
#54948=CARTESIAN_POINT('Ctrl Pts',(6.96992703207091,3.74220330565532,129.791631638365));
#54949=CARTESIAN_POINT('Ctrl Pts',(6.97318160791635,3.73613525940729,129.791355778087));
#54950=CARTESIAN_POINT('Ctrl Pts',(6.97891353453246,3.72541469644168,129.79086926035));
#54951=CARTESIAN_POINT('Ctrl Pts',(6.98139416334596,3.72076394294004,129.790658483422));
#54952=CARTESIAN_POINT('Ctrl Pts',(6.98706046349019,3.710114985596,129.790176506358));
#54953=CARTESIAN_POINT('Ctrl Pts',(6.99024306444631,3.70411514765395,129.789905418144));
#54954=CARTESIAN_POINT('Ctrl Pts',(6.99897160518982,3.68760879346859,129.78916089943));
#54955=CARTESIAN_POINT('Ctrl Pts',(7.00450162070745,3.67709385127044,129.788688048122));
#54956=CARTESIAN_POINT('Ctrl Pts',(7.03357417576426,3.62151082991424,129.786195990742));
#54957=CARTESIAN_POINT('Ctrl Pts',(7.0567057497454,3.57622852511627,129.784191699709));
#54958=CARTESIAN_POINT('Ctrl Pts',(7.33623988730976,3.01573928471543,129.759693960859));
#54959=CARTESIAN_POINT('Ctrl Pts',(7.53613457561179,2.47423775956985,129.739426712922));
#54960=CARTESIAN_POINT('Ctrl Pts',(7.78175836120098,1.4901746636461,129.704630106344));
#54961=CARTESIAN_POINT('Ctrl Pts',(7.85240419935489,1.05645206810225,129.689882829755));
#54962=CARTESIAN_POINT('Ctrl Pts',(7.89189627365271,0.553392608066614,129.671517693239));
#54963=CARTESIAN_POINT('Ctrl Pts',(7.89623517872882,0.4875857633679,129.669089836548));
#54964=CARTESIAN_POINT('Ctrl Pts',(7.90142894480188,0.390298131621056,129.665453328132));
#54965=CARTESIAN_POINT('Ctrl Pts',(7.90291947863621,0.358853281744243,129.664270674074));
#54966=CARTESIAN_POINT('Ctrl Pts',(7.90914218715489,0.208622464443032,129.658582233375));
#54967=CARTESIAN_POINT('Ctrl Pts',(7.91138390237421,0.0897536189072339,
129.653967339659));
#54968=CARTESIAN_POINT('Ctrl Pts',(7.91090739964824,-0.0397183049235798,
129.648773925764));
#54969=CARTESIAN_POINT('Ctrl Pts',(7.91084705873395,-0.0503213750072018,
129.64834739304));
#54970=CARTESIAN_POINT('Ctrl Pts',(7.91073288312687,-0.0651466138367077,
129.647749269595));
#54971=CARTESIAN_POINT('Ctrl Pts',(7.91069698433689,-0.069368950915418,
129.647578721792));
#54972=CARTESIAN_POINT('Ctrl Pts',(7.91062905017654,-0.0766715024336212,
129.647283413328));
#54973=CARTESIAN_POINT('Ctrl Pts',(7.91059859616372,-0.0797517341501573,
129.647158745351));
#54974=CARTESIAN_POINT('Ctrl Pts',(7.91053171446854,-0.0861390295293632,
129.646900006965));
#54975=CARTESIAN_POINT('Ctrl Pts',(7.91049501205948,-0.089446085388177,
129.646765920428));
#54976=CARTESIAN_POINT('Ctrl Pts',(7.91040463386372,-0.0971539956987106,
129.646453109994));
#54977=CARTESIAN_POINT('Ctrl Pts',(7.91034935952926,-0.101554814625001,
129.646274292468));
#54978=CARTESIAN_POINT('Ctrl Pts',(7.91017303965176,-0.114718269392096,
129.645738774668));
#54979=CARTESIAN_POINT('Ctrl Pts',(7.91004110655744,-0.123480726956874,
129.645381437396));
#54980=CARTESIAN_POINT('Ctrl Pts',(7.90969290272184,-0.144307972731015,
129.644530074622));
#54981=CARTESIAN_POINT('Ctrl Pts',(7.90946358783047,-0.156372491319765,
129.644035299601));
#54982=CARTESIAN_POINT('Ctrl Pts',(7.90692252491599,-0.275692275676478,
129.639126315437));
#54983=CARTESIAN_POINT('Ctrl Pts',(7.90245697727143,-0.382886144758461,
129.634591676301));
#54984=CARTESIAN_POINT('Ctrl Pts',(7.88285869803527,-0.698722364194374,
129.620930994689));
#54985=CARTESIAN_POINT('Ctrl Pts',(7.8616296712863,-0.906886636209906,129.611541876902));
#54986=CARTESIAN_POINT('Ctrl Pts',(7.79915128432483,-1.34617114277955,129.591241951095));
#54987=CARTESIAN_POINT('Ctrl Pts',(7.75581255659185,-1.57680218338523,129.580295971233));
#54988=CARTESIAN_POINT('Ctrl Pts',(7.6428324482774,-2.05886745411721,129.557190648255));
#54989=CARTESIAN_POINT('Ctrl Pts',(7.57087182499121,-2.30948694244284,129.545047239426));
#54990=CARTESIAN_POINT('Ctrl Pts',(7.33052846009506,-3.0134381865324,129.511055926809));
#54991=CARTESIAN_POINT('Ctrl Pts',(7.13279493832639,-3.4555468762655,129.489921457265));
#54992=CARTESIAN_POINT('Ctrl Pts',(6.87913559696617,-3.90673603390423,129.468867828611));
#54993=CARTESIAN_POINT('Ctrl Pts',(6.86216484522073,-3.93646880807375,129.467482476924));
#54994=CARTESIAN_POINT('Ctrl Pts',(6.83956830570848,-3.97546775100461,129.465667932728));
#54995=CARTESIAN_POINT('Ctrl Pts',(6.83411585527522,-3.98483361329514,129.465232352156));
#54996=CARTESIAN_POINT('Ctrl Pts',(6.82564832217963,-3.99931008925879,129.464559385364));
#54997=CARTESIAN_POINT('Ctrl Pts',(6.82264671667153,-4.00442854697359,129.464321501119));
#54998=CARTESIAN_POINT('Ctrl Pts',(6.81694308592173,-4.01412957738808,129.463870745154));
#54999=CARTESIAN_POINT('Ctrl Pts',(6.8142421923661,-4.0187128094301,129.463657831735));
#55000=CARTESIAN_POINT('Ctrl Pts',(6.80798760732958,-4.02930197904195,129.463166016779));
#55001=CARTESIAN_POINT('Ctrl Pts',(6.80443058532779,-4.03530594994363,129.462887238866));
#55002=CARTESIAN_POINT('Ctrl Pts',(6.79444293932496,-4.05211354913787,129.462107036371));
#55003=CARTESIAN_POINT('Ctrl Pts',(6.78799448524417,-4.0629065877836,129.461606273661));
#55004=CARTESIAN_POINT('Ctrl Pts',(6.75076134636459,-4.12488912559466,129.458731849942));
#55005=CARTESIAN_POINT('Ctrl Pts',(6.71942301739954,-4.17574467222141,129.456378840039));
#55006=CARTESIAN_POINT('Ctrl Pts',(6.62796946964134,-4.32045875950526,129.449695682521));
#55007=CARTESIAN_POINT('Ctrl Pts',(6.56644195907552,-4.4134096102045,129.445418581052));
#55008=CARTESIAN_POINT('Ctrl Pts',(6.3816689699917,-4.68012761580694,129.433164291611));
#55009=CARTESIAN_POINT('Ctrl Pts',(6.2533426760697,-4.85025826413037,129.425373838104));
#55010=CARTESIAN_POINT('Ctrl Pts',(6.04927732170652,-5.09921762141308,129.413868457297));
#55011=CARTESIAN_POINT('Ctrl Pts',(5.97852144814181,-5.18199366637929,129.410023598275));
#55012=CARTESIAN_POINT('Ctrl Pts',(5.85666426283911,-5.31873303507879,129.403610540762));
#55013=CARTESIAN_POINT('Ctrl Pts',(5.80647125119308,-5.37348389081887,129.401025310812));
#55014=CARTESIAN_POINT('Ctrl Pts',(5.73447987952777,-5.44982582348347,129.397387155292));
#55015=CARTESIAN_POINT('Ctrl Pts',(5.71331582082688,-5.47200907647653,129.396325896581));
#55016=CARTESIAN_POINT('Ctrl Pts',(5.67239885792624,-5.51440030161698,129.394289106614));
#55017=CARTESIAN_POINT('Ctrl Pts',(5.65266559469655,-5.5346265608705,129.393313387513));
#55018=CARTESIAN_POINT('Ctrl Pts',(5.26090063342465,-5.93189818182047,129.374064368405));
#55019=CARTESIAN_POINT('Ctrl Pts',(4.8520701733755,-6.27071072240029,129.356212789774));
#55020=CARTESIAN_POINT('Ctrl Pts',(4.39788981038583,-6.57592550202536,129.335461655056));
#55021=CARTESIAN_POINT('Ctrl Pts',(4.38324372108593,-6.58569703731295,129.334791500982));
#55022=CARTESIAN_POINT('Ctrl Pts',(4.35852925151662,-6.60206700003122,129.333658794064));
#55023=CARTESIAN_POINT('Ctrl Pts',(4.34847816834512,-6.60869151393633,129.333197620576));
#55024=CARTESIAN_POINT('Ctrl Pts',(4.26209319297185,-6.66534412411727,129.329229279156));
#55025=CARTESIAN_POINT('Ctrl Pts',(4.18492255806142,-6.71406531869149,129.32564926758));
#55026=CARTESIAN_POINT('Ctrl Pts',(4.09667450041951,-6.76766745399532,129.321511150001));
#55027=CARTESIAN_POINT('Ctrl Pts',(4.08641375227872,-6.7738679772388,129.3210294072));
#55028=CARTESIAN_POINT('Ctrl Pts',(4.07132982387217,-6.78293638129537,129.320320382868));
#55029=CARTESIAN_POINT('Ctrl Pts',(4.06651759015735,-6.78582251286835,129.320094058331));
#55030=CARTESIAN_POINT('Ctrl Pts',(4.05796264947474,-6.79094096032369,129.319691495099));
#55031=CARTESIAN_POINT('Ctrl Pts',(4.05422115726168,-6.79317531048874,129.319515361595));
#55032=CARTESIAN_POINT('Ctrl Pts',(4.04650864681758,-6.79777243830464,129.319152141992));
#55033=CARTESIAN_POINT('Ctrl Pts',(4.04253740141914,-6.80013483026173,129.318965036301));
#55034=CARTESIAN_POINT('Ctrl Pts',(4.03247077087613,-6.80611127569958,129.318490546266));
#55035=CARTESIAN_POINT('Ctrl Pts',(4.02637260348466,-6.80972061634238,129.318202924359));
#55036=CARTESIAN_POINT('Ctrl Pts',(4.01303271792971,-6.81759195112436,129.31757335311));
#55037=CARTESIAN_POINT('Ctrl Pts',(4.00578904836507,-6.82185060715984,129.317231238989));
#55038=CARTESIAN_POINT('Ctrl Pts',(3.984889500332,-6.83409298249173,129.316243469407));
#55039=CARTESIAN_POINT('Ctrl Pts',(3.97121649103379,-6.84204726668123,129.315596390136));
#55040=CARTESIAN_POINT('Ctrl Pts',(3.92507886680906,-6.86870297690741,129.313410254035));
#55041=CARTESIAN_POINT('Ctrl Pts',(3.89250557087163,-6.887214604848,129.311862416122));
#55042=CARTESIAN_POINT('Ctrl Pts',(3.75518395834791,-6.96397005377833,129.305322151524));
#55043=CARTESIAN_POINT('Ctrl Pts',(3.64925306414891,-7.020059534667,129.300240884743));
#55044=CARTESIAN_POINT('Ctrl Pts',(3.29646283485409,-7.19671561998329,129.283287143524));
#55045=CARTESIAN_POINT('Ctrl Pts',(3.04459970065764,-7.30683158574461,129.271140629791));
#55046=CARTESIAN_POINT('Ctrl Pts',(2.23340153544673,-7.61225475989284,129.232694668417));
#55047=CARTESIAN_POINT('Ctrl Pts',(1.65754935171165,-7.75803801676341,129.206541513892));
#55048=CARTESIAN_POINT('Ctrl Pts',(0.921091465282835,-7.85864757810112,
129.175609146083));
#55049=CARTESIAN_POINT('Ctrl Pts',(0.770826777392061,-7.87480663680732,
129.169413399779));
#55050=CARTESIAN_POINT('Ctrl Pts',(0.595787264230321,-7.88857132780115,
129.162317635424));
#55051=CARTESIAN_POINT('Ctrl Pts',(0.571378065165727,-7.89037687147383,
129.16133084789));
#55052=CARTESIAN_POINT('Ctrl Pts',(0.534988279795762,-7.89289886986167,
129.159863660815));
#55053=CARTESIAN_POINT('Ctrl Pts',(0.52301387961296,-7.89370138225325,129.159381504125));
#55054=CARTESIAN_POINT('Ctrl Pts',(0.50165419328376,-7.89508407105961,129.158522559316));
#55055=CARTESIAN_POINT('Ctrl Pts',(0.492269619898394,-7.89567476790448,
129.158145558017));
#55056=CARTESIAN_POINT('Ctrl Pts',(0.472564442680712,-7.89687981035193,
129.157354750841));
#55057=CARTESIAN_POINT('Ctrl Pts',(0.462243636710388,-7.89749065923035,
129.156941016903));
#55058=CARTESIAN_POINT('Ctrl Pts',(0.4352207889315,-7.89903688412155,129.155858943012));
#55059=CARTESIAN_POINT('Ctrl Pts',(0.418516899953101,-7.89993952123505,
129.15519127125));
#55060=CARTESIAN_POINT('Ctrl Pts',(0.34508054095335,-7.90367427224265,129.152261190549));
#55061=CARTESIAN_POINT('Ctrl Pts',(0.288320950494298,-7.90594831276918,
129.150010282648));
#55062=CARTESIAN_POINT('Ctrl Pts',(0.0248547349322873,-7.91366281803928,
129.139624025146));
#55063=CARTESIAN_POINT('Ctrl Pts',(-0.181994581528782,-7.91160919168103,
129.131649478971));
#55064=CARTESIAN_POINT('Ctrl Pts',(-0.50846275614695,-7.89555600854718,
129.119278936484));
#55065=CARTESIAN_POINT('Ctrl Pts',(-0.628244752409664,-7.88692895884645,
129.114785522644));
#55066=CARTESIAN_POINT('Ctrl Pts',(-0.832733076930153,-7.86751280488607,
129.107168119196));
#55067=CARTESIAN_POINT('Ctrl Pts',(-0.917545013881621,-7.85807314090975,
129.104024560447));
#55068=CARTESIAN_POINT('Ctrl Pts',(-1.06895012503899,-7.83873691797351,
129.098429753467));
#55069=CARTESIAN_POINT('Ctrl Pts',(-1.1356007192113,-7.82935897305758,129.095972757889));
#55070=CARTESIAN_POINT('Ctrl Pts',(-1.25714099059186,-7.81067320804819,
129.091496724122));
#55071=CARTESIAN_POINT('Ctrl Pts',(-1.31206748912966,-7.80163433965268,
129.089475559399));
#55072=CARTESIAN_POINT('Ctrl Pts',(-1.4899928020783,-7.77042225616164,129.082926607717));
#55073=CARTESIAN_POINT('Ctrl Pts',(-1.61256261272887,-7.74591392162776,
129.078412733197));
#55074=CARTESIAN_POINT('Ctrl Pts',(-2.05378137362495,-7.6467634549912,129.062055053318));
#55075=CARTESIAN_POINT('Ctrl Pts',(-2.36829112373877,-7.55527562981762,
129.050198239783));
#55076=CARTESIAN_POINT('Ctrl Pts',(-2.82376859410245,-7.39153819703612,
129.031823584912));
#55077=CARTESIAN_POINT('Ctrl Pts',(-2.96970486199796,-7.33412264768154,
129.025743108026));
#55078=CARTESIAN_POINT('Ctrl Pts',(-3.12658481318704,-7.26695127595329,
129.018909481708));
#55079=CARTESIAN_POINT('Ctrl Pts',(-3.13932289118435,-7.26145751364896,
129.01835244914));
#55080=CARTESIAN_POINT('Ctrl Pts',(-3.15715369779857,-7.25371163856656,
129.01756959496));
#55081=CARTESIAN_POINT('Ctrl Pts',(-3.16225864733913,-7.25148758904731,
129.017345105355));
#55082=CARTESIAN_POINT('Ctrl Pts',(-3.17109868464323,-7.24762518121592,
129.01695573737));
#55083=CARTESIAN_POINT('Ctrl Pts',(-3.17483486542168,-7.24598931908854,
129.016790979019));
#55084=CARTESIAN_POINT('Ctrl Pts',(-3.18233818183134,-7.24269712408581,
129.016459703236));
#55085=CARTESIAN_POINT('Ctrl Pts',(-3.18610529319005,-7.24104073979634,
129.01629318334));
#55086=CARTESIAN_POINT('Ctrl Pts',(-3.19503256705952,-7.23710713672802,
129.015898088563));
#55087=CARTESIAN_POINT('Ctrl Pts',(-3.20019158523816,-7.23482733937533,
129.015669387445));
#55088=CARTESIAN_POINT('Ctrl Pts',(-3.21594190812643,-7.22784704556899,
129.014970002825));
#55089=CARTESIAN_POINT('Ctrl Pts',(-3.22652529393118,-7.22312880931818,
129.014498439677));
#55090=CARTESIAN_POINT('Ctrl Pts',(-3.25091391035351,-7.21219169231584,
129.013407957208));
#55091=CARTESIAN_POINT('Ctrl Pts',(-3.26471169690569,-7.20595641051553,
129.012788203914));
#55092=CARTESIAN_POINT('Ctrl Pts',(-3.30987569331427,-7.18539025451225,
129.010750098722));
#55093=CARTESIAN_POINT('Ctrl Pts',(-3.34116575711271,-7.17089405819668,
129.009322975773));
#55094=CARTESIAN_POINT('Ctrl Pts',(-3.44542471623478,-7.12176196274324,
129.004515166055));
#55095=CARTESIAN_POINT('Ctrl Pts',(-3.51795535294535,-7.08621438474711,
129.001085133643));
#55096=CARTESIAN_POINT('Ctrl Pts',(-3.72555200901987,-6.98049765596603,
128.991047145746));
#55097=CARTESIAN_POINT('Ctrl Pts',(-3.85915065363965,-6.90753485709335,
128.984313902631));
#55098=CARTESIAN_POINT('Ctrl Pts',(-4.8020564877276,-6.35668629550347,128.935231515196));
#55099=CARTESIAN_POINT('Ctrl Pts',(-5.52289895765142,-5.74156978568193,
128.890439753823));
#55100=CARTESIAN_POINT('Ctrl Pts',(-6.15415533931288,-4.97125639215908,
128.849629002045));
#55101=CARTESIAN_POINT('Ctrl Pts',(-6.18897452030067,-4.92784056284967,
128.847367171728));
#55102=CARTESIAN_POINT('Ctrl Pts',(-6.23056801416275,-4.87484159219013,
128.844651692421));
#55103=CARTESIAN_POINT('Ctrl Pts',(-6.23778238747645,-4.86560676751734,
128.844180188424));
#55104=CARTESIAN_POINT('Ctrl Pts',(-6.24957389195036,-4.85044361505746,
128.84340870318));
#55105=CARTESIAN_POINT('Ctrl Pts',(-6.25416315872756,-4.8445247732076,128.843108230985));
#55106=CARTESIAN_POINT('Ctrl Pts',(-6.26237244798331,-4.83390603094904,
128.842570367938));
#55107=CARTESIAN_POINT('Ctrl Pts',(-6.26599559911505,-4.82920856304417,
128.842332850796));
#55108=CARTESIAN_POINT('Ctrl Pts',(-6.27366293469632,-4.81924459568909,
128.841829932976));
#55109=CARTESIAN_POINT('Ctrl Pts',(-6.27770578057585,-4.8139770693335,128.841564586344));
#55110=CARTESIAN_POINT('Ctrl Pts',(-6.28845733872629,-4.79993201519237,
128.840858473963));
#55111=CARTESIAN_POINT('Ctrl Pts',(-6.29515431560334,-4.79114549930291,
128.84041818067));
#55112=CARTESIAN_POINT('Ctrl Pts',(-6.3262598330114,-4.75015686839619,128.838370944721));
#55113=CARTESIAN_POINT('Ctrl Pts',(-6.35044003915959,-4.71778180092387,
128.836773168659));
#55114=CARTESIAN_POINT('Ctrl Pts',(-6.52854172573438,-4.47546966424367,
128.824955111149));
#55115=CARTESIAN_POINT('Ctrl Pts',(-6.67227129524531,-4.25822686897696,
128.815146732692));
#55116=CARTESIAN_POINT('Ctrl Pts',(-7.16149193801664,-3.43300768199062,
128.780242608167));
#55117=CARTESIAN_POINT('Ctrl Pts',(-7.43665934655047,-2.78720803995153,
128.757676826845));
#55118=CARTESIAN_POINT('Ctrl Pts',(-7.62986155918095,-2.09038704010946,
128.73236860291));
#55119=CARTESIAN_POINT('Ctrl Pts',(-7.63621363906149,-2.06706232111607,
128.731520024128));
#55120=CARTESIAN_POINT('Ctrl Pts',(-7.68145996812508,-1.89786347245794,
128.725351856212));
#55121=CARTESIAN_POINT('Ctrl Pts',(-7.71627710689242,-1.75093618387331,
128.719928564604));
#55122=CARTESIAN_POINT('Ctrl Pts',(-7.75115366938685,-1.58239851251141,
128.713546804146));
#55123=CARTESIAN_POINT('Ctrl Pts',(-7.75535617579685,-1.56167180775897,
128.712759220317));
#55124=CARTESIAN_POINT('Ctrl Pts',(-7.76385738555075,-1.5188632522641,128.711126440375));
#55125=CARTESIAN_POINT('Ctrl Pts',(-7.76814510519658,-1.49677944015832,
128.710280779733));
#55126=CARTESIAN_POINT('Ctrl Pts',(-7.77419697540246,-1.46488285624314,
128.709054155996));
#55127=CARTESIAN_POINT('Ctrl Pts',(-7.77603688367703,-1.45508445691838,
128.708676638923));
#55128=CARTESIAN_POINT('Ctrl Pts',(-7.77981816489373,-1.43473530957747,
128.707891104335));
#55129=CARTESIAN_POINT('Ctrl Pts',(-7.78175660734259,-1.42418404351131,
128.707482951751));
#55130=CARTESIAN_POINT('Ctrl Pts',(-7.78529349746118,-1.40470934399531,
128.706728008242));
#55131=CARTESIAN_POINT('Ctrl Pts',(-7.78689808210129,-1.39578703270446,
128.706381509813));
#55132=CARTESIAN_POINT('Ctrl Pts',(-7.78999616521076,-1.378388487765,128.70570459182));
#55133=CARTESIAN_POINT('Ctrl Pts',(-7.79149117478306,-1.36991253355285,
128.705374246068));
#55134=CARTESIAN_POINT('Ctrl Pts',(-7.79482982655388,-1.35080178897157,
128.704628086421));
#55135=CARTESIAN_POINT('Ctrl Pts',(-7.79666553954444,-1.34016564673749,
128.704211882274));
#55136=CARTESIAN_POINT('Ctrl Pts',(-7.81081944440454,-1.25714436603091,
128.700955717339));
#55137=CARTESIAN_POINT('Ctrl Pts',(-7.82215074580334,-1.18459673614096,
128.698066172737));
#55138=CARTESIAN_POINT('Ctrl Pts',(-7.83379587279434,-1.10256617792574,
128.694739142725));
#55139=CARTESIAN_POINT('Ctrl Pts',(-7.83510478100933,-1.0932259704374,128.69435944617));
#55140=CARTESIAN_POINT('Ctrl Pts',(-7.83698441685395,-1.0796363430689,128.693805706632));
#55141=CARTESIAN_POINT('Ctrl Pts',(-7.83756840187929,-1.07538873390447,
128.693632444242));
#55142=CARTESIAN_POINT('Ctrl Pts',(-7.83859400836142,-1.06788378460026,
128.693325984708));
#55143=CARTESIAN_POINT('Ctrl Pts',(-7.83903705233508,-1.06462664691495,
128.693192872231));
#55144=CARTESIAN_POINT('Ctrl Pts',(-7.83995417095694,-1.05785263174646,
128.692915805569));
#55145=CARTESIAN_POINT('Ctrl Pts',(-7.84042790936712,-1.0543357108317,128.692771831662));
#55146=CARTESIAN_POINT('Ctrl Pts',(-7.84138198588751,-1.04721667166443,
128.692480140976));
#55147=CARTESIAN_POINT('Ctrl Pts',(-7.84186220867543,-1.04361453903094,
128.692332417475));
#55148=CARTESIAN_POINT('Ctrl Pts',(-7.8430327658275,-1.03478780781344,128.691970111676));
#55149=CARTESIAN_POINT('Ctrl Pts',(-7.84372036102039,-1.02956285427189,
128.691755370107));
#55150=CARTESIAN_POINT('Ctrl Pts',(-7.84559523237534,-1.01520503777121,
128.691164524982));
#55151=CARTESIAN_POINT('Ctrl Pts',(-7.84677177881892,-1.00607080702518,
128.690787804594));
#55152=CARTESIAN_POINT('Ctrl Pts',(-7.88984058046698,-0.667030463361971,
128.676774516862));
#55153=CARTESIAN_POINT('Ctrl Pts',(-7.9109004823013,-0.33484439240435,128.66198909247));
#55154=CARTESIAN_POINT('Ctrl Pts',(-7.91099964813049,-0.00235950828826645,
128.646812588333));
#55155=CARTESIAN_POINT('',(-7.89935487361401,-0.000512643485807648,126.642299148188));
#55156=CARTESIAN_POINT('Ctrl Pts',(-7.91099958186279,-0.00257211328256086,
128.642116733665));
#55157=CARTESIAN_POINT('Ctrl Pts',(-7.91106172871082,0.188571757426559,
128.634395854378));
#55158=CARTESIAN_POINT('Ctrl Pts',(-7.90419210364439,0.38000650194112,128.62667497509));
#55159=CARTESIAN_POINT('Ctrl Pts',(-7.89035363924545,0.571174620975065,
128.618954095803));
#55160=CARTESIAN_POINT('Ctrl Pts',(-7.87652865224551,0.762156559740664,
128.611240735946));
#55161=CARTESIAN_POINT('Ctrl Pts',(-7.85574836118812,0.952872032041322,
128.603527376088));
#55162=CARTESIAN_POINT('Ctrl Pts',(-7.82802767564603,1.14276144024897,128.595814016231));
#55163=CARTESIAN_POINT('Ctrl Pts',(-7.8003282871574,1.33250496155664,128.58810658234));
#55164=CARTESIAN_POINT('Ctrl Pts',(-7.76569917123154,1.52142332597649,128.580399148449));
#55165=CARTESIAN_POINT('Ctrl Pts',(-7.72420720923037,1.7089599143554,128.572691714558));
#55166=CARTESIAN_POINT('Ctrl Pts',(-7.68273860412503,1.89639093355058,128.56498861938));
#55167=CARTESIAN_POINT('Ctrl Pts',(-7.63441492322061,2.08244137308628,128.557285524202));
#55168=CARTESIAN_POINT('Ctrl Pts',(-7.57935450900709,2.26656264568044,128.549582429024));
#55169=CARTESIAN_POINT('Ctrl Pts',(-7.52430732046374,2.45063969181429,128.541881184152));
#55170=CARTESIAN_POINT('Ctrl Pts',(-7.46252671801311,2.63278814539991,128.53417993928));
#55171=CARTESIAN_POINT('Ctrl Pts',(-7.39418155640331,2.81247224180881,128.526478694408));
#55172=CARTESIAN_POINT('Ctrl Pts',(-7.32584333515808,2.99213809152539,128.518778231587));
#55173=CARTESIAN_POINT('Ctrl Pts',(-7.25094200948829,3.16933974335435,128.511077768767));
#55174=CARTESIAN_POINT('Ctrl Pts',(-7.16969543935455,3.34355922736515,128.503377305946));
#55175=CARTESIAN_POINT('Ctrl Pts',(-7.08844202745983,3.51779338237148,128.495676194671));
#55176=CARTESIAN_POINT('Ctrl Pts',(-7.00084246024951,3.68904454119845,128.487975083396));
#55177=CARTESIAN_POINT('Ctrl Pts',(-6.90716162491653,3.85681724836431,128.480273972121));
#55178=CARTESIAN_POINT('Ctrl Pts',(-6.81345549385595,4.0246352575675,128.472570781389));
#55179=CARTESIAN_POINT('Ctrl Pts',(-6.71366500237783,4.18897262927833,128.464867590657));
#55180=CARTESIAN_POINT('Ctrl Pts',(-6.60809962107566,4.34936091833499,128.457164399926));
#55181=CARTESIAN_POINT('Ctrl Pts',(-6.50242721631475,4.50991181097648,128.449453399606));
#55182=CARTESIAN_POINT('Ctrl Pts',(-6.39096842749255,4.6665053217451,128.441742399287));
#55183=CARTESIAN_POINT('Ctrl Pts',(-6.27407502337237,4.81870351869618,128.434031398967));
#55184=CARTESIAN_POINT('Ctrl Pts',(-6.15712015557712,4.97098174292163,128.42631634413));
#55185=CARTESIAN_POINT('Ctrl Pts',(-6.03472521100803,5.11885977170499,128.418601289292));
#55186=CARTESIAN_POINT('Ctrl Pts',(-5.90728030952362,5.26193503805534,128.410886234455));
#55187=CARTESIAN_POINT('Ctrl Pts',(-5.77965213476975,5.40521605505981,128.403160084914));
#55188=CARTESIAN_POINT('Ctrl Pts',(-5.64695974637582,5.54368025222585,128.395433935374));
#55189=CARTESIAN_POINT('Ctrl Pts',(-5.50962884540655,5.6769631834163,128.387707785833));
#55190=CARTESIAN_POINT('Ctrl Pts',(-5.39040784340672,5.79267002356551,128.381000487743));
#55191=CARTESIAN_POINT('Ctrl Pts',(-5.26769167971134,5.90447255479126,128.374293189652));
#55192=CARTESIAN_POINT('Ctrl Pts',(-5.14177698783451,6.01215854809032,128.367585891562));
#55193=CARTESIAN_POINT('Ctrl Pts',(-4.99326218119857,6.13917283239523,128.359674717226));
#55194=CARTESIAN_POINT('Ctrl Pts',(-4.83983861260918,6.26085156460908,128.35176354289));
#55195=CARTESIAN_POINT('Ctrl Pts',(-4.68192541788834,6.37679350311197,128.343852368553));
#55196=CARTESIAN_POINT('Ctrl Pts',(-4.52418342157298,6.4926097455004,128.335949770957));
#55197=CARTESIAN_POINT('Ctrl Pts',(-4.36196176958607,6.60270138012032,128.328047173361));
#55198=CARTESIAN_POINT('Ctrl Pts',(-4.19571460999561,6.70670559302176,128.320144575765));
#55199=CARTESIAN_POINT('Ctrl Pts',(-4.02961682378772,6.81061635794419,128.312249078667));
#55200=CARTESIAN_POINT('Ctrl Pts',(-3.85950102570916,6.90845041525919,128.30435358157));
#55201=CARTESIAN_POINT('Ctrl Pts',(-3.68585267577465,6.9998865028288,128.296458084472));
#55202=CARTESIAN_POINT('Ctrl Pts',(-3.51232812523016,7.09125740272533,128.288568216324));
#55203=CARTESIAN_POINT('Ctrl Pts',(-3.33527634435184,7.17623926057323,128.280678348175));
#55204=CARTESIAN_POINT('Ctrl Pts',(-3.15521012463939,7.25455512553134,128.272788480027));
#55205=CARTESIAN_POINT('Ctrl Pts',(-2.97523887235613,7.33282968648267,128.264902773017));
#55206=CARTESIAN_POINT('Ctrl Pts',(-2.79225666464164,7.40444512278129,128.257017066007));
#55207=CARTESIAN_POINT('Ctrl Pts',(-2.60679940000116,7.469171164738,128.249131358998));
#55208=CARTESIAN_POINT('Ctrl Pts',(-2.42140554399758,7.53387507658241,128.241248348145));
#55209=CARTESIAN_POINT('Ctrl Pts',(-2.23353864282103,7.59169417522488,128.233365337292));
#55210=CARTESIAN_POINT('Ctrl Pts',(-2.0437532717983,7.64244683095759,128.22548232644));
#55211=CARTESIAN_POINT('Ctrl Pts',(-1.85396506851317,7.69320024409768,128.217599197945));
#55212=CARTESIAN_POINT('Ctrl Pts',(-1.66225866908416,7.73688690636788,128.20971606945));
#55213=CARTESIAN_POINT('Ctrl Pts',(-1.46920302329791,7.77337529496243,128.201832940955));
#55214=CARTESIAN_POINT('Ctrl Pts',(-1.27613544068857,7.80986593967044,128.193949325039));
#55215=CARTESIAN_POINT('Ctrl Pts',(-1.08171878440958,7.83915735916659,128.186065709122));
#55216=CARTESIAN_POINT('Ctrl Pts',(-0.886531428151984,7.86116931676826,
128.178182093206));
#55217=CARTESIAN_POINT('Ctrl Pts',(-0.691299193308703,7.88318633548426,
128.170296664644));
#55218=CARTESIAN_POINT('Ctrl Pts',(-0.495296248158198,7.89792051846848,
128.162411236081));
#55219=CARTESIAN_POINT('Ctrl Pts',(-0.299105555518819,7.90534356411268,
128.154525807519));
#55220=CARTESIAN_POINT('Ctrl Pts',(-0.102836774566898,7.91276956429617,
128.146637240379));
#55221=CARTESIAN_POINT('Ctrl Pts',(0.0936195583692437,7.91287861566962,
128.138748673239));
#55222=CARTESIAN_POINT('Ctrl Pts',(0.289680765627241,7.90569453331114,128.130860106098));
#55223=CARTESIAN_POINT('Ctrl Pts',(0.485950624630045,7.89850280552733,128.122963143808));
#55224=CARTESIAN_POINT('Ctrl Pts',(0.681824173259923,7.88400245382682,128.115066181517));
#55225=CARTESIAN_POINT('Ctrl Pts',(0.876723026443754,7.86226924843606,128.107169219226));
#55226=CARTESIAN_POINT('Ctrl Pts',(1.0717407419997,7.84052278868128,128.099267440839));
#55227=CARTESIAN_POINT('Ctrl Pts',(1.26578223682056,7.81153473195795,128.091365662452));
#55228=CARTESIAN_POINT('Ctrl Pts',(1.45827932920525,7.77543197501031,128.083463884065));
#55229=CARTESIAN_POINT('Ctrl Pts',(1.65102538679948,7.73928252473168,128.07555188595));
#55230=CARTESIAN_POINT('Ctrl Pts',(1.84222271693521,7.69600007051652,128.067639887835));
#55231=CARTESIAN_POINT('Ctrl Pts',(2.03131720799035,7.64576166255019,128.05972788972));
#55232=CARTESIAN_POINT('Ctrl Pts',(2.1105458553854,7.62471228618686,128.056412843865));
#55233=CARTESIAN_POINT('Ctrl Pts',(2.18940556887713,7.60244236409492,128.05309779801));
#55234=CARTESIAN_POINT('Ctrl Pts',(2.26785664693886,7.5789674249818,128.049782752154));
#55235=CARTESIAN_POINT('Ctrl Pts',(2.45507563422432,7.52294583246921,128.041871585818));
#55236=CARTESIAN_POINT('Ctrl Pts',(2.64046920377942,7.45990767774175,128.033960419481));
#55237=CARTESIAN_POINT('Ctrl Pts',(2.82347302936848,7.38998789257661,128.026049253144));
#55238=CARTESIAN_POINT('Ctrl Pts',(3.00627848460446,7.32014389824494,128.018146662261));
#55239=CARTESIAN_POINT('Ctrl Pts',(3.1866990363679,7.24343325359218,128.010244071378));
#55240=CARTESIAN_POINT('Ctrl Pts',(3.36418369101412,7.16004113766915,128.002341480496));
#55241=CARTESIAN_POINT('Ctrl Pts',(3.54150890401893,7.07672393625562,127.99444598883));
#55242=CARTESIAN_POINT('Ctrl Pts',(3.715903163777,6.98673736627402,127.986550497164));
#55243=CARTESIAN_POINT('Ctrl Pts',(3.8868334398217,6.89031543625427,127.978655005498));
#55244=CARTESIAN_POINT('Ctrl Pts',(4.05764188186214,6.7939622329113,127.970765141503));
#55245=CARTESIAN_POINT('Ctrl Pts',(4.22499096021781,6.69118297700458,127.962875277508));
#55246=CARTESIAN_POINT('Ctrl Pts',(4.38837008345159,6.58225865570984,127.954985413513));
#55247=CARTESIAN_POINT('Ctrl Pts',(4.55166306643892,6.4733917638326,127.947099709381));
#55248=CARTESIAN_POINT('Ctrl Pts',(4.7109899789148,6.35838645340526,127.93921400525));
#55249=CARTESIAN_POINT('Ctrl Pts',(4.86586694901607,6.23756842322976,127.931328301118));
#55250=CARTESIAN_POINT('Ctrl Pts',(5.02069099100115,6.11679168176707,127.92344529187));
#55251=CARTESIAN_POINT('Ctrl Pts',(5.17106784993921,5.99020639148181,127.915562282623));
#55252=CARTESIAN_POINT('Ctrl Pts',(5.31654442003831,5.85818030020923,127.907679273375));
#55253=CARTESIAN_POINT('Ctrl Pts',(5.46202319627846,5.72615220677108,127.899796144582));
#55254=CARTESIAN_POINT('Ctrl Pts',(5.60260127418626,5.58868337294279,127.89191301579));
#55255=CARTESIAN_POINT('Ctrl Pts',(5.73785987772008,5.44618077405168,127.884029886997));
#55256=CARTESIAN_POINT('Ctrl Pts',(5.873126864792,5.30366934262839,127.876146269595));
#55257=CARTESIAN_POINT('Ctrl Pts',(6.00307348253585,5.15612377428628,127.868262652194));
#55258=CARTESIAN_POINT('Ctrl Pts',(6.12731895789229,5.00398674940829,127.860379034793));
#55259=CARTESIAN_POINT('Ctrl Pts',(6.2515930191803,4.85181472141595,127.852493603558));
#55260=CARTESIAN_POINT('Ctrl Pts',(6.37016310612351,4.69504939904889,127.844608172324));
#55261=CARTESIAN_POINT('Ctrl Pts',(6.48268961331282,4.53416545545551,127.836722741089));
#55262=CARTESIAN_POINT('Ctrl Pts',(6.59526092552886,4.37321745220568,127.828834170088));
#55263=CARTESIAN_POINT('Ctrl Pts',(6.70178366549696,4.20814784245497,127.820945599088));
#55264=CARTESIAN_POINT('Ctrl Pts',(6.80196218870793,4.03945929344358,127.813057028087));
#55265=CARTESIAN_POINT('Ctrl Pts',(6.90224734612939,3.8705911852845,127.805160060161));
#55266=CARTESIAN_POINT('Ctrl Pts',(6.99617462204756,3.69809674021043,127.797263092235));
#55267=CARTESIAN_POINT('Ctrl Pts',(7.08349436800469,3.52250316372403,127.789366124309));
#55268=CARTESIAN_POINT('Ctrl Pts',(7.17086737866326,3.34680247584693,127.781464339264));
#55269=CARTESIAN_POINT('Ctrl Pts',(7.25162468227645,3.16799920115032,127.773562554219));
#55270=CARTESIAN_POINT('Ctrl Pts',(7.32556513212973,2.98663966606704,127.765660769173));
#55271=CARTESIAN_POINT('Ctrl Pts',(7.39960122658241,2.80504553598045,127.757748762888));
#55272=CARTESIAN_POINT('Ctrl Pts',(7.46680273664315,2.6208888638439,127.749836756604));
#55273=CARTESIAN_POINT('Ctrl Pts',(7.52701829413885,2.43473131981726,127.741924750319));
#55274=CARTESIAN_POINT('Ctrl Pts',(7.5522479675282,2.35673330352235,127.738609704461));
#55275=CARTESIAN_POINT('Ctrl Pts',(7.57625185913851,2.27838416024166,127.735294658604));
#55276=CARTESIAN_POINT('Ctrl Pts',(7.59902151349563,2.19972567322168,127.731979612747));
#55277=CARTESIAN_POINT('Ctrl Pts',(7.65287352100478,2.0136922197831,127.724139270877));
#55278=CARTESIAN_POINT('Ctrl Pts',(7.69997090489175,1.82540023104041,127.716298929008));
#55279=CARTESIAN_POINT('Ctrl Pts',(7.74011829435845,1.63538673999076,127.708458587139));
#55280=CARTESIAN_POINT('Ctrl Pts',(7.78022079784872,1.44558568967996,127.700627011005));
#55281=CARTESIAN_POINT('Ctrl Pts',(7.81338870739113,1.25406730994041,127.692795434872));
#55282=CARTESIAN_POINT('Ctrl Pts',(7.83947589528888,1.06138526802695,127.684963858738));
#55283=CARTESIAN_POINT('Ctrl Pts',(7.86553898941218,0.868881184645354,127.677139515743));
#55284=CARTESIAN_POINT('Ctrl Pts',(7.88453433858239,0.675215925305001,127.669315172747));
#55285=CARTESIAN_POINT('Ctrl Pts',(7.89636645732686,0.480955061937415,127.661490829751));
#55286=CARTESIAN_POINT('Ctrl Pts',(7.90818994755206,0.28683586242901,127.653672192622));
#55287=CARTESIAN_POINT('Ctrl Pts',(7.91286059039629,0.0921222733201361,
127.645853555494));
#55288=CARTESIAN_POINT('Ctrl Pts',(7.91033447821782,-0.102613072843991,
127.638034918365));
#55289=CARTESIAN_POINT('Ctrl Pts',(7.90780971744413,-0.297244240626218,
127.630220464005));
#55290=CARTESIAN_POINT('Ctrl Pts',(7.89809587570351,-0.491896791618777,
127.622406009645));
#55291=CARTESIAN_POINT('Ctrl Pts',(7.88120108631204,-0.685995945406346,
127.614591555286));
#55292=CARTESIAN_POINT('Ctrl Pts',(7.86431205381443,-0.880028959971861,
127.606779763698));
#55293=CARTESIAN_POINT('Ctrl Pts',(7.84024697948718,-1.07350860319827,127.598967972111));
#55294=CARTESIAN_POINT('Ctrl Pts',(7.8090660238239,-1.26586288181586,127.591156180524));
#55295=CARTESIAN_POINT('Ctrl Pts',(7.77788360884144,-1.45822616292499,127.583344023333));
#55296=CARTESIAN_POINT('Ctrl Pts',(7.73958469440379,-1.64946362564282,127.575531866141));
#55297=CARTESIAN_POINT('Ctrl Pts',(7.69428104737915,-1.83901064813178,127.56771970895));
#55298=CARTESIAN_POINT('Ctrl Pts',(7.64897369674031,-2.02857316626157,127.559906913107));
#55299=CARTESIAN_POINT('Ctrl Pts',(7.59666055379395,-2.21644462644084,127.552094117265));
#55300=CARTESIAN_POINT('Ctrl Pts',(7.53750401571364,-2.40207289920618,127.544281321422));
#55301=CARTESIAN_POINT('Ctrl Pts',(7.47833223243184,-2.58774901013972,127.536466512148));
#55302=CARTESIAN_POINT('Ctrl Pts',(7.41231364743956,-2.77118044686703,127.528651702874));
#55303=CARTESIAN_POINT('Ctrl Pts',(7.33965986070732,-2.95183233418192,127.5208368936));
#55304=CARTESIAN_POINT('Ctrl Pts',(7.26697456525496,-3.13256256716894,127.513018695175));
#55305=CARTESIAN_POINT('Ctrl Pts',(7.18764846688821,-3.3105105234454,127.50520049675));
#55306=CARTESIAN_POINT('Ctrl Pts',(7.10194048161173,-3.48516318063366,127.497382298325));
#55307=CARTESIAN_POINT('Ctrl Pts',(7.01613273270517,-3.6600191325678,127.489554999559));
#55308=CARTESIAN_POINT('Ctrl Pts',(6.92392841514536,-3.83157180867922,127.481727700794));
#55309=CARTESIAN_POINT('Ctrl Pts',(6.8256319507697,-3.99933362857262,127.473900402028));
#55310=CARTESIAN_POINT('Ctrl Pts',(6.72727131806158,-4.1672049640656,127.46606799357));
#55311=CARTESIAN_POINT('Ctrl Pts',(6.62281080130682,-4.33128021613375,127.458235585112));
#55312=CARTESIAN_POINT('Ctrl Pts',(6.51259701665135,-4.4911024368972,127.450403176654));
#55313=CARTESIAN_POINT('Ctrl Pts',(6.40222505968386,-4.65115402506918,127.442559527586));
#55314=CARTESIAN_POINT('Ctrl Pts',(6.28608355310373,-4.80694011032984,127.434715878518));
#55315=CARTESIAN_POINT('Ctrl Pts',(6.16455883936316,-4.95803744600921,127.426872229451));
#55316=CARTESIAN_POINT('Ctrl Pts',(6.09899207259603,-5.03955966040235,127.422640310747));
#55317=CARTESIAN_POINT('Ctrl Pts',(6.03185890404331,-5.11971762872589,127.418408392043));
#55318=CARTESIAN_POINT('Ctrl Pts',(5.96322422567988,-5.19844956061561,127.41417647334));
#55319=CARTESIAN_POINT('Ctrl Pts',(5.83481144673563,-5.34575390306584,127.406258720187));
#55320=CARTESIAN_POINT('Ctrl Pts',(5.70075682129387,-5.48850438542768,127.398340967034));
#55321=CARTESIAN_POINT('Ctrl Pts',(5.56141446608958,-5.62624120851298,127.390423213881));
#55322=CARTESIAN_POINT('Ctrl Pts',(5.42223220522564,-5.7638197818988,127.382514557657));
#55323=CARTESIAN_POINT('Ctrl Pts',(5.27777455793322,-5.89639592985943,127.374605901433));
#55324=CARTESIAN_POINT('Ctrl Pts',(5.1284360564711,-6.02354253032941,127.366697245209));
#55325=CARTESIAN_POINT('Ctrl Pts',(4.97924148956077,-6.15056658511443,127.358796211459));
#55326=CARTESIAN_POINT('Ctrl Pts',(4.82517570004318,-6.27217129531622,127.350895177709));
#55327=CARTESIAN_POINT('Ctrl Pts',(4.66667045601083,-6.38796586207187,127.342994143959));
#55328=CARTESIAN_POINT('Ctrl Pts',(4.50828865030388,-6.50367025207977,127.335099263257));
#55329=CARTESIAN_POINT('Ctrl Pts',(4.34547455493314,-6.61357331112474,127.327204382555));
#55330=CARTESIAN_POINT('Ctrl Pts',(4.17869366249202,-6.71732389237329,127.319309501853));
#55331=CARTESIAN_POINT('Ctrl Pts',(4.01201179833126,-6.82101287039201,127.311419308837));
#55332=CARTESIAN_POINT('Ctrl Pts',(3.84136812198953,-6.91855646840522,127.303529115822));
#55333=CARTESIAN_POINT('Ctrl Pts',(3.66725803943821,-7.00964617310859,127.295638922806));
#55334=CARTESIAN_POINT('Ctrl Pts',(3.4932191321903,-7.10069864081066,127.28775195526));
#55335=CARTESIAN_POINT('Ctrl Pts',(3.31571694760427,-7.18530231387692,127.279864987715));
#55336=CARTESIAN_POINT('Ctrl Pts',(3.13527272864077,-7.26319391982904,127.271978020169));
#55337=CARTESIAN_POINT('Ctrl Pts',(2.95484418002647,-7.34107876142665,127.264091737553));
#55338=CARTESIAN_POINT('Ctrl Pts',(2.77147441962109,-7.41225255487031,127.256205454936));
#55339=CARTESIAN_POINT('Ctrl Pts',(2.58570644708443,-7.47649939273093,127.24831917232));
#55340=CARTESIAN_POINT('Ctrl Pts',(2.39993880106107,-7.54074611766872,127.240432903565));
#55341=CARTESIAN_POINT('Ctrl Pts',(2.21177327678238,-7.5980657981353,127.23254663481));
#55342=CARTESIAN_POINT('Ctrl Pts',(2.02176998328062,-7.64829177886837,127.224660366055));
#55343=CARTESIAN_POINT('Ctrl Pts',(1.83173517819691,-7.69852608945761,127.216772789381));
#55344=CARTESIAN_POINT('Ctrl Pts',(1.63986232970381,-7.74166426807933,127.208885212708));
#55345=CARTESIAN_POINT('Ctrl Pts',(1.44672398292726,-7.77759028987919,127.200997636034));
#55346=CARTESIAN_POINT('Ctrl Pts',(1.25352123350256,-7.81352829133498,127.193107429221));
#55347=CARTESIAN_POINT('Ctrl Pts',(1.05905248352351,-7.84224928124183,127.185217222408));
#55348=CARTESIAN_POINT('Ctrl Pts',(0.863897930628899,-7.86368878869549,
127.177327015595));
#55349=CARTESIAN_POINT('Ctrl Pts',(0.668554924532715,-7.88514899945204,
127.169429189514));
#55350=CARTESIAN_POINT('Ctrl Pts',(0.472525135347926,-7.89931364542681,
127.161531363434));
#55351=CARTESIAN_POINT('Ctrl Pts',(0.276392376396081,-7.90617026469011,
127.153633537353));
#55352=CARTESIAN_POINT('Ctrl Pts',(0.080151015028995,-7.91303068059308,
127.145731338097));
#55353=CARTESIAN_POINT('Ctrl Pts',(-0.116193085992988,-7.91257500240236,
127.137829138841));
#55354=CARTESIAN_POINT('Ctrl Pts',(-0.312058386067501,-7.90484285509111,
127.129926939585));
#55355=CARTESIAN_POINT('Ctrl Pts',(-0.508160110409938,-7.89710137449179,
127.122015201775));
#55356=CARTESIAN_POINT('Ctrl Pts',(-0.703781536764284,-7.88206590697657,
127.114103463965));
#55357=CARTESIAN_POINT('Ctrl Pts',(-0.89834741166975,-7.85982779251214,
127.106191726155));
#55358=CARTESIAN_POINT('Ctrl Pts',(-0.978832218720607,-7.85062869553424,
127.102918928747));
#55359=CARTESIAN_POINT('Ctrl Pts',(-1.05913653073782,-7.84019770321675,
127.099646131339));
#55360=CARTESIAN_POINT('Ctrl Pts',(-1.13922025614804,-7.82854381146213,
127.096373333932));
#55361=CARTESIAN_POINT('Ctrl Pts',(-1.34268065491317,-7.79893597976579,
127.08805847767));
#55362=CARTESIAN_POINT('Ctrl Pts',(-1.54516044360248,-7.76136674831017,
127.079743621408));
#55363=CARTESIAN_POINT('Ctrl Pts',(-1.74602739208576,-7.71591273577444,
127.071428765146));
#55364=CARTESIAN_POINT('Ctrl Pts',(-1.94664697990449,-7.67051469827508,
127.063124148341));
#55365=CARTESIAN_POINT('Ctrl Pts',(-2.14565740416364,-7.61725130988443,
127.054819531536));
#55366=CARTESIAN_POINT('Ctrl Pts',(-2.34243424426202,-7.55625057891205,
127.04651491473));
#55367=CARTESIAN_POINT('Ctrl Pts',(-2.5389817401369,-7.49532094454468,127.03821997699));
#55368=CARTESIAN_POINT('Ctrl Pts',(-2.73330056505798,-7.42667204064051,
127.029925039251));
#55369=CARTESIAN_POINT('Ctrl Pts',(-2.924778318474,-7.35048248673408,127.021630101511));
#55370=CARTESIAN_POINT('Ctrl Pts',(-3.11596908234092,-7.27440712680231,
127.01334759634));
#55371=CARTESIAN_POINT('Ctrl Pts',(-3.30432700101088,-7.19081377987862,
127.005065091169));
#55372=CARTESIAN_POINT('Ctrl Pts',(-3.48925653830335,-7.0999302679609,126.996782585999));
#55373=CARTESIAN_POINT('Ctrl Pts',(-3.67401619147872,-7.00913024549223,
126.988507689489));
#55374=CARTESIAN_POINT('Ctrl Pts',(-3.85535348153576,-6.91105354190999,
126.980232792979));
#55375=CARTESIAN_POINT('Ctrl Pts',(-4.03269282144953,-6.80597602169075,
126.971957896468));
#55376=CARTESIAN_POINT('Ctrl Pts',(-4.20982930841732,-6.70101869637324,
126.963692465355));
#55377=CARTESIAN_POINT('Ctrl Pts',(-4.38297671897432,-6.5890766830643,126.955427034241));
#55378=CARTESIAN_POINT('Ctrl Pts',(-4.55158379852518,-6.47047184716873,
126.947161603127));
#55379=CARTESIAN_POINT('Ctrl Pts',(-4.6174716881255,-6.42412372018398,126.943931656827));
#55380=CARTESIAN_POINT('Ctrl Pts',(-4.68266649919513,-6.37675862865773,
126.940701710528));
#55381=CARTESIAN_POINT('Ctrl Pts',(-4.74713639940072,-6.32839766492947,
126.937471764228));
#55382=CARTESIAN_POINT('Ctrl Pts',(-4.91213757985737,-6.20462492636871,
126.929205194083));
#55383=CARTESIAN_POINT('Ctrl Pts',(-5.07220235932771,-6.07446541213496,
126.920938623938));
#55384=CARTESIAN_POINT('Ctrl Pts',(-5.22685289177513,-5.93834403245063,
126.912672053793));
#55385=CARTESIAN_POINT('Ctrl Pts',(-5.38164199289033,-5.80210068643394,
126.904398076705));
#55386=CARTESIAN_POINT('Ctrl Pts',(-5.53100694168514,-5.65988500454373,
126.896124099618));
#55387=CARTESIAN_POINT('Ctrl Pts',(-5.67450643526183,-5.51215907936011,
126.88785012253));
#55388=CARTESIAN_POINT('Ctrl Pts',(-5.81814382043432,-5.36429120131619,
126.879568194809));
#55389=CARTESIAN_POINT('Ctrl Pts',(-5.95590429362663,-5.21090271949208,
126.871286267088));
#55390=CARTESIAN_POINT('Ctrl Pts',(-6.08738599883386,-5.05248975270623,
126.863004339367));
#55391=CARTESIAN_POINT('Ctrl Pts',(-6.21908565043997,-4.89381419778622,
126.854708683376));
#55392=CARTESIAN_POINT('Ctrl Pts',(-6.34448553839401,-4.73009773313712,
126.846413027385));
#55393=CARTESIAN_POINT('Ctrl Pts',(-6.46322521665564,-4.561868125975,126.838117371394));
#55394=CARTESIAN_POINT('Ctrl Pts',(-6.58207221260689,-4.39348647180526,
126.829814217735));
#55395=CARTESIAN_POINT('Ctrl Pts',(-6.69424681966151,-4.22058377639063,
126.821511064077));
#55396=CARTESIAN_POINT('Ctrl Pts',(-6.7994332954081,-4.04371461175189,126.813207910418));
#55397=CARTESIAN_POINT('Ctrl Pts',(-6.9047801423241,-3.86657578587996,126.804892097466));
#55398=CARTESIAN_POINT('Ctrl Pts',(-7.00311741704465,-3.68545865853627,
126.796576284514));
#55399=CARTESIAN_POINT('Ctrl Pts',(-7.09417562213484,-3.50094176505519,
126.788260471562));
#55400=CARTESIAN_POINT('Ctrl Pts',(-7.12954515401619,-3.42927028701362,
126.785030379216));
#55401=CARTESIAN_POINT('Ctrl Pts',(-7.16381696594036,-3.35708607204337,
126.78180028687));
#55402=CARTESIAN_POINT('Ctrl Pts',(-7.19697725308157,-3.28442375746895,
126.778570194524));
#55403=CARTESIAN_POINT('Ctrl Pts',(-7.28407650476369,-3.09356795462343,
126.770085990964));
#55404=CARTESIAN_POINT('Ctrl Pts',(-7.36365819743208,-2.89907415392788,
126.761601787403));
#55405=CARTESIAN_POINT('Ctrl Pts',(-7.43542987574275,-2.70153725921229,
126.753117583843));
#55406=CARTESIAN_POINT('Ctrl Pts',(-7.50707789014547,-2.50434072416134,
126.74464799872));
#55407=CARTESIAN_POINT('Ctrl Pts',(-7.57094264450145,-2.30411180287135,
126.736178413597));
#55408=CARTESIAN_POINT('Ctrl Pts',(-7.62677904215236,-2.10146673592174,
126.727708828474));
#55409=CARTESIAN_POINT('Ctrl Pts',(-7.68247546284319,-1.89932968241211,
126.719260475859));
#55410=CARTESIAN_POINT('Ctrl Pts',(-7.73018361712663,-1.69478882443706,
126.710812123245));
#55411=CARTESIAN_POINT('Ctrl Pts',(-7.76970775347896,-1.48847654517262,
126.70236377063));
#55412=CARTESIAN_POINT('Ctrl Pts',(-7.80917011504265,-1.28248672450233,
126.693928622483));
#55413=CARTESIAN_POINT('Ctrl Pts',(-7.84047392002923,-1.07473126313879,
126.685493474337));
#55414=CARTESIAN_POINT('Ctrl Pts',(-7.86347335872907,-0.865856648965776,
126.67705832619));
#55415=CARTESIAN_POINT('Ctrl Pts',(-7.88642176547576,-0.657445493038951,
126.668641894243));
#55416=CARTESIAN_POINT('Ctrl Pts',(-7.9011025401978,-0.447920401316483,
126.660225462296));
#55417=CARTESIAN_POINT('Ctrl Pts',(-7.90742101320104,-0.237936798303012,
126.651809030349));
#55418=CARTESIAN_POINT('Ctrl Pts',(-7.90979270182071,-0.159117798628721,
126.648649856312));
#55419=CARTESIAN_POINT('Ctrl Pts',(-7.9109867088849,-0.0802343115594641,
126.645490682274));
#55420=CARTESIAN_POINT('Ctrl Pts',(-7.91099988964655,-0.00132136755638792,
126.642331508237));
#55421=CARTESIAN_POINT('',(-7.91057951044591,-1.0961900785361E-6,124.642534073604));
#55422=CARTESIAN_POINT('Ctrl Pts',(-7.89590378815153,-0.000272972207095395,
126.642289558051));
#55423=CARTESIAN_POINT('Ctrl Pts',(-7.89525879231852,0.244182270797831,
126.632484421598));
#55424=CARTESIAN_POINT('Ctrl Pts',(-7.88346689406167,0.489073252446727,
126.622890110621));
#55425=CARTESIAN_POINT('Ctrl Pts',(-7.86064702013486,0.733159060168601,
126.613430455262));
#55426=CARTESIAN_POINT('Ctrl Pts',(-7.83768760356675,0.978737443108859,
126.603912954478));
#55427=CARTESIAN_POINT('Ctrl Pts',(-7.8035656702398,1.22350018880843,126.594531761177));
#55428=CARTESIAN_POINT('Ctrl Pts',(-7.75843803336029,1.46622231357713,126.58520929961));
#55429=CARTESIAN_POINT('Ctrl Pts',(-7.71215904724558,1.71513705005877,126.575648992464));
#55430=CARTESIAN_POINT('Ctrl Pts',(-7.65430637076432,1.96190507839382,126.566150452148));
#55431=CARTESIAN_POINT('Ctrl Pts',(-7.58507521641603,2.20525554097891,126.556630012532));
#55432=CARTESIAN_POINT('Ctrl Pts',(-7.517710985487,2.44204368805782,126.547366306057));
#55433=CARTESIAN_POINT('Ctrl Pts',(-7.43957455068223,2.67559611108232,126.538081865451));
#55434=CARTESIAN_POINT('Ctrl Pts',(-7.35085768859411,2.90479295349016,126.528699612255));
#55435=CARTESIAN_POINT('Ctrl Pts',(-7.25845279536768,3.14351769253126,126.518927331265));
#55436=CARTESIAN_POINT('Ctrl Pts',(-7.15457041498237,3.37751673678469,126.509048936354));
#55437=CARTESIAN_POINT('Ctrl Pts',(-7.03942703122764,3.60558499376228,126.498977331278));
#55438=CARTESIAN_POINT('Ctrl Pts',(-6.92428364747292,3.83365325073987,126.488905726203));
#55439=CARTESIAN_POINT('Ctrl Pts',(-6.79788019574378,4.0557908697991,126.478640910961));
#55440=CARTESIAN_POINT('Ctrl Pts',(-6.6604189393482,4.27085362223415,126.46809578931));
#55441=CARTESIAN_POINT('Ctrl Pts',(-6.53065020558335,4.47388116465065,126.458140787297));
#55442=CARTESIAN_POINT('Ctrl Pts',(-6.3910274142673,4.67060441864484,126.447935973715));
#55443=CARTESIAN_POINT('Ctrl Pts',(-6.24257616274397,4.86064634215427,126.437408071393));
#55444=CARTESIAN_POINT('Ctrl Pts',(-6.10913696387804,5.03147037875764,126.427944797509));
#55445=CARTESIAN_POINT('Ctrl Pts',(-5.96856459495533,5.19689684478606,126.418220475277));
#55446=CARTESIAN_POINT('Ctrl Pts',(-5.82157948367676,5.35667837550104,126.408181885613));
#55447=CARTESIAN_POINT('Ctrl Pts',(-5.74017026894573,5.44517501867041,126.402621909541));
#55448=CARTESIAN_POINT('Ctrl Pts',(-5.65669728192142,5.53177480412959,126.397073971827));
#55449=CARTESIAN_POINT('Ctrl Pts',(-5.57106832213004,5.61622362318462,126.391705186412));
#55450=CARTESIAN_POINT('Ctrl Pts',(-5.48571564414274,5.70039996815918,126.386353723381));
#55451=CARTESIAN_POINT('Ctrl Pts',(-5.39822060300345,5.78243891205619,126.381180258445));
#55452=CARTESIAN_POINT('Ctrl Pts',(-5.30852766599007,5.86205167675951,126.37635029318));
#55453=CARTESIAN_POINT('Ctrl Pts',(-5.1012393575636,6.0460438156505,126.365187816368));
#55454=CARTESIAN_POINT('Ctrl Pts',(-4.88405257074258,6.2192397713721,126.354216226508));
#55455=CARTESIAN_POINT('Ctrl Pts',(-4.65847571308924,6.38096910882099,126.343375235685));
#55456=CARTESIAN_POINT('Ctrl Pts',(-4.43090782437457,6.54412593372466,126.332438557965));
#55457=CARTESIAN_POINT('Ctrl Pts',(-4.19480129197745,6.69561356116855,126.321634794895));
#55458=CARTESIAN_POINT('Ctrl Pts',(-3.95165450541081,6.8347617989245,126.310902048054));
#55459=CARTESIAN_POINT('Ctrl Pts',(-3.70677037942015,6.97490428267748,126.300092613282));
#55460=CARTESIAN_POINT('Ctrl Pts',(-3.45474506663523,7.10253126782972,126.289355213218));
#55461=CARTESIAN_POINT('Ctrl Pts',(-3.1970568016103,7.21696440524782,126.278626613105));
#55462=CARTESIAN_POINT('Ctrl Pts',(-2.93964967973582,7.33127269378013,126.267909718113));
#55463=CARTESIAN_POINT('Ctrl Pts',(-2.67659177292291,7.43241685886757,126.25720160388));
#55464=CARTESIAN_POINT('Ctrl Pts',(-2.40930549423133,7.51971345444516,126.246439242392));
#55465=CARTESIAN_POINT('Ctrl Pts',(-2.14547058041334,7.60588282267298,126.235815851137));
#55466=CARTESIAN_POINT('Ctrl Pts',(-1.87751538500848,7.67856087462327,126.22513960453));
#55467=CARTESIAN_POINT('Ctrl Pts',(-1.60676274543931,7.73706912373422,126.214349884736));
#55468=CARTESIAN_POINT('Ctrl Pts',(-1.34509704141678,7.79361373293583,126.203922286945));
#55469=CARTESIAN_POINT('Ctrl Pts',(-1.08081792752042,7.83692446044875,126.193388704872));
#55470=CARTESIAN_POINT('Ctrl Pts',(-0.81508448245884,7.86635676154958,126.182694421459));
#55471=CARTESIAN_POINT('Ctrl Pts',(-0.549351037397265,7.89578906265042,
126.172000138045));
#55472=CARTESIAN_POINT('Ctrl Pts',(-0.282162777800421,7.91134390915374,
126.161145153291));
#55473=CARTESIAN_POINT('Ctrl Pts',(-0.0146508286642535,7.9123310740961,
126.150074750138));
#55474=CARTESIAN_POINT('Ctrl Pts',(0.251092225934842,7.91331171151444,126.139077548857));
#55475=CARTESIAN_POINT('Ctrl Pts',(0.517155297956743,7.89991576666261,126.127867768622));
#55476=CARTESIAN_POINT('Ctrl Pts',(0.782460672384277,7.87279628714158,126.116391770645));
#55477=CARTESIAN_POINT('Ctrl Pts',(1.03037699804824,7.84745431383524,126.105667949999));
#55478=CARTESIAN_POINT('Ctrl Pts',(1.2767839336486,7.8097077836232,126.095037915708));
#55479=CARTESIAN_POINT('Ctrl Pts',(1.52075398454111,7.7602225636823,126.084495441738));
#55480=CARTESIAN_POINT('Ctrl Pts',(1.7767834028631,7.70829130396147,126.073431856398));
#55481=CARTESIAN_POINT('Ctrl Pts',(2.03012966018809,7.64343225965122,126.062464701477));
#55482=CARTESIAN_POINT('Ctrl Pts',(2.2797351064227,7.56635891108657,126.051586781298));
#55483=CARTESIAN_POINT('Ctrl Pts',(2.53575241247222,7.4873057038533,126.040429429318));
#55484=CARTESIAN_POINT('Ctrl Pts',(2.78783504942617,7.39540241387966,126.029365955485));
#55485=CARTESIAN_POINT('Ctrl Pts',(3.03484557046376,7.29136263958527,126.018388595228));
#55486=CARTESIAN_POINT('Ctrl Pts',(3.28564332865553,7.18572769721033,126.00724292689));
#55487=CARTESIAN_POINT('Ctrl Pts',(3.53121315723989,7.06758092367902,125.99618603301));
#55488=CARTESIAN_POINT('Ctrl Pts',(3.77035524889978,6.93761615226074,125.985209786367));
#55489=CARTESIAN_POINT('Ctrl Pts',(4.00938538319851,6.80771222547567,125.974238678391));
#55490=CARTESIAN_POINT('Ctrl Pts',(4.24199470785378,6.66600088648738,125.963348142159));
#55491=CARTESIAN_POINT('Ctrl Pts',(4.46696222334666,6.51312867884672,125.952530061859));
#55492=CARTESIAN_POINT('Ctrl Pts',(4.68565687270186,6.36451907282034,125.942013626752));
#55493=CARTESIAN_POINT('Ctrl Pts',(4.89713060704942,6.20536172926908,125.931565663272));
#55494=CARTESIAN_POINT('Ctrl Pts',(5.10022868738935,6.0362150263091,125.921178715744));
#55495=CARTESIAN_POINT('Ctrl Pts',(5.29824962882789,5.87129673015732,125.911051425891));
#55496=CARTESIAN_POINT('Ctrl Pts',(5.48830900713355,5.6968817792442,125.900982139511));
#55497=CARTESIAN_POINT('Ctrl Pts',(5.66929564701769,5.51346125802735,125.89096394621));
#55498=CARTESIAN_POINT('Ctrl Pts',(5.84313639376888,5.33728272684824,125.881341301105));
#55499=CARTESIAN_POINT('Ctrl Pts',(6.00860702598225,5.15279527887537,125.871765794112));
#55500=CARTESIAN_POINT('Ctrl Pts',(6.16467841740571,4.96041613331724,125.862231301475));
#55501=CARTESIAN_POINT('Ctrl Pts',(6.23236974654909,4.8769773945226,125.858095998564));
#55502=CARTESIAN_POINT('Ctrl Pts',(6.29829234471388,4.79205392592341,125.853968410999));
#55503=CARTESIAN_POINT('Ctrl Pts',(6.36235925507139,4.70567896073921,125.84984803915));
#55504=CARTESIAN_POINT('Ctrl Pts',(6.46054940887198,4.57329906183929,125.843533079628));
#55505=CARTESIAN_POINT('Ctrl Pts',(6.55444152696451,4.43787560876014,125.837090858175));
#55506=CARTESIAN_POINT('Ctrl Pts',(6.64372079618492,4.29954037237058,125.830546692025));
#55507=CARTESIAN_POINT('Ctrl Pts',(6.78171323046985,4.08572571882934,125.820431853215));
#55508=CARTESIAN_POINT('Ctrl Pts',(6.90868661329275,3.86495256094039,125.81007347237));
#55509=CARTESIAN_POINT('Ctrl Pts',(7.02445911752514,3.63839446700022,125.799565031978));
#55510=CARTESIAN_POINT('Ctrl Pts',(7.14067492739179,3.41096885723494,125.789016353614));
#55511=CARTESIAN_POINT('Ctrl Pts',(7.24560298045697,3.17771376223105,125.778316464314));
#55512=CARTESIAN_POINT('Ctrl Pts',(7.33904695897157,2.9398675721495,125.767559924547));
#55513=CARTESIAN_POINT('Ctrl Pts',(7.43277384202596,2.70130129535914,125.756770819024));
#55514=CARTESIAN_POINT('Ctrl Pts',(7.51494603697236,2.45811614005707,125.745924719492));
#55515=CARTESIAN_POINT('Ctrl Pts',(7.58536736127838,2.21161406445729,125.73511704788));
#55516=CARTESIAN_POINT('Ctrl Pts',(7.63190133520942,2.04872702316763,125.727975405572));
#55517=CARTESIAN_POINT('Ctrl Pts',(7.67330437430786,1.88439274736401,125.720850542754));
#55518=CARTESIAN_POINT('Ctrl Pts',(7.70952348573126,1.71899887370687,125.713769991952));
#55519=CARTESIAN_POINT('Ctrl Pts',(7.7592398181954,1.49197020052525,125.704050840823));
#55520=CARTESIAN_POINT('Ctrl Pts',(7.7991789160809,1.26291754830903,125.694426102973));
#55521=CARTESIAN_POINT('Ctrl Pts',(7.82932224132061,1.03264414334578,125.684900439759));
#55522=CARTESIAN_POINT('Ctrl Pts',(7.85973059201407,0.800346133825817,125.675291025228));
#55523=CARTESIAN_POINT('Ctrl Pts',(7.88017019939908,0.566804925514715,125.665782435155));
#55524=CARTESIAN_POINT('Ctrl Pts',(7.89056995547163,0.332838287613528,125.656379454933));
#55525=CARTESIAN_POINT('Ctrl Pts',(7.90088891275422,0.10068940592751,125.647049529254));
#55526=CARTESIAN_POINT('Ctrl Pts',(7.90132332167632,-0.131879176590046,
125.637823578772));
#55527=CARTESIAN_POINT('Ctrl Pts',(7.89175331818299,-0.364062246507516,
125.628706278206));
#55528=CARTESIAN_POINT('Ctrl Pts',(7.88242822988306,-0.590303295451428,
125.619822307277));
#55529=CARTESIAN_POINT('Ctrl Pts',(7.86360401924518,-0.816179005692197,
125.611041496294));
#55530=CARTESIAN_POINT('Ctrl Pts',(7.83512431819111,-1.04092707177344,125.602368170178));
#55531=CARTESIAN_POINT('Ctrl Pts',(7.81326926485723,-1.21339661285348,125.595712341716));
#55532=CARTESIAN_POINT('Ctrl Pts',(7.78572729891087,-1.3852018418126,125.58911980983));
#55533=CARTESIAN_POINT('Ctrl Pts',(7.75240995369105,-1.55598728154999,125.582592528981));
#55534=CARTESIAN_POINT('Ctrl Pts',(7.704696574801,-1.80056710450204,125.573244886719));
#55535=CARTESIAN_POINT('Ctrl Pts',(7.64563886056102,-2.04301353573977,125.563753397419));
#55536=CARTESIAN_POINT('Ctrl Pts',(7.5750843874418,-2.28203217332167,125.554127720513));
#55537=CARTESIAN_POINT('Ctrl Pts',(7.50559804389413,-2.5174322894454,125.544647767467));
#55538=CARTESIAN_POINT('Ctrl Pts',(7.42496042501464,-2.74950672460934,125.535037659012));
#55539=CARTESIAN_POINT('Ctrl Pts',(7.33307592637004,-2.97702152106806,125.525306622484));
#55540=CARTESIAN_POINT('Ctrl Pts',(7.29528362711784,-3.07059886435126,125.521304225453));
#55541=CARTESIAN_POINT('Ctrl Pts',(7.25558928898099,-3.16340496065179,125.517281371078));
#55542=CARTESIAN_POINT('Ctrl Pts',(7.21398876103173,-3.2553546114445,125.513238701394));
#55543=CARTESIAN_POINT('Ctrl Pts',(7.11242351002883,-3.479844295176,125.503368760279));
#55544=CARTESIAN_POINT('Ctrl Pts',(6.99949282415126,-3.69922720361958,125.493380707321));
#55545=CARTESIAN_POINT('Ctrl Pts',(6.87617750823767,-3.91272100540851,125.483283885776));
#55546=CARTESIAN_POINT('Ctrl Pts',(6.75156946206384,-4.128452890082,125.473081217957));
#55547=CARTESIAN_POINT('Ctrl Pts',(6.61635857760223,-4.33817092337202,125.462767489129));
#55548=CARTESIAN_POINT('Ctrl Pts',(6.47160077363162,-4.54109904828406,125.45235233948));
#55549=CARTESIAN_POINT('Ctrl Pts',(6.32732674454847,-4.74334899538394,125.441971996852));
#55550=CARTESIAN_POINT('Ctrl Pts',(6.17357025888858,-4.93885379496384,125.43149091016));
#55551=CARTESIAN_POINT('Ctrl Pts',(6.01140929001699,-5.12688461360331,125.420918623264));
#55552=CARTESIAN_POINT('Ctrl Pts',(5.88420144238739,-5.27438617266281,125.412625148763));
#55553=CARTESIAN_POINT('Ctrl Pts',(5.75182250090869,-5.41728916979181,125.404275552543));
#55554=CARTESIAN_POINT('Ctrl Pts',(5.61480240349224,-5.55526214589234,125.395874441697));
#55555=CARTESIAN_POINT('Ctrl Pts',(5.47545207294324,-5.69558156026265,125.387330457307));
#55556=CARTESIAN_POINT('Ctrl Pts',(5.3309152373884,-5.83058168527743,125.378979025504));
#55557=CARTESIAN_POINT('Ctrl Pts',(5.18166485115756,-5.96008197030643,125.370759811148));
#55558=CARTESIAN_POINT('Ctrl Pts',(5.0313840659925,-6.0904763029761,125.362483852754));
#55559=CARTESIAN_POINT('Ctrl Pts',(4.87632421001643,-6.21529523085981,125.354341943722));
#55560=CARTESIAN_POINT('Ctrl Pts',(4.71691597298543,-6.33434478870322,125.346272490636));
#55561=CARTESIAN_POINT('Ctrl Pts',(4.55734288271084,-6.45351746255446,125.338194692463));
#55562=CARTESIAN_POINT('Ctrl Pts',(4.39341211775056,-6.56690949397952,125.330189500176));
#55563=CARTESIAN_POINT('Ctrl Pts',(4.22550754581221,-6.67430688684188,125.322195129067));
#55564=CARTESIAN_POINT('Ctrl Pts',(4.16655942901025,-6.7120120784611,125.319388456703));
#55565=CARTESIAN_POINT('Ctrl Pts',(4.10712109687097,-6.74897816105583,125.316583118135));
#55566=CARTESIAN_POINT('Ctrl Pts',(4.04720786296046,-6.78519506688655,125.313776439721));
#55567=CARTESIAN_POINT('Ctrl Pts',(3.87147408838441,-6.89142424447699,125.305544065011));
#55568=CARTESIAN_POINT('Ctrl Pts',(3.69128912667578,-6.99090306358223,125.297551796561));
#55569=CARTESIAN_POINT('Ctrl Pts',(3.50736398910526,-7.08321704061147,125.289710530334));
#55570=CARTESIAN_POINT('Ctrl Pts',(3.32364035610237,-7.1754298803613,125.281877854836));
#55571=CARTESIAN_POINT('Ctrl Pts',(3.13618541275297,-7.26049381834744,125.274195850871));
#55572=CARTESIAN_POINT('Ctrl Pts',(2.94569003733961,-7.33804445665589,125.266575706942));
#55573=CARTESIAN_POINT('Ctrl Pts',(2.75565232501483,-7.4154087803907,125.258973870327));
#55574=CARTESIAN_POINT('Ctrl Pts',(2.56258934948931,-7.48529620126047,125.251433596868));
#55575=CARTESIAN_POINT('Ctrl Pts',(2.36715993274988,-7.54738903389064,125.243866713637));
#55576=CARTESIAN_POINT('Ctrl Pts',(2.17117638430508,-7.60965792807701,125.236278374834));
#55577=CARTESIAN_POINT('Ctrl Pts',(1.97281347304944,-7.66408835342329,125.228663275142));
#55578=CARTESIAN_POINT('Ctrl Pts',(1.77270010343906,-7.71039893332288,125.220932489474));
#55579=CARTESIAN_POINT('Ctrl Pts',(1.57258673382868,-7.75670951322246,125.213201703805));
#55580=CARTESIAN_POINT('Ctrl Pts',(1.37072331133005,-7.79490072675831,125.20535523216));
#55581=CARTESIAN_POINT('Ctrl Pts',(1.16769634284776,-7.82472364305471,125.197304149447));
#55582=CARTESIAN_POINT('Ctrl Pts',(0.965813858357259,-7.85437844449156,
125.18929845152));
#55583=CARTESIAN_POINT('Ctrl Pts',(0.762781187986504,-7.87575977590004,
125.181090442852));
#55584=CARTESIAN_POINT('Ctrl Pts',(0.559208285894424,-7.88926781703919,
125.172592693732));
#55585=CARTESIAN_POINT('Ctrl Pts',(0.356459147674568,-7.90272119748351,
125.164129331009));
#55586=CARTESIAN_POINT('Ctrl Pts',(0.15317432145551,-7.90836561736718,125.155378567978));
#55587=CARTESIAN_POINT('Ctrl Pts',(-0.0500937518569253,-7.90660820598672,
125.146254031998));
#55588=CARTESIAN_POINT('Ctrl Pts',(-0.149919802184598,-7.90574513175153,
125.141772923022));
#55589=CARTESIAN_POINT('Ctrl Pts',(-0.249742595932376,-7.90309696089872,
125.137201665795));
#55590=CARTESIAN_POINT('Ctrl Pts',(-0.349501308744162,-7.89871215899861,
125.132530029736));
#55591=CARTESIAN_POINT('Ctrl Pts',(-0.536340080188239,-7.8904998337094,
125.123780490801));
#55592=CARTESIAN_POINT('Ctrl Pts',(-0.722728550015766,-7.87503750680139,
125.11536121481));
#55593=CARTESIAN_POINT('Ctrl Pts',(-0.90822169714376,-7.85269664800584,
125.107185686861));
#55594=CARTESIAN_POINT('Ctrl Pts',(-1.09477681054902,-7.83022788562456,
125.09896335322));
#55595=CARTESIAN_POINT('Ctrl Pts',(-1.2804265969939,-7.80080201738374,125.090987566571));
#55596=CARTESIAN_POINT('Ctrl Pts',(-1.46476571484636,-7.76477314121034,
125.083170317571));
#55597=CARTESIAN_POINT('Ctrl Pts',(-1.65058136729158,-7.72845567798809,
125.075290453328));
#55598=CARTESIAN_POINT('Ctrl Pts',(-1.83506559767051,-7.68542941634956,
125.06757167664));
#55599=CARTESIAN_POINT('Ctrl Pts',(-2.01784670126836,-7.63602668685808,
125.059923846344));
#55600=CARTESIAN_POINT('Ctrl Pts',(-2.11626352911673,-7.60942623512704,
125.055805941469));
#55601=CARTESIAN_POINT('Ctrl Pts',(-2.21418730376919,-7.58097656982377,
125.051708605274));
#55602=CARTESIAN_POINT('Ctrl Pts',(-2.31156460429401,-7.55072534553676,
125.04761776636));
#55603=CARTESIAN_POINT('Ctrl Pts',(-2.54981033105506,-7.47671194737491,
125.037609018068));
#55604=CARTESIAN_POINT('Ctrl Pts',(-2.78498729435328,-7.3914957108001,125.02782080113));
#55605=CARTESIAN_POINT('Ctrl Pts',(-3.01591873950803,-7.29560419056322,
125.018171102507));
#55606=CARTESIAN_POINT('Ctrl Pts',(-3.24777425835197,-7.19932895978053,
125.008482790551));
#55607=CARTESIAN_POINT('Ctrl Pts',(-3.47535007178051,-7.09229375475358,
124.998934107693));
#55608=CARTESIAN_POINT('Ctrl Pts',(-3.69750661335462,-6.97504307815172,
124.98944205242));
#55609=CARTESIAN_POINT('Ctrl Pts',(-3.91984755346553,-6.85769507894549,
124.979942118374));
#55610=CARTESIAN_POINT('Ctrl Pts',(-4.13676027527797,-6.73011552110335,
124.970498905959));
#55611=CARTESIAN_POINT('Ctrl Pts',(-4.34715435964132,-6.59284735276243,
124.961029206809));
#55612=CARTESIAN_POINT('Ctrl Pts',(-4.55706810742043,-6.45589257214487,
124.951581127293));
#55613=CARTESIAN_POINT('Ctrl Pts',(-4.76049319839731,-6.3092941786778,124.942106681844));
#55614=CARTESIAN_POINT('Ctrl Pts',(-4.95639607436519,-6.15357587240645,
124.9325232307));
#55615=CARTESIAN_POINT('Ctrl Pts',(-5.15135536486482,-5.99860759867143,
124.92298593919));
#55616=CARTESIAN_POINT('Ctrl Pts',(-5.33886515785193,-5.8346077715742,124.913340689529));
#55617=CARTESIAN_POINT('Ctrl Pts',(-5.51795063617884,-5.6620657728485,124.903506030338));
#55618=CARTESIAN_POINT('Ctrl Pts',(-5.6654274504436,-5.51997751121685,124.895407192731));
#55619=CARTESIAN_POINT('Ctrl Pts',(-5.8071922583387,-5.37209604074902,124.887179906759));
#55620=CARTESIAN_POINT('Ctrl Pts',(-5.94271957325834,-5.21867595122357,
124.878778685289));
#55621=CARTESIAN_POINT('Ctrl Pts',(-6.10495330646991,-5.03502357171522,
124.868721955962));
#55622=CARTESIAN_POINT('Ctrl Pts',(-6.25824881491363,-4.8434361227992,124.858415987131));
#55623=CARTESIAN_POINT('Ctrl Pts',(-6.40246678594291,-4.64499312136272,
124.847782754194));
#55624=CARTESIAN_POINT('Ctrl Pts',(-6.48344627840437,-4.53356586008476,
124.84181211267));
#55625=CARTESIAN_POINT('Ctrl Pts',(-6.56156416342577,-4.41997629990883,
124.835738287774));
#55626=CARTESIAN_POINT('Ctrl Pts',(-6.63679849650785,-4.30440884672953,
124.829547466172));
#55627=CARTESIAN_POINT('Ctrl Pts',(-6.72011499660551,-4.17642637742798,
124.822691585786));
#55628=CARTESIAN_POINT('Ctrl Pts',(-6.79965595586647,-4.04601823311049,
124.815814270083));
#55629=CARTESIAN_POINT('Ctrl Pts',(-6.87518476737688,-3.91329963578802,
124.809047070757));
#55630=CARTESIAN_POINT('Ctrl Pts',(-6.95065926439568,-3.78067647943699,
124.80228473788));
#55631=CARTESIAN_POINT('Ctrl Pts',(-7.02212695112648,-3.64574585579345,
124.795632363062));
#55632=CARTESIAN_POINT('Ctrl Pts',(-7.08931967748596,-3.50866362545707,
124.789221214395));
#55633=CARTESIAN_POINT('Ctrl Pts',(-7.11346374519179,-3.45940646877021,
124.786917524459));
#55634=CARTESIAN_POINT('Ctrl Pts',(-7.13705558281161,-3.40987191498426,
124.784644980414));
#55635=CARTESIAN_POINT('Ctrl Pts',(-7.16008190363514,-3.36006860698215,
124.782409672347));
#55636=CARTESIAN_POINT('Ctrl Pts',(-7.26384175661325,-3.13564786883096,
124.772337058573));
#55637=CARTESIAN_POINT('Ctrl Pts',(-7.35716995380072,-2.90649307648692,
124.762305051782));
#55638=CARTESIAN_POINT('Ctrl Pts',(-7.4398793877542,-2.67359956042123,124.752302142289));
#55639=CARTESIAN_POINT('Ctrl Pts',(-7.52394297711727,-2.43689300877343,
124.742135460741));
#55640=CARTESIAN_POINT('Ctrl Pts',(-7.59703764473626,-2.19632357951533,
124.731998837077));
#55641=CARTESIAN_POINT('Ctrl Pts',(-7.65892336395348,-1.95290543871292,
124.72188018698));
#55642=CARTESIAN_POINT('Ctrl Pts',(-7.67718095646074,-1.88109195282541,
124.718894971771));
#55643=CARTESIAN_POINT('Ctrl Pts',(-7.69446264413822,-1.80903036140325,
124.715911320936));
#55644=CARTESIAN_POINT('Ctrl Pts',(-7.7107614762586,-1.73674635135296,124.712928924174));
#55645=CARTESIAN_POINT('Ctrl Pts',(-7.76604171847109,-1.49158292159577,
124.702813621792));
#55646=CARTESIAN_POINT('Ctrl Pts',(-7.81001965507663,-1.24386161844227,
124.692712745543));
#55647=CARTESIAN_POINT('Ctrl Pts',(-7.84250939741529,-0.994603241615372,
124.682614188839));
#55648=CARTESIAN_POINT('Ctrl Pts',(-7.87446930152253,-0.749409735976667,
124.672680318004));
#55649=CARTESIAN_POINT('Ctrl Pts',(-7.89531272647988,-0.502728051252808,
124.662748691678));
#55650=CARTESIAN_POINT('Ctrl Pts',(-7.9048127147597,-0.255527884110175,
124.652807785965));
#55651=CARTESIAN_POINT('Ctrl Pts',(-7.90808419112052,-0.170400462962063,
124.649384472473));
#55652=CARTESIAN_POINT('Ctrl Pts',(-7.91001002324155,-0.0852115949657462,
124.645960058556));
#55653=CARTESIAN_POINT('Ctrl Pts',(-7.91057951044591,-1.09619007819858E-6,
124.642534073604));
#55654=CARTESIAN_POINT('',(-7.911,6.17617068598975E-12,120.642331508237));
#55655=CARTESIAN_POINT('Ctrl Pts',(-7.91099999999379,-9.9090788532874E-6,
124.642291611247));
#55656=CARTESIAN_POINT('Ctrl Pts',(-7.91100077170824,0.616095093624387,
124.619899103357));
#55657=CARTESIAN_POINT('Ctrl Pts',(-7.83902979552628,1.23004343623821,124.598290807754));
#55658=CARTESIAN_POINT('Ctrl Pts',(-7.69060049730395,1.85452253341298,124.572895390152));
#55659=CARTESIAN_POINT('Ctrl Pts',(-7.68449683023176,1.8796537662833,124.571867207376));
#55660=CARTESIAN_POINT('Ctrl Pts',(-7.67537217560989,1.91643623128281,124.570352751203));
#55661=CARTESIAN_POINT('Ctrl Pts',(-7.67244761460173,1.92811137169331,124.569870627421));
#55662=CARTESIAN_POINT('Ctrl Pts',(-7.66712052415858,1.94917360889316,124.568998235471));
#55663=CARTESIAN_POINT('Ctrl Pts',(-7.66472736624521,1.95856306753437,124.568608382226));
#55664=CARTESIAN_POINT('Ctrl Pts',(-7.66102280173064,1.97298699868632,124.568008014787));
#55665=CARTESIAN_POINT('Ctrl Pts',(-7.65972366394776,1.97802463518305,124.567798055208));
#55666=CARTESIAN_POINT('Ctrl Pts',(-7.65734992081426,1.98719183732612,124.567415471357));
#55667=CARTESIAN_POINT('Ctrl Pts',(-7.65627694102972,1.99132182488932,124.567242921453));
#55668=CARTESIAN_POINT('Ctrl Pts',(-7.65393547617231,2.00030444776745,124.566867214661));
#55669=CARTESIAN_POINT('Ctrl Pts',(-7.65266571716323,2.00515674657815,124.566663999038));
#55670=CARTESIAN_POINT('Ctrl Pts',(-7.64920601422565,2.01832661625434,124.56611171833));
#55671=CARTESIAN_POINT('Ctrl Pts',(-7.64700712327769,2.02664181186375,124.565762235964));
#55672=CARTESIAN_POINT('Ctrl Pts',(-7.63657216286874,2.06584326514629,124.564110865558));
#55673=CARTESIAN_POINT('Ctrl Pts',(-7.6281625923931,2.09668266809594,124.562800737611));
#55674=CARTESIAN_POINT('Ctrl Pts',(-7.48845729261123,2.59703936891187,124.541354085422));
#55675=CARTESIAN_POINT('Ctrl Pts',(-7.31423891381664,3.05342230686368,124.518990924046));
#55676=CARTESIAN_POINT('Ctrl Pts',(-7.06745681925023,3.55529748413452,124.493215560518));
#55677=CARTESIAN_POINT('Ctrl Pts',(-7.03486673291457,3.61935576461539,124.489901059271));
#55678=CARTESIAN_POINT('Ctrl Pts',(-6.95920363056495,3.76319336261129,124.482412807041));
#55679=CARTESIAN_POINT('Ctrl Pts',(-6.91562269220845,3.84269468159141,124.478241508865));
#55680=CARTESIAN_POINT('Ctrl Pts',(-6.78625666644176,4.06935516682283,124.466277698181));
#55681=CARTESIAN_POINT('Ctrl Pts',(-6.69707152517261,4.21451856458861,124.458528238528));
#55682=CARTESIAN_POINT('Ctrl Pts',(-6.37126356878239,4.70833282361316,124.431997655447));
#55683=CARTESIAN_POINT('Ctrl Pts',(-6.11152425154984,5.04090670998819,124.413872811678));
#55684=CARTESIAN_POINT('Ctrl Pts',(-5.81428038503819,5.36454946432255,124.39611853848));
#55685=CARTESIAN_POINT('Ctrl Pts',(-5.8020149435884,5.37781274786763,124.395390625951));
#55686=CARTESIAN_POINT('Ctrl Pts',(-5.7841947673019,5.39695073677408,124.394339813085));
#55687=CARTESIAN_POINT('Ctrl Pts',(-5.77867633361254,5.40285907581428,124.394015335394));
#55688=CARTESIAN_POINT('Ctrl Pts',(-5.76903586370807,5.41314902737378,124.393450105277));
#55689=CARTESIAN_POINT('Ctrl Pts',(-5.76491787374394,5.41753441138149,124.393209176539));
#55690=CARTESIAN_POINT('Ctrl Pts',(-5.75695672290038,5.42599314896151,124.392744386498));
#55691=CARTESIAN_POINT('Ctrl Pts',(-5.75311423215649,5.43006712609012,124.392520496135));
#55692=CARTESIAN_POINT('Ctrl Pts',(-5.74400106406117,5.43970877482316,124.391990546226));
#55693=CARTESIAN_POINT('Ctrl Pts',(-5.7387266078904,5.44527287646475,124.391684652842));
#55694=CARTESIAN_POINT('Ctrl Pts',(-5.72020758113734,5.46475207823111,124.390613528363));
#55695=CARTESIAN_POINT('Ctrl Pts',(-5.70692037056824,5.47862664712957,124.389850177573));
#55696=CARTESIAN_POINT('Ctrl Pts',(-5.5453225682028,5.64614205297307,124.380628484054));
#55697=CARTESIAN_POINT('Ctrl Pts',(-5.39089492648068,5.79377104313747,124.372450516427));
#55698=CARTESIAN_POINT('Ctrl Pts',(-4.87541783818458,6.24807648957828,124.346929873478));
#55699=CARTESIAN_POINT('Ctrl Pts',(-4.49275309126979,6.52865706021101,124.330663986209));
#55700=CARTESIAN_POINT('Ctrl Pts',(-3.98659592446996,6.83409126212303,124.31058699436));
#55701=CARTESIAN_POINT('Ctrl Pts',(-3.88456682397703,6.89259682255909,124.306602508755));
#55702=CARTESIAN_POINT('Ctrl Pts',(-3.68721300581236,6.9999891420614,124.298958209091));
#55703=CARTESIAN_POINT('Ctrl Pts',(-3.59212552978188,7.04925680904181,124.295301980547));
#55704=CARTESIAN_POINT('Ctrl Pts',(-3.25682776757225,7.21443835311452,124.282419437024));
#55705=CARTESIAN_POINT('Ctrl Pts',(-3.01179252639721,7.32011873371692,124.273025544921));
#55706=CARTESIAN_POINT('Ctrl Pts',(-2.63708880669378,7.45972017139538,124.258085556628));
#55707=CARTESIAN_POINT('Ctrl Pts',(-2.51112437378818,7.50306026981479,124.252968597139));
#55708=CARTESIAN_POINT('Ctrl Pts',(-2.36427861709037,7.54947290627293,124.246833707374));
#55709=CARTESIAN_POINT('Ctrl Pts',(-2.34440048449791,7.55566945375918,124.245999684416));
#55710=CARTESIAN_POINT('Ctrl Pts',(-2.31884807796263,7.56352427993053,124.244922762561));
#55711=CARTESIAN_POINT('Ctrl Pts',(-2.31319592572444,7.56525482390469,124.244684246638));
#55712=CARTESIAN_POINT('Ctrl Pts',(-2.30409854152164,7.56802906111833,124.244299850877));
#55713=CARTESIAN_POINT('Ctrl Pts',(-2.30065451735323,7.56907674361673,124.244154215097));
#55714=CARTESIAN_POINT('Ctrl Pts',(-2.29407626692484,7.57107296257164,124.243875824814));
#55715=CARTESIAN_POINT('Ctrl Pts',(-2.29094217432202,7.57202190150692,124.243743095974));
#55716=CARTESIAN_POINT('Ctrl Pts',(-2.28375498802345,7.57419316339067,124.24343850323));
#55717=CARTESIAN_POINT('Ctrl Pts',(-2.27970150359107,7.57541417851784,124.243266559717));
#55718=CARTESIAN_POINT('Ctrl Pts',(-2.2691112945865,7.57859495568256,124.242816930959));
#55719=CARTESIAN_POINT('Ctrl Pts',(-2.26257302429417,7.58054951033666,124.242538931718));
#55720=CARTESIAN_POINT('Ctrl Pts',(-2.22148671867581,7.59277398570733,124.240789496881));
#55721=CARTESIAN_POINT('Ctrl Pts',(-2.1868718733217,7.6028160157105,124.239304536962));
#55722=CARTESIAN_POINT('Ctrl Pts',(-1.61369271236818,7.76486145960954,124.214548021526));
#55723=CARTESIAN_POINT('Ctrl Pts',(-1.06059668918216,7.85952508999731,124.18833111026));
#55724=CARTESIAN_POINT('Ctrl Pts',(-0.203109163965433,7.91406844103551,
124.148570421414));
#55725=CARTESIAN_POINT('Ctrl Pts',(0.0968240754261465,7.91608321280031,
124.134803966405));
#55726=CARTESIAN_POINT('Ctrl Pts',(0.444946279826982,7.89862835436435,124.119259843359));
#55727=CARTESIAN_POINT('Ctrl Pts',(0.493709201092214,7.89573039008704,124.117092089108));
#55728=CARTESIAN_POINT('Ctrl Pts',(0.605850564029667,7.88802292399882,124.112130231664));
#55729=CARTESIAN_POINT('Ctrl Pts',(0.669204500677268,7.88290086957189,124.109344270367));
#55730=CARTESIAN_POINT('Ctrl Pts',(0.999083139047645,7.85222515977152,124.094932921075));
#55731=CARTESIAN_POINT('Ctrl Pts',(1.26425908898607,7.81391547534457,124.083680554268));
#55732=CARTESIAN_POINT('Ctrl Pts',(1.54519317138068,7.75864954809616,124.072119948267));
#55733=CARTESIAN_POINT('Ctrl Pts',(1.56337236757229,7.75500687257187,124.071373449657));
#55734=CARTESIAN_POINT('Ctrl Pts',(1.58950608629844,7.74967467213716,124.070302567913));
#55735=CARTESIAN_POINT('Ctrl Pts',(1.59747100329485,7.74803675239752,124.069976491257));
#55736=CARTESIAN_POINT('Ctrl Pts',(1.61129472320905,7.74517179575376,124.069411081564));
#55737=CARTESIAN_POINT('Ctrl Pts',(1.61715467749298,7.7439503859496,124.069171563865));
#55738=CARTESIAN_POINT('Ctrl Pts',(1.62842222555588,7.74158850610722,124.068711329701));
#55739=CARTESIAN_POINT('Ctrl Pts',(1.63383001993956,7.74044901854383,124.068490581123));
#55740=CARTESIAN_POINT('Ctrl Pts',(1.64656966863446,7.73775067524648,124.067970867144));
#55741=CARTESIAN_POINT('Ctrl Pts',(1.6539005166104,7.73618706259885,124.067672058329));
#55742=CARTESIAN_POINT('Ctrl Pts',(1.67924594526784,7.7307434076153,124.066639837052));
#55743=CARTESIAN_POINT('Ctrl Pts',(1.6972492490136,7.72681082801006,124.065908153714));
#55744=CARTESIAN_POINT('Ctrl Pts',(1.8982753896191,7.68216288477946,124.057754864898));
#55745=CARTESIAN_POINT('Ctrl Pts',(2.07981512192932,7.63501479599362,124.050549286224));
#55746=CARTESIAN_POINT('Ctrl Pts',(2.65554284825593,7.46342956325596,124.028075424218));
#55747=CARTESIAN_POINT('Ctrl Pts',(3.04172714893981,7.31454807896272,124.013616363521));
#55748=CARTESIAN_POINT('Ctrl Pts',(3.70556229176986,6.99691531539792,123.988336358649));
#55749=CARTESIAN_POINT('Ctrl Pts',(3.98780137093101,6.83998888561804,123.977422504333));
#55750=CARTESIAN_POINT('Ctrl Pts',(4.48204975463995,6.52417039791635,123.956850845358));
#55751=CARTESIAN_POINT('Ctrl Pts',(4.69717222860623,6.37103794993058,123.947333995196));
#55752=CARTESIAN_POINT('Ctrl Pts',(4.9488906743264,6.1721667442069,123.934992719629));
#55753=CARTESIAN_POINT('Ctrl Pts',(4.99317280140977,6.13639848137497,123.9327735766));
#55754=CARTESIAN_POINT('Ctrl Pts',(5.0607393016651,6.08060699341461,123.929306321449));
#55755=CARTESIAN_POINT('Ctrl Pts',(5.08430017988199,6.0609203360521,123.928081773871));
#55756=CARTESIAN_POINT('Ctrl Pts',(5.11293829151014,6.03670682308196,123.926573502344));
#55757=CARTESIAN_POINT('Ctrl Pts',(5.11812535075823,6.0323096849034,123.926299516304));
#55758=CARTESIAN_POINT('Ctrl Pts',(5.12625974439981,6.02539600793448,123.925868581109));
#55759=CARTESIAN_POINT('Ctrl Pts',(5.12921088905831,6.02288399979204,123.925711976545));
#55760=CARTESIAN_POINT('Ctrl Pts',(5.13445529031209,6.01841332638514,123.92543321453));
#55761=CARTESIAN_POINT('Ctrl Pts',(5.13674927696884,6.01645551474748,123.925311121298));
#55762=CARTESIAN_POINT('Ctrl Pts',(5.14204549564431,6.01193019971306,123.925028875424));
#55763=CARTESIAN_POINT('Ctrl Pts',(5.14504692311312,6.00936176015015,123.924868652703));
#55764=CARTESIAN_POINT('Ctrl Pts',(5.15328495714737,6.00230145439448,123.92442814762));
#55765=CARTESIAN_POINT('Ctrl Pts',(5.15851760302444,5.99780499330445,123.924147523613));
#55766=CARTESIAN_POINT('Ctrl Pts',(5.18589919665489,5.97421339785629,123.922674777655));
#55767=CARTESIAN_POINT('Ctrl Pts',(5.20794776572334,5.95500262204447,123.921474158988));
#55768=CARTESIAN_POINT('Ctrl Pts',(5.23904542034123,5.92760263595197,123.919760500473));
#55769=CARTESIAN_POINT('Ctrl Pts',(5.24818307620973,5.91951385856859,123.919254458469));
#55770=CARTESIAN_POINT('Ctrl Pts',(5.27100527749317,5.89921695402138,123.917984371663));
#55771=CARTESIAN_POINT('Ctrl Pts',(5.28466610461629,5.88698237291208,123.917218525034));
#55772=CARTESIAN_POINT('Ctrl Pts',(5.30010485133022,5.87305845161526,123.916346764332));
#55773=CARTESIAN_POINT('Ctrl Pts',(5.30192476912948,5.87141556642451,123.916243902561));
#55774=CARTESIAN_POINT('Ctrl Pts',(5.3048351506227,5.8687858359032,123.916079250216));
#55775=CARTESIAN_POINT('Ctrl Pts',(5.30592610448748,5.86779953105878,123.916017494983));
#55776=CARTESIAN_POINT('Ctrl Pts',(5.30785786185848,5.866052096988,123.915908081987));
#55777=CARTESIAN_POINT('Ctrl Pts',(5.30869877710007,5.86529109083975,123.915860432249));
#55778=CARTESIAN_POINT('Ctrl Pts',(5.31033717022359,5.86380774721387,123.915767553123));
#55779=CARTESIAN_POINT('Ctrl Pts',(5.31113466448161,5.86308542778319,123.915722324908));
#55780=CARTESIAN_POINT('Ctrl Pts',(5.31286271665923,5.86151962645638,123.915624281056));
#55781=CARTESIAN_POINT('Ctrl Pts',(5.31379322101497,5.86067608571681,123.915571461599));
#55782=CARTESIAN_POINT('Ctrl Pts',(5.6857690934152,5.52330313541561,123.894446205186));
#55783=CARTESIAN_POINT('Ctrl Pts',(6.02398907474198,5.15231401385136,123.871208182852));
#55784=CARTESIAN_POINT('Ctrl Pts',(6.57527815338424,4.41853722665878,123.828827043769));
#55785=CARTESIAN_POINT('Ctrl Pts',(6.79898926746699,4.06590042785956,123.809711049112));
#55786=CARTESIAN_POINT('Ctrl Pts',(7.09309535526644,3.5095575321169,123.782180581988));
#55787=CARTESIAN_POINT('Ctrl Pts',(7.18472708804641,3.31793632075104,123.773120485363));
#55788=CARTESIAN_POINT('Ctrl Pts',(7.30586444551254,3.03598487377043,123.760403725367));
#55789=CARTESIAN_POINT('Ctrl Pts',(7.34162584189052,2.94845557139175,123.756538116745));
#55790=CARTESIAN_POINT('Ctrl Pts',(7.38109670292707,2.84667283325192,123.752135182576));
#55791=CARTESIAN_POINT('Ctrl Pts',(7.38634509750873,2.83302680202614,123.751546772124));
#55792=CARTESIAN_POINT('Ctrl Pts',(7.39424746612072,2.81230909735581,123.750656285061));
#55793=CARTESIAN_POINT('Ctrl Pts',(7.39692917813153,2.80524807876505,123.750353289898));
#55794=CARTESIAN_POINT('Ctrl Pts',(7.40174037957929,2.79252519137455,123.749808237648));
#55795=CARTESIAN_POINT('Ctrl Pts',(7.40387349353825,2.78686470483313,123.749566060814));
#55796=CARTESIAN_POINT('Ctrl Pts',(7.40812987002628,2.77553049488348,123.749081779572));
#55797=CARTESIAN_POINT('Ctrl Pts',(7.41025311199192,2.76985676807067,123.748839675958));
#55798=CARTESIAN_POINT('Ctrl Pts',(7.41616540501368,2.75400248471894,123.748164048706));
#55799=CARTESIAN_POINT('Ctrl Pts',(7.41994001405548,2.7438165371201,123.747731001661));
#55800=CARTESIAN_POINT('Ctrl Pts',(7.43505477364246,2.70276941688366,123.74599002222));
#55801=CARTESIAN_POINT('Ctrl Pts',(7.44622353626729,2.67184525910684,123.744687732599));
#55802=CARTESIAN_POINT('Ctrl Pts',(7.62433074617252,2.16890874868837,123.723656448207));
#55803=CARTESIAN_POINT('Ctrl Pts',(7.74629278605102,1.68214098881059,123.705524311749));
#55804=CARTESIAN_POINT('Ctrl Pts',(7.87007455811576,0.866569145374262,123.676663484459));
#55805=CARTESIAN_POINT('Ctrl Pts',(7.89897191501195,0.543373826803735,123.665578024828));
#55806=CARTESIAN_POINT('Ctrl Pts',(7.91666798732602,-0.0946874406580678,
123.643216466774));
#55807=CARTESIAN_POINT('Ctrl Pts',(7.90666549952213,-0.408915775281337,
123.631971970887));
#55808=CARTESIAN_POINT('Ctrl Pts',(7.8725152598048,-0.781700473469742,123.617568585183));
#55809=CARTESIAN_POINT('Ctrl Pts',(7.86633271057288,-0.841642158574129,
123.615219369987));
#55810=CARTESIAN_POINT('Ctrl Pts',(7.85577490281161,-0.933686722963544,
123.611553253189));
#55811=CARTESIAN_POINT('Ctrl Pts',(7.85188611331099,-0.965843998667573,
123.610261381146));
#55812=CARTESIAN_POINT('Ctrl Pts',(7.84689833289713,-1.00506648546604,123.608671231957));
#55813=CARTESIAN_POINT('Ctrl Pts',(7.8459870641719,-1.0121556576277,123.608383247767));
#55814=CARTESIAN_POINT('Ctrl Pts',(7.84454859224729,-1.02322750332178,123.607932561268));
#55815=CARTESIAN_POINT('Ctrl Pts',(7.84402795867968,-1.02721104113258,123.607770223999));
#55816=CARTESIAN_POINT('Ctrl Pts',(7.84310152080668,-1.03425774447642,123.60748272687));
#55817=CARTESIAN_POINT('Ctrl Pts',(7.84269695689589,-1.03732106405509,123.607357636677));
#55818=CARTESIAN_POINT('Ctrl Pts',(7.84175908128332,-1.04439065761155,123.607068696005));
#55819=CARTESIAN_POINT('Ctrl Pts',(7.84122449573997,-1.04839674832143,123.606904774762));
#55820=CARTESIAN_POINT('Ctrl Pts',(7.83974725213902,-1.05940261854323,123.606453921429));
#55821=CARTESIAN_POINT('Ctrl Pts',(7.83879829138257,-1.06640153414271,123.606166639636));
#55822=CARTESIAN_POINT('Ctrl Pts',(7.83407953580485,-1.10085735710837,123.604749557759));
#55823=CARTESIAN_POINT('Ctrl Pts',(7.83017488703788,-1.12829530602195,123.603612387179));
#55824=CARTESIAN_POINT('Ctrl Pts',(7.76131019396325,-1.5946258840028,123.584143694424));
#55825=CARTESIAN_POINT('Ctrl Pts',(7.65969031639534,-2.027275885833,123.563984035821));
#55826=CARTESIAN_POINT('Ctrl Pts',(7.37074422554263,-2.9147733859221,123.521172573966));
#55827=CARTESIAN_POINT('Ctrl Pts',(7.17619799029957,-3.36541643435674,123.498607944311));
#55828=CARTESIAN_POINT('Ctrl Pts',(6.84302540837918,-3.97477224277497,123.468324563319));
#55829=CARTESIAN_POINT('Ctrl Pts',(6.73790152207192,-4.1504821559099,123.45960813468));
#55830=CARTESIAN_POINT('Ctrl Pts',(6.57571754718104,-4.39913131483919,123.447315930482));
#55831=CARTESIAN_POINT('Ctrl Pts',(6.52401305311312,-4.47545215760701,123.443548526978));
#55832=CARTESIAN_POINT('Ctrl Pts',(6.46262897620268,-4.56273588221103,123.439245020194));
#55833=CARTESIAN_POINT('Ctrl Pts',(6.45423985936206,-4.57459504826287,123.438660412993));
#55834=CARTESIAN_POINT('Ctrl Pts',(6.44145058423301,-4.59256922897236,123.437774510486));
#55835=CARTESIAN_POINT('Ctrl Pts',(6.43707429860603,-4.59870114561147,123.437472310096));
#55836=CARTESIAN_POINT('Ctrl Pts',(6.42913649341898,-4.60978982194953,123.436925870435));
#55837=CARTESIAN_POINT('Ctrl Pts',(6.42557798634211,-4.61474872503483,123.436681516868));
#55838=CARTESIAN_POINT('Ctrl Pts',(6.41846158332143,-4.62464148933245,123.436194075358));
#55839=CARTESIAN_POINT('Ctrl Pts',(6.41490372869521,-4.62957537504377,123.4359509861));
#55840=CARTESIAN_POINT('Ctrl Pts',(6.40490390247358,-4.64340906072584,123.435269451836));
#55841=CARTESIAN_POINT('Ctrl Pts',(6.39844906542288,-4.65229956726581,123.434831498747));
#55842=CARTESIAN_POINT('Ctrl Pts',(6.37205586752091,-4.68849314962892,123.433048757232));
#55843=CARTESIAN_POINT('Ctrl Pts',(6.35196096816326,-4.71568191120208,123.431709979664));
#55844=CARTESIAN_POINT('Ctrl Pts',(6.04001201484681,-5.13214249092462,123.411207636524));
#55845=CARTESIAN_POINT('Ctrl Pts',(5.71302646410046,-5.49381704819989,123.393553679844));
#55846=CARTESIAN_POINT('Ctrl Pts',(4.98662054970738,-6.16180066265601,123.359112905146));
#55847=CARTESIAN_POINT('Ctrl Pts',(4.58712483576216,-6.46470545458634,123.342426188916));
#55848=CARTESIAN_POINT('Ctrl Pts',(4.02955933794191,-6.80960529652429,123.318908866944));
#55849=CARTESIAN_POINT('Ctrl Pts',(3.89501794876902,-6.88744540717358,123.313211719332));
#55850=CARTESIAN_POINT('Ctrl Pts',(3.66459793120062,-7.01184545719884,123.303279379229));
#55851=CARTESIAN_POINT('Ctrl Pts',(3.56991086900105,-7.06052330781336,123.299149722552));
#55852=CARTESIAN_POINT('Ctrl Pts',(3.45780710298393,-7.1153233937583,123.294172807741));
#55853=CARTESIAN_POINT('Ctrl Pts',(3.44131228576678,-7.12331570975056,123.293438314718));
#55854=CARTESIAN_POINT('Ctrl Pts',(3.41958066878851,-7.13375233977967,123.292467567576));
#55855=CARTESIAN_POINT('Ctrl Pts',(3.41436864218453,-7.13624839608318,123.292234516003));
#55856=CARTESIAN_POINT('Ctrl Pts',(3.40585257517752,-7.14031530259428,123.291853342184));
#55857=CARTESIAN_POINT('Ctrl Pts',(3.40255016415048,-7.14188957942224,123.291705433965));
#55858=CARTESIAN_POINT('Ctrl Pts',(3.39618174678333,-7.14492001800214,123.291420021603));
#55859=CARTESIAN_POINT('Ctrl Pts',(3.3931158922795,-7.14637649878061,123.29128253755));
#55860=CARTESIAN_POINT('Ctrl Pts',(3.38608315878731,-7.14971195982811,123.290966973913));
#55861=CARTESIAN_POINT('Ctrl Pts',(3.38211565300836,-7.15158961184786,123.290788810421));
#55862=CARTESIAN_POINT('Ctrl Pts',(3.36944076900796,-7.1575751898068,123.290219187289));
#55863=CARTESIAN_POINT('Ctrl Pts',(3.36072748439498,-7.16167050817418,123.289826926901));
#55864=CARTESIAN_POINT('Ctrl Pts',(3.28243091479241,-7.19829621187365,123.286296215133));
#55865=CARTESIAN_POINT('Ctrl Pts',(3.21238686256765,-7.22982648263096,123.283095831702));
#55866=CARTESIAN_POINT('Ctrl Pts',(3.04163948813402,-7.30371714833326,123.275214911289));
#55867=CARTESIAN_POINT('Ctrl Pts',(2.9404974910153,-7.34502060720955,123.270480922168));
#55868=CARTESIAN_POINT('Ctrl Pts',(2.78632583582631,-7.40428511840419,123.263203041203));
#55869=CARTESIAN_POINT('Ctrl Pts',(2.73390440513996,-7.42380066373664,123.260717761089));
#55870=CARTESIAN_POINT('Ctrl Pts',(2.59807059408156,-7.47273529687531,123.254258543009));
#55871=CARTESIAN_POINT('Ctrl Pts',(2.51436451923565,-7.50131416022644,123.250259457766));
#55872=CARTESIAN_POINT('Ctrl Pts',(2.07230157174148,-7.64401232509467,123.229103261318));
#55873=CARTESIAN_POINT('Ctrl Pts',(1.7066232729393,-7.73387346870796,123.21150578569));
#55874=CARTESIAN_POINT('Ctrl Pts',(1.027657488484,-7.85020177798744,123.179917548129));
#55875=CARTESIAN_POINT('Ctrl Pts',(0.71649905408271,-7.88469410262551,123.165841072037));
#55876=CARTESIAN_POINT('Ctrl Pts',(0.228787208891369,-7.90963911821695,
123.14468844352));
#55877=CARTESIAN_POINT('Ctrl Pts',(0.0532221101480262,-7.91276862218067,
123.137253380729));
#55878=CARTESIAN_POINT('Ctrl Pts',(-0.205490886865128,-7.90876824939127,
123.126567976629));
#55879=CARTESIAN_POINT('Ctrl Pts',(-0.288647972187168,-7.90617003649517,
123.123174393269));
#55880=CARTESIAN_POINT('Ctrl Pts',(-0.385474860921468,-7.90161495576565,
123.119269399932));
#55881=CARTESIAN_POINT('Ctrl Pts',(-0.399197658306523,-7.90093355305107,
123.118717050117));
#55882=CARTESIAN_POINT('Ctrl Pts',(-0.420103370630517,-7.89984087935348,
123.11787722653));
#55883=CARTESIAN_POINT('Ctrl Pts',(-0.42728758064708,-7.89945555623338,
123.117588918256));
#55884=CARTESIAN_POINT('Ctrl Pts',(-0.439764142176992,-7.89876930910933,
123.117088734832));
#55885=CARTESIAN_POINT('Ctrl Pts',(-0.445056729466244,-7.8984728654958,
123.116876715644));
#55886=CARTESIAN_POINT('Ctrl Pts',(-0.456071739729784,-7.89784479615776,
123.116435789805));
#55887=CARTESIAN_POINT('Ctrl Pts',(-0.461794109508233,-7.89751227011302,
123.116206912255));
#55888=CARTESIAN_POINT('Ctrl Pts',(-0.477485910769263,-7.89658330862678,
123.115579796605));
#55889=CARTESIAN_POINT('Ctrl Pts',(-0.487454597998916,-7.89597421227564,
123.115181966239));
#55890=CARTESIAN_POINT('Ctrl Pts',(-0.525695410727995,-7.89356496688971,
123.113658000531));
#55891=CARTESIAN_POINT('Ctrl Pts',(-0.553959104914379,-7.8916318263737,
123.112536148718));
#55892=CARTESIAN_POINT('Ctrl Pts',(-1.01258588467649,-7.85778729528332,
123.094403867211));
#55893=CARTESIAN_POINT('Ctrl Pts',(-1.43965336392091,-7.7908665892607,123.078604742236));
#55894=CARTESIAN_POINT('Ctrl Pts',(-2.39867216381311,-7.5589926621849,123.04398015812));
#55895=CARTESIAN_POINT('Ctrl Pts',(-2.92291016732958,-7.37214593848863,
123.02571224305));
#55896=CARTESIAN_POINT('Ctrl Pts',(-3.6637565331755,-7.01655022020611,122.996321897063));
#55897=CARTESIAN_POINT('Ctrl Pts',(-3.89824830688274,-6.88902937648518,
122.98641035275));
#55898=CARTESIAN_POINT('Ctrl Pts',(-4.13709715609504,-6.74303510914143,
122.975201569294));
#55899=CARTESIAN_POINT('Ctrl Pts',(-4.14834644434193,-6.73612033263785,
122.974670975217));
#55900=CARTESIAN_POINT('Ctrl Pts',(-4.16382220109497,-6.72655413790629,
122.973937253869));
#55901=CARTESIAN_POINT('Ctrl Pts',(-4.16806360752852,-6.7239268032817,122.973735772429));
#55902=CARTESIAN_POINT('Ctrl Pts',(-4.17520072783732,-6.71949637388267,
122.973396069169));
#55903=CARTESIAN_POINT('Ctrl Pts',(-4.17809777105323,-6.71769541225293,
122.973257994661));
#55904=CARTESIAN_POINT('Ctrl Pts',(-4.1838163211202,-6.7141353163762,122.972985078713));
#55905=CARTESIAN_POINT('Ctrl Pts',(-4.18663787430333,-6.71237628302267,
122.972850244168));
#55906=CARTESIAN_POINT('Ctrl Pts',(-4.19287210075292,-6.7084842358551,122.972551935545));
#55907=CARTESIAN_POINT('Ctrl Pts',(-4.19628424109712,-6.70635040568176,
122.972388404895));
#55908=CARTESIAN_POINT('Ctrl Pts',(-4.20831561679855,-6.69881363768957,
122.971810877096));
#55909=CARTESIAN_POINT('Ctrl Pts',(-4.21692602464757,-6.69339670002084,
122.971395911806));
#55910=CARTESIAN_POINT('Ctrl Pts',(-4.3067251245238,-6.63666067842869,122.967051140182));
#55911=CARTESIAN_POINT('Ctrl Pts',(-4.38698015261712,-6.58388562656992,
122.963022494602));
#55912=CARTESIAN_POINT('Ctrl Pts',(-4.46799128577512,-6.52847450135255,
122.958822245555));
#55913=CARTESIAN_POINT('Ctrl Pts',(-4.46973090975815,-6.52728358805647,
122.95873198606));
#55914=CARTESIAN_POINT('Ctrl Pts',(-4.47486210140349,-6.52376785921554,
122.958465568988));
#55915=CARTESIAN_POINT('Ctrl Pts',(-4.47825232899043,-6.52144109728049,
122.958289302421));
#55916=CARTESIAN_POINT('Ctrl Pts',(-4.48524972462477,-6.51663065457331,
122.957924992106));
#55917=CARTESIAN_POINT('Ctrl Pts',(-4.48885664675389,-6.51414661986824,
122.957736928731));
#55918=CARTESIAN_POINT('Ctrl Pts',(-4.50144104186227,-6.50546451514848,
122.95707983326));
#55919=CARTESIAN_POINT('Ctrl Pts',(-4.51040772566597,-6.49925089203213,
122.95660994656));
#55920=CARTESIAN_POINT('Ctrl Pts',(-4.54167226356457,-6.4774897122576,122.95496574359));
#55921=CARTESIAN_POINT('Ctrl Pts',(-4.56390263737819,-6.46184591355575,
122.953786269859));
#55922=CARTESIAN_POINT('Ctrl Pts',(-4.60732908589169,-6.43095028519993,
122.95146249307));
#55923=CARTESIAN_POINT('Ctrl Pts',(-4.62853118190996,-6.41570743964944,
122.950318646232));
#55924=CARTESIAN_POINT('Ctrl Pts',(-4.72320859996949,-6.34692731794189,
122.945170388786));
#55925=CARTESIAN_POINT('Ctrl Pts',(-4.79583164614981,-6.29223202403923,
122.941111666598));
#55926=CARTESIAN_POINT('Ctrl Pts',(-5.22253045967726,-5.95918930215106,
122.916680389774));
#55927=CARTESIAN_POINT('Ctrl Pts',(-5.55324910241791,-5.65227223508802,
122.89535686636));
#55928=CARTESIAN_POINT('Ctrl Pts',(-6.08953686390049,-5.06182358652705,
122.858407862712));
#55929=CARTESIAN_POINT('Ctrl Pts',(-6.30585488355206,-4.78964973631621,
122.842624683838));
#55930=CARTESIAN_POINT('Ctrl Pts',(-6.65567615128221,-4.2845351402578,122.815865347209));
#55931=CARTESIAN_POINT('Ctrl Pts',(-6.79654203363834,-4.0573762125847,122.804632354272));
#55932=CARTESIAN_POINT('Ctrl Pts',(-6.93478562452122,-3.80697073827943,
122.793071254846));
#55933=CARTESIAN_POINT('Ctrl Pts',(-6.94385658868818,-3.79040018237023,
122.792309882101));
#55934=CARTESIAN_POINT('Ctrl Pts',(-6.95679602863177,-3.76656047537226,
122.791219754553));
#55935=CARTESIAN_POINT('Ctrl Pts',(-6.96071261033063,-3.759317591738,122.790889248756));
#55936=CARTESIAN_POINT('Ctrl Pts',(-6.96748326292111,-3.7467498555765,122.790316956143));
#55937=CARTESIAN_POINT('Ctrl Pts',(-6.97034255148287,-3.74142783099522,
122.790074979957));
#55938=CARTESIAN_POINT('Ctrl Pts',(-6.97582342406232,-3.73119813385528,
122.7896105775));
#55939=CARTESIAN_POINT('Ctrl Pts',(-6.97844593176093,-3.7262909622612,122.78938811784));
#55940=CARTESIAN_POINT('Ctrl Pts',(-6.98460326355255,-3.71474021738282,
122.788865216846));
#55941=CARTESIAN_POINT('Ctrl Pts',(-6.98813379236155,-3.70809435321542,
122.788564930986));
#55942=CARTESIAN_POINT('Ctrl Pts',(-7.00026211755722,-3.68518516529812,
122.787531766979));
#55943=CARTESIAN_POINT('Ctrl Pts',(-7.00881269682523,-3.66889683744644,
122.786800593004));
#55944=CARTESIAN_POINT('Ctrl Pts',(-7.10153851085845,-3.49075271161947,
122.778840565128));
#55945=CARTESIAN_POINT('Ctrl Pts',(-7.18015041098444,-3.32605608849256,
122.771813868933));
#55946=CARTESIAN_POINT('Ctrl Pts',(-7.30469813288273,-3.04007721381244,
122.760104387756));
#55947=CARTESIAN_POINT('Ctrl Pts',(-7.35347459527433,-2.92011938333986,
122.755334783222));
#55948=CARTESIAN_POINT('Ctrl Pts',(-7.40426282111513,-2.78585910184103,
122.7501293237));
#55949=CARTESIAN_POINT('Ctrl Pts',(-7.40920455840562,-2.7726894295842,122.749620112209));
#55950=CARTESIAN_POINT('Ctrl Pts',(-7.446254215918,-2.67314617162757,122.745781519234));
#55951=CARTESIAN_POINT('Ctrl Pts',(-7.47688629920675,-2.58622968908943,
122.74248839436));
#55952=CARTESIAN_POINT('Ctrl Pts',(-7.69747606098773,-1.92361266243879,
122.717752633397));
#55953=CARTESIAN_POINT('Ctrl Pts',(-7.82219736372114,-1.32837152058472,
122.697793767267));
#55954=CARTESIAN_POINT('Ctrl Pts',(-7.89991731924511,-0.483608628044147,
122.667040804672));
#55955=CARTESIAN_POINT('Ctrl Pts',(-7.91101908225667,-0.241560065370663,
122.657921223825));
#55956=CARTESIAN_POINT('Ctrl Pts',(-7.91099898971197,0.0131177057046245,
122.647717697107));
#55957=CARTESIAN_POINT('Ctrl Pts',(-7.91096840802572,0.0256112072325062,
122.647215780486));
#55958=CARTESIAN_POINT('Ctrl Pts',(-7.91088074343932,0.0438113139206872,
122.646482655408));
#55959=CARTESIAN_POINT('Ctrl Pts',(-7.9108470804344,0.0495180560510775,
122.646252500751));
#55960=CARTESIAN_POINT('Ctrl Pts',(-7.91077671606195,0.0595975771277445,
122.645845502707));
#55961=CARTESIAN_POINT('Ctrl Pts',(-7.9107425639728,0.0639703761392062,
122.645668772545));
#55962=CARTESIAN_POINT('Ctrl Pts',(-7.91066440397266,0.0730173807747486,
122.645302797952));
#55963=CARTESIAN_POINT('Ctrl Pts',(-7.91061987890489,0.0776915794218354,
122.645113530867));
#55964=CARTESIAN_POINT('Ctrl Pts',(-7.91049517073094,0.089668804761709,
122.644628084037));
#55965=CARTESIAN_POINT('Ctrl Pts',(-7.9104090171749,0.0969717545807434,
122.644331645045));
#55966=CARTESIAN_POINT('Ctrl Pts',(-7.91001554117607,0.126821013156039,
122.643118223367));
#55967=CARTESIAN_POINT('Ctrl Pts',(-7.90962194002565,0.149365933678764,
122.642197560484));
#55968=CARTESIAN_POINT('Ctrl Pts',(-7.90629911262924,0.302241737802288,
122.635927560987));
#55969=CARTESIAN_POINT('Ctrl Pts',(-7.90024518235169,0.432480547795013,
122.630452965029));
#55970=CARTESIAN_POINT('Ctrl Pts',(-7.877415769931,0.752737674729313,122.616748103068));
#55971=CARTESIAN_POINT('Ctrl Pts',(-7.85698084752433,0.942412348686668,
122.608420909713));
#55972=CARTESIAN_POINT('Ctrl Pts',(-7.71230220748,1.9438579867356,122.563830673718));
#55973=CARTESIAN_POINT('Ctrl Pts',(-7.46904038444182,2.73349578421431,122.527179625295));
#55974=CARTESIAN_POINT('Ctrl Pts',(-7.08692234162318,3.51594849227904,122.491744644552));
#55975=CARTESIAN_POINT('Ctrl Pts',(-7.06482556210901,3.56014071777909,122.489743822403));
#55976=CARTESIAN_POINT('Ctrl Pts',(-7.03479674630671,3.61881584865546,122.487087263748));
#55977=CARTESIAN_POINT('Ctrl Pts',(-7.02723144802852,3.63348477180967,122.486423115339));
#55978=CARTESIAN_POINT('Ctrl Pts',(-7.01535042069485,3.65634588189986,122.485388019352));
#55979=CARTESIAN_POINT('Ctrl Pts',(-7.01106613528865,3.66455432219336,122.485016353029));
#55980=CARTESIAN_POINT('Ctrl Pts',(-7.0024648592051,3.68096356740355,122.484273341823));
#55981=CARTESIAN_POINT('Ctrl Pts',(-6.99814784646895,3.68916435096894,122.483901997374));
#55982=CARTESIAN_POINT('Ctrl Pts',(-6.98843768678979,3.70753181302431,122.483070256731));
#55983=CARTESIAN_POINT('Ctrl Pts',(-6.98303674050181,3.71769435651607,122.482610040309));
#55984=CARTESIAN_POINT('Ctrl Pts',(-6.96721239344636,3.74731366118479,122.481268643125));
#55985=CARTESIAN_POINT('Ctrl Pts',(-6.956729689726,3.76673867442626,122.480388835628));
#55986=CARTESIAN_POINT('Ctrl Pts',(-6.87969584823007,3.90806802665629,122.473986898395));
#55987=CARTESIAN_POINT('Ctrl Pts',(-6.81002478386326,4.02824710508736,122.468539409477));
#55988=CARTESIAN_POINT('Ctrl Pts',(-6.57231633488453,4.41447227471011,122.450992014207));
#55989=CARTESIAN_POINT('Ctrl Pts',(-6.39156777059872,4.67234231956193,122.439224261795));
#55990=CARTESIAN_POINT('Ctrl Pts',(-6.0061195887776,5.15787231355369,122.416484681092));
#55991=CARTESIAN_POINT('Ctrl Pts',(-5.8026226599834,5.38578599519231,122.405516736655));
#55992=CARTESIAN_POINT('Ctrl Pts',(-5.47051517116804,5.71700990823731,122.388514450244));
#55993=CARTESIAN_POINT('Ctrl Pts',(-5.35100357598925,5.82902202238421,122.382551593238));
#55994=CARTESIAN_POINT('Ctrl Pts',(-5.13530597928823,6.01895690236552,122.371922124156));
#55995=CARTESIAN_POINT('Ctrl Pts',(-5.0406068114037,6.09848271181901,122.367296989372));
#55996=CARTESIAN_POINT('Ctrl Pts',(-4.83044480169104,6.26673078797632,122.357043246888));
#55997=CARTESIAN_POINT('Ctrl Pts',(-4.71431939876835,6.35454963750633,122.35138416733));
#55998=CARTESIAN_POINT('Ctrl Pts',(-4.58475519957932,6.44702460868448,122.345009088054));
#55999=CARTESIAN_POINT('Ctrl Pts',(-4.573647696602,6.45490923941755,122.344462072423));
#56000=CARTESIAN_POINT('Ctrl Pts',(-4.55800643257105,6.46595150658281,122.343691031088));
#56001=CARTESIAN_POINT('Ctrl Pts',(-4.55348960134361,6.46913317030027,122.343468284786));
#56002=CARTESIAN_POINT('Ctrl Pts',(-4.54564168514022,6.47464896458877,122.343081108871));
#56003=CARTESIAN_POINT('Ctrl Pts',(-4.54231212270046,6.47698526509097,122.342916796037));
#56004=CARTESIAN_POINT('Ctrl Pts',(-4.53537718384896,6.4818434228822,122.342574453532));
#56005=CARTESIAN_POINT('Ctrl Pts',(-4.53177150336566,6.48436484165583,122.342396400234));
#56006=CARTESIAN_POINT('Ctrl Pts',(-4.52326980431445,6.49029944596295,122.34197643125));
#56007=CARTESIAN_POINT('Ctrl Pts',(-4.51837202765,6.49371009826778,122.341734377492));
#56008=CARTESIAN_POINT('Ctrl Pts',(-4.50232542696383,6.50485748524082,122.34094095447));
#56009=CARTESIAN_POINT('Ctrl Pts',(-4.49116059841535,6.51257104600539,122.340388308254));
#56010=CARTESIAN_POINT('Ctrl Pts',(-4.25703254554483,6.67343713728488,122.328785563534));
#56011=CARTESIAN_POINT('Ctrl Pts',(-4.02642181989327,6.81505428345463,122.317020456955));
#56012=CARTESIAN_POINT('Ctrl Pts',(-3.20754612325854,7.26184456429803,122.275176114511));
#56013=CARTESIAN_POINT('Ctrl Pts',(-2.5884750206989,7.50484344292046,122.243754729958));
#56014=CARTESIAN_POINT('Ctrl Pts',(-1.92317601439024,7.67371384821835,122.213486901719));
#56015=CARTESIAN_POINT('Ctrl Pts',(-1.90002473933197,7.67947890206059,122.212437475859));
#56016=CARTESIAN_POINT('Ctrl Pts',(-1.77601512153942,7.70976425557096,122.20683709894));
#56017=CARTESIAN_POINT('Ctrl Pts',(-1.67470558921842,7.73240304047764,122.202335790536));
#56018=CARTESIAN_POINT('Ctrl Pts',(-1.3733266573602,7.79354836239417,122.189173536629));
#56019=CARTESIAN_POINT('Ctrl Pts',(-1.17217746495979,7.8263293075822,122.18068661455));
#56020=CARTESIAN_POINT('Ctrl Pts',(-0.95117611264396,7.85363252483614,122.171684637346));
#56021=CARTESIAN_POINT('Ctrl Pts',(-0.932367800733935,7.85588760887096,
122.170921036352));
#56022=CARTESIAN_POINT('Ctrl Pts',(-0.90598174313536,7.85895515679507,122.169853283365));
#56023=CARTESIAN_POINT('Ctrl Pts',(-0.898410722442848,7.85982425055597,
122.169547313693));
#56024=CARTESIAN_POINT('Ctrl Pts',(-0.885285686308703,7.86131168970705,
122.169017585303));
#56025=CARTESIAN_POINT('Ctrl Pts',(-0.879732255837745,7.86193509177762,
122.168793664285));
#56026=CARTESIAN_POINT('Ctrl Pts',(-0.868191324210793,7.86321824127082,
122.168328768267));
#56027=CARTESIAN_POINT('Ctrl Pts',(-0.862203719349696,7.86387703565133,
122.168087824012));
#56028=CARTESIAN_POINT('Ctrl Pts',(-0.848131275867929,7.86540910988773,
122.167522129125));
#56029=CARTESIAN_POINT('Ctrl Pts',(-0.840045824628685,7.86627676477594,
122.167197559404));
#56030=CARTESIAN_POINT('Ctrl Pts',(-0.814138880182746,7.86901645652173,
122.166159045004));
#56031=CARTESIAN_POINT('Ctrl Pts',(-0.796312299321744,7.87084041489324,
122.165446645681));
#56032=CARTESIAN_POINT('Ctrl Pts',(-0.75465181987634,7.87495999643322,122.163786877156));
#56033=CARTESIAN_POINT('Ctrl Pts',(-0.730813335064466,7.87720802042438,
122.162841039141));
#56034=CARTESIAN_POINT('Ctrl Pts',(-0.489788201262861,7.89883370667428,
122.153316725506));
#56035=CARTESIAN_POINT('Ctrl Pts',(-0.271890820431771,7.90933313663197,
122.145028614522));
#56036=CARTESIAN_POINT('Ctrl Pts',(0.0663507461625947,7.91163458447523,
122.132559376718));
#56037=CARTESIAN_POINT('Ctrl Pts',(0.186533187647513,7.90971369851967,122.128205587216));
#56038=CARTESIAN_POINT('Ctrl Pts',(0.717179148423632,7.8891305639653,122.10924617128));
#56039=CARTESIAN_POINT('Ctrl Pts',(1.12587516059205,7.84124630562983,122.095381023819));
#56040=CARTESIAN_POINT('Ctrl Pts',(1.9985387475787,7.66934050286066,122.065174511261));
#56041=CARTESIAN_POINT('Ctrl Pts',(2.45867125354383,7.5344401071068,122.048855244614));
#56042=CARTESIAN_POINT('Ctrl Pts',(2.97557297852029,7.33047403139126,122.027412475692));
#56043=CARTESIAN_POINT('Ctrl Pts',(3.04698290774495,7.30108063940185,122.024377112767));
#56044=CARTESIAN_POINT('Ctrl Pts',(3.12586603544205,7.26725235127308,122.020930898447));
#56045=CARTESIAN_POINT('Ctrl Pts',(3.13377760587751,7.26384423872412,122.0205842109));
#56046=CARTESIAN_POINT('Ctrl Pts',(3.14559907277191,7.25872892972647,122.020064597731));
#56047=CARTESIAN_POINT('Ctrl Pts',(3.14951320023668,7.25703147321371,122.019892290609));
#56048=CARTESIAN_POINT('Ctrl Pts',(3.15625294838881,7.25410213792726,122.019595140919));
#56049=CARTESIAN_POINT('Ctrl Pts',(3.15907921921633,7.25287177526149,122.019470395469));
#56050=CARTESIAN_POINT('Ctrl Pts',(3.16493655608878,7.25031782304069,122.019211579493));
#56051=CARTESIAN_POINT('Ctrl Pts',(3.16796749746225,7.24899399048767,122.019077493817));
#56052=CARTESIAN_POINT('Ctrl Pts',(3.17507401028476,7.24588475116813,122.018762738764));
#56053=CARTESIAN_POINT('Ctrl Pts',(3.17914890382533,7.24409780753582,122.018581971494));
#56054=CARTESIAN_POINT('Ctrl Pts',(3.19233920023547,7.23830025671263,122.017995913402));
#56055=CARTESIAN_POINT('Ctrl Pts',(3.20144850619626,7.23427588885807,122.01758975346));
#56056=CARTESIAN_POINT('Ctrl Pts',(3.41222296996353,7.14068252060574,122.008159318141));
#56057=CARTESIAN_POINT('Ctrl Pts',(3.61004626403791,7.04273835772738,121.998619257022));
#56058=CARTESIAN_POINT('Ctrl Pts',(4.11488661174169,6.76592505130574,121.972971129971));
#56059=CARTESIAN_POINT('Ctrl Pts',(4.41441300108641,6.5744183991391,121.95644778251));
#56060=CARTESIAN_POINT('Ctrl Pts',(5.09911673693276,6.06869516498249,121.917037424049));
#56061=CARTESIAN_POINT('Ctrl Pts',(5.46961080371063,5.73702965473006,121.894374412123));
#56062=CARTESIAN_POINT('Ctrl Pts',(5.82116352830283,5.35709200687632,121.872242688405));
#56063=CARTESIAN_POINT('Ctrl Pts',(5.83564372284456,5.34131462683544,121.871329668968));
#56064=CARTESIAN_POINT('Ctrl Pts',(5.97007082082082,5.19364591571794,121.862840368074));
#56065=CARTESIAN_POINT('Ctrl Pts',(6.08559581346082,5.05778931317478,121.855447512981));
#56066=CARTESIAN_POINT('Ctrl Pts',(6.20773968387526,4.90389840289548,121.847514544748));
#56067=CARTESIAN_POINT('Ctrl Pts',(6.21899309682663,4.88961924859358,121.846782495844));
#56068=CARTESIAN_POINT('Ctrl Pts',(6.23478987736962,4.86943238194534,121.845753219815));
#56069=CARTESIAN_POINT('Ctrl Pts',(6.23937423024006,4.8635569034091,121.845454315077));
#56070=CARTESIAN_POINT('Ctrl Pts',(6.24733704117666,4.85332167850024,121.844934779275));
#56071=CARTESIAN_POINT('Ctrl Pts',(6.25071925119004,4.84896486520914,121.844713995054));
#56072=CARTESIAN_POINT('Ctrl Pts',(6.25776774235955,4.83986568142513,121.844253649861));
#56073=CARTESIAN_POINT('Ctrl Pts',(6.26143319628479,4.83512267271776,121.844014122655));
#56074=CARTESIAN_POINT('Ctrl Pts',(6.2699873445855,4.82402777193339,121.843454821852));
#56075=CARTESIAN_POINT('Ctrl Pts',(6.27487178740784,4.81767260175915,121.843135221216));
#56076=CARTESIAN_POINT('Ctrl Pts',(6.29069599459921,4.79701876512474,121.842099024715));
#56077=CARTESIAN_POINT('Ctrl Pts',(6.30159664599239,4.78269012651688,121.841384014736));
#56078=CARTESIAN_POINT('Ctrl Pts',(6.3270111805672,4.74904561638597,121.839714075018));
#56079=CARTESIAN_POINT('Ctrl Pts',(6.34148571191461,4.72970017280138,121.838760729592));
#56080=CARTESIAN_POINT('Ctrl Pts',(6.48880249365922,4.53091691157574,121.829034066761));
#56081=CARTESIAN_POINT('Ctrl Pts',(6.61408563806126,4.34599199150036,121.820566528056));
#56082=CARTESIAN_POINT('Ctrl Pts',(6.93768988768544,3.82185767977699,121.797905082628));
#56083=CARTESIAN_POINT('Ctrl Pts',(7.11883425924436,3.47280240196834,121.784298794586));
#56084=CARTESIAN_POINT('Ctrl Pts',(7.44091362066871,2.71997880553356,121.756241128683));
#56085=CARTESIAN_POINT('Ctrl Pts',(7.57658212731326,2.31534957153605,121.741857059236));
#56086=CARTESIAN_POINT('Ctrl Pts',(7.72735446450345,1.70656541446234,121.718929521799));
#56087=CARTESIAN_POINT('Ctrl Pts',(7.76823900840801,1.50957757846335,121.711313390728));
#56088=CARTESIAN_POINT('Ctrl Pts',(7.80359118598854,1.29924365815713,121.702775201048));
#56089=CARTESIAN_POINT('Ctrl Pts',(7.80558313897974,1.28722233456636,121.702285815255));
#56090=CARTESIAN_POINT('Ctrl Pts',(7.80827613409839,1.27073414123407,121.701612609798));
#56091=CARTESIAN_POINT('Ctrl Pts',(7.80900113784034,1.26627116880586,121.701430189888));
#56092=CARTESIAN_POINT('Ctrl Pts',(7.81023622266611,1.25862684197347,121.701117395825));
#56093=CARTESIAN_POINT('Ctrl Pts',(7.8107481864475,1.25544579693071,121.700987131961));
#56094=CARTESIAN_POINT('Ctrl Pts',(7.81174107534961,1.24925244726036,121.700733319945));
#56095=CARTESIAN_POINT('Ctrl Pts',(7.8122222018676,1.24624017503894,121.700609783458));
#56096=CARTESIAN_POINT('Ctrl Pts',(7.81336972546731,1.23902889752914,121.700313828573));
#56097=CARTESIAN_POINT('Ctrl Pts',(7.81403447957754,1.23482963505367,121.700141315867));
#56098=CARTESIAN_POINT('Ctrl Pts',(7.81601987538471,1.22222205494573,121.699622861715));
#56099=CARTESIAN_POINT('Ctrl Pts',(7.81733032918121,1.21381216314836,121.699276340863));
#56100=CARTESIAN_POINT('Ctrl Pts',(7.8286289516604,1.14052553452458,121.696250770049));
#56101=CARTESIAN_POINT('Ctrl Pts',(7.8378226091525,1.0755305889621,121.693527448176));
#56102=CARTESIAN_POINT('Ctrl Pts',(7.88313958171352,0.723634743299232,121.678595299931));
#56103=CARTESIAN_POINT('Ctrl Pts',(7.90431814033631,0.435048798668523,121.665683408695));
#56104=CARTESIAN_POINT('Ctrl Pts',(7.92028773737084,-0.430259446040728,
121.626222230339));
#56105=CARTESIAN_POINT('Ctrl Pts',(7.86791894076184,-1.0059962344632,121.599118911335));
#56106=CARTESIAN_POINT('Ctrl Pts',(7.72127117233947,-1.72978690912439,121.566453017165));
#56107=CARTESIAN_POINT('Ctrl Pts',(7.68421050449914,-1.88761859824214,121.559405528435));
#56108=CARTESIAN_POINT('Ctrl Pts',(7.59354626755409,-2.22656952633821,121.544461613735));
#56109=CARTESIAN_POINT('Ctrl Pts',(7.53825330531857,-2.4071352941949,121.536621868198));
#56110=CARTESIAN_POINT('Ctrl Pts',(7.47034455127823,-2.60350414456133,121.528223832656));
#56111=CARTESIAN_POINT('Ctrl Pts',(7.46407405902389,-2.6214270910041,121.527458495005));
#56112=CARTESIAN_POINT('Ctrl Pts',(7.45514821956075,-2.64664813121113,121.526383132741));
#56113=CARTESIAN_POINT('Ctrl Pts',(7.4525465863842,-2.65396508723531,121.52607134795));
#56114=CARTESIAN_POINT('Ctrl Pts',(7.44800286427662,-2.66668470085902,121.525529680322));
#56115=CARTESIAN_POINT('Ctrl Pts',(7.446065662357,-2.67208909135222,121.525299637277));
#56116=CARTESIAN_POINT('Ctrl Pts',(7.44201289248213,-2.68335684593689,121.52482023044));
#56117=CARTESIAN_POINT('Ctrl Pts',(7.43989627370082,-2.68921982948789,121.524570901358));
#56118=CARTESIAN_POINT('Ctrl Pts',(7.43493674177987,-2.70290694339625,121.523989126646));
#56119=CARTESIAN_POINT('Ctrl Pts',(7.43208840159596,-2.71072910677733,121.523656859655));
#56120=CARTESIAN_POINT('Ctrl Pts',(7.42281752280494,-2.73606450666283,121.522581366044));
#56121=CARTESIAN_POINT('Ctrl Pts',(7.41634536514838,-2.75355958576317,121.521839772259));
#56122=CARTESIAN_POINT('Ctrl Pts',(7.36285834336792,-2.89658528396057,121.515785700627));
#56123=CARTESIAN_POINT('Ctrl Pts',(7.31272061198845,-3.02092844213587,121.510577326969));
#56124=CARTESIAN_POINT('Ctrl Pts',(7.16793870968177,-3.3552337703441,121.496687269359));
#56125=CARTESIAN_POINT('Ctrl Pts',(7.06724763830835,-3.56243709419914,121.48820527525));
#56126=CARTESIAN_POINT('Ctrl Pts',(6.83539278860705,-3.99090536149231,121.470694839771));
#56127=CARTESIAN_POINT('Ctrl Pts',(6.70219325556437,-4.21076368456621,121.461728140067));
#56128=CARTESIAN_POINT('Ctrl Pts',(6.45665229432585,-4.5747955810532,121.446503393383));
#56129=CARTESIAN_POINT('Ctrl Pts',(6.34958781301564,-4.72227143418863,121.440218885865));
#56130=CARTESIAN_POINT('Ctrl Pts',(6.00223184329185,-5.16754041441322,121.420539185315));
#56131=CARTESIAN_POINT('Ctrl Pts',(5.7453854079956,-5.45167492711195,121.406962873621));
#56132=CARTESIAN_POINT('Ctrl Pts',(5.42462290209186,-5.75857304108338,121.389667667717));
#56133=CARTESIAN_POINT('Ctrl Pts',(5.37972980076654,-5.80053480440244,121.387239672802));
#56134=CARTESIAN_POINT('Ctrl Pts',(5.32745987636202,-5.84826293952433,121.384398229197));
#56135=CARTESIAN_POINT('Ctrl Pts',(5.32055515685786,-5.85454532526164,121.384022594869));
#56136=CARTESIAN_POINT('Ctrl Pts',(5.31032475933408,-5.86382059478943,121.383465583872));
#56137=CARTESIAN_POINT('Ctrl Pts',(5.30700761559721,-5.86682292091001,121.383284906498));
#56138=CARTESIAN_POINT('Ctrl Pts',(5.30112071032094,-5.87214204408134,121.382964132394));
#56139=CARTESIAN_POINT('Ctrl Pts',(5.29855197094898,-5.87445997368359,121.38282412016));
#56140=CARTESIAN_POINT('Ctrl Pts',(5.29313896155335,-5.87933802206616,121.382528985581));
#56141=CARTESIAN_POINT('Ctrl Pts',(5.29029436192597,-5.88189775566576,121.382373835826));
#56142=CARTESIAN_POINT('Ctrl Pts',(5.28276809049238,-5.88866044912273,121.381963201507));
#56143=CARTESIAN_POINT('Ctrl Pts',(5.2780832680002,-5.89285988282625,121.381707456557));
#56144=CARTESIAN_POINT('Ctrl Pts',(5.25683000380046,-5.91186544556353,121.380546624219));
#56145=CARTESIAN_POINT('Ctrl Pts',(5.24020437451017,-5.92660719388316,121.379636859479));
#56146=CARTESIAN_POINT('Ctrl Pts',(5.11568359582629,-6.03608470761905,121.372811990902));
#56147=CARTESIAN_POINT('Ctrl Pts',(5.00529424728843,-6.12793298147834,121.366700521332));
#56148=CARTESIAN_POINT('Ctrl Pts',(4.61161072482582,-6.43775638963521,121.344885223092));
#56149=CARTESIAN_POINT('Ctrl Pts',(4.31610407780815,-6.63949430205039,121.32849290198));
#56150=CARTESIAN_POINT('Ctrl Pts',(3.70230022648243,-7.00018620540454,121.295795048771));
#56151=CARTESIAN_POINT('Ctrl Pts',(3.38486776352805,-7.15907301267768,121.279530436843));
#56152=CARTESIAN_POINT('Ctrl Pts',(2.87541132958568,-7.37258806962727,121.255021681037));
#56153=CARTESIAN_POINT('Ctrl Pts',(2.69017660354091,-7.44217721421419,121.246414235522));
#56154=CARTESIAN_POINT('Ctrl Pts',(2.43550200956483,-7.5271004869822,121.235021806527));
#56155=CARTESIAN_POINT('Ctrl Pts',(2.3681869713717,-7.54854970042682,121.23205126208));
#56156=CARTESIAN_POINT('Ctrl Pts',(2.19563086339127,-7.60099735784208,121.224540417272));
#56157=CARTESIAN_POINT('Ctrl Pts',(2.09001450812166,-7.63071401228195,121.220041122402));
#56158=CARTESIAN_POINT('Ctrl Pts',(1.9677336511134,-7.66239003939273,121.214941806159));
#56159=CARTESIAN_POINT('Ctrl Pts',(1.95164283221605,-7.66650422926275,121.214272961597));
#56160=CARTESIAN_POINT('Ctrl Pts',(1.92790774631201,-7.67249338009361,121.213289545575));
#56161=CARTESIAN_POINT('Ctrl Pts',(1.92027349643221,-7.67440764132515,121.212973719226));
#56162=CARTESIAN_POINT('Ctrl Pts',(1.90666405947096,-7.67779858080349,121.21241156025));
#56163=CARTESIAN_POINT('Ctrl Pts',(1.90068998745135,-7.67927968333541,121.212165086533));
#56164=CARTESIAN_POINT('Ctrl Pts',(1.888205105117,-7.68235949610116,121.211650608599));
#56165=CARTESIAN_POINT('Ctrl Pts',(1.88169397724214,-7.68395690530725,121.211382646058));
#56166=CARTESIAN_POINT('Ctrl Pts',(1.86850471379202,-7.68717492699112,121.210840551327));
#56167=CARTESIAN_POINT('Ctrl Pts',(1.86182648098654,-7.68879511878323,121.210566432733));
#56168=CARTESIAN_POINT('Ctrl Pts',(1.8341065080344,-7.69548196946485,121.209430131718));
#56169=CARTESIAN_POINT('Ctrl Pts',(1.81304603809453,-7.7004709919821,121.208570424355));
#56170=CARTESIAN_POINT('Ctrl Pts',(1.59939765043249,-7.75015716026447,121.199885236114));
#56171=CARTESIAN_POINT('Ctrl Pts',(1.40521242755915,-7.78770784373213,121.192291093556));
#56172=CARTESIAN_POINT('Ctrl Pts',(0.918508583447293,-7.86302451954987,
121.173881856097));
#56173=CARTESIAN_POINT('Ctrl Pts',(0.624900715665895,-7.8917884899893,121.163336769281));
#56174=CARTESIAN_POINT('Ctrl Pts',(-0.412867854801866,-7.93516317003822,
121.127030017453));
#56175=CARTESIAN_POINT('Ctrl Pts',(-1.15664239592262,-7.86124231507165,
121.103009621466));
#56176=CARTESIAN_POINT('Ctrl Pts',(-1.92117657731123,-7.67430028416338,
121.072079164334));
#56177=CARTESIAN_POINT('Ctrl Pts',(-1.96324533251526,-7.6636461248158,121.070355601954));
#56178=CARTESIAN_POINT('Ctrl Pts',(-2.01239957239572,-7.65076623559946,
121.068314236314));
#56179=CARTESIAN_POINT('Ctrl Pts',(-2.0195729127643,-7.64887581806204,121.068015640901));
#56180=CARTESIAN_POINT('Ctrl Pts',(-2.03103035652773,-7.64583915331536,
121.067537602108));
#56181=CARTESIAN_POINT('Ctrl Pts',(-2.03531618608657,-7.64469938519352,
121.067358535107));
#56182=CARTESIAN_POINT('Ctrl Pts',(-2.04288747383055,-7.64267906816102,
121.067041753555));
#56183=CARTESIAN_POINT('Ctrl Pts',(-2.04617333010059,-7.64180000214327,
121.066904125886));
#56184=CARTESIAN_POINT('Ctrl Pts',(-2.05297345229626,-7.63997606325084,
121.066618995548));
#56185=CARTESIAN_POINT('Ctrl Pts',(-2.05648763451495,-7.63903088433876,
121.066471474856));
#56186=CARTESIAN_POINT('Ctrl Pts',(-2.06551375459497,-7.636596527822,121.066092129709));
#56187=CARTESIAN_POINT('Ctrl Pts',(-2.07102468903805,-7.63510381960646,
121.065860095625));
#56188=CARTESIAN_POINT('Ctrl Pts',(-2.0943338691581,-7.62876313199913,121.06487688757));
#56189=CARTESIAN_POINT('Ctrl Pts',(-2.11211658491264,-7.62385891792775,
121.064122381269));
#56190=CARTESIAN_POINT('Ctrl Pts',(-2.23506160015944,-7.5894893094451,121.058876221857));
#56191=CARTESIAN_POINT('Ctrl Pts',(-2.33961690560369,-7.55791234776072,
121.054264264876));
#56192=CARTESIAN_POINT('Ctrl Pts',(-2.66094247323907,-7.45356177994734,
121.039699538887));
#56193=CARTESIAN_POINT('Ctrl Pts',(-2.87522972530162,-7.37355007618528,
121.029431187133));
#56194=CARTESIAN_POINT('Ctrl Pts',(-3.30689585474702,-7.19069178779376,
121.008017501065));
#56195=CARTESIAN_POINT('Ctrl Pts',(-3.52367006988198,-7.0869849497371,120.996866064828));
#56196=CARTESIAN_POINT('Ctrl Pts',(-3.84324873672381,-6.91580307121205,
120.980102827979));
#56197=CARTESIAN_POINT('Ctrl Pts',(-3.94975566060977,-6.85553234873503,
120.974458274201));
#56198=CARTESIAN_POINT('Ctrl Pts',(-4.18465885537609,-6.71531200965327,
120.961921135795));
#56199=CARTESIAN_POINT('Ctrl Pts',(-4.31224909661232,-6.63410092024267,
120.955050887824));
#56200=CARTESIAN_POINT('Ctrl Pts',(-4.57673142187179,-6.45490208768314,
120.94073562544));
#56201=CARTESIAN_POINT('Ctrl Pts',(-4.71298454998941,-6.35610039430935,
120.933317018692));
#56202=CARTESIAN_POINT('Ctrl Pts',(-4.85431967852244,-6.24656806247061,
120.925595967097));
#56203=CARTESIAN_POINT('Ctrl Pts',(-4.8626381582432,-6.24009473032769,120.925141430621));
#56204=CARTESIAN_POINT('Ctrl Pts',(-5.04942175880539,-6.09414187730191,
120.914932986074));
#56205=CARTESIAN_POINT('Ctrl Pts',(-5.22183613861035,-5.94707189871628,
120.905468238983));
#56206=CARTESIAN_POINT('Ctrl Pts',(-5.401897692818,-5.77960185808028,120.895534300931));
#56207=CARTESIAN_POINT('Ctrl Pts',(-5.41603520152699,-5.7663557837307,120.894753958288));
#56208=CARTESIAN_POINT('Ctrl Pts',(-5.43569344783515,-5.74780100512732,
120.893668327003));
#56209=CARTESIAN_POINT('Ctrl Pts',(-5.44125529145944,-5.74253606927912,
120.893361109616));
#56210=CARTESIAN_POINT('Ctrl Pts',(-5.45084796561571,-5.7334290319795,120.892831130927));
#56211=CARTESIAN_POINT('Ctrl Pts',(-5.4548823963522,-5.72959074028389,120.892608201294));
#56212=CARTESIAN_POINT('Ctrl Pts',(-5.4632247945004,-5.72163712053802,120.892147155015));
#56213=CARTESIAN_POINT('Ctrl Pts',(-5.46753217341492,-5.71752117855677,
120.891909065839));
#56214=CARTESIAN_POINT('Ctrl Pts',(-5.47605691446778,-5.70935686787689,
120.891437782357));
#56215=CARTESIAN_POINT('Ctrl Pts',(-5.48027444664626,-5.70530868270013,
120.891204580167));
#56216=CARTESIAN_POINT('Ctrl Pts',(-5.49003737973757,-5.69591694759352,
120.890664660423));
#56217=CARTESIAN_POINT('Ctrl Pts',(-5.49557947735191,-5.6905699638392,120.890358096066));
#56218=CARTESIAN_POINT('Ctrl Pts',(-5.52582253257544,-5.66130625246897,
120.88868479371));
#56219=CARTESIAN_POINT('Ctrl Pts',(-5.55037536504422,-5.6372366006608,120.887324900041));
#56220=CARTESIAN_POINT('Ctrl Pts',(-5.77264199520862,-5.4164840876372,120.874999746493));
#56221=CARTESIAN_POINT('Ctrl Pts',(-5.95999096563526,-5.2096276781117,120.864515327959));
#56222=CARTESIAN_POINT('Ctrl Pts',(-6.23458264255635,-4.87219426990906,
120.848735903576));
#56223=CARTESIAN_POINT('Ctrl Pts',(-6.32952492460112,-4.74820113940357,
120.843189448095));
#56224=CARTESIAN_POINT('Ctrl Pts',(-6.87364290614378,-3.99224389957678,
120.810567887238));
#56225=CARTESIAN_POINT('Ctrl Pts',(-7.23151145011653,-3.29997431842656,
120.785931279604));
#56226=CARTESIAN_POINT('Ctrl Pts',(-7.49733648154149,-2.52503925339601,
120.753753275093));
#56227=CARTESIAN_POINT('Ctrl Pts',(-7.51133728667385,-2.48308066140297,
120.751996466743));
#56228=CARTESIAN_POINT('Ctrl Pts',(-7.52723972002103,-2.43405763749413,
120.7499246011));
#56229=CARTESIAN_POINT('Ctrl Pts',(-7.52948457516554,-2.42710453359414,
120.749630291228));
#56230=CARTESIAN_POINT('Ctrl Pts',(-7.53304477993711,-2.41602485548254,
120.749160581224));
#56231=CARTESIAN_POINT('Ctrl Pts',(-7.53436638296822,-2.41190028107878,
120.748985563481));
#56232=CARTESIAN_POINT('Ctrl Pts',(-7.53668909986274,-2.40463080423764,
120.748676810942));
#56233=CARTESIAN_POINT('Ctrl Pts',(-7.53769163516902,-2.40148635343119,
120.748543163705));
#56234=CARTESIAN_POINT('Ctrl Pts',(-7.53975971560277,-2.39498576823043,
120.748266674712));
#56235=CARTESIAN_POINT('Ctrl Pts',(-7.54082498410571,-2.3916295611969,120.748123816385));
#56236=CARTESIAN_POINT('Ctrl Pts',(-7.54356506636366,-2.38297669923729,
120.747755223943));
#56237=CARTESIAN_POINT('Ctrl Pts',(-7.54523653901415,-2.3776790005352,120.747529284077));
#56238=CARTESIAN_POINT('Ctrl Pts',(-7.55217770718717,-2.35559808235918,
120.746586451675));
#56239=CARTESIAN_POINT('Ctrl Pts',(-7.55739695902635,-2.33879918774146,
120.745866484908));
#56240=CARTESIAN_POINT('Ctrl Pts',(-7.59239735959962,-2.22480497897762,
120.740963531655));
#56241=CARTESIAN_POINT('Ctrl Pts',(-7.62035756342835,-2.12706459226016,
120.736674124732));
#56242=CARTESIAN_POINT('Ctrl Pts',(-7.82192065062473,-1.36739168276504,
120.702828987298));
#56243=CARTESIAN_POINT('Ctrl Pts',(-7.9108511900503,-0.686017634366207,
120.669782581568));
#56244=CARTESIAN_POINT('Ctrl Pts',(-7.91099981341223,-0.00171819428687214,
120.63838888384));
#56245=CARTESIAN_POINT('',(-7.91183059010191,0.0010273813645225,118.643768829136));
#56246=CARTESIAN_POINT('Ctrl Pts',(-7.911,6.17617068598975E-12,120.642331508237));
#56247=CARTESIAN_POINT('Ctrl Pts',(-7.91099999999828,2.20167589667282,120.553744072504));
#56248=CARTESIAN_POINT('Ctrl Pts',(-6.9421457667204,4.38610418339201,120.465156636771));
#56249=CARTESIAN_POINT('Ctrl Pts',(-3.67820201487755,7.34180684107895,120.287981765306));
#56250=CARTESIAN_POINT('Ctrl Pts',(-1.40868175871174,8.08992666571432,120.199394329573));
#56251=CARTESIAN_POINT('Ctrl Pts',(2.9730927052179,7.65454228025053,120.022219458108));
#56252=CARTESIAN_POINT('Ctrl Pts',(5.05102072676026,6.47444880833891,119.933632022375));
#56253=CARTESIAN_POINT('Ctrl Pts',(7.66951518848053,2.93425195367223,119.75645715091));
#56254=CARTESIAN_POINT('Ctrl Pts',(8.18956872247105,0.601881960094159,119.667869715177));
#56255=CARTESIAN_POINT('Ctrl Pts',(7.32306689761123,-3.71537198232875,119.490694843711));
#56256=CARTESIAN_POINT('Ctrl Pts',(5.94329958849879,-5.66643518936844,119.402107407979));
#56257=CARTESIAN_POINT('Ctrl Pts',(2.16154501637422,-7.92205913233111,119.224932536513));
#56258=CARTESIAN_POINT('Ctrl Pts',(-0.210816529304628,-8.20894963712988,
119.136345100781));
#56259=CARTESIAN_POINT('Ctrl Pts',(-4.42123908576775,-6.91982244717612,
118.959170229315));
#56260=CARTESIAN_POINT('Ctrl Pts',(-6.22631625634439,-5.35390358803224,
118.870582793582));
#56261=CARTESIAN_POINT('Ctrl Pts',(-7.65317280859622,-2.3133485751411,118.735440741312));
#56262=CARTESIAN_POINT('Ctrl Pts',(-7.91100000000081,-1.15702837836028,
118.688886124774));
#56263=CARTESIAN_POINT('Ctrl Pts',(-7.911,5.55555601522428E-12,118.642331508237));
#56264=CARTESIAN_POINT('',(-7.9109991690038,0.00362602002780672,116.642331508237));
#56265=CARTESIAN_POINT('Ctrl Pts',(-7.91099779079968,0.00591218762721216,
118.642331508237));
#56266=CARTESIAN_POINT('Ctrl Pts',(-7.91083671603242,0.221443596363675,
118.633703450411));
#56267=CARTESIAN_POINT('Ctrl Pts',(-7.90186360606107,0.436646946205818,
118.625075392585));
#56268=CARTESIAN_POINT('Ctrl Pts',(-7.88418278797969,0.650832363765712,
118.616447334758));
#56269=CARTESIAN_POINT('Ctrl Pts',(-7.86640982052795,0.866134078731944,
118.607774308985));
#56270=CARTESIAN_POINT('Ctrl Pts',(-7.83983822169058,1.08040700633278,118.599101283211));
#56271=CARTESIAN_POINT('Ctrl Pts',(-7.80462415415228,1.29296667104098,118.590428257438));
#56272=CARTESIAN_POINT('Ctrl Pts',(-7.76931804459715,1.50608192110483,118.581732562236));
#56273=CARTESIAN_POINT('Ctrl Pts',(-7.72532433869049,1.71747473790199,118.573036867034));
#56274=CARTESIAN_POINT('Ctrl Pts',(-7.67284929109888,1.92647469645552,118.564341171832));
#56275=CARTESIAN_POINT('Ctrl Pts',(-7.62016465055611,2.13630943115729,118.555610744762));
#56276=CARTESIAN_POINT('Ctrl Pts',(-7.55893089031879,2.34373195410072,118.546880317692));
#56277=CARTESIAN_POINT('Ctrl Pts',(-7.48940430250673,2.54808637875438,118.538149890622));
#56278=CARTESIAN_POINT('Ctrl Pts',(-7.42977915574986,2.72333822044306,118.530662783723));
#56279=CARTESIAN_POINT('Ctrl Pts',(-7.36405581900405,2.89633391464973,118.523175676823));
#56280=CARTESIAN_POINT('Ctrl Pts',(-7.29242264774207,3.06667457137181,118.515688569924));
#56281=CARTESIAN_POINT('Ctrl Pts',(-7.216669252574,3.24681294657604,118.507770816771));
#56282=CARTESIAN_POINT('Ctrl Pts',(-7.13413070695464,3.42439597308405,118.499853063618));
#56283=CARTESIAN_POINT('Ctrl Pts',(-7.04499911081336,3.59887600906713,118.491935310466));
#56284=CARTESIAN_POINT('Ctrl Pts',(-6.95596992046277,3.77315558004322,118.484026654241));
#56285=CARTESIAN_POINT('Ctrl Pts',(-6.86036292271164,3.94433895788806,118.476117998017));
#56286=CARTESIAN_POINT('Ctrl Pts',(-6.75841884047851,4.11189685870951,118.468209341793));
#56287=CARTESIAN_POINT('Ctrl Pts',(-6.65657301338832,4.2792932648651,118.460308308043));
#56288=CARTESIAN_POINT('Ctrl Pts',(-6.54840244666605,4.44307086265501,118.452407274293));
#56289=CARTESIAN_POINT('Ctrl Pts',(-6.43419461001667,4.60272318529286,118.444506240544));
#56290=CARTESIAN_POINT('Ctrl Pts',(-6.32007571442572,4.76225117630012,118.436611359842));
#56291=CARTESIAN_POINT('Ctrl Pts',(-6.19992911548144,4.91766001388852,118.42871647914));
#56292=CARTESIAN_POINT('Ctrl Pts',(-6.07408673908301,5.06847031027073,118.420821598438));
#56293=CARTESIAN_POINT('Ctrl Pts',(-5.94831908319837,5.21919106111867,118.412931405422));
#56294=CARTESIAN_POINT('Ctrl Pts',(-5.81686260878021,5.36531844774603,118.405041212406));
#56295=CARTESIAN_POINT('Ctrl Pts',(-5.68009101375787,5.50640418743731,118.397151019391));
#56296=CARTESIAN_POINT('Ctrl Pts',(-5.5433753302584,5.64743225200561,118.389264051845));
#56297=CARTESIAN_POINT('Ctrl Pts',(-5.40134909585611,5.78342253022632,118.381377084299));
#56298=CARTESIAN_POINT('Ctrl Pts',(-5.25442472713145,5.91396159836278,118.373490116754));
#56299=CARTESIAN_POINT('Ctrl Pts',(-5.10751311778582,6.04448933007176,118.365603834137));
#56300=CARTESIAN_POINT('Ctrl Pts',(-4.95570447470364,6.16956656137185,118.357717551521));
#56301=CARTESIAN_POINT('Ctrl Pts',(-4.79944672457402,6.28881802391958,118.349831268905));
#56302=CARTESIAN_POINT('Ctrl Pts',(-4.64318924908982,6.40806927686574,118.34194500015));
#56303=CARTESIAN_POINT('Ctrl Pts',(-4.48248295573017,6.52149457197276,118.334058731395));
#56304=CARTESIAN_POINT('Ctrl Pts',(-4.31780745996508,6.62876004533803,118.32617246264));
#56305=CARTESIAN_POINT('Ctrl Pts',(-4.1531046531704,6.73604330842061,118.318284885966));
#56306=CARTESIAN_POINT('Ctrl Pts',(-3.98443162102727,6.83716452613187,118.310397309293));
#56307=CARTESIAN_POINT('Ctrl Pts',(-3.81229566226637,6.93183401297702,118.302509732619));
#56308=CARTESIAN_POINT('Ctrl Pts',(-3.6401023041762,7.02653506768913,118.294619525806));
#56309=CARTESIAN_POINT('Ctrl Pts',(-3.46444402041368,7.11477993907158,118.286729318993));
#56310=CARTESIAN_POINT('Ctrl Pts',(-3.2858515401473,7.19632549681514,118.27883911218));
#56311=CARTESIAN_POINT('Ctrl Pts',(-3.10708660003226,7.27794979994891,118.270941286099));
#56312=CARTESIAN_POINT('Ctrl Pts',(-2.92538211741085,7.35286172449167,118.263043460019));
#56313=CARTESIAN_POINT('Ctrl Pts',(-2.7412885612694,7.42086639307389,118.255145633938));
#56314=CARTESIAN_POINT('Ctrl Pts',(-2.55709306904711,7.48890871712619,118.247243434682));
#56315=CARTESIAN_POINT('Ctrl Pts',(-2.37050619243673,7.55003605246322,118.239341235426));
#56316=CARTESIAN_POINT('Ctrl Pts',(-2.18209257317945,7.60410369485287,118.23143903617));
#56317=CARTESIAN_POINT('Ctrl Pts',(-1.9934515243977,7.65823660098645,118.22352729836));
#56318=CARTESIAN_POINT('Ctrl Pts',(-1.80297966214709,7.70529271029314,118.21561556055));
#56319=CARTESIAN_POINT('Ctrl Pts',(-1.61125187231184,7.74517839716889,118.207703822741));
#56320=CARTESIAN_POINT('Ctrl Pts',(-1.53194107755394,7.76167765128483,118.204431025333));
#56321=CARTESIAN_POINT('Ctrl Pts',(-1.45241543903234,7.77695053402871,118.201158227925));
#56322=CARTESIAN_POINT('Ctrl Pts',(-1.37271584731438,7.79099301774376,118.197885430517));
#56323=CARTESIAN_POINT('Ctrl Pts',(-1.17023137710682,7.82666929680805,118.189570574255));
#56324=CARTESIAN_POINT('Ctrl Pts',(-0.966181923830737,7.85447815505976,
118.181255717993));
#56325=CARTESIAN_POINT('Ctrl Pts',(-0.761191861567461,7.87429412391253,
118.172940861731));
#56326=CARTESIAN_POINT('Ctrl Pts',(-0.556454237440179,7.89408569008849,
118.164636244926));
#56327=CARTESIAN_POINT('Ctrl Pts',(-0.350778605037622,7.90590397008626,
118.156331628121));
#56328=CARTESIAN_POINT('Ctrl Pts',(-0.144798034947215,7.90967474230612,
118.148027011316));
#56329=CARTESIAN_POINT('Ctrl Pts',(0.0609424639345085,7.91344111967532,
118.139732073576));
#56330=CARTESIAN_POINT('Ctrl Pts',(0.266986899509766,7.90917869147408,118.131437135836));
#56331=CARTESIAN_POINT('Ctrl Pts',(0.472697746957,7.89686506406319,118.123142198096));
#56332=CARTESIAN_POINT('Ctrl Pts',(0.678100272093222,7.88456989249023,118.114859692925));
#56333=CARTESIAN_POINT('Ctrl Pts',(0.883169915056289,7.86424762120578,118.106577187755));
#56334=CARTESIAN_POINT('Ctrl Pts',(1.08726973854097,7.83592786564891,118.098294682584));
#56335=CARTESIAN_POINT('Ctrl Pts',(1.29118206726784,7.8076341258211,118.090019786074));
#56336=CARTESIAN_POINT('Ctrl Pts',(1.49412606370222,7.77135759262824,118.081744889564));
#56337=CARTESIAN_POINT('Ctrl Pts',(1.69546867099022,7.72717975626882,118.073469993054));
#56338=CARTESIAN_POINT('Ctrl Pts',(1.89658096874354,7.68305245355984,118.065204561941));
#56339=CARTESIAN_POINT('Ctrl Pts',(2.09609524681368,7.63104194528221,118.056939130827));
#56340=CARTESIAN_POINT('Ctrl Pts',(2.29338713114806,7.5712810320767,118.048673699713));
#56341=CARTESIAN_POINT('Ctrl Pts',(2.37048440328183,7.54792779885116,118.045443753413));
#56342=CARTESIAN_POINT('Ctrl Pts',(2.44724239369957,7.52339157676419,118.042213807113));
#56343=CARTESIAN_POINT('Ctrl Pts',(2.52362426201262,7.49768241419849,118.038983860813));
#56344=CARTESIAN_POINT('Ctrl Pts',(2.71911236414118,7.43188361262053,118.030717290668));
#56345=CARTESIAN_POINT('Ctrl Pts',(2.91191542388773,7.35847235377821,118.022450720523));
#56346=CARTESIAN_POINT('Ctrl Pts',(3.10144646655632,7.27770230327439,118.014184150378));
#56347=CARTESIAN_POINT('Ctrl Pts',(3.2911473312336,7.19685988187013,118.00591017329));
#56348=CARTESIAN_POINT('Ctrl Pts',(3.47757005578809,7.10864562070118,117.997636196203));
#56349=CARTESIAN_POINT('Ctrl Pts',(3.66015070824269,7.01335995033411,117.989362219115));
#56350=CARTESIAN_POINT('Ctrl Pts',(3.84290680617902,6.91798271801832,117.981080291394));
#56351=CARTESIAN_POINT('Ctrl Pts',(4.02181320126577,6.81552064636116,117.972798363673));
#56352=CARTESIAN_POINT('Ctrl Pts',(4.19633275112753,6.70631884432991,117.964516435952));
#56353=CARTESIAN_POINT('Ctrl Pts',(4.37114158767991,6.59693602746139,117.956220779961));
#56354=CARTESIAN_POINT('Ctrl Pts',(4.54154879166722,6.48079130082324,117.94792512397));
#56355=CARTESIAN_POINT('Ctrl Pts',(4.70704661993294,6.35827280932314,117.939629467979));
#56356=CARTESIAN_POINT('Ctrl Pts',(4.87269402620684,6.23564358481755,117.93132631432));
#56357=CARTESIAN_POINT('Ctrl Pts',(5.03342296815703,6.10662927642654,117.923023160661));
#56358=CARTESIAN_POINT('Ctrl Pts',(5.18875974805491,5.97165749829686,117.914720007003));
#56359=CARTESIAN_POINT('Ctrl Pts',(5.34433336011951,5.83647993723102,117.906404194051));
#56360=CARTESIAN_POINT('Ctrl Pts',(5.49449816012126,5.69532694839535,117.898088381099));
#56361=CARTESIAN_POINT('Ctrl Pts',(5.63881685028556,5.54866340021952,117.889772568147));
#56362=CARTESIAN_POINT('Ctrl Pts',(5.69487423146808,5.49169521116297,117.886542475801));
#56363=CARTESIAN_POINT('Ctrl Pts',(5.75005000122328,5.43389596882698,117.883312383455));
#56364=CARTESIAN_POINT('Ctrl Pts',(5.80432019090631,5.37529423580117,117.880082291109));
#56365=CARTESIAN_POINT('Ctrl Pts',(5.93723577686808,5.23177007034328,117.872171325266));
#56366=CARTESIAN_POINT('Ctrl Pts',(6.06499253895526,5.08313191158827,117.864260359422));
#56367=CARTESIAN_POINT('Ctrl Pts',(6.18717483688316,4.9297858511136,117.856349393579));
#56368=CARTESIAN_POINT('Ctrl Pts',(6.30923349761745,4.77659496268013,117.848446432902));
#56369=CARTESIAN_POINT('Ctrl Pts',(6.42572871750585,4.61870592930406,117.840543472226));
#56370=CARTESIAN_POINT('Ctrl Pts',(6.53628214802461,4.45656108242834,117.832640511549));
#56371=CARTESIAN_POINT('Ctrl Pts',(6.64674416788173,4.29455030437041,117.824744085403));
#56372=CARTESIAN_POINT('Ctrl Pts',(6.75127399285098,4.12829100613005,117.816847659258));
#56373=CARTESIAN_POINT('Ctrl Pts',(6.8495338025682,3.95825816331826,117.808951233112));
#56374=CARTESIAN_POINT('Ctrl Pts',(6.94773054572438,3.78833445349471,117.801059875168));
#56375=CARTESIAN_POINT('Ctrl Pts',(7.03966512005126,3.61464232196076,117.793168517223));
#56376=CARTESIAN_POINT('Ctrl Pts',(7.12504311495439,3.43768550190984,117.785277159278));
#56377=CARTESIAN_POINT('Ctrl Pts',(7.21038210406012,3.26080952636549,117.77738940658));
#56378=CARTESIAN_POINT('Ctrl Pts',(7.28917033346571,3.08067214410774,117.769501653882));
#56379=CARTESIAN_POINT('Ctrl Pts',(7.36115930315627,2.89780170362913,117.761613901183));
#56380=CARTESIAN_POINT('Ctrl Pts',(7.4331286981632,2.71498098786575,117.753728293262));
#56381=CARTESIAN_POINT('Ctrl Pts',(7.49830239240097,2.52942901533257,117.74584268534));
#56382=CARTESIAN_POINT('Ctrl Pts',(7.55647989391253,2.34169438930355,117.737957077419));
#56383=CARTESIAN_POINT('Ctrl Pts',(7.61466425695561,2.15393762160428,117.730070539458));
#56384=CARTESIAN_POINT('Ctrl Pts',(7.66585067006356,1.96399801311556,117.722184001497));
#56385=CARTESIAN_POINT('Ctrl Pts',(7.70988823705659,1.77244023089536,117.714297463537));
#56386=CARTESIAN_POINT('Ctrl Pts',(7.75393135195071,1.58085831601523,117.706409932021));
#56387=CARTESIAN_POINT('Ctrl Pts',(7.79082374821383,1.38765815696165,117.698522400506));
#56388=CARTESIAN_POINT('Ctrl Pts',(7.82046548532773,1.19341551556772,117.690634868991));
#56389=CARTESIAN_POINT('Ctrl Pts',(7.85011592503815,0.999115845959503,117.682745021754));
#56390=CARTESIAN_POINT('Ctrl Pts',(7.87251141148446,0.80377342468765,117.674855174517));
#56391=CARTESIAN_POINT('Ctrl Pts',(7.88760376240749,0.607970301293734,117.66696532728));
#56392=CARTESIAN_POINT('Ctrl Pts',(7.90270307404301,0.412076871939257,117.659071841183));
#56393=CARTESIAN_POINT('Ctrl Pts',(7.91049251161675,0.215722660212971,117.651178355086));
#56394=CARTESIAN_POINT('Ctrl Pts',(7.91097598880074,0.0194911420416452,
117.643284868989));
#56395=CARTESIAN_POINT('Ctrl Pts',(7.9114600248837,-0.176967219493072,117.635382258033));
#56396=CARTESIAN_POINT('Ctrl Pts',(7.90462123006718,-0.373302259600198,
117.627479647077));
#56397=CARTESIAN_POINT('Ctrl Pts',(7.8905155855907,-0.568933030813101,117.619577036121));
#56398=CARTESIAN_POINT('Ctrl Pts',(7.87640058548218,-0.764693555013525,
117.611669183722));
#56399=CARTESIAN_POINT('Ctrl Pts',(7.85500916458256,-0.959748537756036,
117.603761331324));
#56400=CARTESIAN_POINT('Ctrl Pts',(7.82644873420673,-1.15352555707879,117.595853478925));
#56401=CARTESIAN_POINT('Ctrl Pts',(7.79784922506148,-1.3475677183254,117.587934806342));
#56402=CARTESIAN_POINT('Ctrl Pts',(7.76206117628894,-1.54032808603793,117.580016133759));
#56403=CARTESIAN_POINT('Ctrl Pts',(7.7192425890873,-1.73124661756229,117.572097461175));
#56404=CARTESIAN_POINT('Ctrl Pts',(7.70154576191687,-1.81015282341411,117.568824691351));
#56405=CARTESIAN_POINT('Ctrl Pts',(7.68264859531561,-1.88874461788705,117.565551921526));
#56406=CARTESIAN_POINT('Ctrl Pts',(7.66256466949527,-1.96698339743956,117.562279151701));
#56407=CARTESIAN_POINT('Ctrl Pts',(7.61443390925768,-2.15448119909491,117.554436018783));
#56408=CARTESIAN_POINT('Ctrl Pts',(7.55934159075306,-2.34050541276033,117.546592885864));
#56409=CARTESIAN_POINT('Ctrl Pts',(7.49738959448499,-2.52449406188809,117.538749752945));
#56410=CARTESIAN_POINT('Ctrl Pts',(7.43551035424263,-2.70826663593039,117.530915830951));
#56411=CARTESIAN_POINT('Ctrl Pts',(7.36678758798236,-2.89000807604153,117.523081908957));
#56412=CARTESIAN_POINT('Ctrl Pts',(7.29137408996509,-3.06916680553301,117.515247986962));
#56413=CARTESIAN_POINT('Ctrl Pts',(7.216034490447,-3.24814997545531,117.507421741513));
#56414=CARTESIAN_POINT('Ctrl Pts',(7.1340173508897,-3.42455515323873,117.499595496063));
#56415=CARTESIAN_POINT('Ctrl Pts',(7.04552521067031,-3.59784595359628,117.491769250614));
#56416=CARTESIAN_POINT('Ctrl Pts',(6.95710258478053,-3.77100062667987,117.483949153012));
#56417=CARTESIAN_POINT('Ctrl Pts',(6.86221524779078,-3.9410454834532,117.47612905541));
#56418=CARTESIAN_POINT('Ctrl Pts',(6.76111385728658,-4.10746398752411,117.468308957809));
#56419=CARTESIAN_POINT('Ctrl Pts',(6.66007224322784,-4.27378409624572,117.460493483859));
#56420=CARTESIAN_POINT('Ctrl Pts',(6.55282407636424,-4.43648182369307,117.452678009909));
#56421=CARTESIAN_POINT('Ctrl Pts',(6.43966606259968,-4.59506496169552,117.444862535959));
#56422=CARTESIAN_POINT('Ctrl Pts',(6.3265529743179,-4.75358513973786,117.437050164873));
#56423=CARTESIAN_POINT('Ctrl Pts',(6.20753491778364,-4.90799369723403,117.429237793788));
#56424=CARTESIAN_POINT('Ctrl Pts',(6.08295215386101,-5.05782701304005,117.421425422702));
#56425=CARTESIAN_POINT('Ctrl Pts',(5.95837410584057,-5.20765465712041,117.413613347342));
#56426=CARTESIAN_POINT('Ctrl Pts',(5.82823198787705,-5.35290712848169,117.405801271983));
#56427=CARTESIAN_POINT('Ctrl Pts',(5.69290691429884,-5.49315318056291,117.397989196623));
#56428=CARTESIAN_POINT('Ctrl Pts',(5.55757788288406,-5.633403334404,117.390176892785));
#56429=CARTESIAN_POINT('Ctrl Pts',(5.41706583763429,-5.76864652356256,117.382364588946));
#56430=CARTESIAN_POINT('Ctrl Pts',(5.27178936098721,-5.89848776665528,117.374552285108));
#56431=CARTESIAN_POINT('Ctrl Pts',(5.12648307359517,-6.02835565318178,117.366738378184));
#56432=CARTESIAN_POINT('Ctrl Pts',(4.97641066951175,-6.15281915105685,117.35892447126));
#56433=CARTESIAN_POINT('Ctrl Pts',(4.82202457226624,-6.27152294299085,117.351110564336));
#56434=CARTESIAN_POINT('Ctrl Pts',(4.66757962833394,-6.39027198074031,117.343293679019));
#56435=CARTESIAN_POINT('Ctrl Pts',(4.50881799462534,-6.5032567252031,117.335476793702));
#56436=CARTESIAN_POINT('Ctrl Pts',(4.34622199373894,-6.61016455023171,117.327659908384));
#56437=CARTESIAN_POINT('Ctrl Pts',(4.18344961058971,-6.71718834763349,117.3198345434));
#56438=CARTESIAN_POINT('Ctrl Pts',(4.01683484662423,-6.8181218659688,117.312009178416));
#56439=CARTESIAN_POINT('Ctrl Pts',(3.84688651504871,-6.91269738527128,117.304183813432));
#56440=CARTESIAN_POINT('Ctrl Pts',(3.67683489640687,-7.00733038338419,117.296353692538));
#56441=CARTESIAN_POINT('Ctrl Pts',(3.50344598497656,-7.09559752255831,117.288523571644));
#56442=CARTESIAN_POINT('Ctrl Pts',(3.32724966263928,-7.17727877976513,117.280693450749));
#56443=CARTESIAN_POINT('Ctrl Pts',(3.15081249160492,-7.25907168983798,117.272852626599));
#56444=CARTESIAN_POINT('Ctrl Pts',(2.97156056807867,-7.33426060170491,117.265011802448));
#56445=CARTESIAN_POINT('Ctrl Pts',(2.79004113115738,-7.40267461708605,117.257170978297));
#56446=CARTESIAN_POINT('Ctrl Pts',(2.69207595825905,-7.43959733433968,117.252939322963));
#56447=CARTESIAN_POINT('Ctrl Pts',(2.59345055539616,-7.47454759113312,117.248707667628));
#56448=CARTESIAN_POINT('Ctrl Pts',(2.49425224523058,-7.50750469444823,117.244476012294));
#56449=CARTESIAN_POINT('Ctrl Pts',(2.3087987846975,-7.56911873654966,117.236564837957));
#56450=CARTESIAN_POINT('Ctrl Pts',(2.12081166575402,-7.62393979439585,117.228653663621));
#56451=CARTESIAN_POINT('Ctrl Pts',(1.93083040962673,-7.67175435798493,117.220742489285));
#56452=CARTESIAN_POINT('Ctrl Pts',(1.74105511784712,-7.71951708437911,117.212839891688));
#56453=CARTESIAN_POINT('Ctrl Pts',(1.54929032645702,-7.76028836311641,117.204937294092));
#56454=CARTESIAN_POINT('Ctrl Pts',(1.35609348820962,-7.79390347972282,117.197034696496));
#56455=CARTESIAN_POINT('Ctrl Pts',(1.16307023768138,-7.82748839308432,117.189139199399));
#56456=CARTESIAN_POINT('Ctrl Pts',(0.968617841097546,-7.8539298943556,117.181243702301));
#56457=CARTESIAN_POINT('Ctrl Pts',(0.773307077361525,-7.87311356225112,
117.173348205204));
#56458=CARTESIAN_POINT('Ctrl Pts',(0.578135556833815,-7.89228355350428,
117.165458337055));
#56459=CARTESIAN_POINT('Ctrl Pts',(0.382107230160541,-7.90420598686831,
117.157568468907));
#56460=CARTESIAN_POINT('Ctrl Pts',(0.185801475095989,-7.90881778851,117.149678600758));
#56461=CARTESIAN_POINT('Ctrl Pts',(-0.0104007477622928,-7.91342715787455,
117.141792893749));
#56462=CARTESIAN_POINT('Ctrl Pts',(-0.206879763543778,-7.91073357034298,
117.133907186739));
#56463=CARTESIAN_POINT('Ctrl Pts',(-0.403052401971563,-7.90072590090714,
117.126021479729));
#56464=CARTESIAN_POINT('Ctrl Pts',(-0.599157968129581,-7.89072165313658,
117.118138468876));
#56465=CARTESIAN_POINT('Ctrl Pts',(-0.79495702174133,-7.8734083250332,117.110255458024));
#56466=CARTESIAN_POINT('Ctrl Pts',(-0.989867441810694,-7.84882688353127,
117.102372447171));
#56467=CARTESIAN_POINT('Ctrl Pts',(-1.18478077062658,-7.82424507518808,
117.094489318677));
#56468=CARTESIAN_POINT('Ctrl Pts',(-1.37880509625493,-7.79239497147145,
117.086606190182));
#56469=CARTESIAN_POINT('Ctrl Pts',(-1.57136388485958,-7.75336936701451,
117.078723061687));
#56470=CARTESIAN_POINT('Ctrl Pts',(-1.76393457956659,-7.71434134956544,
117.070839445771));
#56471=CARTESIAN_POINT('Ctrl Pts',(-1.95503921840713,-7.66813701526065,
117.062955829854));
#56472=CARTESIAN_POINT('Ctrl Pts',(-2.14411188438199,-7.61490021124715,
117.055072213938));
#56473=CARTESIAN_POINT('Ctrl Pts',(-2.33322802301851,-7.56165116672519,
117.047186785375));
#56474=CARTESIAN_POINT('Ctrl Pts',(-2.52031092577487,-7.50136652396782,
117.039301356813));
#56475=CARTESIAN_POINT('Ctrl Pts',(-2.70481001492635,-7.43423996001973,
117.031415928251));
#56476=CARTESIAN_POINT('Ctrl Pts',(-2.88938253886896,-7.36708667818796,
117.023527361111));
#56477=CARTESIAN_POINT('Ctrl Pts',(-3.07136887611023,-7.29308616669873,
117.01563879397));
#56478=CARTESIAN_POINT('Ctrl Pts',(-3.25023837094958,-7.21248026215719,
117.00775022683));
#56479=CARTESIAN_POINT('Ctrl Pts',(-3.42929822181413,-7.13178857541108,
116.999853264539));
#56480=CARTESIAN_POINT('Ctrl Pts',(-3.60523429033463,-7.04447759645699,
116.991956302249));
#56481=CARTESIAN_POINT('Ctrl Pts',(-3.77753949333058,-6.95083566028775,
116.984059339958));
#56482=CARTESIAN_POINT('Ctrl Pts',(-3.94994977957764,-6.85713661499515,
116.976157561571));
#56483=CARTESIAN_POINT('Ctrl Pts',(-4.11872448979214,-6.757099090351,116.968255783184));
#56484=CARTESIAN_POINT('Ctrl Pts',(-4.28338527494833,-6.65105492281907,
116.960354004797));
#56485=CARTESIAN_POINT('Ctrl Pts',(-4.44825902335697,-6.54487360356156,
116.952442006682));
#56486=CARTESIAN_POINT('Ctrl Pts',(-4.60900793715952,-6.43267032105508,
116.944530008567));
#56487=CARTESIAN_POINT('Ctrl Pts',(-4.76518561554445,-6.31481805354741,
116.936618010452));
#56488=CARTESIAN_POINT('Ctrl Pts',(-4.83062245689491,-6.26543916527449,
116.933302964597));
#56489=CARTESIAN_POINT('Ctrl Pts',(-4.89525723688726,-6.21506904459781,
116.929987918742));
#56490=CARTESIAN_POINT('Ctrl Pts',(-4.95905904380867,-6.16373704825404,
116.926672872886));
#56491=CARTESIAN_POINT('Ctrl Pts',(-5.10925161418515,-6.04289902115986,
116.918869092995));
#56492=CARTESIAN_POINT('Ctrl Pts',(-5.2552544282984,-5.91638324043838,116.911065313103));
#56493=CARTESIAN_POINT('Ctrl Pts',(-5.396602472448,-5.78451404651836,116.903261533211));
#56494=CARTESIAN_POINT('Ctrl Pts',(-5.53779613515862,-5.65278888116298,
116.895466276668));
#56495=CARTESIAN_POINT('Ctrl Pts',(-5.67434489294149,-5.51572218409021,
116.887671020126));
#56496=CARTESIAN_POINT('Ctrl Pts',(-5.80581449285359,-5.37368021699944,
116.879875763584));
#56497=CARTESIAN_POINT('Ctrl Pts',(-5.93716663718702,-5.2317651508915,116.872087471361));
#56498=CARTESIAN_POINT('Ctrl Pts',(-6.0634484198576,-5.08488392492899,116.864299179139));
#56499=CARTESIAN_POINT('Ctrl Pts',(-6.18426024755322,-4.93344161722149,
116.856510886916));
#56500=CARTESIAN_POINT('Ctrl Pts',(-6.30498814006934,-4.78210452551413,
116.848728005685));
#56501=CARTESIAN_POINT('Ctrl Pts',(-6.4202534256128,-4.62621293980114,116.840945124453));
#56502=CARTESIAN_POINT('Ctrl Pts',(-6.52969474849135,-4.46620728264201,
116.833162243222));
#56503=CARTESIAN_POINT('Ctrl Pts',(-6.64150407003033,-4.30273955857937,
116.825210962598));
#56504=CARTESIAN_POINT('Ctrl Pts',(-6.74723427532696,-4.13497797762956,
116.817259681973));
#56505=CARTESIAN_POINT('Ctrl Pts',(-6.84654425013144,-3.96342690496395,
116.809308401349));
#56506=CARTESIAN_POINT('Ctrl Pts',(-6.94368381291583,-3.79562506807155,
116.801530895364));
#56507=CARTESIAN_POINT('Ctrl Pts',(-7.03468067239163,-3.62419798061624,
116.793753389378));
#56508=CARTESIAN_POINT('Ctrl Pts',(-7.1192601520836,-3.44964576253193,116.785975883393));
#56509=CARTESIAN_POINT('Ctrl Pts',(-7.20383518237405,-3.27510272696933,
116.778198786553));
#56510=CARTESIAN_POINT('Ctrl Pts',(-7.28199334988041,-3.09743520791403,
116.770421689712));
#56511=CARTESIAN_POINT('Ctrl Pts',(-7.35350673591185,-2.91716637936528,
116.762644592872));
#56512=CARTESIAN_POINT('Ctrl Pts',(-7.42502921607158,-2.73687462660684,
116.754866507043));
#56513=CARTESIAN_POINT('Ctrl Pts',(-7.48990510123846,-2.55398123613032,
116.747088421214));
#56514=CARTESIAN_POINT('Ctrl Pts',(-7.54795522932732,-2.36902782931529,
116.739310335385));
#56515=CARTESIAN_POINT('Ctrl Pts',(-7.60827034050064,-2.17685796404203,
116.731228766456));
#56516=CARTESIAN_POINT('Ctrl Pts',(-7.6612161953595,-1.98246449310634,116.723147197527));
#56517=CARTESIAN_POINT('Ctrl Pts',(-7.70664948242962,-1.78646991437507,
116.715065628598));
#56518=CARTESIAN_POINT('Ctrl Pts',(-7.75043061863374,-1.59760254641514,
116.707277940477));
#56519=CARTESIAN_POINT('Ctrl Pts',(-7.78723591500723,-1.40724882405409,
116.699490252356));
#56520=CARTESIAN_POINT('Ctrl Pts',(-7.8169897571167,-1.21597374031375,116.691702564234));
#56521=CARTESIAN_POINT('Ctrl Pts',(-7.84676024076048,-1.02459167506634,
116.683910520404));
#56522=CARTESIAN_POINT('Ctrl Pts',(-7.86947137020366,-0.832287573381514,
116.676118476574));
#56523=CARTESIAN_POINT('Ctrl Pts',(-7.88509953641388,-0.63962981547581,
116.668326432744));
#56524=CARTESIAN_POINT('Ctrl Pts',(-7.90074499513318,-0.446758882461544,
116.660525767045));
#56525=CARTESIAN_POINT('Ctrl Pts',(-7.90929183229359,-0.253533865349083,
116.652725101347));
#56526=CARTESIAN_POINT('Ctrl Pts',(-7.91076848804177,-0.0605221331858206,
116.644924435648));
#56527=CARTESIAN_POINT('Ctrl Pts',(-7.91093210062368,-0.0391365476305301,
116.644060126511));
#56528=CARTESIAN_POINT('Ctrl Pts',(-7.91100896837752,-0.0177535743505116,
116.643195817374));
#56529=CARTESIAN_POINT('Ctrl Pts',(-7.9109991690038,0.00362602002780673,
116.642331508237));
#56530=CARTESIAN_POINT('',(-7.911,5.49282841433296E-12,112.642331508237));
#56531=CARTESIAN_POINT('Ctrl Pts',(-7.91099906790742,0.00384025622421617,
116.648271708555));
#56532=CARTESIAN_POINT('Ctrl Pts',(-7.91090181332933,0.204186491404295,
116.641038596631));
#56533=CARTESIAN_POINT('Ctrl Pts',(-7.90319391388634,0.404448063733921,
116.633586206934));
#56534=CARTESIAN_POINT('Ctrl Pts',(-7.88397113197543,0.655407277402388,
116.623744455381));
#56535=CARTESIAN_POINT('Ctrl Pts',(-7.87954944499618,0.706583214937105,
116.621711092525));
#56536=CARTESIAN_POINT('Ctrl Pts',(-7.87398382771249,0.764424729315218,
116.619379512643));
#56537=CARTESIAN_POINT('Ctrl Pts',(-7.87332927737647,0.771137196198854,
116.619108425336));
#56538=CARTESIAN_POINT('Ctrl Pts',(-7.87224356805935,0.782125741787089,
116.618663800835));
#56539=CARTESIAN_POINT('Ctrl Pts',(-7.87181750573578,0.786402331549728,
116.618490549528));
#56540=CARTESIAN_POINT('Ctrl Pts',(-7.87105729432813,0.793970411920566,
116.618183580638));
#56541=CARTESIAN_POINT('Ctrl Pts',(-7.87072456471077,0.797262047257542,
116.618049943328));
#56542=CARTESIAN_POINT('Ctrl Pts',(-7.87006300203117,0.803765992781635,
116.617785640008));
#56543=CARTESIAN_POINT('Ctrl Pts',(-7.86973426680427,0.806978312546824,
116.617654979584));
#56544=CARTESIAN_POINT('Ctrl Pts',(-7.86907631285033,0.81336903876038,116.617394797561));
#56545=CARTESIAN_POINT('Ctrl Pts',(-7.86874713499281,0.816547448811426,
116.617265278323));
#56546=CARTESIAN_POINT('Ctrl Pts',(-7.86795797392982,0.824122480200145,
116.616956314078));
#56547=CARTESIAN_POINT('Ctrl Pts',(-7.86749623185531,0.828518909638366,
116.616776767759));
#56548=CARTESIAN_POINT('Ctrl Pts',(-7.865816677121,0.844382604564224,116.616128080102));
#56549=CARTESIAN_POINT('Ctrl Pts',(-7.86457748367141,0.855847522405284,
116.615657705902));
#56550=CARTESIAN_POINT('Ctrl Pts',(-7.84549494040132,1.02885611074588,116.608536564253));
#56551=CARTESIAN_POINT('Ctrl Pts',(-7.82270358772423,1.18980585930489,116.601608509287));
#56552=CARTESIAN_POINT('Ctrl Pts',(-7.78345939719205,1.41641585629904,116.591539026345));
#56553=CARTESIAN_POINT('Ctrl Pts',(-7.77109529531072,1.48275137302747,116.588552735429));
#56554=CARTESIAN_POINT('Ctrl Pts',(-7.75347795334157,1.57098921857877,116.58453611901));
#56555=CARTESIAN_POINT('Ctrl Pts',(-7.74897739584507,1.5930401142245,116.58352864544));
#56556=CARTESIAN_POINT('Ctrl Pts',(-7.62546753531652,2.18527873177784,116.556375634767));
#56557=CARTESIAN_POINT('Ctrl Pts',(-7.44394297185286,2.74061542260714,116.528726923268));
#56558=CARTESIAN_POINT('Ctrl Pts',(-7.09460680014913,3.50988620283875,116.490693269253));
#56559=CARTESIAN_POINT('Ctrl Pts',(-6.97431221853708,3.74322482906473,116.47916753938));
#56560=CARTESIAN_POINT('Ctrl Pts',(-6.76427975646116,4.10521845657186,116.46141565878));
#56561=CARTESIAN_POINT('Ctrl Pts',(-6.68193912303167,4.23792313924182,116.454935371928));
#56562=CARTESIAN_POINT('Ctrl Pts',(-6.57960044723064,4.39245163669582,116.447419374038));
#56563=CARTESIAN_POINT('Ctrl Pts',(-6.56334475899924,4.41670454354117,116.44624061879));
#56564=CARTESIAN_POINT('Ctrl Pts',(-6.54148324135061,4.44893391924601,116.44467525233));
#56565=CARTESIAN_POINT('Ctrl Pts',(-6.53599650422043,4.45699065653201,116.444284029478));
#56566=CARTESIAN_POINT('Ctrl Pts',(-6.52693013911629,4.47025098282459,116.443640270824));
#56567=CARTESIAN_POINT('Ctrl Pts',(-6.52335915320187,4.47546045105217,116.443387399354));
#56568=CARTESIAN_POINT('Ctrl Pts',(-6.51640399976914,4.4855808410209,116.442896217192));
#56569=CARTESIAN_POINT('Ctrl Pts',(-6.51302051051227,4.49049222239547,116.442657880337));
#56570=CARTESIAN_POINT('Ctrl Pts',(-6.50516250980977,4.50187111885236,116.442105763316));
#56571=CARTESIAN_POINT('Ctrl Pts',(-6.50068389815598,4.50833580232435,116.441792143475));
#56572=CARTESIAN_POINT('Ctrl Pts',(-6.48617988896869,4.52920516763934,116.440779881201));
#56573=CARTESIAN_POINT('Ctrl Pts',(-6.4761161627448,4.54358321751534,116.440082738899));
#56574=CARTESIAN_POINT('Ctrl Pts',(-6.38202976527669,4.67705683074392,116.433613296936));
#56575=CARTESIAN_POINT('Ctrl Pts',(-6.29477634304091,4.79384585985468,116.427969963229));
#56576=CARTESIAN_POINT('Ctrl Pts',(-6.19911203479009,4.91477385661273,116.422126893477));
#56577=CARTESIAN_POINT('Ctrl Pts',(-6.19387068605095,4.92137765331141,116.421807805507));
#56578=CARTESIAN_POINT('Ctrl Pts',(-6.17561253032216,4.94430650536352,116.420699887674));
#56579=CARTESIAN_POINT('Ctrl Pts',(-6.16254161237168,4.96058845572453,116.419913108852));
#56580=CARTESIAN_POINT('Ctrl Pts',(-6.13845694019903,4.99034771544492,116.41847488029));
#56581=CARTESIAN_POINT('Ctrl Pts',(-6.1274628936193,5.00384076678697,116.41782270261));
#56582=CARTESIAN_POINT('Ctrl Pts',(-6.08131523549221,5.06009787773319,116.415103060957));
#56583=CARTESIAN_POINT('Ctrl Pts',(-6.04575746103112,5.10252901804449,116.413050631394));
#56584=CARTESIAN_POINT('Ctrl Pts',(-5.53750371260452,5.69625661621901,116.384293694912));
#56585=CARTESIAN_POINT('Ctrl Pts',(-4.9916025985403,6.18021649218671,116.360800591652));
#56586=CARTESIAN_POINT('Ctrl Pts',(-4.234206288446,6.68500581428937,116.328510164025));
#56587=CARTESIAN_POINT('Ctrl Pts',(-4.07752112375769,6.78171224647276,116.321820514977));
#56588=CARTESIAN_POINT('Ctrl Pts',(-3.84798855843084,6.91254857526785,116.311805379098));
#56589=CARTESIAN_POINT('Ctrl Pts',(-3.77776622745434,6.95117438599509,116.308713400882));
#56590=CARTESIAN_POINT('Ctrl Pts',(-3.67194976963609,7.00730172534992,116.303994709643));
#56591=CARTESIAN_POINT('Ctrl Pts',(-3.63678969351032,7.02561408005244,116.302417151656));
#56592=CARTESIAN_POINT('Ctrl Pts',(-3.59499930613283,7.04698192126174,116.300528977499));
#56593=CARTESIAN_POINT('Ctrl Pts',(-3.5884999875473,7.05029375617576,116.30023495115));
#56594=CARTESIAN_POINT('Ctrl Pts',(-3.5791268698679,7.05505366422214,116.299810363572));
#56595=CARTESIAN_POINT('Ctrl Pts',(-3.57625673635926,7.05650898895833,116.299680276545));
#56596=CARTESIAN_POINT('Ctrl Pts',(-3.57060552760912,7.05937014732746,116.29942399092));
#56597=CARTESIAN_POINT('Ctrl Pts',(-3.56782450787089,7.06077608990344,116.299297799523));
#56598=CARTESIAN_POINT('Ctrl Pts',(-3.56228884039312,7.06357053717609,116.299046471669));
#56599=CARTESIAN_POINT('Ctrl Pts',(-3.5595342195601,7.0649590696443,116.298921337677));
#56600=CARTESIAN_POINT('Ctrl Pts',(-3.5529599104722,7.06826818628319,116.298622520478));
#56601=CARTESIAN_POINT('Ctrl Pts',(-3.54913948482629,7.07018728152267,116.298448739739));
#56602=CARTESIAN_POINT('Ctrl Pts',(-3.53758441794462,7.07597995441549,116.297922731515));
#56603=CARTESIAN_POINT('Ctrl Pts',(-3.52984500250232,7.0798439309398,116.29756987778));
#56604=CARTESIAN_POINT('Ctrl Pts',(-3.45193740902376,7.11858053278858,116.294012617268));
#56605=CARTESIAN_POINT('Ctrl Pts',(-3.38126336080635,7.15242042655522,116.290742337232));
#56606=CARTESIAN_POINT('Ctrl Pts',(-3.2981757548262,7.19069746791441,116.286857986446));
#56607=CARTESIAN_POINT('Ctrl Pts',(-3.28623719012119,7.1961613733691,116.286298909992));
#56608=CARTESIAN_POINT('Ctrl Pts',(-3.18444086313071,7.24244420062179,116.28152413666));
#56609=CARTESIAN_POINT('Ctrl Pts',(-3.0938429616586,7.28160669287414,116.277223617874));
#56610=CARTESIAN_POINT('Ctrl Pts',(-2.96924740462947,7.3327202136533,116.271263926551));
#56611=CARTESIAN_POINT('Ctrl Pts',(-2.93586300467866,7.34615030107099,116.26966268054));
#56612=CARTESIAN_POINT('Ctrl Pts',(-2.65645843244351,7.45634215135389,116.256231545564));
#56613=CARTESIAN_POINT('Ctrl Pts',(-2.40583014848456,7.54094027553931,116.24399697626));
#56614=CARTESIAN_POINT('Ctrl Pts',(-2.12185186155035,7.62119489548043,116.230249011718));
#56615=CARTESIAN_POINT('Ctrl Pts',(-2.09220617728504,7.62938662438005,116.228815094235));
#56616=CARTESIAN_POINT('Ctrl Pts',(-2.02906059098436,7.64643935641497,116.225764394876));
#56617=CARTESIAN_POINT('Ctrl Pts',(-1.99554868917345,7.65525356469257,116.224147483659));
#56618=CARTESIAN_POINT('Ctrl Pts',(-1.92388335229802,7.67360021887583,116.220695358925));
#56619=CARTESIAN_POINT('Ctrl Pts',(-1.88571451422883,7.68306893409005,116.218860164627));
#56620=CARTESIAN_POINT('Ctrl Pts',(-1.80370339383224,7.70276584689238,116.214925842413));
#56621=CARTESIAN_POINT('Ctrl Pts',(-1.75984111724073,7.7129052167111,116.212827035881));
#56622=CARTESIAN_POINT('Ctrl Pts',(-1.66500130565015,7.73397760859545,116.20830280711));
#56623=CARTESIAN_POINT('Ctrl Pts',(-1.61399727606799,7.74478223271647,116.205878309065));
#56624=CARTESIAN_POINT('Ctrl Pts',(-1.50270659440359,7.76721076318736,116.200609930504));
#56625=CARTESIAN_POINT('Ctrl Pts',(-1.44238367434907,7.77863867162948,116.197768216039));
#56626=CARTESIAN_POINT('Ctrl Pts',(-1.174567705809,7.82615267629989,116.185222828359));
#56627=CARTESIAN_POINT('Ctrl Pts',(-0.965808590787287,7.8546480169439,116.175635044654));
#56628=CARTESIAN_POINT('Ctrl Pts',(-0.393591458958936,7.90959352423486,
116.150040502727));
#56629=CARTESIAN_POINT('Ctrl Pts',(-0.0290336427505016,7.91933007611112,
116.134503568535));
#56630=CARTESIAN_POINT('Ctrl Pts',(0.352782493072675,7.90315029781344,116.119064140596));
#56631=CARTESIAN_POINT('Ctrl Pts',(0.370627792324953,7.90233352639464,116.118344371987));
#56632=CARTESIAN_POINT('Ctrl Pts',(0.396508118067032,7.90106113606163,116.117303158974));
#56633=CARTESIAN_POINT('Ctrl Pts',(0.404545393383706,7.90065369375698,116.11698017385));
#56634=CARTESIAN_POINT('Ctrl Pts',(0.418583479330228,7.89992056834951,116.11641668238));
#56635=CARTESIAN_POINT('Ctrl Pts',(0.424584559312617,7.8996003106233,116.116176002723));
#56636=CARTESIAN_POINT('Ctrl Pts',(0.436186985433,7.89896786840578,116.11571106964));
#56637=CARTESIAN_POINT('Ctrl Pts',(0.441788374317177,7.89865656329278,116.11548678827));
#56638=CARTESIAN_POINT('Ctrl Pts',(0.455081633405319,7.89790358681932,116.114954942356));
#56639=CARTESIAN_POINT('Ctrl Pts',(0.462773205864404,7.8974566361674,116.114647546675));
#56640=CARTESIAN_POINT('Ctrl Pts',(0.489861386752654,7.89584285626502,116.113566130658));
#56641=CARTESIAN_POINT('Ctrl Pts',(0.509254411105159,7.89461579437881,116.112794034822));
#56642=CARTESIAN_POINT('Ctrl Pts',(0.752594531968337,7.87831846331943,116.103132047586));
#56643=CARTESIAN_POINT('Ctrl Pts',(0.975814751531368,7.85379497354143,116.094551078133));
#56644=CARTESIAN_POINT('Ctrl Pts',(1.60689149870922,7.757137655432,116.070874600331));
#56645=CARTESIAN_POINT('Ctrl Pts',(2.01054410206709,7.66244223681423,116.056462604569));
#56646=CARTESIAN_POINT('Ctrl Pts',(2.77568705046096,7.41828359616922,116.028787511476));
#56647=CARTESIAN_POINT('Ctrl Pts',(3.13718223019088,7.27278709330631,116.015531733195));
#56648=CARTESIAN_POINT('Ctrl Pts',(3.60268807190867,7.0442400289475,115.996702295834));
#56649=CARTESIAN_POINT('Ctrl Pts',(3.71746907004695,6.98434681082448,115.991905971416));
#56650=CARTESIAN_POINT('Ctrl Pts',(3.8943716936779,6.88644188416451,115.984197494795));
#56651=CARTESIAN_POINT('Ctrl Pts',(3.95752897593229,6.85034137118276,115.981380532285));
#56652=CARTESIAN_POINT('Ctrl Pts',(4.04294151447298,6.79994437031201,115.977470411399));
#56653=CARTESIAN_POINT('Ctrl Pts',(4.06563651089896,6.78639958027024,115.97642175276));
#56654=CARTESIAN_POINT('Ctrl Pts',(4.09886672812555,6.76634066202132,115.97487247072));
#56655=CARTESIAN_POINT('Ctrl Pts',(4.10945537794118,6.75991500712004,115.974376725403));
#56656=CARTESIAN_POINT('Ctrl Pts',(4.12607604377352,6.74977537844769,115.973595355229));
#56657=CARTESIAN_POINT('Ctrl Pts',(4.13211826766775,6.74607810509266,115.973310628537));
#56658=CARTESIAN_POINT('Ctrl Pts',(4.14229902657093,6.73982962771544,115.972829761851));
#56659=CARTESIAN_POINT('Ctrl Pts',(4.14644019853362,6.73728271011331,115.972633849068));
#56660=CARTESIAN_POINT('Ctrl Pts',(4.15455974076809,6.73227868000615,115.972249114284));
#56661=CARTESIAN_POINT('Ctrl Pts',(4.15853828601928,6.72982185413918,115.972060307348));
#56662=CARTESIAN_POINT('Ctrl Pts',(4.16612658234032,6.72512664123397,115.971699647776));
#56663=CARTESIAN_POINT('Ctrl Pts',(4.169736714723,6.72288887090255,115.971527827203));
#56664=CARTESIAN_POINT('Ctrl Pts',(4.1780509273921,6.71772596441377,115.971131577839));
#56665=CARTESIAN_POINT('Ctrl Pts',(4.18275373753407,6.71479879488276,115.970907044369));
#56666=CARTESIAN_POINT('Ctrl Pts',(4.19705172758589,6.70587844967117,115.970223181513));
#56667=CARTESIAN_POINT('Ctrl Pts',(4.20663710283854,6.69986964566608,115.969763056974));
#56668=CARTESIAN_POINT('Ctrl Pts',(4.27471133874205,6.65699213027726,115.966483634586));
#56669=CARTESIAN_POINT('Ctrl Pts',(4.33272640076335,6.61937933579364,115.963627444815));
#56670=CARTESIAN_POINT('Ctrl Pts',(4.7628140245435,6.33246482382478,115.942030524016));
#56671=CARTESIAN_POINT('Ctrl Pts',(5.11359491994557,6.05273702622087,115.922071124785));
#56672=CARTESIAN_POINT('Ctrl Pts',(5.90902990068829,5.29967688001256,115.87347903305));
#56673=CARTESIAN_POINT('Ctrl Pts',(6.32286901234377,4.7984071611308,115.845304962315));
#56674=CARTESIAN_POINT('Ctrl Pts',(6.69494585501499,4.21468938097619,115.817176650297));
#56675=CARTESIAN_POINT('Ctrl Pts',(6.71857960990425,4.17691209643038,115.8153738654));
#56676=CARTESIAN_POINT('Ctrl Pts',(6.7498832973406,4.12592168017611,115.812963551817));
#56677=CARTESIAN_POINT('Ctrl Pts',(6.75783581144726,4.11288334218295,115.812349233119));
#56678=CARTESIAN_POINT('Ctrl Pts',(6.77094147546803,4.09125565862892,115.811333496288));
#56679=CARTESIAN_POINT('Ctrl Pts',(6.77611614609079,4.08267942701656,115.810931567106));
#56680=CARTESIAN_POINT('Ctrl Pts',(6.78617431426053,4.06593773917696,115.810148606209));
#56681=CARTESIAN_POINT('Ctrl Pts',(6.79105939864988,4.05777325228817,115.809767536982));
#56682=CARTESIAN_POINT('Ctrl Pts',(6.80234599346721,4.03883239240284,115.808885249042));
#56683=CARTESIAN_POINT('Ctrl Pts',(6.80873665126472,4.02804956817804,115.80838428727));
#56684=CARTESIAN_POINT('Ctrl Pts',(6.82929834264459,3.99316750654709,115.806767927087));
#56685=CARTESIAN_POINT('Ctrl Pts',(6.84336731071729,3.96900824543168,115.805654950098));
#56686=CARTESIAN_POINT('Ctrl Pts',(6.98006732455026,3.73137894057308,115.794771039067));
#56687=CARTESIAN_POINT('Ctrl Pts',(7.09280210049344,3.5123632550971,115.785244587339));
#56688=CARTESIAN_POINT('Ctrl Pts',(7.43284713766094,2.76834046273727,115.754292665549));
#56689=CARTESIAN_POINT('Ctrl Pts',(7.61345241698799,2.22401991848581,115.734016104148));
#56690=CARTESIAN_POINT('Ctrl Pts',(7.77557796106222,1.47095307467421,115.70593025629));
#56691=CARTESIAN_POINT('Ctrl Pts',(7.81003303182561,1.2754196656315,115.698617994516));
#56692=CARTESIAN_POINT('Ctrl Pts',(7.85306928074295,0.962777758997314,115.686667827457));
#56693=CARTESIAN_POINT('Ctrl Pts',(7.86646167605596,0.846414387519442,115.682163362771));
#56694=CARTESIAN_POINT('Ctrl Pts',(7.88065136374469,0.6932547232068,115.676118192187));
#56695=CARTESIAN_POINT('Ctrl Pts',(7.88378276295673,0.656686619546123,115.674666168826));
#56696=CARTESIAN_POINT('Ctrl Pts',(7.88788077509335,0.6045664661074,115.672582797481));
#56697=CARTESIAN_POINT('Ctrl Pts',(7.8890561053163,0.58903098085984,115.671960058646));
#56698=CARTESIAN_POINT('Ctrl Pts',(7.89078802671747,0.565202965195084,115.6710021159));
#56699=CARTESIAN_POINT('Ctrl Pts',(7.89137745896507,0.556912806318153,115.670668312633));
#56700=CARTESIAN_POINT('Ctrl Pts',(7.89232636199662,0.543262784569546,115.670117820148));
#56701=CARTESIAN_POINT('Ctrl Pts',(7.89269344026632,0.53790344406409,115.669901461163));
#56702=CARTESIAN_POINT('Ctrl Pts',(7.89339296164801,0.527535543119284,115.669482469001));
#56703=CARTESIAN_POINT('Ctrl Pts',(7.89372609724392,0.522527030661014,115.669279866311));
#56704=CARTESIAN_POINT('Ctrl Pts',(7.89432487212466,0.513393513420458,115.668910037227));
#56705=CARTESIAN_POINT('Ctrl Pts',(7.89459204585982,0.509268608511942,115.668742878958));
#56706=CARTESIAN_POINT('Ctrl Pts',(7.89517761394497,0.500116801778324,115.668371706981));
#56707=CARTESIAN_POINT('Ctrl Pts',(7.89549444028891,0.49508980432794,115.668167623222));
#56708=CARTESIAN_POINT('Ctrl Pts',(7.89634493891155,0.4813867107484,115.667610751676));
#56709=CARTESIAN_POINT('Ctrl Pts',(7.89686911170679,0.47271004982859,115.667257534852));
#56710=CARTESIAN_POINT('Ctrl Pts',(7.89930735816456,0.43121348771975,115.665565268938));
#56711=CARTESIAN_POINT('Ctrl Pts',(7.90103111392026,0.398383100949825,115.664217477952));
#56712=CARTESIAN_POINT('Ctrl Pts',(7.92358590531018,-0.0892208495931408,
115.644056057509));
#56713=CARTESIAN_POINT('Ctrl Pts',(7.90532444936921,-0.544893638295657,
115.623297776831));
#56714=CARTESIAN_POINT('Ctrl Pts',(7.80992642604498,-1.29628346053187,115.588424057613));
#56715=CARTESIAN_POINT('Ctrl Pts',(7.7546939890279,-1.59374755679164,115.574439893761));
#56716=CARTESIAN_POINT('Ctrl Pts',(7.63589573263551,-2.07732949870228,115.551891281789));
#56717=CARTESIAN_POINT('Ctrl Pts',(7.58218442227572,-2.26554332923599,115.543159966489));
#56718=CARTESIAN_POINT('Ctrl Pts',(7.44378190449087,-2.69016803723906,115.523663193885));
#56719=CARTESIAN_POINT('Ctrl Pts',(7.35470417322022,-2.92493330692503,115.513033787937));
#56720=CARTESIAN_POINT('Ctrl Pts',(7.23594940239037,-3.19799103149877,115.500872744973));
#56721=CARTESIAN_POINT('Ctrl Pts',(7.21690761680385,-3.24073370431275,115.498974941931));
#56722=CARTESIAN_POINT('Ctrl Pts',(7.19266433846465,-3.29387852959899,115.49662229893));
#56723=CARTESIAN_POINT('Ctrl Pts',(7.18781785887241,-3.30444102425456,115.496155060772));
#56724=CARTESIAN_POINT('Ctrl Pts',(7.18011193114909,-3.32113827875267,115.495416992489));
#56725=CARTESIAN_POINT('Ctrl Pts',(7.17726786370809,-3.327280093907,115.495145622847));
#56726=CARTESIAN_POINT('Ctrl Pts',(7.17192348302463,-3.33878264378533,115.494637612243));
#56727=CARTESIAN_POINT('Ctrl Pts',(7.16942503378652,-3.34414423641057,115.49440090596));
#56728=CARTESIAN_POINT('Ctrl Pts',(7.16383136121043,-3.3561129991475,115.493872699833));
#56729=CARTESIAN_POINT('Ctrl Pts',(7.16073300413596,-3.36271870348419,115.493581310656));
#56730=CARTESIAN_POINT('Ctrl Pts',(7.152899230657,-3.37936040412829,115.492847551501));
#56731=CARTESIAN_POINT('Ctrl Pts',(7.14815182079555,-3.38939075544526,115.492405605259));
#56732=CARTESIAN_POINT('Ctrl Pts',(7.12280578086598,-3.44265188587129,115.490060487041));
#56733=CARTESIAN_POINT('Ctrl Pts',(7.10183583181089,-3.48570539800617,115.488170487759));
#56734=CARTESIAN_POINT('Ctrl Pts',(7.07436548015585,-3.540827831956,115.485757453502));
#56735=CARTESIAN_POINT('Ctrl Pts',(7.06822309401343,-3.5530734551986,115.485221822784));
#56736=CARTESIAN_POINT('Ctrl Pts',(6.64679847104864,-4.38781911778258,115.448738321643));
#56737=CARTESIAN_POINT('Ctrl Pts',(6.09114533849994,-5.13133949425804,115.419251059324));
#56738=CARTESIAN_POINT('Ctrl Pts',(5.25418110055923,-5.91856052692249,115.379186349169));
#56739=CARTESIAN_POINT('Ctrl Pts',(5.08165324824459,-6.06733609464714,115.37104384702));
#56740=CARTESIAN_POINT('Ctrl Pts',(4.81154683374247,-6.2806453311819,115.358079316186));
#56741=CARTESIAN_POINT('Ctrl Pts',(4.71855499950254,-6.35080507554742,115.353579302401));
#56742=CARTESIAN_POINT('Ctrl Pts',(4.61376281470051,-6.42629555079542,115.348428964343));
#56743=CARTESIAN_POINT('Ctrl Pts',(4.60345558394729,-6.4336831208573,115.347921549043));
#56744=CARTESIAN_POINT('Ctrl Pts',(4.58774034795296,-6.444889706652,115.347146564977));
#56745=CARTESIAN_POINT('Ctrl Pts',(4.58234519740399,-6.44872679855975,115.34688026838));
#56746=CARTESIAN_POINT('Ctrl Pts',(4.57237374290582,-6.45579977762838,115.34638763896));
#56747=CARTESIAN_POINT('Ctrl Pts',(4.56779880022876,-6.45903758573642,115.346161442868));
#56748=CARTESIAN_POINT('Ctrl Pts',(4.56036080449279,-6.46428979763383,115.345793398809));
#56749=CARTESIAN_POINT('Ctrl Pts',(4.55749984192238,-6.46630717224482,115.345651763647));
#56750=CARTESIAN_POINT('Ctrl Pts',(4.55195416979389,-6.47021212996013,115.345377081885));
#56751=CARTESIAN_POINT('Ctrl Pts',(4.5492696318142,-6.47209993646396,115.345244052576));
#56752=CARTESIAN_POINT('Ctrl Pts',(4.54313503038467,-6.47640817561383,115.344939919457));
#56753=CARTESIAN_POINT('Ctrl Pts',(4.53968420846513,-6.47882752114685,115.344768738353));
#56754=CARTESIAN_POINT('Ctrl Pts',(4.53056840666725,-6.485207683078,115.344316278718));
#56755=CARTESIAN_POINT('Ctrl Pts',(4.52490017805842,-6.48916382580535,115.344034671215));
#56756=CARTESIAN_POINT('Ctrl Pts',(4.48850914283008,-6.51449210107582,115.342225032297));
#56757=CARTESIAN_POINT('Ctrl Pts',(4.45764065546592,-6.53565309340281,115.340682398058));
#56758=CARTESIAN_POINT('Ctrl Pts',(3.93458242925358,-6.8887910125632,115.31443248094));
#56759=CARTESIAN_POINT('Ctrl Pts',(3.406739498924,-7.16452613142196,115.286445106328));
#56760=CARTESIAN_POINT('Ctrl Pts',(2.51326301751179,-7.5100039648883,115.242192396197));
#56761=CARTESIAN_POINT('Ctrl Pts',(2.16476895094236,-7.61777272368432,115.225595298003));
#56762=CARTESIAN_POINT('Ctrl Pts',(1.56378171512177,-7.75902792204781,115.198661016452));
#56763=CARTESIAN_POINT('Ctrl Pts',(1.31485052534034,-7.80506961066854,115.187969104255));
#56764=CARTESIAN_POINT('Ctrl Pts',(1.02494801678207,-7.84442257563391,115.176059686907));
#56765=CARTESIAN_POINT('Ctrl Pts',(0.985733056024901,-7.84944675665488,
115.174459895589));
#56766=CARTESIAN_POINT('Ctrl Pts',(0.935655542244121,-7.85548143742645,
115.172431016765));
#56767=CARTESIAN_POINT('Ctrl Pts',(0.924826681624134,-7.85676367964011,
115.171993124981));
#56768=CARTESIAN_POINT('Ctrl Pts',(0.907465239926092,-7.85878305179962,
115.171292406771));
#56769=CARTESIAN_POINT('Ctrl Pts',(0.90093434994248,-7.85953443368617,115.171029118682));
#56770=CARTESIAN_POINT('Ctrl Pts',(0.888554272140645,-7.86094313363883,
115.170530596381));
#56771=CARTESIAN_POINT('Ctrl Pts',(0.882705274659372,-7.86160206593607,
115.170295310027));
#56772=CARTESIAN_POINT('Ctrl Pts',(0.869453242053805,-7.86308002855273,
115.169762769259));
#56773=CARTESIAN_POINT('Ctrl Pts',(0.862049769791817,-7.86389513347848,
115.169465642142));
#56774=CARTESIAN_POINT('Ctrl Pts',(0.843026764398102,-7.8659623349778,115.168703169819));
#56775=CARTESIAN_POINT('Ctrl Pts',(0.831405568861974,-7.86719914343043,
115.168238319652));
#56776=CARTESIAN_POINT('Ctrl Pts',(0.76403082555413,-7.87421867803947,115.165548761716));
#56777=CARTESIAN_POINT('Ctrl Pts',(0.708219147866111,-7.87943454176536,
115.163342417494));
#56778=CARTESIAN_POINT('Ctrl Pts',(-0.296873217622958,-7.96259959581657,
115.123983272364));
#56779=CARTESIAN_POINT('Ctrl Pts',(-1.25227004437144,-7.86909068245732,
115.093841062277));
#56780=CARTESIAN_POINT('Ctrl Pts',(-2.31832385121852,-7.56529557336172,
115.054215274145));
#56781=CARTESIAN_POINT('Ctrl Pts',(-2.46724638868333,-7.51804588946125,
115.048504191553));
#56782=CARTESIAN_POINT('Ctrl Pts',(-2.71444502946125,-7.43147938887357,
115.038583546642));
#56783=CARTESIAN_POINT('Ctrl Pts',(-2.81350958885966,-7.3945425675753,115.034486100323));
#56784=CARTESIAN_POINT('Ctrl Pts',(-2.9286072683571,-7.34898001146861,115.02954978517));
#56785=CARTESIAN_POINT('Ctrl Pts',(-2.94539130330259,-7.34226925422444,
115.028825527766));
#56786=CARTESIAN_POINT('Ctrl Pts',(-2.96740674226264,-7.33337918971146,
115.027869528586));
#56787=CARTESIAN_POINT('Ctrl Pts',(-2.97265909361747,-7.3312516685059,115.027640999898));
#56788=CARTESIAN_POINT('Ctrl Pts',(-2.98127204410904,-7.32775212291198,
115.027265511959));
#56789=CARTESIAN_POINT('Ctrl Pts',(-2.9846339619335,-7.32638343857433,115.027118761856));
#56790=CARTESIAN_POINT('Ctrl Pts',(-2.991147843542,-7.32372631745953,115.02683406977));
#56791=CARTESIAN_POINT('Ctrl Pts',(-2.99429992048068,-7.32243815823089,
115.026696144918));
#56792=CARTESIAN_POINT('Ctrl Pts',(-3.00157621866272,-7.3194590696334,115.026377385005));
#56793=CARTESIAN_POINT('Ctrl Pts',(-3.00569984116402,-7.31776669026507,
115.026196461101));
#56794=CARTESIAN_POINT('Ctrl Pts',(-3.01889358013371,-7.31233880321456,
115.025616706514));
#56795=CARTESIAN_POINT('Ctrl Pts',(-3.02795814986253,-7.30858992297624,
115.025217063334));
#56796=CARTESIAN_POINT('Ctrl Pts',(-3.10781721396611,-7.27538813421967,
115.021684610535));
#56797=CARTESIAN_POINT('Ctrl Pts',(-3.17818491582602,-7.24492513839153,
115.018491645827));
#56798=CARTESIAN_POINT('Ctrl Pts',(-3.26343107511898,-7.20654018551908,
115.014535265325));
#56799=CARTESIAN_POINT('Ctrl Pts',(-3.27874351568692,-7.1995864311048,115.013821088294));
#56800=CARTESIAN_POINT('Ctrl Pts',(-3.30008663153042,-7.18981178813383,
115.012820857425));
#56801=CARTESIAN_POINT('Ctrl Pts',(-3.30613617506278,-7.1870319963067,115.012536812));
#56802=CARTESIAN_POINT('Ctrl Pts',(-3.32798594055171,-7.17695850795335,
115.011508971098));
#56803=CARTESIAN_POINT('Ctrl Pts',(-3.34376551305338,-7.16962035479225,
115.010763039261));
#56804=CARTESIAN_POINT('Ctrl Pts',(-3.37600400594731,-7.15449854511342,
115.009231796671));
#56805=CARTESIAN_POINT('Ctrl Pts',(-3.39246052387339,-7.14671001692831,
115.008446263732));
#56806=CARTESIAN_POINT('Ctrl Pts',(-3.44367529872468,-7.12225437390386,
115.005989771782));
#56807=CARTESIAN_POINT('Ctrl Pts',(-3.47833841040738,-7.10539012027898,
115.004310157035));
#56808=CARTESIAN_POINT('Ctrl Pts',(-4.21224268021214,-6.74167460247681,
114.96840730019));
#56809=CARTESIAN_POINT('Ctrl Pts',(-4.85649522620086,-6.29347811850427,
114.930802124614));
#56810=CARTESIAN_POINT('Ctrl Pts',(-5.63933860977059,-5.5559615477231,114.883476861699));
#56811=CARTESIAN_POINT('Ctrl Pts',(-5.84248052901552,-5.34193730675529,
114.870936859068));
#56812=CARTESIAN_POINT('Ctrl Pts',(-6.06150482349919,-5.08369877083443,
114.857126993756));
#56813=CARTESIAN_POINT('Ctrl Pts',(-6.08951825665932,-5.05010904826316,
114.855354502633));
#56814=CARTESIAN_POINT('Ctrl Pts',(-6.12460169334882,-5.00732557836908,
114.853126466242));
#56815=CARTESIAN_POINT('Ctrl Pts',(-6.13193171092298,-4.99834661103127,
114.852660499792));
#56816=CARTESIAN_POINT('Ctrl Pts',(-6.14359003952098,-4.98400140006619,
114.851918639451));
#56817=CARTESIAN_POINT('Ctrl Pts',(-6.1479311019895,-4.97864556833096,114.851642236749));
#56818=CARTESIAN_POINT('Ctrl Pts',(-6.15610882925944,-4.96852920537994,
114.851121231903));
#56819=CARTESIAN_POINT('Ctrl Pts',(-6.15994698563641,-4.96376988958623,
114.85087657046));
#56820=CARTESIAN_POINT('Ctrl Pts',(-6.16858057874928,-4.95303879468147,
114.850325927352));
#56821=CARTESIAN_POINT('Ctrl Pts',(-6.17337287159187,-4.94706448784086,
114.850020070592));
#56822=CARTESIAN_POINT('Ctrl Pts',(-6.18556994534602,-4.93181369626165,
114.849241084323));
#56823=CARTESIAN_POINT('Ctrl Pts',(-6.19296255037568,-4.92252747423548,
114.848768436781));
#56824=CARTESIAN_POINT('Ctrl Pts',(-6.234214633144,-4.87046864908639,114.84612809672));
#56825=CARTESIAN_POINT('Ctrl Pts',(-6.2676522601347,-4.82736286683613,114.843977031312));
#56826=CARTESIAN_POINT('Ctrl Pts',(-6.86012938247671,-4.04704239753016,
114.80565061011));
#56827=CARTESIAN_POINT('Ctrl Pts',(-7.28593320415537,-3.21789268654761,
114.775773351169));
#56828=CARTESIAN_POINT('Ctrl Pts',(-7.59000785595909,-2.23312559008803,
114.738715804427));
#56829=CARTESIAN_POINT('Ctrl Pts',(-7.61913541542674,-2.13162934573914,
114.734866028635));
#56830=CARTESIAN_POINT('Ctrl Pts',(-7.68596551022528,-1.87985459738685,
114.725178933269));
#56831=CARTESIAN_POINT('Ctrl Pts',(-7.72130034791914,-1.72899834857297,
114.719255656064));
#56832=CARTESIAN_POINT('Ctrl Pts',(-7.75681897312978,-1.55441992752245,
114.712169327939));
#56833=CARTESIAN_POINT('Ctrl Pts',(-7.76135515938823,-1.53160959859086,
114.711238915955));
#56834=CARTESIAN_POINT('Ctrl Pts',(-7.7670102646236,-1.50250239357352,114.710045544368));
#56835=CARTESIAN_POINT('Ctrl Pts',(-7.76822226070017,-1.49622351317799,
114.709787753039));
#56836=CARTESIAN_POINT('Ctrl Pts',(-7.77015172419558,-1.48616217311393,
114.709374075768));
#56837=CARTESIAN_POINT('Ctrl Pts',(-7.77087404800033,-1.48238063662222,
114.709218462483));
#56838=CARTESIAN_POINT('Ctrl Pts',(-7.77217188291264,-1.47555914656806,
114.70893750969));
#56839=CARTESIAN_POINT('Ctrl Pts',(-7.77274837022012,-1.47251938720994,
114.708812225698));
#56840=CARTESIAN_POINT('Ctrl Pts',(-7.77411234721491,-1.46530415531789,
114.708514642878));
#56841=CARTESIAN_POINT('Ctrl Pts',(-7.77489825510597,-1.46112839180911,
114.708342255209));
#56842=CARTESIAN_POINT('Ctrl Pts',(-7.77687603994566,-1.45057305192077,
114.707906089931));
#56843=CARTESIAN_POINT('Ctrl Pts',(-7.778063429352,-1.4441926492463,114.707642061916));
#56844=CARTESIAN_POINT('Ctrl Pts',(-7.78439794848421,-1.40991987635502,
114.706221812726));
#56845=CARTESIAN_POINT('Ctrl Pts',(-7.78940284152846,-1.38200174138548,
114.705057769813));
#56846=CARTESIAN_POINT('Ctrl Pts',(-7.87156588342275,-0.909052962050528,
114.685225000803));
#56847=CARTESIAN_POINT('Ctrl Pts',(-7.91061575441299,-0.458278575113945,
114.66466740998));
#56848=CARTESIAN_POINT('Ctrl Pts',(-7.91150122343188,0.590095865630536,
114.616562902213));
#56849=CARTESIAN_POINT('Ctrl Pts',(-7.84447459963245,1.18509353893569,114.589167834301));
#56850=CARTESIAN_POINT('Ctrl Pts',(-7.70010911675395,1.81512687398723,114.561755470135));
#56851=CARTESIAN_POINT('Ctrl Pts',(-7.68861338522194,1.86322041220235,114.559671826483));
#56852=CARTESIAN_POINT('Ctrl Pts',(-7.64589242441081,2.03481626361016,114.552269593527));
#56853=CARTESIAN_POINT('Ctrl Pts',(-7.61213546433998,2.15767092858362,114.547030092214));
#56854=CARTESIAN_POINT('Ctrl Pts',(-7.57042389038027,2.29628054693532,114.54118470337));
#56855=CARTESIAN_POINT('Ctrl Pts',(-7.56536783001319,2.31288387772137,114.540485592137));
#56856=CARTESIAN_POINT('Ctrl Pts',(-7.55789748460164,2.33712875749698,114.539466276754));
#56857=CARTESIAN_POINT('Ctrl Pts',(-7.5555261800531,2.34478343560438,114.539144682096));
#56858=CARTESIAN_POINT('Ctrl Pts',(-7.55130656431015,2.35833168189141,114.538575881687));
#56859=CARTESIAN_POINT('Ctrl Pts',(-7.54946297603595,2.36422670733805,114.538328523085));
#56860=CARTESIAN_POINT('Ctrl Pts',(-7.5456236437485,2.37645300705303,114.53781577755));
#56861=CARTESIAN_POINT('Ctrl Pts',(-7.54362683028941,2.38278394182943,114.537550425565));
#56862=CARTESIAN_POINT('Ctrl Pts',(-7.53846692518996,2.39907202213077,114.536868128858));
#56863=CARTESIAN_POINT('Ctrl Pts',(-7.53529206906851,2.40902544288219,114.536451566715));
#56864=CARTESIAN_POINT('Ctrl Pts',(-7.52205182381373,2.45025237509161,114.534727731417));
#56865=CARTESIAN_POINT('Ctrl Pts',(-7.51181132248268,2.4814695303517,114.533426162941));
#56866=CARTESIAN_POINT('Ctrl Pts',(-7.30846560723666,3.08855354275673,114.508184421553));
#56867=CARTESIAN_POINT('Ctrl Pts',(-7.04987682696602,3.6403513549266,114.486697291546));
#56868=CARTESIAN_POINT('Ctrl Pts',(-6.40509552785112,4.68428372647476,114.444421976861));
#56869=CARTESIAN_POINT('Ctrl Pts',(-6.01877404344938,5.17126004935686,114.423725553408));
#56870=CARTESIAN_POINT('Ctrl Pts',(-5.57435211485233,5.61342819134297,114.399027162713));
#56871=CARTESIAN_POINT('Ctrl Pts',(-5.56901318660006,5.61872491643253,114.398730325039));
#56872=CARTESIAN_POINT('Ctrl Pts',(-5.54079458777866,5.64664072163285,114.397160665173));
#56873=CARTESIAN_POINT('Ctrl Pts',(-5.51778492817767,5.6691274051102,114.395878185609));
#56874=CARTESIAN_POINT('Ctrl Pts',(-5.48982104367894,5.69612418727276,114.394315581653));
#56875=CARTESIAN_POINT('Ctrl Pts',(-5.4849971500352,5.70076943158283,114.394045883204));
#56876=CARTESIAN_POINT('Ctrl Pts',(-5.4770922277948,5.70836227909637,114.393603684081));
#56877=CARTESIAN_POINT('Ctrl Pts',(-5.47401469704151,5.71131353347008,114.393431467554));
#56878=CARTESIAN_POINT('Ctrl Pts',(-5.46850207577078,5.71659141361181,114.393122873989));
#56879=CARTESIAN_POINT('Ctrl Pts',(-5.46606788056069,5.71891897721289,114.392986570383));
#56880=CARTESIAN_POINT('Ctrl Pts',(-5.46091332779494,5.7238414338761,114.392697855796));
#56881=CARTESIAN_POINT('Ctrl Pts',(-5.45819260626598,5.72643594277061,114.39254541471));
#56882=CARTESIAN_POINT('Ctrl Pts',(-5.45093435159827,5.73334761912903,114.392138602921));
#56883=CARTESIAN_POINT('Ctrl Pts',(-5.44639357780424,5.73766130248945,114.391883959673));
#56884=CARTESIAN_POINT('Ctrl Pts',(-5.42448668206845,5.75842316618419,114.390654767073));
#56885=CARTESIAN_POINT('Ctrl Pts',(-5.40705132218461,5.77479775406727,114.389674457737));
#56886=CARTESIAN_POINT('Ctrl Pts',(-5.26623745052928,5.90584768139919,114.381743177298));
#56887=CARTESIAN_POINT('Ctrl Pts',(-5.13930613276481,6.01662857498759,114.374508597872));
#56888=CARTESIAN_POINT('Ctrl Pts',(-4.86460079320475,6.24134256698503,114.3588669934));
#56889=CARTESIAN_POINT('Ctrl Pts',(-4.71613239345001,6.35427320065368,114.350422629969));
#56890=CARTESIAN_POINT('Ctrl Pts',(-4.43257918872856,6.55453875103664,114.334515246114));
#56891=CARTESIAN_POINT('Ctrl Pts',(-4.29854723023253,6.64320910692246,114.327081486576));
#56892=CARTESIAN_POINT('Ctrl Pts',(-3.87428048504851,6.90566887179359,114.303992480968));
#56893=CARTESIAN_POINT('Ctrl Pts',(-3.5755236402543,7.06498142123424,114.288369901359));
#56894=CARTESIAN_POINT('Ctrl Pts',(-2.9134483279361,7.36524643234313,114.255847807305));
#56895=CARTESIAN_POINT('Ctrl Pts',(-2.54804195562352,7.49950503779965,114.239161662206));
#56896=CARTESIAN_POINT('Ctrl Pts',(-2.15008285076706,7.61325778860508,114.222400886701));
#56897=CARTESIAN_POINT('Ctrl Pts',(-2.12592787847292,7.62003812930556,114.221388781452));
#56898=CARTESIAN_POINT('Ctrl Pts',(-2.09258626203811,7.62922629812788,114.21999888458));
#56899=CARTESIAN_POINT('Ctrl Pts',(-2.08342705887356,7.63173262525021,114.219617809274));
#56900=CARTESIAN_POINT('Ctrl Pts',(-2.06882576587508,7.63569988281892,114.219011486479));
#56901=CARTESIAN_POINT('Ctrl Pts',(-2.0633866037437,7.63717149694125,114.218785883176));
#56902=CARTESIAN_POINT('Ctrl Pts',(-2.05279813065841,7.64002416601828,114.218347202487));
#56903=CARTESIAN_POINT('Ctrl Pts',(-2.04764898697989,7.64140582935227,114.218134104919));
#56904=CARTESIAN_POINT('Ctrl Pts',(-2.03532496956186,7.64469936637174,114.217624627555));
#56905=CARTESIAN_POINT('Ctrl Pts',(-2.0281487872562,7.64660634733251,114.217328410688));
#56906=CARTESIAN_POINT('Ctrl Pts',(-2.00661116098096,7.65229725096662,114.216440724345));
#56907=CARTESIAN_POINT('Ctrl Pts',(-1.99224169792055,7.65605084810427,114.215850263146));
#56908=CARTESIAN_POINT('Ctrl Pts',(-1.86690511802338,7.68841456343842,114.210715446017));
#56909=CARTESIAN_POINT('Ctrl Pts',(-1.75533649285171,7.71465154167654,114.206250352622));
#56910=CARTESIAN_POINT('Ctrl Pts',(-1.33983526939512,7.80288177173758,114.189981967903));
#56911=CARTESIAN_POINT('Ctrl Pts',(-1.03289807400134,7.84941168923707,114.178686900753));
#56912=CARTESIAN_POINT('Ctrl Pts',(0.0588799863000562,7.94975086287487,
114.140011739207));
#56913=CARTESIAN_POINT('Ctrl Pts',(0.847967369154513,7.90459197026372,114.115144751372));
#56914=CARTESIAN_POINT('Ctrl Pts',(1.68431394085534,7.7299219381343,114.082019335349));
#56915=CARTESIAN_POINT('Ctrl Pts',(1.7511335334382,7.71505913495567,114.079321329593));
#56916=CARTESIAN_POINT('Ctrl Pts',(1.82678330603892,7.69719883478677,114.076199620795));
#56917=CARTESIAN_POINT('Ctrl Pts',(1.83581283990184,7.69505025096701,114.075825923681));
#56918=CARTESIAN_POINT('Ctrl Pts',(1.84899686870546,7.69188857600627,114.075278666567));
#56919=CARTESIAN_POINT('Ctrl Pts',(1.85315438556888,7.69088799224674,114.075105856044));
#56920=CARTESIAN_POINT('Ctrl Pts',(1.86051047390233,7.68911130168749,114.074799673773));
#56921=CARTESIAN_POINT('Ctrl Pts',(1.86370937934513,7.68833656797847,114.074666384998));
#56922=CARTESIAN_POINT('Ctrl Pts',(1.87035243493749,7.68672331585019,114.074389294576));
#56923=CARTESIAN_POINT('Ctrl Pts',(1.87379649371323,7.68588448165218,114.074245473806));
#56924=CARTESIAN_POINT('Ctrl Pts',(1.88274041433374,7.68369973334673,114.073871557327));
#56925=CARTESIAN_POINT('Ctrl Pts',(1.88823938672965,7.68235023141181,114.073641244299));
#56926=CARTESIAN_POINT('Ctrl Pts',(1.91171013888337,7.67656355530988,114.072656447187));
#56927=CARTESIAN_POINT('Ctrl Pts',(1.92966763024812,7.67206924495204,114.071898537022));
#56928=CARTESIAN_POINT('Ctrl Pts',(2.05449275917079,7.6403626693165,114.066600103834));
#56929=CARTESIAN_POINT('Ctrl Pts',(2.16079255226994,7.6109825667969,114.061934455314));
#56930=CARTESIAN_POINT('Ctrl Pts',(2.50380509418856,7.50841274039745,114.046458814773));
#56931=CARTESIAN_POINT('Ctrl Pts',(2.73769287654617,7.4263264640513,114.035251988419));
#56932=CARTESIAN_POINT('Ctrl Pts',(3.15479090092532,7.25755546955799,114.014527643675));
#56933=CARTESIAN_POINT('Ctrl Pts',(3.33927393124967,7.17454281985285,114.005084804466));
#56934=CARTESIAN_POINT('Ctrl Pts',(3.89376392774937,6.8990123644565,113.976192124441));
#56935=CARTESIAN_POINT('Ctrl Pts',(4.25192966638275,6.68422848173635,113.956845897423));
#56936=CARTESIAN_POINT('Ctrl Pts',(4.8626118366503,6.24898031886751,113.9236344417));
#56937=CARTESIAN_POINT('Ctrl Pts',(5.1212611733734,6.03883013881877,113.909473258998));
#56938=CARTESIAN_POINT('Ctrl Pts',(5.3822513094109,5.79791218556196,113.895093966686));
#56939=CARTESIAN_POINT('Ctrl Pts',(5.39851734326731,5.78276969750192,113.894197294112));
#56940=CARTESIAN_POINT('Ctrl Pts',(5.42066801867198,5.76197412397302,113.892975501419));
#56941=CARTESIAN_POINT('Ctrl Pts',(5.4266079614961,5.75638025209686,113.892647792545));
#56942=CARTESIAN_POINT('Ctrl Pts',(5.43670604587886,5.74684097801868,113.892090551353));
#56943=CARTESIAN_POINT('Ctrl Pts',(5.44086856724014,5.74290023334393,113.891860814908));
#56944=CARTESIAN_POINT('Ctrl Pts',(5.44919961476439,5.73499587141712,113.891400935756));
#56945=CARTESIAN_POINT('Ctrl Pts',(5.4533681084395,5.73103222471857,113.891170794579));
#56946=CARTESIAN_POINT('Ctrl Pts',(5.46289314610155,5.72195546213095,113.890644832419));
#56947=CARTESIAN_POINT('Ctrl Pts',(5.46824684495901,5.71683936098624,113.890349143244));
#56948=CARTESIAN_POINT('Ctrl Pts',(5.48425334796483,5.70150017175247,113.889464894832));
#56949=CARTESIAN_POINT('Ctrl Pts',(5.49488475173091,5.69125474402982,113.888877322696));
#56950=CARTESIAN_POINT('Ctrl Pts',(5.51903674805535,5.66784883122372,113.887541872946));
#56951=CARTESIAN_POINT('Ctrl Pts',(5.53253908791069,5.65466959663575,113.886794829965));
#56952=CARTESIAN_POINT('Ctrl Pts',(5.65164444441297,5.53757939112244,113.88020081793));
#56953=CARTESIAN_POINT('Ctrl Pts',(5.75435917667658,5.43076640795265,113.874485146649));
#56954=CARTESIAN_POINT('Ctrl Pts',(6.02854405522238,5.12912303299153,113.859088550451));
#56955=CARTESIAN_POINT('Ctrl Pts',(6.19352483388177,4.92864156006523,113.84966904665));
#56956=CARTESIAN_POINT('Ctrl Pts',(6.82867221923104,4.07444695933599,113.811984482845));
#56957=CARTESIAN_POINT('Ctrl Pts',(7.20749988035636,3.35908245583782,113.786347561572));
#56958=CARTESIAN_POINT('Ctrl Pts',(7.4870047275012,2.55554329361777,113.752919138255));
#56959=CARTESIAN_POINT('Ctrl Pts',(7.50175231976099,2.5119222201467,113.751089566115));
#56960=CARTESIAN_POINT('Ctrl Pts',(7.51890708148125,2.45968234143464,113.748882736262));
#56961=CARTESIAN_POINT('Ctrl Pts',(7.52168183986271,2.45118404441712,113.74852323687));
#56962=CARTESIAN_POINT('Ctrl Pts',(7.52616685384855,2.43736839383444,113.747938014027));
#56963=CARTESIAN_POINT('Ctrl Pts',(7.52788589874087,2.43205388396971,113.74771270577));
#56964=CARTESIAN_POINT('Ctrl Pts',(7.53093099026241,2.422605676911,113.747311819562));
#56965=CARTESIAN_POINT('Ctrl Pts',(7.53225926684657,2.41847269630847,113.747136345548));
#56966=CARTESIAN_POINT('Ctrl Pts',(7.53504121021527,2.4097920563301,113.746767558863));
#56967=CARTESIAN_POINT('Ctrl Pts',(7.53649416312275,2.40524417127762,113.746574213396));
#56968=CARTESIAN_POINT('Ctrl Pts',(7.54029525891965,2.39330910927881,113.746066468241));
#56969=CARTESIAN_POINT('Ctrl Pts',(7.54263665943547,2.38591980321354,113.74575176189));
#56970=CARTESIAN_POINT('Ctrl Pts',(7.55292174158578,2.35329431502966,113.744360758988));
#56971=CARTESIAN_POINT('Ctrl Pts',(7.56074959699998,2.32802200922963,113.743279299989));
#56972=CARTESIAN_POINT('Ctrl Pts',(7.75756735472088,1.68112999105057,113.715503962785));
#56973=CARTESIAN_POINT('Ctrl Pts',(7.86938896930225,1.03863170025377,113.685944336042));
#56974=CARTESIAN_POINT('Ctrl Pts',(7.92641764586476,-0.117614165030195,
113.635016451404));
#56975=CARTESIAN_POINT('Ctrl Pts',(7.90252346158347,-0.62620806724524,113.613344034359));
#56976=CARTESIAN_POINT('Ctrl Pts',(7.82518086677541,-1.16258964015839,113.591379570098));
#56977=CARTESIAN_POINT('Ctrl Pts',(7.82012697233585,-1.19611221478048,113.590010111831));
#56978=CARTESIAN_POINT('Ctrl Pts',(7.81288533224873,-1.24213719873356,113.588134155333));
#56979=CARTESIAN_POINT('Ctrl Pts',(7.81088277490538,-1.25466820845354,113.587623830588));
#56980=CARTESIAN_POINT('Ctrl Pts',(7.80727400160041,-1.27690660402853,113.586718924017));
#56981=CARTESIAN_POINT('Ctrl Pts',(7.80567981208698,-1.28661590354036,113.586324095544));
#56982=CARTESIAN_POINT('Ctrl Pts',(7.80251173316728,-1.30568824637023,113.58554900914));
#56983=CARTESIAN_POINT('Ctrl Pts',(7.8009390932224,-1.31505148467227,113.585168725657));
#56984=CARTESIAN_POINT('Ctrl Pts',(7.79723441097925,-1.33686804520771,113.584283193993));
#56985=CARTESIAN_POINT('Ctrl Pts',(7.79508938154828,-1.34931914867162,113.583778213904));
#56986=CARTESIAN_POINT('Ctrl Pts',(7.78813676358106,-1.38910659673721,113.582165850738));
#56987=CARTESIAN_POINT('Ctrl Pts',(7.78321511944348,-1.41642288989412,113.581060835815));
#56988=CARTESIAN_POINT('Ctrl Pts',(7.66678450436959,-2.04370467583689,113.55572993481));
#56989=CARTESIAN_POINT('Ctrl Pts',(7.4863738679513,-2.62879948481135,113.533259426344));
#56990=CARTESIAN_POINT('Ctrl Pts',(7.06392079686754,-3.58845200226038,113.495310003127));
#56991=CARTESIAN_POINT('Ctrl Pts',(6.85434488320203,-3.97415172240473,113.479643838835));
#56992=CARTESIAN_POINT('Ctrl Pts',(6.53959894218909,-4.4537534603533,113.457727623592));
#56993=CARTESIAN_POINT('Ctrl Pts',(6.46237452036348,-4.56508347149693,113.452449317373));
#56994=CARTESIAN_POINT('Ctrl Pts',(6.3742674321451,-4.68538387186075,113.446476530752));
#56995=CARTESIAN_POINT('Ctrl Pts',(6.36617359083058,-4.69637531840089,113.445928285819));
#56996=CARTESIAN_POINT('Ctrl Pts',(6.35484678790306,-4.71167404498058,113.445161586739));
#56997=CARTESIAN_POINT('Ctrl Pts',(6.35163778310411,-4.71599909625832,113.444944432054));
#56998=CARTESIAN_POINT('Ctrl Pts',(6.3460182225041,-4.72355692050891,113.444564252095));
#56999=CARTESIAN_POINT('Ctrl Pts',(6.34360960439008,-4.72679113655732,113.444401333316));
#57000=CARTESIAN_POINT('Ctrl Pts',(6.33855057286811,-4.73357341219581,113.444059203664));
#57001=CARTESIAN_POINT('Ctrl Pts',(6.33589965165436,-4.73712108959628,113.443879964625));
#57002=CARTESIAN_POINT('Ctrl Pts',(6.32957316061572,-4.74557290164447,113.443452287811));
#57003=CARTESIAN_POINT('Ctrl Pts',(6.32589487201399,-4.75047498975805,113.44320369758));
#57004=CARTESIAN_POINT('Ctrl Pts',(6.31350720015219,-4.76694425043252,113.442366704036));
#57005=CARTESIAN_POINT('Ctrl Pts',(6.30477179427587,-4.77849173598575,113.441776820024));
#57006=CARTESIAN_POINT('Ctrl Pts',(6.08666405560422,-5.06517295359002,113.427055254306));
#57007=CARTESIAN_POINT('Ctrl Pts',(5.85955233316282,-5.32625656427809,113.411753347226));
#57008=CARTESIAN_POINT('Ctrl Pts',(5.39869151786496,-5.79080179627688,113.381995723101));
#57009=CARTESIAN_POINT('Ctrl Pts',(5.16858957679347,-5.99707730297325,113.367662346137));
#57010=CARTESIAN_POINT('Ctrl Pts',(4.58845575924935,-6.45889000144918,113.333622188026));
#57011=CARTESIAN_POINT('Ctrl Pts',(4.22831924378883,-6.70019168064386,113.314157838926));
#57012=CARTESIAN_POINT('Ctrl Pts',(3.69616826818806,-6.9966677571959,113.288276197032));
#57013=CARTESIAN_POINT('Ctrl Pts',(3.53928302775982,-7.07732298161823,113.280961283663));
#57014=CARTESIAN_POINT('Ctrl Pts',(3.36468926893079,-7.15982313962474,113.273157454912));
#57015=CARTESIAN_POINT('Ctrl Pts',(3.34953012987038,-7.16692745748346,113.272482597376));
#57016=CARTESIAN_POINT('Ctrl Pts',(3.32704583357555,-7.17737778512299,113.271485630024));
#57017=CARTESIAN_POINT('Ctrl Pts',(3.31973798389758,-7.18076079310896,113.271162218404));
#57018=CARTESIAN_POINT('Ctrl Pts',(3.30724600029924,-7.18652053620013,113.270610441837));
#57019=CARTESIAN_POINT('Ctrl Pts',(3.30206444543268,-7.18890283159546,113.270381881455));
#57020=CARTESIAN_POINT('Ctrl Pts',(3.29167140158531,-7.19366757777455,113.269924062897));
#57021=CARTESIAN_POINT('Ctrl Pts',(3.28645989090551,-7.19604997350592,113.269694806739));
#57022=CARTESIAN_POINT('Ctrl Pts',(3.27445417039002,-7.20152251931124,113.269167390882));
#57023=CARTESIAN_POINT('Ctrl Pts',(3.26765816165978,-7.20460872282955,113.268869369869));
#57024=CARTESIAN_POINT('Ctrl Pts',(3.24816418322325,-7.21342807170229,113.268016028233));
#57025=CARTESIAN_POINT('Ctrl Pts',(3.23545539294149,-7.21913731062699,113.267461546307));
#57026=CARTESIAN_POINT('Ctrl Pts',(3.20609059306456,-7.23223590117682,113.266184588281));
#57027=CARTESIAN_POINT('Ctrl Pts',(3.18942397469236,-7.23960135205334,113.265462949212));
#57028=CARTESIAN_POINT('Ctrl Pts',(3.13593070440558,-7.26302096518825,113.263156703382));
#57029=CARTESIAN_POINT('Ctrl Pts',(3.09900689494922,-7.27885233053718,113.261579857334));
#57030=CARTESIAN_POINT('Ctrl Pts',(2.95584546753655,-7.33894705868507,113.255522971119));
#57031=CARTESIAN_POINT('Ctrl Pts',(2.84876536721906,-7.38117223719992,113.251113276011));
#57032=CARTESIAN_POINT('Ctrl Pts',(2.49948272882219,-7.5101720318603,113.237087251311));
#57033=CARTESIAN_POINT('Ctrl Pts',(2.2539543452568,-7.58747646056536,113.227781532307));
#57034=CARTESIAN_POINT('Ctrl Pts',(1.17205725711898,-7.87094498829714,113.188429609568));
#57035=CARTESIAN_POINT('Ctrl Pts',(0.30916061301062,-7.95169086946019,113.161798096139));
#57036=CARTESIAN_POINT('Ctrl Pts',(-0.595606776303615,-7.88868179284596,
113.126216452307));
#57037=CARTESIAN_POINT('Ctrl Pts',(-0.641583470141476,-7.88507567170836,
113.124385924291));
#57038=CARTESIAN_POINT('Ctrl Pts',(-0.695584827526059,-7.88036472512556,
113.122206944979));
#57039=CARTESIAN_POINT('Ctrl Pts',(-0.703643425308883,-7.87964925503474,
113.12188101817));
#57040=CARTESIAN_POINT('Ctrl Pts',(-0.715810113849971,-7.87855024128623,
113.121387777422));
#57041=CARTESIAN_POINT('Ctrl Pts',(-0.719919046565194,-7.87817584151481,
113.121220999717));
#57042=CARTESIAN_POINT('Ctrl Pts',(-0.727272001827565,-7.87750005077193,
113.120922188529));
#57043=CARTESIAN_POINT('Ctrl Pts',(-0.730516131327986,-7.87719987027768,
113.120790226636));
#57044=CARTESIAN_POINT('Ctrl Pts',(-0.737411737973479,-7.87655752084076,
113.120509466215));
#57045=CARTESIAN_POINT('Ctrl Pts',(-0.74106316604755,-7.87621481641108,
113.120360636165));
#57046=CARTESIAN_POINT('Ctrl Pts',(-0.750838307265465,-7.8752905136588,
113.119961783876));
#57047=CARTESIAN_POINT('Ctrl Pts',(-0.756961571848057,-7.87470431295756,
113.119711493232));
#57048=CARTESIAN_POINT('Ctrl Pts',(-0.785993051777178,-7.87189085735959,
113.118522733498));
#57049=CARTESIAN_POINT('Ctrl Pts',(-0.80889194799356,-7.86957079788246,
113.117578922005));
#57050=CARTESIAN_POINT('Ctrl Pts',(-0.988510200437143,-7.85058007281931,
113.110129193246));
#57051=CARTESIAN_POINT('Ctrl Pts',(-1.14470153439236,-7.82933027936056,
113.103373570541));
#57052=CARTESIAN_POINT('Ctrl Pts',(-1.542930816378,-7.76298055049504,113.08562738993));
#57053=CARTESIAN_POINT('Ctrl Pts',(-1.78368706416445,-7.71122248394325,
113.074402377143));
#57054=CARTESIAN_POINT('Ctrl Pts',(-2.31499858640699,-7.57078482436854,
113.049067791044));
#57055=CARTESIAN_POINT('Ctrl Pts',(-2.60367181645543,-7.47642290844188,
113.034921593991));
#57056=CARTESIAN_POINT('Ctrl Pts',(-3.05455905556037,-7.29974537617735,
113.012742248698));
#57057=CARTESIAN_POINT('Ctrl Pts',(-3.22060071417901,-7.22802522629254,
113.004552534517));
#57058=CARTESIAN_POINT('Ctrl Pts',(-3.70784019814695,-6.99744005022162,
112.980579426672));
#57059=CARTESIAN_POINT('Ctrl Pts',(-4.02087626336123,-6.82237828610346,
112.965279104118));
#57060=CARTESIAN_POINT('Ctrl Pts',(-4.34117711907326,-6.61352270456729,
112.949800663924));
#57061=CARTESIAN_POINT('Ctrl Pts',(-4.3612963721988,-6.60027236639864,112.94882905397));
#57062=CARTESIAN_POINT('Ctrl Pts',(-4.38835059883131,-6.58227700831028,
112.947523357466));
#57063=CARTESIAN_POINT('Ctrl Pts',(-4.39533888667246,-6.57761261129523,
112.947186161516));
#57064=CARTESIAN_POINT('Ctrl Pts',(-4.40711457031713,-6.56972567673556,
112.946618088214));
#57065=CARTESIAN_POINT('Ctrl Pts',(-4.41190588733069,-6.56650902268415,
112.946386983429));
#57066=CARTESIAN_POINT('Ctrl Pts',(-4.4214747627516,-6.56006975058397,112.94592550455));
#57067=CARTESIAN_POINT('Ctrl Pts',(-4.42625232816286,-6.55684714918671,
112.945695130024));
#57068=CARTESIAN_POINT('Ctrl Pts',(-4.43698240846079,-6.54959233830433,
112.945177798636));
#57069=CARTESIAN_POINT('Ctrl Pts',(-4.44293296007714,-6.54555722636256,
112.944890954718));
#57070=CARTESIAN_POINT('Ctrl Pts',(-4.45531895069065,-6.53713352486124,
112.944293996935));
#57071=CARTESIAN_POINT('Ctrl Pts',(-4.46175342713752,-6.53274353010524,
112.943983938132));
#57072=CARTESIAN_POINT('Ctrl Pts',(-4.47844544623616,-6.52131904492611,
112.943179745593));
#57073=CARTESIAN_POINT('Ctrl Pts',(-4.48869291986336,-6.51426984194363,
112.942686185144));
#57074=CARTESIAN_POINT('Ctrl Pts',(-4.51871576048691,-6.49351275071951,
112.941240565419));
#57075=CARTESIAN_POINT('Ctrl Pts',(-4.53844534209447,-6.47973871834073,
112.940291089055));
#57076=CARTESIAN_POINT('Ctrl Pts',(-4.60590931666847,-6.43218005786104,
112.937045983586));
#57077=CARTESIAN_POINT('Ctrl Pts',(-4.65333226732243,-6.39795591778388,
112.934767598431));
#57078=CARTESIAN_POINT('Ctrl Pts',(-4.82168783247279,-6.27359510542896,
112.926685149101));
#57079=CARTESIAN_POINT('Ctrl Pts',(-4.94041929840592,-6.18052822270472,
112.920997108455));
#57080=CARTESIAN_POINT('Ctrl Pts',(-5.20538048682271,-5.96032294486073,
112.908272664376));
#57081=CARTESIAN_POINT('Ctrl Pts',(-5.34974655763972,-5.83109353661543,
112.901317619394));
#57082=CARTESIAN_POINT('Ctrl Pts',(-6.05050445451427,-5.15585597485429,
112.867037859177));
#57083=CARTESIAN_POINT('Ctrl Pts',(-6.52867205715385,-4.53514374839793,
112.842325521851));
#57084=CARTESIAN_POINT('Ctrl Pts',(-6.94081453738616,-3.79650555720081,
112.809519852572));
#57085=CARTESIAN_POINT('Ctrl Pts',(-6.97254440708817,-3.73791183799385,
112.806893877122));
#57086=CARTESIAN_POINT('Ctrl Pts',(-7.00782656225619,-3.67074559937355,
112.803849158977));
#57087=CARTESIAN_POINT('Ctrl Pts',(-7.01210928499735,-3.66255781606667,
112.803477418164));
#57088=CARTESIAN_POINT('Ctrl Pts',(-7.01837268125978,-3.65053209268946,
112.802930550645));
#57089=CARTESIAN_POINT('Ctrl Pts',(-7.02036458387028,-3.6466999824783,112.802756155788));
#57090=CARTESIAN_POINT('Ctrl Pts',(-7.02391148859713,-3.63986261416544,
112.802444765479));
#57091=CARTESIAN_POINT('Ctrl Pts',(-7.02546770404296,-3.63685798307104,
112.80230784829));
#57092=CARTESIAN_POINT('Ctrl Pts',(-7.02871769563886,-3.63057325816955,
112.802021297804));
#57093=CARTESIAN_POINT('Ctrl Pts',(-7.03041110411858,-3.62729297616298,
112.801871641044));
#57094=CARTESIAN_POINT('Ctrl Pts',(-7.0348175238976,-3.61874267378419,112.80148130938));
#57095=CARTESIAN_POINT('Ctrl Pts',(-7.03752690523141,-3.61347079570145,
112.801240404346));
#57096=CARTESIAN_POINT('Ctrl Pts',(-7.04917846290029,-3.59073653946237,
112.800200528583));
#57097=CARTESIAN_POINT('Ctrl Pts',(-7.058061521376,-3.57324410659505,112.799397861659));
#57098=CARTESIAN_POINT('Ctrl Pts',(-7.12023786558303,-3.44967058241966,
112.793710528407));
#57099=CARTESIAN_POINT('Ctrl Pts',(-7.17120023135378,-3.34243910032111,
112.788687452431));
#57100=CARTESIAN_POINT('Ctrl Pts',(-7.28510033603492,-3.08817172352702,
112.776645170133));
#57101=CARTESIAN_POINT('Ctrl Pts',(-7.34603010978106,-2.94029401555891,
112.769541268623));
#57102=CARTESIAN_POINT('Ctrl Pts',(-7.73854961810325,-1.89911352877953,
112.719321585755));
#57103=CARTESIAN_POINT('Ctrl Pts',(-7.91092258247302,-0.953821026728434,
112.673985643915));
#57104=CARTESIAN_POINT('Ctrl Pts',(-7.91099997392412,-0.000642317922101565,
112.635042636927));
#57105=CARTESIAN_POINT('',(-7.911,4.87276885507981E-12,110.642331508237));
#57106=CARTESIAN_POINT('Ctrl Pts',(-7.911,5.49282841433296E-12,112.642331508237));
#57107=CARTESIAN_POINT('Ctrl Pts',(-7.91099999999847,2.20167589667229,112.553744072504));
#57108=CARTESIAN_POINT('Ctrl Pts',(-6.94214576672064,4.38610418339171,112.465156636771));
#57109=CARTESIAN_POINT('Ctrl Pts',(-3.67820201487766,7.34180684107894,112.287981765306));
#57110=CARTESIAN_POINT('Ctrl Pts',(-1.40868175871167,8.08992666571438,112.199394329573));
#57111=CARTESIAN_POINT('Ctrl Pts',(2.97309270521825,7.65454228025044,112.022219458108));
#57112=CARTESIAN_POINT('Ctrl Pts',(5.05102072676072,6.4744488083386,111.933632022375));
#57113=CARTESIAN_POINT('Ctrl Pts',(7.66951518848087,2.93425195367147,111.75645715091));
#57114=CARTESIAN_POINT('Ctrl Pts',(8.18956872247117,0.60188196009315,111.667869715177));
#57115=CARTESIAN_POINT('Ctrl Pts',(7.32306689761068,-3.71537198232993,111.490694843711));
#57116=CARTESIAN_POINT('Ctrl Pts',(5.9432995884978,-5.66643518936954,111.402107407979));
#57117=CARTESIAN_POINT('Ctrl Pts',(2.16154501637252,-7.92205913233161,111.224932536513));
#57118=CARTESIAN_POINT('Ctrl Pts',(-0.210816529306575,-8.20894963712987,
111.13634510078));
#57119=CARTESIAN_POINT('Ctrl Pts',(-4.42123908576965,-6.91982244717495,
110.959170229315));
#57120=CARTESIAN_POINT('Ctrl Pts',(-6.22631625634599,-5.35390358803044,
110.870582793582));
#57121=CARTESIAN_POINT('Ctrl Pts',(-7.65317280859649,-2.31334857513966,
110.735440741312));
#57122=CARTESIAN_POINT('Ctrl Pts',(-7.91100000000071,-1.15702837835991,
110.688886124774));
#57123=CARTESIAN_POINT('Ctrl Pts',(-7.911,4.87276885507981E-12,110.642331508237));
#57124=CARTESIAN_POINT('',(-7.91812613509609,-0.0016953829844947,108.642276941385));
#57125=CARTESIAN_POINT('Ctrl Pts',(-7.911,4.87276885507981E-12,110.642331508237));
#57126=CARTESIAN_POINT('Ctrl Pts',(-7.91099999999864,2.20167589667137,110.553744072504));
#57127=CARTESIAN_POINT('Ctrl Pts',(-6.94214576672126,4.38610418339058,110.465156636771));
#57128=CARTESIAN_POINT('Ctrl Pts',(-3.67820201487929,7.34180684107803,110.287981765306));
#57129=CARTESIAN_POINT('Ctrl Pts',(-1.40868175871384,8.08992666571392,110.199394329573));
#57130=CARTESIAN_POINT('Ctrl Pts',(2.97309270521562,7.65454228025138,110.022219458108));
#57131=CARTESIAN_POINT('Ctrl Pts',(5.05102072675818,6.47444880834048,109.933632022375));
#57132=CARTESIAN_POINT('Ctrl Pts',(7.66951518847946,2.93425195367492,109.75645715091));
#57133=CARTESIAN_POINT('Ctrl Pts',(8.18956872247078,0.601881960097223,109.667869715177));
#57134=CARTESIAN_POINT('Ctrl Pts',(7.32306689761272,-3.71537198232573,109.490694843712));
#57135=CARTESIAN_POINT('Ctrl Pts',(5.9432995885012,-5.66643518936585,109.402107407979));
#57136=CARTESIAN_POINT('Ctrl Pts',(2.1615450163779,-7.92205913233006,109.224932536513));
#57137=CARTESIAN_POINT('Ctrl Pts',(-0.210816529300619,-8.20894963712995,
109.136345100781));
#57138=CARTESIAN_POINT('Ctrl Pts',(-4.42123908576411,-6.9198224471784,108.959170229315));
#57139=CARTESIAN_POINT('Ctrl Pts',(-6.22631625634144,-5.35390358803561,
108.870582793583));
#57140=CARTESIAN_POINT('Ctrl Pts',(-7.65292805026068,-2.31387014206744,
108.73546392314));
#57141=CARTESIAN_POINT('Ctrl Pts',(-7.91074317242851,-1.15817992851268,
108.688932488431));
#57142=CARTESIAN_POINT('Ctrl Pts',(-7.91099980821568,-0.00172842309520182,
108.642401053722));
#57143=CARTESIAN_POINT('',(-7.90355940251074,-0.00222154607187651,106.642331508237));
#57144=CARTESIAN_POINT('Ctrl Pts',(-7.92321969856481,-0.00167176746646912,
108.642188231721));
#57145=CARTESIAN_POINT('Ctrl Pts',(-7.90990747858981,2.44136070272242,108.543454857439));
#57146=CARTESIAN_POINT('Ctrl Pts',(-5.38153242390624,7.53592095794861,108.338787103357));
#57147=CARTESIAN_POINT('Ctrl Pts',(3.28116688241203,8.75427127644514,108.028184969472));
#57148=CARTESIAN_POINT('Ctrl Pts',(9.14177665892542,1.98895403673894,107.710381830063));
#57149=CARTESIAN_POINT('Ctrl Pts',(6.61600493471317,-6.61592908789789,107.392578690655));
#57150=CARTESIAN_POINT('Ctrl Pts',(-0.534690503584316,-8.70980249966465,
107.12774274115));
#57151=CARTESIAN_POINT('Ctrl Pts',(-5.36923601473013,-6.22858863134672,
106.915873981543));
#57152=CARTESIAN_POINT('Ctrl Pts',(-7.52371069543634,-3.22405648818859,
106.771725967208));
#57153=CARTESIAN_POINT('Ctrl Pts',(-7.90357192039929,-0.955852324005775,
106.680545142771));
#57154=CARTESIAN_POINT('Ctrl Pts',(-7.89827895664709,-0.00379813367885562,
106.642331508237));
#57155=CARTESIAN_POINT('',(-7.9109999128679,0.00033058666535775,104.642331508237));
#57156=CARTESIAN_POINT('Ctrl Pts',(-7.911,4.53193038651989E-12,106.642331508237));
#57157=CARTESIAN_POINT('Ctrl Pts',(-7.91099999999874,2.20167589667133,106.553744072504));
#57158=CARTESIAN_POINT('Ctrl Pts',(-6.94214576672117,4.38610418339086,106.465156636771));
#57159=CARTESIAN_POINT('Ctrl Pts',(-3.67820201487855,7.34180684107849,106.287981765306));
#57160=CARTESIAN_POINT('Ctrl Pts',(-1.40868175871265,8.08992666571421,106.199394329573));
#57161=CARTESIAN_POINT('Ctrl Pts',(2.97309270521732,7.6545422802508,106.022219458108));
#57162=CARTESIAN_POINT('Ctrl Pts',(5.05102072675993,6.47444880833922,105.933632022375));
#57163=CARTESIAN_POINT('Ctrl Pts',(7.66951518848051,2.9342519536724,105.75645715091));
#57164=CARTESIAN_POINT('Ctrl Pts',(8.18956872247109,0.601881960094145,105.667869715177));
#57165=CARTESIAN_POINT('Ctrl Pts',(7.32306689761113,-3.71537198232904,105.490694843711));
#57166=CARTESIAN_POINT('Ctrl Pts',(5.94329958849849,-5.66643518936882,105.402107407979));
#57167=CARTESIAN_POINT('Ctrl Pts',(2.16154501637348,-7.92205913233135,105.224932536513));
#57168=CARTESIAN_POINT('Ctrl Pts',(-0.210816529305578,-8.2089496371299,
105.13634510078));
#57169=CARTESIAN_POINT('Ctrl Pts',(-4.42123908576881,-6.91982244717548,
104.959170229315));
#57170=CARTESIAN_POINT('Ctrl Pts',(-6.22631625634534,-5.35390358803119,
104.870582793582));
#57171=CARTESIAN_POINT('Ctrl Pts',(-7.65317280859634,-2.31334857514032,
104.735440741312));
#57172=CARTESIAN_POINT('Ctrl Pts',(-7.9110000000007,-1.15702837836027,104.688886124774));
#57173=CARTESIAN_POINT('Ctrl Pts',(-7.911,4.81115147721312E-12,104.642331508237));
#57174=CARTESIAN_POINT('',(-7.91099995190663,0.000872314928047417,102.642418784884));
#57175=CARTESIAN_POINT('Ctrl Pts',(-7.9109989008751,0.004170174215462,104.642331508237));
#57176=CARTESIAN_POINT('Ctrl Pts',(-7.91087854410085,0.232492124240155,
104.633166418883));
#57177=CARTESIAN_POINT('Ctrl Pts',(-7.9008690756303,0.460503234003182,104.624001329529));
#57178=CARTESIAN_POINT('Ctrl Pts',(-7.88107863799055,0.687401266953312,
104.614836240174));
#57179=CARTESIAN_POINT('Ctrl Pts',(-7.86178446149252,0.908609649227945,
104.605900972807));
#57180=CARTESIAN_POINT('Ctrl Pts',(-7.83319402724638,1.12875997869005,104.59696570544));
#57181=CARTESIAN_POINT('Ctrl Pts',(-7.79545881515053,1.34712392202496,104.588030438073));
#57182=CARTESIAN_POINT('Ctrl Pts',(-7.75626773479519,1.57391259961897,104.578750437725));
#57183=CARTESIAN_POINT('Ctrl Pts',(-7.70721240269764,1.79877409903119,104.569470437378));
#57184=CARTESIAN_POINT('Ctrl Pts',(-7.64851849464034,2.02091212999097,104.56019043703));
#57185=CARTESIAN_POINT('Ctrl Pts',(-7.58982458658305,2.24305016095075,104.550910436682));
#57186=CARTESIAN_POINT('Ctrl Pts',(-7.52149222134172,2.46246455165217,104.541630436334));
#57187=CARTESIAN_POINT('Ctrl Pts',(-7.44380231317566,2.67838162373487,104.532350435986));
#57188=CARTESIAN_POINT('Ctrl Pts',(-7.37757362925124,2.86244547267503,104.524439470143));
#57189=CARTESIAN_POINT('Ctrl Pts',(-7.30443025259769,3.04428369458642,104.5165285043));
#57190=CARTESIAN_POINT('Ctrl Pts',(-7.22454135979477,3.22334036996013,104.508617538457));
#57191=CARTESIAN_POINT('Ctrl Pts',(-7.14473330716828,3.40221585652622,104.50071457778));
#57192=CARTESIAN_POINT('Ctrl Pts',(-7.05819347429968,3.57831509117353,104.492811617103));
#57193=CARTESIAN_POINT('Ctrl Pts',(-6.96514037610916,3.75109857789608,104.484908656427));
#57194=CARTESIAN_POINT('Ctrl Pts',(-6.87216421850044,3.92373919928417,104.477012230281));
#57195=CARTESIAN_POINT('Ctrl Pts',(-6.77268568681204,4.09306923292176,104.469115804136));
#57196=CARTESIAN_POINT('Ctrl Pts',(-6.66697093203234,4.25857013461512,104.461219377991));
#57197=CARTESIAN_POINT('Ctrl Pts',(-6.56132402865668,4.42396481207731,104.453328020046));
#57198=CARTESIAN_POINT('Ctrl Pts',(-6.44944906193141,4.5855349650534,104.445436662101));
#57199=CARTESIAN_POINT('Ctrl Pts',(-6.33165769508611,4.742787348412,104.437545304157));
#57200=CARTESIAN_POINT('Ctrl Pts',(-6.21392014241337,4.8999678894351,104.429657551459));
#57201=CARTESIAN_POINT('Ctrl Pts',(-6.09027178201926,5.05283431658878,104.42176979876));
#57202=CARTESIAN_POINT('Ctrl Pts',(-5.96106726325917,5.20092281070387,104.413882046062));
#57203=CARTESIAN_POINT('Ctrl Pts',(-5.83189787679232,5.34897103774122,104.405996438141));
#57204=CARTESIAN_POINT('Ctrl Pts',(-5.69717556947778,5.49224366193245,104.398110830219));
#57205=CARTESIAN_POINT('Ctrl Pts',(-5.55729507127935,5.63031015937259,104.390225222298));
#57206=CARTESIAN_POINT('Ctrl Pts',(-5.41739807538984,5.76839294055817,104.382338684337));
#57207=CARTESIAN_POINT('Ctrl Pts',(-5.27234191345448,5.90126812124871,104.374452146377));
#57208=CARTESIAN_POINT('Ctrl Pts',(-5.12255840636323,6.02854181153266,104.366565608416));
#57209=CARTESIAN_POINT('Ctrl Pts',(-4.97275602938126,6.15583153589588,104.358678076901));
#57210=CARTESIAN_POINT('Ctrl Pts',(-4.81822538273729,6.27751813995468,104.350790545386));
#57211=CARTESIAN_POINT('Ctrl Pts',(-4.65943159300754,6.39324786240008,104.34290301387));
#57212=CARTESIAN_POINT('Ctrl Pts',(-4.50059118258624,6.50901156224285,104.335013166634));
#57213=CARTESIAN_POINT('Ctrl Pts',(-4.33748541328695,6.61881469235311,104.327123319397));
#57214=CARTESIAN_POINT('Ctrl Pts',(-4.17060881936156,6.72234654535628,104.31923347216));
#57215=CARTESIAN_POINT('Ctrl Pts',(-4.00365526062135,6.82592614807503,104.311339986063));
#57216=CARTESIAN_POINT('Ctrl Pts',(-3.83292770407638,6.92322852849717,104.303446499966));
#57217=CARTESIAN_POINT('Ctrl Pts',(-3.65894593145937,7.01398857075323,104.295553013869));
#57218=CARTESIAN_POINT('Ctrl Pts',(-3.48476303615417,7.10485353149244,104.287650402913));
#57219=CARTESIAN_POINT('Ctrl Pts',(-3.30731871620451,7.18916088826047,104.279747791957));
#57220=CARTESIAN_POINT('Ctrl Pts',(-3.12715447685737,7.26669291203852,104.271845181001));
#57221=CARTESIAN_POINT('Ctrl Pts',(-2.94687074276943,7.34427635927952,104.263937328603));
#57222=CARTESIAN_POINT('Ctrl Pts',(-2.76386381314278,7.41507539097209,104.256029476205));
#57223=CARTESIAN_POINT('Ctrl Pts',(-2.57869129941304,7.47892185962198,104.248121623806));
#57224=CARTESIAN_POINT('Ctrl Pts',(-2.39326541716374,7.54285568834986,104.240202951223));
#57225=CARTESIAN_POINT('Ctrl Pts',(-2.2056683607187,7.59981785305497,104.23228427864));
#57226=CARTESIAN_POINT('Ctrl Pts',(-2.01647003972864,7.64969081590078,104.224365606057));
#57227=CARTESIAN_POINT('Ctrl Pts',(-1.93827479305112,7.67030320089374,104.221092836231));
#57228=CARTESIAN_POINT('Ctrl Pts',(-1.85980611506728,7.68970525345834,104.217820066405));
#57229=CARTESIAN_POINT('Ctrl Pts',(-1.78110452738176,7.70789125912789,104.21454729658));
#57230=CARTESIAN_POINT('Ctrl Pts',(-1.59249761457652,7.75147368848496,104.206704163661));
#57231=CARTESIAN_POINT('Ctrl Pts',(-1.40199427875364,7.78819766795832,104.198861030742));
#57232=CARTESIAN_POINT('Ctrl Pts',(-1.21014031245643,7.81789494839678,104.191017897823));
#57233=CARTESIAN_POINT('Ctrl Pts',(-1.0185116582224,7.84755735254023,104.183183975829));
#57234=CARTESIAN_POINT('Ctrl Pts',(-0.825535875346164,7.87020943587607,
104.175350053835));
#57235=CARTESIAN_POINT('Ctrl Pts',(-0.63177296092783,7.8857329352344,104.167516131841));
#57236=CARTESIAN_POINT('Ctrl Pts',(-0.438199916876828,7.90124122294846,
104.159689886391));
#57237=CARTESIAN_POINT('Ctrl Pts',(-0.243841624972492,7.90963480966726,
104.151863640942));
#57238=CARTESIAN_POINT('Ctrl Pts',(-0.0492674952268234,7.9108465864226,
104.144037395492));
#57239=CARTESIAN_POINT('Ctrl Pts',(0.145153788286887,7.9120574112759,104.13621729789));
#57240=CARTESIAN_POINT('Ctrl Pts',(0.339790222195503,7.90609766032266,104.128397200289));
#57241=CARTESIAN_POINT('Ctrl Pts',(0.534067867171041,7.89295207848466,104.120577102687));
#57242=CARTESIAN_POINT('Ctrl Pts',(0.728230645011801,7.87981426900422,104.112761628737));
#57243=CARTESIAN_POINT('Ctrl Pts',(0.922034706765155,7.85949911554536,104.104946154787));
#57244=CARTESIAN_POINT('Ctrl Pts',(1.11490651313295,7.83204344133597,104.097130680837));
#57245=CARTESIAN_POINT('Ctrl Pts',(1.30770174640816,7.80459866745422,104.089318309752));
#57246=CARTESIAN_POINT('Ctrl Pts',(1.49956511415679,7.770019070504,104.081505938666));
#57247=CARTESIAN_POINT('Ctrl Pts',(1.68992840562266,7.72839329898975,104.07369356758));
#57248=CARTESIAN_POINT('Ctrl Pts',(1.88028449115895,7.68676910315943,104.06588149222));
#57249=CARTESIAN_POINT('Ctrl Pts',(2.06914026820764,7.63809933040576,104.058069416861));
#57250=CARTESIAN_POINT('Ctrl Pts',(2.25593746052766,7.58252379977722,104.050257341501));
#57251=CARTESIAN_POINT('Ctrl Pts',(2.44274011608328,7.52694664373765,104.042445037663));
#57252=CARTESIAN_POINT('Ctrl Pts',(2.62748372953017,7.46446342707425,104.034632733824));
#57253=CARTESIAN_POINT('Ctrl Pts',(2.80962497138708,7.39526392498322,104.026820429986));
#57254=CARTESIAN_POINT('Ctrl Pts',(2.99180358864167,7.32605022314871,104.019006523062));
#57255=CARTESIAN_POINT('Ctrl Pts',(3.17137844169123,7.25011761537827,104.011192616138));
#57256=CARTESIAN_POINT('Ctrl Pts',(3.34782583481584,7.16770417775033,104.003378709214));
#57257=CARTESIAN_POINT('Ctrl Pts',(3.52434048363695,7.08525932694565,103.995561823897));
#57258=CARTESIAN_POINT('Ctrl Pts',(3.69772497954674,6.99632887435923,103.98774493858));
#57259=CARTESIAN_POINT('Ctrl Pts',(3.8674797624686,6.90119709086009,103.979928053262));
#57260=CARTESIAN_POINT('Ctrl Pts',(4.03741869341718,6.80596210950162,103.972102688278));
#57261=CARTESIAN_POINT('Ctrl Pts',(4.20371974027894,6.70451253332006,103.964277323294));
#57262=CARTESIAN_POINT('Ctrl Pts',(4.36591101402899,6.59717682176098,103.95645195831));
#57263=CARTESIAN_POINT('Ctrl Pts',(4.52820086044954,6.48977587631181,103.948621837416));
#57264=CARTESIAN_POINT('Ctrl Pts',(4.68637567093829,6.37648187032801,103.940791716522));
#57265=CARTESIAN_POINT('Ctrl Pts',(4.83999620088008,6.25766392317983,103.932961595627));
#57266=CARTESIAN_POINT('Ctrl Pts',(4.99382671990661,6.13868355977139,103.925120771477));
#57267=CARTESIAN_POINT('Ctrl Pts',(5.1430902552499,6.01416439830458,103.917279947326));
#57268=CARTESIAN_POINT('Ctrl Pts',(5.28738318273056,5.88451358049058,103.909439123175));
#57269=CARTESIAN_POINT('Ctrl Pts',(5.3652573863346,5.81454165352118,103.905207467841));
#57270=CARTESIAN_POINT('Ctrl Pts',(5.44168446242181,5.74307562955914,103.900975812506));
#57271=CARTESIAN_POINT('Ctrl Pts',(5.51660584373181,5.67018350363585,103.896744157171));
#57272=CARTESIAN_POINT('Ctrl Pts',(5.65667304254243,5.53391004317758,103.888832982835));
#57273=CARTESIAN_POINT('Ctrl Pts',(5.79187609005824,5.39226033010117,103.880921808499));
#57274=CARTESIAN_POINT('Ctrl Pts',(5.92177708633773,5.24561503922328,103.873010634162));
#57275=CARTESIAN_POINT('Ctrl Pts',(6.05153725307177,5.09912873088015,103.865108036566));
#57276=CARTESIAN_POINT('Ctrl Pts',(6.17600659136928,4.94765788810591,103.85720543897));
#57277=CARTESIAN_POINT('Ctrl Pts',(6.29478226508762,4.79162156635292,103.849302841374));
#57278=CARTESIAN_POINT('Ctrl Pts',(6.41345121864179,4.63572544352578,103.841407344276));
#57279=CARTESIAN_POINT('Ctrl Pts',(6.52643649113257,4.47527228610266,103.833511847178));
#57280=CARTESIAN_POINT('Ctrl Pts',(6.63337375974589,4.31071613116831,103.825616350081));
#57281=CARTESIAN_POINT('Ctrl Pts',(6.74023478940494,4.14627729351104,103.817726481933));
#57282=CARTESIAN_POINT('Ctrl Pts',(6.84105621866451,3.97774157421741,103.809836613784));
#57283=CARTESIAN_POINT('Ctrl Pts',(6.93551535006845,3.80559428065642,103.801946745636));
#57284=CARTESIAN_POINT('Ctrl Pts',(7.02992466346148,3.63353777806103,103.794061038626));
#57285=CARTESIAN_POINT('Ctrl Pts',(7.11797819979438,3.45787379827077,103.786175331616));
#57286=CARTESIAN_POINT('Ctrl Pts',(7.19939763332376,3.27911492895449,103.778289624606));
#57287=CARTESIAN_POINT('Ctrl Pts',(7.28078922919831,3.1004171780652,103.770406613753));
#57288=CARTESIAN_POINT('Ctrl Pts',(7.3555511001764,2.91862696002967,103.762523602901));
#57289=CARTESIAN_POINT('Ctrl Pts',(7.42345164809672,2.73427991039142,103.754640592048));
#57290=CARTESIAN_POINT('Ctrl Pts',(7.49135320933112,2.5499301096493,103.746757463553));
#57291=CARTESIAN_POINT('Ctrl Pts',(7.55239311580177,2.36302372168847,103.738874335059));
#57292=CARTESIAN_POINT('Ctrl Pts',(7.60638835125973,2.17411527979089,103.730991206564));
#57293=CARTESIAN_POINT('Ctrl Pts',(7.66038692529708,1.98519515749554,103.723107590647));
#57294=CARTESIAN_POINT('Ctrl Pts',(7.70733986497832,1.79427306618492,103.715223974731));
#57295=CARTESIAN_POINT('Ctrl Pts',(7.74711436309768,1.60191761494953,103.707340358814));
#57296=CARTESIAN_POINT('Ctrl Pts',(7.78689800639556,1.40951793625629,103.699454930252));
#57297=CARTESIAN_POINT('Ctrl Pts',(7.81949984938443,1.21568457873006,103.69156950169));
#57298=CARTESIAN_POINT('Ctrl Pts',(7.84483838239496,1.02099547212648,103.683684073128));
#57299=CARTESIAN_POINT('Ctrl Pts',(7.87018700071214,0.826228874874966,103.675795505987));
#57300=CARTESIAN_POINT('Ctrl Pts',(7.88826650406258,0.630606191624877,103.667906938847));
#57301=CARTESIAN_POINT('Ctrl Pts',(7.89904730704057,0.434709835562825,103.660018371706));
#57302=CARTESIAN_POINT('Ctrl Pts',(7.90983958313647,0.238605003193925,103.652121409416));
#57303=CARTESIAN_POINT('Ctrl Pts',(7.91331762524989,0.0422262607709591,
103.644224447125));
#57304=CARTESIAN_POINT('Ctrl Pts',(7.90950397795936,-0.153843500496655,
103.636327484835));
#57305=CARTESIAN_POINT('Ctrl Pts',(7.90568800485134,-0.35003283823409,103.628425706448));
#57306=CARTESIAN_POINT('Ctrl Pts',(7.89457149619237,-0.545912475716475,
103.620523928061));
#57307=CARTESIAN_POINT('Ctrl Pts',(7.87622884207967,-0.740905005511776,
103.612622149674));
#57308=CARTESIAN_POINT('Ctrl Pts',(7.85786246458148,-0.936149727979011,
103.604710151559));
#57309=CARTESIAN_POINT('Ctrl Pts',(7.83225131902566,-1.1305047102084,103.596798153444));
#57310=CARTESIAN_POINT('Ctrl Pts',(7.79952102573957,-1.32340196805295,103.588886155329));
#57311=CARTESIAN_POINT('Ctrl Pts',(7.78580736940212,-1.40422393562269,103.585571109474));
#57312=CARTESIAN_POINT('Ctrl Pts',(7.77084453631388,-1.48479016593419,103.582256063619));
#57313=CARTESIAN_POINT('Ctrl Pts',(7.75464435836518,-1.56505970342194,103.578941017764));
#57314=CARTESIAN_POINT('Ctrl Pts',(7.71598356510864,-1.75661833959485,103.571029851427));
#57315=CARTESIAN_POINT('Ctrl Pts',(7.67016864698014,-1.94700105378001,103.56311868509));
#57316=CARTESIAN_POINT('Ctrl Pts',(7.6172823481017,-2.13563354283883,103.555207518754));
#57317=CARTESIAN_POINT('Ctrl Pts',(7.56445337629691,-2.32406156025142,103.547304927871));
#57318=CARTESIAN_POINT('Ctrl Pts',(7.50456838383806,-2.51074280242541,103.539402336988));
#57319=CARTESIAN_POINT('Ctrl Pts',(7.43776137105443,-2.69511164652793,103.531499746105));
#57320=CARTESIAN_POINT('Ctrl Pts',(7.37101437371167,-2.879314864643,103.523604254439));
#57321=CARTESIAN_POINT('Ctrl Pts',(7.29735786024608,-3.06120950073037,103.515708762773));
#57322=CARTESIAN_POINT('Ctrl Pts',(7.21697609892851,-3.24024335312868,103.507813271107));
#57323=CARTESIAN_POINT('Ctrl Pts',(7.13665163133336,-3.41914959553594,103.499923407112));
#57324=CARTESIAN_POINT('Ctrl Pts',(7.0496116069562,-3.59519880350818,103.492033543117));
#57325=CARTESIAN_POINT('Ctrl Pts',(6.95608912836604,-3.76785682294693,103.484143679123));
#57326=CARTESIAN_POINT('Ctrl Pts',(6.86261595870346,-3.94042380992051,103.476257974991));
#57327=CARTESIAN_POINT('Ctrl Pts',(6.76266730914396,-4.10960286866247,103.468372270859));
#57328=CARTESIAN_POINT('Ctrl Pts',(6.65652325060428,-4.27488236261124,103.460486566728));
#57329=CARTESIAN_POINT('Ctrl Pts',(6.55041546605112,-4.44010537345376,103.45260355748));
#57330=CARTESIAN_POINT('Ctrl Pts',(6.43811667836659,-4.60143118572496,103.444720548233));
#57331=CARTESIAN_POINT('Ctrl Pts',(6.31995164554021,-4.75837495349343,103.436837538985));
#57332=CARTESIAN_POINT('Ctrl Pts',(6.20178482075016,-4.91532110130211,103.428954410192));
#57333=CARTESIAN_POINT('Ctrl Pts',(6.07775177370286,-5.06788479128838,103.4210712814));
#57334=CARTESIAN_POINT('Ctrl Pts',(5.94821946573796,-5.21561177499016,103.413188152607));
#57335=CARTESIAN_POINT('Ctrl Pts',(5.81867912915963,-5.3633479150396,103.405304535206));
#57336=CARTESIAN_POINT('Ctrl Pts',(5.68363907950052,-5.50624649161836,103.397420917804));
#57337=CARTESIAN_POINT('Ctrl Pts',(5.54350530979244,-5.64388783378116,103.389537300403));
#57338=CARTESIAN_POINT('Ctrl Pts',(5.40333929863348,-5.78156084394648,103.381651869169));
#57339=CARTESIAN_POINT('Ctrl Pts',(5.25807747823787,-5.91397396772881,103.373766437934));
#57340=CARTESIAN_POINT('Ctrl Pts',(5.10816146609277,-6.04074560268225,103.3658810067));
#57341=CARTESIAN_POINT('Ctrl Pts',(4.95818576142647,-6.16756771468882,103.357992435699));
#57342=CARTESIAN_POINT('Ctrl Pts',(4.80355243556228,-6.28874363938329,103.350103864698));
#57343=CARTESIAN_POINT('Ctrl Pts',(4.6447350040477,-6.4039329901377,103.342215293697));
#57344=CARTESIAN_POINT('Ctrl Pts',(4.48574852061556,-6.51924495325552,103.334318325771));
#57345=CARTESIAN_POINT('Ctrl Pts',(4.32256931490728,-6.62855741168161,103.326421357845));
#57346=CARTESIAN_POINT('Ctrl Pts',(4.15569954535654,-6.73157353734797,103.31852438992));
#57347=CARTESIAN_POINT('Ctrl Pts',(3.98872798590351,-6.8346525024453,103.310622604874));
#57348=CARTESIAN_POINT('Ctrl Pts',(3.81806167368665,-6.93142730806685,103.302720819829));
#57349=CARTESIAN_POINT('Ctrl Pts',(3.64422624461561,-7.02164767544305,103.294819034784));
#57350=CARTESIAN_POINT('Ctrl Pts',(3.47016595323962,-7.11198474607054,103.286907028499));
#57351=CARTESIAN_POINT('Ctrl Pts',(3.29292866776747,-7.19575029677638,103.278995022214));
#57352=CARTESIAN_POINT('Ctrl Pts',(3.11305985701368,-7.27274221505547,103.271083015929));
#57353=CARTESIAN_POINT('Ctrl Pts',(3.03769675257106,-7.30500100385931,103.267767970072));
#57354=CARTESIAN_POINT('Ctrl Pts',(2.96187186449698,-7.33607126962668,103.264452924214));
#57355=CARTESIAN_POINT('Ctrl Pts',(2.88562602738774,-7.36594077019782,103.261137878356));
#57356=CARTESIAN_POINT('Ctrl Pts',(2.70529867907432,-7.43658446744941,103.253297536487));
#57357=CARTESIAN_POINT('Ctrl Pts',(2.52210438325268,-7.50070846118149,103.245457194618));
#57358=CARTESIAN_POINT('Ctrl Pts',(2.33656004971482,-7.55806907444466,103.237616852749));
#57359=CARTESIAN_POINT('Ctrl Pts',(2.15122316026426,-7.61536555683495,103.229785276615));
#57360=CARTESIAN_POINT('Ctrl Pts',(1.96354179724364,-7.66591361294437,103.221953700481));
#57361=CARTESIAN_POINT('Ctrl Pts',(1.77405393949023,-7.70951708084101,103.214122124348));
#57362=CARTESIAN_POINT('Ctrl Pts',(1.58474109016318,-7.75308027716356,103.206297781352));
#57363=CARTESIAN_POINT('Ctrl Pts',(1.39362540894185,-7.7897115801307,103.198473438356));
#57364=CARTESIAN_POINT('Ctrl Pts',(1.20126136194246,-7.81926416872484,103.190649095361));
#57365=CARTESIAN_POINT('Ctrl Pts',(1.00903759555761,-7.84879520622691,103.182830458232));
#57366=CARTESIAN_POINT('Ctrl Pts',(0.815567622522301,-7.8712577577781,103.175011821103));
#57367=CARTESIAN_POINT('Ctrl Pts',(0.621417658063136,-7.88655571807157,
103.167193183974));
#57368=CARTESIAN_POINT('Ctrl Pts',(0.427371558820727,-7.90184549435137,
103.159378729614));
#57369=CARTESIAN_POINT('Ctrl Pts',(0.232646542418804,-7.90997828705685,
103.151564275255));
#57370=CARTESIAN_POINT('Ctrl Pts',(0.0378157234129442,-7.91090961717189,
103.143749820895));
#57371=CARTESIAN_POINT('Ctrl Pts',(-0.156948707055732,-7.91184062993651,
103.135938029307));
#57372=CARTESIAN_POINT('Ctrl Pts',(-0.351818517124127,-7.90557506772958,
103.12812623772));
#57373=CARTESIAN_POINT('Ctrl Pts',(-0.54621860849317,-7.89212051553547,
103.120314446133));
#57374=CARTESIAN_POINT('Ctrl Pts',(-0.740627798100354,-7.87866533364658,
103.112502288942));
#57375=CARTESIAN_POINT('Ctrl Pts',(-0.934566873670922,-7.85802050473307,
103.10469013175));
#57376=CARTESIAN_POINT('Ctrl Pts',(-1.12746335672154,-7.8302456780902,103.096877974558));
#57377=CARTESIAN_POINT('Ctrl Pts',(-1.32037560923414,-7.80246858083012,
103.089065178716));
#57378=CARTESIAN_POINT('Ctrl Pts',(-1.51224475103333,-7.76756037405695,
103.081252382873));
#57379=CARTESIAN_POINT('Ctrl Pts',(-1.70250611220949,-7.72563226783992,
103.073439587031));
#57380=CARTESIAN_POINT('Ctrl Pts',(-1.89281650554473,-7.68369335635186,
103.065624777757));
#57381=CARTESIAN_POINT('Ctrl Pts',(-2.08151794931597,-7.6347310171212,103.057809968482));
#57382=CARTESIAN_POINT('Ctrl Pts',(-2.2680584546872,-7.57890703506264,103.049995159208));
#57383=CARTESIAN_POINT('Ctrl Pts',(-2.45467985952475,-7.52305884308598,
103.042176960783));
#57384=CARTESIAN_POINT('Ctrl Pts',(-2.63913812246811,-7.46034318111028,
103.034358762358));
#57385=CARTESIAN_POINT('Ctrl Pts',(-2.8208986876382,-7.39097095069931,103.026540563933));
#57386=CARTESIAN_POINT('Ctrl Pts',(-3.00287082112093,-7.32151797138817,
103.018713265168));
#57387=CARTESIAN_POINT('Ctrl Pts',(-3.18213865655702,-7.24539307377926,
103.010885966402));
#57388=CARTESIAN_POINT('Ctrl Pts',(-3.35818881071883,-7.16285480179257,
103.003058667637));
#57389=CARTESIAN_POINT('Ctrl Pts',(-3.53435389113834,-7.08026264848574,
102.995226259179));
#57390=CARTESIAN_POINT('Ctrl Pts',(-3.70729679275847,-6.99124893784943,
102.98739385072));
#57391=CARTESIAN_POINT('Ctrl Pts',(-3.87653077669679,-6.89611703332553,
102.979561442262));
#57392=CARTESIAN_POINT('Ctrl Pts',(-4.04600763524994,-6.80084860111298,
102.971717793194));
#57393=CARTESIAN_POINT('Ctrl Pts',(-4.21176464617896,-6.69944462072016,
102.963874144127));
#57394=CARTESIAN_POINT('Ctrl Pts',(-4.37334499653641,-6.59225109816593,
102.956030495059));
#57395=CARTESIAN_POINT('Ctrl Pts',(-4.46052315823942,-6.5344165024241,102.951798576355));
#57396=CARTESIAN_POINT('Ctrl Pts',(-4.54648608082056,-6.47489727741504,
102.947566657652));
#57397=CARTESIAN_POINT('Ctrl Pts',(-4.63116629696624,-6.41375239074943,
102.943334738948));
#57398=CARTESIAN_POINT('Ctrl Pts',(-4.78851743264026,-6.30013414796009,
102.935471069671));
#57399=CARTESIAN_POINT('Ctrl Pts',(-4.94192080499853,-6.1805515432417,102.927607400395));
#57400=CARTESIAN_POINT('Ctrl Pts',(-5.09088992028185,-6.05530848261033,
102.919743731118));
#57401=CARTESIAN_POINT('Ctrl Pts',(-5.23968758544185,-5.93020956553617,
102.911889112221));
#57402=CARTESIAN_POINT('Ctrl Pts',(-5.38406089155956,-5.79946338873537,
102.904034493323));
#57403=CARTESIAN_POINT('Ctrl Pts',(-5.52355189827762,-5.66341729232747,
102.896179874426));
#57404=CARTESIAN_POINT('Ctrl Pts',(-5.6629091908213,-5.52750160784995,102.88833278486));
#57405=CARTESIAN_POINT('Ctrl Pts',(-5.79739325653309,-5.38629636478731,
102.880485695293));
#57406=CARTESIAN_POINT('Ctrl Pts',(-5.92657870535733,-5.24018948600192,
102.872638605726));
#57407=CARTESIAN_POINT('Ctrl Pts',(-6.05566515247872,-5.09419457671409,
102.864797529803));
#57408=CARTESIAN_POINT('Ctrl Pts',(-6.1794608405758,-4.94330577508444,102.85695645388));
#57409=CARTESIAN_POINT('Ctrl Pts',(-6.29757663468409,-4.78794836336829,
102.849115377957));
#57410=CARTESIAN_POINT('Ctrl Pts',(-6.4156246087182,-4.63268015522787,102.841278804245));
#57411=CARTESIAN_POINT('Ctrl Pts',(-6.52799897499263,-4.47294872652082,
102.833442230534));
#57412=CARTESIAN_POINT('Ctrl Pts',(-6.63435023162384,-4.30921315371526,
102.825605656823));
#57413=CARTESIAN_POINT('Ctrl Pts',(-6.74066952816474,-4.14552678581674,
102.817771438115));
#57414=CARTESIAN_POINT('Ctrl Pts',(-6.84096912777522,-3.977838962193,102.809937219408));
#57415=CARTESIAN_POINT('Ctrl Pts',(-6.9349421079913,-3.80663880067564,102.802103000701));
#57416=CARTESIAN_POINT('Ctrl Pts',(-7.02890201322643,-3.63546245918447,
102.794269872011));
#57417=CARTESIAN_POINT('Ctrl Pts',(-7.1165368833799,-3.46077505951376,102.786436743322));
#57418=CARTESIAN_POINT('Ctrl Pts',(-7.19758505811575,-3.28309158129787,
102.778603614633));
#57419=CARTESIAN_POINT('Ctrl Pts',(-7.27863606234484,-3.10540189992932,
102.770770212479));
#57420=CARTESIAN_POINT('Ctrl Pts',(-7.35309976778337,-2.92471625007048,
102.762936810326));
#57421=CARTESIAN_POINT('Ctrl Pts',(-7.42076202748746,-2.74157106991597,
102.755103408172));
#57422=CARTESIAN_POINT('Ctrl Pts',(-7.48843842601733,-2.55838761941986,
102.747268369137));
#57423=CARTESIAN_POINT('Ctrl Pts',(-7.54931042678635,-2.37274394318788,
102.739433330102));
#57424=CARTESIAN_POINT('Ctrl Pts',(-7.60321320776555,-2.18519333635709,
102.731598291066));
#57425=CARTESIAN_POINT('Ctrl Pts',(-7.65716262412294,-1.9974804652921,102.723756473346));
#57426=CARTESIAN_POINT('Ctrl Pts',(-7.70413067826067,-1.80785770437767,
102.715914655625));
#57427=CARTESIAN_POINT('Ctrl Pts',(-7.74400307466978,-1.61689127015547,
102.708072837904));
#57428=CARTESIAN_POINT('Ctrl Pts',(-7.78389362392783,-1.42583789395975,
102.700227450011));
#57429=CARTESIAN_POINT('Ctrl Pts',(-7.81668201633006,-1.23343996951669,
102.692382062117));
#57430=CARTESIAN_POINT('Ctrl Pts',(-7.84230563603277,-1.04027078736673,
102.684536674224));
#57431=CARTESIAN_POINT('Ctrl Pts',(-7.86796117739653,-0.84686095689197,
102.676681512621));
#57432=CARTESIAN_POINT('Ctrl Pts',(-7.88643407801548,-0.652678297003844,
102.668826351018));
#57433=CARTESIAN_POINT('Ctrl Pts',(-7.89771376744866,-0.45829929898697,
102.660971189416));
#57434=CARTESIAN_POINT('Ctrl Pts',(-7.90659393108899,-0.305270501442419,
102.654787054572));
#57435=CARTESIAN_POINT('Ctrl Pts',(-7.91101682177921,-0.152120092814248,
102.648602919728));
#57436=CARTESIAN_POINT('Ctrl Pts',(-7.91099995190663,0.000872314928047417,
102.642418784884));
#57437=CARTESIAN_POINT('',(-7.91099999491492,-0.00028364795766521,98.635032539653));
#57438=CARTESIAN_POINT('Ctrl Pts',(-7.91099993013027,0.00105141757446709,
102.647258864909));
#57439=CARTESIAN_POINT('Ctrl Pts',(-7.91097619318975,0.179651185499931,
102.640642093266));
#57440=CARTESIAN_POINT('Ctrl Pts',(-7.90490459988792,0.35819593563781,102.63379939406));
#57441=CARTESIAN_POINT('Ctrl Pts',(-7.89220454811321,0.545072556459039,
102.626295665916));
#57442=CARTESIAN_POINT('Ctrl Pts',(-7.89160021739073,0.553753310620412,
102.625946399728));
#57443=CARTESIAN_POINT('Ctrl Pts',(-7.89058727690093,0.567964948982951,
102.625373465286));
#57444=CARTESIAN_POINT('Ctrl Pts',(-7.89018717026809,0.573496447735965,
102.625150184159));
#57445=CARTESIAN_POINT('Ctrl Pts',(-7.88946979434076,0.583271353134799,
102.624755123277));
#57446=CARTESIAN_POINT('Ctrl Pts',(-7.88915491705159,0.587514937562228,
102.624583451073));
#57447=CARTESIAN_POINT('Ctrl Pts',(-7.88852861687332,0.595864258755811,
102.624245362585));
#57448=CARTESIAN_POINT('Ctrl Pts',(-7.88821741205822,0.599970011002315,
102.624078956052));
#57449=CARTESIAN_POINT('Ctrl Pts',(-7.88759128868958,0.608145810706466,
102.623747288526));
#57450=CARTESIAN_POINT('Ctrl Pts',(-7.88727642496625,0.612215861096921,
102.62358203));
#57451=CARTESIAN_POINT('Ctrl Pts',(-7.8865235349574,0.62185102311047,102.623190458366));
#57452=CARTESIAN_POINT('Ctrl Pts',(-7.88608276864437,0.627415913274009,
102.622964025717));
#57453=CARTESIAN_POINT('Ctrl Pts',(-7.88451967146883,0.646888897059917,
102.622170722648));
#57454=CARTESIAN_POINT('Ctrl Pts',(-7.88336643893215,0.660794431650021,
102.621602521431));
#57455=CARTESIAN_POINT('Ctrl Pts',(-7.8684776900109,0.83473293188157,102.614474309575));
#57456=CARTESIAN_POINT('Ctrl Pts',(-7.84990870092257,0.994308438496762,
102.607714747561));
#57457=CARTESIAN_POINT('Ctrl Pts',(-7.8237344739426,1.17194663699994,102.600015381335));
#57458=CARTESIAN_POINT('Ctrl Pts',(-7.82090501308979,1.19068249731943,102.599201120564));
#57459=CARTESIAN_POINT('Ctrl Pts',(-7.8137411971457,1.23699174550653,102.59718333632));
#57460=CARTESIAN_POINT('Ctrl Pts',(-7.80932818433038,1.26455263536201,102.595977904239));
#57461=CARTESIAN_POINT('Ctrl Pts',(-7.72050994056059,1.80105257813195,102.572430226951));
#57462=CARTESIAN_POINT('Ctrl Pts',(-7.58666811392793,2.30055422518567,102.549156478115));
#57463=CARTESIAN_POINT('Ctrl Pts',(-7.25202901720152,3.19082707971832,102.507563032799));
#57464=CARTESIAN_POINT('Ctrl Pts',(-7.0655526334846,3.58487391081999,102.489092294102));
#57465=CARTESIAN_POINT('Ctrl Pts',(-6.82481117722698,4.00099283638436,102.469552829782));
#57466=CARTESIAN_POINT('Ctrl Pts',(-6.80168635647896,4.04017995262355,102.467711734066));
#57467=CARTESIAN_POINT('Ctrl Pts',(-6.77028616356006,4.0923566908158,102.465258438393));
#57468=CARTESIAN_POINT('Ctrl Pts',(-6.76230924216551,4.10552453858889,102.464639134205));
#57469=CARTESIAN_POINT('Ctrl Pts',(-6.74906508852445,4.12724391086071,102.463617333667));
#57470=CARTESIAN_POINT('Ctrl Pts',(-6.74381993105232,4.13580882138465,102.46321431375));
#57471=CARTESIAN_POINT('Ctrl Pts',(-6.73358078677488,4.15245723277549,102.46243076269));
#57472=CARTESIAN_POINT('Ctrl Pts',(-6.72858851708777,4.16054177365766,102.462050191014));
#57473=CARTESIAN_POINT('Ctrl Pts',(-6.71701562020045,4.1792077513163,102.46117133034));
#57474=CARTESIAN_POINT('Ctrl Pts',(-6.7104245272021,4.18978268369556,102.460673292121));
#57475=CARTESIAN_POINT('Ctrl Pts',(-6.692657991791,4.21813833899796,102.459337486896));
#57476=CARTESIAN_POINT('Ctrl Pts',(-6.68143666386314,4.23589024344511,102.458500827832));
#57477=CARTESIAN_POINT('Ctrl Pts',(-6.60053914302513,4.3627471445224,102.452519097253));
#57478=CARTESIAN_POINT('Ctrl Pts',(-6.5282636383704,4.47017391349305,102.447438707664));
#57479=CARTESIAN_POINT('Ctrl Pts',(-6.08991358756491,5.088394238714,102.41807289235));
#57480=CARTESIAN_POINT('Ctrl Pts',(-5.66667411316083,5.55586456609055,102.395571857204));
#57481=CARTESIAN_POINT('Ctrl Pts',(-5.09935993276306,6.04943927067375,102.368313011645));
#57482=CARTESIAN_POINT('Ctrl Pts',(-5.00425814755397,6.12834292841191,102.363818351838));
#57483=CARTESIAN_POINT('Ctrl Pts',(-4.78876014827182,6.2987742180952,102.353725830385));
#57484=CARTESIAN_POINT('Ctrl Pts',(-4.66751010816992,6.38914138732312,102.348108337351));
#57485=CARTESIAN_POINT('Ctrl Pts',(-4.45298562732648,6.53965849992211,102.338161081202));
#57486=CARTESIAN_POINT('Ctrl Pts',(-4.36089638846656,6.60142376053902,102.33388830735));
#57487=CARTESIAN_POINT('Ctrl Pts',(-4.23797158991794,6.68017597935315,102.328145428691));
#57488=CARTESIAN_POINT('Ctrl Pts',(-4.20827550925301,6.69892315965258,102.326755098169));
#57489=CARTESIAN_POINT('Ctrl Pts',(-4.16564985920987,6.72543750977358,102.32475392299));
#57490=CARTESIAN_POINT('Ctrl Pts',(-4.15282112479293,6.73336655385158,102.324150936989));
#57491=CARTESIAN_POINT('Ctrl Pts',(-4.13015268970366,6.74728778731678,102.323084088224));
#57492=CARTESIAN_POINT('Ctrl Pts',(-4.12032240085698,6.75329527239323,102.322620991194));
#57493=CARTESIAN_POINT('Ctrl Pts',(-4.10572529558253,6.76217211794273,102.32193261631));
#57494=CARTESIAN_POINT('Ctrl Pts',(-4.10096848982942,6.76505797467126,102.321708180755));
#57495=CARTESIAN_POINT('Ctrl Pts',(-4.09265419191567,6.77009009745385,102.321315692805));
#57496=CARTESIAN_POINT('Ctrl Pts',(-4.08909804193423,6.77223858599228,102.321147755104));
#57497=CARTESIAN_POINT('Ctrl Pts',(-4.08202162619004,6.77650627732625,102.320813442693));
#57498=CARTESIAN_POINT('Ctrl Pts',(-4.07850139817033,6.77862554124064,102.320647071217));
#57499=CARTESIAN_POINT('Ctrl Pts',(-4.07010628986744,6.78367069620361,102.320250147693));
#57500=CARTESIAN_POINT('Ctrl Pts',(-4.06522990835805,6.78659407341233,102.320019464226));
#57501=CARTESIAN_POINT('Ctrl Pts',(-4.05052996952463,6.79538511770749,102.31932367235));
#57502=CARTESIAN_POINT('Ctrl Pts',(-4.040696859153,6.80123671270748,102.318857714628));
#57503=CARTESIAN_POINT('Ctrl Pts',(-3.92850446450238,6.86767220470696,102.313534939814));
#57504=CARTESIAN_POINT('Ctrl Pts',(-3.82481786982913,6.92595355047103,102.308545762944));
#57505=CARTESIAN_POINT('Ctrl Pts',(-3.69979027117438,6.99256677234025,102.302463787982));
#57506=CARTESIAN_POINT('Ctrl Pts',(-3.67967499574954,7.00317285422648,102.301483453866));
#57507=CARTESIAN_POINT('Ctrl Pts',(-3.40709862087158,7.14539426618797,102.288177417609));
#57508=CARTESIAN_POINT('Ctrl Pts',(-3.14776965808816,7.26336761434618,102.275272202322));
#57509=CARTESIAN_POINT('Ctrl Pts',(-2.85431605766383,7.37819269488221,102.260813395882));
#57510=CARTESIAN_POINT('Ctrl Pts',(-2.82590506180737,7.38912093370939,102.259414933542));
#57511=CARTESIAN_POINT('Ctrl Pts',(-2.76582490602053,7.4118334675935,102.256461367515));
#57512=CARTESIAN_POINT('Ctrl Pts',(-2.73414186751939,7.42357939289169,102.254905991946));
#57513=CARTESIAN_POINT('Ctrl Pts',(-2.66677082559187,7.44806620935744,102.25160432986));
#57514=CARTESIAN_POINT('Ctrl Pts',(-2.6310645324822,7.46075440662486,102.249857838216));
#57515=CARTESIAN_POINT('Ctrl Pts',(-2.5547493702244,7.48725693817743,102.246133708878));
#57516=CARTESIAN_POINT('Ctrl Pts',(-2.5141164657259,7.50099854696139,102.244156038204));
#57517=CARTESIAN_POINT('Ctrl Pts',(-2.42674948512295,7.52975545933348,102.239916883274));
#57518=CARTESIAN_POINT('Ctrl Pts',(-2.37998325470231,7.54466765775602,102.237655732956));
#57519=CARTESIAN_POINT('Ctrl Pts',(-2.27861747871593,7.57595355408697,102.232774824085));
#57520=CARTESIAN_POINT('Ctrl Pts',(-2.22397346184015,7.5921743896793,102.230156165179));
#57521=CARTESIAN_POINT('Ctrl Pts',(-1.96450378655201,7.66615512754583,102.217789977196));
#57522=CARTESIAN_POINT('Ctrl Pts',(-1.75757164823691,7.71622688304804,102.208130903311));
#57523=CARTESIAN_POINT('Ctrl Pts',(-1.37393010219411,7.79282101426147,102.190729656883));
#57524=CARTESIAN_POINT('Ctrl Pts',(-1.19785723343373,7.82182116270348,102.182934513702));
#57525=CARTESIAN_POINT('Ctrl Pts',(-0.886246271514019,7.86237497129892,
102.169511000969));
#57526=CARTESIAN_POINT('Ctrl Pts',(-0.751112268389215,7.87643354791872,
102.163811234974));
#57527=CARTESIAN_POINT('Ctrl Pts',(-0.546083352752086,7.89243859485094,
102.155348575693));
#57528=CARTESIAN_POINT('Ctrl Pts',(-0.476418213367624,7.8969500454934,102.152505228884));
#57529=CARTESIAN_POINT('Ctrl Pts',(-0.393549480976554,7.90121593385416,
102.14916043382));
#57530=CARTESIAN_POINT('Ctrl Pts',(-0.380396001030403,7.90186011721237,
102.148630644501));
#57531=CARTESIAN_POINT('Ctrl Pts',(-0.360140564698243,7.90280142087243,
102.147816519767));
#57532=CARTESIAN_POINT('Ctrl Pts',(-0.353039744358613,7.90312181756908,
102.147531441379));
#57533=CARTESIAN_POINT('Ctrl Pts',(-0.340094389964134,7.90368844431816,
102.147012310148));
#57534=CARTESIAN_POINT('Ctrl Pts',(-0.334250000218825,7.90393776269027,
102.146778158805));
#57535=CARTESIAN_POINT('Ctrl Pts',(-0.321512568785072,7.90446698141622,
102.146268318279));
#57536=CARTESIAN_POINT('Ctrl Pts',(-0.314619423483892,7.90474434822975,
102.145992710243));
#57537=CARTESIAN_POINT('Ctrl Pts',(-0.29584696728772,7.90547512140316,102.145242956579));
#57538=CARTESIAN_POINT('Ctrl Pts',(-0.283966961026479,7.90591076915511,
102.144769378979));
#57539=CARTESIAN_POINT('Ctrl Pts',(-0.227272508236372,7.90786183699207,
102.142513604787));
#57540=CARTESIAN_POINT('Ctrl Pts',(-0.182446272295308,7.90902301612059,
102.140742753471));
#57541=CARTESIAN_POINT('Ctrl Pts',(-0.121808602386883,7.91007796993064,
102.138363987727));
#57542=CARTESIAN_POINT('Ctrl Pts',(-0.106004262811609,7.91030555199766,
102.137745530848));
#57543=CARTESIAN_POINT('Ctrl Pts',(0.780549246606244,7.92041447550463,102.103137906176));
#57544=CARTESIAN_POINT('Ctrl Pts',(1.64684287660674,7.78652997427673,102.074813652592));
#57545=CARTESIAN_POINT('Ctrl Pts',(2.70480258652009,7.43821515039594,102.036384232167));
#57546=CARTESIAN_POINT('Ctrl Pts',(2.9320407002333,7.35160715009197,102.027822986929));
#57547=CARTESIAN_POINT('Ctrl Pts',(3.24886335761303,7.2138271732473,102.015009688091));
#57548=CARTESIAN_POINT('Ctrl Pts',(3.34200202500479,7.17115309131828,102.011130737214));
#57549=CARTESIAN_POINT('Ctrl Pts',(3.47339244222461,7.1078372748321,102.00546346647));
#57550=CARTESIAN_POINT('Ctrl Pts',(3.51234587938199,7.08866927409591,102.00375842055));
#57551=CARTESIAN_POINT('Ctrl Pts',(3.57340584622635,7.05799635822397,102.001043547455));
#57552=CARTESIAN_POINT('Ctrl Pts',(3.59561958174149,7.04670573611469,102.000047002708));
#57553=CARTESIAN_POINT('Ctrl Pts',(3.6233820451247,7.03242939855693,101.998789958992));
#57554=CARTESIAN_POINT('Ctrl Pts',(3.628981265905,7.02954163952994,101.998535842494));
#57555=CARTESIAN_POINT('Ctrl Pts',(3.63733304208231,7.02522163130205,101.998155910825));
#57556=CARTESIAN_POINT('Ctrl Pts',(3.64008822588083,7.02379444002228,101.998030429279));
#57557=CARTESIAN_POINT('Ctrl Pts',(3.64544570798496,7.02101525350872,101.997786145462));
#57558=CARTESIAN_POINT('Ctrl Pts',(3.64804809448055,7.01966343211415,101.997667354707));
#57559=CARTESIAN_POINT('Ctrl Pts',(3.65349119151277,7.01683214649027,101.997418622664));
#57560=CARTESIAN_POINT('Ctrl Pts',(3.65633175710737,7.01535240315055,101.997288662939));
#57561=CARTESIAN_POINT('Ctrl Pts',(3.66419317609988,7.01125106168745,101.996928564923));
#57562=CARTESIAN_POINT('Ctrl Pts',(3.66921210523156,7.00862580027559,101.996698186207));
#57563=CARTESIAN_POINT('Ctrl Pts',(3.68893526399893,6.99828217535659,101.995790968387));
#57564=CARTESIAN_POINT('Ctrl Pts',(3.70361790033703,6.9905229581518,101.995111476691));
#57565=CARTESIAN_POINT('Ctrl Pts',(3.95239237194866,6.85805130878709,101.983529949603));
#57566=CARTESIAN_POINT('Ctrl Pts',(4.18007288285763,6.72169922156217,101.97190165355));
#57567=CARTESIAN_POINT('Ctrl Pts',(4.40388284763992,6.57189119476423,101.959749236539));
#57568=CARTESIAN_POINT('Ctrl Pts',(4.40730859039656,6.56959427974921,101.959563047092));
#57569=CARTESIAN_POINT('Ctrl Pts',(4.41411424894203,6.56502345706303,101.959192805852));
#57570=CARTESIAN_POINT('Ctrl Pts',(4.41749420790928,6.56274961561038,101.959008756072));
#57571=CARTESIAN_POINT('Ctrl Pts',(4.79175050178151,6.31055144771266,101.938610192457));
#57572=CARTESIAN_POINT('Ctrl Pts',(5.14076639969692,6.02963193599232,101.917568020216));
#57573=CARTESIAN_POINT('Ctrl Pts',(5.51183238703923,5.67520638298301,101.894082991572));
#57574=CARTESIAN_POINT('Ctrl Pts',(5.55891651236179,5.6290950538082,101.891078956005));
#57575=CARTESIAN_POINT('Ctrl Pts',(5.66148119870899,5.52610744111659,101.884486686933));
#57576=CARTESIAN_POINT('Ctrl Pts',(5.71669252692006,5.46897245571656,101.880905688421));
#57577=CARTESIAN_POINT('Ctrl Pts',(5.85214545315515,5.32450721670695,101.872046766253));
#57578=CARTESIAN_POINT('Ctrl Pts',(5.93130275489698,5.23618492350482,101.866803188947));
#57579=CARTESIAN_POINT('Ctrl Pts',(6.13589716174251,4.9973067057493,101.853089797723));
#57580=CARTESIAN_POINT('Ctrl Pts',(6.25778080825266,4.84380996680798,101.844752450794));
#57581=CARTESIAN_POINT('Ctrl Pts',(6.4263270822239,4.6145521406595,101.832980815322));
#57582=CARTESIAN_POINT('Ctrl Pts',(6.47760668544398,4.54228836010891,101.829363063229));
#57583=CARTESIAN_POINT('Ctrl Pts',(6.53555274278236,4.45765256665546,101.825230429409));
#57584=CARTESIAN_POINT('Ctrl Pts',(6.54341227073,4.4461075016959,101.82466891598));
#57585=CARTESIAN_POINT('Ctrl Pts',(6.55530086618688,4.42854423073005,101.82381804049));
#57586=CARTESIAN_POINT('Ctrl Pts',(6.55935229071512,4.42254123512997,101.823527808502));
#57587=CARTESIAN_POINT('Ctrl Pts',(6.56664086477851,4.41170970787824,101.82300518936));
#57588=CARTESIAN_POINT('Ctrl Pts',(6.56988094365253,4.40688315933032,101.82277268853));
#57589=CARTESIAN_POINT('Ctrl Pts',(6.57636132243499,4.39720670173508,101.822307319365));
#57590=CARTESIAN_POINT('Ctrl Pts',(6.57960158453984,4.39235677170207,101.822074452563));
#57591=CARTESIAN_POINT('Ctrl Pts',(6.5886536739918,4.37877537443949,101.821423411064));
#57592=CARTESIAN_POINT('Ctrl Pts',(6.59445351452491,4.37003591077846,101.82100570022));
#57593=CARTESIAN_POINT('Ctrl Pts',(6.61784793439725,4.33463150713187,101.819318451357));
#57594=CARTESIAN_POINT('Ctrl Pts',(6.63529841675315,4.30787146249326,101.818054470776));
#57595=CARTESIAN_POINT('Ctrl Pts',(6.9018825556959,3.89360576545395,101.798658665059));
#57596=CARTESIAN_POINT('Ctrl Pts',(7.11687693210921,3.48515009148752,101.781917112215));
#57597=CARTESIAN_POINT('Ctrl Pts',(7.39140709839853,2.83072231598911,101.757159938033));
#57598=CARTESIAN_POINT('Ctrl Pts',(7.47681553189919,2.59675166362009,101.748668432677));
#57599=CARTESIAN_POINT('Ctrl Pts',(7.6241720772216,2.12509873357997,101.731752705972));
#57600=CARTESIAN_POINT('Ctrl Pts',(7.68637097421647,1.88778699413457,101.723337552833));
#57601=CARTESIAN_POINT('Ctrl Pts',(7.77858415927764,1.45483523743107,101.70762076493));
#57602=CARTESIAN_POINT('Ctrl Pts',(7.81247274905533,1.26022969233395,101.7004253305));
#57603=CARTESIAN_POINT('Ctrl Pts',(7.84827264998825,0.996614599443258,101.690270189082));
#57604=CARTESIAN_POINT('Ctrl Pts',(7.85661709764574,0.928542706448378,101.687611437046));
#57605=CARTESIAN_POINT('Ctrl Pts',(7.86659422609799,0.837348633381466,101.683990888177));
#57606=CARTESIAN_POINT('Ctrl Pts',(7.86901203324911,0.814313853528825,101.683071372994));
#57607=CARTESIAN_POINT('Ctrl Pts',(7.8723634172595,0.780975198023991,101.6817328954));
#57608=CARTESIAN_POINT('Ctrl Pts',(7.87337800910295,0.77067941273266,101.681318486895));
#57609=CARTESIAN_POINT('Ctrl Pts',(7.87514927217471,0.752336539923534,101.680578257216));
#57610=CARTESIAN_POINT('Ctrl Pts',(7.87591381589302,0.744290193865863,101.68025288648));
#57611=CARTESIAN_POINT('Ctrl Pts',(7.8770482494476,0.732153497230544,101.679761102085));
#57612=CARTESIAN_POINT('Ctrl Pts',(7.87742728719592,0.728064009855788,101.67959522142));
#57613=CARTESIAN_POINT('Ctrl Pts',(7.87808178660637,0.720942185282276,101.679306042363));
#57614=CARTESIAN_POINT('Ctrl Pts',(7.87835868284953,0.717909977158523,101.679182826431));
#57615=CARTESIAN_POINT('Ctrl Pts',(7.87892659818121,0.71165100798842,101.678928295369));
#57616=CARTESIAN_POINT('Ctrl Pts',(7.87921738567086,0.708424227411561,101.678796967058));
#57617=CARTESIAN_POINT('Ctrl Pts',(7.8799146940792,0.700632867281794,101.678479608142));
#57618=CARTESIAN_POINT('Ctrl Pts',(7.88031923073747,0.696068116048889,101.678293465046));
#57619=CARTESIAN_POINT('Ctrl Pts',(7.88155504074823,0.68198419729996,101.677718500795));
#57620=CARTESIAN_POINT('Ctrl Pts',(7.88237303123551,0.67246390287261,101.677328933718));
#57621=CARTESIAN_POINT('Ctrl Pts',(7.89169490534443,0.561615695186437,101.672782676084));
#57622=CARTESIAN_POINT('Ctrl Pts',(7.89826131812768,0.460138225407757,101.668519764074));
#57623=CARTESIAN_POINT('Ctrl Pts',(7.90326108228446,0.349942555656956,101.663802430475));
#57624=CARTESIAN_POINT('Ctrl Pts',(7.90363825123258,0.341317916025791,101.663432634978));
#57625=CARTESIAN_POINT('Ctrl Pts',(7.90471838697994,0.315656414240807,101.662330648095));
#57626=CARTESIAN_POINT('Ctrl Pts',(7.9053803869428,0.298617950679037,101.661596722377));
#57627=CARTESIAN_POINT('Ctrl Pts',(7.90665661102096,0.26278480148346,101.660048701701));
#57628=CARTESIAN_POINT('Ctrl Pts',(7.90725891690065,0.243989812291861,101.659234128818));
#57629=CARTESIAN_POINT('Ctrl Pts',(7.91088304914098,0.116726109894249,101.653701641022));
#57630=CARTESIAN_POINT('Ctrl Pts',(7.91173980970498,0.00821021824212436,
101.648901223505));
#57631=CARTESIAN_POINT('Ctrl Pts',(7.90165874434802,-0.786968130354667,
101.613278636282));
#57632=CARTESIAN_POINT('Ctrl Pts',(7.80358378605594,-1.46961676903034,101.580577598229));
#57633=CARTESIAN_POINT('Ctrl Pts',(7.53619871956156,-2.42551030567191,101.536792535712));
#57634=CARTESIAN_POINT('Ctrl Pts',(7.43683791213763,-2.71493282556897,101.523765462613));
#57635=CARTESIAN_POINT('Ctrl Pts',(7.30409212781048,-3.03910207651414,101.509475340094));
#57636=CARTESIAN_POINT('Ctrl Pts',(7.28687252749589,-3.08016105018375,101.50767074036));
#57637=CARTESIAN_POINT('Ctrl Pts',(7.26470581916521,-3.13178964499847,101.505408091542));
#57638=CARTESIAN_POINT('Ctrl Pts',(7.26008089185093,-3.14249621556035,101.504939225055));
#57639=CARTESIAN_POINT('Ctrl Pts',(7.2526779895193,-3.15953014412524,101.504193824657));
#57640=CARTESIAN_POINT('Ctrl Pts',(7.24991537968331,-3.16586413780434,101.503916773446));
#57641=CARTESIAN_POINT('Ctrl Pts',(7.24469371815047,-3.17779346160022,101.503395209691));
#57642=CARTESIAN_POINT('Ctrl Pts',(7.24223647548086,-3.18338957525258,101.503150636385));
#57643=CARTESIAN_POINT('Ctrl Pts',(7.23669536265386,-3.19596925962113,101.502601064543));
#57644=CARTESIAN_POINT('Ctrl Pts',(7.23360786197535,-3.20295122970732,101.502296188862));
#57645=CARTESIAN_POINT('Ctrl Pts',(7.22572640056235,-3.22070457949131,101.501521339586));
#57646=CARTESIAN_POINT('Ctrl Pts',(7.22091845067828,-3.23146974832196,101.501051839164));
#57647=CARTESIAN_POINT('Ctrl Pts',(7.19413993619844,-3.29106959884842,101.49845440975));
#57648=CARTESIAN_POINT('Ctrl Pts',(7.17169779408785,-3.3396915151882,101.496342482017));
#57649=CARTESIAN_POINT('Ctrl Pts',(6.79524496636827,-4.13399692486191,101.461945981394));
#57650=CARTESIAN_POINT('Ctrl Pts',(6.32722201323277,-4.8199049684268,101.434487131371));
#57651=CARTESIAN_POINT('Ctrl Pts',(5.61066582405834,-5.58147543859712,101.397711741201));
#57652=CARTESIAN_POINT('Ctrl Pts',(5.45309762544546,-5.73551717662546,101.389823643687));
#57653=CARTESIAN_POINT('Ctrl Pts',(5.1838218846574,-5.97762806844629,101.376284307568));
#57654=CARTESIAN_POINT('Ctrl Pts',(5.07580078994123,-6.06962018986386,101.370838044886));
#57655=CARTESIAN_POINT('Ctrl Pts',(4.95402821506918,-6.16779844908681,101.364611780146));
#57656=CARTESIAN_POINT('Ctrl Pts',(4.94266095763329,-6.17691151929386,101.364029756897));
#57657=CARTESIAN_POINT('Ctrl Pts',(4.92544702115388,-6.19063389891782,101.363147042981));
#57658=CARTESIAN_POINT('Ctrl Pts',(4.9196188540688,-6.19526648003415,101.362847950794));
#57659=CARTESIAN_POINT('Ctrl Pts',(4.90887428015409,-6.20378219730299,101.362296117204));
#57660=CARTESIAN_POINT('Ctrl Pts',(4.90395977827138,-6.2076677377753,101.362043543186));
#57661=CARTESIAN_POINT('Ctrl Pts',(4.89607551691126,-6.21388604610928,101.361638063364));
#57662=CARTESIAN_POINT('Ctrl Pts',(4.89310868548351,-6.21622253891251,101.361485418916));
#57663=CARTESIAN_POINT('Ctrl Pts',(4.88742531663828,-6.2206918186541,101.361192884421));
#57664=CARTESIAN_POINT('Ctrl Pts',(4.88470906164277,-6.22282494622495,101.361053019188));
#57665=CARTESIAN_POINT('Ctrl Pts',(4.87851097366141,-6.22768586586458,101.360733745228));
#57666=CARTESIAN_POINT('Ctrl Pts',(4.87502825266005,-6.23041251440632,101.360554256603));
#57667=CARTESIAN_POINT('Ctrl Pts',(4.865986565639,-6.23747909657683,101.360088052759));
#57668=CARTESIAN_POINT('Ctrl Pts',(4.86042409075307,-6.24181451139192,101.359801023918));
#57669=CARTESIAN_POINT('Ctrl Pts',(4.82660988220073,-6.26809683024638,101.358054892878));
#57670=CARTESIAN_POINT('Ctrl Pts',(4.79821573081392,-6.28985902502156,101.356583202458));
#57671=CARTESIAN_POINT('Ctrl Pts',(4.30761808661232,-6.66061373563912,101.331076833713));
#57672=CARTESIAN_POINT('Ctrl Pts',(3.80863955449585,-6.95798414860458,101.304068741185));
#57673=CARTESIAN_POINT('Ctrl Pts',(2.74200745312272,-7.44426932886802,101.250345207927));
#57674=CARTESIAN_POINT('Ctrl Pts',(2.17626920047898,-7.62887885566547,101.223882076375));
#57675=CARTESIAN_POINT('Ctrl Pts',(1.54325771945928,-7.75919343962312,101.197443963005));
#57676=CARTESIAN_POINT('Ctrl Pts',(1.49126538578825,-7.76935357109912,101.195293361842));
#57677=CARTESIAN_POINT('Ctrl Pts',(1.42701668325811,-7.78124008440692,101.192661112911));
#57678=CARTESIAN_POINT('Ctrl Pts',(1.41485382736987,-7.78346083143229,101.192163920056));
#57679=CARTESIAN_POINT('Ctrl Pts',(1.39573138450325,-7.78690598606026,101.191383977268));
#57680=CARTESIAN_POINT('Ctrl Pts',(1.38877530248622,-7.78814959364303,101.19110062341));
#57681=CARTESIAN_POINT('Ctrl Pts',(1.37641846030216,-7.79034166706965,101.190597912631));
#57682=CARTESIAN_POINT('Ctrl Pts',(1.3710183668916,-7.79129384026519,101.190378439187));
#57683=CARTESIAN_POINT('Ctrl Pts',(1.35949214114425,-7.7933138514888,101.189910447001));
#57684=CARTESIAN_POINT('Ctrl Pts',(1.35336572928745,-7.79438008263954,101.189661978934));
#57685=CARTESIAN_POINT('Ctrl Pts',(1.33574913426386,-7.7974246510065,101.188948304212));
#57686=CARTESIAN_POINT('Ctrl Pts',(1.32425580446123,-7.79938481571741,101.188483669175));
#57687=CARTESIAN_POINT('Ctrl Pts',(1.27401758228586,-7.80783859524756,101.186456957174));
#57688=CARTESIAN_POINT('Ctrl Pts',(1.23522865231797,-7.81406901440788,101.184903157739));
#57689=CARTESIAN_POINT('Ctrl Pts',(0.638933879964946,-7.90529700461379,
101.161182224305));
#57690=CARTESIAN_POINT('Ctrl Pts',(0.073921455706333,-7.93073599718231,
101.141089579641));
#57691=CARTESIAN_POINT('Ctrl Pts',(-0.9063774347419,-7.87002272239105,101.107158435465));
#57692=CARTESIAN_POINT('Ctrl Pts',(-1.32101243080726,-7.81112525796685,
101.093047575357));
#57693=CARTESIAN_POINT('Ctrl Pts',(-1.87928904056887,-7.6860850732928,101.07251351499));
#57694=CARTESIAN_POINT('Ctrl Pts',(-2.02852692444375,-7.64805242923836,
101.06686557821));
#57695=CARTESIAN_POINT('Ctrl Pts',(-2.27835446602918,-7.57655819124616,
101.05700636134));
#57696=CARTESIAN_POINT('Ctrl Pts',(-2.37955619778753,-7.54538559025373,
101.052898147011));
#57697=CARTESIAN_POINT('Ctrl Pts',(-2.49744462419737,-7.50646555029554,
101.047946330544));
#57698=CARTESIAN_POINT('Ctrl Pts',(-2.51477139247207,-7.50067860544299,
101.047214284137));
#57699=CARTESIAN_POINT('Ctrl Pts',(-2.53754579985817,-7.49298442710936,
101.046246299686));
#57700=CARTESIAN_POINT('Ctrl Pts',(-2.54301173368562,-7.49113113176432,
101.046013541344));
#57701=CARTESIAN_POINT('Ctrl Pts',(-2.55193750858615,-7.48809383786527,
101.045632726764));
#57702=CARTESIAN_POINT('Ctrl Pts',(-2.55539857351451,-7.48691341627509,
101.045484883781));
#57703=CARTESIAN_POINT('Ctrl Pts',(-2.5620711261004,-7.48463252735323,101.04519951322));
#57704=CARTESIAN_POINT('Ctrl Pts',(-2.56528272704113,-7.48353239152389,
101.045062005561));
#57705=CARTESIAN_POINT('Ctrl Pts',(-2.5726486846059,-7.48100387946494,101.044746268814));
#57706=CARTESIAN_POINT('Ctrl Pts',(-2.57680256007557,-7.47957410988401,
101.044567955501));
#57707=CARTESIAN_POINT('Ctrl Pts',(-2.59007549949146,-7.47499317686568,
101.043997350104));
#57708=CARTESIAN_POINT('Ctrl Pts',(-2.59918995798751,-7.4718288021053,101.043604253362));
#57709=CARTESIAN_POINT('Ctrl Pts',(-2.68135509803504,-7.44313402047717,
101.040049301053));
#57710=CARTESIAN_POINT('Ctrl Pts',(-2.75403108214714,-7.41655049537198,
101.036824583172));
#57711=CARTESIAN_POINT('Ctrl Pts',(-2.84250899455956,-7.38270713730397,
101.03281088229));
#57712=CARTESIAN_POINT('Ctrl Pts',(-2.85869441468221,-7.37645499511943,
101.032073020297));
#57713=CARTESIAN_POINT('Ctrl Pts',(-3.59900682991811,-7.08768286441425,
100.998161774338));
#57714=CARTESIAN_POINT('Ctrl Pts',(-4.27758514548638,-6.70003935796028,
100.96046698622));
#57715=CARTESIAN_POINT('Ctrl Pts',(-5.03260917231484,-6.10657327914682,
100.91749461562));
#57716=CARTESIAN_POINT('Ctrl Pts',(-5.17248568598446,-5.98855487793442,
100.909453772229));
#57717=CARTESIAN_POINT('Ctrl Pts',(-5.45389990521558,-5.73389359797819,
100.893157306934));
#57718=CARTESIAN_POINT('Ctrl Pts',(-5.59468912316628,-5.59660799971827,
100.884936279293));
#57719=CARTESIAN_POINT('Ctrl Pts',(-5.75353757489532,-5.42972095784023,
100.875576982976));
#57720=CARTESIAN_POINT('Ctrl Pts',(-5.77669262697199,-5.40507970684385,
100.874210421121));
#57721=CARTESIAN_POINT('Ctrl Pts',(-5.8066963163013,-5.37273720213874,100.872436546115));
#57722=CARTESIAN_POINT('Ctrl Pts',(-5.81368870592683,-5.36517015430477,
100.872022918943));
#57723=CARTESIAN_POINT('Ctrl Pts',(-5.82502718977465,-5.35285164211235,
100.871351833239));
#57724=CARTESIAN_POINT('Ctrl Pts',(-5.82938228956825,-5.34810850548187,
100.871093980771));
#57725=CARTESIAN_POINT('Ctrl Pts',(-5.83772881947123,-5.33899599672367,
100.870599634621));
#57726=CARTESIAN_POINT('Ctrl Pts',(-5.84172114623067,-5.33462745396524,
100.870363101856));
#57727=CARTESIAN_POINT('Ctrl Pts',(-5.85081322321812,-5.32465614150758,
100.869824249268));
#57728=CARTESIAN_POINT('Ctrl Pts',(-5.8559098381162,-5.31905051363067,100.869522065972));
#57729=CARTESIAN_POINT('Ctrl Pts',(-5.86930864174531,-5.30427093530072,
100.868727300169));
#57730=CARTESIAN_POINT('Ctrl Pts',(-5.87759738968799,-5.29508479759359,
100.868235300866));
#57731=CARTESIAN_POINT('Ctrl Pts',(-5.9070337350238,-5.26230721510433,100.866486784868));
#57732=CARTESIAN_POINT('Ctrl Pts',(-5.92806125341561,-5.23860807648435,
100.865235449168));
#57733=CARTESIAN_POINT('Ctrl Pts',(-6.29239053119782,-4.82298672313823,
100.843511586092));
#57734=CARTESIAN_POINT('Ctrl Pts',(-6.59630891523287,-4.39819983262814,
100.82484794742));
#57735=CARTESIAN_POINT('Ctrl Pts',(-7.1101005549623,-3.505607731158,100.789270467862));
#57736=CARTESIAN_POINT('Ctrl Pts',(-7.32078269633412,-3.04119959820609,
100.772376901192));
#57737=CARTESIAN_POINT('Ctrl Pts',(-7.55590825743394,-2.35364552567562,
100.745933261476));
#57738=CARTESIAN_POINT('Ctrl Pts',(-7.61785960523315,-2.1446673945528,100.737705504192));
#57739=CARTESIAN_POINT('Ctrl Pts',(-7.67353438125915,-1.92376975046819,
100.728561496283));
#57740=CARTESIAN_POINT('Ctrl Pts',(-7.6759473079877,-1.91411934749301,100.728161136767));
#57741=CARTESIAN_POINT('Ctrl Pts',(-7.67941267725341,-1.90014781325215,
100.727580198348));
#57742=CARTESIAN_POINT('Ctrl Pts',(-7.68047969603304,-1.89583027152591,
100.727400493305));
#57743=CARTESIAN_POINT('Ctrl Pts',(-7.6823337947966,-1.88830066520649,100.727086776274));
#57744=CARTESIAN_POINT('Ctrl Pts',(-7.68312250348036,-1.88508899878534,
100.726952862701));
#57745=CARTESIAN_POINT('Ctrl Pts',(-7.68464259216893,-1.87888231023703,
100.726693871579));
#57746=CARTESIAN_POINT('Ctrl Pts',(-7.68537423323436,-1.87588736339735,
100.726568810346));
#57747=CARTESIAN_POINT('Ctrl Pts',(-7.68711466754766,-1.86874484827184,
100.726270345925));
#57748=CARTESIAN_POINT('Ctrl Pts',(-7.68812185275036,-1.86459689937094,
100.726096845743));
#57749=CARTESIAN_POINT('Ctrl Pts',(-7.69115355554793,-1.85206704524543,
100.725572239546));
#57750=CARTESIAN_POINT('Ctrl Pts',(-7.69316771976651,-1.84368267048238,
100.725220511862));
#57751=CARTESIAN_POINT('Ctrl Pts',(-7.71314481190045,-1.75992116134604,
100.721699953486));
#57752=CARTESIAN_POINT('Ctrl Pts',(-7.73001248888562,-1.68428962078129,
100.718466705807));
#57753=CARTESIAN_POINT('Ctrl Pts',(-7.74862849116477,-1.59463968851177,
100.714580421355));
#57754=CARTESIAN_POINT('Ctrl Pts',(-7.75145422817076,-1.58084679034245,
100.713981007621));
#57755=CARTESIAN_POINT('Ctrl Pts',(-7.85852014414527,-1.05105067840116,
100.690901565655));
#57756=CARTESIAN_POINT('Ctrl Pts',(-7.91102681554453,-0.525965126627474,
100.66609000105));
#57757=CARTESIAN_POINT('Ctrl Pts',(-7.91098891369753,0.217733859368774,
100.631422342524));
#57758=CARTESIAN_POINT('Ctrl Pts',(-7.90202210829038,0.434976997559752,
100.621340051967));
#57759=CARTESIAN_POINT('Ctrl Pts',(-7.84520037423542,1.12252005132096,100.589872468359));
#57760=CARTESIAN_POINT('Ctrl Pts',(-7.76416035555382,1.58906817388382,100.569248301842));
#57761=CARTESIAN_POINT('Ctrl Pts',(-7.63333321063003,2.07780002494947,100.548676478644));
#57762=CARTESIAN_POINT('Ctrl Pts',(-7.62452355610278,2.10989796598658,100.547329863717));
#57763=CARTESIAN_POINT('Ctrl Pts',(-7.6126100912286,2.15225542933883,100.545558580184));
#57764=CARTESIAN_POINT('Ctrl Pts',(-7.60968770066091,2.16256535942939,100.54512789623));
#57765=CARTESIAN_POINT('Ctrl Pts',(-7.60512132096831,2.17855126444294,100.544460799971));
#57766=CARTESIAN_POINT('Ctrl Pts',(-7.60349191104736,2.18423136990829,100.544223903722));
#57767=CARTESIAN_POINT('Ctrl Pts',(-7.60021911169365,2.19559227231814,100.543750353279));
#57768=CARTESIAN_POINT('Ctrl Pts',(-7.59857571360581,2.20127306275619,100.543513699564));
#57769=CARTESIAN_POINT('Ctrl Pts',(-7.59489617636393,2.213939025482,100.542986354258));
#57770=CARTESIAN_POINT('Ctrl Pts',(-7.59285676623179,2.22092324634593,100.542695771597));
#57771=CARTESIAN_POINT('Ctrl Pts',(-7.58687704036646,2.24129707569235,100.541848698057));
#57772=CARTESIAN_POINT('Ctrl Pts',(-7.58291091225359,2.25467911388393,100.541293065586));
#57773=CARTESIAN_POINT('Ctrl Pts',(-7.55416342296259,2.35074161494049,100.537309760978));
#57774=CARTESIAN_POINT('Ctrl Pts',(-7.52806535271193,2.43302359283986,100.533926120139));
#57775=CARTESIAN_POINT('Ctrl Pts',(-7.44117717061716,2.692169128023,100.523348487333));
#57776=CARTESIAN_POINT('Ctrl Pts',(-7.37545898387805,2.86731621398184,100.516318913368));
#57777=CARTESIAN_POINT('Ctrl Pts',(-7.0972527190762,3.53571116420255,100.489755922394));
#57778=CARTESIAN_POINT('Ctrl Pts',(-6.8409701164598,4.00916287686097,100.471612824162));
#57779=CARTESIAN_POINT('Ctrl Pts',(-6.29125336167091,4.81636062961772,100.437805691332));
#57780=CARTESIAN_POINT('Ctrl Pts',(-6.01393983171896,5.1584582346803,100.42229326878));
#57781=CARTESIAN_POINT('Ctrl Pts',(-5.68853786615748,5.4977622586455,100.403662002656));
#57782=CARTESIAN_POINT('Ctrl Pts',(-5.66728086402671,5.51967213473167,100.402443582324));
#57783=CARTESIAN_POINT('Ctrl Pts',(-5.63997745995344,5.54749012492507,100.400877519969));
#57784=CARTESIAN_POINT('Ctrl Pts',(-5.63404745637223,5.55351255454037,100.400537324226));
#57785=CARTESIAN_POINT('Ctrl Pts',(-5.62460746586162,5.56306899689698,100.399995680124));
#57786=CARTESIAN_POINT('Ctrl Pts',(-5.62110376148191,5.56660922930184,100.399794627289));
#57787=CARTESIAN_POINT('Ctrl Pts',(-5.61456170068763,5.57320702015331,100.399419193729));
#57788=CARTESIAN_POINT('Ctrl Pts',(-5.61152418266586,5.57626541043042,100.399244865275));
#57789=CARTESIAN_POINT('Ctrl Pts',(-5.60477230968753,5.5830525751418,100.398857338946));
#57790=CARTESIAN_POINT('Ctrl Pts',(-5.60105673230687,5.58678012647022,100.398644065484));
#57791=CARTESIAN_POINT('Ctrl Pts',(-5.59028928004631,5.59756074019381,100.398025975019));
#57792=CARTESIAN_POINT('Ctrl Pts',(-5.58322779988125,5.60460416158775,100.397620570276));
#57793=CARTESIAN_POINT('Ctrl Pts',(-5.53480451098001,5.65272128054489,100.394840321496));
#57794=CARTESIAN_POINT('Ctrl Pts',(-5.49300384585131,5.69334939710183,100.392439166055));
#57795=CARTESIAN_POINT('Ctrl Pts',(-5.36177473005591,5.81810685244853,100.384907386279));
#57796=CARTESIAN_POINT('Ctrl Pts',(-5.27083583596546,5.90061720582818,100.379697276894));
#57797=CARTESIAN_POINT('Ctrl Pts',(-4.97600865338472,6.15586321369664,100.362923665834));
#57798=CARTESIAN_POINT('Ctrl Pts',(-4.76527492016384,6.32040044497628,100.351111917005));
#57799=CARTESIAN_POINT('Ctrl Pts',(-4.3405024610174,6.61871607962593,100.328090856406));
#57800=CARTESIAN_POINT('Ctrl Pts',(-4.12757841522293,6.75355195359641,100.31689862308));
#57801=CARTESIAN_POINT('Ctrl Pts',(-3.4884110280167,7.11677358936094,100.284645966265));
#57802=CARTESIAN_POINT('Ctrl Pts',(-3.04721746686609,7.31655764942556,100.264100636953));
#57803=CARTESIAN_POINT('Ctrl Pts',(-2.56117772095599,7.48500191762332,100.243268466401));
#57804=CARTESIAN_POINT('Ctrl Pts',(-2.53178106810832,7.49499630868627,100.242014864729));
#57805=CARTESIAN_POINT('Ctrl Pts',(-2.49072378741304,7.50868600998582,100.240272667893));
#57806=CARTESIAN_POINT('Ctrl Pts',(-2.47911240445294,7.51252768839941,100.239780920752));
#57807=CARTESIAN_POINT('Ctrl Pts',(-2.45904707462449,7.51911480760394,100.238932789674));
#57808=CARTESIAN_POINT('Ctrl Pts',(-2.45059733485904,7.52187295212698,100.238576134571));
#57809=CARTESIAN_POINT('Ctrl Pts',(-2.4331304482501,7.52754189645614,100.237839904728));
#57810=CARTESIAN_POINT('Ctrl Pts',(-2.42411267685445,7.53045075089275,100.237460371161));
#57811=CARTESIAN_POINT('Ctrl Pts',(-2.40317266166712,7.53716384123068,100.236580371915));
#57812=CARTESIAN_POINT('Ctrl Pts',(-2.39124656175302,7.5409560065983,100.236080164084));
#57813=CARTESIAN_POINT('Ctrl Pts',(-2.35345110416821,7.55287522535579,100.234498040935));
#57814=CARTESIAN_POINT('Ctrl Pts',(-2.32754885274308,7.56089760676024,100.233418368921));
#57815=CARTESIAN_POINT('Ctrl Pts',(-1.84952057948756,7.70626207151502,100.213576909518));
#57816=CARTESIAN_POINT('Ctrl Pts',(-1.38601637328704,7.80296139722256,100.195802078976));
#57817=CARTESIAN_POINT('Ctrl Pts',(-0.271320596930701,7.93299374670284,
100.154764227382));
#57818=CARTESIAN_POINT('Ctrl Pts',(0.380732266471482,7.92848616729232,100.132170235629));
#57819=CARTESIAN_POINT('Ctrl Pts',(1.09092546501898,7.8357033645753,100.104154546035));
#57820=CARTESIAN_POINT('Ctrl Pts',(1.15691834915784,7.82623186274593,100.101516249931));
#57821=CARTESIAN_POINT('Ctrl Pts',(1.23369796513583,7.81421988423362,100.098398743971));
#57822=CARTESIAN_POINT('Ctrl Pts',(1.2446100124443,7.81248929493555,100.097954546016));
#57823=CARTESIAN_POINT('Ctrl Pts',(1.26101037227166,7.80985305768122,100.097285188924));
#57824=CARTESIAN_POINT('Ctrl Pts',(1.26650144289608,7.80896446633357,100.097060784342));
#57825=CARTESIAN_POINT('Ctrl Pts',(1.27627339036216,7.80737254482427,100.096660901859));
#57826=CARTESIAN_POINT('Ctrl Pts',(1.28055463843317,7.8066714826806,100.096485525548));
#57827=CARTESIAN_POINT('Ctrl Pts',(1.28955818251721,7.80518953029417,100.096116320886));
#57828=CARTESIAN_POINT('Ctrl Pts',(1.29428034944928,7.80440787547584,100.095922458047));
#57829=CARTESIAN_POINT('Ctrl Pts',(1.30670112901621,7.80234029517795,100.095411945606));
#57830=CARTESIAN_POINT('Ctrl Pts',(1.31439853977679,7.80104726304728,100.095094971715));
#57831=CARTESIAN_POINT('Ctrl Pts',(1.34867588245901,7.79523708826217,100.093680742644));
#57832=CARTESIAN_POINT('Ctrl Pts',(1.37523429381286,7.79059551681751,100.092577716693));
#57833=CARTESIAN_POINT('Ctrl Pts',(1.56200759307776,7.75696862496428,100.084766542404));
#57834=CARTESIAN_POINT('Ctrl Pts',(1.72129906038946,7.72318250001323,100.07780818696));
#57835=CARTESIAN_POINT('Ctrl Pts',(2.25330803439449,7.59306781266034,100.053800174322));
#57836=CARTESIAN_POINT('Ctrl Pts',(2.6200104509564,7.47446309144602,100.036001483499));
#57837=CARTESIAN_POINT('Ctrl Pts',(3.44424906383342,7.13973567394389,99.9949966121014));
#57838=CARTESIAN_POINT('Ctrl Pts',(3.89268937192721,6.90548663796145,99.9719819802656));
#57839=CARTESIAN_POINT('Ctrl Pts',(4.47866573998773,6.52405147965715,99.9421302858493));
#57840=CARTESIAN_POINT('Ctrl Pts',(4.63759468630427,6.41205249657729,99.934045434477));
#57841=CARTESIAN_POINT('Ctrl Pts',(4.80713027099167,6.28297457861285,99.9254324633464));
#57842=CARTESIAN_POINT('Ctrl Pts',(4.82197510311782,6.27158888233892,99.9246783729532));
#57843=CARTESIAN_POINT('Ctrl Pts',(4.84277771869976,6.25551615968285,99.9236217232832));
#57844=CARTESIAN_POINT('Ctrl Pts',(4.84876930861334,6.25087311093805,99.9233173959582));
#57845=CARTESIAN_POINT('Ctrl Pts',(4.85915829190651,6.24279847558177,99.9227897296545));
#57846=CARTESIAN_POINT('Ctrl Pts',(4.86355874150425,6.23937084012838,99.9225662314126));
#57847=CARTESIAN_POINT('Ctrl Pts',(4.87261443890336,6.23230169853359,99.9221063025599));
#57848=CARTESIAN_POINT('Ctrl Pts',(4.87726923921309,6.22865962307974,99.9218698952015));
#57849=CARTESIAN_POINT('Ctrl Pts',(4.88816527876279,6.22011448450788,99.9213165184604));
#57850=CARTESIAN_POINT('Ctrl Pts',(4.8944032348228,6.21520723454384,99.9209997191926));
#57851=CARTESIAN_POINT('Ctrl Pts',(4.90754525431525,6.20483666910452,99.9203323045868));
#57852=CARTESIAN_POINT('Ctrl Pts',(4.91444760642111,6.19937119696953,99.9199817775487));
#57853=CARTESIAN_POINT('Ctrl Pts',(4.9329402264708,6.18467793886277,99.9190426676083));
#57854=CARTESIAN_POINT('Ctrl Pts',(4.94451374657122,6.17542907808645,99.9184549447598));
#57855=CARTESIAN_POINT('Ctrl Pts',(5.21982013822596,5.95415067181425,99.9044744998658));
#57856=CARTESIAN_POINT('Ctrl Pts',(5.46971662557255,5.72543998247453,99.8918085124557));
#57857=CARTESIAN_POINT('Ctrl Pts',(6.24134696630462,4.92244433237357,99.8518663506104));
#57858=CARTESIAN_POINT('Ctrl Pts',(6.69332862510937,4.28765573010511,99.8274158127032));
#57859=CARTESIAN_POINT('Ctrl Pts',(7.13955321567155,3.41368341028276,99.7916598837286));
#57860=CARTESIAN_POINT('Ctrl Pts',(7.2261101768101,3.22641821892297,99.7838618870723));
#57861=CARTESIAN_POINT('Ctrl Pts',(7.31004807840962,3.0244461688235,99.7751015101087));
#57862=CARTESIAN_POINT('Ctrl Pts',(7.31482215439826,3.01288140869288,99.7745987019441));
#57863=CARTESIAN_POINT('Ctrl Pts',(7.32128166379366,2.99712798934742,99.7739120949657));
#57864=CARTESIAN_POINT('Ctrl Pts',(7.32299099783204,2.99294908587488,99.7737297978207));
#57865=CARTESIAN_POINT('Ctrl Pts',(7.3258862654845,2.98585353600751,99.7734199902282));
#57866=CARTESIAN_POINT('Ctrl Pts',(7.32707403849465,2.98293763724927,99.7732925961569));
#57867=CARTESIAN_POINT('Ctrl Pts',(7.32937048147655,2.97729038467326,99.7730457160712));
#57868=CARTESIAN_POINT('Ctrl Pts',(7.33047936282902,2.97455912708031,99.7729262442863));
#57869=CARTESIAN_POINT('Ctrl Pts',(7.33311572869248,2.96805513364818,99.7726415789999));
#57870=CARTESIAN_POINT('Ctrl Pts',(7.33464182741804,2.96428184053807,99.772476298312));
#57871=CARTESIAN_POINT('Ctrl Pts',(7.3391630799882,2.95307813432367,99.7719851570559));
#57872=CARTESIAN_POINT('Ctrl Pts',(7.34214985165806,2.94564436702189,99.7716587739686));
#57873=CARTESIAN_POINT('Ctrl Pts',(7.36598969705877,2.88604791739027,99.769038192788));
#57874=CARTESIAN_POINT('Ctrl Pts',(7.38629743357124,2.83367018607658,99.7667106857001));
#57875=CARTESIAN_POINT('Ctrl Pts',(7.49688445954315,2.53917597906776,99.7535080186805));
#57876=CARTESIAN_POINT('Ctrl Pts',(7.57581090604522,2.29298081468585,99.7420371661199));
#57877=CARTESIAN_POINT('Ctrl Pts',(7.7446870897463,1.66136070277169,99.7123228657999));
#57878=CARTESIAN_POINT('Ctrl Pts',(7.81804112351122,1.27221624981311,99.6937804089862));
#57879=CARTESIAN_POINT('Ctrl Pts',(7.88914287150531,0.636421606287519,99.6644236750676));
#57880=CARTESIAN_POINT('Ctrl Pts',(7.90503448577778,0.392489546487242,99.6533715694086));
#57881=CARTESIAN_POINT('Ctrl Pts',(7.91552880907088,-0.167596809893812,
99.6287048777381));
#57882=CARTESIAN_POINT('Ctrl Pts',(7.90252856392297,-0.483485702841372,
99.6153170579792));
#57883=CARTESIAN_POINT('Ctrl Pts',(7.86854159552577,-0.818791939995101,
99.6016914699375));
#57884=CARTESIAN_POINT('Ctrl Pts',(7.86632754754467,-0.839796407199824,
99.6008403105791));
#57885=CARTESIAN_POINT('Ctrl Pts',(7.86316473365714,-0.868691268266269,
99.5996726542763));
#57886=CARTESIAN_POINT('Ctrl Pts',(7.86228816642209,-0.87658937753575,99.5993538213362));
#57887=CARTESIAN_POINT('Ctrl Pts',(7.86076852500718,-0.890096099282285,
99.5988091466243));
#57888=CARTESIAN_POINT('Ctrl Pts',(7.86013134593871,-0.895705361421367,
99.5985831140884));
#57889=CARTESIAN_POINT('Ctrl Pts',(7.85882727334779,-0.907076918639451,
99.5981252211192));
#57890=CARTESIAN_POINT('Ctrl Pts',(7.8581600450813,-0.912839172431544,99.5978933716748));
#57891=CARTESIAN_POINT('Ctrl Pts',(7.85666658519136,-0.925613864363987,
99.5973797602184));
#57892=CARTESIAN_POINT('Ctrl Pts',(7.85583730131153,-0.932625944540598,
99.5970980972742));
#57893=CARTESIAN_POINT('Ctrl Pts',(7.85404800477728,-0.947583766617605,
99.5964978208854));
#57894=CARTESIAN_POINT('Ctrl Pts',(7.8530853194676,-0.955529184149296,99.5961792942968));
#57895=CARTESIAN_POINT('Ctrl Pts',(7.85053371720083,-0.976324224779369,
99.5953465017483));
#57896=CARTESIAN_POINT('Ctrl Pts',(7.84892530663879,-0.989171456168629,
99.5948328672741));
#57897=CARTESIAN_POINT('Ctrl Pts',(7.84406618424682,-1.02722570745312,99.5933139955531));
#57898=CARTESIAN_POINT('Ctrl Pts',(7.8407255165817,-1.05242118288927,99.5923116698681));
#57899=CARTESIAN_POINT('Ctrl Pts',(7.80414095386732,-1.31849651984598,99.5817608905861));
#57900=CARTESIAN_POINT('Ctrl Pts',(7.7599282718119,-1.55774650110608,99.5725765794849));
#57901=CARTESIAN_POINT('Ctrl Pts',(7.62382272278114,-2.14209092537623,99.5506371570535));
#57902=CARTESIAN_POINT('Ctrl Pts',(7.51946514300476,-2.48372432936004,99.5382572869988));
#57903=CARTESIAN_POINT('Ctrl Pts',(7.1751619024553,-3.3871986679991,99.5051024354206));
#57904=CARTESIAN_POINT('Ctrl Pts',(6.89274652289731,-3.93012949201877,99.4847860442526));
#57905=CARTESIAN_POINT('Ctrl Pts',(6.5399624588176,-4.45120071478618,99.4600034720082));
#57906=CARTESIAN_POINT('Ctrl Pts',(6.52903593324065,-4.4672123899258,99.4592362668394));
#57907=CARTESIAN_POINT('Ctrl Pts',(6.50591298124005,-4.50083059243569,99.4576131019517));
#57908=CARTESIAN_POINT('Ctrl Pts',(6.49370370174506,-4.51842804064291,99.4567562829169));
#57909=CARTESIAN_POINT('Ctrl Pts',(6.4778103344398,-4.54113796032228,99.4556409312745));
#57910=CARTESIAN_POINT('Ctrl Pts',(6.4741912973672,-4.54629604718704,99.4553869572314));
#57911=CARTESIAN_POINT('Ctrl Pts',(6.46861538554569,-4.55422303909627,99.4549956499527));
#57912=CARTESIAN_POINT('Ctrl Pts',(6.4666629040217,-4.55699499469011,99.4548586278604));
#57913=CARTESIAN_POINT('Ctrl Pts',(6.4627949933157,-4.56247881063084,99.4545871843959));
#57914=CARTESIAN_POINT('Ctrl Pts',(6.46087963747219,-4.56519072253496,99.4544527681612));
#57915=CARTESIAN_POINT('Ctrl Pts',(6.45662406367177,-4.57120805727374,99.4541541216499));
#57916=CARTESIAN_POINT('Ctrl Pts',(6.45428301498237,-4.57451288826081,99.4539898335175));
#57917=CARTESIAN_POINT('Ctrl Pts',(6.44757153365971,-4.58397199972684,99.453518848336));
#57918=CARTESIAN_POINT('Ctrl Pts',(6.44319483941243,-4.59012181064578,99.4532117183186));
#57919=CARTESIAN_POINT('Ctrl Pts',(6.41503966310326,-4.62956379232805,99.4512360680225));
#57920=CARTESIAN_POINT('Ctrl Pts',(6.39101241269682,-4.6626768077657,99.4495505791869));
#57921=CARTESIAN_POINT('Ctrl Pts',(6.31768939550816,-4.76209492282766,99.4444124328677));
#57922=CARTESIAN_POINT('Ctrl Pts',(6.26761176420726,-4.827814132025,99.4409104506965));
#57923=CARTESIAN_POINT('Ctrl Pts',(6.11762108727093,-5.01838635958545,99.4304726699977));
#57924=CARTESIAN_POINT('Ctrl Pts',(6.01494369595003,-5.14100548211801,99.4233919433543));
#57925=CARTESIAN_POINT('Ctrl Pts',(5.85849568780882,-5.31673141549757,99.4127982282299));
#57926=CARTESIAN_POINT('Ctrl Pts',(5.80756328980176,-5.37231914584692,99.4093777565908));
#57927=CARTESIAN_POINT('Ctrl Pts',(5.71588497968593,-5.46954959330668,99.4032823619629));
#57928=CARTESIAN_POINT('Ctrl Pts',(5.67545848518531,-5.51148661822496,99.4006149083414));
#57929=CARTESIAN_POINT('Ctrl Pts',(5.53958396480704,-5.64935778658685,99.3917261557212));
#57930=CARTESIAN_POINT('Ctrl Pts',(5.44213811231875,-5.74328880260512,99.3854748160144));
#57931=CARTESIAN_POINT('Ctrl Pts',(5.319697986479,-5.85539717556687,99.3778078028305));
#57932=CARTESIAN_POINT('Ctrl Pts',(5.29694400311783,-5.87598902149385,99.3763906445448));
#57933=CARTESIAN_POINT('Ctrl Pts',(5.25254054486855,-5.91570564121164,99.3736405720194));
#57934=CARTESIAN_POINT('Ctrl Pts',(5.23090498330669,-5.9348452775191,99.37230761675));
#57935=CARTESIAN_POINT('Ctrl Pts',(5.18861773342125,-5.97184329935418,99.3697164283078));
#57936=CARTESIAN_POINT('Ctrl Pts',(5.16797745524289,-5.98971413359468,99.3684581240923));
#57937=CARTESIAN_POINT('Ctrl Pts',(5.1275820444983,-6.02432517757995,99.3660084056036));
#57938=CARTESIAN_POINT('Ctrl Pts',(5.10783640679561,-6.04107595670407,99.3648169031677));
#57939=CARTESIAN_POINT('Ctrl Pts',(4.80785530833912,-6.29303611408109,99.3468074680148));
#57940=CARTESIAN_POINT('Ctrl Pts',(4.51169882551256,-6.50863936762877,99.3302694052976));
#57941=CARTESIAN_POINT('Ctrl Pts',(3.98985185790774,-6.83575120035174,99.3036202952102));
#57942=CARTESIAN_POINT('Ctrl Pts',(3.77185765655132,-6.95841340132563,99.2931406400967));
#57943=CARTESIAN_POINT('Ctrl Pts',(3.53014048909022,-7.07972081224955,99.2822028599964));
#57944=CARTESIAN_POINT('Ctrl Pts',(3.51183954113399,-7.08881666412164,99.2813788016947));
#57945=CARTESIAN_POINT('Ctrl Pts',(3.4856733465493,-7.10169546549257,99.280206338258));
#57946=CARTESIAN_POINT('Ctrl Pts',(3.47783684264528,-7.10553643717401,99.2798559312727));
#57947=CARTESIAN_POINT('Ctrl Pts',(3.46441424037888,-7.11208784545819,99.2792569942295));
#57948=CARTESIAN_POINT('Ctrl Pts',(3.45883128573846,-7.11480468371943,99.2790082438401));
#57949=CARTESIAN_POINT('Ctrl Pts',(3.44764800449408,-7.12023053976132,99.2785107068077));
#57950=CARTESIAN_POINT('Ctrl Pts',(3.44204766931522,-7.12293952976081,99.2782619212313));
#57951=CARTESIAN_POINT('Ctrl Pts',(3.43076228383155,-7.12838207055006,99.2777613292051));
#57952=CARTESIAN_POINT('Ctrl Pts',(3.42507714766687,-7.13111543341331,99.2775095293181));
#57953=CARTESIAN_POINT('Ctrl Pts',(3.40442249326649,-7.14101560960262,99.2765960869383));
#57954=CARTESIAN_POINT('Ctrl Pts',(3.38943365237568,-7.14814213412406,99.2759358251418));
#57955=CARTESIAN_POINT('Ctrl Pts',(3.21965351888269,-7.22821091951527,99.2684862663342));
#57956=CARTESIAN_POINT('Ctrl Pts',(3.06255245716724,-7.29616191113857,99.261869431837));
#57957=CARTESIAN_POINT('Ctrl Pts',(2.61090898559797,-7.47435074683545,99.2435334435158));
#57958=CARTESIAN_POINT('Ctrl Pts',(2.3118249078126,-7.57220227122811,99.2322081383494));
#57959=CARTESIAN_POINT('Ctrl Pts',(1.3467074025626,-7.82542558847317,99.1971158273906));
#57960=CARTESIAN_POINT('Ctrl Pts',(0.666120213178818,-7.91245681984313,
99.1746722991833));
#57961=CARTESIAN_POINT('Ctrl Pts',(-0.098538931491644,-7.91080566486328,
99.1451680353399));
#57962=CARTESIAN_POINT('Ctrl Pts',(-0.179985399648391,-7.90937169722905,
99.1419682129775));
#57963=CARTESIAN_POINT('Ctrl Pts',(-0.271393606983445,-7.90634976698278,
99.1382990547919));
#57964=CARTESIAN_POINT('Ctrl Pts',(-0.281393852452829,-7.90600016607141,
99.1378965928149));
#57965=CARTESIAN_POINT('Ctrl Pts',(-0.29560068183747,-7.90547651710202,
99.1373233139094));
#57966=CARTESIAN_POINT('Ctrl Pts',(-0.299807865784511,-7.90531808145919,
99.1371533544922));
#57967=CARTESIAN_POINT('Ctrl Pts',(-0.307521790600614,-7.90502142088696,
99.1368413808688));
#57968=CARTESIAN_POINT('Ctrl Pts',(-0.311028574181621,-7.90488422068152,
99.1366994233292));
#57969=CARTESIAN_POINT('Ctrl Pts',(-0.318159174690539,-7.90460048915112,
99.1364104982692));
#57970=CARTESIAN_POINT('Ctrl Pts',(-0.321782981055823,-7.90445379938105,
99.1362635221709));
#57971=CARTESIAN_POINT('Ctrl Pts',(-0.330788520227108,-7.90408305676143,
99.135897918106));
#57972=CARTESIAN_POINT('Ctrl Pts',(-0.336170120865733,-7.90385599962892,
99.1356791242157));
#57973=CARTESIAN_POINT('Ctrl Pts',(-0.356283091097092,-7.90298682681752,
99.1348602529049));
#57974=CARTESIAN_POINT('Ctrl Pts',(-0.371012810324826,-7.90230902427222,
99.1342582268371));
#57975=CARTESIAN_POINT('Ctrl Pts',(-0.740791280567599,-7.88425714921521,
99.119087924579));
#57976=CARTESIAN_POINT('Ctrl Pts',(-1.09424116330351,-7.84301433389644,
99.1032839521145));
#57977=CARTESIAN_POINT('Ctrl Pts',(-1.52769732588647,-7.76256165084227,
99.0832370562986));
#57978=CARTESIAN_POINT('Ctrl Pts',(-1.61145246815014,-7.74560799526967,
99.0793312559627));
#57979=CARTESIAN_POINT('Ctrl Pts',(-1.76458597635585,-7.71201950140238,
99.0721471778858));
#57980=CARTESIAN_POINT('Ctrl Pts',(-1.83404613116639,-7.6957964630024,99.0688721675812));
#57981=CARTESIAN_POINT('Ctrl Pts',(-2.14685899130905,-7.618260614275,99.0540703182836));
#57982=CARTESIAN_POINT('Ctrl Pts',(-2.38743541568688,-7.54632731602424,
99.0425470344009));
#57983=CARTESIAN_POINT('Ctrl Pts',(-2.77057569825167,-7.41160641280549,
99.0242225481883));
#57984=CARTESIAN_POINT('Ctrl Pts',(-2.91541930951471,-7.35583661023385,
99.0173002280066));
#57985=CARTESIAN_POINT('Ctrl Pts',(-3.35057297761001,-7.17341324995474,
98.9965870539977));
#57986=CARTESIAN_POINT('Ctrl Pts',(-3.63501578979728,-7.03355436400988,
98.983177140739));
#57987=CARTESIAN_POINT('Ctrl Pts',(-3.9291347920294,-6.86631550834635,98.9694867559329));
#57988=CARTESIAN_POINT('Ctrl Pts',(-3.94789419339772,-6.85554668290083,
98.9686142699369));
#57989=CARTESIAN_POINT('Ctrl Pts',(-3.97434578211093,-6.8402175812297,98.9673849938465));
#57990=CARTESIAN_POINT('Ctrl Pts',(-3.98207468439408,-6.83572104191864,
98.9670259283266));
#57991=CARTESIAN_POINT('Ctrl Pts',(-3.99519676543901,-6.82805703872501,
98.9664165050521));
#57992=CARTESIAN_POINT('Ctrl Pts',(-4.00059383327869,-6.82489627027542,
98.9661659077507));
#57993=CARTESIAN_POINT('Ctrl Pts',(-4.0113146395125,-6.81860059194601,98.9656682287564));
#57994=CARTESIAN_POINT('Ctrl Pts',(-4.01663846502505,-6.8154658396295,98.965421141666));
#57995=CARTESIAN_POINT('Ctrl Pts',(-4.0293752111622,-6.80794613570203,98.9648301378263));
#57996=CARTESIAN_POINT('Ctrl Pts',(-4.03678466090763,-6.80355530447192,
98.9644864328149));
#57997=CARTESIAN_POINT('Ctrl Pts',(-4.06202747552514,-6.78854068858828,
98.9633158335948));
#57998=CARTESIAN_POINT('Ctrl Pts',(-4.07982625955739,-6.77785877639054,
98.9624910358902));
#57999=CARTESIAN_POINT('Ctrl Pts',(-4.44833205168706,-6.55472309196552,
98.9454261307017));
#58000=CARTESIAN_POINT('Ctrl Pts',(-4.78205177830485,-6.31538444416365,
98.9302408317226));
#58001=CARTESIAN_POINT('Ctrl Pts',(-5.6396114194999,-5.59323335150966,98.8904533757213));
#58002=CARTESIAN_POINT('Ctrl Pts',(-6.11918817126435,-5.0640708433679,98.8674850588575));
#58003=CARTESIAN_POINT('Ctrl Pts',(-6.60913177132474,-4.35054227799108,
98.8351870114317));
#58004=CARTESIAN_POINT('Ctrl Pts',(-6.69291548296431,-4.22051159831969,
98.8292415453167));
#58005=CARTESIAN_POINT('Ctrl Pts',(-6.77883859686389,-4.07816177656102,
98.8225807160462));
#58006=CARTESIAN_POINT('Ctrl Pts',(-6.78482526762402,-4.06819398299678,
98.8221135171696));
#58007=CARTESIAN_POINT('Ctrl Pts',(-6.79308466360197,-4.0543731653533,98.8214645874316));
#58008=CARTESIAN_POINT('Ctrl Pts',(-6.79537615361268,-4.05053131595882,
98.8212840795219));
#58009=CARTESIAN_POINT('Ctrl Pts',(-6.79930657072544,-4.04392896374125,
98.8209736586407));
#58010=CARTESIAN_POINT('Ctrl Pts',(-6.80094708032332,-4.04116939970067,
98.8208438495583));
#58011=CARTESIAN_POINT('Ctrl Pts',(-6.80414612212475,-4.03578070392252,
98.8205902415996));
#58012=CARTESIAN_POINT('Ctrl Pts',(-6.8057048110604,-4.0331516666281,98.8204664531762));
#58013=CARTESIAN_POINT('Ctrl Pts',(-6.80944599912511,-4.02683306845275,
98.8201688002715));
#58014=CARTESIAN_POINT('Ctrl Pts',(-6.81162702197271,-4.0231426384842,98.8199948380175));
#58015=CARTESIAN_POINT('Ctrl Pts',(-6.81828733685086,-4.01185201860703,
98.8194622535595));
#58016=CARTESIAN_POINT('Ctrl Pts',(-6.82275689610632,-4.00424614154016,
98.8191029826965));
#58017=CARTESIAN_POINT('Ctrl Pts',(-6.8710693211684,-3.92171685672283,98.8151993889385));
#58018=CARTESIAN_POINT('Ctrl Pts',(-6.91368736612001,-3.84608666870855,
98.8115753563138));
#58019=CARTESIAN_POINT('Ctrl Pts',(-7.08479923543061,-3.53039348504515,
98.7963088409027));
#58020=CARTESIAN_POINT('Ctrl Pts',(-7.20209468422893,-3.28448942377354,
98.7840941466115));
#58021=CARTESIAN_POINT('Ctrl Pts',(-7.63002497484085,-2.2536250589279,98.7330514647578));
#58022=CARTESIAN_POINT('Ctrl Pts',(-7.82686484827529,-1.42719750252555,
98.6932871739802));
#58023=CARTESIAN_POINT('Ctrl Pts',(-7.89183441038454,-0.551383313984055,
98.6570776901287));
#58024=CARTESIAN_POINT('Ctrl Pts',(-7.89412831978794,-0.517505584026996,
98.6556846913589));
#58025=CARTESIAN_POINT('Ctrl Pts',(-7.89904588043883,-0.43721412235109,
98.6524011691919));
#58026=CARTESIAN_POINT('Ctrl Pts',(-7.90147868979835,-0.39078974393681,
98.650516831017));
#58027=CARTESIAN_POINT('Ctrl Pts',(-7.90402390803983,-0.33237136883006,
98.6481631937581));
#58028=CARTESIAN_POINT('Ctrl Pts',(-7.90451841767839,-0.320395461818897,
98.6476816180501));
#58029=CARTESIAN_POINT('Ctrl Pts',(-7.90525422919175,-0.30153608536691,
98.6469246929327));
#58030=CARTESIAN_POINT('Ctrl Pts',(-7.90551376135401,-0.294653369731292,
98.6466487574776));
#58031=CARTESIAN_POINT('Ctrl Pts',(-7.90595820000235,-0.282443537613245,
98.6461597892126));
#58032=CARTESIAN_POINT('Ctrl Pts',(-7.9061467114931,-0.277116561429293,
98.6459466406075));
#58033=CARTESIAN_POINT('Ctrl Pts',(-7.9065201654134,-0.266252819273748,
98.6455123177222));
#58034=CARTESIAN_POINT('Ctrl Pts',(-7.90670467616242,-0.260716040888589,
98.6452911574367));
#58035=CARTESIAN_POINT('Ctrl Pts',(-7.90709860651436,-0.248509861907359,
98.6448040246742));
#58036=CARTESIAN_POINT('Ctrl Pts',(-7.90730540428417,-0.241840377672786,
98.6445381366036));
#58037=CARTESIAN_POINT('Ctrl Pts',(-7.90779464743842,-0.225389802611338,
98.6438830058172));
#58038=CARTESIAN_POINT('Ctrl Pts',(-7.90806738453865,-0.215608422095326,
98.6434940751755));
#58039=CARTESIAN_POINT('Ctrl Pts',(-7.91010476584352,-0.13732761564452,
98.6403862582804));
#58040=CARTESIAN_POINT('Ctrl Pts',(-7.91099753799733,-0.0688075858804266,
98.637695474162));
#58041=CARTESIAN_POINT('Ctrl Pts',(-7.91099999491492,-0.00028364795766521,
98.635032539653));
#58042=CARTESIAN_POINT('',(-7.91859353182819,-0.00199197810995972,94.6422060731203));
#58043=CARTESIAN_POINT('Ctrl Pts',(-7.91099999474075,-0.000288464720890058,
98.6350327268391));
#58044=CARTESIAN_POINT('Ctrl Pts',(-7.91103062328953,0.839684092487076,
98.6023902214954));
#58045=CARTESIAN_POINT('Ctrl Pts',(-7.77730583138597,1.67422711870364,98.5749578136994));
#58046=CARTESIAN_POINT('Ctrl Pts',(-7.42655689965386,2.74042479551888,98.5358029537483));
#58047=CARTESIAN_POINT('Ctrl Pts',(-7.32400907867107,3.00375520449944,98.5256894808569));
#58048=CARTESIAN_POINT('Ctrl Pts',(-7.17009196186592,3.34394782886831,98.5113637873219));
#58049=CARTESIAN_POINT('Ctrl Pts',(-7.13114478758396,3.42621929651382,98.5077975022605));
#58050=CARTESIAN_POINT('Ctrl Pts',(-7.08685851709105,3.51574115993614,98.5037849221163));
#58051=CARTESIAN_POINT('Ctrl Pts',(-7.08291546091925,3.52367820851707,98.5034280145292));
#58052=CARTESIAN_POINT('Ctrl Pts',(-7.07706555912408,3.53540408767884,98.5028990067856));
#58053=CARTESIAN_POINT('Ctrl Pts',(-7.0751689790302,3.53919806020053,98.5027275757076));
#58054=CARTESIAN_POINT('Ctrl Pts',(-7.07193735667936,3.5456497103934,98.5024355984758));
#58055=CARTESIAN_POINT('Ctrl Pts',(-7.07060386268146,3.54830816905994,98.5023151540936));
#58056=CARTESIAN_POINT('Ctrl Pts',(-7.06788346172296,3.55372394789592,98.5020695147125));
#58057=CARTESIAN_POINT('Ctrl Pts',(-7.06649644473882,3.55648119955044,98.5019443123776));
#58058=CARTESIAN_POINT('Ctrl Pts',(-7.06318139287089,3.56306159715924,98.5016451642826));
#58059=CARTESIAN_POINT('Ctrl Pts',(-7.0612518713527,3.56688398227045,98.5014711204842));
#58060=CARTESIAN_POINT('Ctrl Pts',(-7.05540317668943,3.57844691037621,98.5009437962916));
#58061=CARTESIAN_POINT('Ctrl Pts',(-7.05147438489161,3.58618254889646,98.5005898853308));
#58062=CARTESIAN_POINT('Ctrl Pts',(-7.01156596432635,3.66444154128579,98.4969981625974));
#58063=CARTESIAN_POINT('Ctrl Pts',(-6.9745434661366,3.73442521569144,98.4936930956724));
#58064=CARTESIAN_POINT('Ctrl Pts',(-6.93233398209062,3.81139618049242,98.4899642829674));
#58065=CARTESIAN_POINT('Ctrl Pts',(-6.92817747305319,3.81894647577177,98.4895975027331));
#58066=CARTESIAN_POINT('Ctrl Pts',(-6.92361816357868,3.8271965166025,98.4891956367143));
#58067=CARTESIAN_POINT('Ctrl Pts',(-6.92322757148096,3.82790303498091,98.4891612128658));
#58068=CARTESIAN_POINT('Ctrl Pts',(-6.91927544433564,3.83504921470213,98.4888129392829));
#58069=CARTESIAN_POINT('Ctrl Pts',(-6.91570504349921,3.84148394562412,98.4884986098132));
#58070=CARTESIAN_POINT('Ctrl Pts',(-6.90845613855813,3.85450537654047,98.4878610651518));
#58071=CARTESIAN_POINT('Ctrl Pts',(-6.9047771806402,3.86109181465925,98.4875378259152));
#58072=CARTESIAN_POINT('Ctrl Pts',(-6.89679718717741,3.87533051689597,98.4868374131411));
#58073=CARTESIAN_POINT('Ctrl Pts',(-6.89249282852016,3.88298089926368,98.4864600657942));
#58074=CARTESIAN_POINT('Ctrl Pts',(-6.88509922021377,3.89607095178625,98.4858126864471));
#58075=CARTESIAN_POINT('Ctrl Pts',(-6.88201622828243,3.90151416335293,98.4855429756838));
#58076=CARTESIAN_POINT('Ctrl Pts',(-6.8654389046754,3.93070165934789,98.4840940107957));
#58077=CARTESIAN_POINT('Ctrl Pts',(-6.85182825999647,3.95437938945336,98.482908878132));
#58078=CARTESIAN_POINT('Ctrl Pts',(-6.82567006959681,3.99934490832982,98.4806404255342));
#58079=CARTESIAN_POINT('Ctrl Pts',(-6.8131448212225,4.02064537357291,98.4795581668644));
#58080=CARTESIAN_POINT('Ctrl Pts',(-6.77045281847062,4.09247515225899,98.4758834363703));
#58081=CARTESIAN_POINT('Ctrl Pts',(-6.7398225072289,4.14272574171468,98.4732704293331));
#58082=CARTESIAN_POINT('Ctrl Pts',(-6.30489273367682,4.83865783395751,98.436538955058));
#58083=CARTESIAN_POINT('Ctrl Pts',(-5.80994425430318,5.4230138527528,98.3995968292326));
#58084=CARTESIAN_POINT('Ctrl Pts',(-5.1406475965354,6.01455679953584,98.3600487731515));
#58085=CARTESIAN_POINT('Ctrl Pts',(-5.04014193459184,6.0990263652341,98.3543235445333));
#58086=CARTESIAN_POINT('Ctrl Pts',(-4.82746261223385,6.26892245021479,98.3426536058549));
#58087=CARTESIAN_POINT('Ctrl Pts',(-4.71501325342544,6.35393081206213,98.3367259783309));
#58088=CARTESIAN_POINT('Ctrl Pts',(-4.54076388835753,6.47848351235244,98.3279001669359));
#58089=CARTESIAN_POINT('Ctrl Pts',(-4.48058964161118,6.52024555994305,98.3249148271406));
#58090=CARTESIAN_POINT('Ctrl Pts',(-4.40879917934463,6.56860625310678,98.3214251338252));
#58091=CARTESIAN_POINT('Ctrl Pts',(-4.39773656800285,6.57601789785428,98.3208893781535));
#58092=CARTESIAN_POINT('Ctrl Pts',(-4.38178586962855,6.58664617471966,98.3201197451903));
#58093=CARTESIAN_POINT('Ctrl Pts',(-4.37691287415178,6.58988535033082,98.3198850012067));
#58094=CARTESIAN_POINT('Ctrl Pts',(-4.36732289497881,6.5962446676921,98.3194237771986));
#58095=CARTESIAN_POINT('Ctrl Pts',(-4.3626061509536,6.59936516317258,98.3191972836696));
#58096=CARTESIAN_POINT('Ctrl Pts',(-4.35321797362151,6.605561714071,98.3187471771981));
#58097=CARTESIAN_POINT('Ctrl Pts',(-4.34854661675347,6.60863787828811,98.3185235601602));
#58098=CARTESIAN_POINT('Ctrl Pts',(-4.33748690415214,6.61590407454525,98.3179949508565));
#58099=CARTESIAN_POINT('Ctrl Pts',(-4.33109572772815,6.62008981547634,98.3176901225879));
#58100=CARTESIAN_POINT('Ctrl Pts',(-4.30874384170872,6.63468240026392,98.3166262870595));
#58101=CARTESIAN_POINT('Ctrl Pts',(-4.29275154692513,6.64504087337539,98.3158691223763));
#58102=CARTESIAN_POINT('Ctrl Pts',(-4.10150413376521,6.7679364453558,98.3068614933759));
#58103=CARTESIAN_POINT('Ctrl Pts',(-3.92190203461756,6.87357200238294,98.2988760650579));
#58104=CARTESIAN_POINT('Ctrl Pts',(-3.53496792098419,7.08104296237951,98.2825184857444));
#58105=CARTESIAN_POINT('Ctrl Pts',(-3.32692550442964,7.18113790300319,98.2742062002916));
#58106=CARTESIAN_POINT('Ctrl Pts',(-2.97282975724784,7.33280688163681,98.2606186684839));
#58107=CARTESIAN_POINT('Ctrl Pts',(-2.82911022444385,7.38944585188904,98.2552500457254));
#58108=CARTESIAN_POINT('Ctrl Pts',(-2.42160049744456,7.53641001501459,98.2402816425567));
#58109=CARTESIAN_POINT('Ctrl Pts',(-2.15456613759086,7.61705101941511,98.2307696106032));
#58110=CARTESIAN_POINT('Ctrl Pts',(-1.66061579052986,7.73815863733083,98.2129938161668));
#58111=CARTESIAN_POINT('Ctrl Pts',(-1.4351249485373,7.7831324781503,98.2048100142019));
#58112=CARTESIAN_POINT('Ctrl Pts',(-1.09707295936599,7.83536547998387,98.1920607380509));
#58113=CARTESIAN_POINT('Ctrl Pts',(-0.985789996760458,7.85014251977632,
98.1877869993949));
#58114=CARTESIAN_POINT('Ctrl Pts',(-0.819622733686073,7.86861861349604,
98.1812450557757));
#58115=CARTESIAN_POINT('Ctrl Pts',(-0.764952136581349,7.87412141438865,
98.1790661095606));
#58116=CARTESIAN_POINT('Ctrl Pts',(-0.700465852246928,7.87993430857362,
98.1764671723144));
#58117=CARTESIAN_POINT('Ctrl Pts',(-0.690699889029933,7.88079632902611,
98.1760728124853));
#58118=CARTESIAN_POINT('Ctrl Pts',(-0.675724804958643,7.88209009776201,
98.1754669462412));
#58119=CARTESIAN_POINT('Ctrl Pts',(-0.670516792644889,7.88253484304782,
98.1752560245704));
#58120=CARTESIAN_POINT('Ctrl Pts',(-0.661430342221076,7.88330172253212,
98.1748876583817));
#58121=CARTESIAN_POINT('Ctrl Pts',(-0.657552095951879,7.88362615723995,
98.1747303161144));
#58122=CARTESIAN_POINT('Ctrl Pts',(-0.649440117962912,7.88429873729437,
98.1744009656177));
#58123=CARTESIAN_POINT('Ctrl Pts',(-0.645206342919183,7.88464633453357,
98.1742289333189));
#58124=CARTESIAN_POINT('Ctrl Pts',(-0.633492193008744,7.8855985798844,98.1737525680257));
#58125=CARTESIAN_POINT('Ctrl Pts',(-0.626011247001237,7.88619599298329,
98.1734479200408));
#58126=CARTESIAN_POINT('Ctrl Pts',(-0.596619157148946,7.88850109946786,
98.1722493214382));
#58127=CARTESIAN_POINT('Ctrl Pts',(-0.574701921391014,7.89012811701314,
98.1713519236345));
#58128=CARTESIAN_POINT('Ctrl Pts',(-0.190394621470284,7.91704725096131,
98.1555561179059));
#58129=CARTESIAN_POINT('Ctrl Pts',(0.173287754408456,7.91743819494948,98.1396859477806));
#58130=CARTESIAN_POINT('Ctrl Pts',(0.876783607160662,7.86969231320218,98.1085077294422));
#58131=CARTESIAN_POINT('Ctrl Pts',(1.216032846893,7.8244538951565,98.0932554166211));
#58132=CARTESIAN_POINT('Ctrl Pts',(1.99705461786198,7.66826866151834,98.0583952027387));
#58133=CARTESIAN_POINT('Ctrl Pts',(2.43433014304468,7.54086654960135,98.0391066239844));
#58134=CARTESIAN_POINT('Ctrl Pts',(2.89204107640193,7.36351349495035,98.0192029221403));
#58135=CARTESIAN_POINT('Ctrl Pts',(2.9257202941035,7.35019682516418,98.0177396516237));
#58136=CARTESIAN_POINT('Ctrl Pts',(2.97236040762036,7.33138409298264,98.0157147440098));
#58137=CARTESIAN_POINT('Ctrl Pts',(2.98539969212397,7.32608406938041,98.0151487968078));
#58138=CARTESIAN_POINT('Ctrl Pts',(3.00745910818325,7.31704899692897,98.014191595302));
#58139=CARTESIAN_POINT('Ctrl Pts',(3.0164865813896,7.31333200502505,98.0137999461504));
#58140=CARTESIAN_POINT('Ctrl Pts',(3.03424534237298,7.30598149733122,98.0130296270588));
#58141=CARTESIAN_POINT('Ctrl Pts',(3.04297704129478,7.30234901684003,98.0126509351407));
#58142=CARTESIAN_POINT('Ctrl Pts',(3.06375326808353,7.29366214798591,98.0117500192264));
#58143=CARTESIAN_POINT('Ctrl Pts',(3.07579184434141,7.28859356448904,98.0112281084987));
#58144=CARTESIAN_POINT('Ctrl Pts',(3.11512726115402,7.27191742224343,98.0095231621728));
#58145=CARTESIAN_POINT('Ctrl Pts',(3.14237147573479,7.2601861115074,98.0083428788613));
#58146=CARTESIAN_POINT('Ctrl Pts',(3.49152641311007,7.10750707289723,97.9932235847153));
#58147=CARTESIAN_POINT('Ctrl Pts',(3.80377448883215,6.94541114067332,97.9798034219212));
#58148=CARTESIAN_POINT('Ctrl Pts',(4.53682438160458,6.50055438265888,97.9479551901981));
#58149=CARTESIAN_POINT('Ctrl Pts',(4.94322454817824,6.19713655633724,97.9300385815423));
#58150=CARTESIAN_POINT('Ctrl Pts',(5.45146371245044,5.73568052074982,97.9048716968738));
#58151=CARTESIAN_POINT('Ctrl Pts',(5.5808772896782,5.60983891370074,97.8981722591362));
#58152=CARTESIAN_POINT('Ctrl Pts',(5.79597196089109,5.38586581871726,97.8863311581107));
#58153=CARTESIAN_POINT('Ctrl Pts',(5.8837428038153,5.28984025364703,97.881278223978));
#58154=CARTESIAN_POINT('Ctrl Pts',(5.98388133289996,5.17470697560628,97.8751949407279));
#58155=CARTESIAN_POINT('Ctrl Pts',(5.99858677314492,5.15765303214884,97.8742932363095));
#58156=CARTESIAN_POINT('Ctrl Pts',(6.01796247917411,5.13498801229907,97.8730937129871));
#58157=CARTESIAN_POINT('Ctrl Pts',(6.02269817219764,5.12943281594483,97.8727996196094));
#58158=CARTESIAN_POINT('Ctrl Pts',(6.03045320258931,5.12031024587037,97.8723165075815));
#58159=CARTESIAN_POINT('Ctrl Pts',(6.03347708637872,5.11674672918151,97.8721277510668));
#58160=CARTESIAN_POINT('Ctrl Pts',(6.03932441141383,5.10984351806587,97.8717620118368));
#58161=CARTESIAN_POINT('Ctrl Pts',(6.04214824523947,5.10650415723458,97.8715850520534));
#58162=CARTESIAN_POINT('Ctrl Pts',(6.04865190629147,5.0988002223273,97.8711767149903));
#58163=CARTESIAN_POINT('Ctrl Pts',(6.05232977797308,5.09443400674606,97.8709452234577));
#58164=CARTESIAN_POINT('Ctrl Pts',(6.06404827904625,5.08049169106819,97.8702057959547));
#58165=CARTESIAN_POINT('Ctrl Pts',(6.07207090267749,5.07090054168168,97.8696967971465));
#58166=CARTESIAN_POINT('Ctrl Pts',(6.15048601704781,4.97670135573191,97.8646940085584));
#58167=CARTESIAN_POINT('Ctrl Pts',(6.21911944045624,4.89066300621524,97.8600879812803));
#58168=CARTESIAN_POINT('Ctrl Pts',(6.78918291423936,4.14462587330208,97.819916693381));
#58169=CARTESIAN_POINT('Ctrl Pts',(7.18582867158503,3.41101931780166,97.7797379126986));
#58170=CARTESIAN_POINT('Ctrl Pts',(7.56019750592523,2.34857712119468,97.7301028480254));
#58171=CARTESIAN_POINT('Ctrl Pts',(7.64315750718252,2.0626607488169,97.7174316340397));
#58172=CARTESIAN_POINT('Ctrl Pts',(7.71617822900833,1.74508427469245,97.704139359267));
#58173=CARTESIAN_POINT('Ctrl Pts',(7.72238574655146,1.71740618125558,97.7029871603612));
#58174=CARTESIAN_POINT('Ctrl Pts',(7.73144848490893,1.67595440187964,97.7012708971637));
#58175=CARTESIAN_POINT('Ctrl Pts',(7.7344160194328,1.66220566508413,97.700703175499));
#58176=CARTESIAN_POINT('Ctrl Pts',(7.73976473955366,1.63710030728881,97.6996692857803));
#58177=CARTESIAN_POINT('Ctrl Pts',(7.74215763290902,1.62574623741598,97.6992027370078));
#58178=CARTESIAN_POINT('Ctrl Pts',(7.74589706205311,1.60780747421338,97.6984672445526));
#58179=CARTESIAN_POINT('Ctrl Pts',(7.7472601974562,1.6012262810927,97.698197759984));
#58180=CARTESIAN_POINT('Ctrl Pts',(7.7496862370617,1.5894377850813,97.6977156655051));
#58181=CARTESIAN_POINT('Ctrl Pts',(7.75075228285058,1.58423113704496,97.6975029533019));
#58182=CARTESIAN_POINT('Ctrl Pts',(7.75319642646384,1.57223223677979,97.6970132458772));
#58183=CARTESIAN_POINT('Ctrl Pts',(7.75457084785914,1.56543923534461,97.696736370617));
#58184=CARTESIAN_POINT('Ctrl Pts',(7.75830561854607,1.54685472483215,97.6959798828393));
#58185=CARTESIAN_POINT('Ctrl Pts',(7.7606480157795,1.5350596038438,97.695500855593));
#58186=CARTESIAN_POINT('Ctrl Pts',(7.77186746763788,1.47788207416338,97.6931840265366));
#58187=CARTESIAN_POINT('Ctrl Pts',(7.78037347612177,1.43242731956261,97.6913583264785));
#58188=CARTESIAN_POINT('Ctrl Pts',(7.89690744740592,0.778001972829458,97.6652990699414));
#58189=CARTESIAN_POINT('Ctrl Pts',(7.93356207358035,0.15849534543688,97.6436748423889));
#58190=CARTESIAN_POINT('Ctrl Pts',(7.87599193376859,-0.832039215783152,
97.6099191098755));
#58191=CARTESIAN_POINT('Ctrl Pts',(7.82791166507928,-1.2030455904179,97.597400382183));
#58192=CARTESIAN_POINT('Ctrl Pts',(7.72315450416746,-1.72065955025918,97.57871467027));
#58193=CARTESIAN_POINT('Ctrl Pts',(7.68808432706997,-1.87113351773135,97.5731299358965));
#58194=CARTESIAN_POINT('Ctrl Pts',(7.61511522158514,-2.14736213019957,97.5624452902443));
#58195=CARTESIAN_POINT('Ctrl Pts',(7.57844674478341,-2.2733863844321,97.5574003481183));
#58196=CARTESIAN_POINT('Ctrl Pts',(7.53240725752627,-2.41809586659111,97.5513503408022));
#58197=CARTESIAN_POINT('Ctrl Pts',(7.52607501833165,-2.43773286406106,97.5505238223494));
#58198=CARTESIAN_POINT('Ctrl Pts',(7.51783596263814,-2.46294501600872,97.5494552666602));
#58199=CARTESIAN_POINT('Ctrl Pts',(7.51599958616362,-2.46854328166255,97.5492175290945));
#58200=CARTESIAN_POINT('Ctrl Pts',(7.51303246372053,-2.47755466682522,97.5488340865821));
#58201=CARTESIAN_POINT('Ctrl Pts',(7.51190563859322,-2.48096908584139,97.548688623508));
#58202=CARTESIAN_POINT('Ctrl Pts',(7.50974777017838,-2.48749274545329,97.5484103599258));
#58203=CARTESIAN_POINT('Ctrl Pts',(7.50871712600336,-2.49060210631536,97.5482775846585));
#58204=CARTESIAN_POINT('Ctrl Pts',(7.50634746221691,-2.49773632895663,97.5479726048631));
#58205=CARTESIAN_POINT('Ctrl Pts',(7.50500713715356,-2.50176075268644,97.5478003200286));
#58206=CARTESIAN_POINT('Ctrl Pts',(7.50149332571056,-2.51228299163291,97.5473492270486));
#58207=CARTESIAN_POINT('Ctrl Pts',(7.4993146377957,-2.51877905114278,97.5470701015766));
#58208=CARTESIAN_POINT('Ctrl Pts',(7.4854862962818,-2.5598331749768,97.5453020843156));
#58209=CARTESIAN_POINT('Ctrl Pts',(7.47360640837212,-2.59431265371224,97.5437993399137));
#58210=CARTESIAN_POINT('Ctrl Pts',(7.27326670990972,-3.16296930268619,97.5187349091876));
#58211=CARTESIAN_POINT('Ctrl Pts',(7.02822016210335,-3.67543575339453,97.4921630072294));
#58212=CARTESIAN_POINT('Ctrl Pts',(6.53399001681676,-4.47558325333099,97.4486546516073));
#58213=CARTESIAN_POINT('Ctrl Pts',(6.31505682868153,-4.77953603394728,97.431538199999));
#58214=CARTESIAN_POINT('Ctrl Pts',(5.88640863203758,-5.29350579782384,97.4022131556574));
#58215=CARTESIAN_POINT('Ctrl Pts',(5.68485226007152,-5.50940018598597,97.389747079382));
#58216=CARTESIAN_POINT('Ctrl Pts',(5.4614183339711,-5.72337600292911,97.3772429288809));
#58217=CARTESIAN_POINT('Ctrl Pts',(5.45112475483649,-5.73318079250761,97.3766695838246));
#58218=CARTESIAN_POINT('Ctrl Pts',(5.43461007812739,-5.74882658595001,97.3757540563638));
#58219=CARTESIAN_POINT('Ctrl Pts',(5.42840588515143,-5.75468534007516,97.375411085317));
#58220=CARTESIAN_POINT('Ctrl Pts',(5.41656534588007,-5.76583043169145,97.3747583798875));
#58221=CARTESIAN_POINT('Ctrl Pts',(5.41093071220174,-5.77111856934268,97.3744485658628));
#58222=CARTESIAN_POINT('Ctrl Pts',(5.40102613526343,-5.78038681746712,97.3739053614396));
#58223=CARTESIAN_POINT('Ctrl Pts',(5.39675952294974,-5.78437046920302,97.3736718147524));
#58224=CARTESIAN_POINT('Ctrl Pts',(5.38841240834321,-5.79214673086284,97.3732157868127));
#58225=CARTESIAN_POINT('Ctrl Pts',(5.38433230223921,-5.79593975930175,97.3729932871693));
#58226=CARTESIAN_POINT('Ctrl Pts',(5.37462719476904,-5.80494291989034,97.3724650094431));
#58227=CARTESIAN_POINT('Ctrl Pts',(5.36899861373186,-5.81014919534193,97.3721594008083));
#58228=CARTESIAN_POINT('Ctrl Pts',(5.3490837804728,-5.82851619284444,97.3710808250136));
#58229=CARTESIAN_POINT('Ctrl Pts',(5.33475658011445,-5.84163252342766,97.3703098012611));
#58230=CARTESIAN_POINT('Ctrl Pts',(5.15104940200479,-6.00857410413087,97.3604859332803));
#58231=CARTESIAN_POINT('Ctrl Pts',(4.97511535242341,-6.1550394160176,97.3517578594723));
#58232=CARTESIAN_POINT('Ctrl Pts',(4.20555875145421,-6.74110958580798,97.3160106768834));
#58233=CARTESIAN_POINT('Ctrl Pts',(3.55837042889229,-7.10402463619165,97.292126285281));
#58234=CARTESIAN_POINT('Ctrl Pts',(2.58965136890302,-7.4811975796568,97.2552687244209));
#58235=CARTESIAN_POINT('Ctrl Pts',(2.30303676950454,-7.57433831039145,97.2441778146889));
#58236=CARTESIAN_POINT('Ctrl Pts',(2.00159784898675,-7.65360302245741,97.2316829495804));
#58237=CARTESIAN_POINT('Ctrl Pts',(1.99134946309288,-7.65627588898199,97.2312571652177));
#58238=CARTESIAN_POINT('Ctrl Pts',(1.97663439589886,-7.66008216017931,97.2306443587212));
#58239=CARTESIAN_POINT('Ctrl Pts',(1.97217201576983,-7.66123226221728,97.2304583324528));
#58240=CARTESIAN_POINT('Ctrl Pts',(1.96439891896064,-7.66322840347944,97.2301339601485));
#58241=CARTESIAN_POINT('Ctrl Pts',(1.96108864468724,-7.66407620032041,97.2299957178634));
#58242=CARTESIAN_POINT('Ctrl Pts',(1.95470340669017,-7.66570712071519,97.2297288609134));
#58243=CARTESIAN_POINT('Ctrl Pts',(1.95162851841142,-7.66649053966545,97.2296002636309));
#58244=CARTESIAN_POINT('Ctrl Pts',(1.94435507284219,-7.66833900613128,97.2292958659644));
#58245=CARTESIAN_POINT('Ctrl Pts',(1.94015611433258,-7.66940245482756,97.2291199724013));
#58246=CARTESIAN_POINT('Ctrl Pts',(1.92549819789716,-7.67310198216848,97.2285053852268));
#58247=CARTESIAN_POINT('Ctrl Pts',(1.91503476413194,-7.67572010881576,97.2280656549363));
#58248=CARTESIAN_POINT('Ctrl Pts',(1.79171308720687,-7.70630940144599,97.2228713699366));
#58249=CARTESIAN_POINT('Ctrl Pts',(1.67826155591636,-7.73180936952574,97.2179781574631));
#58250=CARTESIAN_POINT('Ctrl Pts',(1.54700860990204,-7.75828565632762,97.2122193604017));
#58251=CARTESIAN_POINT('Ctrl Pts',(1.52971110488684,-7.76171475207178,97.2114584752931));
#58252=CARTESIAN_POINT('Ctrl Pts',(1.47402506449754,-7.77256069769861,97.2090030067418));
#58253=CARTESIAN_POINT('Ctrl Pts',(1.43559331801603,-7.7797507313171,97.2072992900871));
#58254=CARTESIAN_POINT('Ctrl Pts',(0.784062469934928,-7.89665078917537,
97.1782808343046));
#58255=CARTESIAN_POINT('Ctrl Pts',(0.160173348218243,-7.9338659838256,97.1486653187389));
#58256=CARTESIAN_POINT('Ctrl Pts',(-0.944464206621942,-7.86929673197473,
97.0985651305772));
#58257=CARTESIAN_POINT('Ctrl Pts',(-1.42373331740787,-7.79685410944183,
97.0775873709844));
#58258=CARTESIAN_POINT('Ctrl Pts',(-1.91165181435241,-7.6765786788436,97.0572816980415));
#58259=CARTESIAN_POINT('Ctrl Pts',(-1.92984890895361,-7.67202424830974,
97.0565257971353));
#58260=CARTESIAN_POINT('Ctrl Pts',(-1.95613539972124,-7.66534573526553,
97.0554358706597));
#58261=CARTESIAN_POINT('Ctrl Pts',(-1.96423783056654,-7.66327349692795,
97.0551001924466));
#58262=CARTESIAN_POINT('Ctrl Pts',(-1.9783514766435,-7.65964000502872,97.054515951078));
#58263=CARTESIAN_POINT('Ctrl Pts',(-1.98436416020023,-7.65808451583731,
97.0542672042068));
#58264=CARTESIAN_POINT('Ctrl Pts',(-1.99596215424604,-7.65506952316407,
97.0537876810943));
#58265=CARTESIAN_POINT('Ctrl Pts',(-2.00154770952764,-7.65361098386329,
97.0535568742796));
#58266=CARTESIAN_POINT('Ctrl Pts',(-2.01476324621697,-7.65014459403056,
97.0530110865562));
#58267=CARTESIAN_POINT('Ctrl Pts',(-2.02239183716026,-7.64813143881188,
97.0526962752672));
#58268=CARTESIAN_POINT('Ctrl Pts',(-2.04905904217515,-7.64105137943291,
97.051596630049));
#58269=CARTESIAN_POINT('Ctrl Pts',(-2.06808180045149,-7.63592475180237,
97.0508137053821));
#58270=CARTESIAN_POINT('Ctrl Pts',(-2.29707558458299,-7.57329250795526,
97.0414065991472));
#58271=CARTESIAN_POINT('Ctrl Pts',(-2.50461298827936,-7.50721239689595,
97.0330638404919));
#58272=CARTESIAN_POINT('Ctrl Pts',(-3.37448376529839,-7.1901480976028,96.9985912197845));
#58273=CARTESIAN_POINT('Ctrl Pts',(-4.00416266530335,-6.8594443966711,96.9752132996989));
#58274=CARTESIAN_POINT('Ctrl Pts',(-4.73127418515022,-6.34292949258007,
96.9434764196706));
#58275=CARTESIAN_POINT('Ctrl Pts',(-4.87736879414416,-6.23129025629814,
96.9368009531319));
#58276=CARTESIAN_POINT('Ctrl Pts',(-5.11391640284901,-6.03711202913383,
96.9252596042317));
#58277=CARTESIAN_POINT('Ctrl Pts',(-5.20658246249291,-5.95737855214634,
96.9205379163792));
#58278=CARTESIAN_POINT('Ctrl Pts',(-5.3123013031363,-5.86206282547851,96.9148653713794));
#58279=CARTESIAN_POINT('Ctrl Pts',(-5.32719093719876,-5.84853506534418,
96.9140596525386));
#58280=CARTESIAN_POINT('Ctrl Pts',(-5.34650396682319,-5.83085355227314,
96.9130054667608));
#58281=CARTESIAN_POINT('Ctrl Pts',(-5.35097451863605,-5.82675119735221,
96.9127608068036));
#58282=CARTESIAN_POINT('Ctrl Pts',(-5.35821996701821,-5.82008711683847,
96.9123632396936));
#58283=CARTESIAN_POINT('Ctrl Pts',(-5.36099776344828,-5.81752853390104,
96.9122105685375));
#58284=CARTESIAN_POINT('Ctrl Pts',(-5.36632732351144,-5.81261250437512,
96.9119171668694));
#58285=CARTESIAN_POINT('Ctrl Pts',(-5.36887936196677,-5.81025537008366,
96.9117764596559));
#58286=CARTESIAN_POINT('Ctrl Pts',(-5.37473316796677,-5.80484148092104,
96.9114532208598));
#58287=CARTESIAN_POINT('Ctrl Pts',(-5.37803388001659,-5.80178359047776,
96.9112706035782));
#58288=CARTESIAN_POINT('Ctrl Pts',(-5.38680420246663,-5.79364455408345,
96.9107844265311));
#58289=CARTESIAN_POINT('Ctrl Pts',(-5.39226921995256,-5.7885584901245,96.9104804981609));
#58290=CARTESIAN_POINT('Ctrl Pts',(-5.42864588562386,-5.75460802607219,
96.9084509876503));
#58291=CARTESIAN_POINT('Ctrl Pts',(-5.45933233624993,-5.7255043451088,96.9067077044633));
#58292=CARTESIAN_POINT('Ctrl Pts',(-6.04085123980206,-5.16505400895148,
96.8730979799399));
#58293=CARTESIAN_POINT('Ctrl Pts',(-6.51193319830862,-4.55680401131707,
96.8363714951854));
#58294=CARTESIAN_POINT('Ctrl Pts',(-6.98551451496333,-3.71827483474916,
96.7931407226837));
#58295=CARTESIAN_POINT('Ctrl Pts',(-7.07622549551358,-3.54260069036832,
96.7844122518932));
#58296=CARTESIAN_POINT('Ctrl Pts',(-7.25427466057304,-3.16359040556691,
96.7663415805362));
#58297=CARTESIAN_POINT('Ctrl Pts',(-7.33985743820359,-2.9596128293226,96.7570583219185));
#58298=CARTESIAN_POINT('Ctrl Pts',(-7.42962216189515,-2.71771899361371,
96.7465605196102));
#58299=CARTESIAN_POINT('Ctrl Pts',(-7.4422151182252,-2.68304233632671,96.7450674896062));
#58300=CARTESIAN_POINT('Ctrl Pts',(-7.45821650276812,-2.63800048686436,
96.7431433785664));
#58301=CARTESIAN_POINT('Ctrl Pts',(-7.46184659423552,-2.62771485823343,
96.7427050166952));
#58302=CARTESIAN_POINT('Ctrl Pts',(-7.46768573813538,-2.61106035126055,
96.7419968678546));
#58303=CARTESIAN_POINT('Ctrl Pts',(-7.46990793680914,-2.60469611612557,
96.7417266494842));
#58304=CARTESIAN_POINT('Ctrl Pts',(-7.47414020983483,-2.59252519399573,
96.7412106263256));
#58305=CARTESIAN_POINT('Ctrl Pts',(-7.47615165808868,-2.58671899193715,
96.7409647766034));
#58306=CARTESIAN_POINT('Ctrl Pts',(-7.48074276589454,-2.57341631340396,
96.7404022415784));
#58307=CARTESIAN_POINT('Ctrl Pts',(-7.48331792751358,-2.56591828548731,
96.7400857038874));
#58308=CARTESIAN_POINT('Ctrl Pts',(-7.4912067603749,-2.54283569782629,96.7391128836655));
#58309=CARTESIAN_POINT('Ctrl Pts',(-7.49648306633123,-2.52723836493505,
96.7384578251028));
#58310=CARTESIAN_POINT('Ctrl Pts',(-7.53554001963557,-2.4105832081675,96.7335755300657));
#58311=CARTESIAN_POINT('Ctrl Pts',(-7.56732525490818,-2.30886646748193,
96.7294138602341));
#58312=CARTESIAN_POINT('Ctrl Pts',(-7.60067265469127,-2.19405223036691,
96.7248160019466));
#58313=CARTESIAN_POINT('Ctrl Pts',(-7.60426777669348,-2.18155943663766,
96.7243170257901));
#58314=CARTESIAN_POINT('Ctrl Pts',(-7.61592926683549,-2.14065750266921,
96.7226875988423));
#58315=CARTESIAN_POINT('Ctrl Pts',(-7.62386739121038,-2.1122119126991,96.7215610879662));
#58316=CARTESIAN_POINT('Ctrl Pts',(-7.63698072819023,-2.06418423447807,
96.7196700504169));
#58317=CARTESIAN_POINT('Ctrl Pts',(-7.64224033152176,-2.04462561818233,
96.7189030064159));
#58318=CARTESIAN_POINT('Ctrl Pts',(-7.66548484278247,-1.95684461499868,
96.7154738553882));
#58319=CARTESIAN_POINT('Ctrl Pts',(-7.68263194283628,-1.8884028770051,96.7128365084654));
#58320=CARTESIAN_POINT('Ctrl Pts',(-7.83974466683613,-1.2236985072228,96.6875456135794));
#58321=CARTESIAN_POINT('Ctrl Pts',(-7.9109317711384,-0.613344488602599,
96.6670372056062));
#58322=CARTESIAN_POINT('Ctrl Pts',(-7.91101242576093,0.111181534452813,
96.6419010833049));
#58323=CARTESIAN_POINT('Ctrl Pts',(-7.90864379419039,0.223229965881314,
96.6379849084005));
#58324=CARTESIAN_POINT('Ctrl Pts',(-7.89454116945423,0.55577610161645,96.6261922541451));
#58325=CARTESIAN_POINT('Ctrl Pts',(-7.87595655219195,0.775864345783876,
96.6181662688479));
#58326=CARTESIAN_POINT('Ctrl Pts',(-7.84721533378392,1.00259316009575,96.6094266656964));
#58327=CARTESIAN_POINT('Ctrl Pts',(-7.84622545995603,1.01031063063012,96.6091286140298));
#58328=CARTESIAN_POINT('Ctrl Pts',(-7.84440492471485,1.02434023164507,96.6085857293842));
#58329=CARTESIAN_POINT('Ctrl Pts',(-7.84357802507125,1.03065285005739,96.6083410695011));
#58330=CARTESIAN_POINT('Ctrl Pts',(-7.83164117232685,1.12093335521034,96.6048363958647));
#58331=CARTESIAN_POINT('Ctrl Pts',(-7.81919137533511,1.20471588297486,96.6015140913077));
#58332=CARTESIAN_POINT('Ctrl Pts',(-7.80375591026096,1.29823592672715,96.5977119409698));
#58333=CARTESIAN_POINT('Ctrl Pts',(-7.80209358286066,1.30818903485749,96.5973060955238));
#58334=CARTESIAN_POINT('Ctrl Pts',(-7.79966086636241,1.32258523514935,96.5967173209093));
#58335=CARTESIAN_POINT('Ctrl Pts',(-7.79890570888939,1.32703092586222,96.5965352585944));
#58336=CARTESIAN_POINT('Ctrl Pts',(-7.79757215536432,1.33484124043352,96.5962149760306));
#58337=CARTESIAN_POINT('Ctrl Pts',(-7.79699538104706,1.33820614373744,96.5960768488786));
#58338=CARTESIAN_POINT('Ctrl Pts',(-7.79580427132759,1.34512816999395,96.5957924133221));
#58339=CARTESIAN_POINT('Ctrl Pts',(-7.79518967916424,1.34868524731664,96.5956460901138));
#58340=CARTESIAN_POINT('Ctrl Pts',(-7.79361989610751,1.35773376749065,96.5952734672555));
#58341=CARTESIAN_POINT('Ctrl Pts',(-7.79266134349221,1.36322457934425,96.5950469724143));
#58342=CARTESIAN_POINT('Ctrl Pts',(-7.78870571988583,1.38574280563983,96.5941165388882));
#58343=CARTESIAN_POINT('Ctrl Pts',(-7.78565866342316,1.40276123485916,96.5934096979755));
#58344=CARTESIAN_POINT('Ctrl Pts',(-7.76489014763892,1.51660516842505,96.5886575269258));
#58345=CARTESIAN_POINT('Ctrl Pts',(-7.74541928441796,1.61309914602549,96.5845143465535));
#58346=CARTESIAN_POINT('Ctrl Pts',(-7.67484520212179,1.93203479706354,96.5704972841864));
#58347=CARTESIAN_POINT('Ctrl Pts',(-7.61591933615756,2.15261891438979,96.5602798822387));
#58348=CARTESIAN_POINT('Ctrl Pts',(-7.40049836046155,2.83855604864864,96.5275013703022));
#58349=CARTESIAN_POINT('Ctrl Pts',(-7.21018808598541,3.29211219139292,96.5044061538131));
#58350=CARTESIAN_POINT('Ctrl Pts',(-6.77675913635513,4.10415242373941,96.4628974326378));
#58351=CARTESIAN_POINT('Ctrl Pts',(-6.54388146844187,4.46611958430109,96.4443169523507));
#58352=CARTESIAN_POINT('Ctrl Pts',(-6.26576455361047,4.82958534178484,96.4257630011086));
#58353=CARTESIAN_POINT('Ctrl Pts',(-6.24868617022989,4.85166169291655,96.4246362373281));
#58354=CARTESIAN_POINT('Ctrl Pts',(-6.22537607679404,4.88146619689521,96.4231151904258));
#58355=CARTESIAN_POINT('Ctrl Pts',(-6.21924623645517,4.88927354320106,96.4227167639095));
#58356=CARTESIAN_POINT('Ctrl Pts',(-6.20956101399402,4.90156156035102,96.4220896968384));
#58357=CARTESIAN_POINT('Ctrl Pts',(-6.20601544916333,4.90604993465733,96.4218606554426));
#58358=CARTESIAN_POINT('Ctrl Pts',(-6.19917274986115,4.91469290485161,96.4214196115396));
#58359=CARTESIAN_POINT('Ctrl Pts',(-6.19587629957406,4.91884803710618,96.4212075812104));
#58360=CARTESIAN_POINT('Ctrl Pts',(-6.18808238639251,4.92865189624494,96.4207073099323));
#58361=CARTESIAN_POINT('Ctrl Pts',(-6.18358136022797,4.93429779167698,96.4204192153971));
#58362=CARTESIAN_POINT('Ctrl Pts',(-6.17041615704708,4.95076535747961,96.4195789290689));
#58363=CARTESIAN_POINT('Ctrl Pts',(-6.16173123658752,4.96157045164196,96.4190275908163));
#58364=CARTESIAN_POINT('Ctrl Pts',(-6.09891567633802,5.03930131507524,96.4150613168749));
#58365=CARTESIAN_POINT('Ctrl Pts',(-6.04372336392814,5.10536371573891,96.4116905487208));
#58366=CARTESIAN_POINT('Ctrl Pts',(-5.86529457670188,5.31198452574972,96.4011384051676));
#58367=CARTESIAN_POINT('Ctrl Pts',(-5.73814716425488,5.44908547273671,96.3941239854296));
#58368=CARTESIAN_POINT('Ctrl Pts',(-5.37924052860825,5.80958021610153,96.3755058460303));
#58369=CARTESIAN_POINT('Ctrl Pts',(-5.13851793240377,6.02354531109611,96.3642701795929));
#58370=CARTESIAN_POINT('Ctrl Pts',(-4.78131289246753,6.30400584539876,96.3486541259081));
#58371=CARTESIAN_POINT('Ctrl Pts',(-4.67516442566243,6.38312466080315,96.3441315841764));
#58372=CARTESIAN_POINT('Ctrl Pts',(-4.44885679575818,6.54313059641601,96.3346484133025));
#58373=CARTESIAN_POINT('Ctrl Pts',(-4.32836137464931,6.6234561897225,96.3296883597387));
#58374=CARTESIAN_POINT('Ctrl Pts',(-3.8788135012559,6.90562876539424,96.3112882736169));
#58375=CARTESIAN_POINT('Ctrl Pts',(-3.53734659762423,7.08660869166393,96.2975251323113));
#58376=CARTESIAN_POINT('Ctrl Pts',(-3.16033565001871,7.25237011756868,96.2811759425317));
#58377=CARTESIAN_POINT('Ctrl Pts',(-3.13654106038979,7.26269260603235,96.2801393037005));
#58378=CARTESIAN_POINT('Ctrl Pts',(-3.10657306277045,7.27551848111512,96.2788272024673));
#58379=CARTESIAN_POINT('Ctrl Pts',(-3.1004464331563,7.27813144137852,96.2785586167917));
#58380=CARTESIAN_POINT('Ctrl Pts',(-3.09079979236863,7.28223126828615,96.2781351699607));
#58381=CARTESIAN_POINT('Ctrl Pts',(-3.0872819792554,7.28372333231947,96.2779806384275));
#58382=CARTESIAN_POINT('Ctrl Pts',(-3.08107304680822,7.28635151589261,96.2777076865322));
#58383=CARTESIAN_POINT('Ctrl Pts',(-3.07838237409141,7.28748869582368,96.2775893338576));
#58384=CARTESIAN_POINT('Ctrl Pts',(-3.07220750777794,7.29009439756027,96.2773175681336));
#58385=CARTESIAN_POINT('Ctrl Pts',(-3.06872289730959,7.29156190918982,96.2771640905632));
#58386=CARTESIAN_POINT('Ctrl Pts',(-3.05903343260587,7.29563436201795,96.2767370090156));
#58387=CARTESIAN_POINT('Ctrl Pts',(-3.05282631402452,7.298233881009,96.2764630597826));
#58388=CARTESIAN_POINT('Ctrl Pts',(-3.01843808015325,7.31258400356743,96.2749433927296));
#58389=CARTESIAN_POINT('Ctrl Pts',(-2.99019279262271,7.32417915305233,96.2736879343907));
#58390=CARTESIAN_POINT('Ctrl Pts',(-2.90937067494452,7.35681250209504,96.2700763863128));
#58391=CARTESIAN_POINT('Ctrl Pts',(-2.85663492969077,7.3774497285887,96.2676968832453));
#58392=CARTESIAN_POINT('Ctrl Pts',(-2.56208704443017,7.48908432858149,96.254297989862));
#58393=CARTESIAN_POINT('Ctrl Pts',(-2.31616577948795,7.56875362615606,96.2427102251037));
#58394=CARTESIAN_POINT('Ctrl Pts',(-1.69949489723706,7.73566031037718,96.2134164926229));
#58395=CARTESIAN_POINT('Ctrl Pts',(-1.32548972226909,7.80844428460587,96.1954656300268));
#58396=CARTESIAN_POINT('Ctrl Pts',(-0.373670040999901,7.92329465183099,
96.1510911589718));
#58397=CARTESIAN_POINT('Ctrl Pts',(0.206291507140203,7.9294300211983,96.1253621958436));
#58398=CARTESIAN_POINT('Ctrl Pts',(0.821585396059392,7.8683235584578,96.1001591034313));
#58399=CARTESIAN_POINT('Ctrl Pts',(0.861324412788489,7.86407264096575,96.0985398492904));
#58400=CARTESIAN_POINT('Ctrl Pts',(0.912335613862318,7.85822462306197,96.0964719624382));
#58401=CARTESIAN_POINT('Ctrl Pts',(0.92363853841978,7.85690411998279,96.0960144396939));
#58402=CARTESIAN_POINT('Ctrl Pts',(0.941671159765812,7.85475794637879,96.0952855780316));
#58403=CARTESIAN_POINT('Ctrl Pts',(0.948402691753518,7.85394800746179,96.0950137333293));
#58404=CARTESIAN_POINT('Ctrl Pts',(0.961003937724138,7.85241538682511,96.094505289953));
#58405=CARTESIAN_POINT('Ctrl Pts',(0.966873895970737,7.85169477533735,96.0942686248819));
#58406=CARTESIAN_POINT('Ctrl Pts',(0.979968085285564,7.85007239166202,96.0937410927008));
#58407=CARTESIAN_POINT('Ctrl Pts',(0.987191894947225,7.8491672275112,96.0934503348867));
#58408=CARTESIAN_POINT('Ctrl Pts',(1.00828188472015,7.84649501585229,96.092602252508));
#58409=CARTESIAN_POINT('Ctrl Pts',(1.02214467650056,7.84470118333229,96.092045789505));
#58410=CARTESIAN_POINT('Ctrl Pts',(1.12206971331923,7.83150160222718,96.0880418176562));
#58411=CARTESIAN_POINT('Ctrl Pts',(1.20794535777824,7.81871641685071,96.0846388643084));
#58412=CARTESIAN_POINT('Ctrl Pts',(1.47995026465021,7.77363175057574,96.0739703756444));
#58413=CARTESIAN_POINT('Ctrl Pts',(1.66514509046851,7.73607785304665,96.0668729920068));
#58414=CARTESIAN_POINT('Ctrl Pts',(2.19791205870354,7.6080224184368,96.0467817592011));
#58415=CARTESIAN_POINT('Ctrl Pts',(2.5408915497368,7.50044721911272,96.0342751639329));
#58416=CARTESIAN_POINT('Ctrl Pts',(3.22335765049642,7.2341828902578,96.0090172477693));
#58417=CARTESIAN_POINT('Ctrl Pts',(3.56126482398948,7.07395290000678,95.9963035989677));
#58418=CARTESIAN_POINT('Ctrl Pts',(4.10987154105077,6.76451047309412,95.973629768836));
#58419=CARTESIAN_POINT('Ctrl Pts',(4.32691273155878,6.62778045055618,95.9640539688491));
#58420=CARTESIAN_POINT('Ctrl Pts',(4.55208049507337,6.47014883878998,95.9530852815463));
#58421=CARTESIAN_POINT('Ctrl Pts',(4.56718921423601,6.45949266600812,95.952344411044));
#58422=CARTESIAN_POINT('Ctrl Pts',(4.58795927230733,6.44473425297556,95.9513193449102));
#58423=CARTESIAN_POINT('Ctrl Pts',(4.59365282044811,6.44067726567226,95.9510376657455));
#58424=CARTESIAN_POINT('Ctrl Pts',(4.60271302661466,6.43420321184034,95.9505883434147));
#58425=CARTESIAN_POINT('Ctrl Pts',(4.60608318490636,6.43179103129553,95.9504209681172));
#58426=CARTESIAN_POINT('Ctrl Pts',(4.61292012632336,6.42688938167106,95.9500809353272));
#58427=CARTESIAN_POINT('Ctrl Pts',(4.61638679316003,6.42439975343267,95.9499082691961));
#58428=CARTESIAN_POINT('Ctrl Pts',(4.62433833192559,6.41867950149711,95.9495116452716));
#58429=CARTESIAN_POINT('Ctrl Pts',(4.62882183307099,6.41544698275524,95.9492875853979));
#58430=CARTESIAN_POINT('Ctrl Pts',(4.63822938347108,6.40864932281908,95.9488165682628));
#58431=CARTESIAN_POINT('Ctrl Pts',(4.64315271592294,6.40508320108781,95.9485695588241));
#58432=CARTESIAN_POINT('Ctrl Pts',(4.65616594568902,6.3956344281398,95.9479153342462));
#58433=CARTESIAN_POINT('Ctrl Pts',(4.66424878956958,6.38974211372425,95.9475076111499));
#58434=CARTESIAN_POINT('Ctrl Pts',(4.68854045188261,6.37196307676189,95.9462781937171));
#58435=CARTESIAN_POINT('Ctrl Pts',(4.70471508863984,6.36002994844121,95.9454541124694));
#58436=CARTESIAN_POINT('Ctrl Pts',(4.86344359001757,6.24198831145528,95.9373143581233));
#58437=CARTESIAN_POINT('Ctrl Pts',(5.0024237335047,6.13117060847886,95.9297685174195));
#58438=CARTESIAN_POINT('Ctrl Pts',(5.51429814914899,5.69402321241479,95.9006716992088));
#58439=CARTESIAN_POINT('Ctrl Pts',(5.85998946726534,5.33759476389158,95.8783451970682));
#58440=CARTESIAN_POINT('Ctrl Pts',(6.47242387740073,4.57438877954085,95.8354146718432));
#58441=CARTESIAN_POINT('Ctrl Pts',(6.7396453995751,4.17067808196937,95.8148765266282));
#58442=CARTESIAN_POINT('Ctrl Pts',(6.98314797155833,3.71759850361982,95.7940447956728));
#58443=CARTESIAN_POINT('Ctrl Pts',(6.99775387182588,3.69003184204701,95.7927851906566));
#58444=CARTESIAN_POINT('Ctrl Pts',(7.01787030259318,3.65151579844336,95.7910359863309));
#58445=CARTESIAN_POINT('Ctrl Pts',(7.02351896186821,3.64063903782347,95.790543201772));
#58446=CARTESIAN_POINT('Ctrl Pts',(7.03322365724367,3.62184553947672,95.7896937629072));
#58447=CARTESIAN_POINT('Ctrl Pts',(7.03729165348537,3.61393501724022,95.7893368354693));
#58448=CARTESIAN_POINT('Ctrl Pts',(7.04566369985572,3.59758721097279,95.7886004772886));
#58449=CARTESIAN_POINT('Ctrl Pts',(7.04996596030238,3.58914901769213,95.7882210869907));
#58450=CARTESIAN_POINT('Ctrl Pts',(7.05990676247647,3.56956489355508,95.7873421666059));
#58451=CARTESIAN_POINT('Ctrl Pts',(7.0655340867857,3.55841328316873,95.7868428923687));
#58452=CARTESIAN_POINT('Ctrl Pts',(7.08323791279317,3.52312222643507,95.7852666438951));
#58453=CARTESIAN_POINT('Ctrl Pts',(7.09521733419043,3.4989342012077,95.7841918891196));
#58454=CARTESIAN_POINT('Ctrl Pts',(7.30385967126524,3.07218007163691,95.7653272167629));
#58455=CARTESIAN_POINT('Ctrl Pts',(7.46610399375868,2.65367464547184,95.7484151715762));
#58456=CARTESIAN_POINT('Ctrl Pts',(7.77065112702025,1.61388463516782,95.70868260423));
#58457=CARTESIAN_POINT('Ctrl Pts',(7.87512193502151,0.984871284622181,95.6865733832196));
#58458=CARTESIAN_POINT('Ctrl Pts',(7.90781296147897,0.247110931022991,95.6580643207213));
#58459=CARTESIAN_POINT('Ctrl Pts',(7.91036337754415,0.143943204957923,95.6540147659644));
#58460=CARTESIAN_POINT('Ctrl Pts',(7.9109604597805,0.0280537537648842,95.6493701330604));
#58461=CARTESIAN_POINT('Ctrl Pts',(7.91099531099237,0.0153491394390962,
95.6488596630811));
#58462=CARTESIAN_POINT('Ctrl Pts',(7.91100147895069,-0.00310191107860394,
95.6481163626843));
#58463=CARTESIAN_POINT('Ctrl Pts',(7.91099713867137,-0.00884836093567081,
95.6478845938201));
#58464=CARTESIAN_POINT('Ctrl Pts',(7.9109784577727,-0.0189741893473824,
95.6474757052003));
#58465=CARTESIAN_POINT('Ctrl Pts',(7.91096674178525,-0.0233535748588086,
95.6472987013354));
#58466=CARTESIAN_POINT('Ctrl Pts',(7.91093538774854,-0.0322974604931215,
95.6469368794338));
#58467=CARTESIAN_POINT('Ctrl Pts',(7.91091543571675,-0.0368619572749811,
95.6467520474831));
#58468=CARTESIAN_POINT('Ctrl Pts',(7.91085485507063,-0.0484305851894007,
95.6462831414925));
#58469=CARTESIAN_POINT('Ctrl Pts',(7.9108088749487,-0.0554346744395597,
95.6459988270105));
#58470=CARTESIAN_POINT('Ctrl Pts',(7.91068970315355,-0.0705333082266814,
95.6453850108176));
#58471=CARTESIAN_POINT('Ctrl Pts',(7.9106133891904,-0.0786278141427979,
95.6450553669859));
#58472=CARTESIAN_POINT('Ctrl Pts',(7.91036130516155,-0.101622130730678,
95.644117281685));
#58473=CARTESIAN_POINT('Ctrl Pts',(7.9101558622616,-0.116521523949013,95.6435074651082));
#58474=CARTESIAN_POINT('Ctrl Pts',(7.90789931916879,-0.252338191318515,
95.6379299946108));
#58475=CARTESIAN_POINT('Ctrl Pts',(7.90311821115909,-0.373180210877427,
95.6328236809456));
#58476=CARTESIAN_POINT('Ctrl Pts',(7.88418649428543,-0.675852062245692,
95.6197327206794));
#58477=CARTESIAN_POINT('Ctrl Pts',(7.86651429446798,-0.857391148501546,
95.6116138226172));
#58478=CARTESIAN_POINT('Ctrl Pts',(7.7396488046092,-1.8157835800511,95.5678713233792));
#58479=CARTESIAN_POINT('Ctrl Pts',(7.52158521407871,-2.57398035063378,95.5307291673917));
#58480=CARTESIAN_POINT('Ctrl Pts',(7.12630885129493,-3.43909238697278,95.490428268475));
#58481=CARTESIAN_POINT('Ctrl Pts',(7.0523608937518,-3.58829271828867,95.4835338276845));
#58482=CARTESIAN_POINT('Ctrl Pts',(6.96597612026184,-3.74958254701549,95.4761406356499));
#58483=CARTESIAN_POINT('Ctrl Pts',(6.95815001769743,-3.76408566859512,95.4754763723515));
#58484=CARTESIAN_POINT('Ctrl Pts',(6.94646287912882,-3.78558295252171,95.4744925383661));
#58485=CARTESIAN_POINT('Ctrl Pts',(6.94263650005714,-3.79259584586781,95.4741717121122));
#58486=CARTESIAN_POINT('Ctrl Pts',(6.93606874107987,-3.80458982612083,95.4736232180157));
#58487=CARTESIAN_POINT('Ctrl Pts',(6.93333260574277,-3.80957376937896,95.4733953597574));
#58488=CARTESIAN_POINT('Ctrl Pts',(6.92800003494938,-3.81926241456342,95.4729525281461));
#58489=CARTESIAN_POINT('Ctrl Pts',(6.92540417430987,-3.8239674290153,95.4727375340056));
#58490=CARTESIAN_POINT('Ctrl Pts',(6.91918593370908,-3.8352109313663,95.47222389482));
#58491=CARTESIAN_POINT('Ctrl Pts',(6.91555907373427,-3.84174694265455,95.4719254134196));
#58492=CARTESIAN_POINT('Ctrl Pts',(6.90466663136792,-3.86131094659894,95.4710322894314));
#58493=CARTESIAN_POINT('Ctrl Pts',(6.89737343954427,-3.87432357390493,95.4704386567344));
#58494=CARTESIAN_POINT('Ctrl Pts',(6.8342466184071,-3.98621223752896,95.465337782217));
#58495=CARTESIAN_POINT('Ctrl Pts',(6.77632565822755,-4.08389847780468,95.4609079636657));
#58496=CARTESIAN_POINT('Ctrl Pts',(6.55271971283597,-4.44315659688029,95.4446800500562));
#58497=CARTESIAN_POINT('Ctrl Pts',(6.37382339793422,-4.69618696554919,95.4333921661365));
#58498=CARTESIAN_POINT('Ctrl Pts',(6.12826189041585,-5.0035330466164,95.4195294767092));
#58499=CARTESIAN_POINT('Ctrl Pts',(6.07494189191457,-5.06813753133873,95.4166053423248));
#58500=CARTESIAN_POINT('Ctrl Pts',(5.97789021372658,-5.18199628056737,95.411419967502));
#58501=CARTESIAN_POINT('Ctrl Pts',(5.9345507152443,-5.23157383298663,95.4091508968986));
#58502=CARTESIAN_POINT('Ctrl Pts',(5.8730807791824,-5.30014450562309,95.405991042055));
#58503=CARTESIAN_POINT('Ctrl Pts',(5.85546735330848,-5.31959694890057,95.4050921668097));
#58504=CARTESIAN_POINT('Ctrl Pts',(5.55213582317947,-5.65126742785444,95.3897188542991));
#58505=CARTESIAN_POINT('Ctrl Pts',(5.24192488393845,-5.94013769148073,95.3756480182444));
#58506=CARTESIAN_POINT('Ctrl Pts',(4.80148059006422,-6.28879165578663,95.3558333616111));
#58507=CARTESIAN_POINT('Ctrl Pts',(4.6906124217845,-6.37191251300519,95.3508544034811));
#58508=CARTESIAN_POINT('Ctrl Pts',(4.55278050932077,-6.46970157012527,95.3446047539564));
#58509=CARTESIAN_POINT('Ctrl Pts',(4.52783700989365,-6.48718280547461,95.3434714176188));
#58510=CARTESIAN_POINT('Ctrl Pts',(4.49499273027959,-6.50991945924464,95.3419752280939));
#58511=CARTESIAN_POINT('Ctrl Pts',(4.48718237500114,-6.51530546816884,95.3416191495336));
#58512=CARTESIAN_POINT('Ctrl Pts',(4.46081176082387,-6.53342069296401,95.3404158729057));
#58513=CARTESIAN_POINT('Ctrl Pts',(4.44220698416954,-6.54608467805241,95.3395652384501));
#58514=CARTESIAN_POINT('Ctrl Pts',(4.3333908894268,-6.61947659312442,95.334578603352));
#58515=CARTESIAN_POINT('Ctrl Pts',(4.24199269292435,-6.6784162044943,95.3303445840752));
#58516=CARTESIAN_POINT('Ctrl Pts',(4.14063981682945,-6.74085521857821,95.3255685132271));
#58517=CARTESIAN_POINT('Ctrl Pts',(4.13185652479245,-6.74624257102798,95.3251539613083));
#58518=CARTESIAN_POINT('Ctrl Pts',(4.11951277513632,-6.75378062997216,95.324570410515));
#58519=CARTESIAN_POINT('Ctrl Pts',(4.11596107489648,-6.75594573188014,95.3244023933466));
#58520=CARTESIAN_POINT('Ctrl Pts',(4.10979757449692,-6.75969631210862,95.3241106275984));
#58521=CARTESIAN_POINT('Ctrl Pts',(4.10718656696544,-6.76128307641224,95.3239869680038));
#58522=CARTESIAN_POINT('Ctrl Pts',(4.10173077160193,-6.7645943517686,95.3237284499449));
#58523=CARTESIAN_POINT('Ctrl Pts',(4.09888582659349,-6.76631857417094,95.3235935729748));
#58524=CARTESIAN_POINT('Ctrl Pts',(4.0932252602235,-6.76974436682504,95.3233250680442));
#58525=CARTESIAN_POINT('Ctrl Pts',(4.09040966320588,-6.77144597631699,95.3231914428002));
#58526=CARTESIAN_POINT('Ctrl Pts',(4.08076953315591,-6.77726379409537,95.3227336974347));
#58527=CARTESIAN_POINT('Ctrl Pts',(4.07393986171649,-6.78137143354564,95.3224089991073));
#58528=CARTESIAN_POINT('Ctrl Pts',(4.01934903745053,-6.81409232130996,95.3198104914728));
#58529=CARTESIAN_POINT('Ctrl Pts',(3.97129431555447,-6.84221031664508,95.3175039705246));
#58530=CARTESIAN_POINT('Ctrl Pts',(3.88357842027876,-6.8922996915149,95.3132654707816));
#58531=CARTESIAN_POINT('Ctrl Pts',(3.84401702244457,-6.91444208687771,95.3113435409427));
#58532=CARTESIAN_POINT('Ctrl Pts',(3.63155808427749,-7.03096782006894,95.3009769505302));
#58533=CARTESIAN_POINT('Ctrl Pts',(3.45537899008134,-7.11920432783974,95.2922232941175));
#58534=CARTESIAN_POINT('Ctrl Pts',(3.11123331981325,-7.27577873463573,95.2750923021324));
#58535=CARTESIAN_POINT('Ctrl Pts',(2.9438407174519,-7.34510232297456,95.2667461559348));
#58536=CARTESIAN_POINT('Ctrl Pts',(2.06707970768347,-7.6734129808907,95.2234325262404));
#58537=CARTESIAN_POINT('Ctrl Pts',(1.32550737130842,-7.83565855316587,95.1886640535721));
#58538=CARTESIAN_POINT('Ctrl Pts',(0.521653668279351,-7.89394435891763,
95.1557175455155));
#58539=CARTESIAN_POINT('Ctrl Pts',(0.471164131292514,-7.89711875185553,
95.1536652463703));
#58540=CARTESIAN_POINT('Ctrl Pts',(0.409399090820432,-7.90040760074296,
95.1511750679712));
#58541=CARTESIAN_POINT('Ctrl Pts',(0.398149916969068,-7.90098250336392,
95.150722363599));
#58542=CARTESIAN_POINT('Ctrl Pts',(0.379591352055105,-7.90189122570356,
95.1499768633924));
#58543=CARTESIAN_POINT('Ctrl Pts',(0.372282675856617,-7.90223893254604,
95.1496836202885));
#58544=CARTESIAN_POINT('Ctrl Pts',(0.359106631340507,-7.90284745652252,
95.1491555870889));
#58545=CARTESIAN_POINT('Ctrl Pts',(0.35323943976293,-7.90311188027419,95.1489206809553));
#58546=CARTESIAN_POINT('Ctrl Pts',(0.340721676997566,-7.90366206580223,
95.1484199785691));
#58547=CARTESIAN_POINT('Ctrl Pts',(0.334071026284338,-7.90394596775951,
95.1481542424011));
#58548=CARTESIAN_POINT('Ctrl Pts',(0.31615561358695,-7.90468808571513,95.1474391729731));
#58549=CARTESIAN_POINT('Ctrl Pts',(0.304890197781676,-7.90513061708256,
95.1469903451119));
#58550=CARTESIAN_POINT('Ctrl Pts',(0.250163444438829,-7.90716325004988,
95.1448139015453));
#58551=CARTESIAN_POINT('Ctrl Pts',(0.20669004047878,-7.90841904034461,95.1430970606715));
#58552=CARTESIAN_POINT('Ctrl Pts',(-0.140689022857492,-7.91558717594761,
95.1294719355703));
#58553=CARTESIAN_POINT('Ctrl Pts',(-0.444706584661031,-7.90433876599977,
95.1181337303915));
#58554=CARTESIAN_POINT('Ctrl Pts',(-0.835557652057764,-7.86724958881508,
95.1040209634873));
#58555=CARTESIAN_POINT('Ctrl Pts',(-0.923625238184442,-7.85739711939494,
95.1008705287899));
#58556=CARTESIAN_POINT('Ctrl Pts',(-1.07937530838483,-7.83731792219948,
95.0953362966764));
#58557=CARTESIAN_POINT('Ctrl Pts',(-1.14712488797719,-7.8276885414694,95.0929415519603));
#58558=CARTESIAN_POINT('Ctrl Pts',(-1.26982234701836,-7.80862211688347,
95.0886195023416));
#58559=CARTESIAN_POINT('Ctrl Pts',(-1.32481141386337,-7.79948093997826,
95.0866879634762));
#58560=CARTESIAN_POINT('Ctrl Pts',(-1.4257120843574,-7.78160970646244,95.0831490827152));
#58561=CARTESIAN_POINT('Ctrl Pts',(-1.47165165390885,-7.77305255389568,
95.0815398910726));
#58562=CARTESIAN_POINT('Ctrl Pts',(-1.55664063001131,-7.75644122129672,
95.0785636718615));
#58563=CARTESIAN_POINT('Ctrl Pts',(-1.59571011310113,-7.74849790060409,
95.0771958202496));
#58564=CARTESIAN_POINT('Ctrl Pts',(-1.66839039044674,-7.73314805965238,
95.0746498727215));
#58565=CARTESIAN_POINT('Ctrl Pts',(-1.70201610058914,-7.72581688913321,
95.073471439474));
#58566=CARTESIAN_POINT('Ctrl Pts',(-1.76481763856816,-7.71169481851153,
95.0712681943196));
#58567=CARTESIAN_POINT('Ctrl Pts',(-1.79400479677381,-7.70495717451094,
95.070243286642));
#58568=CARTESIAN_POINT('Ctrl Pts',(-2.05607277280654,-7.6428908369447,95.0610279870779));
#58569=CARTESIAN_POINT('Ctrl Pts',(-2.28636442937645,-7.57718607263496,
95.0528430246915));
#58570=CARTESIAN_POINT('Ctrl Pts',(-2.5985746387371,-7.47257757876964,95.0412541892609));
#58571=CARTESIAN_POINT('Ctrl Pts',(-2.68333735706123,-7.44256044172943,
95.0380561930982));
#58572=CARTESIAN_POINT('Ctrl Pts',(-2.8208036564316,-7.39122567103771,95.0327591034406));
#58573=CARTESIAN_POINT('Ctrl Pts',(-2.87382234159582,-7.37077303711419,
95.030688828321));
#58574=CARTESIAN_POINT('Ctrl Pts',(-3.02771963097993,-7.30949230095951,
95.0245876584046));
#58575=CARTESIAN_POINT('Ctrl Pts',(-3.1279791622638,-7.26715271925829,95.0204969962022));
#58576=CARTESIAN_POINT('Ctrl Pts',(-3.29685533113464,-7.19169415343764,
95.0133577850994));
#58577=CARTESIAN_POINT('Ctrl Pts',(-3.36592649425091,-7.15962694649186,
95.0103654147929));
#58578=CARTESIAN_POINT('Ctrl Pts',(-3.44317354892224,-7.12239911465496,
95.0069251974037));
#58579=CARTESIAN_POINT('Ctrl Pts',(-3.45181759066862,-7.11821385992573,
95.0065389007169));
#58580=CARTESIAN_POINT('Ctrl Pts',(-3.46439729215422,-7.11209474285413,
95.0059747497932));
#58581=CARTESIAN_POINT('Ctrl Pts',(-3.46833902625495,-7.11017331912517,
95.0057976956941));
#58582=CARTESIAN_POINT('Ctrl Pts',(-3.47532836852941,-7.10675912404705,
95.0054832510523));
#58583=CARTESIAN_POINT('Ctrl Pts',(-3.47837662203386,-7.10526766501806,
95.0053459442695));
#58584=CARTESIAN_POINT('Ctrl Pts',(-3.48471077716072,-7.10216341672086,
95.005060277344));
#58585=CARTESIAN_POINT('Ctrl Pts',(-3.48799652032283,-7.10055030771549,
95.0049118969289));
#58586=CARTESIAN_POINT('Ctrl Pts',(-3.49464347753956,-7.09728131080127,
95.004611334652));
#58587=CARTESIAN_POINT('Ctrl Pts',(-3.49800463687692,-7.09562531423809,
95.0044591459555));
#58588=CARTESIAN_POINT('Ctrl Pts',(-3.51171456280598,-7.08885851507637,
95.0038375518356));
#58589=CARTESIAN_POINT('Ctrl Pts',(-3.52205326952894,-7.08372747791444,
95.003366880561));
#58590=CARTESIAN_POINT('Ctrl Pts',(-3.54670056530895,-7.07142787736745,
95.0022402792389));
#58591=CARTESIAN_POINT('Ctrl Pts',(-3.56099865858581,-7.06423850612756,
95.0015830760549));
#58592=CARTESIAN_POINT('Ctrl Pts',(-3.61213601179585,-7.03833090575854,
94.9992197514299));
#58593=CARTESIAN_POINT('Ctrl Pts',(-3.64884979673683,-7.01936774610433,
94.9974991058404));
#58594=CARTESIAN_POINT('Ctrl Pts',(-3.82474630719198,-6.92676198961938,
94.9891463181309));
#58595=CARTESIAN_POINT('Ctrl Pts',(-3.96185200239226,-6.84926563281959,
94.9823052165882));
#58596=CARTESIAN_POINT('Ctrl Pts',(-4.24703799965829,-6.67664098756959,
94.9675123647928));
#58597=CARTESIAN_POINT('Ctrl Pts',(-4.39444466433054,-6.58055611967386,
94.9595287808172));
#58598=CARTESIAN_POINT('Ctrl Pts',(-5.22817358315865,-5.99658921201034,
94.912881515185));
#58599=CARTESIAN_POINT('Ctrl Pts',(-5.83648164011667,-5.40638005550013,
94.8735945380329));
#58600=CARTESIAN_POINT('Ctrl Pts',(-6.35351839553867,-4.71351426008008,
94.838188725876));
#58601=CARTESIAN_POINT('Ctrl Pts',(-6.36670511139438,-4.6956872465497,94.837283488634));
#58602=CARTESIAN_POINT('Ctrl Pts',(-6.39796056288868,-4.653059549026,94.8351324641867));
#58603=CARTESIAN_POINT('Ctrl Pts',(-6.4159603599717,-4.62820864026608,94.8338893336724));
#58604=CARTESIAN_POINT('Ctrl Pts',(-6.44150492378747,-4.592505847453,94.8321187169016));
#58605=CARTESIAN_POINT('Ctrl Pts',(-6.44916767898572,-4.58173895945378,
94.8315867354146));
#58606=CARTESIAN_POINT('Ctrl Pts',(-6.46141661383981,-4.56443644798761,
94.8307349989255));
#58607=CARTESIAN_POINT('Ctrl Pts',(-6.46601992554832,-4.5579130167451,94.8304145939304));
#58608=CARTESIAN_POINT('Ctrl Pts',(-6.47416422596977,-4.54633442105535,
94.8298471689599));
#58609=CARTESIAN_POINT('Ctrl Pts',(-6.47770918566968,-4.54128206556374,
94.8295999987868));
#58610=CARTESIAN_POINT('Ctrl Pts',(-6.48506212336788,-4.53077636785321,
94.8290869270475));
#58611=CARTESIAN_POINT('Ctrl Pts',(-6.48886914460541,-4.52532236021936,
94.8288210617022));
#58612=CARTESIAN_POINT('Ctrl Pts',(-6.49867150071204,-4.51124152442456,
94.8281359380797));
#58613=CARTESIAN_POINT('Ctrl Pts',(-6.50465654649882,-4.50260753109031,
94.827717067546));
#58614=CARTESIAN_POINT('Ctrl Pts',(-6.5295641324309,-4.46652267986299,94.8259715463715));
#58615=CARTESIAN_POINT('Ctrl Pts',(-6.54833036445675,-4.43896407750389,
94.8246507634209));
#58616=CARTESIAN_POINT('Ctrl Pts',(-6.9111097859029,-3.89890764743114,94.7990036478572));
#58617=CARTESIAN_POINT('Ctrl Pts',(-7.1941493870557,-3.34801661001925,94.7772041452471));
#58618=CARTESIAN_POINT('Ctrl Pts',(-7.5166397559977,-2.48522205699581,94.7452885636553));
#58619=CARTESIAN_POINT('Ctrl Pts',(-7.60651665330224,-2.19478873464313,
94.7348434541119));
#58620=CARTESIAN_POINT('Ctrl Pts',(-7.68550613291464,-1.87551284303654,
94.7231039859478));
#58621=CARTESIAN_POINT('Ctrl Pts',(-7.69142704885645,-1.85108154474591,
94.7222040048995));
#58622=CARTESIAN_POINT('Ctrl Pts',(-7.75976796656916,-1.56309875417223,
94.7115720109154));
#58623=CARTESIAN_POINT('Ctrl Pts',(-7.80872562243552,-1.29655632823456,
94.7015029458659));
#58624=CARTESIAN_POINT('Ctrl Pts',(-7.84617868433132,-1.01079375066152,
94.6900007419919));
#58625=CARTESIAN_POINT('Ctrl Pts',(-7.84838359321396,-0.993528518801242,
94.6893030667345));
#58626=CARTESIAN_POINT('Ctrl Pts',(-7.85126729831774,-0.970339302682182,
94.6883621782437));
#58627=CARTESIAN_POINT('Ctrl Pts',(-7.85199641434497,-0.964421516102439,
94.688121733019));
#58628=CARTESIAN_POINT('Ctrl Pts',(-7.85312814531741,-0.955149593307012,
94.6877444744673));
#58629=CARTESIAN_POINT('Ctrl Pts',(-7.8535353045176,-0.951796003879657,
94.6876079137751));
#58630=CARTESIAN_POINT('Ctrl Pts',(-7.85431269415618,-0.945358529794674,
94.6873455642451));
#58631=CARTESIAN_POINT('Ctrl Pts',(-7.85468325563197,-0.942274695110274,
94.6872197942365));
#58632=CARTESIAN_POINT('Ctrl Pts',(-7.85544404598348,-0.935911718842001,
94.6869600974984));
#58633=CARTESIAN_POINT('Ctrl Pts',(-7.85583403745094,-0.932632554122576,
94.6868261578452));
#58634=CARTESIAN_POINT('Ctrl Pts',(-7.8567080606465,-0.925244060060944,
94.6865241354947));
#58635=CARTESIAN_POINT('Ctrl Pts',(-7.85719092152125,-0.921134595786033,
94.6863559879775));
#58636=CARTESIAN_POINT('Ctrl Pts',(-7.8583991339679,-0.910781837859483,
94.6859319747023));
#58637=CARTESIAN_POINT('Ctrl Pts',(-7.85912026847479,-0.904538064512101,
94.6856758775308));
#58638=CARTESIAN_POINT('Ctrl Pts',(-7.86114391800167,-0.886831657786628,
94.6849485780216));
#58639=CARTESIAN_POINT('Ctrl Pts',(-7.86242879718593,-0.875367063256885,
94.6844764211321));
#58640=CARTESIAN_POINT('Ctrl Pts',(-7.89514288584353,-0.577585515755989,
94.6721810951628));
#58641=CARTESIAN_POINT('Ctrl Pts',(-7.91093383073369,-0.289793073497133,
94.6595472812891));
#58642=CARTESIAN_POINT('Ctrl Pts',(-7.91099979248103,-0.00181200581611723,
94.6465781220462));
#58643=CARTESIAN_POINT('',(-7.90011696396554,-0.00322646772645097,92.6423315082368));
#58644=CARTESIAN_POINT('Ctrl Pts',(-7.91859353182819,-0.00199197810995973,
94.6422060731203));
#58645=CARTESIAN_POINT('Ctrl Pts',(-7.90063021708447,2.30671988041081,94.5490207070605));
#58646=CARTESIAN_POINT('Ctrl Pts',(-5.62081845448744,7.26898411856701,94.3499009611984));
#58647=CARTESIAN_POINT('Ctrl Pts',(2.82775288885835,8.91884816508282,94.0448468355335));
#58648=CARTESIAN_POINT('Ctrl Pts',(7.97825124714588,3.53469384178973,93.7800108860271));
#58649=CARTESIAN_POINT('Ctrl Pts',(8.0010321747323,-1.8993409012976,93.568142126422));
#58650=CARTESIAN_POINT('Ctrl Pts',(5.53837391557236,-6.74336473053567,93.3562733668169));
#58651=CARTESIAN_POINT('Ctrl Pts',(-1.48249292472398,-9.23819537141634,
93.0914374173105));
#58652=CARTESIAN_POINT('Ctrl Pts',(-7.18564508454347,-4.8210665441833,92.8358010678166));
#58653=CARTESIAN_POINT('Ctrl Pts',(-7.90503420534493,-1.0943581354185,92.6860990981254));
#58654=CARTESIAN_POINT('Ctrl Pts',(-7.90011696396554,-0.00322646772645097,
92.6423315082368));
#58655=CARTESIAN_POINT('',(-7.91099997228721,-0.000662171981131852,88.6422897498906));
#58656=CARTESIAN_POINT('Ctrl Pts',(-7.91099969560253,-0.00219457893313992,
92.6359954548207));
#58657=CARTESIAN_POINT('Ctrl Pts',(-7.91105851759497,0.209846445081939,
92.6268999841067));
#58658=CARTESIAN_POINT('Ctrl Pts',(-7.9025923153044,0.421815546310325,92.6180528499363));
#58659=CARTESIAN_POINT('Ctrl Pts',(-7.88438988738471,0.648500291604092,
92.6088487635085));
#58660=CARTESIAN_POINT('Ctrl Pts',(-7.88311700052855,0.66379430843469,92.6082290211759));
#58661=CARTESIAN_POINT('Ctrl Pts',(-7.88101772303028,0.688159586406447,
92.6072436550318));
#58662=CARTESIAN_POINT('Ctrl Pts',(-7.88022015914638,0.697233254499654,
92.6068771366448));
#58663=CARTESIAN_POINT('Ctrl Pts',(-7.87882641729278,0.712781566837111,
92.6062498227486));
#58664=CARTESIAN_POINT('Ctrl Pts',(-7.87823792579363,0.719256880884172,
92.6059887887333));
#58665=CARTESIAN_POINT('Ctrl Pts',(-7.87711755418358,0.731418246590784,
92.6054989485463));
#58666=CARTESIAN_POINT('Ctrl Pts',(-7.87658749899853,0.737104459807619,
92.6052700858565));
#58667=CARTESIAN_POINT('Ctrl Pts',(-7.87547113004988,0.748941692255273,
92.604794002735));
#58668=CARTESIAN_POINT('Ctrl Pts',(-7.87488376609128,0.755092609830475,
92.604546815086));
#58669=CARTESIAN_POINT('Ctrl Pts',(-7.87351668311397,0.769233704006001,
92.6039789759759));
#58670=CARTESIAN_POINT('Ctrl Pts',(-7.87273200591303,0.777223400451342,
92.6036584787005));
#58671=CARTESIAN_POINT('Ctrl Pts',(-7.87020481733334,0.802559064060222,
92.6026432118215));
#58672=CARTESIAN_POINT('Ctrl Pts',(-7.86841712478824,0.819900526493182,
92.6019498454834));
#58673=CARTESIAN_POINT('Ctrl Pts',(-7.85288242772919,0.965862732405452,
92.5961267035342));
#58674=CARTESIAN_POINT('Ctrl Pts',(-7.83603969881355,1.09413755258958,92.5910939722459));
#58675=CARTESIAN_POINT('Ctrl Pts',(-7.80584624329514,1.28726711135937,92.5836267029349));
#58676=CARTESIAN_POINT('Ctrl Pts',(-7.79481542313479,1.35245884996004,92.5811250777143));
#58677=CARTESIAN_POINT('Ctrl Pts',(-7.77699466231457,1.45030567744718,92.5773956392605));
#58678=CARTESIAN_POINT('Ctrl Pts',(-7.77081347839506,1.48306791736901,92.5761511793994));
#58679=CARTESIAN_POINT('Ctrl Pts',(-7.6015663204633,2.35001297557888,92.5433254814008));
#58680=CARTESIAN_POINT('Ctrl Pts',(-7.30537456069535,3.15238720903557,92.516238157304));
#58681=CARTESIAN_POINT('Ctrl Pts',(-6.81143773150459,4.02641317570069,92.4788927379328));
#58682=CARTESIAN_POINT('Ctrl Pts',(-6.73168681114499,4.15837408036783,92.4729968154714));
#58683=CARTESIAN_POINT('Ctrl Pts',(-6.63556652386427,4.30740243070224,92.4659427291885));
#58684=CARTESIAN_POINT('Ctrl Pts',(-6.62291139060358,4.32683527358116,92.4650149656115));
#58685=CARTESIAN_POINT('Ctrl Pts',(-6.60666146678254,4.35154984729354,92.4638245350057));
#58686=CARTESIAN_POINT('Ctrl Pts',(-6.6031453634022,4.35688341816635,92.4635670051766));
#58687=CARTESIAN_POINT('Ctrl Pts',(-6.59750073511855,4.36542321667416,92.4631536487802));
#58688=CARTESIAN_POINT('Ctrl Pts',(-6.59537631833245,4.36863216923219,92.4629980941192));
#58689=CARTESIAN_POINT('Ctrl Pts',(-6.59134021137476,4.37471909443704,92.4627025899146));
#58690=CARTESIAN_POINT('Ctrl Pts',(-6.58942898139068,4.37759735887083,92.4625626708715));
#58691=CARTESIAN_POINT('Ctrl Pts',(-6.58506060195004,4.38416668594942,92.4622428948387));
#58692=CARTESIAN_POINT('Ctrl Pts',(-6.58260223660566,4.38785693204065,92.46206295701));
#58693=CARTESIAN_POINT('Ctrl Pts',(-6.57620583053257,4.39744108782498,92.4615948353808));
#58694=CARTESIAN_POINT('Ctrl Pts',(-6.57226297632234,4.4033317630924,92.4613063337003));
#58695=CARTESIAN_POINT('Ctrl Pts',(-6.54807674663601,4.43936144908981,92.4595369950926));
#58696=CARTESIAN_POINT('Ctrl Pts',(-6.52763429067639,4.46936568711325,92.4580431850561));
#58697=CARTESIAN_POINT('Ctrl Pts',(-6.00413677071108,5.22647144726505,92.4198534733533));
#58698=CARTESIAN_POINT('Ctrl Pts',(-5.38292425930104,5.86430720502408,92.3768012509461));
#58699=CARTESIAN_POINT('Ctrl Pts',(-4.54610465492637,6.47611322922637,92.3312036225391));
#58700=CARTESIAN_POINT('Ctrl Pts',(-4.42060228472279,6.56242246675968,92.3246124638779));
#58701=CARTESIAN_POINT('Ctrl Pts',(-4.18949681892611,6.71171571718086,92.3129318597991));
#58702=CARTESIAN_POINT('Ctrl Pts',(-4.08477002398745,6.7759624461401,92.3077998653555));
#58703=CARTESIAN_POINT('Ctrl Pts',(-3.94192354482427,6.85907858193862,92.3010135394244));
#58704=CARTESIAN_POINT('Ctrl Pts',(-3.90508950567532,6.88011600570095,92.2992822670268));
#58705=CARTESIAN_POINT('Ctrl Pts',(-3.84322658782748,6.91479158455034,92.2964053739942));
#58706=CARTESIAN_POINT('Ctrl Pts',(-3.81829022167556,6.92859243051359,92.295253998719));
#58707=CARTESIAN_POINT('Ctrl Pts',(-3.78461970882579,6.94699014281267,92.293710372752));
#58708=CARTESIAN_POINT('Ctrl Pts',(-3.77595090210772,6.95170577416422,92.2933139299413));
#58709=CARTESIAN_POINT('Ctrl Pts',(-3.76224404624432,6.95912878510216,92.2926886268815));
#58710=CARTESIAN_POINT('Ctrl Pts',(-3.75721185951068,6.96184693555287,92.2924593871027));
#58711=CARTESIAN_POINT('Ctrl Pts',(-3.74677648450689,6.96746902413583,92.2919846832596));
#58712=CARTESIAN_POINT('Ctrl Pts',(-3.74137285653161,6.97037214040768,92.291739248224));
#58713=CARTESIAN_POINT('Ctrl Pts',(-3.72905217612777,6.97697301030253,92.2911804907319));
#58714=CARTESIAN_POINT('Ctrl Pts',(-3.72213298526401,6.98066677039058,92.2908673088237));
#58715=CARTESIAN_POINT('Ctrl Pts',(-3.70104726704151,6.99188296554728,92.2899147662972));
#58716=CARTESIAN_POINT('Ctrl Pts',(-3.68686330557181,6.99937263236242,92.2892765561656));
#58717=CARTESIAN_POINT('Ctrl Pts',(-3.58598624415169,7.05224780997988,92.2847555245803));
#58718=CARTESIAN_POINT('Ctrl Pts',(-3.49847871492722,7.09606539169732,92.2809277782003));
#58719=CARTESIAN_POINT('Ctrl Pts',(-3.39661733613499,7.14472795544981,92.2765744928683));
#58720=CARTESIAN_POINT('Ctrl Pts',(-3.38303745771577,7.15116804781961,92.2759961946749));
#58721=CARTESIAN_POINT('Ctrl Pts',(-3.3513091810233,7.16610419373216,92.2746498236176));
#58722=CARTESIAN_POINT('Ctrl Pts',(-3.33314665921872,7.17457008448912,92.2738827409246));
#58723=CARTESIAN_POINT('Ctrl Pts',(-3.28587445936161,7.19638628934921,92.2718955196939));
#58724=CARTESIAN_POINT('Ctrl Pts',(-3.25671542540773,7.20962906489997,92.2706788547085));
#58725=CARTESIAN_POINT('Ctrl Pts',(-2.94408995168285,7.34932643068024,92.2577293056811));
#58726=CARTESIAN_POINT('Ctrl Pts',(-2.65348603731244,7.45917514808436,92.2465377561428));
#58727=CARTESIAN_POINT('Ctrl Pts',(-2.19018988732876,7.60378763692748,92.2295013132248));
#58728=CARTESIAN_POINT('Ctrl Pts',(-2.02153022868916,7.65035522292941,92.2234563463252));
#58729=CARTESIAN_POINT('Ctrl Pts',(-1.80418506162899,7.70267499569685,92.2157628921704));
#58730=CARTESIAN_POINT('Ctrl Pts',(-1.75680216213463,7.71361990225679,92.2140913479165));
#58731=CARTESIAN_POINT('Ctrl Pts',(-1.6554992877257,7.7360378607968,92.210525620853));
#58732=CARTESIAN_POINT('Ctrl Pts',(-1.6015542545544,7.74738560019631,92.2086316207692));
#58733=CARTESIAN_POINT('Ctrl Pts',(-1.48518141744433,7.77059808771909,92.2045497162404));
#58734=CARTESIAN_POINT('Ctrl Pts',(-1.4227204399175,7.78227633726094,92.2023612500642));
#58735=CARTESIAN_POINT('Ctrl Pts',(-1.16967108472931,7.82644034014148,92.1934856010407));
#58736=CARTESIAN_POINT('Ctrl Pts',(-0.978066289309218,7.8526862631623,92.1867446703331));
#58737=CARTESIAN_POINT('Ctrl Pts',(-0.630835780870365,7.88734356043161,
92.1742286322654));
#58738=CARTESIAN_POINT('Ctrl Pts',(-0.475556835398854,7.89822664976303,
92.1685237897499));
#58739=CARTESIAN_POINT('Ctrl Pts',(-0.213602466437318,7.90883352515315,
92.158580021996));
#58740=CARTESIAN_POINT('Ctrl Pts',(-0.107068222776297,7.91099288418527,
92.1544470213325));
#58741=CARTESIAN_POINT('Ctrl Pts',(0.0178117056317007,7.91100120425473,
92.1494661920746));
#58742=CARTESIAN_POINT('Ctrl Pts',(0.0361502868546076,7.91093865840583,
92.1487313178149));
#58743=CARTESIAN_POINT('Ctrl Pts',(0.0602682416766564,7.91077253799182,
92.1477601402533));
#58744=CARTESIAN_POINT('Ctrl Pts',(0.0660480795086562,7.91072639266852,
92.1475270430651));
#58745=CARTESIAN_POINT('Ctrl Pts',(0.0754864062318918,7.91064069394077,
92.1471458133601));
#58746=CARTESIAN_POINT('Ctrl Pts',(0.0791449359376056,7.9106049367408,92.1469978949909));
#58747=CARTESIAN_POINT('Ctrl Pts',(0.0861973944782431,7.91053111550779,
92.1467124761048));
#58748=CARTESIAN_POINT('Ctrl Pts',(0.0895913269889974,7.9104934052366,92.1465749957036));
#58749=CARTESIAN_POINT('Ctrl Pts',(0.0973737452483848,7.91040192502701,
92.1462594589034));
#58750=CARTESIAN_POINT('Ctrl Pts',(0.101762210858887,7.91034668734927,92.146081318644));
#58751=CARTESIAN_POINT('Ctrl Pts',(0.113495557822266,7.9101892339032,92.1456044604224));
#58752=CARTESIAN_POINT('Ctrl Pts',(0.120840329490297,7.91008044029093,92.1453053641667));
#58753=CARTESIAN_POINT('Ctrl Pts',(0.172571573389788,7.90924210938661,92.1431946086891));
#58754=CARTESIAN_POINT('Ctrl Pts',(0.216950567435492,7.90814921434101,92.1413623840763));
#58755=CARTESIAN_POINT('Ctrl Pts',(1.04327903554448,7.88083892319907,92.1068788200323));
#58756=CARTESIAN_POINT('Ctrl Pts',(1.81707851426582,7.73914574533819,92.0689208229441));
#58757=CARTESIAN_POINT('Ctrl Pts',(2.77641978593125,7.41140519833461,92.0231714256398));
#58758=CARTESIAN_POINT('Ctrl Pts',(2.99195000986717,7.32705122680046,92.012943285491));
#58759=CARTESIAN_POINT('Ctrl Pts',(3.335583903202,7.17486403319679,91.9968092227138));
#58760=CARTESIAN_POINT('Ctrl Pts',(3.46605983125185,7.11275095054063,91.9907243895281));
#58761=CARTESIAN_POINT('Ctrl Pts',(3.64105116944718,7.02348681896551,91.9826219832238));
#58762=CARTESIAN_POINT('Ctrl Pts',(3.68710274780054,6.99942098899477,91.9804952591379));
#58763=CARTESIAN_POINT('Ctrl Pts',(3.75233349247625,6.96450999501693,91.9774904057377));
#58764=CARTESIAN_POINT('Ctrl Pts',(3.77170909898301,6.95403599305077,91.9765988295734));
#58765=CARTESIAN_POINT('Ctrl Pts',(3.80571597703659,6.93546872687078,91.9750356361475));
#58766=CARTESIAN_POINT('Ctrl Pts',(3.8203657573067,6.92740976442581,91.9743627704967));
#58767=CARTESIAN_POINT('Ctrl Pts',(3.8417791514485,6.91554149754192,91.9733800240035));
#58768=CARTESIAN_POINT('Ctrl Pts',(3.84856283499525,6.91176861290071,91.9730688074556));
#58769=CARTESIAN_POINT('Ctrl Pts',(3.8602224921159,6.90526136817879,91.9725340882551));
#58770=CARTESIAN_POINT('Ctrl Pts',(3.86510113403027,6.90253181632539,91.9723104090511));
#58771=CARTESIAN_POINT('Ctrl Pts',(3.87478876125025,6.89709819372525,91.9718663591969));
#58772=CARTESIAN_POINT('Ctrl Pts',(3.879597818738,6.89439425933837,91.9716459837322));
#58773=CARTESIAN_POINT('Ctrl Pts',(3.89090152200664,6.88802308176808,91.9711281218101));
#58774=CARTESIAN_POINT('Ctrl Pts',(3.89739382351398,6.8843516770843,91.9708307889606));
#58775=CARTESIAN_POINT('Ctrl Pts',(3.91649264885619,6.87351559159765,91.9699564018111));
#58776=CARTESIAN_POINT('Ctrl Pts',(3.92908470926034,6.86632540787878,91.9693802896286));
#58777=CARTESIAN_POINT('Ctrl Pts',(4.03575050220723,6.80502874669055,91.9645032485918));
#58778=CARTESIAN_POINT('Ctrl Pts',(4.12872354670779,6.74902521993854,91.9602732473172));
#58779=CARTESIAN_POINT('Ctrl Pts',(4.23101653106929,6.68450253966849,91.9556354516165));
#58780=CARTESIAN_POINT('Ctrl Pts',(4.24150009486671,6.67785534703741,91.9551603338924));
#58781=CARTESIAN_POINT('Ctrl Pts',(4.25929448415285,6.66651385509158,91.9543541897186));
#58782=CARTESIAN_POINT('Ctrl Pts',(4.26661328583846,6.66183214683053,91.9540227111495));
#58783=CARTESIAN_POINT('Ctrl Pts',(4.28141078327883,6.65233206115481,91.9533526798065));
#58784=CARTESIAN_POINT('Ctrl Pts',(4.28888909376237,6.6475131055954,91.9530141485019));
#58785=CARTESIAN_POINT('Ctrl Pts',(4.73030618450376,6.3620129802022,91.9330367479649));
#58786=CARTESIAN_POINT('Ctrl Pts',(5.13572487761194,6.03948529488066,91.9150848828523));
#58787=CARTESIAN_POINT('Ctrl Pts',(5.58580309405722,5.60310937385431,91.8936207349291));
#58788=CARTESIAN_POINT('Ctrl Pts',(5.66320286701521,5.52486779076524,91.8898618441282));
#58789=CARTESIAN_POINT('Ctrl Pts',(5.78497962464739,5.39651786250108,91.8837979753463));
#58790=CARTESIAN_POINT('Ctrl Pts',(5.83039679853534,5.34741689065184,91.8815012044588));
#58791=CARTESIAN_POINT('Ctrl Pts',(5.93820070393985,5.22786265966529,91.8759495718037));
#58792=CARTESIAN_POINT('Ctrl Pts',(5.99996322696375,5.1568611102235,91.8726856574339));
#58793=CARTESIAN_POINT('Ctrl Pts',(6.21340168416049,4.9024680155054,91.8610459156392));
#58794=CARTESIAN_POINT('Ctrl Pts',(6.35804763520046,4.71336089429345,91.8524927759235));
#58795=CARTESIAN_POINT('Ctrl Pts',(6.55149008387126,4.43531874509479,91.8396254038887));
#58796=CARTESIAN_POINT('Ctrl Pts',(6.60745030550028,4.35151394614097,91.835711093587));
#58797=CARTESIAN_POINT('Ctrl Pts',(6.67123673038275,4.25192052190159,91.8309895518037));
#58798=CARTESIAN_POINT('Ctrl Pts',(6.68063197414507,4.23714338370838,91.8302872203552));
#58799=CARTESIAN_POINT('Ctrl Pts',(6.69295003746793,4.21762632333132,91.829357108169));
#58800=CARTESIAN_POINT('Ctrl Pts',(6.69591708820335,4.21291423540735,91.8291323557244));
#58801=CARTESIAN_POINT('Ctrl Pts',(6.70076065163518,4.20520394274539,91.8287642783993));
#58802=CARTESIAN_POINT('Ctrl Pts',(6.70264013738476,4.2022075983015,91.82862115881));
#58803=CARTESIAN_POINT('Ctrl Pts',(6.70626469944769,4.19642057165022,91.8283445889791));
#58804=CARTESIAN_POINT('Ctrl Pts',(6.70801004464978,4.19363005928078,91.8282111574633));
#58805=CARTESIAN_POINT('Ctrl Pts',(6.71203957803949,4.18717856355431,91.8279025108358));
#58806=CARTESIAN_POINT('Ctrl Pts',(6.71432250580529,4.18351681103088,91.8277272092351));
#58807=CARTESIAN_POINT('Ctrl Pts',(6.72045992298259,4.17365460075944,91.8272547518482));
#58808=CARTESIAN_POINT('Ctrl Pts',(6.72430881778806,4.16745068658818,91.8269572112453));
#58809=CARTESIAN_POINT('Ctrl Pts',(6.75166185439961,4.12322462810395,91.8248337779397));
#58810=CARTESIAN_POINT('Ctrl Pts',(6.77485151406607,4.08500990672952,91.8229866366889));
#58811=CARTESIAN_POINT('Ctrl Pts',(7.1739823285814,3.41452683702469,91.7903935004589));
#58812=CARTESIAN_POINT('Ctrl Pts',(7.46024472898376,2.73308460483765,91.7547431644953));
#58813=CARTESIAN_POINT('Ctrl Pts',(7.7341648173293,1.69694305319584,91.705450632146));
#58814=CARTESIAN_POINT('Ctrl Pts',(7.79928497369899,1.36678738881675,91.6903604151424));
#58815=CARTESIAN_POINT('Ctrl Pts',(7.86861384634824,0.840634469668327,91.6675578410158));
#58816=CARTESIAN_POINT('Ctrl Pts',(7.88690344147466,0.64692473099016,91.6594195857258));
#58817=CARTESIAN_POINT('Ctrl Pts',(7.89931258540803,0.430441597255867,91.6506034591018));
#58818=CARTESIAN_POINT('Ctrl Pts',(7.900495719312,0.408150328583057,91.6496989164236));
#58819=CARTESIAN_POINT('Ctrl Pts',(7.90239526889608,0.369251048749467,91.648126065074));
#58820=CARTESIAN_POINT('Ctrl Pts',(7.90315371397624,0.352645290101455,91.647456413518));
#58821=CARTESIAN_POINT('Ctrl Pts',(7.90419787802373,0.328085728384394,91.6464686287293));
#58822=CARTESIAN_POINT('Ctrl Pts',(7.90452394071199,0.320133739749633,91.6461492053482));
#58823=CARTESIAN_POINT('Ctrl Pts',(7.9050756390237,0.306164016452225,91.6455887643589));
#58824=CARTESIAN_POINT('Ctrl Pts',(7.90530640416391,0.300146497812528,91.6453475829545));
#58825=CARTESIAN_POINT('Ctrl Pts',(7.90573816802365,0.288541638690467,91.6448829054079));
#58826=CARTESIAN_POINT('Ctrl Pts',(7.90594011493599,0.282954338737594,91.6446593791277));
#58827=CARTESIAN_POINT('Ctrl Pts',(7.90640368717738,0.269740554815243,91.6441312141144));
#58828=CARTESIAN_POINT('Ctrl Pts',(7.90666020140344,0.262113890338347,91.6438267387128));
#58829=CARTESIAN_POINT('Ctrl Pts',(7.90751703773239,0.235491988386449,91.6427652049478));
#58830=CARTESIAN_POINT('Ctrl Pts',(7.90805994820152,0.216494897966537,91.6420099786938));
#58831=CARTESIAN_POINT('Ctrl Pts',(7.91368255097154,-0.00865679662528287,
91.633085678986));
#58832=CARTESIAN_POINT('Ctrl Pts',(7.91076830002816,-0.214939291528602,
91.6251763070342));
#58833=CARTESIAN_POINT('Ctrl Pts',(7.87282463497009,-0.927126694883613,
91.5985888920336));
#58834=CARTESIAN_POINT('Ctrl Pts',(7.79725179328093,-1.4296240408593,91.5811707702051));
#58835=CARTESIAN_POINT('Ctrl Pts',(7.59019735496319,-2.25658963339416,91.5518199338051));
#58836=CARTESIAN_POINT('Ctrl Pts',(7.48441898664359,-2.58587376219204,91.5399085395635));
#58837=CARTESIAN_POINT('Ctrl Pts',(7.3298239755355,-2.97712254262954,91.5244786569774));
#58838=CARTESIAN_POINT('Ctrl Pts',(7.30118833010489,-3.04667469000373,91.5216841877781));
#58839=CARTESIAN_POINT('Ctrl Pts',(7.22497729860908,-3.22453346722947,91.5143811006636));
#58840=CARTESIAN_POINT('Ctrl Pts',(7.1759572205056,-3.33219915739021,91.5098057939485));
#58841=CARTESIAN_POINT('Ctrl Pts',(7.11488044280174,-3.45874125915353,91.5042094169378));
#58842=CARTESIAN_POINT('Ctrl Pts',(7.10513688919724,-3.47871306425574,91.503319889227));
#58843=CARTESIAN_POINT('Ctrl Pts',(7.09209717134167,-3.50515783790371,91.5021339741567));
#58844=CARTESIAN_POINT('Ctrl Pts',(7.08887598570677,-3.51166783951926,91.5018413808267));
#58845=CARTESIAN_POINT('Ctrl Pts',(7.08357099117738,-3.52235216584513,91.5013601097756));
#58846=CARTESIAN_POINT('Ctrl Pts',(7.08149244213387,-3.52652910935761,91.501171694133));
#58847=CARTESIAN_POINT('Ctrl Pts',(7.07745693809509,-3.53462069302065,91.500806180636));
#58848=CARTESIAN_POINT('Ctrl Pts',(7.075500426787,-3.538535553664,91.5006291046928));
#58849=CARTESIAN_POINT('Ctrl Pts',(7.07097514305463,-3.547571613319,91.5002198515517));
#58850=CARTESIAN_POINT('Ctrl Pts',(7.06840405592205,-3.55269164540033,91.4999875613087));
#58851=CARTESIAN_POINT('Ctrl Pts',(7.06036317761945,-3.56866087264581,91.499261820975));
#58852=CARTESIAN_POINT('Ctrl Pts',(7.05487396970901,-3.57950022950289,91.4987674343322));
#58853=CARTESIAN_POINT('Ctrl Pts',(7.00760921971471,-3.67230131523403,91.4945197303969));
#58854=CARTESIAN_POINT('Ctrl Pts',(6.96443297884162,-3.75353917035897,91.4907008136383));
#58855=CARTESIAN_POINT('Ctrl Pts',(6.60878412099147,-4.39543667205015,91.459816050411));
#58856=CARTESIAN_POINT('Ctrl Pts',(6.23055008895123,-4.91692655628546,91.4305803681068));
#58857=CARTESIAN_POINT('Ctrl Pts',(5.51647024023934,-5.68488768762701,91.3847582652302));
#58858=CARTESIAN_POINT('Ctrl Pts',(5.21689485469562,-5.96099344088897,91.3674743386727));
#58859=CARTESIAN_POINT('Ctrl Pts',(4.84815191393325,-6.25166177674386,91.3483116490339));
#58860=CARTESIAN_POINT('Ctrl Pts',(4.79845288858413,-6.28988886905801,91.3457685847753));
#58861=CARTESIAN_POINT('Ctrl Pts',(4.73444271552863,-6.33792343860169,91.342542078425));
#58862=CARTESIAN_POINT('Ctrl Pts',(4.72054707528075,-6.34827981846333,91.3418445486037));
#58863=CARTESIAN_POINT('Ctrl Pts',(4.69819923135228,-6.36482165318867,91.3407273299827));
#58864=CARTESIAN_POINT('Ctrl Pts',(4.68976860495549,-6.37103611095264,91.3403069071088));
#58865=CARTESIAN_POINT('Ctrl Pts',(4.67393470523936,-6.38265927594394,91.3395192356602));
#58866=CARTESIAN_POINT('Ctrl Pts',(4.66653432099559,-6.38807189166788,91.339151888711));
#58867=CARTESIAN_POINT('Ctrl Pts',(4.64997430251653,-6.40013969970884,91.3383316309322));
#58868=CARTESIAN_POINT('Ctrl Pts',(4.64080974879188,-6.40678812403415,91.3378788904879));
#58869=CARTESIAN_POINT('Ctrl Pts',(4.61444776255602,-6.42582618029135,91.3365800169426));
#58870=CARTESIAN_POINT('Ctrl Pts',(4.59721472988969,-6.43816643042406,91.3357351266424));
#58871=CARTESIAN_POINT('Ctrl Pts',(4.49652401020729,-6.50965874207843,91.330822795498));
#58872=CARTESIAN_POINT('Ctrl Pts',(4.41197376671182,-6.56725766600531,91.3267948257203));
#58873=CARTESIAN_POINT('Ctrl Pts',(3.77404644271607,-6.98395695642861,91.2970933059629));
#58874=CARTESIAN_POINT('Ctrl Pts',(3.1788284885799,-7.27421179263632,91.2734690803399));
#58875=CARTESIAN_POINT('Ctrl Pts',(2.23527777216359,-7.59613087496458,91.2373270311647));
#58876=CARTESIAN_POINT('Ctrl Pts',(1.909453578009,-7.68450614308912,91.2250007442387));
#58877=CARTESIAN_POINT('Ctrl Pts',(1.48294763486537,-7.77138322814377,91.2081570835866));
#58878=CARTESIAN_POINT('Ctrl Pts',(1.38653695802092,-7.78916203181984,91.2043028896633));
#58879=CARTESIAN_POINT('Ctrl Pts',(1.27869868732133,-7.80698263169832,91.1999184965402));
#58880=CARTESIAN_POINT('Ctrl Pts',(1.2675698495,-7.80879727098547,91.1994651616009));
#58881=CARTESIAN_POINT('Ctrl Pts',(1.25097549686911,-7.81146669380853,91.1987878495902));
#58882=CARTESIAN_POINT('Ctrl Pts',(1.24551287279229,-7.81233955263828,91.1985646720871));
#58883=CARTESIAN_POINT('Ctrl Pts',(1.23616721465634,-7.81382282036077,91.1981824762726));
#58884=CARTESIAN_POINT('Ctrl Pts',(1.23228462708304,-7.81443606720079,91.1980235848994));
#58885=CARTESIAN_POINT('Ctrl Pts',(1.22433433591922,-7.81568572712306,91.1976979969782));
#58886=CARTESIAN_POINT('Ctrl Pts',(1.22026658941661,-7.81632185890083,91.1975312877873));
#58887=CARTESIAN_POINT('Ctrl Pts',(1.21054963936562,-7.81783366739128,91.1971327591652));
#58888=CARTESIAN_POINT('Ctrl Pts',(1.2048999854946,-7.81870639588479,91.1969008058573));
#58889=CARTESIAN_POINT('Ctrl Pts',(1.18466586919018,-7.82180960265599,91.1960691975298));
#58890=CARTESIAN_POINT('Ctrl Pts',(1.17007618469181,-7.82400539361137,91.1954679488935));
#58891=CARTESIAN_POINT('Ctrl Pts',(0.950260351221596,-7.85645973934033,
91.1863837841669));
#58892=CARTESIAN_POINT('Ctrl Pts',(0.743962456177103,-7.87867050852365,
91.1774839310529));
#58893=CARTESIAN_POINT('Ctrl Pts',(-0.0211807592265673,-7.93073417279431,
91.1435842264521));
#58894=CARTESIAN_POINT('Ctrl Pts',(-0.581868266284063,-7.90938929797473,
91.1171747745959));
#58895=CARTESIAN_POINT('Ctrl Pts',(-1.42690149520752,-7.78681611606584,
91.0784354972897));
#58896=CARTESIAN_POINT('Ctrl Pts',(-1.71561666175553,-7.7283396430826,91.0653695573615));
#58897=CARTESIAN_POINT('Ctrl Pts',(-2.17775769513064,-7.60755477159421,
91.0449413266898));
#58898=CARTESIAN_POINT('Ctrl Pts',(-2.35343855390713,-7.55505467615469,
91.0372903870975));
#58899=CARTESIAN_POINT('Ctrl Pts',(-2.55782757103749,-7.48615305007275,
91.0285260113585));
#58900=CARTESIAN_POINT('Ctrl Pts',(-2.58844609119514,-7.47562146168603,
91.0272166719071));
#58901=CARTESIAN_POINT('Ctrl Pts',(-2.62861482409304,-7.4615285930385,91.0255035929168));
#58902=CARTESIAN_POINT('Ctrl Pts',(-2.63822380687272,-7.45813649540232,
91.0250941492467));
#58903=CARTESIAN_POINT('Ctrl Pts',(-2.65390254353873,-7.45256760243809,
91.0244266397378));
#58904=CARTESIAN_POINT('Ctrl Pts',(-2.65997622278917,-7.4504019404303,91.024168197514));
#58905=CARTESIAN_POINT('Ctrl Pts',(-2.67167846343614,-7.44621319607253,
91.0236705213851));
#58906=CARTESIAN_POINT('Ctrl Pts',(-2.67730739033785,-7.44419115224769,
91.023431252509));
#58907=CARTESIAN_POINT('Ctrl Pts',(-2.6902092902807,-7.43953995774249,91.0228831043623));
#58908=CARTESIAN_POINT('Ctrl Pts',(-2.69748071736787,-7.43690652006835,
91.0225743708268));
#58909=CARTESIAN_POINT('Ctrl Pts',(-2.72039117645356,-7.42857119082878,
91.0216022519872));
#58910=CARTESIAN_POINT('Ctrl Pts',(-2.73601612791031,-7.42283058154975,
91.0209401834845));
#58911=CARTESIAN_POINT('Ctrl Pts',(-2.86293482521028,-7.37574544205321,
91.0155696615044));
#58912=CARTESIAN_POINT('Ctrl Pts',(-2.97330574376928,-7.33194865922051,
91.0109456749634));
#58913=CARTESIAN_POINT('Ctrl Pts',(-3.89287881950393,-6.94286721201783,
90.9727458628391));
#58914=CARTESIAN_POINT('Ctrl Pts',(-4.64012222742711,-6.4673785988233,90.9447268046663));
#58915=CARTESIAN_POINT('Ctrl Pts',(-5.53760730902066,-5.65919302882644,
90.9023808821957));
#58916=CARTESIAN_POINT('Ctrl Pts',(-5.76749474851314,-5.42471420250105,
90.8904188083037));
#58917=CARTESIAN_POINT('Ctrl Pts',(-5.99121335698095,-5.16618580200786,
90.8767360084477));
#58918=CARTESIAN_POINT('Ctrl Pts',(-6.00025827479084,-5.15567782749045,
90.8761790589719));
#58919=CARTESIAN_POINT('Ctrl Pts',(-6.01257076010891,-5.14129745554785,
90.8754156805187));
#58920=CARTESIAN_POINT('Ctrl Pts',(-6.01586234700275,-5.13744556111512,
90.8752110883139));
#58921=CARTESIAN_POINT('Ctrl Pts',(-6.02136729150627,-5.13099099723098,
90.8748680582291));
#58922=CARTESIAN_POINT('Ctrl Pts',(-6.02358266247359,-5.12839005743327,
90.874729776476));
#58923=CARTESIAN_POINT('Ctrl Pts',(-6.02794872438443,-5.12325738288254,
90.8744567857774));
#58924=CARTESIAN_POINT('Ctrl Pts',(-6.030099496285,-5.12072573957135,90.8743220848618));
#58925=CARTESIAN_POINT('Ctrl Pts',(-6.03482393522903,-5.1151575650319,90.8740257094361));
#58926=CARTESIAN_POINT('Ctrl Pts',(-6.03739690486433,-5.11212044628599,
90.8738639818439));
#58927=CARTESIAN_POINT('Ctrl Pts',(-6.04630310439021,-5.10159151706491,
90.8733030683934));
#58928=CARTESIAN_POINT('Ctrl Pts',(-6.05262466763104,-5.09408989597374,
90.8729030021323));
#58929=CARTESIAN_POINT('Ctrl Pts',(-6.1123303586295,-5.02297079831646,90.8691063050673));
#58930=CARTESIAN_POINT('Ctrl Pts',(-6.16472182029456,-4.95853022560046,
90.8656369133556));
#58931=CARTESIAN_POINT('Ctrl Pts',(-6.66168682937597,-4.32721984900792,
90.8314772691184));
#58932=CARTESIAN_POINT('Ctrl Pts',(-7.02787940775434,-3.7029553723878,90.7967384002758));
#58933=CARTESIAN_POINT('Ctrl Pts',(-7.42290222059974,-2.75308620273604,
90.7501273254391));
#58934=CARTESIAN_POINT('Ctrl Pts',(-7.52454740478917,-2.46174201257003,
90.736525971094));
#58935=CARTESIAN_POINT('Ctrl Pts',(-7.63927991404165,-2.05854710626559,
90.7187897070337));
#58936=CARTESIAN_POINT('Ctrl Pts',(-7.66738063817991,-1.95127888799704,
90.7141707675575));
#58937=CARTESIAN_POINT('Ctrl Pts',(-7.70707720114953,-1.78561454275931,
90.7071886383224));
#58938=CARTESIAN_POINT('Ctrl Pts',(-7.72028382263607,-1.7276215402261,90.7047725877386));
#58939=CARTESIAN_POINT('Ctrl Pts',(-7.73547006985905,-1.65728080406908,
90.7018754753632));
#58940=CARTESIAN_POINT('Ctrl Pts',(-7.73807585209953,-1.64507111526698,
90.7013738077295));
#58941=CARTESIAN_POINT('Ctrl Pts',(-7.74208200362152,-1.62607970295307,
90.7005953669043));
#58942=CARTESIAN_POINT('Ctrl Pts',(-7.74350238436165,-1.61930224938565,
90.7003179354531));
#58943=CARTESIAN_POINT('Ctrl Pts',(-7.74598940520069,-1.6073571403591,90.6998296190175));
#58944=CARTESIAN_POINT('Ctrl Pts',(-7.74705977629082,-1.60219027111887,
90.6996186114533));
#58945=CARTESIAN_POINT('Ctrl Pts',(-7.74931261494286,-1.591260382961,90.6991727023025));
#58946=CARTESIAN_POINT('Ctrl Pts',(-7.75049382527249,-1.58549710662088,
90.6989378421424));
#58947=CARTESIAN_POINT('Ctrl Pts',(-7.75381292697297,-1.56921044017725,
90.6982748897011));
#58948=CARTESIAN_POINT('Ctrl Pts',(-7.7559358260403,-1.55868398836987,90.6978472899915));
#58949=CARTESIAN_POINT('Ctrl Pts',(-7.7646665462295,-1.51493298752023,90.6960737040128));
#58950=CARTESIAN_POINT('Ctrl Pts',(-7.77108240959782,-1.48167025729222,
90.6947340180458));
#58951=CARTESIAN_POINT('Ctrl Pts',(-7.86620710105452,-0.970880000486219,
90.6742925969767));
#58952=CARTESIAN_POINT('Ctrl Pts',(-7.91097364017281,-0.486193375633732,
90.6567465537409));
#58953=CARTESIAN_POINT('Ctrl Pts',(-7.91103644331997,0.671667830417302,
90.6165305979411));
#58954=CARTESIAN_POINT('Ctrl Pts',(-7.82542677478422,1.34093832443821,90.5947062374235));
#58955=CARTESIAN_POINT('Ctrl Pts',(-7.6528318959326,2.00456340857716,90.5684468110225));
#58956=CARTESIAN_POINT('Ctrl Pts',(-7.64933231993946,2.01787649323009,90.5679179769197));
#58957=CARTESIAN_POINT('Ctrl Pts',(-7.62554163487146,2.10742973079592,90.5643465180999));
#58958=CARTESIAN_POINT('Ctrl Pts',(-7.60414636988768,2.18336953185054,90.5612489019157));
#58959=CARTESIAN_POINT('Ctrl Pts',(-7.57884936431733,2.26827190472345,90.5576949780685));
#58960=CARTESIAN_POINT('Ctrl Pts',(-7.57606200183496,2.27756441479243,90.5573047761293));
#58961=CARTESIAN_POINT('Ctrl Pts',(-7.57198488142962,2.29106641952895,90.5567359970455));
#58962=CARTESIAN_POINT('Ctrl Pts',(-7.57070868308965,2.2952800306039,90.5565582389325));
#58963=CARTESIAN_POINT('Ctrl Pts',(-7.56844176523037,2.30274223073878,90.5562429803134));
#58964=CARTESIAN_POINT('Ctrl Pts',(-7.56745246818332,2.30599125684134,90.5561055650138));
#58965=CARTESIAN_POINT('Ctrl Pts',(-7.56539486989071,2.31273318917736,90.5558201049253));
#58966=CARTESIAN_POINT('Ctrl Pts',(-7.56432624142065,2.31622599393089,90.5556720406734));
#58967=CARTESIAN_POINT('Ctrl Pts',(-7.56156834578994,2.32521789208126,90.5552904136801));
#58968=CARTESIAN_POINT('Ctrl Pts',(-7.5598755011901,2.33071587712521,90.555056639499));
#58969=CARTESIAN_POINT('Ctrl Pts',(-7.55282868431633,2.35351393095204,90.5540854848258));
#58970=CARTESIAN_POINT('Ctrl Pts',(-7.54742134946775,2.37079731763974,90.5533449858794));
#58971=CARTESIAN_POINT('Ctrl Pts',(-7.51043400788925,2.4876103962893,90.5483120952514));
#58972=CARTESIAN_POINT('Ctrl Pts',(-7.4769466009413,2.58652126773107,90.543912421778));
#58973=CARTESIAN_POINT('Ctrl Pts',(-7.36003421414467,2.91057731419382,90.529109004484));
#58974=CARTESIAN_POINT('Ctrl Pts',(-7.26832105776938,3.13258042113028,90.5183425129204));
#58975=CARTESIAN_POINT('Ctrl Pts',(-6.79495912436123,4.1452277344965,90.4673535755859));
#58976=CARTESIAN_POINT('Ctrl Pts',(-6.29336779692856,4.8732506367016,90.4260997860459));
#58977=CARTESIAN_POINT('Ctrl Pts',(-5.65041374680111,5.53704437451131,90.388229622283));
#58978=CARTESIAN_POINT('Ctrl Pts',(-5.61813006991555,5.56979806867234,90.386357475511));
#58979=CARTESIAN_POINT('Ctrl Pts',(-5.57126581387673,5.61652257099746,90.3836813445754));
#58980=CARTESIAN_POINT('Ctrl Pts',(-5.55691479424308,5.63072167103939,90.3828673601251));
#58981=CARTESIAN_POINT('Ctrl Pts',(-5.53682053933631,5.65045156433449,90.3817352489327));
#58982=CARTESIAN_POINT('Ctrl Pts',(-5.53112311775544,5.65602878549963,90.3814151055096));
#58983=CARTESIAN_POINT('Ctrl Pts',(-5.52127040598132,5.66564450698911,90.3808629342966));
#58984=CARTESIAN_POINT('Ctrl Pts',(-5.51711909687641,5.66968706778568,90.3806307307921));
#58985=CARTESIAN_POINT('Ctrl Pts',(-5.5085189140592,5.67804356938654,90.380150601091));
#58986=CARTESIAN_POINT('Ctrl Pts',(-5.5040694045107,5.68235685195471,90.3799027033462));
#58987=CARTESIAN_POINT('Ctrl Pts',(-5.49366228086857,5.69242165661466,90.3793240713696));
#58988=CARTESIAN_POINT('Ctrl Pts',(-5.48770069019601,5.69816906631303,90.3789935141765));
#58989=CARTESIAN_POINT('Ctrl Pts',(-5.46852761298895,5.71659531902221,90.3779333033456));
#58990=CARTESIAN_POINT('Ctrl Pts',(-5.45528108309509,5.72923769847399,90.3772052126631));
#58991=CARTESIAN_POINT('Ctrl Pts',(-5.18302412786111,5.98727717112551,90.3623300416581));
#58992=CARTESIAN_POINT('Ctrl Pts',(-4.90773989433601,6.21492951175404,90.3489674283416));
#58993=CARTESIAN_POINT('Ctrl Pts',(-4.47543237032722,6.52573822362952,90.3297955900048));
#58994=CARTESIAN_POINT('Ctrl Pts',(-4.32948553160389,6.6234667292334,90.3235975338785));
#58995=CARTESIAN_POINT('Ctrl Pts',(-3.60488375268019,7.07448101063024,90.2937785234339));
#58996=CARTESIAN_POINT('Ctrl Pts',(-2.98578643850993,7.35719428982956,90.2713672781674));
#58997=CARTESIAN_POINT('Ctrl Pts',(-2.29962520076352,7.56949719673342,90.2430819346046));
#58998=CARTESIAN_POINT('Ctrl Pts',(-2.26081300272504,7.58117987766749,90.2414702183407));
#58999=CARTESIAN_POINT('Ctrl Pts',(-2.21484979615396,7.594630705138,90.2395458848578));
#59000=CARTESIAN_POINT('Ctrl Pts',(-2.20778336582223,7.59668794777799,90.2392495997125));
#59001=CARTESIAN_POINT('Ctrl Pts',(-2.19642239885298,7.59997826374602,90.2387725357218));
#59002=CARTESIAN_POINT('Ctrl Pts',(-2.19212965862894,7.60121756846702,90.2385921131943));
#59003=CARTESIAN_POINT('Ctrl Pts',(-2.18450183122812,7.6034127065301,90.2382712232249));
#59004=CARTESIAN_POINT('Ctrl Pts',(-2.18116715752563,7.60436998490964,90.2381308389686));
#59005=CARTESIAN_POINT('Ctrl Pts',(-2.17418665322266,7.60636889547045,90.2378367603777));
#59006=CARTESIAN_POINT('Ctrl Pts',(-2.17054071202144,7.60741009768743,90.2376830420841));
#59007=CARTESIAN_POINT('Ctrl Pts',(-2.16099352404171,7.6101291466699,90.2372802069598));
#59008=CARTESIAN_POINT('Ctrl Pts',(-2.15509108091983,7.6118027478709,90.2370308471644));
#59009=CARTESIAN_POINT('Ctrl Pts',(-2.12923451257058,7.61910173203166,90.2359371435879));
#59010=CARTESIAN_POINT('Ctrl Pts',(-2.10926041968613,7.6246554859746,90.2350887579614));
#59011=CARTESIAN_POINT('Ctrl Pts',(-1.57481904687058,7.77099499934802,90.2122996744269));
#59012=CARTESIAN_POINT('Ctrl Pts',(-1.04748248265556,7.85946030993799,90.1876925563904));
#59013=CARTESIAN_POINT('Ctrl Pts',(0.148146788967754,7.93750737468365,90.1326662581752));
#59014=CARTESIAN_POINT('Ctrl Pts',(0.814522869031433,7.89701169705485,90.1027043333793));
#59015=CARTESIAN_POINT('Ctrl Pts',(1.51261333030705,7.76517735044155,90.0737061813983));
#59016=CARTESIAN_POINT('Ctrl Pts',(1.55711100278836,7.75637697540344,90.0718668227398));
#59017=CARTESIAN_POINT('Ctrl Pts',(1.61345217296389,7.74472990314489,90.0695491240123));
#59018=CARTESIAN_POINT('Ctrl Pts',(1.625367656162,7.74223799499316,90.0690595964059));
#59019=CARTESIAN_POINT('Ctrl Pts',(1.64422009331379,7.73824990828686,90.0682860779094));
#59020=CARTESIAN_POINT('Ctrl Pts',(1.65116084421602,7.73677188659604,90.0680015130439));
#59021=CARTESIAN_POINT('Ctrl Pts',(1.66405926572821,7.73400704096028,90.067473086985));
#59022=CARTESIAN_POINT('Ctrl Pts',(1.67001745296989,7.73272266775862,90.0672291484178));
#59023=CARTESIAN_POINT('Ctrl Pts',(1.68319129851719,7.72986691912171,90.066690136323));
#59024=CARTESIAN_POINT('Ctrl Pts',(1.69040625678016,7.72829232250906,90.0663951651149));
#59025=CARTESIAN_POINT('Ctrl Pts',(1.71112168067951,7.72374097940484,90.0655489106209));
#59026=CARTESIAN_POINT('Ctrl Pts',(1.72461659252415,7.72073893706344,90.0649984301003));
#59027=CARTESIAN_POINT('Ctrl Pts',(1.81282493550354,7.70087353558119,90.0614054728505));
#59028=CARTESIAN_POINT('Ctrl Pts',(1.88729914355363,7.68296100537467,90.0583964758123));
#59029=CARTESIAN_POINT('Ctrl Pts',(2.1036882192955,7.62757876659699,90.0497195371574));
#59030=CARTESIAN_POINT('Ctrl Pts',(2.24483704377802,7.5872373904524,90.0441434662331));
#59031=CARTESIAN_POINT('Ctrl Pts',(2.709041785495,7.44047476456881,90.0260133967217));
#59032=CARTESIAN_POINT('Ctrl Pts',(3.02636012445742,7.31715346808188,90.0139775561131));
#59033=CARTESIAN_POINT('Ctrl Pts',(3.95750835273183,6.88430489162142,89.9783720468342));
#59034=CARTESIAN_POINT('Ctrl Pts',(4.53981523142303,6.51500952788348,89.9558549705293));
#59035=CARTESIAN_POINT('Ctrl Pts',(5.08029683888361,6.06422315401861,89.9281702659051));
#59036=CARTESIAN_POINT('Ctrl Pts',(5.09350488234076,6.0531336048777,89.9274889880731));
#59037=CARTESIAN_POINT('Ctrl Pts',(5.1268794965567,6.02492550689082,89.9257551925243));
#59038=CARTESIAN_POINT('Ctrl Pts',(5.14699653313801,6.00774894559352,89.9246986555212));
#59039=CARTESIAN_POINT('Ctrl Pts',(5.17216789066655,5.98603762141822,89.9233616716148));
#59040=CARTESIAN_POINT('Ctrl Pts',(5.17730323096243,5.98159663872512,89.9230881169896));
#59041=CARTESIAN_POINT('Ctrl Pts',(5.18536047374489,5.97461067951697,89.922657662781));
#59042=CARTESIAN_POINT('Ctrl Pts',(5.18828624408523,5.97207014893574,89.9225010948829));
#59043=CARTESIAN_POINT('Ctrl Pts',(5.19368778464296,5.96737287059228,89.9222115569459));
#59044=CARTESIAN_POINT('Ctrl Pts',(5.19616408253067,5.96521672769655,89.9220786324132));
#59045=CARTESIAN_POINT('Ctrl Pts',(5.2010317354334,5.96097307185073,89.9218169715996));
#59046=CARTESIAN_POINT('Ctrl Pts',(5.20342317775739,5.95888566004011,89.921688242974));
#59047=CARTESIAN_POINT('Ctrl Pts',(5.21047258017884,5.95272498770904,89.9213082584521));
#59048=CARTESIAN_POINT('Ctrl Pts',(5.21512697752014,5.94864773673067,89.9210566961871));
#59049=CARTESIAN_POINT('Ctrl Pts',(5.23713000864485,5.9293274153709,89.9198642763862));
#59050=CARTESIAN_POINT('Ctrl Pts',(5.25441645215651,5.91401403888302,89.9189180665562));
#59051=CARTESIAN_POINT('Ctrl Pts',(5.38941391052038,5.79336603334328,89.9114566265191));
#59052=CARTESIAN_POINT('Ctrl Pts',(5.50400698401703,5.68460849406302,89.9046916062721));
#59053=CARTESIAN_POINT('Ctrl Pts',(5.69000864861778,5.49717955558866,89.8930946582375));
#59054=CARTESIAN_POINT('Ctrl Pts',(5.76323128031356,5.42036396287902,89.8883578464256));
#59055=CARTESIAN_POINT('Ctrl Pts',(6.47142951840073,4.64683778879506,89.8410212693392));
#59056=CARTESIAN_POINT('Ctrl Pts',(6.97883726939091,3.84307474239805,89.7959439565106));
#59057=CARTESIAN_POINT('Ctrl Pts',(7.35418555031589,2.91601272883977,89.7549702798263));
#59058=CARTESIAN_POINT('Ctrl Pts',(7.37502215974999,2.86290476091524,89.7526530690141));
#59059=CARTESIAN_POINT('Ctrl Pts',(7.39945926455861,2.79858212039492,89.7498820806442));
#59060=CARTESIAN_POINT('Ctrl Pts',(7.40361122110666,2.78757962769762,89.7494093447176));
#59061=CARTESIAN_POINT('Ctrl Pts',(7.41036068272521,2.7695724153076,89.74863767024));
#59062=CARTESIAN_POINT('Ctrl Pts',(7.41297281858815,2.76257322129083,89.7483382294199));
#59063=CARTESIAN_POINT('Ctrl Pts',(7.41762611777935,2.75005062695556,89.7478033768049));
#59064=CARTESIAN_POINT('Ctrl Pts',(7.41967103429557,2.74452863293776,89.7475678363881));
#59065=CARTESIAN_POINT('Ctrl Pts',(7.42398130900293,2.732849349572,89.7470703096822));
#59066=CARTESIAN_POINT('Ctrl Pts',(7.42624517751905,2.7266915130852,89.7468083745672));
#59067=CARTESIAN_POINT('Ctrl Pts',(7.43223113291634,2.71034665971032,89.7461141287476));
#59068=CARTESIAN_POINT('Ctrl Pts',(7.43593994162164,2.70015477606857,89.7456822727326));
#59069=CARTESIAN_POINT('Ctrl Pts',(7.45286779620974,2.65333729223237,89.7437032596434));
#59070=CARTESIAN_POINT('Ctrl Pts',(7.46583739013405,2.61662173320734,89.7421646307633));
#59071=CARTESIAN_POINT('Ctrl Pts',(7.55892542484002,2.34677172473099,89.7309519969572));
#59072=CARTESIAN_POINT('Ctrl Pts',(7.62838192035115,2.11009305165641,89.7216470141069));
#59073=CARTESIAN_POINT('Ctrl Pts',(7.76931143190361,1.53096737910977,89.6998740487694));
#59074=CARTESIAN_POINT('Ctrl Pts',(7.82935615194035,1.18627942710046,89.6877435992011));
#59075=CARTESIAN_POINT('Ctrl Pts',(7.93160570893311,0.227298638090453,89.6546725653809));
#59076=CARTESIAN_POINT('Ctrl Pts',(7.92528001307849,-0.389579946987129,
89.6342296068678));
#59077=CARTESIAN_POINT('Ctrl Pts',(7.84278711280587,-1.0373398129147,89.6084952837222));
#59078=CARTESIAN_POINT('Ctrl Pts',(7.83768079455049,-1.07524102109694,89.6069733389227));
#59079=CARTESIAN_POINT('Ctrl Pts',(7.83123335987005,-1.12060810542224,89.6051305920217));
#59080=CARTESIAN_POINT('Ctrl Pts',(7.83015598830162,-1.12811154624582,89.6048251233334));
#59081=CARTESIAN_POINT('Ctrl Pts',(7.82849628823628,-1.13955373632641,89.6043582387046));
#59082=CARTESIAN_POINT('Ctrl Pts',(7.82792176550284,-1.14349363179619,89.6041972829286));
#59083=CARTESIAN_POINT('Ctrl Pts',(7.82688350789978,-1.15057622319718,89.6039075892593));
#59084=CARTESIAN_POINT('Ctrl Pts',(7.82642085360621,-1.15371907923898,89.6037789155641));
#59085=CARTESIAN_POINT('Ctrl Pts',(7.82551114225162,-1.15987310924376,89.603526715274));
#59086=CARTESIAN_POINT('Ctrl Pts',(7.82506424104106,-1.16288429799642,89.6034031980997));
#59087=CARTESIAN_POINT('Ctrl Pts',(7.82380430391604,-1.17134005241748,89.603056027072));
#59088=CARTESIAN_POINT('Ctrl Pts',(7.8229873241902,-1.17678401995889,89.6028321384201));
#59089=CARTESIAN_POINT('Ctrl Pts',(7.81959827355985,-1.1992075557689,89.6019084213369));
#59090=CARTESIAN_POINT('Ctrl Pts',(7.81697661659254,-1.2161794638618,89.601205672199));
#59091=CARTESIAN_POINT('Ctrl Pts',(7.79905205139171,-1.32976562046447,89.5964789331431));
#59092=CARTESIAN_POINT('Ctrl Pts',(7.78201416038242,-1.42609382709904,89.592356371783));
#59093=CARTESIAN_POINT('Ctrl Pts',(7.71980619048592,-1.74337901838519,89.5784572399857));
#59094=CARTESIAN_POINT('Ctrl Pts',(7.66697650549332,-1.96271165599338,89.5683341494993));
#59095=CARTESIAN_POINT('Ctrl Pts',(7.38383394785498,-2.95068333325408,89.5212675758226));
#59096=CARTESIAN_POINT('Ctrl Pts',(7.04671261031696,-3.68399408740623,89.4828137421131));
#59097=CARTESIAN_POINT('Ctrl Pts',(6.499159546993,-4.51462525144733,89.4403110165798));
#59098=CARTESIAN_POINT('Ctrl Pts',(6.38747391051129,-4.67130603880937,89.4323109147705));
#59099=CARTESIAN_POINT('Ctrl Pts',(6.25879149078323,-4.83857407053081,89.4237802753773));
#59100=CARTESIAN_POINT('Ctrl Pts',(6.24734851250089,-4.85333972959324,89.4230272956891));
#59101=CARTESIAN_POINT('Ctrl Pts',(6.23119189570707,-4.8740358986809,89.4219719498613));
#59102=CARTESIAN_POINT('Ctrl Pts',(6.22652192100375,-4.88000032278956,89.4216678172619));
#59103=CARTESIAN_POINT('Ctrl Pts',(6.21839918837262,-4.89034391759876,89.4211403957451));
#59104=CARTESIAN_POINT('Ctrl Pts',(6.21495035732997,-4.89472615724815,89.4209169477376));
#59105=CARTESIAN_POINT('Ctrl Pts',(6.20776145957406,-4.90384084621998,89.4204521997571));
#59106=CARTESIAN_POINT('Ctrl Pts',(6.20402060733639,-4.90857267319028,89.4202109319286));
#59107=CARTESIAN_POINT('Ctrl Pts',(6.1951942981292,-4.91971091754983,89.4196430163892));
#59108=CARTESIAN_POINT('Ctrl Pts',(6.19010430556414,-4.92611374113469,89.4193165535764));
#59109=CARTESIAN_POINT('Ctrl Pts',(6.17341553080725,-4.9470402415968,89.4182495719807));
#59110=CARTESIAN_POINT('Ctrl Pts',(6.16177545252874,-4.96153098818865,89.4175107382099));
#59111=CARTESIAN_POINT('Ctrl Pts',(5.98032873670946,-5.18579082547538,89.4060761734248));
#59112=CARTESIAN_POINT('Ctrl Pts',(5.79994125966426,-5.38678528454571,89.3958324919353));
#59113=CARTESIAN_POINT('Ctrl Pts',(5.53659318569436,-5.65161775271878,89.3821427094179));
#59114=CARTESIAN_POINT('Ctrl Pts',(5.46212947239637,-5.72361683266199,89.3783982600544));
#59115=CARTESIAN_POINT('Ctrl Pts',(5.06745547971587,-6.09050884676048,89.3591332550095));
#59116=CARTESIAN_POINT('Ctrl Pts',(4.7247156171568,-6.36006826030291,89.3443877444445));
#59117=CARTESIAN_POINT('Ctrl Pts',(4.33896271471279,-6.61498727071398,89.3283719608302));
#59118=CARTESIAN_POINT('Ctrl Pts',(4.31629827732005,-6.62979812715324,89.3274327848463));
#59119=CARTESIAN_POINT('Ctrl Pts',(4.2716612775224,-6.65864179977781,89.3255858970384));
#59120=CARTESIAN_POINT('Ctrl Pts',(4.24969449197723,-6.67268292414749,89.324678320952));
#59121=CARTESIAN_POINT('Ctrl Pts',(3.9025432626319,-6.89217169318522,89.3103506686897));
#59122=CARTESIAN_POINT('Ctrl Pts',(3.56287649826949,-7.07373798187514,89.2965490421296));
#59123=CARTESIAN_POINT('Ctrl Pts',(3.18654451040363,-7.24089723580959,89.2801986917944));
#59124=CARTESIAN_POINT('Ctrl Pts',(3.16166606070507,-7.25179470120666,89.2791135038575));
#59125=CARTESIAN_POINT('Ctrl Pts',(3.12937872866705,-7.26573973753404,89.2777000202331));
#59126=CARTESIAN_POINT('Ctrl Pts',(3.12202042797337,-7.26890456723875,89.2773775431543));
#59127=CARTESIAN_POINT('Ctrl Pts',(3.11023351509155,-7.27395295846982,89.2768604468178));
#59128=CARTESIAN_POINT('Ctrl Pts',(3.10580795564316,-7.27584366949584,89.2766661751491));
#59129=CARTESIAN_POINT('Ctrl Pts',(3.09742654276568,-7.27941538083581,89.276298025907));
#59130=CARTESIAN_POINT('Ctrl Pts',(3.09347103767822,-7.28109719846654,89.2761241876593));
#59131=CARTESIAN_POINT('Ctrl Pts',(3.08463313487316,-7.28484643182711,89.2757355671302));
#59132=CARTESIAN_POINT('Ctrl Pts',(3.07975002827901,-7.28691216326764,89.2755207049849));
#59133=CARTESIAN_POINT('Ctrl Pts',(3.06550553767511,-7.29292122430907,89.2748935247054));
#59134=CARTESIAN_POINT('Ctrl Pts',(3.0561386533032,-7.29685142482024,89.2744805920009));
#59135=CARTESIAN_POINT('Ctrl Pts',(2.98912729391316,-7.32481669350729,89.2715229097021));
#59136=CARTESIAN_POINT('Ctrl Pts',(2.93120858293906,-7.34818600197914,89.26894789772));
#59137=CARTESIAN_POINT('Ctrl Pts',(2.79937928928677,-7.39957049555669,89.2630537468386));
#59138=CARTESIAN_POINT('Ctrl Pts',(2.72531359035409,-7.42716858938268,89.259718928896));
#59139=CARTESIAN_POINT('Ctrl Pts',(2.48864030209973,-7.51134008422862,89.2490131471434));
#59140=CARTESIAN_POINT('Ctrl Pts',(2.32459649619534,-7.56371656309882,89.241520017253));
#59141=CARTESIAN_POINT('Ctrl Pts',(1.69625746811555,-7.74196188608367,89.2128111863276));
#59142=CARTESIAN_POINT('Ctrl Pts',(1.22250279643838,-7.83075861067771,89.1912226327961));
#59143=CARTESIAN_POINT('Ctrl Pts',(0.355586806039759,-7.91260965087965,
89.1534498721026));
#59144=CARTESIAN_POINT('Ctrl Pts',(-0.0346427271704981,-7.92052217273406,
89.137051902306));
#59145=CARTESIAN_POINT('Ctrl Pts',(-0.454066400820371,-7.89801607180187,
89.1200456741745));
#59146=CARTESIAN_POINT('Ctrl Pts',(-0.484232254232896,-7.89622399050183,
89.1188257751384));
#59147=CARTESIAN_POINT('Ctrl Pts',(-0.526451993314145,-7.89347296662957,
89.1171227557901));
#59148=CARTESIAN_POINT('Ctrl Pts',(-0.538514946732419,-7.89265917352457,
89.1166366676261));
#59149=CARTESIAN_POINT('Ctrl Pts',(-0.559406663639106,-7.8912016540365,
89.1157956590906));
#59150=CARTESIAN_POINT('Ctrl Pts',(-0.568236288369278,-7.89057075761805,
89.1154404782081));
#59151=CARTESIAN_POINT('Ctrl Pts',(-0.586535984417261,-7.88923232775255,
89.1147048870573));
#59152=CARTESIAN_POINT('Ctrl Pts',(-0.596005885657964,-7.88852255920834,
89.1143245220054));
#59153=CARTESIAN_POINT('Ctrl Pts',(-0.618084668208749,-7.88682777143586,
89.1134383992471));
#59154=CARTESIAN_POINT('Ctrl Pts',(-0.630692523789674,-7.88582956289625,
89.1129329107276));
#59155=CARTESIAN_POINT('Ctrl Pts',(-0.671030336334267,-7.88253851827012,
89.1113173048225));
#59156=CARTESIAN_POINT('Ctrl Pts',(-0.698750702845061,-7.88012961015698,
89.1102095691903));
#59157=CARTESIAN_POINT('Ctrl Pts',(-1.35235739907148,-7.8198549976142,89.0841492654076));
#59158=CARTESIAN_POINT('Ctrl Pts',(-1.96914830990073,-7.68775162937227,
89.0610759037641));
#59159=CARTESIAN_POINT('Ctrl Pts',(-2.84946623624924,-7.38617804129616,
89.0274148742448));
#59160=CARTESIAN_POINT('Ctrl Pts',(-3.12925990640804,-7.27205668559302,
89.0165517271842));
#59161=CARTESIAN_POINT('Ctrl Pts',(-3.62789555974646,-7.03455679761102,
88.9960599973247));
#59162=CARTESIAN_POINT('Ctrl Pts',(-3.84870077825114,-6.91622031359848,
88.9865453355541));
#59163=CARTESIAN_POINT('Ctrl Pts',(-4.06694093101584,-6.78556765952266,
88.9763686875647));
#59164=CARTESIAN_POINT('Ctrl Pts',(-4.07037118107815,-6.78351055475691,
88.9762085330883));
#59165=CARTESIAN_POINT('Ctrl Pts',(-4.07915945447243,-6.77823120263155,
88.9757977018391));
#59166=CARTESIAN_POINT('Ctrl Pts',(-4.08451521415381,-6.77500520711007,
88.9755468397382));
#59167=CARTESIAN_POINT('Ctrl Pts',(-4.09743618762421,-6.7672014804172,88.9749404224538));
#59168=CARTESIAN_POINT('Ctrl Pts',(-4.10499755047477,-6.76261741472149,
88.9745845493052));
#59169=CARTESIAN_POINT('Ctrl Pts',(-4.11682830684305,-6.75541788199236,
88.9740261523946));
#59170=CARTESIAN_POINT('Ctrl Pts',(-4.12110294489782,-6.75281101362623,
88.9738240698017));
#59171=CARTESIAN_POINT('Ctrl Pts',(-4.12875011361243,-6.74813745744278,
88.9734619647517));
#59172=CARTESIAN_POINT('Ctrl Pts',(-4.13212357734966,-6.74607229331455,
88.973302021409));
#59173=CARTESIAN_POINT('Ctrl Pts',(-4.13971081869726,-6.74141971607086,
88.9729418298523));
#59174=CARTESIAN_POINT('Ctrl Pts',(-4.14392371937384,-6.73883088217161,
88.9727415072194));
#59175=CARTESIAN_POINT('Ctrl Pts',(-4.15538303274237,-6.73177430715766,
88.9721957346512));
#59176=CARTESIAN_POINT('Ctrl Pts',(-4.16262465106402,-6.72729882529389,
88.9718498744976));
#59177=CARTESIAN_POINT('Ctrl Pts',(-4.19923122548385,-6.7045934065648,88.9700965957868));
#59178=CARTESIAN_POINT('Ctrl Pts',(-4.22848335818853,-6.68618307114781,
88.9686794297301));
#59179=CARTESIAN_POINT('Ctrl Pts',(-4.69752510172632,-6.38667441708362,
88.945681252535));
#59180=CARTESIAN_POINT('Ctrl Pts',(-5.10850401283036,-6.06295370217041,
88.9215726310023));
#59181=CARTESIAN_POINT('Ctrl Pts',(-5.66154109280362,-5.5309294247509,88.8861948247786));
#59182=CARTESIAN_POINT('Ctrl Pts',(-5.83049875783167,-5.35252442675633,
88.8748914044515));
#59183=CARTESIAN_POINT('Ctrl Pts',(-6.28721580259361,-4.82293649576689,
88.8432752308974));
#59184=CARTESIAN_POINT('Ctrl Pts',(-6.55345991249902,-4.45444168925678,
88.8235576805654));
#59185=CARTESIAN_POINT('Ctrl Pts',(-6.80264324137362,-4.03843196793117,
88.8038577727579));
#59186=CARTESIAN_POINT('Ctrl Pts',(-6.81846369651466,-4.01166308127975,
88.8026004478593));
#59187=CARTESIAN_POINT('Ctrl Pts',(-6.83937710423244,-3.97579558135538,
88.8009293820926));
#59188=CARTESIAN_POINT('Ctrl Pts',(-6.84461037545567,-3.96677935962294,
88.800510458813));
#59189=CARTESIAN_POINT('Ctrl Pts',(-6.85275279673124,-3.9526869768047,88.7998574569564));
#59190=CARTESIAN_POINT('Ctrl Pts',(-6.85567415440904,-3.94761790431529,
88.7996229282094));
#59191=CARTESIAN_POINT('Ctrl Pts',(-6.86124633256004,-3.93792434874941,
88.7991751229777));
#59192=CARTESIAN_POINT('Ctrl Pts',(-6.86389810695387,-3.93330041950039,
88.7989618114114));
#59193=CARTESIAN_POINT('Ctrl Pts',(-6.87007894387121,-3.92249753837498,
88.798464142224));
#59194=CARTESIAN_POINT('Ctrl Pts',(-6.87360434974099,-3.91631649348638,
88.7981799192967));
#59195=CARTESIAN_POINT('Ctrl Pts',(-6.88364814905541,-3.89865150148067,
88.7973691297412));
#59196=CARTESIAN_POINT('Ctrl Pts',(-6.89014614972879,-3.88715595359739,
88.7968433129656));
#59197=CARTESIAN_POINT('Ctrl Pts',(-6.93113556606187,-3.81421627517419,
88.7935183714467));
#59198=CARTESIAN_POINT('Ctrl Pts',(-6.96483406765398,-3.75232897935832,
88.7907483851077));
#59199=CARTESIAN_POINT('Ctrl Pts',(-7.06126245321642,-3.56946249255917,
88.7827081949463));
#59200=CARTESIAN_POINT('Ctrl Pts',(-7.12169974173409,-3.44730110506133,
88.7775205647258));
#59201=CARTESIAN_POINT('Ctrl Pts',(-7.25722827981026,-3.1545635264496,88.7654802538966));
#59202=CARTESIAN_POINT('Ctrl Pts',(-7.32950846528954,-2.98277446092834,
88.75872036824));
#59203=CARTESIAN_POINT('Ctrl Pts',(-7.57982224969622,-2.3236406137841,88.7336882429323));
#59204=CARTESIAN_POINT('Ctrl Pts',(-7.71583711485545,-1.82177387711307,
88.7165431482427));
#59205=CARTESIAN_POINT('Ctrl Pts',(-7.86387864189126,-0.940246937721175,
88.6857869976885));
#59206=CARTESIAN_POINT('Ctrl Pts',(-7.89960940394838,-0.566367179265717,
88.6725147964476));
#59207=CARTESIAN_POINT('Ctrl Pts',(-7.90917464792165,-0.171138357543796,
88.6570488046087));
#59208=CARTESIAN_POINT('Ctrl Pts',(-7.90958721712047,-0.150870773477243,
88.6562517007972));
#59209=CARTESIAN_POINT('Ctrl Pts',(-7.91046489100661,-0.097714372109889,
88.6541501364947));
#59210=CARTESIAN_POINT('Ctrl Pts',(-7.91080278230201,-0.0648241440126914,
88.6528387870776));
#59211=CARTESIAN_POINT('Ctrl Pts',(-7.91096447986695,-0.0247662112375243,
88.6512272635093));
#59212=CARTESIAN_POINT('Ctrl Pts',(-7.91098367050681,-0.0175991834095908,
88.6509383740784));
#59213=CARTESIAN_POINT('Ctrl Pts',(-7.91099755755862,-0.00706825328387941,
88.650513055333));
#59214=CARTESIAN_POINT('Ctrl Pts',(-7.91099984791095,-0.00370434700711826,
88.6503770698615));
#59215=CARTESIAN_POINT('Ctrl Pts',(-7.91099999267456,-0.000340445432580282,
88.6502409582738));
#59216=CARTESIAN_POINT('',(-7.91148363736201,-0.000479168433414057,86.6431685549391));
#59217=CARTESIAN_POINT('Ctrl Pts',(-7.91099997228721,-0.000662171981131852,
88.6422897498906));
#59218=CARTESIAN_POINT('Ctrl Pts',(-7.91101617651205,0.192930468445108,
88.6344460078403));
#59219=CARTESIAN_POINT('Ctrl Pts',(-7.90392191612403,0.386827054223198,
88.6266022657899));
#59220=CARTESIAN_POINT('Ctrl Pts',(-7.88967614590761,0.580457847475918,
88.6187585237396));
#59221=CARTESIAN_POINT('Ctrl Pts',(-7.87544710215177,0.773861291994232,
88.6109239913031));
#59222=CARTESIAN_POINT('Ctrl Pts',(-7.8540832936897,0.966999218801397,88.6030894588665));
#59223=CARTESIAN_POINT('Ctrl Pts',(-7.82559557608183,1.15929930544638,88.59525492643));
#59224=CARTESIAN_POINT('Ctrl Pts',(-7.79713576860348,1.35141099088641,88.5874280696808));
#59225=CARTESIAN_POINT('Ctrl Pts',(-7.76156600219742,1.54268612587329,88.5796012129317));
#59226=CARTESIAN_POINT('Ctrl Pts',(-7.71894909251944,1.73255473422727,88.5717743561825));
#59227=CARTESIAN_POINT('Ctrl Pts',(-7.67636565537242,1.92227421438498,88.5639536468689));
#59228=CARTESIAN_POINT('Ctrl Pts',(-7.62674617561062,2.11058902696814,88.5561329375553));
#59229=CARTESIAN_POINT('Ctrl Pts',(-7.57020501125693,2.29693645700976,88.5483122282417));
#59230=CARTESIAN_POINT('Ctrl Pts',(-7.51369727458084,2.48317371666689,88.5404961426063));
#59231=CARTESIAN_POINT('Ctrl Pts',(-7.45027610663762,2.66744557537262,88.5326800569709));
#59232=CARTESIAN_POINT('Ctrl Pts',(-7.38010651687637,2.84920143190315,88.5248639713355));
#59233=CARTESIAN_POINT('Ctrl Pts',(-7.30996478748406,3.03088512347963,88.5170509890249));
#59234=CARTESIAN_POINT('Ctrl Pts',(-7.23308010113027,3.21005447575066,88.5092380067143));
#59235=CARTESIAN_POINT('Ctrl Pts',(-7.14966676290338,3.38617574550328,88.5014250244038));
#59236=CARTESIAN_POINT('Ctrl Pts',(-7.06625658934013,3.56229033329605,88.4936123385141));
#59237=CARTESIAN_POINT('Ctrl Pts',(-6.976318399643,3.73535674746131,88.4857996526245));
#59238=CARTESIAN_POINT('Ctrl Pts',(-6.88011412013965,3.90486244237297,88.4779869667348));
#59239=CARTESIAN_POINT('Ctrl Pts',(-6.78390704196175,4.07437306836749,88.4701740535667));
#59240=CARTESIAN_POINT('Ctrl Pts',(-6.68143368381306,4.24032246244598,88.4623611403986));
#59241=CARTESIAN_POINT('Ctrl Pts',(-6.57300128222326,4.40222388616156,88.4545482272304));
#59242=CARTESIAN_POINT('Ctrl Pts',(-6.46454665411085,4.56415849650404,88.4467337125678));
#59243=CARTESIAN_POINT('Ctrl Pts',(-6.35013074497053,4.72204319132242,88.4389191979052));
#59244=CARTESIAN_POINT('Ctrl Pts',(-6.23010343430226,4.87542123286749,88.4311046832426));
#59245=CARTESIAN_POINT('Ctrl Pts',(-6.1100304073688,5.02885769337723,88.4232871921705));
#59246=CARTESIAN_POINT('Ctrl Pts',(-5.98434193808971,5.17778380469005,88.4154697010984));
#59247=CARTESIAN_POINT('Ctrl Pts',(-5.85342748423666,5.32177674153876,88.4076522100263));
#59248=CARTESIAN_POINT('Ctrl Pts',(-5.72237101359378,5.46592588279459,88.3998262384927));
#59249=CARTESIAN_POINT('Ctrl Pts',(-5.58607747208317,5.60513090081631,88.3920002669591));
#59250=CARTESIAN_POINT('Ctrl Pts',(-5.44497314654521,5.7390058750102,88.3841742954255));
#59251=CARTESIAN_POINT('Ctrl Pts',(-5.30378311612996,5.87296216307021,88.3763435705017));
#59252=CARTESIAN_POINT('Ctrl Pts',(-5.15777674140503,6.00158172369272,88.3685128455778));
#59253=CARTESIAN_POINT('Ctrl Pts',(-5.00741258114924,6.12451959276385,88.3606821206539));
#59254=CARTESIAN_POINT('Ctrl Pts',(-4.85684276259342,6.24762560824114,88.3528406853748));
#59255=CARTESIAN_POINT('Ctrl Pts',(-4.70190353317579,6.365034199289,88.3449992500957));
#59256=CARTESIAN_POINT('Ctrl Pts',(-4.54308248666159,6.47644366295182,88.3371578148165));
#59257=CARTESIAN_POINT('Ctrl Pts',(-4.45688458062388,6.53690959420772,88.3329019852761));
#59258=CARTESIAN_POINT('Ctrl Pts',(-4.36954368044602,6.59560919825888,88.3286461557357));
#59259=CARTESIAN_POINT('Ctrl Pts',(-4.28114058291619,6.65250000445757,88.3243903261953));
#59260=CARTESIAN_POINT('Ctrl Pts',(-4.11680779895752,6.75825449525617,88.316479151859));
#59261=CARTESIAN_POINT('Ctrl Pts',(-3.94833321133267,6.85805839596443,88.3085679775227));
#59262=CARTESIAN_POINT('Ctrl Pts',(-3.77618638520901,6.95157085730715,88.3006568031864));
#59263=CARTESIAN_POINT('Ctrl Pts',(-3.60422618859514,7.04498193900081,88.2927542055903));
#59264=CARTESIAN_POINT('Ctrl Pts',(-3.42860198368221,7.13211500411089,88.2848516079941));
#59265=CARTESIAN_POINT('Ctrl Pts',(-3.24981282724334,7.21267201443991,88.2769490103979));
#59266=CARTESIAN_POINT('Ctrl Pts',(-3.07118431319469,7.29315664414503,88.2690535133004));
#59267=CARTESIAN_POINT('Ctrl Pts',(-2.88939682496358,7.3670768487532,88.2611580162029));
#59268=CARTESIAN_POINT('Ctrl Pts',(-2.7049748219933,7.4341799959634,88.2532625191054));
#59269=CARTESIAN_POINT('Ctrl Pts',(-2.52068429929008,7.50123530322188,88.245372650957));
#59270=CARTESIAN_POINT('Ctrl Pts',(-2.33376332664721,7.5614831186337,88.2374827828085));
#59271=CARTESIAN_POINT('Ctrl Pts',(-2.14475744898914,7.61471841140601,88.2295929146601));
#59272=CARTESIAN_POINT('Ctrl Pts',(-1.9558512535615,7.66792562773547,88.2217072076503));
#59273=CARTESIAN_POINT('Ctrl Pts',(-1.76486267531535,7.7141275977776,88.2138215006405));
#59274=CARTESIAN_POINT('Ctrl Pts',(-1.57235383840462,7.7531686687995,88.2059357936307));
#59275=CARTESIAN_POINT('Ctrl Pts',(-1.37991082109503,7.79219639151094,88.1980527827781));
#59276=CARTESIAN_POINT('Ctrl Pts',(-1.18594891861128,7.82406802638898,88.1901697719255));
#59277=CARTESIAN_POINT('Ctrl Pts',(-0.991042179878032,7.84867864023637,
88.1822867610729));
#59278=CARTESIAN_POINT('Ctrl Pts',(-0.796132532452158,7.8732896213605,88.1744036325781));
#59279=CARTESIAN_POINT('Ctrl Pts',(-0.600278361625732,7.89063931335327,
88.1665205040834));
#59280=CARTESIAN_POINT('Ctrl Pts',(-0.404061179831432,7.900674373935,88.1586373755886));
#59281=CARTESIAN_POINT('Ctrl Pts',(-0.207831865732971,7.91071005499455,
88.1507537596721));
#59282=CARTESIAN_POINT('Ctrl Pts',(-0.0112398404968657,7.91343018521715,
88.1428701437557));
#59283=CARTESIAN_POINT('Ctrl Pts',(0.185130984511696,7.90883351187606,88.1349865278392));
#59284=CARTESIAN_POINT('Ctrl Pts',(0.38154696021655,7.9042357816417,88.1271010992769));
#59285=CARTESIAN_POINT('Ctrl Pts',(0.577741289492026,7.89231790362637,88.1192156707147));
#59286=CARTESIAN_POINT('Ctrl Pts',(0.773132540163403,7.87313070356008,88.1113302421524));
#59287=CARTESIAN_POINT('Ctrl Pts',(0.968601560950822,7.85393586655626,88.1034416750121));
#59288=CARTESIAN_POINT('Ctrl Pts',(1.16326652321196,7.8274659759085,88.0955531078717));
#59289=CARTESIAN_POINT('Ctrl Pts',(1.35655332800381,7.79382345631987,88.0876645407314));
#59290=CARTESIAN_POINT('Ctrl Pts',(1.55004583197328,7.76014513377707,88.0797675784408));
#59291=CARTESIAN_POINT('Ctrl Pts',(1.74215690905336,7.71927899479134,88.0718706161502));
#59292=CARTESIAN_POINT('Ctrl Pts',(1.93232374226966,7.67137836083327,88.0639736538596));
#59293=CARTESIAN_POINT('Ctrl Pts',(2.12260655195499,7.62344851386105,88.0560718754725));
#59294=CARTESIAN_POINT('Ctrl Pts',(2.31094242366053,7.56847571537108,88.0481700970855));
#59295=CARTESIAN_POINT('Ctrl Pts',(2.49678556671969,7.50666256293836,88.0402683186985));
#59296=CARTESIAN_POINT('Ctrl Pts',(2.68286906913444,7.44476946475546,88.0323563205836));
#59297=CARTESIAN_POINT('Ctrl Pts',(2.86645308139283,7.37601846231122,88.0244443224686));
#59298=CARTESIAN_POINT('Ctrl Pts',(3.04701253864999,7.30065994204016,88.0165323243536));
#59299=CARTESIAN_POINT('Ctrl Pts',(3.12266509464356,7.26908549691829,88.0132172784984));
#59300=CARTESIAN_POINT('Ctrl Pts',(3.19778698486359,7.23635163904106,88.0099022326431));
#59301=CARTESIAN_POINT('Ctrl Pts',(3.27234097360833,7.20247912544313,88.0065871867878));
#59302=CARTESIAN_POINT('Ctrl Pts',(3.45025978130267,7.12164431922523,87.9986760204511));
#59303=CARTESIAN_POINT('Ctrl Pts',(3.62542070534692,7.03410441248774,87.9907648541143));
#59304=CARTESIAN_POINT('Ctrl Pts',(3.79728286212815,6.94006944237504,87.9828536877776));
#59305=CARTESIAN_POINT('Ctrl Pts',(3.96895872577255,6.84613640319283,87.9749510968948));
#59306=CARTESIAN_POINT('Ctrl Pts',(4.13734264475762,6.74572248817744,87.9670485060119));
#59307=CARTESIAN_POINT('Ctrl Pts',(4.30191374327858,6.63908571607498,87.9591459151291));
#59308=CARTESIAN_POINT('Ctrl Pts',(4.46633700092785,6.53254474009641,87.9512504234631));
#59309=CARTESIAN_POINT('Ctrl Pts',(4.62695397386723,6.41979222962641,87.9433549317972));
#59310=CARTESIAN_POINT('Ctrl Pts',(4.78326819030697,6.30113215379566,87.9354594401312));
#59311=CARTESIAN_POINT('Ctrl Pts',(4.93947099063381,6.18255665532905,87.9275695761363));
#59312=CARTESIAN_POINT('Ctrl Pts',(5.09137687119333,6.05808218837905,87.9196797121413));
#59313=CARTESIAN_POINT('Ctrl Pts',(5.23851794852022,5.92805623311988,87.9117898481464));
#59314=CARTESIAN_POINT('Ctrl Pts',(5.38558144697159,5.79809883293439,87.9039041440149));
#59315=CARTESIAN_POINT('Ctrl Pts',(5.52788489031669,5.66259600463352,87.8960184398834));
#59316=CARTESIAN_POINT('Ctrl Pts',(5.66499291790816,5.52193591415641,87.8881327357518));
#59317=CARTESIAN_POINT('Ctrl Pts',(5.80205408979531,5.38132389327614,87.8802497265042));
#59318=CARTESIAN_POINT('Ctrl Pts',(5.93392314415944,5.23555836949925,87.8723667172566));
#59319=CARTESIAN_POINT('Ctrl Pts',(6.06020089225338,5.0850650089779,87.864483708009));
#59320=CARTESIAN_POINT('Ctrl Pts',(6.18648055533892,4.93456936623717,87.8566005792162));
#59321=CARTESIAN_POINT('Ctrl Pts',(6.30716851462362,4.77934600219118,87.8487174504234));
#59322=CARTESIAN_POINT('Ctrl Pts',(6.4219049024596,4.61985480548528,87.8408343216306));
#59323=CARTESIAN_POINT('Ctrl Pts',(6.53664840183501,4.46035372326741,87.8329507042292));
#59324=CARTESIAN_POINT('Ctrl Pts',(6.64543939272819,4.29658456102768,87.8250670868279));
#59325=CARTESIAN_POINT('Ctrl Pts',(6.7479604915137,4.1290374429121,87.8171834694265));
#59326=CARTESIAN_POINT('Ctrl Pts',(6.85050517796842,3.96145177618513,87.8092980381921));
#59327=CARTESIAN_POINT('Ctrl Pts',(6.94677691775842,3.79008671576593,87.8014126069577));
#59328=CARTESIAN_POINT('Ctrl Pts',(7.03650344463055,3.61545851500228,87.7935271757232));
#59329=CARTESIAN_POINT('Ctrl Pts',(7.12626569819126,3.44076078198807,87.7856386047223));
#59330=CARTESIAN_POINT('Ctrl Pts',(7.20947738837047,3.26279762621829,87.7777500337213));
#59331=CARTESIAN_POINT('Ctrl Pts',(7.28591359288956,3.08210709044107,87.7698614627204));
#59332=CARTESIAN_POINT('Ctrl Pts',(7.3624311593015,2.90122422010065,87.7619644947945));
#59333=CARTESIAN_POINT('Ctrl Pts',(7.43215870012965,2.71760848876809,87.7540675268687));
#59334=CARTESIAN_POINT('Ctrl Pts',(7.49492018598347,2.53181602920464,87.7461705589428));
#59335=CARTESIAN_POINT('Ctrl Pts',(7.55771995609665,2.34591023697208,87.7382687738976));
#59336=CARTESIAN_POINT('Ctrl Pts',(7.61354510185648,2.15782539911996,87.7303669888524));
#59337=CARTESIAN_POINT('Ctrl Pts',(7.66227023652275,1.96813003190787,87.7224652038072));
#59338=CARTESIAN_POINT('Ctrl Pts',(7.71105839888217,1.77818928699738,87.7145531975222));
#59339=CARTESIAN_POINT('Ctrl Pts',(7.75272813269699,1.5866341875338,87.7066411912373));
#59340=CARTESIAN_POINT('Ctrl Pts',(7.78720544793176,1.39404171806369,87.6987291849523));
#59341=CARTESIAN_POINT('Ctrl Pts',(7.80165107359589,1.31334753695498,87.6954141390949));
#59342=CARTESIAN_POINT('Ctrl Pts',(7.8148346838919,1.23247128898822,87.6920990932375));
#59343=CARTESIAN_POINT('Ctrl Pts',(7.82675355380094,1.15145551718874,87.68878404738));
#59344=CARTESIAN_POINT('Ctrl Pts',(7.85494261024235,0.959846901495308,87.6809437055108));
#59345=CARTESIAN_POINT('Ctrl Pts',(7.87613359187413,0.766914325471691,87.6731033636416));
#59346=CARTESIAN_POINT('Ctrl Pts',(7.89020557749282,0.573216315976064,87.6652630217724));
#59347=CARTESIAN_POINT('Ctrl Pts',(7.9042618302128,0.379734866619543,87.6574314456388));
#59348=CARTESIAN_POINT('Ctrl Pts',(7.91121491034272,0.1854900348259,87.6495998695051));
#59349=CARTESIAN_POINT('Ctrl Pts',(7.91099493745802,-0.00894983315554786,
87.6417682933715));
#59350=CARTESIAN_POINT('Ctrl Pts',(7.91077516773731,-0.203210119100259,
87.6339439503758));
#59351=CARTESIAN_POINT('Ctrl Pts',(7.90339553874417,-0.397664733449155,
87.6261196073801));
#59352=CARTESIAN_POINT('Ctrl Pts',(7.88883795724331,-0.591740385944079,
87.6182952643844));
#59353=CARTESIAN_POINT('Ctrl Pts',(7.87429099179311,-0.785674509644466,
87.6104766272556));
#59354=CARTESIAN_POINT('Ctrl Pts',(7.85257652571912,-0.97922987291739,87.6026579901268));
#59355=CARTESIAN_POINT('Ctrl Pts',(7.82372852464297,-1.17183316760019,87.594839352998));
#59356=CARTESIAN_POINT('Ctrl Pts',(7.79489595650251,-1.36433342449357,87.5870248986381));
#59357=CARTESIAN_POINT('Ctrl Pts',(7.75893750744041,-1.55588228058694,87.5792104442783));
#59358=CARTESIAN_POINT('Ctrl Pts',(7.71593899617526,-1.74591134004619,87.5713959899184));
#59359=CARTESIAN_POINT('Ctrl Pts',(7.67295513663862,-1.93587564716625,87.5635841983313));
#59360=CARTESIAN_POINT('Ctrl Pts',(7.62293607211913,-2.1243208469729,87.5557724067442));
#59361=CARTESIAN_POINT('Ctrl Pts',(7.56601879313652,-2.31068834374196,87.5479606151571));
#59362=CARTESIAN_POINT('Ctrl Pts',(7.50909885033314,-2.49706456281148,87.5401484579655));
#59363=CARTESIAN_POINT('Ctrl Pts',(7.44528014202093,-2.68136254560945,87.5323363007739));
#59364=CARTESIAN_POINT('Ctrl Pts',(7.37474979339316,-2.8630379817333,87.5245241435823));
#59365=CARTESIAN_POINT('Ctrl Pts',(7.30421367884538,-3.04472826998895,87.5167113477398));
#59366=CARTESIAN_POINT('Ctrl Pts',(7.22696495757362,-3.22379525616171,87.5088985518972));
#59367=CARTESIAN_POINT('Ctrl Pts',(7.14323922955342,-3.39971385698401,87.5010857560547));
#59368=CARTESIAN_POINT('Ctrl Pts',(7.05949192461862,-3.57567779369907,87.4932709467805));
#59369=CARTESIAN_POINT('Ctrl Pts',(6.96926443882062,-3.74849141107556,87.4854561375064));
#59370=CARTESIAN_POINT('Ctrl Pts',(6.87283878831291,-3.91765337796257,87.4776413282322));
#59371=CARTESIAN_POINT('Ctrl Pts',(6.77637131962863,-4.08688870753847,87.4698231298072));
#59372=CARTESIAN_POINT('Ctrl Pts',(6.67370050552191,-4.25246892663546,87.4620049313822));
#59373=CARTESIAN_POINT('Ctrl Pts',(6.56515228678159,-4.41392075725952,87.4541867329572));
#59374=CARTESIAN_POINT('Ctrl Pts',(6.45647771850363,-4.57556051693841,87.4463594341917));
#59375=CARTESIAN_POINT('Ctrl Pts',(6.34191227797189,-4.73306199849868,87.4385321354261));
#59376=CARTESIAN_POINT('Ctrl Pts',(6.2218235514863,-4.88598328836381,87.4307048366606));
#59377=CARTESIAN_POINT('Ctrl Pts',(6.10165643059092,-5.03900440586982,87.4228724282025));
#59378=CARTESIAN_POINT('Ctrl Pts',(5.9759590648151,-5.18743910578546,87.4150400197445));
#59379=CARTESIAN_POINT('Ctrl Pts',(5.84513670267974,-5.33088153376027,87.4072076112864));
#59380=CARTESIAN_POINT('Ctrl Pts',(5.71412659201988,-5.47452982183241,87.3993639622185));
#59381=CARTESIAN_POINT('Ctrl Pts',(5.57797704021789,-5.61317127831506,87.3915203131506));
#59382=CARTESIAN_POINT('Ctrl Pts',(5.4371280975494,-5.74643881467808,87.3836766640827));
#59383=CARTESIAN_POINT('Ctrl Pts',(5.36113524400898,-5.81834123851355,87.3794447453792));
#59384=CARTESIAN_POINT('Ctrl Pts',(5.28377495384006,-5.88868004508179,87.3752128266758));
#59385=CARTESIAN_POINT('Ctrl Pts',(5.20511988185005,-5.9574027911137,87.3709809079724));
#59386=CARTESIAN_POINT('Ctrl Pts',(5.05795934123553,-6.08598034120298,87.3630631548195));
#59387=CARTESIAN_POINT('Ctrl Pts',(4.90582489946001,-6.20928263008101,87.3551454016667));
#59388=CARTESIAN_POINT('Ctrl Pts',(4.74912962242098,-6.32690199303289,87.3472276485139));
#59389=CARTESIAN_POINT('Ctrl Pts',(4.5926143769801,-6.44438621980016,87.3393189922896));
#59390=CARTESIAN_POINT('Ctrl Pts',(4.43154900633982,-6.55620032110361,87.3314103360654));
#59391=CARTESIAN_POINT('Ctrl Pts',(4.26638219957893,-6.66197447661848,87.3235016798412));
#59392=CARTESIAN_POINT('Ctrl Pts',(4.10137458291387,-6.76764668551173,87.3156006460914));
#59393=CARTESIAN_POINT('Ctrl Pts',(3.93227369282455,-6.86729036074609,87.3076996123415));
#59394=CARTESIAN_POINT('Ctrl Pts',(3.7595601978472,-6.96057670877659,87.2997985785916));
#59395=CARTESIAN_POINT('Ctrl Pts',(3.58698120608346,-7.05379040867037,87.2919036978897));
#59396=CARTESIAN_POINT('Ctrl Pts',(3.41079551620029,-7.1406564821353,87.2840088171879));
#59397=CARTESIAN_POINT('Ctrl Pts',(3.23151184679387,-7.22088998559256,87.276113936486));
#59398=CARTESIAN_POINT('Ctrl Pts',(3.05233462934893,-7.30107584938555,87.2682237434701));
#59399=CARTESIAN_POINT('Ctrl Pts',(2.87006341120434,-7.3746368500975,87.2603335504542));
#59400=CARTESIAN_POINT('Ctrl Pts',(2.68523078157349,-7.44133433261067,87.2524433574383));
#59401=CARTESIAN_POINT('Ctrl Pts',(2.50047371056953,-7.50800454953655,87.2445563898926));
#59402=CARTESIAN_POINT('Ctrl Pts',(2.31315763840243,-7.56781672335792,87.236669422347));
#59403=CARTESIAN_POINT('Ctrl Pts',(2.12383463325769,-7.62058051926329,87.2287824548013));
#59404=CARTESIAN_POINT('Ctrl Pts',(1.9345280695243,-7.67333973299296,87.220896172185));
#59405=CARTESIAN_POINT('Ctrl Pts',(1.74321524998539,-7.71905168968404,87.2130098895686));
#59406=CARTESIAN_POINT('Ctrl Pts',(1.55046339164132,-7.75757592751628,87.2051236069523));
#59407=CARTESIAN_POINT('Ctrl Pts',(1.35771187208615,-7.79610009763668,87.1972373381973));
#59408=CARTESIAN_POINT('Ctrl Pts',(1.16352165655767,-7.82743650599629,87.1893510694422));
#59409=CARTESIAN_POINT('Ctrl Pts',(0.96847025096779,-7.85149580481263,87.1814648006871));
#59410=CARTESIAN_POINT('Ctrl Pts',(0.773386496578017,-7.87555909380501,
87.1735772240136));
#59411=CARTESIAN_POINT('Ctrl Pts',(0.577441609510269,-7.89234282628704,
87.1656896473401));
#59412=CARTESIAN_POINT('Ctrl Pts',(0.381218567815195,-7.90180950185164,
87.1578020706666));
#59413=CARTESIAN_POINT('Ctrl Pts',(0.184930094871308,-7.91127933411181,
87.1499118638535));
#59414=CARTESIAN_POINT('Ctrl Pts',(-0.0116363735729002,-7.91342723140898,
87.1420216570404));
#59415=CARTESIAN_POINT('Ctrl Pts',(-0.207897251873945,-7.90826780860785,
87.1341314502273));
#59416=CARTESIAN_POINT('Ctrl Pts',(-0.404347651713557,-7.9031034035517,
87.1262336241466));
#59417=CARTESIAN_POINT('Ctrl Pts',(-0.600491527419305,-7.89061759293021,
87.118335798066));
#59418=CARTESIAN_POINT('Ctrl Pts',(-0.795748747031074,-7.87087701159143,
87.1104379719854));
#59419=CARTESIAN_POINT('Ctrl Pts',(-0.991114084255854,-7.85112549951966,
87.1025357727292));
#59420=CARTESIAN_POINT('Ctrl Pts',(-1.18559144598008,-7.82411125464705,
87.094633573473));
#59421=CARTESIAN_POINT('Ctrl Pts',(-1.37860999873653,-7.7899522123941,87.0867313742168));
#59422=CARTESIAN_POINT('Ctrl Pts',(-1.57186153952061,-7.75575193758724,
87.078819636407));
#59423=CARTESIAN_POINT('Ctrl Pts',(-1.76365041813369,-7.71438971118454,
87.0709078985972));
#59424=CARTESIAN_POINT('Ctrl Pts',(-1.9534190268028,-7.66603385759056,87.0629961607873));
#59425=CARTESIAN_POINT('Ctrl Pts',(-2.03191937974922,-7.64603080439449,
87.0597233633798));
#59426=CARTESIAN_POINT('Ctrl Pts',(-2.11007423792459,-7.62483159989217,
87.0564505659722));
#59427=CARTESIAN_POINT('Ctrl Pts',(-2.1878450953644,-7.60245058114092,87.0531777685646));
#59428=CARTESIAN_POINT('Ctrl Pts',(-2.38542943084931,-7.54558945265377,
87.044862912303));
#59429=CARTESIAN_POINT('Ctrl Pts',(-2.58096509958468,-7.48097278119449,
87.0365480560414));
#59430=CARTESIAN_POINT('Ctrl Pts',(-2.77383604934864,-7.40876201340912,
87.0282331997798));
#59431=CARTESIAN_POINT('Ctrl Pts',(-2.9664694852428,-7.33664017067399,87.0199285829747));
#59432=CARTESIAN_POINT('Ctrl Pts',(-3.1564444736579,-7.25694298576827,87.0116239661695));
#59433=CARTESIAN_POINT('Ctrl Pts',(-3.34315965244035,-7.16988176599133,
87.0033193493644));
#59434=CARTESIAN_POINT('Ctrl Pts',(-3.52965721390785,-7.08292201642697,
86.9950244116246));
#59435=CARTESIAN_POINT('Ctrl Pts',(-3.71290227882356,-6.98861547418967,
86.9867294738847));
#59436=CARTESIAN_POINT('Ctrl Pts',(-3.89231224160578,-6.88722196635521,
86.9784345361449));
#59437=CARTESIAN_POINT('Ctrl Pts',(-4.07145330221265,-6.78598042853625,
86.9701520309744));
#59438=CARTESIAN_POINT('Ctrl Pts',(-4.24677047737049,-6.67767326686733,
86.9618695258039));
#59439=CARTESIAN_POINT('Ctrl Pts',(-4.41770452726697,-6.56260677701818,
86.9535870206334));
#59440=CARTESIAN_POINT('Ctrl Pts',(-4.58848154989358,-6.44764599212813,
86.9453121241235));
#59441=CARTESIAN_POINT('Ctrl Pts',(-4.75488323437949,-6.32593842478341,
86.9370372276136));
#59442=CARTESIAN_POINT('Ctrl Pts',(-4.91637660617609,-6.19783527259675,
86.9287623311037));
#59443=CARTESIAN_POINT('Ctrl Pts',(-5.07768525073537,-6.06987865361534,
86.9204968999902));
#59444=CARTESIAN_POINT('Ctrl Pts',(-5.23409655674919,-5.93554122966022,
86.9122314688767));
#59445=CARTESIAN_POINT('Ctrl Pts',(-5.38510788171419,-5.79521648450683,
86.9039660377632));
#59446=CARTESIAN_POINT('Ctrl Pts',(-5.44411974252883,-5.74038070095378,
86.9007360914624));
#59447=CARTESIAN_POINT('Ctrl Pts',(-5.50230731480781,-5.68463106667982,
86.8975061451616));
#59448=CARTESIAN_POINT('Ctrl Pts',(-5.55964191238288,-5.6279927866048,86.8942761988609));
#59449=CARTESIAN_POINT('Ctrl Pts',(-5.70638134036553,-5.48303548034222,
86.8860096287159));
#59450=CARTESIAN_POINT('Ctrl Pts',(-5.84736570408403,-5.33241794497542,
86.8777430585709));
#59451=CARTESIAN_POINT('Ctrl Pts',(-5.98217903531012,-5.17662583054794,
86.8694764884259));
#59452=CARTESIAN_POINT('Ctrl Pts',(-6.11711316084189,-5.02069412458212,
86.8612025113384));
#59453=CARTESIAN_POINT('Ctrl Pts',(-6.24586502313868,-4.85957880544821,
86.8529285342508));
#59454=CARTESIAN_POINT('Ctrl Pts',(-6.36805989143172,-4.69379741990839,
86.8446545571633));
#59455=CARTESIAN_POINT('Ctrl Pts',(-6.49037217927032,-4.52785673164804,
86.8363726294421));
#59456=CARTESIAN_POINT('Ctrl Pts',(-6.6061147200344,-4.35724126169245,86.8280907017209));
#59457=CARTESIAN_POINT('Ctrl Pts',(-6.71495647049175,-4.18249693357939,
86.8198087739998));
#59458=CARTESIAN_POINT('Ctrl Pts',(-6.82397863896027,-4.00746294617651,
86.8115131180087));
#59459=CARTESIAN_POINT('Ctrl Pts',(-6.92607699242537,-3.82828666728563,
86.8032174620176));
#59460=CARTESIAN_POINT('Ctrl Pts',(-7.02096579852531,-3.64553977566257,
86.7949218060265));
#59461=CARTESIAN_POINT('Ctrl Pts',(-7.11594036574239,-3.46262771621598,
86.7866186523678));
#59462=CARTESIAN_POINT('Ctrl Pts',(-7.20369224976595,-3.27613886560742,
86.7783154987092));
#59463=CARTESIAN_POINT('Ctrl Pts',(-7.28398363721479,-3.08666541315823,
86.7700123450505));
#59464=CARTESIAN_POINT('Ctrl Pts',(-7.3643974398656,-2.89690308251565,86.7616965320985));
#59465=CARTESIAN_POINT('Ctrl Pts',(-7.43732790142503,-2.70414732723279,
86.7533807191463));
#59466=CARTESIAN_POINT('Ctrl Pts',(-7.50258627025342,-2.50900782330484,
86.7450649061943));
#59467=CARTESIAN_POINT('Ctrl Pts',(-7.52793443030262,-2.43321022881555,
86.7418348138485));
#59468=CARTESIAN_POINT('Ctrl Pts',(-7.55212559578346,-2.35705311822049,
86.7386047215028));
#59469=CARTESIAN_POINT('Ctrl Pts',(-7.57515077475619,-2.28057267801548,
86.735374629157));
#59470=CARTESIAN_POINT('Ctrl Pts',(-7.64221455117157,-2.0578136215871,86.7259665723887));
#59471=CARTESIAN_POINT('Ctrl Pts',(-7.69948580999344,-1.83197078554786,
86.7165585156204));
#59472=CARTESIAN_POINT('Ctrl Pts',(-7.7467180442272,-1.60383307836095,86.7071504588521));
#59473=CARTESIAN_POINT('Ctrl Pts',(-7.79374174447566,-1.37670261688337,
86.6977839393856));
#59474=CARTESIAN_POINT('Ctrl Pts',(-7.83081481159807,-1.14729754423536,
86.6884174199192));
#59475=CARTESIAN_POINT('Ctrl Pts',(-7.85774156116296,-0.916416148904123,
86.6790509004527));
#59476=CARTESIAN_POINT('Ctrl Pts',(-7.88444665396917,-0.687435332831672,
86.6697614846983));
#59477=CARTESIAN_POINT('Ctrl Pts',(-7.90117173216421,-0.457002455362897,
86.660472068944));
#59478=CARTESIAN_POINT('Ctrl Pts',(-7.90777360586571,-0.225915024674476,
86.6511826531896));
#59479=CARTESIAN_POINT('Ctrl Pts',(-7.90987040587394,-0.152520084316735,
86.6482322715387));
#59480=CARTESIAN_POINT('Ctrl Pts',(-7.91094640363994,-0.0790592559262316,
86.6452818898878));
#59481=CARTESIAN_POINT('Ctrl Pts',(-7.91099804723377,-0.00555847671740886,
86.6423315082369));
#59482=CARTESIAN_POINT('',(-7.911,2.65620858641569E-12,84.6423315082369));
#59483=CARTESIAN_POINT('Ctrl Pts',(-7.911,3.27626814566884E-12,86.6423315082369));
#59484=CARTESIAN_POINT('Ctrl Pts',(-7.91099999999909,2.20167589667007,86.5537440725042));
#59485=CARTESIAN_POINT('Ctrl Pts',(-6.94214576672187,4.38610418338976,86.4651566367714));
#59486=CARTESIAN_POINT('Ctrl Pts',(-3.67820201487972,7.3418068410779,86.287981765306));
#59487=CARTESIAN_POINT('Ctrl Pts',(-1.40868175871393,8.08992666571398,86.1993943295733));
#59488=CARTESIAN_POINT('Ctrl Pts',(2.97309270521611,7.65454228025127,86.0222194581078));
#59489=CARTESIAN_POINT('Ctrl Pts',(5.05102072675891,6.47444880834002,85.9336320223751));
#59490=CARTESIAN_POINT('Ctrl Pts',(7.66951518848004,2.93425195367362,85.7564571509096));
#59491=CARTESIAN_POINT('Ctrl Pts',(8.18956872247099,0.601881960095445,85.6678697151769));
#59492=CARTESIAN_POINT('Ctrl Pts',(7.32306689761172,-3.71537198232788,85.4906948437114));
#59493=CARTESIAN_POINT('Ctrl Pts',(5.94329958849939,-5.66643518936788,85.4021074079787));
#59494=CARTESIAN_POINT('Ctrl Pts',(2.16154501637474,-7.92205913233101,85.2249325365133));
#59495=CARTESIAN_POINT('Ctrl Pts',(-0.210816529304274,-8.20894963712993,
85.1363451007805));
#59496=CARTESIAN_POINT('Ctrl Pts',(-4.42123908576771,-6.91982244717618,
84.9591702293151));
#59497=CARTESIAN_POINT('Ctrl Pts',(-6.22631625634449,-5.35390358803218,
84.8705827935823));
#59498=CARTESIAN_POINT('Ctrl Pts',(-7.65317280859585,-2.31334857514181,
84.735440741312));
#59499=CARTESIAN_POINT('Ctrl Pts',(-7.91100000000039,-1.15702837836213,
84.6888861247745));
#59500=CARTESIAN_POINT('Ctrl Pts',(-7.911,2.65620858641569E-12,84.6423315082369));
#59501=CARTESIAN_POINT('',(-7.91099994247235,0.000954045336348954,82.6424993008866));
#59502=CARTESIAN_POINT('Ctrl Pts',(-7.9109995798286,0.00257836221761484,
84.6423315082369));
#59503=CARTESIAN_POINT('Ctrl Pts',(-7.91093006408187,0.215868426519756,
84.633779099046));
#59504=CARTESIAN_POINT('Ctrl Pts',(-7.90223050541358,0.428942177783995,
84.6252266898552));
#59505=CARTESIAN_POINT('Ctrl Pts',(-7.88497845690452,0.641120686104887,
84.6166742806643));
#59506=CARTESIAN_POINT('Ctrl Pts',(-7.8671728985271,0.860106669964004,84.6078474783842));
#59507=CARTESIAN_POINT('Ctrl Pts',(-7.84025706044039,1.07813871609647,84.5990206761041));
#59508=CARTESIAN_POINT('Ctrl Pts',(-7.80437267238277,1.29448375446159,84.590193873824));
#59509=CARTESIAN_POINT('Ctrl Pts',(-7.76943768043388,1.50510493494078,84.5816006029539));
#59510=CARTESIAN_POINT('Ctrl Pts',(-7.72600276107914,1.71412702819638,84.5730073320837));
#59511=CARTESIAN_POINT('Ctrl Pts',(-7.67424943977649,1.92088951688799,84.5644140612136));
#59512=CARTESIAN_POINT('Ctrl Pts',(-7.62038643993448,2.13608049623799,84.5554704932285));
#59513=CARTESIAN_POINT('Ctrl Pts',(-7.55751280045111,2.34882350066785,84.5465269252435));
#59514=CARTESIAN_POINT('Ctrl Pts',(-7.48588883338284,2.55839585956397,84.5375833572584));
#59515=CARTESIAN_POINT('Ctrl Pts',(-7.41426486631458,2.7679682184601,84.5286397892734));
#59516=CARTESIAN_POINT('Ctrl Pts',(-7.33389072764557,2.97436967862314,84.5196962212883));
#59517=CARTESIAN_POINT('Ctrl Pts',(-7.24508130678783,3.1769038163019,84.5107526533033));
#59518=CARTESIAN_POINT('Ctrl Pts',(-7.16652560102665,3.35605386561449,84.5028416874587));
#59519=CARTESIAN_POINT('Ctrl Pts',(-7.08122200956264,3.53251459720829,84.494930721614));
#59520=CARTESIAN_POINT('Ctrl Pts',(-6.9893770106968,3.70574284082733,84.4870197557694));
#59521=CARTESIAN_POINT('Ctrl Pts',(-6.89762495048163,3.87879579347335,84.4791167950911));
#59522=CARTESIAN_POINT('Ctrl Pts',(-6.79934482819329,4.04862247186651,84.4712138344127));
#59523=CARTESIAN_POINT('Ctrl Pts',(-6.69479123344108,4.21469943657202,84.4633108737344));
#59524=CARTESIAN_POINT('Ctrl Pts',(-6.59032408841021,4.38063908120398,84.4554144475875));
#59525=CARTESIAN_POINT('Ctrl Pts',(-6.47959398724002,4.5428348988684,84.4475180214406));
#59526=CARTESIAN_POINT('Ctrl Pts',(-6.36290162547618,4.70078758342819,84.4396215952936));
#59527=CARTESIAN_POINT('Ctrl Pts',(-6.24628416092563,4.85863888846555,84.4317302373475));
#59528=CARTESIAN_POINT('Ctrl Pts',(-6.1237122643645,5.01225221047996,84.4238388794013));
#59529=CARTESIAN_POINT('Ctrl Pts',(-5.9955303235939,5.16115656988489,84.4159475214551));
#59530=CARTESIAN_POINT('Ctrl Pts',(-5.86740694403511,5.30999290083216,84.4080597687553));
#59531=CARTESIAN_POINT('Ctrl Pts',(-5.73367885193989,5.45412429566728,84.4001720160556));
#59532=CARTESIAN_POINT('Ctrl Pts',(-5.59473132726087,5.59311204748893,84.3922842633558));
#59533=CARTESIAN_POINT('Ctrl Pts',(-5.45582158411724,5.73206200683694,84.3843986554327));
#59534=CARTESIAN_POINT('Ctrl Pts',(-5.31169548047284,5.86587086750381,84.3765130475096));
#59535=CARTESIAN_POINT('Ctrl Pts',(-5.16277602726376,5.99413585867976,84.3686274395865));
#59536=CARTESIAN_POINT('Ctrl Pts',(-5.01383901029741,6.12241597759843,84.3607409016244));
#59537=CARTESIAN_POINT('Ctrl Pts',(-4.86010777076724,6.24515069055797,84.3528543636623));
#59538=CARTESIAN_POINT('Ctrl Pts',(-4.70203984142614,6.36197629118824,84.3449678257001));
#59539=CARTESIAN_POINT('Ctrl Pts',(-4.54395199851371,6.47881660963597,84.3370802941833));
#59540=CARTESIAN_POINT('Ctrl Pts',(-4.38152665391761,6.58974612692609,84.3291927626665));
#59541=CARTESIAN_POINT('Ctrl Pts',(-4.21525184874517,6.69444343105911,84.3213052311496));
#59542=CARTESIAN_POINT('Ctrl Pts',(-4.04892822650996,6.79917147355241,84.3134153839114));
#59543=CARTESIAN_POINT('Ctrl Pts',(-3.87875318305699,6.89766347302662,84.3055255366732));
#59544=CARTESIAN_POINT('Ctrl Pts',(-3.70524118047121,6.98964296617076,84.297635689435));
#59545=CARTESIAN_POINT('Ctrl Pts',(-3.53164915276753,7.08166488098989,84.2897422033363));
#59546=CARTESIAN_POINT('Ctrl Pts',(-3.35471740313413,7.16716814282994,84.2818487172377));
#59547=CARTESIAN_POINT('Ctrl Pts',(-3.17498249196566,7.24592348674146,84.2739552311391));
#59548=CARTESIAN_POINT('Ctrl Pts',(-2.99503980748883,7.32476987172146,84.2660526201815));
#59549=CARTESIAN_POINT('Ctrl Pts',(-2.81228780450381,7.39685261935806,84.2581500092239));
#59550=CARTESIAN_POINT('Ctrl Pts',(-2.62728150413383,7.46199121535507,84.2502473982662));
#59551=CARTESIAN_POINT('Ctrl Pts',(-2.44215249750421,7.52717301481844,84.2423395458664));
#59552=CARTESIAN_POINT('Ctrl Pts',(-2.25476654067875,7.58540137886259,84.2344316934666));
#59553=CARTESIAN_POINT('Ctrl Pts',(-2.0656913623117,7.63654635261719,84.2265238410668));
#59554=CARTESIAN_POINT('Ctrl Pts',(-1.87635747547357,7.68776130720204,84.2186051684819));
#59555=CARTESIAN_POINT('Ctrl Pts',(-1.68533008489886,7.73187343546429,84.2106864958971));
#59556=CARTESIAN_POINT('Ctrl Pts',(-1.49318575785475,7.76880410954863,84.2027678233123));
#59557=CARTESIAN_POINT('Ctrl Pts',(-1.41377293390896,7.78406747518829,84.1994950535068));
#59558=CARTESIAN_POINT('Ctrl Pts',(-1.33416936762576,7.79810475494626,84.1962222837012));
#59559=CARTESIAN_POINT('Ctrl Pts',(-1.25441587480513,7.8109129948449,84.1929495138956));
#59560=CARTESIAN_POINT('Ctrl Pts',(-1.06328808945263,7.84160770725826,84.1851063809771));
#59561=CARTESIAN_POINT('Ctrl Pts',(-0.870733243483305,7.8653311749436,84.1772632480586));
#59562=CARTESIAN_POINT('Ctrl Pts',(-0.677307280746736,7.88195254029403,
84.1694201151401));
#59563=CARTESIAN_POINT('Ctrl Pts',(-0.484108476215863,7.89855438561996,
84.1615861931465));
#59564=CARTESIAN_POINT('Ctrl Pts',(-0.290040938258333,7.90807070657361,
84.1537522711528));
#59565=CARTESIAN_POINT('Ctrl Pts',(-0.0956713935766871,7.91042147957055,
84.1459183491591));
#59566=CARTESIAN_POINT('Ctrl Pts',(0.098507686294237,7.9127699490197,84.13809210371));
#59567=CARTESIAN_POINT('Ctrl Pts',(0.292987834792579,7.9079668492622,84.1302658582608));
#59568=CARTESIAN_POINT('Ctrl Pts',(0.487196402186665,7.89598383139786,84.1224396128117));
#59569=CARTESIAN_POINT('Ctrl Pts',(0.681252410513519,7.88401022670231,84.1146195152104));
#59570=CARTESIAN_POINT('Ctrl Pts',(0.87503691354045,7.86486795881519,84.106799417609));
#59571=CARTESIAN_POINT('Ctrl Pts',(1.0679762583037,7.83858072049396,84.0989793200076));
#59572=CARTESIAN_POINT('Ctrl Pts',(1.26080152720576,7.81230902456691,84.0911638460581));
#59573=CARTESIAN_POINT('Ctrl Pts',(1.45278228592922,7.7789008206446,84.0833483721087));
#59574=CARTESIAN_POINT('Ctrl Pts',(1.6433488114968,7.73843173283528,84.0755328981592));
#59575=CARTESIAN_POINT('Ctrl Pts',(1.8338396792044,7.69797871188014,84.0677205270738));
#59576=CARTESIAN_POINT('Ctrl Pts',(2.02291708901737,7.65047046517733,84.0599081559885));
#59577=CARTESIAN_POINT('Ctrl Pts',(2.21002014796113,7.5960339615885,84.0520957849031));
#59578=CARTESIAN_POINT('Ctrl Pts',(2.39711612438674,7.5415995186155,84.0442837095439));
#59579=CARTESIAN_POINT('Ctrl Pts',(2.58223755879231,7.48023743076533,84.0364716341847));
#59580=CARTESIAN_POINT('Ctrl Pts',(2.7648369391902,7.41212504614496,84.0286595588254));
#59581=CARTESIAN_POINT('Ctrl Pts',(2.94744166005093,7.34401066944959,84.0208472549873));
#59582=CARTESIAN_POINT('Ctrl Pts',(3.12752385005019,7.26914572494176,84.0130349511492));
#59583=CARTESIAN_POINT('Ctrl Pts',(3.30455429656338,7.18775638854466,84.0052226473111));
#59584=CARTESIAN_POINT('Ctrl Pts',(3.48162106973891,7.10635035104896,83.9974087403876));
#59585=CARTESIAN_POINT('Ctrl Pts',(3.65563453234891,7.01841740160396,83.9895948334642));
#59586=CARTESIAN_POINT('Ctrl Pts',(3.82608833512247,6.92423057471657,83.9817809265407));
#59587=CARTESIAN_POINT('Ctrl Pts',(3.9966071090415,6.83000784704005,83.9739640412237));
#59588=CARTESIAN_POINT('Ctrl Pts',(4.16356321280081,6.72952666356001,83.9661471559068));
#59589=CARTESIAN_POINT('Ctrl Pts',(4.32647750921442,6.62310451089682,83.9583302705899));
#59590=CARTESIAN_POINT('Ctrl Pts',(4.48956853317429,6.51656691271213,83.9505049056061));
#59591=CARTESIAN_POINT('Ctrl Pts',(4.64860869820649,6.40407566594995,83.9426795406223));
#59592=CARTESIAN_POINT('Ctrl Pts',(4.8031494704633,6.28599046804783,83.9348541756385));
#59593=CARTESIAN_POINT('Ctrl Pts',(4.95778416575485,6.16783350319396,83.9270240547446));
#59594=CARTESIAN_POINT('Ctrl Pts',(5.10791374803941,6.04407603479396,83.9191939338507));
#59595=CARTESIAN_POINT('Ctrl Pts',(5.25312500948118,5.91511611337963,83.9113638129568));
#59596=CARTESIAN_POINT('Ctrl Pts',(5.39853476509491,5.78597991229827,83.9035229888065));
#59597=CARTESIAN_POINT('Ctrl Pts',(5.53901251867156,5.65162729675949,83.8956821646562));
#59598=CARTESIAN_POINT('Ctrl Pts',(5.67418317873892,5.51249183710201,83.8878413405058));
#59599=CARTESIAN_POINT('Ctrl Pts',(5.74713413828386,5.43740109415764,83.8836096851666));
#59600=CARTESIAN_POINT('Ctrl Pts',(5.81854000132922,5.36091780652849,83.8793780298273));
#59601=CARTESIAN_POINT('Ctrl Pts',(5.88834694540054,5.2831137836121,83.875146374488));
#59602=CARTESIAN_POINT('Ctrl Pts',(6.01885258915522,5.13765742203531,83.867235200155));
#59603=CARTESIAN_POINT('Ctrl Pts',(6.14414076753762,4.98716696520392,83.859324025822));
#59604=CARTESIAN_POINT('Ctrl Pts',(6.26380039774366,4.83205190133823,83.851412851489));
#59605=CARTESIAN_POINT('Ctrl Pts',(6.3833303013745,4.67710500234118,83.8435102538961));
#59606=CARTESIAN_POINT('Ctrl Pts',(6.49724360253856,4.51754375337019,83.8356076563033));
#59607=CARTESIAN_POINT('Ctrl Pts',(6.60516680373139,4.3538135576624,83.8277050587104));
#59608=CARTESIAN_POINT('Ctrl Pts',(6.71299303572663,4.19023047384086,83.8198095616162));
#59609=CARTESIAN_POINT('Ctrl Pts',(6.81483970081807,4.02248619135834,83.811914064522));
#59610=CARTESIAN_POINT('Ctrl Pts',(6.91037409794283,3.85105840341078,83.8040185674278));
#59611=CARTESIAN_POINT('Ctrl Pts',(7.00584038558016,3.67975283174469,83.7961286992827));
#59612=CARTESIAN_POINT('Ctrl Pts',(7.09500320404474,3.50476928666504,83.7882388311377));
#59613=CARTESIAN_POINT('Ctrl Pts',(7.17757350195661,3.32661383752463,83.7803489629926));
#59614=CARTESIAN_POINT('Ctrl Pts',(7.26010025206162,3.14855234806811,83.7724632559861));
#59615=CARTESIAN_POINT('Ctrl Pts',(7.33604126518389,2.96732260008995,83.7645775489797));
#59616=CARTESIAN_POINT('Ctrl Pts',(7.40515360914334,2.78345487209535,83.7566918419732));
#59617=CARTESIAN_POINT('Ctrl Pts',(7.47424232329485,2.59965000926854,83.7488088311239));
#59618=CARTESIAN_POINT('Ctrl Pts',(7.53650690035275,2.41320928641171,83.7409258202746));
#59619=CARTESIAN_POINT('Ctrl Pts',(7.59175259082938,2.22468280876968,83.7330428094253));
#59620=CARTESIAN_POINT('Ctrl Pts',(7.64699910576532,2.03615351765192,83.7251596809339));
#59621=CARTESIAN_POINT('Ctrl Pts',(7.69522641974634,1.84553873806009,83.7172765524424));
#59622=CARTESIAN_POINT('Ctrl Pts',(7.73628953466395,1.65340413566952,83.7093934239509));
#59623=CARTESIAN_POINT('Ctrl Pts',(7.77735518855499,1.46125765340444,83.7015098080378));
#59624=CARTESIAN_POINT('Ctrl Pts',(7.81125568801351,1.26759149838078,83.6936261921246));
#59625=CARTESIAN_POINT('Ctrl Pts',(7.83789708277303,1.07298197555136,83.6857425762115));
#59626=CARTESIAN_POINT('Ctrl Pts',(7.86454460307338,0.878327706994834,83.6778571476526));
#59627=CARTESIAN_POINT('Ctrl Pts',(7.88392964603437,0.682729980179148,83.6699717190937));
#59628=CARTESIAN_POINT('Ctrl Pts',(7.89601007282437,0.486770921333764,83.6620862905347));
#59629=CARTESIAN_POINT('Ctrl Pts',(7.90809530789625,0.290733866370523,83.6541977233977));
#59630=CARTESIAN_POINT('Ctrl Pts',(7.91287011232309,0.0943355368062724,
83.6463091562606));
#59631=CARTESIAN_POINT('Ctrl Pts',(7.91034445603173,-0.101840988448166,
83.6384205891236));
#59632=CARTESIAN_POINT('Ctrl Pts',(7.90781611189303,-0.298226288171213,
83.6305236268363));
#59633=CARTESIAN_POINT('Ctrl Pts',(7.89797179308439,-0.494388967111445,
83.622626664549));
#59634=CARTESIAN_POINT('Ctrl Pts',(7.88087351197409,-0.689749003816036,
83.6147297022616));
#59635=CARTESIAN_POINT('Ctrl Pts',(7.86376480318697,-0.885228184153381,
83.6068279238779));
#59636=CARTESIAN_POINT('Ctrl Pts',(7.83939335506088,-1.07990340504673,83.5989261454941));
#59637=CARTESIAN_POINT('Ctrl Pts',(7.80787253438817,-1.27320363129659,83.5910243671104));
#59638=CARTESIAN_POINT('Ctrl Pts',(7.77631094641002,-1.4667538614867,83.5831123689986));
#59639=CARTESIAN_POINT('Ctrl Pts',(7.73758158461768,-1.65892520793903,83.5752003708869));
#59640=CARTESIAN_POINT('Ctrl Pts',(7.69184828925866,-1.84915951043403,83.5672883727751));
#59641=CARTESIAN_POINT('Ctrl Pts',(7.67268650849822,-1.92886572816683,83.5639733268769));
#59642=CARTESIAN_POINT('Ctrl Pts',(7.65229576417141,-2.00823210367551,83.5606582809786));
#59643=CARTESIAN_POINT('Ctrl Pts',(7.63069063770581,-2.08721857782766,83.5573432350803));
#59644=CARTESIAN_POINT('Ctrl Pts',(7.57913124618991,-2.27571525484348,83.5494320687359));
#59645=CARTESIAN_POINT('Ctrl Pts',(7.52051391840175,-2.46255367042699,83.5415209023915));
#59646=CARTESIAN_POINT('Ctrl Pts',(7.45496014546727,-2.64716645292558,83.533609736047));
#59647=CARTESIAN_POINT('Ctrl Pts',(7.38947743074717,-2.83157912101295,83.5257071451564));
#59648=CARTESIAN_POINT('Ctrl Pts',(7.31707336173238,-3.01377063936993,83.5178045542659));
#59649=CARTESIAN_POINT('Ctrl Pts',(7.23791997929484,-3.19318577181544,83.5099019633753));
#59650=CARTESIAN_POINT('Ctrl Pts',(7.15883770354123,-3.37243972839302,83.5020064717016));
#59651=CARTESIAN_POINT('Ctrl Pts',(7.07301833106893,-3.5489219540993,83.4941109800279));
#59652=CARTESIAN_POINT('Ctrl Pts',(6.98068314507643,-3.72209401117784,83.4862154883542));
#59653=CARTESIAN_POINT('Ctrl Pts',(6.88841377285106,-3.89514263637808,83.4783256243516));
#59654=CARTESIAN_POINT('Ctrl Pts',(6.78963800167896,-4.06488549062608,83.470435760349));
#59655=CARTESIAN_POINT('Ctrl Pts',(6.68462461307415,-4.23080545313576,83.4625458963463));
#59656=CARTESIAN_POINT('Ctrl Pts',(6.57966659188112,-4.39663793576303,83.4546601922071));
#59657=CARTESIAN_POINT('Ctrl Pts',(6.46847769047691,-4.55865125230619,83.4467744880678));
#59658=CARTESIAN_POINT('Ctrl Pts',(6.35137202397273,-4.71635393212771,83.4388887839285));
#59659=CARTESIAN_POINT('Ctrl Pts',(6.23430637750785,-4.87400271816569,83.4310057746733));
#59660=CARTESIAN_POINT('Ctrl Pts',(6.11132820122546,-5.02734352697304,83.423122765418));
#59661=CARTESIAN_POINT('Ctrl Pts',(5.98279437809521,-5.17591464665254,83.4152397561628));
#59662=CARTESIAN_POINT('Ctrl Pts',(5.85425860576046,-5.32448801940046,83.4073566273623));
#59663=CARTESIAN_POINT('Ctrl Pts',(5.72016723743268,-5.46829129220355,83.3994734985619));
#59664=CARTESIAN_POINT('Ctrl Pts',(5.58091718783104,-5.60689614158958,83.3915903697615));
#59665=CARTESIAN_POINT('Ctrl Pts',(5.44165850729581,-5.74550958191869,83.3837067523526));
#59666=CARTESIAN_POINT('Ctrl Pts',(5.29724075248069,-5.8789237129606,83.3758231349436));
#59667=CARTESIAN_POINT('Ctrl Pts',(5.14809743564973,-6.00674735552085,83.3679395175347));
#59668=CARTESIAN_POINT('Ctrl Pts',(4.99891980448622,-6.13460040726329,83.3600540862928));
#59669=CARTESIAN_POINT('Ctrl Pts',(4.84501470672823,-6.25686018301368,83.3521686550508));
#59670=CARTESIAN_POINT('Ctrl Pts',(4.68684861610154,-6.37317589979651,83.3442832238089));
#59671=CARTESIAN_POINT('Ctrl Pts',(4.52861954799558,-6.48953793036641,83.3363946528005));
#59672=CARTESIAN_POINT('Ctrl Pts',(4.36612638401809,-6.59995098178244,83.3285060817922));
#59673=CARTESIAN_POINT('Ctrl Pts',(4.19986462814982,-6.70410755471718,83.3206175107838));
#59674=CARTESIAN_POINT('Ctrl Pts',(4.03342589631608,-6.80837499626364,83.3127205428506));
#59675=CARTESIAN_POINT('Ctrl Pts',(3.86321085248997,-6.90637247412938,83.3048235749174));
#59676=CARTESIAN_POINT('Ctrl Pts',(3.68974062438688,-6.9978378892876,83.2969266069841));
#59677=CARTESIAN_POINT('Ctrl Pts',(3.5161645801288,-7.08935909798834,83.2890248219316));
#59678=CARTESIAN_POINT('Ctrl Pts',(3.33932970295774,-7.17434015126876,83.2811230368791));
#59679=CARTESIAN_POINT('Ctrl Pts',(3.15977738802902,-7.25256698404782,83.2732212518266));
#59680=CARTESIAN_POINT('Ctrl Pts',(2.97999281580384,-7.33089500601344,83.2653092455344));
#59681=CARTESIAN_POINT('Ctrl Pts',(2.79748410483198,-7.40245123103485,83.2573972392423));
#59682=CARTESIAN_POINT('Ctrl Pts',(2.61280917189454,-7.46707099412238,83.2494852329502));
#59683=CARTESIAN_POINT('Ctrl Pts',(2.53543235612082,-7.49414598163819,83.246170187191));
#59684=CARTESIAN_POINT('Ctrl Pts',(2.45767540044514,-7.52000387236544,83.2428551414317));
#59685=CARTESIAN_POINT('Ctrl Pts',(2.37957987550948,-7.54463522087518,83.2395400956725));
#59686=CARTESIAN_POINT('Ctrl Pts',(2.19487786588614,-7.60289028188194,83.2316997538063));
#59687=CARTESIAN_POINT('Ctrl Pts',(2.00775753756321,-7.65444626410038,83.2238594119401));
#59688=CARTESIAN_POINT('Ctrl Pts',(1.81875113205706,-7.69909509745406,83.2160190700738));
#59689=CARTESIAN_POINT('Ctrl Pts',(1.62995604133662,-7.74369401208341,83.2081874939431));
#59690=CARTESIAN_POINT('Ctrl Pts',(1.4392794108911,-7.78140107487166,83.2003559178124));
#59691=CARTESIAN_POINT('Ctrl Pts',(1.24727128131272,-7.81205704989489,83.1925243416816));
#59692=CARTESIAN_POINT('Ctrl Pts',(1.05544048784877,-7.84268471147377,83.1846999986888));
#59693=CARTESIAN_POINT('Ctrl Pts',(0.862280988958657,-7.86627419927192,
83.176875655696));
#59694=CARTESIAN_POINT('Ctrl Pts',(0.668355929292285,-7.88271662257244,
83.1690513127032));
#59695=CARTESIAN_POINT('Ctrl Pts',(0.474572288600763,-7.89914705530995,
83.1612326755772));
#59696=CARTESIAN_POINT('Ctrl Pts',(0.280024547811638,-7.90844077482352,
83.1534140384512));
#59697=CARTESIAN_POINT('Ctrl Pts',(0.0852841351561738,-7.91054028599126,
83.1455954013252));
#59698=CARTESIAN_POINT('Ctrl Pts',(-0.109352096408714,-7.91263867397475,
83.1377809469681));
#59699=CARTESIAN_POINT('Ctrl Pts',(-0.304180443843766,-7.90755051662476,
83.1299664926111));
#59700=CARTESIAN_POINT('Ctrl Pts',(-0.498626095695033,-7.89527029408696,
83.122152038254));
#59701=CARTESIAN_POINT('Ctrl Pts',(-0.693005490256475,-7.88299425603082,
83.1143402466696));
#59702=CARTESIAN_POINT('Ctrl Pts',(-0.88700209858081,-7.86353105783853,
83.1065284550851));
#59703=CARTESIAN_POINT('Ctrl Pts',(-1.08004265994247,-7.83692725835224,
83.0987166635007));
#59704=CARTESIAN_POINT('Ctrl Pts',(-1.27309225591602,-7.81032221376492,
83.0909045063118));
#59705=CARTESIAN_POINT('Ctrl Pts',(-1.46518536595255,-7.77657593916149,
83.0830923491228));
#59706=CARTESIAN_POINT('Ctrl Pts',(-1.65575487304225,-7.73578676027183,
83.0752801919339));
#59707=CARTESIAN_POINT('Ctrl Pts',(-1.84633995936271,-7.69499424682964,
83.067467396094));
#59708=CARTESIAN_POINT('Ctrl Pts',(-2.03540085035699,-7.64715775500881,
83.059654600254));
#59709=CARTESIAN_POINT('Ctrl Pts',(-2.22238171541002,-7.59242652325403,
83.0518418044141));
#59710=CARTESIAN_POINT('Ctrl Pts',(-2.40941076720844,-7.53768118674083,
83.0440269951425));
#59711=CARTESIAN_POINT('Ctrl Pts',(-2.59435838759789,-7.47603766936701,
83.0362121858709));
#59712=CARTESIAN_POINT('Ctrl Pts',(-2.77668482680089,-7.40769480827968,
83.0283973765992));
#59713=CARTESIAN_POINT('Ctrl Pts',(-2.95909033790246,-7.33932230804729,
83.0205791781768));
#59714=CARTESIAN_POINT('Ctrl Pts',(-3.13887207431502,-7.26424479973415,
83.0127609797542));
#59715=CARTESIAN_POINT('Ctrl Pts',(-3.31551100918296,-7.18270894217402,
83.0049427813318));
#59716=CARTESIAN_POINT('Ctrl Pts',(-3.49235555081547,-7.10107817731679,
82.9971154825686));
#59717=CARTESIAN_POINT('Ctrl Pts',(-3.66604966510608,-7.01297419616484,
82.9892881838055));
#59718=CARTESIAN_POINT('Ctrl Pts',(-3.83609867925429,-6.91868975478909,
82.9814608850423));
#59719=CARTESIAN_POINT('Ctrl Pts',(-4.00625870209264,-6.82434376414538,
82.9736284765866));
#59720=CARTESIAN_POINT('Ctrl Pts',(-4.17276858281325,-6.7238094540847,82.9657960681309));
#59721=CARTESIAN_POINT('Ctrl Pts',(-4.33516327038756,-6.61742249059878,
82.9579636596752));
#59722=CARTESIAN_POINT('Ctrl Pts',(-4.49779101722459,-6.5108828468273,82.9501200106095));
#59723=CARTESIAN_POINT('Ctrl Pts',(-4.6562914895126,-6.3984739763138,82.9422763615439));
#59724=CARTESIAN_POINT('Ctrl Pts',(-4.81023238443817,-6.2805720605453,82.9344327124782));
#59725=CARTESIAN_POINT('Ctrl Pts',(-4.89328879763165,-6.21695991747503,
82.9302007937405));
#59726=CARTESIAN_POINT('Ctrl Pts',(-4.97501855115026,-6.15174941395189,
82.9259688750027));
#59727=CARTESIAN_POINT('Ctrl Pts',(-5.05535833089065,-6.08500395614453,
82.921736956265));
#59728=CARTESIAN_POINT('Ctrl Pts',(-5.20399385829731,-5.96151909776858,
82.9139075413031));
#59729=CARTESIAN_POINT('Ctrl Pts',(-5.34833352264433,-5.83239276955187,
82.9060781263413));
#59730=CARTESIAN_POINT('Ctrl Pts',(-5.48791468024828,-5.69795695511255,
82.8982487113795));
#59731=CARTESIAN_POINT('Ctrl Pts',(-5.62733478723547,-5.56367625452385,
82.890428330102));
#59732=CARTESIAN_POINT('Ctrl Pts',(-5.76200706819059,-5.42409850837976,
82.8826079488245));
#59733=CARTESIAN_POINT('Ctrl Pts',(-5.8915001616145,-5.27959722381322,82.8747875675469));
#59734=CARTESIAN_POINT('Ctrl Pts',(-6.02086927695928,-5.13523428632929,
82.8669746735865));
#59735=CARTESIAN_POINT('Ctrl Pts',(-6.14506884560285,-4.98595745894551,
82.859161779626));
#59736=CARTESIAN_POINT('Ctrl Pts',(-6.26370262716065,-4.83217863892684,
82.8513488856655));
#59737=CARTESIAN_POINT('Ctrl Pts',(-6.38224611130333,-4.67851686676558,
82.843541938444));
#59738=CARTESIAN_POINT('Ctrl Pts',(-6.49523203143791,-4.52036020543207,
82.8357349912225));
#59739=CARTESIAN_POINT('Ctrl Pts',(-6.60230278563192,-4.35815545005418,
82.827928044001));
#59740=CARTESIAN_POINT('Ctrl Pts',(-6.70931260165946,-4.19604301176569,
82.8201255400194));
#59741=CARTESIAN_POINT('Ctrl Pts',(-6.81041376450384,-4.02988736331785,
82.8123230360378));
#59742=CARTESIAN_POINT('Ctrl Pts',(-6.90529047660876,-3.8601663738311,82.8045205320562));
#59743=CARTESIAN_POINT('Ctrl Pts',(-7.00013829400394,-3.69049707288436,
82.7967204043277));
#59744=CARTESIAN_POINT('Ctrl Pts',(-7.08876526282641,-3.51726490078991,
82.7889202765993));
#59745=CARTESIAN_POINT('Ctrl Pts',(-7.17090011100932,-3.34097479755932,
82.7811201488709));
#59746=CARTESIAN_POINT('Ctrl Pts',(-7.25302453423391,-3.16470706993443,
82.773321011173));
#59747=CARTESIAN_POINT('Ctrl Pts',(-7.3286583287584,-2.98538250430967,82.765521873475));
#59748=CARTESIAN_POINT('Ctrl Pts',(-7.39757714600128,-2.80352873517636,
82.7577227357771));
#59749=CARTESIAN_POINT('Ctrl Pts',(-7.46649945756484,-2.62166574569638,
82.7499232026475));
#59750=CARTESIAN_POINT('Ctrl Pts',(-7.52870598929783,-2.43727362793176,
82.7421236695178));
#59751=CARTESIAN_POINT('Ctrl Pts',(-7.58402127213157,-2.25089811938608,
82.7343241363882));
#59752=CARTESIAN_POINT('Ctrl Pts',(-7.63937274340732,-2.0644006799935,82.726519500637));
#59753=CARTESIAN_POINT('Ctrl Pts',(-7.68782385647299,-1.87591759612322,
82.7187148648858));
#59754=CARTESIAN_POINT('Ctrl Pts',(-7.72924936756948,-1.68600866365711,
82.7109102291347));
#59755=CARTESIAN_POINT('Ctrl Pts',(-7.7706883216808,-1.4960381037414,82.703103060697));
#59756=CARTESIAN_POINT('Ctrl Pts',(-7.80509706483003,-1.30464112026713,
82.6952958922593));
#59757=CARTESIAN_POINT('Ctrl Pts',(-7.83240185020259,-1.11238583995981,
82.6874887238215));
#59758=CARTESIAN_POINT('Ctrl Pts',(-7.85973685435271,-0.919917786709097,
82.6796729150271));
#59759=CARTESIAN_POINT('Ctrl Pts',(-7.87995215144126,-0.726589889817072,
82.6718571062327));
#59760=CARTESIAN_POINT('Ctrl Pts',(-7.89302597221011,-0.532974672959839,
82.6640412974382));
#59761=CARTESIAN_POINT('Ctrl Pts',(-7.90503736302606,-0.355093388008408,
82.656860631921));
#59762=CARTESIAN_POINT('Ctrl Pts',(-7.91102139961202,-0.176969816629341,
82.6496799664038));
#59763=CARTESIAN_POINT('Ctrl Pts',(-7.91099994247235,0.000954045336348954,
82.6424993008866));
#59764=CARTESIAN_POINT('',(-7.91099999409123,-0.000305758797192468,78.6348799381992));
#59765=CARTESIAN_POINT('Ctrl Pts',(-7.91099993152671,0.00104085748967774,
82.6449938270835));
#59766=CARTESIAN_POINT('Ctrl Pts',(-7.91095410811255,0.349320069428504,
82.6327410013806));
#59767=CARTESIAN_POINT('Ctrl Pts',(-7.88790906178625,0.697220106659238,
82.6200633058441));
#59768=CARTESIAN_POINT('Ctrl Pts',(-7.84031239578766,1.0552673544758,82.6056534138883));
#59769=CARTESIAN_POINT('Ctrl Pts',(-7.83857994710769,1.06805995277639,82.605136902858));
#59770=CARTESIAN_POINT('Ctrl Pts',(-7.8358192623798,1.0880766201622,82.6043261674288));
#59771=CARTESIAN_POINT('Ctrl Pts',(-7.83481232507473,1.09530364481255,82.6040329310423));
#59772=CARTESIAN_POINT('Ctrl Pts',(-7.83310538536042,1.1074319547877,82.6035399628812));
#59773=CARTESIAN_POINT('Ctrl Pts',(-7.83241077663093,1.11233400496469,82.6033404772588));
#59774=CARTESIAN_POINT('Ctrl Pts',(-7.83103186182475,1.12200006380831,82.6029466609751));
#59775=CARTESIAN_POINT('Ctrl Pts',(-7.83034780909842,1.12676410685477,82.6027523418164));
#59776=CARTESIAN_POINT('Ctrl Pts',(-7.82903972718962,1.13581544294007,82.6023827317705));
#59777=CARTESIAN_POINT('Ctrl Pts',(-7.82841652253502,1.14010285497647,82.6022074777285));
#59778=CARTESIAN_POINT('Ctrl Pts',(-7.82699214290545,1.14984581568054,82.6018088184936));
#59779=CARTESIAN_POINT('Ctrl Pts',(-7.8261887859552,1.15530103925643,82.601585316975));
#59780=CARTESIAN_POINT('Ctrl Pts',(-7.82410022827398,1.16938131561839,82.6010077129413));
#59781=CARTESIAN_POINT('Ctrl Pts',(-7.82280647093958,1.17800507670697,82.600653237421));
#59782=CARTESIAN_POINT('Ctrl Pts',(-7.81504522389425,1.22916234804201,82.5985462948037));
#59783=CARTESIAN_POINT('Ctrl Pts',(-7.80824519577419,1.27164412977541,82.5967796408973));
#59784=CARTESIAN_POINT('Ctrl Pts',(-7.74055447517696,1.67349709365284,82.5799189930328));
#59785=CARTESIAN_POINT('Ctrl Pts',(-7.6552444295412,2.02829509620599,82.5639209969348));
#59786=CARTESIAN_POINT('Ctrl Pts',(-7.53364049099852,2.41450153487727,82.5459902384341));
#59787=CARTESIAN_POINT('Ctrl Pts',(-7.52119826841894,2.45298457133671,82.5441974417473));
#59788=CARTESIAN_POINT('Ctrl Pts',(-7.31680728128888,3.06897560740725,82.5154133272331));
#59789=CARTESIAN_POINT('Ctrl Pts',(-7.05912230764937,3.62259623559259,82.4885337622097));
#59790=CARTESIAN_POINT('Ctrl Pts',(-6.67075725325308,4.25472275394273,82.4577336694805));
#59791=CARTESIAN_POINT('Ctrl Pts',(-6.59816353232833,4.36645251706056,82.4522747302298));
#59792=CARTESIAN_POINT('Ctrl Pts',(-6.50698590993662,4.49931490619557,82.4457558860335));
#59793=CARTESIAN_POINT('Ctrl Pts',(-6.4910688198935,4.52224787537569,82.4446296545503));
#59794=CARTESIAN_POINT('Ctrl Pts',(-6.46775471402853,4.55546159448804,82.442996879238));
#59795=CARTESIAN_POINT('Ctrl Pts',(-6.46045392627537,4.56580950625715,82.442487943421));
#59796=CARTESIAN_POINT('Ctrl Pts',(-6.44763347937972,4.58388849668556,82.441598342086));
#59797=CARTESIAN_POINT('Ctrl Pts',(-6.44212469200145,4.59162723744189,82.441217407596));
#59798=CARTESIAN_POINT('Ctrl Pts',(-6.43145803269192,4.60655477069941,82.4404823318367));
#59799=CARTESIAN_POINT('Ctrl Pts',(-6.4263020124273,4.61374487019525,82.4401281456488));
#59800=CARTESIAN_POINT('Ctrl Pts',(-6.41408181961623,4.63072577172773,82.4392913653364));
#59801=CARTESIAN_POINT('Ctrl Pts',(-6.40700726891939,4.64050909047417,82.4388090317134));
#59802=CARTESIAN_POINT('Ctrl Pts',(-6.38220596218085,4.67464171673893,82.4371254101558));
#59803=CARTESIAN_POINT('Ctrl Pts',(-6.36436250542876,4.69890604717129,82.435927076478));
#59804=CARTESIAN_POINT('Ctrl Pts',(-6.11820406375286,5.02966885131248,82.4195708628429));
#59805=CARTESIAN_POINT('Ctrl Pts',(-5.86810265449696,5.31934104552486,82.4050343347008));
#59806=CARTESIAN_POINT('Ctrl Pts',(-5.42488588443359,5.76320895976115,82.3818462421943));
#59807=CARTESIAN_POINT('Ctrl Pts',(-5.24378071055835,5.92846786234193,82.3729589097175));
#59808=CARTESIAN_POINT('Ctrl Pts',(-4.98502196560202,6.14343746088104,82.3607908954917));
#59809=CARTESIAN_POINT('Ctrl Pts',(-4.91374205154513,6.20059729883503,82.3574899009976));
#59810=CARTESIAN_POINT('Ctrl Pts',(-4.65517115362206,6.40068776760248,82.345654461163));
#59811=CARTESIAN_POINT('Ctrl Pts',(-4.46251075846352,6.53646808519185,82.3370937673916));
#59812=CARTESIAN_POINT('Ctrl Pts',(-4.1277686526447,6.75067687240102,82.3222593284048));
#59813=CARTESIAN_POINT('Ctrl Pts',(-3.98881273478963,6.83370189781156,82.3161110370332));
#59814=CARTESIAN_POINT('Ctrl Pts',(-3.80805868169157,6.93430881401271,82.308019196914));
#59815=CARTESIAN_POINT('Ctrl Pts',(-3.76851769623517,6.9558769338767,82.3062434169424));
#59816=CARTESIAN_POINT('Ctrl Pts',(-3.70473674296157,6.98996357603652,82.3033670011697));
#59817=CARTESIAN_POINT('Ctrl Pts',(-3.68061213539441,7.00269658145944,82.3022762865488));
#59818=CARTESIAN_POINT('Ctrl Pts',(-3.65127064892156,7.0179895553017,82.300945890571));
#59819=CARTESIAN_POINT('Ctrl Pts',(-3.64611598531127,7.02066898318087,82.300712026446));
#59820=CARTESIAN_POINT('Ctrl Pts',(-3.63709290071563,7.02534662412765,82.3003023982281));
#59821=CARTESIAN_POINT('Ctrl Pts',(-3.63322576852647,7.02734732828695,82.3001267567561));
#59822=CARTESIAN_POINT('Ctrl Pts',(-3.62544207191943,7.0313661685012,82.2997730599499));
#59823=CARTESIAN_POINT('Ctrl Pts',(-3.6215254693127,7.03338422719767,82.2995950008692));
#59824=CARTESIAN_POINT('Ctrl Pts',(-3.61399856992614,7.03725456423063,82.2992526399619));
#59825=CARTESIAN_POINT('Ctrl Pts',(-3.61038852870959,7.03910733949198,82.2990883630479));
#59826=CARTESIAN_POINT('Ctrl Pts',(-3.60189258473144,7.04345944311424,82.2987015725752));
#59827=CARTESIAN_POINT('Ctrl Pts',(-3.59700550815519,7.04595646401543,82.2984789429059));
#59828=CARTESIAN_POINT('Ctrl Pts',(-3.58016239491584,7.05454025588007,82.2977111708477));
#59829=CARTESIAN_POINT('Ctrl Pts',(-3.56819352276807,7.06060167241029,82.2971647390002));
#59830=CARTESIAN_POINT('Ctrl Pts',(-3.40576436646243,7.1423424558724,82.2897369962797));
#59831=CARTESIAN_POINT('Ctrl Pts',(-3.25296393131615,7.21321691824653,82.2825836462355));
#59832=CARTESIAN_POINT('Ctrl Pts',(-2.94790826134799,7.34304961336763,82.2681025797864));
#59833=CARTESIAN_POINT('Ctrl Pts',(-2.79584831437437,7.40228133953197,82.2607973658941));
#59834=CARTESIAN_POINT('Ctrl Pts',(-2.41032368413647,7.53887992847459,82.2422404171352));
#59835=CARTESIAN_POINT('Ctrl Pts',(-2.17487643449026,7.61014324717112,82.230878467541));
#59836=CARTESIAN_POINT('Ctrl Pts',(-1.90660174055661,7.67787350055613,82.2181281060756));
#59837=CARTESIAN_POINT('Ctrl Pts',(-1.87666264549439,7.68524619038826,82.2167078085039));
#59838=CARTESIAN_POINT('Ctrl Pts',(-1.81218739967203,7.70072439578925,82.2136554823284));
#59839=CARTESIAN_POINT('Ctrl Pts',(-1.77763824057219,7.70877303385118,82.2120237930571));
#59840=CARTESIAN_POINT('Ctrl Pts',(-1.70287219656382,7.72566131299856,82.2085021950472));
#59841=CARTESIAN_POINT('Ctrl Pts',(-1.66263799748794,7.73441991057805,82.2066129895662));
#59842=CARTESIAN_POINT('Ctrl Pts',(-1.57495953243013,7.75279089423254,82.20251033634));
#59843=CARTESIAN_POINT('Ctrl Pts',(-1.52749159201165,7.76228276113119,82.2002982916322));
#59844=CARTESIAN_POINT('Ctrl Pts',(-1.3224718239828,7.80132581797672,82.1907877401182));
#59845=CARTESIAN_POINT('Ctrl Pts',(-1.16412556602665,7.82652097633264,82.183553830554));
#59846=CARTESIAN_POINT('Ctrl Pts',(-0.829913214686822,7.86933070682043,
82.1685803218436));
#59847=CARTESIAN_POINT('Ctrl Pts',(-0.653999002608167,7.88589955955905,
82.1608688060668));
#59848=CARTESIAN_POINT('Ctrl Pts',(-0.301288779858691,7.90723531783254,
82.1457861087256));
#59849=CARTESIAN_POINT('Ctrl Pts',(-0.124592729063699,7.91199262744486,
82.1384193394991));
#59850=CARTESIAN_POINT('Ctrl Pts',(0.0837537802743487,7.91061987934015,
82.1299555262898));
#59851=CARTESIAN_POINT('Ctrl Pts',(0.115383602226224,7.91022175582863,82.1286765980149));
#59852=CARTESIAN_POINT('Ctrl Pts',(0.157109611807178,7.90944622577944,82.1269972528528));
#59853=CARTESIAN_POINT('Ctrl Pts',(0.167208445084067,7.90923917741232,82.1265914093773));
#59854=CARTESIAN_POINT('Ctrl Pts',(0.183733645094483,7.9088687099825,82.125928292224));
#59855=CARTESIAN_POINT('Ctrl Pts',(0.190160243090846,7.90871679896842,82.1256706515571));
#59856=CARTESIAN_POINT('Ctrl Pts',(0.202573040155221,7.90840824833334,82.1251734945852));
#59857=CARTESIAN_POINT('Ctrl Pts',(0.208559259209332,7.90825264483315,82.1249339453727));
#59858=CARTESIAN_POINT('Ctrl Pts',(0.222321433810788,7.90787927909634,82.1243837103068));
#59859=CARTESIAN_POINT('Ctrl Pts',(0.230097262210041,7.90765684403865,82.124073173937));
#59860=CARTESIAN_POINT('Ctrl Pts',(0.250812185412887,7.90703369335008,82.1232468407919));
#59861=CARTESIAN_POINT('Ctrl Pts',(0.26375067119878,7.90661268595191,82.1227316929069));
#59862=CARTESIAN_POINT('Ctrl Pts',(0.305369780605691,7.90515616184067,82.1210777433349));
#59863=CARTESIAN_POINT('Ctrl Pts',(0.334045972032011,7.90399632825828,82.1199429182862));
#59864=CARTESIAN_POINT('Ctrl Pts',(0.874073467301036,7.87921027005688,82.0986602074372));
#59865=CARTESIAN_POINT('Ctrl Pts',(1.3819583440441,7.8061659753496,82.0802488480511));
#59866=CARTESIAN_POINT('Ctrl Pts',(2.15421160008185,7.61730952218602,82.0528403729028));
#59867=CARTESIAN_POINT('Ctrl Pts',(2.42534357515986,7.53536604268906,82.0433097326995));
#59868=CARTESIAN_POINT('Ctrl Pts',(2.99689470121121,7.32857547383105,82.0226135272198));
#59869=CARTESIAN_POINT('Ctrl Pts',(3.29518107289733,7.19938578169494,82.0114331868785));
#59870=CARTESIAN_POINT('Ctrl Pts',(3.70359435723555,6.99178863742319,81.9945814472455));
#59871=CARTESIAN_POINT('Ctrl Pts',(3.82097006817931,6.92834065138982,81.9895466769319));
#59872=CARTESIAN_POINT('Ctrl Pts',(3.96840654540199,6.84375688820602,81.982907472444));
#59873=CARTESIAN_POINT('Ctrl Pts',(4.00000589031312,6.82533601028318,81.9814656651118));
#59874=CARTESIAN_POINT('Ctrl Pts',(4.04394021224102,6.79931455506815,81.979433068216));
#59875=CARTESIAN_POINT('Ctrl Pts',(4.05638415891133,6.79189799754665,81.978854199899));
#59876=CARTESIAN_POINT('Ctrl Pts',(4.07788924572791,6.77900084381976,81.9778482342665));
#59877=CARTESIAN_POINT('Ctrl Pts',(4.08695991682346,6.77353613536682,81.9774221974106));
#59878=CARTESIAN_POINT('Ctrl Pts',(4.09994029212038,6.76568042429072,81.9768100090196));
#59879=CARTESIAN_POINT('Ctrl Pts',(4.103858967697,6.76330419067953,81.9766248644763));
#59880=CARTESIAN_POINT('Ctrl Pts',(4.11061535042323,6.75919917461946,81.9763050750291));
#59881=CARTESIAN_POINT('Ctrl Pts',(4.11345403030612,6.75747201117102,81.9761705413588));
#59882=CARTESIAN_POINT('Ctrl Pts',(4.1189039063083,6.7541513877057,81.9759119197916));
#59883=CARTESIAN_POINT('Ctrl Pts',(4.12151526368354,6.75255820327548,81.9757878509932));
#59884=CARTESIAN_POINT('Ctrl Pts',(4.12765789835115,6.74880570225403,81.9754956599812));
#59885=CARTESIAN_POINT('Ctrl Pts',(4.13118840324481,6.74664512994146,81.9753274519744));
#59886=CARTESIAN_POINT('Ctrl Pts',(4.14334745438269,6.73919100085089,81.9747472180452));
#59887=CARTESIAN_POINT('Ctrl Pts',(4.15196750299662,6.7338836733282,81.9743342584221));
#59888=CARTESIAN_POINT('Ctrl Pts',(4.24571417215149,6.67591580603044,81.9698258428693));
#59889=CARTESIAN_POINT('Ctrl Pts',(4.32984089714907,6.62166269762062,81.9656245351131));
#59890=CARTESIAN_POINT('Ctrl Pts',(4.53171736565351,6.48598098442369,81.9552078245128));
#59891=CARTESIAN_POINT('Ctrl Pts',(4.64832868325318,6.40292500012817,81.9489054984122));
#59892=CARTESIAN_POINT('Ctrl Pts',(4.90792516191172,6.20719814018196,81.9343374883738));
#59893=CARTESIAN_POINT('Ctrl Pts',(5.04940558820169,6.09266260456133,81.9260079742405));
#59894=CARTESIAN_POINT('Ctrl Pts',(5.5297986120203,5.67552586657647,81.896665140721));
#59895=CARTESIAN_POINT('Ctrl Pts',(5.84652500511829,5.34868736937799,81.8754335022059));
#59896=CARTESIAN_POINT('Ctrl Pts',(6.1833718575868,4.93518793006913,81.8515965513555));
#59897=CARTESIAN_POINT('Ctrl Pts',(6.23236844565009,4.87316646557918,81.8480914667673));
#59898=CARTESIAN_POINT('Ctrl Pts',(6.35058417694355,4.71882539065852,81.839545740501));
#59899=CARTESIAN_POINT('Ctrl Pts',(6.41872967928759,4.62570461524448,81.8345412191565));
#59900=CARTESIAN_POINT('Ctrl Pts',(6.56249727213864,4.41994852158946,81.8238169689341));
#59901=CARTESIAN_POINT('Ctrl Pts',(6.63730918255846,4.30679052976544,81.818127790235));
#59902=CARTESIAN_POINT('Ctrl Pts',(6.74620071198438,4.13250277755704,81.8096762095788));
#59903=CARTESIAN_POINT('Ctrl Pts',(6.78243791215391,4.07275576964116,81.8068324143941));
#59904=CARTESIAN_POINT('Ctrl Pts',(6.82452177268674,4.00124918917944,81.8034909722707));
#59905=CARTESIAN_POINT('Ctrl Pts',(6.83113607104152,3.98994642581898,81.8029646240616));
#59906=CARTESIAN_POINT('Ctrl Pts',(6.8412715600567,3.97252743811785,81.8021562414801));
#59907=CARTESIAN_POINT('Ctrl Pts',(6.84481266796036,3.96642286524181,81.8018734647728));
#59908=CARTESIAN_POINT('Ctrl Pts',(6.85125020235128,3.9552908021355,81.8013587580069));
#59909=CARTESIAN_POINT('Ctrl Pts',(6.85414927366205,3.95026485178207,81.8011267296217));
#59910=CARTESIAN_POINT('Ctrl Pts',(6.86045186064145,3.93931059911893,81.8006217829872));
#59911=CARTESIAN_POINT('Ctrl Pts',(6.86385322853061,3.93338106290382,81.8003489446296));
#59912=CARTESIAN_POINT('Ctrl Pts',(6.87308674181776,3.91723601658111,81.7996073824649));
#59913=CARTESIAN_POINT('Ctrl Pts',(6.87890380579557,3.90701187640129,81.7991392180383));
#59914=CARTESIAN_POINT('Ctrl Pts',(6.9064701849403,3.85830847211923,81.7969159116814));
#59915=CARTESIAN_POINT('Ctrl Pts',(6.92791976770768,3.81965999222267,81.7951718547462));
#59916=CARTESIAN_POINT('Ctrl Pts',(7.26051732100637,3.20835687556068,81.7678973235601));
#59917=CARTESIAN_POINT('Ctrl Pts',(7.50005253087681,2.59960697854877,81.7453148272109));
#59918=CARTESIAN_POINT('Ctrl Pts',(7.74077814414052,1.66251646614667,81.7122072572788));
#59919=CARTESIAN_POINT('Ctrl Pts',(7.80095448329226,1.35229551315584,81.701442421204));
#59920=CARTESIAN_POINT('Ctrl Pts',(7.86159249353426,0.894737971947177,81.6849281755559));
#59921=CARTESIAN_POINT('Ctrl Pts',(7.87675082844901,0.749657155091485,81.6795977920532));
#59922=CARTESIAN_POINT('Ctrl Pts',(7.89423124280928,0.521466039641838,81.6709572232594));
#59923=CARTESIAN_POINT('Ctrl Pts',(7.89926886042242,0.438593681160197,81.6677662677672));
#59924=CARTESIAN_POINT('Ctrl Pts',(7.90500286083162,0.311180342830223,81.6627586655194));
#59925=CARTESIAN_POINT('Ctrl Pts',(7.90662899877267,0.266685518775396,81.6609909131456));
#59926=CARTESIAN_POINT('Ctrl Pts',(7.90809181614032,0.214620639765248,81.6588977602746));
#59927=CARTESIAN_POINT('Ctrl Pts',(7.90829336875327,0.207060824881036,81.6585932267067));
#59928=CARTESIAN_POINT('Ctrl Pts',(7.90858665969487,0.195434367222767,81.6581239265766));
#59929=CARTESIAN_POINT('Ctrl Pts',(7.90868610189198,0.19136793727716,81.6579596077544));
#59930=CARTESIAN_POINT('Ctrl Pts',(7.90886177919013,0.183949982951515,81.6576595360611));
#59931=CARTESIAN_POINT('Ctrl Pts',(7.9089390203217,0.180598480971753,81.6575238407844));
#59932=CARTESIAN_POINT('Ctrl Pts',(7.90910144913942,0.173350672660625,81.6572301341967));
#59933=CARTESIAN_POINT('Ctrl Pts',(7.90918588800026,0.169454352100039,81.6570720803693));
#59934=CARTESIAN_POINT('Ctrl Pts',(7.90940704302016,0.158889024909371,81.656643064766));
#59935=CARTESIAN_POINT('Ctrl Pts',(7.90953820336808,0.152219917756961,81.6563717899213));
#59936=CARTESIAN_POINT('Ctrl Pts',(7.91011513058217,0.120867959138215,81.6550943282579));
#59937=CARTESIAN_POINT('Ctrl Pts',(7.9104537891038,0.0961835106746757,81.6540821916067));
#59938=CARTESIAN_POINT('Ctrl Pts',(7.91399145912493,-0.295230367590466,
81.6379368962473));
#59939=CARTESIAN_POINT('Ctrl Pts',(7.89179994655053,-0.661715260893554,
81.6214970964371));
#59940=CARTESIAN_POINT('Ctrl Pts',(7.77738821514561,-1.53704646598482,81.5810738179645));
#59941=CARTESIAN_POINT('Ctrl Pts',(7.66057470335867,-2.04106300048223,81.5569111373424));
#59942=CARTESIAN_POINT('Ctrl Pts',(7.43576308455397,-2.70707035110996,81.5256533045396));
#59943=CARTESIAN_POINT('Ctrl Pts',(7.3697813278697,-2.88186249507884,81.5175034262463));
#59944=CARTESIAN_POINT('Ctrl Pts',(7.2516506401699,-3.16412607353471,81.50446478609));
#59945=CARTESIAN_POINT('Ctrl Pts',(7.20314902896742,-3.27303780911606,81.4994641214581));
#59946=CARTESIAN_POINT('Ctrl Pts',(7.11809171708981,-3.45297878506476,81.4912528491654));
#59947=CARTESIAN_POINT('Ctrl Pts',(7.08288946110985,-3.52462332043045,81.4879971489856));
#59948=CARTESIAN_POINT('Ctrl Pts',(7.04025243632213,-3.60817989743418,81.4842149562247));
#59949=CARTESIAN_POINT('Ctrl Pts',(7.03386357397253,-3.620618699161,81.4836523010286));
#59950=CARTESIAN_POINT('Ctrl Pts',(7.02403480044597,-3.63963063493679,81.4827928981793));
#59951=CARTESIAN_POINT('Ctrl Pts',(7.02061858347789,-3.64621594839851,81.4824953269814));
#59952=CARTESIAN_POINT('Ctrl Pts',(7.01437810045636,-3.6582042086026,81.4819538046204));
#59953=CARTESIAN_POINT('Ctrl Pts',(7.01155684438841,-3.66360871083721,81.4817097488941));
#59954=CARTESIAN_POINT('Ctrl Pts',(7.00545121895645,-3.67527198693532,81.481183212731));
#59955=CARTESIAN_POINT('Ctrl Pts',(7.0021647020214,-3.68152963389216,81.480900807466));
#59956=CARTESIAN_POINT('Ctrl Pts',(6.99325151252046,-3.69844555732297,81.4801376514594));
#59957=CARTESIAN_POINT('Ctrl Pts',(6.98760885257729,-3.70909541301738,81.4796574593718));
#59958=CARTESIAN_POINT('Ctrl Pts',(6.96117166444038,-3.75871804512183,81.4774212610621));
#59959=CARTESIAN_POINT('Ctrl Pts',(6.94007509879729,-3.79752945829967,81.4756758415387));
#59960=CARTESIAN_POINT('Ctrl Pts',(6.60228843886009,-4.40673960485565,81.4483290604531));
#59961=CARTESIAN_POINT('Ctrl Pts',(6.21657185626718,-4.93597740523132,81.4255674108692));
#59962=CARTESIAN_POINT('Ctrl Pts',(5.39617753006396,-5.81069224921571,81.384051081077));
#59963=CARTESIAN_POINT('Ctrl Pts',(4.98183974493874,-6.16960362719655,81.3652417160758));
#59964=CARTESIAN_POINT('Ctrl Pts',(4.52238692721028,-6.49092706742245,81.3429133278599));
#59965=CARTESIAN_POINT('Ctrl Pts',(4.51087206895067,-6.49893459631084,81.3423528163554));
#59966=CARTESIAN_POINT('Ctrl Pts',(4.49076066454459,-6.51284103531373,81.3413721476225));
#59967=CARTESIAN_POINT('Ctrl Pts',(4.48217361027547,-6.51875367098348,81.3409528890094));
#59968=CARTESIAN_POINT('Ctrl Pts',(4.46972587013052,-6.527288366993,81.340344319096));
#59969=CARTESIAN_POINT('Ctrl Pts',(4.4658744831024,-6.52992403332532,81.3401559121244));
#59970=CARTESIAN_POINT('Ctrl Pts',(4.45912744427861,-6.53453255502487,81.3398256508177));
#59971=CARTESIAN_POINT('Ctrl Pts',(4.45623280413449,-6.53650690142316,81.339683896082));
#59972=CARTESIAN_POINT('Ctrl Pts',(4.45064438721672,-6.54031315388104,81.3394100965607));
#59973=CARTESIAN_POINT('Ctrl Pts',(4.44795079405254,-6.54214531678457,81.3392780698327));
#59974=CARTESIAN_POINT('Ctrl Pts',(4.44155164910195,-6.54649219072924,81.3389642825131));
#59975=CARTESIAN_POINT('Ctrl Pts',(4.43784509576301,-6.54900541768312,81.3387824231388));
#59976=CARTESIAN_POINT('Ctrl Pts',(4.4267384622008,-6.55652250718289,81.3382371735094));
#59977=CARTESIAN_POINT('Ctrl Pts',(4.41933206190127,-6.56151696830178,81.3378731641488));
#59978=CARTESIAN_POINT('Ctrl Pts',(4.34917346643827,-6.60865531771014,81.3344212421775));
#59979=CARTESIAN_POINT('Ctrl Pts',(4.28583049611086,-6.64990911498071,81.3312761720035));
#59980=CARTESIAN_POINT('Ctrl Pts',(4.12386226779007,-6.75211982522031,81.3231831251911));
#59981=CARTESIAN_POINT('Ctrl Pts',(4.02447166577212,-6.81182706739457,81.3181699788015));
#59982=CARTESIAN_POINT('Ctrl Pts',(3.83491235761234,-6.92010471198551,81.3085740730283));
#59983=CARTESIAN_POINT('Ctrl Pts',(3.74504054400367,-6.96915148181296,81.3040103501888));
#59984=CARTESIAN_POINT('Ctrl Pts',(3.06456111211367,-7.32355321466,81.2694837001809));
#59985=CARTESIAN_POINT('Ctrl Pts',(2.43841449632265,-7.55514848936832,81.2381622509165));
#59986=CARTESIAN_POINT('Ctrl Pts',(1.59277945183619,-7.75166147393109,81.2003219684324));
#59987=CARTESIAN_POINT('Ctrl Pts',(1.39316952355342,-7.79001209403564,81.1916719248529));
#59988=CARTESIAN_POINT('Ctrl Pts',(1.10158562245328,-7.83446548302403,81.1794604986999));
#59989=CARTESIAN_POINT('Ctrl Pts',(1.01064148290011,-7.84671554332603,81.175710527792));
#59990=CARTESIAN_POINT('Ctrl Pts',(0.905091670906483,-7.85906741221714,
81.1714246899081));
#59991=CARTESIAN_POINT('Ctrl Pts',(0.89067595719092,-7.86071420830755,81.1708407684653));
#59992=CARTESIAN_POINT('Ctrl Pts',(0.868772239969556,-7.86315537767869,
81.1699556926036));
#59993=CARTESIAN_POINT('Ctrl Pts',(0.861287535167033,-7.86397873093686,
81.1696536356744));
#59994=CARTESIAN_POINT('Ctrl Pts',(0.84773398997766,-7.86545010362807,81.1691073499916));
#59995=CARTESIAN_POINT('Ctrl Pts',(0.841665558142616,-7.86610178798091,
81.1688630072369));
#59996=CARTESIAN_POINT('Ctrl Pts',(0.829545608937983,-7.86738915444406,
81.1683755003018));
#59997=CARTESIAN_POINT('Ctrl Pts',(0.823494100307288,-7.86802487869369,
81.1681323349625));
#59998=CARTESIAN_POINT('Ctrl Pts',(0.806504612368069,-7.86978984627448,
81.1674503460731));
#59999=CARTESIAN_POINT('Ctrl Pts',(0.795564984225235,-7.87090326909271,
81.167012015533));
#60000=CARTESIAN_POINT('Ctrl Pts',(0.750909025319721,-7.87535424997989,
81.165226004247));
#60001=CARTESIAN_POINT('Ctrl Pts',(0.717173512987805,-7.87849802406941,
81.1638843621613));
#60002=CARTESIAN_POINT('Ctrl Pts',(0.192208215082014,-7.92401911144263,
81.1431226357622));
#60003=CARTESIAN_POINT('Ctrl Pts',(-0.301919590915243,-7.92060190416507,
81.1252561627711));
#60004=CARTESIAN_POINT('Ctrl Pts',(-1.22547250410126,-7.82760827199199,
81.0928928448127));
#60005=CARTESIAN_POINT('Ctrl Pts',(-1.65403558472917,-7.74837931732449,
81.0782745500247));
#60006=CARTESIAN_POINT('Ctrl Pts',(-2.22817757196753,-7.59241094609808,
81.0572537402212));
#60007=CARTESIAN_POINT('Ctrl Pts',(-2.38114519287338,-7.54583484475337,
81.05150305348));
#60008=CARTESIAN_POINT('Ctrl Pts',(-2.64809556645041,-7.45562710723083,
81.0410462382729));
#60009=CARTESIAN_POINT('Ctrl Pts',(-2.76267786097776,-7.41393245473913,
81.0364173770764));
#60010=CARTESIAN_POINT('Ctrl Pts',(-2.92530418273471,-7.3504618702623,81.0295868800997));
#60011=CARTESIAN_POINT('Ctrl Pts',(-2.97416865641587,-7.33082634086414,
81.0275002187845));
#60012=CARTESIAN_POINT('Ctrl Pts',(-3.03029653294313,-7.30761856971711,
81.0250598717806));
#60013=CARTESIAN_POINT('Ctrl Pts',(-3.03775589137337,-7.30452088651751,
81.0247346599536));
#60014=CARTESIAN_POINT('Ctrl Pts',(-3.04905173236382,-7.29980971364017,
81.0242408163469));
#60015=CARTESIAN_POINT('Ctrl Pts',(-3.05289172582711,-7.29820460334164,
81.0240726952972));
#60016=CARTESIAN_POINT('Ctrl Pts',(-3.05953261170976,-7.29542256679272,
81.0237815283338));
#60017=CARTESIAN_POINT('Ctrl Pts',(-3.06233409940995,-7.2942470546128,81.0236585693276));
#60018=CARTESIAN_POINT('Ctrl Pts',(-3.06813841484015,-7.29180761415803,
81.0234035458553));
#60019=CARTESIAN_POINT('Ctrl Pts',(-3.07114113972537,-7.29054344437614,
81.0232714664692));
#60020=CARTESIAN_POINT('Ctrl Pts',(-3.07932436179535,-7.28709229359252,
81.0229111065713));
#60021=CARTESIAN_POINT('Ctrl Pts',(-3.08450326615387,-7.28490166174089,
81.0226825985884));
#60022=CARTESIAN_POINT('Ctrl Pts',(-3.1044640648564,-7.27643331470342,81.021800144467));
#60023=CARTESIAN_POINT('Ctrl Pts',(-3.11922904227979,-7.27011616744074,
81.0211437471184));
#60024=CARTESIAN_POINT('Ctrl Pts',(-3.36486126244534,-7.16413720416248,
81.0101643522225));
#60025=CARTESIAN_POINT('Ctrl Pts',(-3.59084958190917,-7.0535758314352,80.999189517539));
#60026=CARTESIAN_POINT('Ctrl Pts',(-4.36283522614617,-6.6291707388327,80.9596049269533));
#60027=CARTESIAN_POINT('Ctrl Pts',(-4.87634183917102,-6.26112078069897,
80.9296437927232));
#60028=CARTESIAN_POINT('Ctrl Pts',(-5.49037197959168,-5.69919576410753,
80.8925336947381));
#60029=CARTESIAN_POINT('Ctrl Pts',(-5.63461226004034,-5.55663289245589,
80.8836819762504));
#60030=CARTESIAN_POINT('Ctrl Pts',(-5.88453970221659,-5.289860363415,80.868144174977));
#60031=CARTESIAN_POINT('Ctrl Pts',(-5.99216502846427,-5.16762931389496,
80.8613779520247));
#60032=CARTESIAN_POINT('Ctrl Pts',(-6.11505578713525,-5.01905495792445,
80.8535567561821));
#60033=CARTESIAN_POINT('Ctrl Pts',(-6.13403408823448,-4.99584284994719,
80.8523460403021));
#60034=CARTESIAN_POINT('Ctrl Pts',(-6.15906967581658,-4.96486441875541,
80.8507449640487));
#60035=CARTESIAN_POINT('Ctrl Pts',(-6.16524494942985,-4.95719403318566,
80.850349720776));
#60036=CARTESIAN_POINT('Ctrl Pts',(-6.17537119248089,-4.94456790870893,
80.8497010634125));
#60037=CARTESIAN_POINT('Ctrl Pts',(-6.17933054785953,-4.93961892753841,
80.8494473034487));
#60038=CARTESIAN_POINT('Ctrl Pts',(-6.18699811094366,-4.93001124028371,
80.8489556154404));
#60039=CARTESIAN_POINT('Ctrl Pts',(-6.19070701398151,-4.92535309611299,
80.8487176588349));
#60040=CARTESIAN_POINT('Ctrl Pts',(-6.19926698357264,-4.91457737996965,
80.8481681858024));
#60041=CARTESIAN_POINT('Ctrl Pts',(-6.20411426368553,-4.90845680035173,
80.8478568249644));
#60042=CARTESIAN_POINT('Ctrl Pts',(-6.21924007506219,-4.88929948894017,
80.8468845713691));
#60043=CARTESIAN_POINT('Ctrl Pts',(-6.22948666698175,-4.87623753257832,
80.846224986714));
#60044=CARTESIAN_POINT('Ctrl Pts',(-6.31687753247868,-4.76411003545732,
80.8405911631473));
#60045=CARTESIAN_POINT('Ctrl Pts',(-6.39169626818635,-4.66325067146858,
80.8357120954722));
#60046=CARTESIAN_POINT('Ctrl Pts',(-6.4672863453654,-4.55611228650474,80.8307114852019));
#60047=CARTESIAN_POINT('Ctrl Pts',(-6.47048307297478,-4.55157122790423,
80.8304998690554));
#60048=CARTESIAN_POINT('Ctrl Pts',(-6.47576475550273,-4.54405161173773,
80.8301500016519));
#60049=CARTESIAN_POINT('Ctrl Pts',(-6.47785244120307,-4.54107497942819,
80.8300116497182));
#60050=CARTESIAN_POINT('Ctrl Pts',(-6.48645134802723,-4.52879662026427,
80.8294415463273));
#60051=CARTESIAN_POINT('Ctrl Pts',(-6.49294460622107,-4.51948229998175,
80.8290104552015));
#60052=CARTESIAN_POINT('Ctrl Pts',(-6.50490073938982,-4.50225275424334,
80.8282155661346));
#60053=CARTESIAN_POINT('Ctrl Pts',(-6.51036927188469,-4.49434149090429,
80.827851563085));
#60054=CARTESIAN_POINT('Ctrl Pts',(-6.52786338850867,-4.46893402404727,
80.8266856811337));
#60055=CARTESIAN_POINT('Ctrl Pts',(-6.53983301452147,-4.45139931712575,
80.8258858156482));
#60056=CARTESIAN_POINT('Ctrl Pts',(-6.56062732757918,-4.42067211773139,
80.8244923210264));
#60057=CARTESIAN_POINT('Ctrl Pts',(-6.56948313153249,-4.40750091211186,
80.8238976027076));
#60058=CARTESIAN_POINT('Ctrl Pts',(-6.70908416530263,-4.19851729016821,
80.8145020049814));
#60059=CARTESIAN_POINT('Ctrl Pts',(-6.83106736452198,-3.99698444657958,
80.8060100437487));
#60060=CARTESIAN_POINT('Ctrl Pts',(-7.187272615697,-3.34441175087375,80.7798193897539));
#60061=CARTESIAN_POINT('Ctrl Pts',(-7.38713656546947,-2.87613696774115,
80.7629736062849));
#60062=CARTESIAN_POINT('Ctrl Pts',(-7.61070169582243,-2.17133736910167,
80.7369917311529));
#60063=CARTESIAN_POINT('Ctrl Pts',(-7.6709612878071,-1.94777499839659,80.7286477080544));
#60064=CARTESIAN_POINT('Ctrl Pts',(-7.74241611886805,-1.62735906029986,
80.7161514838298));
#60065=CARTESIAN_POINT('Ctrl Pts',(-7.76176176050609,-1.53243527661734,
80.7123834536608));
#60066=CARTESIAN_POINT('Ctrl Pts',(-7.78246294606769,-1.42038144426406,
80.7078330499648));
#60067=CARTESIAN_POINT('Ctrl Pts',(-7.78551259693344,-1.40356921755494,
80.7071476211443));
#60068=CARTESIAN_POINT('Ctrl Pts',(-7.78947481769972,-1.38131585850794,
80.7062366344355));
#60069=CARTESIAN_POINT('Ctrl Pts',(-7.79043621609811,-1.37588335230544,
80.7060139503231));
#60070=CARTESIAN_POINT('Ctrl Pts',(-7.79200267918132,-1.36697757020063,
80.7056484057416));
#60071=CARTESIAN_POINT('Ctrl Pts',(-7.79261110748777,-1.36350487977847,
80.705505745146));
#60072=CARTESIAN_POINT('Ctrl Pts',(-7.79378382686972,-1.35678499503354,
80.7052294506657));
#60073=CARTESIAN_POINT('Ctrl Pts',(-7.79434841031616,-1.35353785367166,
80.705095834296));
#60074=CARTESIAN_POINT('Ctrl Pts',(-7.79565230182544,-1.34601079240612,
80.704785854506));
#60075=CARTESIAN_POINT('Ctrl Pts',(-7.79639011228957,-1.34173062910365,
80.7046094022217));
#60076=CARTESIAN_POINT('Ctrl Pts',(-7.79877001337654,-1.3278561764917,80.7040368206264));
#60077=CARTESIAN_POINT('Ctrl Pts',(-7.80039791574616,-1.31825949697215,
80.7036398493334));
#60078=CARTESIAN_POINT('Ctrl Pts',(-7.81557074730891,-1.22780165033215,
80.6998894383681));
#60079=CARTESIAN_POINT('Ctrl Pts',(-7.82787512921349,-1.14674018072412,
80.6964640545968));
#60080=CARTESIAN_POINT('Ctrl Pts',(-7.83937863061201,-1.06210895486184,
80.6928315079482));
#60081=CARTESIAN_POINT('Ctrl Pts',(-7.83983802842581,-1.05871263054713,
80.6926856364009));
#60082=CARTESIAN_POINT('Ctrl Pts',(-7.88740827541019,-0.70529737362485,
80.6774967774005));
#60083=CARTESIAN_POINT('Ctrl Pts',(-7.91102585095933,-0.352541444084006,
80.6613572250108));
#60084=CARTESIAN_POINT('Ctrl Pts',(-7.91097302527927,0.368460252008101,
80.6278855848813));
#60085=CARTESIAN_POINT('Ctrl Pts',(-7.88528480223124,0.735903908438486,
80.6105801409096));
#60086=CARTESIAN_POINT('Ctrl Pts',(-7.7647871228187,1.59390167764492,80.5708910084427));
#60087=CARTESIAN_POINT('Ctrl Pts',(-7.64894176064335,2.07996464741413,80.5490279021577));
#60088=CARTESIAN_POINT('Ctrl Pts',(-7.47858398552469,2.57983930427977,80.5275386428139));
#60089=CARTESIAN_POINT('Ctrl Pts',(-7.46892284816607,2.60767727638752,80.5263449113696));
#60090=CARTESIAN_POINT('Ctrl Pts',(-7.45482773537717,2.64757046849945,80.5246384437715));
#60091=CARTESIAN_POINT('Ctrl Pts',(-7.45051964472956,2.65966971171014,80.5241214453457));
#60092=CARTESIAN_POINT('Ctrl Pts',(-7.44356514229715,2.67905188734254,80.5232941316661));
#60093=CARTESIAN_POINT('Ctrl Pts',(-7.44093747023545,2.68634149117227,80.5229831810283));
#60094=CARTESIAN_POINT('Ctrl Pts',(-7.43626178144472,2.69925314100821,80.5224327650337));
#60095=CARTESIAN_POINT('Ctrl Pts',(-7.434218090674,2.70487674061525,80.5221931530464));
#60096=CARTESIAN_POINT('Ctrl Pts',(-7.42996101121678,2.71654962490099,80.5216960363084));
#60097=CARTESIAN_POINT('Ctrl Pts',(-7.4277466098105,2.7225985369603,80.5214385661861));
#60098=CARTESIAN_POINT('Ctrl Pts',(-7.42202048169807,2.73818118342353,80.5207756454288));
#60099=CARTESIAN_POINT('Ctrl Pts',(-7.41849776757067,2.7477108831825,80.5203705685219));
#60100=CARTESIAN_POINT('Ctrl Pts',(-7.40376035055633,2.78734383314351,80.5186872883973));
#60101=CARTESIAN_POINT('Ctrl Pts',(-7.39238062322057,2.81738561890556,80.517414702715));
#60102=CARTESIAN_POINT('Ctrl Pts',(-7.31565623579296,3.01626782886262,80.5090111578946));
#60103=CARTESIAN_POINT('Ctrl Pts',(-7.24471322721281,3.18289697195793,80.5020739594106));
#60104=CARTESIAN_POINT('Ctrl Pts',(-7.02896788073465,3.64495519586056,80.4830193125638));
#60105=CARTESIAN_POINT('Ctrl Pts',(-6.87137100926708,3.93400125750296,80.4713285802795));
#60106=CARTESIAN_POINT('Ctrl Pts',(-6.32322044836416,4.80536571601678,80.4355112141084));
#60107=CARTESIAN_POINT('Ctrl Pts',(-5.87315429183166,5.34606978727673,80.4125810056982));
#60108=CARTESIAN_POINT('Ctrl Pts',(-5.32610102587594,5.849652584334,80.3833197247313));
#60109=CARTESIAN_POINT('Ctrl Pts',(-5.2940764730732,5.87865134837688,80.3816017613637));
#60110=CARTESIAN_POINT('Ctrl Pts',(-5.2552868516254,5.91320197274771,80.3795165511651));
#60111=CARTESIAN_POINT('Ctrl Pts',(-5.24874757090289,5.91900721400563,80.3791648729786));
#60112=CARTESIAN_POINT('Ctrl Pts',(-5.23806040854657,5.92846309666762,80.378589903719));
#60113=CARTESIAN_POINT('Ctrl Pts',(-5.23391829261839,5.93212026496742,80.3783670039762));
#60114=CARTESIAN_POINT('Ctrl Pts',(-5.22652062471598,5.93863805440755,80.3779688220293));
#60115=CARTESIAN_POINT('Ctrl Pts',(-5.22326654215742,5.94150035019,80.3777936385566));
#60116=CARTESIAN_POINT('Ctrl Pts',(-5.21639853891438,5.9475314530496,80.377423836425));
#60117=CARTESIAN_POINT('Ctrl Pts',(-5.21278408006506,5.95069964258606,80.3772291818897));
#60118=CARTESIAN_POINT('Ctrl Pts',(-5.20322519157263,5.95906292390791,80.37671430107));
#60119=CARTESIAN_POINT('Ctrl Pts',(-5.19727587847815,5.96425240643351,80.3763937523235));
#60120=CARTESIAN_POINT('Ctrl Pts',(-5.17031921012709,5.98769527960476,80.3749409382052));
#60121=CARTESIAN_POINT('Ctrl Pts',(-5.14922356154275,6.00584650001665,80.3738029313946));
#60122=CARTESIAN_POINT('Ctrl Pts',(-4.9874166050611,6.14359004184041,80.3650688046558));
#60123=CARTESIAN_POINT('Ctrl Pts',(-4.8426579324136,6.25832893909334,80.3572248425135));
#60124=CARTESIAN_POINT('Ctrl Pts',(-4.51884517720447,6.49702410034487,80.339822949134));
#60125=CARTESIAN_POINT('Ctrl Pts',(-4.33841510465881,6.61886956266665,80.3302174383871));
#60126=CARTESIAN_POINT('Ctrl Pts',(-3.58419945627548,7.08409313952916,80.2909412784782));
#60127=CARTESIAN_POINT('Ctrl Pts',(-2.97293497985739,7.36156924940989,80.261383389688));
#60128=CARTESIAN_POINT('Ctrl Pts',(-2.23454013695276,7.58957131826241,80.22953921955));
#60129=CARTESIAN_POINT('Ctrl Pts',(-2.13445455763394,7.61832441486272,80.2252925580171));
#60130=CARTESIAN_POINT('Ctrl Pts',(-2.01490932629076,7.6501271026298,80.2202975918372));
#60131=CARTESIAN_POINT('Ctrl Pts',(-1.99597116738945,7.6550900310333,80.2195085808122));
#60132=CARTESIAN_POINT('Ctrl Pts',(-1.9653586495349,7.66299101481573,80.2182368113831));
#60133=CARTESIAN_POINT('Ctrl Pts',(-1.95369570384629,7.66597280273699,80.2177531325557));
#60134=CARTESIAN_POINT('Ctrl Pts',(-1.93288015327237,7.67124398798022,80.2168913773492));
#60135=CARTESIAN_POINT('Ctrl Pts',(-1.92373018206954,7.67354365316913,80.2165130866736));
#60136=CARTESIAN_POINT('Ctrl Pts',(-1.9046589560219,7.67830057564779,80.2157256806043));
#60137=CARTESIAN_POINT('Ctrl Pts',(-1.89473700365983,7.68075498609132,80.2153166255628));
#60138=CARTESIAN_POINT('Ctrl Pts',(-1.86907625303962,7.68704998155722,80.2142602472231));
#60139=CARTESIAN_POINT('Ctrl Pts',(-1.85333034109061,7.69086146722528,80.2136135342467));
#60140=CARTESIAN_POINT('Ctrl Pts',(-1.78693152128647,7.70671833765004,80.2108927059853));
#60141=CARTESIAN_POINT('Ctrl Pts',(-1.73617170472421,7.71831197196389,80.2088281374913));
#60142=CARTESIAN_POINT('Ctrl Pts',(-1.39476922160644,7.79275055331919,80.1950433650332));
#60143=CARTESIAN_POINT('Ctrl Pts',(-1.10088901551697,7.83966834999513,80.18368072138));
#60144=CARTESIAN_POINT('Ctrl Pts',(-0.413876672078214,7.90994603746026,
80.1579272271261));
#60145=CARTESIAN_POINT('Ctrl Pts',(-0.0202562489549062,7.92074091160252,
80.1437905274532));
#60146=CARTESIAN_POINT('Ctrl Pts',(0.79281471282269,7.88241051422963,80.1143249393133));
#60147=CARTESIAN_POINT('Ctrl Pts',(1.21081823110053,7.82910078404111,80.0990223079734));
#60148=CARTESIAN_POINT('Ctrl Pts',(1.66717577250144,7.73346776203641,80.080629823665));
#60149=CARTESIAN_POINT('Ctrl Pts',(1.71170609035062,7.72373360667324,80.078816666842));
#60150=CARTESIAN_POINT('Ctrl Pts',(1.76482283271653,7.71164058428669,80.0766294569681));
#60151=CARTESIAN_POINT('Ctrl Pts',(1.77349314098979,7.70965123789846,80.0762716557538));
#60152=CARTESIAN_POINT('Ctrl Pts',(1.78752670113109,7.70640640204375,80.0756912392515));
#60153=CARTESIAN_POINT('Ctrl Pts',(1.7928920449785,7.70515992407334,80.0754690279908));
#60154=CARTESIAN_POINT('Ctrl Pts',(1.80248530329826,7.7029206533843,80.0750711613642));
#60155=CARTESIAN_POINT('Ctrl Pts',(1.80671371405332,7.70192997996482,80.0748956022065));
#60156=CARTESIAN_POINT('Ctrl Pts',(1.81558161612889,7.69984461651287,80.0745270100957));
#60157=CARTESIAN_POINT('Ctrl Pts',(1.82022093678821,7.69874921428125,80.0743339445756));
#60158=CARTESIAN_POINT('Ctrl Pts',(1.8323695314035,7.69586918252703,80.0738277631398));
#60159=CARTESIAN_POINT('Ctrl Pts',(1.83987717598649,7.69407775830387,80.0735143328916));
#60160=CARTESIAN_POINT('Ctrl Pts',(1.8728061548083,7.68616951198746,80.0721368548667));
#60161=CARTESIAN_POINT('Ctrl Pts',(1.89819947466377,7.67993772037388,80.0710674008728));
#60162=CARTESIAN_POINT('Ctrl Pts',(2.07326134877294,7.63605439377818,80.0636421880189));
#60163=CARTESIAN_POINT('Ctrl Pts',(2.22181352760151,7.59416050701445,80.0570619863029));
#60164=CARTESIAN_POINT('Ctrl Pts',(2.59909595537404,7.47574511436507,80.0397782292706));
#60165=CARTESIAN_POINT('Ctrl Pts',(2.82572908799643,7.39305820051112,80.0288544894765));
#60166=CARTESIAN_POINT('Ctrl Pts',(3.79551912462423,6.98811695278454,79.9806897665835));
#60167=CARTESIAN_POINT('Ctrl Pts',(4.49066904129472,6.56308956521699,79.943062755289));
#60168=CARTESIAN_POINT('Ctrl Pts',(5.14988420903908,6.00545201532558,79.9077090766996));
#60169=CARTESIAN_POINT('Ctrl Pts',(5.19022481684917,5.9706220591907,79.905544023911));
#60170=CARTESIAN_POINT('Ctrl Pts',(5.23886786168367,5.92775823250875,79.9029310894273));
#60171=CARTESIAN_POINT('Ctrl Pts',(5.2475081212879,5.92011086498983,79.9024668749909));
#60172=CARTESIAN_POINT('Ctrl Pts',(5.26168735917662,5.90750559830426,79.9017049138386));
#60173=CARTESIAN_POINT('Ctrl Pts',(5.26723612066034,5.90255875949788,79.9014066964705));
#60174=CARTESIAN_POINT('Ctrl Pts',(5.27719626087805,5.89365385397001,79.900871317809));
#60175=CARTESIAN_POINT('Ctrl Pts',(5.28161017616302,5.88969864029509,79.9006340348636));
#60176=CARTESIAN_POINT('Ctrl Pts',(5.29088511752214,5.88136875568284,79.9001353779689));
#60177=CARTESIAN_POINT('Ctrl Pts',(5.29574517358476,5.87699300866216,79.899874050452));
#60178=CARTESIAN_POINT('Ctrl Pts',(5.30850157049156,5.86547912628823,79.8991880464961));
#60179=CARTESIAN_POINT('Ctrl Pts',(5.3163889524539,5.8583310603127,79.8987637975312));
#60180=CARTESIAN_POINT('Ctrl Pts',(5.33370827804382,5.84257136242672,79.8978320194101));
#60181=CARTESIAN_POINT('Ctrl Pts',(5.34313385115761,5.83395275700235,79.8973247927922));
#60182=CARTESIAN_POINT('Ctrl Pts',(5.37084877399009,5.80848713224403,79.8958329352727));
#60183=CARTESIAN_POINT('Ctrl Pts',(5.38907968838866,5.79157659410226,79.8948510611496));
#60184=CARTESIAN_POINT('Ctrl Pts',(5.57668388104208,5.61590683165143,79.8847410443292));
#60185=CARTESIAN_POINT('Ctrl Pts',(5.73907712141885,5.44984559648409,79.8759429556149));
#60186=CARTESIAN_POINT('Ctrl Pts',(6.137684155715,5.00462620193725,79.8540118248301));
#60187=CARTESIAN_POINT('Ctrl Pts',(6.36228007263128,4.71580985524251,79.8413319640221));
#60188=CARTESIAN_POINT('Ctrl Pts',(6.93845064220596,3.85842570922307,79.8061025996344));
#60189=CARTESIAN_POINT('Ctrl Pts',(7.23911062469615,3.25953675898994,79.7843081166348));
#60190=CARTESIAN_POINT('Ctrl Pts',(7.46355999082669,2.62283303601201,79.7577483753527));
#60191=CARTESIAN_POINT('Ctrl Pts',(7.46612177787413,2.61553177550486,79.7574433585223));
#60192=CARTESIAN_POINT('Ctrl Pts',(7.47995227390394,2.57592806833074,79.7557863888887));
#60193=CARTESIAN_POINT('Ctrl Pts',(7.49102190842974,2.54355698439586,79.7544230541428));
#60194=CARTESIAN_POINT('Ctrl Pts',(7.50399967711359,2.50478629713728,79.7527784216497));
#60195=CARTESIAN_POINT('Ctrl Pts',(7.50611027313306,2.49845434529178,79.7525094493681));
#60196=CARTESIAN_POINT('Ctrl Pts',(7.50951356640925,2.48820096548872,79.7520732842098));
#60197=CARTESIAN_POINT('Ctrl Pts',(7.51081121467751,2.48428117290919,79.7519063958055));
#60198=CARTESIAN_POINT('Ctrl Pts',(7.51312968093741,2.47725938526742,79.7516071738112));
#60199=CARTESIAN_POINT('Ctrl Pts',(7.51415164659003,2.47415777516295,79.7514749115497));
#60200=CARTESIAN_POINT('Ctrl Pts',(7.51630450244715,2.46761033779156,79.7511955151536));
#60201=CARTESIAN_POINT('Ctrl Pts',(7.51743494458023,2.46416436274076,79.7510483533837));
#60202=CARTESIAN_POINT('Ctrl Pts',(7.52041961663174,2.45504489094875,79.7506586063866));
#60203=CARTESIAN_POINT('Ctrl Pts',(7.52226979280268,2.44937008038857,79.7504157737379));
#60204=CARTESIAN_POINT('Ctrl Pts',(7.53064390351867,2.42358625453281,79.7493110923044));
#60205=CARTESIAN_POINT('Ctrl Pts',(7.53709358235142,2.40345340066538,79.7484447730924));
#60206=CARTESIAN_POINT('Ctrl Pts',(7.58456167742715,2.25321024023933,79.7419532894421));
#60207=CARTESIAN_POINT('Ctrl Pts',(7.6222871205614,2.12209035710128,79.7361404023714));
#60208=CARTESIAN_POINT('Ctrl Pts',(7.71029246483093,1.78349794802351,79.7208791567034));
#60209=CARTESIAN_POINT('Ctrl Pts',(7.75559910892461,1.57484880563962,79.7112388799914));
#60210=CARTESIAN_POINT('Ctrl Pts',(7.83521536941418,1.12021955223917,79.6900906088558));
#60211=CARTESIAN_POINT('Ctrl Pts',(7.86649478672846,0.873928003626052,79.6785473503489));
#60212=CARTESIAN_POINT('Ctrl Pts',(7.92227047051475,0.171929409369034,79.645990134639));
#60213=CARTESIAN_POINT('Ctrl Pts',(7.91901289184965,-0.285028556764483,
79.6252614688054));
#60214=CARTESIAN_POINT('Ctrl Pts',(7.85752424863358,-0.940210731153474,
79.5971025091756));
#60215=CARTESIAN_POINT('Ctrl Pts',(7.83097021654703,-1.14043727857879,79.5886983746942));
#60216=CARTESIAN_POINT('Ctrl Pts',(7.79360045864102,-1.35796397947993,79.5797841820767));
#60217=CARTESIAN_POINT('Ctrl Pts',(7.79035206873331,-1.37647699952185,79.5790272203026));
#60218=CARTESIAN_POINT('Ctrl Pts',(7.78570466647016,-1.40241969362595,79.5779688274373));
#60219=CARTESIAN_POINT('Ctrl Pts',(7.78436094857258,-1.40985913243631,79.5776655898506));
#60220=CARTESIAN_POINT('Ctrl Pts',(7.78201350263977,-1.42275000262988,79.5771406161085));
#60221=CARTESIAN_POINT('Ctrl Pts',(7.78101470618975,-1.42820232022114,79.5769187188093));
#60222=CARTESIAN_POINT('Ctrl Pts',(7.77894956359659,-1.43940923275327,79.5764629199714));
#60223=CARTESIAN_POINT('Ctrl Pts',(7.77788256023152,-1.44516370413895,79.5762290400876));
#60224=CARTESIAN_POINT('Ctrl Pts',(7.77537362948569,-1.45861138978029,79.5756828596188));
#60225=CARTESIAN_POINT('Ctrl Pts',(7.7739266672065,-1.46630366495492,79.5753707240387));
#60226=CARTESIAN_POINT('Ctrl Pts',(7.77085231195023,-1.48251494672703,79.5747135089549));
#60227=CARTESIAN_POINT('Ctrl Pts',(7.76922232038534,-1.49103345316784,79.5743685149121));
#60228=CARTESIAN_POINT('Ctrl Pts',(7.76481981989393,-1.51383815043945,79.5734458736839));
#60229=CARTESIAN_POINT('Ctrl Pts',(7.76202188779973,-1.52811943166562,79.5728690588144));
#60230=CARTESIAN_POINT('Ctrl Pts',(7.75337808704979,-1.57160306193506,79.5711157304031));
#60231=CARTESIAN_POINT('Ctrl Pts',(7.74740668009732,-1.60078034200157,79.5699433247036));
#60232=CARTESIAN_POINT('Ctrl Pts',(7.70046947317296,-1.82370714750096,79.5610158764868));
#60233=CARTESIAN_POINT('Ctrl Pts',(7.65240509641148,-2.01589699467982,79.5534969407213));
#60234=CARTESIAN_POINT('Ctrl Pts',(7.54323288431402,-2.39185658241609,79.5390347286315));
#60235=CARTESIAN_POINT('Ctrl Pts',(7.48249259642664,-2.57558716398644,79.5320869407689));
#60236=CARTESIAN_POINT('Ctrl Pts',(7.14228368897107,-3.49062358935137,79.4976913598856));
#60237=CARTESIAN_POINT('Ctrl Pts',(6.76216051405794,-4.1796506963553,79.4728900337485));
#60238=CARTESIAN_POINT('Ctrl Pts',(6.24808266806303,-4.8527865246023,79.4400027022402));
#60239=CARTESIAN_POINT('Ctrl Pts',(6.20834487169694,-4.90352195937002,79.4374612513421));
#60240=CARTESIAN_POINT('Ctrl Pts',(6.16283406394189,-4.96018801741824,79.434544334826));
#60241=CARTESIAN_POINT('Ctrl Pts',(6.15766540368655,-4.96660302853843,79.4342129715344));
#60242=CARTESIAN_POINT('Ctrl Pts',(6.14983351659487,-4.97629244847395,79.4337107140808));
#60243=CARTESIAN_POINT('Ctrl Pts',(6.14717766843573,-4.97957282575399,79.4335403678943));
#60244=CARTESIAN_POINT('Ctrl Pts',(6.14253857056091,-4.985293451475,79.4332427707029));
#60245=CARTESIAN_POINT('Ctrl Pts',(6.14055648427698,-4.9877346512719,79.4331156059192));
#60246=CARTESIAN_POINT('Ctrl Pts',(6.13640407572047,-4.99284266141862,79.4328491709072));
#60247=CARTESIAN_POINT('Ctrl Pts',(6.13423346986049,-4.99550923924397,79.4327098797955));
#60248=CARTESIAN_POINT('Ctrl Pts',(6.12907387219671,-5.00183934415124,79.4323787433379));
#60249=CARTESIAN_POINT('Ctrl Pts',(6.12608333591701,-5.00550160491037,79.4321867849442));
#60250=CARTESIAN_POINT('Ctrl Pts',(6.11610453983743,-5.01769946790715,79.4315461680771));
#60251=CARTESIAN_POINT('Ctrl Pts',(6.10910173666164,-5.02622310102447,79.4310964538033));
#60252=CARTESIAN_POINT('Ctrl Pts',(5.90687112156473,-5.27132604237178,79.4181058013499));
#60253=CARTESIAN_POINT('Ctrl Pts',(5.69808231253967,-5.49634686213858,79.4046050386651));
#60254=CARTESIAN_POINT('Ctrl Pts',(5.1993742622261,-5.97479823347969,79.3733159158589));
#60255=CARTESIAN_POINT('Ctrl Pts',(4.90293846429737,-6.220361833413,79.3553660769933));
#60256=CARTESIAN_POINT('Ctrl Pts',(4.34963794773614,-6.614494227712,79.3242186194346));
#60257=CARTESIAN_POINT('Ctrl Pts',(4.10005992832687,-6.77203153815581,79.3109056383335));
#60258=CARTESIAN_POINT('Ctrl Pts',(3.58993270007486,-7.05546775563662,79.2854194196948));
#60259=CARTESIAN_POINT('Ctrl Pts',(3.33011316986904,-7.18175544236608,79.2732469964317));
#60260=CARTESIAN_POINT('Ctrl Pts',(3.0444149158597,-7.30177429469146,79.2607104027392));
#60261=CARTESIAN_POINT('Ctrl Pts',(3.02484543341494,-7.30990288194682,79.2598557732196));
#60262=CARTESIAN_POINT('Ctrl Pts',(2.99704442625382,-7.32131984465816,79.2586474095015));
#60263=CARTESIAN_POINT('Ctrl Pts',(2.98883975503528,-7.32467313128044,79.2582915035208));
#60264=CARTESIAN_POINT('Ctrl Pts',(2.97485153381493,-7.33036276450165,79.2576859173835));
#60265=CARTESIAN_POINT('Ctrl Pts',(2.96907083334839,-7.33270606899126,79.257436004928));
#60266=CARTESIAN_POINT('Ctrl Pts',(2.95754665489451,-7.33736172738178,79.2569384825089));
#60267=CARTESIAN_POINT('Ctrl Pts',(2.95180322187117,-7.33967418036374,79.2566908693619));
#60268=CARTESIAN_POINT('Ctrl Pts',(2.94024468285565,-7.34431218211625,79.2561932402019));
#60269=CARTESIAN_POINT('Ctrl Pts',(2.93442951805531,-7.34663757287899,79.2559432295743));
#60270=CARTESIAN_POINT('Ctrl Pts',(2.913592252244,-7.35494137244679,79.2550486229524));
#60271=CARTESIAN_POINT('Ctrl Pts',(2.89855454613194,-7.36088065053992,79.2544053287518));
#60272=CARTESIAN_POINT('Ctrl Pts',(2.74515299566154,-7.42092500372552,79.2478664351905));
#60273=CARTESIAN_POINT('Ctrl Pts',(2.60530552162057,-7.4711698467326,79.2421000878005));
#60274=CARTESIAN_POINT('Ctrl Pts',(2.22950887252862,-7.59435106602856,79.2270670596992));
#60275=CARTESIAN_POINT('Ctrl Pts',(1.99141756078703,-7.66023131092465,79.2180215579339));
#60276=CARTESIAN_POINT('Ctrl Pts',(0.953196788596171,-7.89581983280163,
79.1799727570577));
#60277=CARTESIAN_POINT('Ctrl Pts',(0.132689807819647,-7.95201374208558,
79.1538743071341));
#60278=CARTESIAN_POINT('Ctrl Pts',(-0.723066059411459,-7.87799591481916,
79.1200659384808));
#60279=CARTESIAN_POINT('Ctrl Pts',(-0.764393145535784,-7.87409341873729,
79.1184158186872));
#60280=CARTESIAN_POINT('Ctrl Pts',(-0.813067159633271,-7.86911035839927,
79.1164499045633));
#60281=CARTESIAN_POINT('Ctrl Pts',(-0.820446306517562,-7.8683444190132,
79.1161512565424));
#60282=CARTESIAN_POINT('Ctrl Pts',(-0.832285229273103,-7.86709872932681,
79.1156711212081));
#60283=CARTESIAN_POINT('Ctrl Pts',(-0.836745706032739,-7.86662556265975,
79.1154899976521));
#60284=CARTESIAN_POINT('Ctrl Pts',(-0.844657851658747,-7.86577943796962,
79.1151683099738));
#60285=CARTESIAN_POINT('Ctrl Pts',(-0.848109685983407,-7.86540800045981,
79.1150278304882));
#60286=CARTESIAN_POINT('Ctrl Pts',(-0.855322027190808,-7.86462710742375,
79.1147340223114));
#60287=CARTESIAN_POINT('Ctrl Pts',(-0.859082476448986,-7.86421722789931,
79.1145806705307));
#60288=CARTESIAN_POINT('Ctrl Pts',(-0.868902412748709,-7.8631397520487,
79.114179789123));
#60289=CARTESIAN_POINT('Ctrl Pts',(-0.874961415132839,-7.86246784952252,
79.1139320207558));
#60290=CARTESIAN_POINT('Ctrl Pts',(-0.901271790409248,-7.8595194166701,
79.1128543137748));
#60291=CARTESIAN_POINT('Ctrl Pts',(-0.921514946826898,-7.85717165970015,
79.1120204768454));
#60292=CARTESIAN_POINT('Ctrl Pts',(-1.27348219138459,-7.81497237240634,
79.0974444134725));
#60293=CARTESIAN_POINT('Ctrl Pts',(-1.60233683013468,-7.75422649654075,
79.0826276786597));
#60294=CARTESIAN_POINT('Ctrl Pts',(-2.25829195044068,-7.58954412142652,
79.0519304291025));
#60295=CARTESIAN_POINT('Ctrl Pts',(-2.58449083708362,-7.48474931647354,
79.036070613588));
#60296=CARTESIAN_POINT('Ctrl Pts',(-3.08781728245134,-7.28620815438222,
79.0114219608624));
#60297=CARTESIAN_POINT('Ctrl Pts',(-3.26994497427875,-7.20631040466761,
79.0024598851414));
#60298=CARTESIAN_POINT('Ctrl Pts',(-3.76553098955796,-6.9662398813804,78.9781079404444));
#60299=CARTESIAN_POINT('Ctrl Pts',(-4.07162117289454,-6.79188217995465,
78.9631260975853));
#60300=CARTESIAN_POINT('Ctrl Pts',(-4.38379834759552,-6.58534244119041,
78.9479751911803));
#60301=CARTESIAN_POINT('Ctrl Pts',(-4.40243208634364,-6.57290002631632,
78.94707124155));
#60302=CARTESIAN_POINT('Ctrl Pts',(-4.42853992690136,-6.55530605719133,
78.9458052381632));
#60303=CARTESIAN_POINT('Ctrl Pts',(-4.43605832085272,-6.55022060409479,
78.9454407229093));
#60304=CARTESIAN_POINT('Ctrl Pts',(-4.44876670448191,-6.54159271839358,
78.9448246812294));
#60305=CARTESIAN_POINT('Ctrl Pts',(-4.45396124757696,-6.53805702709628,
78.9445729031083));
#60306=CARTESIAN_POINT('Ctrl Pts',(-4.46423481696767,-6.53104634578861,
78.9440750008553));
#60307=CARTESIAN_POINT('Ctrl Pts',(-4.46931401162571,-6.52757161106412,
78.9438288674296));
#60308=CARTESIAN_POINT('Ctrl Pts',(-4.47950172504379,-6.52058461551426,
78.943335231553));
#60309=CARTESIAN_POINT('Ctrl Pts',(-4.48461018019155,-6.51707226940881,
78.9430877325681));
#60310=CARTESIAN_POINT('Ctrl Pts',(-4.50253636826754,-6.50471596320192,
78.9422193182891));
#60311=CARTESIAN_POINT('Ctrl Pts',(-4.51533214954109,-6.4958401375304,78.9415996021579));
#60312=CARTESIAN_POINT('Ctrl Pts',(-4.62957516886812,-6.41609451314089,
78.9360679902825));
#60313=CARTESIAN_POINT('Ctrl Pts',(-4.7293751475187,-6.34288951913152,78.9312454788173));
#60314=CARTESIAN_POINT('Ctrl Pts',(-5.07967108090469,-6.07307536378398,
78.9143197396728));
#60315=CARTESIAN_POINT('Ctrl Pts',(-5.31997250147967,-5.86372028647672,
78.9027255588542));
#60316=CARTESIAN_POINT('Ctrl Pts',(-6.04589473124956,-5.14982191876501,
78.8667663534886));
#60317=CARTESIAN_POINT('Ctrl Pts',(-6.4774195546405,-4.59525263197187,78.8441097279409));
#60318=CARTESIAN_POINT('Ctrl Pts',(-6.86426259511397,-3.9332346530885,78.8153463276482));
#60319=CARTESIAN_POINT('Ctrl Pts',(-6.89742120020961,-3.87479240943078,
78.8127915211652));
#60320=CARTESIAN_POINT('Ctrl Pts',(-6.96706733055241,-3.74831338380656,
78.8072146239791));
#60321=CARTESIAN_POINT('Ctrl Pts',(-7.0033111507173,-3.6801511704084,78.80417992099));
#60322=CARTESIAN_POINT('Ctrl Pts',(-7.04303734580938,-3.60272709785791,
78.8006885061703));
#60323=CARTESIAN_POINT('Ctrl Pts',(-7.04750778531265,-3.59397434749516,
78.8002931704507));
#60324=CARTESIAN_POINT('Ctrl Pts',(-7.05398357179348,-3.58123675135194,
78.7997169002466));
#60325=CARTESIAN_POINT('Ctrl Pts',(-7.05600189206206,-3.57725847534528,
78.7995367817612));
#60326=CARTESIAN_POINT('Ctrl Pts',(-7.05955517299863,-3.57023995812577,
78.7992187739788));
#60327=CARTESIAN_POINT('Ctrl Pts',(-7.06109153898057,-3.56720042572293,
78.799080973737));
#60328=CARTESIAN_POINT('Ctrl Pts',(-7.06426068371198,-3.56092054929427,
78.7987961031376));
#60329=CARTESIAN_POINT('Ctrl Pts',(-7.06589319657912,-3.55768007278312,
78.7986490159099));
#60330=CARTESIAN_POINT('Ctrl Pts',(-7.07006705555556,-3.5493809148498,78.7982720756711));
#60331=CARTESIAN_POINT('Ctrl Pts',(-7.07260518124568,-3.54432066813838,
78.7980420181973));
#60332=CARTESIAN_POINT('Ctrl Pts',(-7.08320168672602,-3.5231377693434,78.7970780223262));
#60333=CARTESIAN_POINT('Ctrl Pts',(-7.09121031415583,-3.50699046859701,
78.79634091263));
#60334=CARTESIAN_POINT('Ctrl Pts',(-7.14559453173661,-3.39639098360176,
78.7912774029081));
#60335=CARTESIAN_POINT('Ctrl Pts',(-7.19013506836218,-3.30105268276544,
78.7868393009624));
#60336=CARTESIAN_POINT('Ctrl Pts',(-7.29552514498684,-3.06320723047647,
78.7756432051801));
#60337=CARTESIAN_POINT('Ctrl Pts',(-7.3541138662016,-2.91974840812836,78.7687826402078));
#60338=CARTESIAN_POINT('Ctrl Pts',(-7.74065183677902,-1.88768026220992,
78.7191456988919));
#60339=CARTESIAN_POINT('Ctrl Pts',(-7.91096337093462,-0.947868983073772,
78.6737611126276));
#60340=CARTESIAN_POINT('Ctrl Pts',(-7.91099999409123,-0.000305758797192468,
78.6348799381992));
#60341=CARTESIAN_POINT('',(-7.91099994932565,-0.00089541584189321,74.6422459153707));
#60342=CARTESIAN_POINT('Ctrl Pts',(-7.91099999420061,-0.000302915639028901,
78.6348798215365));
#60343=CARTESIAN_POINT('Ctrl Pts',(-7.91100231916487,0.0604162741918949,
78.6323883437237));
#60344=CARTESIAN_POINT('Ctrl Pts',(-7.91030558913058,0.121134580029745,
78.6299192893085));
#60345=CARTESIAN_POINT('Ctrl Pts',(-7.90868088875777,0.191798936417204,
78.6270712755329));
#60346=CARTESIAN_POINT('Ctrl Pts',(-7.90843310492471,0.201757423937507,
78.626670503395));
#60347=CARTESIAN_POINT('Ctrl Pts',(-7.90798595190084,0.218459845575327,
78.6259993091337));
#60348=CARTESIAN_POINT('Ctrl Pts',(-7.90779676433721,0.22520402711425,78.625728559936));
#60349=CARTESIAN_POINT('Ctrl Pts',(-7.90743603391781,0.237502093317745,
78.6252353350452));
#60350=CARTESIAN_POINT('Ctrl Pts',(-7.90726726694386,0.243056051391161,
78.6250127702498));
#60351=CARTESIAN_POINT('Ctrl Pts',(-7.90692663841683,0.253889819597429,
78.624578979869));
#60352=CARTESIAN_POINT('Ctrl Pts',(-7.90675533968934,0.259169643744248,
78.6243677363077));
#60353=CARTESIAN_POINT('Ctrl Pts',(-7.90635168343451,0.271238270803548,
78.6238852485638));
#60354=CARTESIAN_POINT('Ctrl Pts',(-7.90611587016403,0.278026958299536,
78.6236141156283));
#60355=CARTESIAN_POINT('Ctrl Pts',(-7.90545459447109,0.296382572294297,
78.6228817385796));
#60356=CARTESIAN_POINT('Ctrl Pts',(-7.90501248885136,0.307948903244428,
78.6224210297718));
#60357=CARTESIAN_POINT('Ctrl Pts',(-7.90283522523646,0.361812785545211,
78.6202791368633));
#60358=CARTESIAN_POINT('Ctrl Pts',(-7.90078594296876,0.404097321005026,
78.6186080622735));
#60359=CARTESIAN_POINT('Ctrl Pts',(-7.89646648899367,0.480529959756134,
78.6156056221322));
#60360=CARTESIAN_POINT('Ctrl Pts',(-7.89431396640791,0.514683486387897,
78.614270560532));
#60361=CARTESIAN_POINT('Ctrl Pts',(-7.83204462021638,1.41010260908118,78.5794354094257));
#60362=CARTESIAN_POINT('Ctrl Pts',(-7.63159789404408,2.25563136562526,78.5514712961313));
#60363=CARTESIAN_POINT('Ctrl Pts',(-7.19648694551417,3.29613080851428,78.5118978442765));
#60364=CARTESIAN_POINT('Ctrl Pts',(-7.08225547351034,3.53490336060398,78.5023490873609));
#60365=CARTESIAN_POINT('Ctrl Pts',(-6.91740883185871,3.8392761291715,78.4890078640274));
#60366=CARTESIAN_POINT('Ctrl Pts',(-6.87742122981216,3.91045553774849,78.4858002875659));
#60367=CARTESIAN_POINT('Ctrl Pts',(-6.83196954441888,3.98850706289354,78.4821710952793));
#60368=CARTESIAN_POINT('Ctrl Pts',(-6.82758620217426,3.99600589305646,78.4818212634931));
#60369=CARTESIAN_POINT('Ctrl Pts',(-6.82106141939508,4.00712612893741,78.4813007475243));
#60370=CARTESIAN_POINT('Ctrl Pts',(-6.81892941325859,4.01075309103175,78.4811307013922));
#60371=CARTESIAN_POINT('Ctrl Pts',(-6.81528802322958,4.01693651607664,78.4808403255222));
#60372=CARTESIAN_POINT('Ctrl Pts',(-6.81378008904254,4.01949383777388,78.4807200946844));
#60373=CARTESIAN_POINT('Ctrl Pts',(-6.81069582667807,4.0247177481155,78.4804742123688));
#60374=CARTESIAN_POINT('Ctrl Pts',(-6.80911937695788,4.02738425107126,78.4803485524277));
#60375=CARTESIAN_POINT('Ctrl Pts',(-6.80533848481893,4.03377091642562,78.4800472162309));
#60376=CARTESIAN_POINT('Ctrl Pts',(-6.80313256252285,4.03749019017393,78.4798714386365));
#60377=CARTESIAN_POINT('Ctrl Pts',(-6.79516225420659,4.05090337322374,78.4792364570196));
#60378=CARTESIAN_POINT('Ctrl Pts',(-6.78938021369226,4.06058672011185,78.4787760514448));
#60379=CARTESIAN_POINT('Ctrl Pts',(-6.7050674897427,4.20110409069561,78.4720663694254));
#60380=CARTESIAN_POINT('Ctrl Pts',(-6.62279256766777,4.32964418097776,78.4655677578941));
#60381=CARTESIAN_POINT('Ctrl Pts',(-6.47828565925252,4.54164622718403,78.4543425047208));
#60382=CARTESIAN_POINT('Ctrl Pts',(-6.41802665673729,4.62640984825984,78.4497115052583));
#60383=CARTESIAN_POINT('Ctrl Pts',(-5.914926715161,5.30534615218292,78.4116005711583));
#60384=CARTESIAN_POINT('Ctrl Pts',(-5.39225904924774,5.83582361271461,78.3758003975096));
#60385=CARTESIAN_POINT('Ctrl Pts',(-4.65315047291624,6.40061189385736,78.3347024824383));
#60386=CARTESIAN_POINT('Ctrl Pts',(-4.49890656263372,6.50995300942389,78.3265356314296));
#60387=CARTESIAN_POINT('Ctrl Pts',(-4.26070365078017,6.66629765427585,78.3145423480617));
#60388=CARTESIAN_POINT('Ctrl Pts',(-4.17956854109272,6.71746438070253,78.3105600496442));
#60389=CARTESIAN_POINT('Ctrl Pts',(-4.06760348778155,6.78525947052007,78.3052016020811));
#60390=CARTESIAN_POINT('Ctrl Pts',(-4.0375659115222,6.8031761529855,78.3037772453164));
#60391=CARTESIAN_POINT('Ctrl Pts',(-3.993240622965,6.82921814043955,78.3016945167937));
#60392=CARTESIAN_POINT('Ctrl Pts',(-3.97904504087964,6.83749893233023,78.301030367026));
#60393=CARTESIAN_POINT('Ctrl Pts',(-3.95340464433383,6.85234900248835,78.2998358911431));
#60394=CARTESIAN_POINT('Ctrl Pts',(-3.94196902241155,6.85893398148249,78.2993049847743));
#60395=CARTESIAN_POINT('Ctrl Pts',(-3.92545019911769,6.86839106489527,78.2985407117115));
#60396=CARTESIAN_POINT('Ctrl Pts',(-3.92038024093545,6.87128618620726,78.2983064965909));
#60397=CARTESIAN_POINT('Ctrl Pts',(-3.91038506852408,6.8769791115831,78.2978454517607));
#60398=CARTESIAN_POINT('Ctrl Pts',(-3.90546004571132,6.87977724325514,78.2976186100745));
#60399=CARTESIAN_POINT('Ctrl Pts',(-3.8956539285142,6.8853346256848,78.2971676120563));
#60400=CARTESIAN_POINT('Ctrl Pts',(-3.89077289799772,6.88809398126724,78.2969434519563));
#60401=CARTESIAN_POINT('Ctrl Pts',(-3.87918670626357,6.89462766960905,78.2964121297934));
#60402=CARTESIAN_POINT('Ctrl Pts',(-3.87247895790787,6.89839741719799,78.2961051358746));
#60403=CARTESIAN_POINT('Ctrl Pts',(-3.84886115456022,6.91162529498397,78.2950263614381));
#60404=CARTESIAN_POINT('Ctrl Pts',(-3.83192179851748,6.92103111843563,78.2942564933217));
#60405=CARTESIAN_POINT('Ctrl Pts',(-3.62044332119733,7.03744320714579,78.2846927052242));
#60406=CARTESIAN_POINT('Ctrl Pts',(-3.42151039836307,7.1362800266393,78.2762009262083));
#60407=CARTESIAN_POINT('Ctrl Pts',(-2.95474596563154,7.34417268838938,78.2572387840704));
#60408=CARTESIAN_POINT('Ctrl Pts',(-2.68457011616749,7.44718011530263,78.2469615141587));
#60409=CARTESIAN_POINT('Ctrl Pts',(-2.23397009589962,7.59125834307041,78.2304685780765));
#60410=CARTESIAN_POINT('Ctrl Pts',(-2.05667982513524,7.64119719606544,78.2241342117598));
#60411=CARTESIAN_POINT('Ctrl Pts',(-1.82680316116796,7.69736760348467,78.2159887550091));
#60412=CARTESIAN_POINT('Ctrl Pts',(-1.77567563327268,7.70932252846788,78.2141812339163));
#60413=CARTESIAN_POINT('Ctrl Pts',(-1.66512333359709,7.73401437749425,78.2102761550466));
#60414=CARTESIAN_POINT('Ctrl Pts',(-1.605663225567,7.74657728738832,78.2081778701038));
#60415=CARTESIAN_POINT('Ctrl Pts',(-1.47518452392972,7.77257840689903,78.2035686872149));
#60416=CARTESIAN_POINT('Ctrl Pts',(-1.40411478023519,7.78573092406636,78.2010550960429));
#60417=CARTESIAN_POINT('Ctrl Pts',(-1.08182289928625,7.84081940454443,78.1896091839499));
#60418=CARTESIAN_POINT('Ctrl Pts',(-0.828856897134209,7.87158004969096,
78.1804989140836));
#60419=CARTESIAN_POINT('Ctrl Pts',(-0.459077700770658,7.89852176828448,
78.1664913289405));
#60420=CARTESIAN_POINT('Ctrl Pts',(-0.343123456843648,7.90440794374743,
78.1619977948945));
#60421=CARTESIAN_POINT('Ctrl Pts',(-0.205144416257173,7.90837013854216,
78.1564991474161));
#60422=CARTESIAN_POINT('Ctrl Pts',(-0.183208454968984,7.90890871908443,
78.155620715135));
#60423=CARTESIAN_POINT('Ctrl Pts',(-0.154052257859593,7.90950321003464,
78.1544477278793));
#60424=CARTESIAN_POINT('Ctrl Pts',(-0.14683362647866,7.90964051100411,78.1541568726735));
#60425=CARTESIAN_POINT('Ctrl Pts',(-0.134965396109451,7.90984999642044,
78.1536779591542));
#60426=CARTESIAN_POINT('Ctrl Pts',(-0.130315892847507,7.90992796376515,
78.1534901592951));
#60427=CARTESIAN_POINT('Ctrl Pts',(-0.121295849598588,7.91007126534257,
78.1531254804098));
#60428=CARTESIAN_POINT('Ctrl Pts',(-0.116925317915763,7.91013707693145,
78.1529486225397));
#60429=CARTESIAN_POINT('Ctrl Pts',(-0.106820304696355,7.91028086182249,
78.1525393511727));
#60430=CARTESIAN_POINT('Ctrl Pts',(-0.101085792920875,7.91035622160142,
78.1523068234726));
#60431=CARTESIAN_POINT('Ctrl Pts',(-0.0856753322377926,7.91054197724541,
78.1516812314373));
#60432=CARTESIAN_POINT('Ctrl Pts',(-0.0759992740138839,7.91064085554851,
78.1512876705758));
#60433=CARTESIAN_POINT('Ctrl Pts',(-0.00738691801866201,7.91121609804258,
78.1484916813759));
#60434=CARTESIAN_POINT('Ctrl Pts',(0.051551899159381,7.91105156525361,78.1460623192176));
#60435=CARTESIAN_POINT('Ctrl Pts',(0.85606681164321,7.89981489411712,78.1125703051692));
#60436=CARTESIAN_POINT('Ctrl Pts',(1.59644498514849,7.78404704202496,78.0782842033726));
#60437=CARTESIAN_POINT('Ctrl Pts',(2.66758803932621,7.45707254141298,78.0297598429838));
#60438=CARTESIAN_POINT('Ctrl Pts',(3.01731143721459,7.3225557329619,78.0140221120751));
#60439=CARTESIAN_POINT('Ctrl Pts',(3.38726620545399,7.14923241046205,77.997464356031));
#60440=CARTESIAN_POINT('Ctrl Pts',(3.41821741103616,7.13448569708714,77.9960795401645));
#60441=CARTESIAN_POINT('Ctrl Pts',(3.46141270124571,7.11355966786809,77.9941472607883));
#60442=CARTESIAN_POINT('Ctrl Pts',(3.47373791654928,7.10754908005618,77.9935959509269));
#60443=CARTESIAN_POINT('Ctrl Pts',(3.49470317765288,7.0972574756243,77.9926582172941));
#60444=CARTESIAN_POINT('Ctrl Pts',(3.50335112431588,7.09299266004929,77.9922714259811));
#60445=CARTESIAN_POINT('Ctrl Pts',(3.52046062435258,7.08451602644398,77.9915061979984));
#60446=CARTESIAN_POINT('Ctrl Pts',(3.52892247272547,7.08030483232313,77.9911277474641));
#60447=CARTESIAN_POINT('Ctrl Pts',(3.54921036562249,7.07016278526083,77.9902204024781));
#60448=CARTESIAN_POINT('Ctrl Pts',(3.56102913233528,7.06421740531984,77.9896918406233));
#60449=CARTESIAN_POINT('Ctrl Pts',(3.60029128030229,7.04434318051033,77.9879359861837));
#60450=CARTESIAN_POINT('Ctrl Pts',(3.62766839378471,7.03028379161677,77.9867117078243));
#60451=CARTESIAN_POINT('Ctrl Pts',(4.05965783436255,6.80524234844587,77.967393682055));
#60452=CARTESIAN_POINT('Ctrl Pts',(4.44536444974195,6.55979594754333,77.9502185071955));
#60453=CARTESIAN_POINT('Ctrl Pts',(4.94558274176568,6.1769930124541,77.9271717512549));
#60454=CARTESIAN_POINT('Ctrl Pts',(5.0798786734273,6.0670309761633,77.9208892620471));
#60455=CARTESIAN_POINT('Ctrl Pts',(5.47297596501409,5.72295183978091,77.9020066888085));
#60456=CARTESIAN_POINT('Ctrl Pts',(5.72000420124256,5.47605513487731,77.8894722384593));
#60457=CARTESIAN_POINT('Ctrl Pts',(6.0703907473165,5.07618869416702,77.8695227018381));
#60458=CARTESIAN_POINT('Ctrl Pts',(6.18605461758261,4.934577782092,77.8625133364679));
#60459=CARTESIAN_POINT('Ctrl Pts',(6.31342845790513,4.76710659522269,77.8541458548615));
#60460=CARTESIAN_POINT('Ctrl Pts',(6.33003687807857,4.74503079848753,77.853041340772));
#60461=CARTESIAN_POINT('Ctrl Pts',(6.35121747269816,4.71656859225312,77.8516147840125));
#60462=CARTESIAN_POINT('Ctrl Pts',(6.35589636996666,4.71026156434367,77.8512985113994));
#60463=CARTESIAN_POINT('Ctrl Pts',(6.36341083734249,4.70010068061032,77.8507887136673));
#60464=CARTESIAN_POINT('Ctrl Pts',(6.36625232352464,4.69625119065728,77.8505955127517));
#60465=CARTESIAN_POINT('Ctrl Pts',(6.3716505796384,4.68892402607748,77.8502276494979));
#60466=CARTESIAN_POINT('Ctrl Pts',(6.37420799986258,4.68544683095546,77.8500530231984));
#60467=CARTESIAN_POINT('Ctrl Pts',(6.38002148224989,4.67752896384282,77.8496552615541));
#60468=CARTESIAN_POINT('Ctrl Pts',(6.3832757555163,4.67308698297217,77.8494320266161));
#60469=CARTESIAN_POINT('Ctrl Pts',(6.39167158689314,4.66160180278562,77.8488545950351));
#60470=CARTESIAN_POINT('Ctrl Pts',(6.39680613142137,4.65455350795798,77.8485000048074));
#60471=CARTESIAN_POINT('Ctrl Pts',(6.42730197276014,4.61254547201776,77.8463851956824));
#60472=CARTESIAN_POINT('Ctrl Pts',(6.45238788924219,4.57738755031577,77.8446093100112));
#60473=CARTESIAN_POINT('Ctrl Pts',(6.87938253865093,3.96846926671857,77.8137211143665));
#60474=CARTESIAN_POINT('Ctrl Pts',(7.20360383596858,3.34405568174492,77.7803109243016));
#60475=CARTESIAN_POINT('Ctrl Pts',(7.55247212101249,2.3772335206943,77.733467319325));
#60476=CARTESIAN_POINT('Ctrl Pts',(7.64436688840126,2.06270644022127,77.7188696471438));
#60477=CARTESIAN_POINT('Ctrl Pts',(7.74719008779793,1.607589407616,77.6989104348551));
#60478=CARTESIAN_POINT('Ctrl Pts',(7.77427808397464,1.4710203439894,77.6930636567347));
#60479=CARTESIAN_POINT('Ctrl Pts',(7.80563577354967,1.28769532773097,77.685406343059));
#60480=CARTESIAN_POINT('Ctrl Pts',(7.81311341061418,1.24151843315557,77.6834935913614));
#60481=CARTESIAN_POINT('Ctrl Pts',(7.82326171629309,1.17512247400958,77.6807660694483));
#60482=CARTESIAN_POINT('Ctrl Pts',(7.82626438459986,1.15495562736639,77.6799406271924));
#60483=CARTESIAN_POINT('Ctrl Pts',(7.83144331836407,1.119224518043,77.678483414497));
#60484=CARTESIAN_POINT('Ctrl Pts',(7.83365122691017,1.10366499874473,77.6778506266134));
#60485=CARTESIAN_POINT('Ctrl Pts',(7.83685752771419,1.08057521180894,77.6769142042168));
#60486=CARTESIAN_POINT('Ctrl Pts',(7.83789145560915,1.07304996555702,77.6766094239358));
#60487=CARTESIAN_POINT('Ctrl Pts',(7.83967947706338,1.05989572638289,77.676077380198));
#60488=CARTESIAN_POINT('Ctrl Pts',(7.84043834956631,1.05426739526424,77.675849962723));
#60489=CARTESIAN_POINT('Ctrl Pts',(7.84193762258739,1.04305658311968,77.6753974356517));
#60490=CARTESIAN_POINT('Ctrl Pts',(7.8426781244356,1.03747411958261,77.6751723229211));
#60491=CARTESIAN_POINT('Ctrl Pts',(7.84443099184918,1.02415055701102,77.6746355854301));
#60492=CARTESIAN_POINT('Ctrl Pts',(7.84543786135467,1.01640873343652,77.6743241381114));
#60493=CARTESIAN_POINT('Ctrl Pts',(7.84844404255318,0.993023575417423,77.6733846681491));
#60494=CARTESIAN_POINT('Ctrl Pts',(7.85040804422048,0.977375697179887,77.6727577848543));
#60495=CARTESIAN_POINT('Ctrl Pts',(7.8696245667757,0.820475484113165,77.666489478042));
#60496=CARTESIAN_POINT('Ctrl Pts',(7.8831101623419,0.678783948545217,77.6609708393846));
#60497=CARTESIAN_POINT('Ctrl Pts',(7.89321217839241,0.530250516965052,77.6553186097386));
#60498=CARTESIAN_POINT('Ctrl Pts',(7.89364951669848,0.523699734232348,77.6550695972594));
#60499=CARTESIAN_POINT('Ctrl Pts',(7.94117090326282,-0.201696615509884,
77.627524871233));
#60500=CARTESIAN_POINT('Ctrl Pts',(7.88986275843466,-0.923549114174577,
77.6037352115985));
#60501=CARTESIAN_POINT('Ctrl Pts',(7.73395698996074,-1.66469142808705,77.5778108903933));
#60502=CARTESIAN_POINT('Ctrl Pts',(7.72609163869864,-1.70082222652563,77.5765422039061));
#60503=CARTESIAN_POINT('Ctrl Pts',(7.70902584912639,-1.77665478956118,77.5738670925913));
#60504=CARTESIAN_POINT('Ctrl Pts',(7.6997713593883,-1.81634324041259,77.572459874676));
#60505=CARTESIAN_POINT('Ctrl Pts',(7.67949497124513,-1.90035897647471,77.5694628867353));
#60506=CARTESIAN_POINT('Ctrl Pts',(7.66839501181587,-1.94466581777949,77.5678716589156));
#60507=CARTESIAN_POINT('Ctrl Pts',(7.57272807113169,-2.3129714225212,77.5545384753036));
#60508=CARTESIAN_POINT('Ctrl Pts',(7.46805917087179,-2.63136772578305,77.5423333106155));
#60509=CARTESIAN_POINT('Ctrl Pts',(7.33957161452393,-2.95207112716206,77.5284738619634));
#60510=CARTESIAN_POINT('Ctrl Pts',(7.33557325037546,-2.96199265879721,77.5280435036701));
#60511=CARTESIAN_POINT('Ctrl Pts',(7.32984099370864,-2.97613387113643,77.5274278001698));
#60512=CARTESIAN_POINT('Ctrl Pts',(7.32812353957319,-2.98036024677558,77.5272434902558));
#60513=CARTESIAN_POINT('Ctrl Pts',(7.32514793858423,-2.98766459542355,77.52692443777));
#60514=CARTESIAN_POINT('Ctrl Pts',(7.32389150559794,-2.990743263973,77.526789804038));
#60515=CARTESIAN_POINT('Ctrl Pts',(7.32147126040238,-2.99666297890638,77.5265306251937));
#60516=CARTESIAN_POINT('Ctrl Pts',(7.32030773322601,-2.99950414516599,77.5264060980802));
#60517=CARTESIAN_POINT('Ctrl Pts',(7.31756205014327,-3.00619759590852,77.526112411856));
#60518=CARTESIAN_POINT('Ctrl Pts',(7.31597850708423,-3.01004930642219,77.5259431655809));
#60519=CARTESIAN_POINT('Ctrl Pts',(7.31049188756423,-3.02336470797847,77.525357233144));
#60520=CARTESIAN_POINT('Ctrl Pts',(7.30657349827935,-3.03282203697197,77.5249395923981));
#60521=CARTESIAN_POINT('Ctrl Pts',(7.26277413660642,-3.13795756135698,77.5202805150726));
#60522=CARTESIAN_POINT('Ctrl Pts',(7.22103628742296,-3.23284688478919,77.5159258199844));
#60523=CARTESIAN_POINT('Ctrl Pts',(6.82759351987256,-4.08166350484498,77.4758045933944));
#60524=CARTESIAN_POINT('Ctrl Pts',(6.36087258131209,-4.77656920304409,77.435219030916));
#60525=CARTESIAN_POINT('Ctrl Pts',(5.56804532416279,-5.62950117403064,77.3837615681504));
#60526=CARTESIAN_POINT('Ctrl Pts',(5.32660281141983,-5.85847683406975,77.3696372159281));
#60527=CARTESIAN_POINT('Ctrl Pts',(5.06017875101148,-6.08101369337981,77.3556012863157));
#60528=CARTESIAN_POINT('Ctrl Pts',(5.04888504766168,-6.09039377297291,77.3550089995715));
#60529=CARTESIAN_POINT('Ctrl Pts',(5.03083115031956,-6.10530385935583,77.3540664563381));
#60530=CARTESIAN_POINT('Ctrl Pts',(5.02408782364861,-6.11085418080099,77.3537153526063));
#60531=CARTESIAN_POINT('Ctrl Pts',(5.0112459541367,-6.12138848782573,77.353048510475));
#60532=CARTESIAN_POINT('Ctrl Pts',(5.00514913552611,-6.12637455297636,77.3527326857101));
#60533=CARTESIAN_POINT('Ctrl Pts',(4.99449102271124,-6.13506438001627,77.352181911525));
#60534=CARTESIAN_POINT('Ctrl Pts',(4.98993303486546,-6.13877217614726,77.351946794867));
#60535=CARTESIAN_POINT('Ctrl Pts',(4.9810597443088,-6.14597393853123,77.3514899032317));
#60536=CARTESIAN_POINT('Ctrl Pts',(4.97674488663466,-6.1494684455644,77.3512681059312));
#60537=CARTESIAN_POINT('Ctrl Pts',(4.96654899581844,-6.15770811057429,77.3507448942524));
#60538=CARTESIAN_POINT('Ctrl Pts',(4.96066483053207,-6.16244939471723,77.3504436398686));
#60539=CARTESIAN_POINT('Ctrl Pts',(4.94019038982152,-6.17889875841927,77.3493978146356));
#60540=CARTESIAN_POINT('Ctrl Pts',(4.92556533205801,-6.19056355434743,77.3486550257474));
#60541=CARTESIAN_POINT('Ctrl Pts',(4.75655828216668,-6.32438376377872,77.3401199275047));
#60542=CARTESIAN_POINT('Ctrl Pts',(4.59770441856821,-6.44079167902885,77.3325656292473));
#60543=CARTESIAN_POINT('Ctrl Pts',(3.80355381121651,-6.97837486647673,77.2967810192411));
#60544=CARTESIAN_POINT('Ctrl Pts',(3.11410864959702,-7.31210936672008,77.2721192410177));
#60545=CARTESIAN_POINT('Ctrl Pts',(2.33059918364441,-7.56014579225543,77.243031830625));
#60546=CARTESIAN_POINT('Ctrl Pts',(2.27338622944995,-7.57754655878987,77.2408992192569));
#60547=CARTESIAN_POINT('Ctrl Pts',(2.14326951117135,-7.61551404054068,77.2360191549871));
#60548=CARTESIAN_POINT('Ctrl Pts',(2.07025715466929,-7.63568550983528,77.2332596699371));
#60549=CARTESIAN_POINT('Ctrl Pts',(1.84399728050741,-7.69471166036746,77.2246133085429));
#60550=CARTESIAN_POINT('Ctrl Pts',(1.68987284640951,-7.73002186009024,77.218590258445));
#60551=CARTESIAN_POINT('Ctrl Pts',(1.51210421096783,-7.76517850641759,77.2113873666949));
#60552=CARTESIAN_POINT('Ctrl Pts',(1.48938617109232,-7.76956788976854,77.2104621124243));
#60553=CARTESIAN_POINT('Ctrl Pts',(1.46054722279686,-7.77500876991651,77.209281173533));
#60554=CARTESIAN_POINT('Ctrl Pts',(1.45444372678084,-7.77615284107149,77.2090308749559));
#60555=CARTESIAN_POINT('Ctrl Pts',(1.44464103028577,-7.77797836469603,77.2086282886564));
#60556=CARTESIAN_POINT('Ctrl Pts',(1.44094272873539,-7.77866435838931,77.2084762697823));
#60557=CARTESIAN_POINT('Ctrl Pts',(1.43391147359225,-7.77996339132317,77.2081869977246));
#60558=CARTESIAN_POINT('Ctrl Pts',(1.4305786113852,-7.78057692725982,77.20804977325));
#60559=CARTESIAN_POINT('Ctrl Pts',(1.42299938880114,-7.78196712755142,77.2077374697973));
#60560=CARTESIAN_POINT('Ctrl Pts',(1.41875278787592,-7.78274245761574,77.2075623144046));
#60561=CARTESIAN_POINT('Ctrl Pts',(1.4058779796865,-7.78508220892517,77.2070307591244));
#60562=CARTESIAN_POINT('Ctrl Pts',(1.39724782833438,-7.78663575612422,77.2066737420667));
#60563=CARTESIAN_POINT('Ctrl Pts',(1.33731457122617,-7.79732172928878,77.2041895590107));
#60564=CARTESIAN_POINT('Ctrl Pts',(1.28592594848808,-7.80596122444017,77.2020349878189));
#60565=CARTESIAN_POINT('Ctrl Pts',(1.22847977350406,-7.81503647227574,77.1996020464743));
#60566=CARTESIAN_POINT('Ctrl Pts',(1.22250164093129,-7.81597385835489,77.1993485682365));
#60567=CARTESIAN_POINT('Ctrl Pts',(1.21338518862078,-7.81739262573166,77.1989615799654));
#60568=CARTESIAN_POINT('Ctrl Pts',(1.21024763467186,-7.81787897984678,77.1988283126916));
#60569=CARTESIAN_POINT('Ctrl Pts',(1.20416611463337,-7.81881793113046,77.1985698471283));
#60570=CARTESIAN_POINT('Ctrl Pts',(1.20122218354781,-7.81927075484094,77.1984446598325));
#60571=CARTESIAN_POINT('Ctrl Pts',(1.19262831629414,-7.82058766127101,77.1980790133012));
#60572=CARTESIAN_POINT('Ctrl Pts',(1.18697770738704,-7.82144728233434,77.1978383396742));
#60573=CARTESIAN_POINT('Ctrl Pts',(0.616437759188743,-7.90761039457926,
77.173512217628));
#60574=CARTESIAN_POINT('Ctrl Pts',(0.0439985209837045,-7.93147570018103,
77.1467131300235));
#60575=CARTESIAN_POINT('Ctrl Pts',(-0.885033914973852,-7.86956960938423,
77.1039127658265));
#60576=CARTESIAN_POINT('Ctrl Pts',(-1.24205478758606,-7.82117279129737,
77.0876079380365));
#60577=CARTESIAN_POINT('Ctrl Pts',(-1.83607688144374,-7.69893126866916,
77.061247148098));
#60578=CARTESIAN_POINT('Ctrl Pts',(-2.07514836208777,-7.63796402727584,
77.0508475949108));
#60579=CARTESIAN_POINT('Ctrl Pts',(-2.34883700456367,-7.55436636609084,
77.0391938746435));
#60580=CARTESIAN_POINT('Ctrl Pts',(-2.38659023234631,-7.54252435122402,
77.0375918281125));
#60581=CARTESIAN_POINT('Ctrl Pts',(-2.43491342263068,-7.52696771864853,
77.0355480973403));
#60582=CARTESIAN_POINT('Ctrl Pts',(-2.44556618081232,-7.5235133062868,77.0350979889858));
#60583=CARTESIAN_POINT('Ctrl Pts',(-2.46268796596274,-7.51792094932336,
77.0343752284431));
#60584=CARTESIAN_POINT('Ctrl Pts',(-2.46916161068641,-7.51579725369055,
77.034102114042));
#60585=CARTESIAN_POINT('Ctrl Pts',(-2.48146414867605,-7.5117437641795,77.033583383063));
#60586=CARTESIAN_POINT('Ctrl Pts',(-2.48729355250034,-7.50981554259232,
77.0333377156408));
#60587=CARTESIAN_POINT('Ctrl Pts',(-2.50054644826687,-7.50541469087283,
77.0327794879836));
#60588=CARTESIAN_POINT('Ctrl Pts',(-2.50796853364924,-7.50293782838312,
77.0324670656315));
#60589=CARTESIAN_POINT('Ctrl Pts',(-2.5304704087447,-7.49539149140103,77.0315204962075));
#60590=CARTESIAN_POINT('Ctrl Pts',(-2.5455386333882,-7.4902875224231,77.0308874721892));
#60591=CARTESIAN_POINT('Ctrl Pts',(-2.65051315125114,-7.45437678234964,
77.0264831868576));
#60592=CARTESIAN_POINT('Ctrl Pts',(-2.7398750074953,-7.42199696107769,77.0227635318252));
#60593=CARTESIAN_POINT('Ctrl Pts',(-2.90834175663681,-7.35749644392028,
77.0157992602163));
#60594=CARTESIAN_POINT('Ctrl Pts',(-2.98755197485169,-7.32569037067155,
77.0125453283614));
#60595=CARTESIAN_POINT('Ctrl Pts',(-3.76791252860589,-6.99758174459804,
76.98064994306));
#60596=CARTESIAN_POINT('Ctrl Pts',(-4.42326166250249,-6.60287579068143,
76.9556592818221));
#60597=CARTESIAN_POINT('Ctrl Pts',(-5.15293580172315,-6.00535565591328,
76.922070489555));
#60598=CARTESIAN_POINT('Ctrl Pts',(-5.28971880859796,-5.88522842024651,
76.9154525529069));
#60599=CARTESIAN_POINT('Ctrl Pts',(-5.48644488400944,-5.70005439946176,
76.9052498439001));
#60600=CARTESIAN_POINT('Ctrl Pts',(-5.54964108693638,-5.63854418526118,
76.9018604170419));
#60601=CARTESIAN_POINT('Ctrl Pts',(-5.64481793100041,-5.54275624049307,
76.8965580407421));
#60602=CARTESIAN_POINT('Ctrl Pts',(-5.67754539181419,-5.50922811097333,
76.8946977003734));
#60603=CARTESIAN_POINT('Ctrl Pts',(-5.71547321328777,-5.46967550335932,
76.8924952797971));
#60604=CARTESIAN_POINT('Ctrl Pts',(-5.72096527006593,-5.46393086904646,
76.8921752090447));
#60605=CARTESIAN_POINT('Ctrl Pts',(-5.72933476981539,-5.45515000653364,
76.8916856627141));
#60606=CARTESIAN_POINT('Ctrl Pts',(-5.73221848981751,-5.45211974219841,
76.8915166651458));
#60607=CARTESIAN_POINT('Ctrl Pts',(-5.73745555006345,-5.44660779825621,
76.8912091602321));
#60608=CARTESIAN_POINT('Ctrl Pts',(-5.73980968870466,-5.44412687529991,
76.8910707141094));
#60609=CARTESIAN_POINT('Ctrl Pts',(-5.74452516706089,-5.43915098207734,
76.8907929593604));
#60610=CARTESIAN_POINT('Ctrl Pts',(-5.74688649138818,-5.43665599941061,
76.8906536496043));
#60611=CARTESIAN_POINT('Ctrl Pts',(-5.75362505611544,-5.42952671515151,
76.8902554642953));
#60612=CARTESIAN_POINT('Ctrl Pts',(-5.75799830528626,-5.42488867653322,
76.8899962826315));
#60613=CARTESIAN_POINT('Ctrl Pts',(-5.77684082401892,-5.40485683653253,
76.8888762970128));
#60614=CARTESIAN_POINT('Ctrl Pts',(-5.79125388712421,-5.38941051771656,
76.8880112357019));
#60615=CARTESIAN_POINT('Ctrl Pts',(-5.82285143963137,-5.35527466293965,
76.8860966855741));
#60616=CARTESIAN_POINT('Ctrl Pts',(-5.84000813221957,-5.33655980878101,
76.885045215306));
#60617=CARTESIAN_POINT('Ctrl Pts',(-6.35941796636103,-4.76447300534346,
76.8528573462661));
#60618=CARTESIAN_POINT('Ctrl Pts',(-6.78082511369048,-4.14280706541201,
76.8169543520969));
#60619=CARTESIAN_POINT('Ctrl Pts',(-7.24517762208962,-3.19186364733059,
76.7691194268557));
#60620=CARTESIAN_POINT('Ctrl Pts',(-7.36502395956801,-2.9046583762339,76.7554152809114));
#60621=CARTESIAN_POINT('Ctrl Pts',(-7.50479702961425,-2.50491551185445,
76.737497419901));
#60622=CARTESIAN_POINT('Ctrl Pts',(-7.53966424528285,-2.39792506559273,
76.7328086081913));
#60623=CARTESIAN_POINT('Ctrl Pts',(-7.58974309522077,-2.2323478306801,76.7257146790602));
#60624=CARTESIAN_POINT('Ctrl Pts',(-7.6065839303791,-2.17427188089323,76.7232567440478));
#60625=CARTESIAN_POINT('Ctrl Pts',(-7.62617507491286,-2.10369626548633,
76.7203057239821));
#60626=CARTESIAN_POINT('Ctrl Pts',(-7.62956279183548,-2.09137654622007,
76.7197919115497));
#60627=CARTESIAN_POINT('Ctrl Pts',(-7.63478654515992,-2.0721983057618,76.7189940956143));
#60628=CARTESIAN_POINT('Ctrl Pts',(-7.63664321282725,-2.06534545509644,
76.7187094215359));
#60629=CARTESIAN_POINT('Ctrl Pts',(-7.63989995854664,-2.05326056738466,
76.7182081150941));
#60630=CARTESIAN_POINT('Ctrl Pts',(-7.64130389225151,-2.04802958000643,
76.7179913575842));
#60631=CARTESIAN_POINT('Ctrl Pts',(-7.64449574742573,-2.03608791492415,
76.7174970628489));
#60632=CARTESIAN_POINT('Ctrl Pts',(-7.64628020763725,-2.02937631215187,
76.7172196381558));
#60633=CARTESIAN_POINT('Ctrl Pts',(-7.65106375511801,-2.01128884536766,
76.7164730247647));
#60634=CARTESIAN_POINT('Ctrl Pts',(-7.6540463135995,-1.99990860671062,76.7160043726224));
#60635=CARTESIAN_POINT('Ctrl Pts',(-7.66764989366914,-1.94752664947359,
76.7138522527632));
#60636=CARTESIAN_POINT('Ctrl Pts',(-7.67796700602383,-1.90644634533213,
76.7121786412781));
#60637=CARTESIAN_POINT('Ctrl Pts',(-7.83608378484873,-1.25475255301284,
76.6858475950965));
#60638=CARTESIAN_POINT('Ctrl Pts',(-7.91096433687506,-0.628760618091075,
76.663847643362));
#60639=CARTESIAN_POINT('Ctrl Pts',(-7.91103092760329,0.544851669213203,
76.6235237229675));
#60640=CARTESIAN_POINT('Ctrl Pts',(-7.85468120141728,1.08863886011775,76.6051102215045));
#60641=CARTESIAN_POINT('Ctrl Pts',(-7.72786842137306,1.69391043821135,76.5811806430569));
#60642=CARTESIAN_POINT('Ctrl Pts',(-7.71185886122117,1.76536546050135,76.5782986969197));
#60643=CARTESIAN_POINT('Ctrl Pts',(-7.69284672224997,1.84502182289784,76.5750120948878));
#60644=CARTESIAN_POINT('Ctrl Pts',(-7.69081939515854,1.85345440974454,76.5746632385904));
#60645=CARTESIAN_POINT('Ctrl Pts',(-7.68775477680314,1.86610996493545,76.5741382590911));
#60646=CARTESIAN_POINT('Ctrl Pts',(-7.68672785891327,1.87033545983041,76.5739627388454));
#60647=CARTESIAN_POINT('Ctrl Pts',(-7.68494785482,1.87763347761757,76.5736591770404));
#60648=CARTESIAN_POINT('Ctrl Pts',(-7.684196407808,1.88070640285607,76.5735312315643));
#60649=CARTESIAN_POINT('Ctrl Pts',(-7.68263403905664,1.88707889784916,76.5732656393601));
#60650=CARTESIAN_POINT('Ctrl Pts',(-7.68182283712073,1.89037838639041,76.5731279761796));
#60651=CARTESIAN_POINT('Ctrl Pts',(-7.67990511219554,1.89815693610578,76.5728030884181));
#60652=CARTESIAN_POINT('Ctrl Pts',(-7.67879679726187,1.90263554907473,76.5726157586643));
#60653=CARTESIAN_POINT('Ctrl Pts',(-7.67514910067372,1.91732050017351,76.5720006395713));
#60654=CARTESIAN_POINT('Ctrl Pts',(-7.6725932924125,1.92752270678593,76.5715718938665));
#60655=CARTESIAN_POINT('Ctrl Pts',(-7.58196658609709,2.28624764423388,76.55644811545));
#60656=CARTESIAN_POINT('Ctrl Pts',(-7.47027001484355,2.62833833941774,76.5404304359116));
#60657=CARTESIAN_POINT('Ctrl Pts',(-7.01311817776944,3.76067338391006,76.484672890547));
#60658=CARTESIAN_POINT('Ctrl Pts',(-6.56200708626946,4.50190991946419,76.4442261511919));
#60659=CARTESIAN_POINT('Ctrl Pts',(-5.9932570524005,5.16380703571983,76.4084796968031));
#60660=CARTESIAN_POINT('Ctrl Pts',(-5.98633762539382,5.17182704991676,76.4080464876772));
#60661=CARTESIAN_POINT('Ctrl Pts',(-5.94863734918117,5.21534681269649,76.405695277769));
#60662=CARTESIAN_POINT('Ctrl Pts',(-5.91755648903749,5.2505860614261,76.4037898234488));
#60663=CARTESIAN_POINT('Ctrl Pts',(-5.87802031141662,5.29461488268659,76.4014067367755));
#60664=CARTESIAN_POINT('Ctrl Pts',(-5.86985649332964,5.30366423209943,76.400916807445));
#60665=CARTESIAN_POINT('Ctrl Pts',(-5.85695893555927,5.31789453413708,76.4001461721181));
#60666=CARTESIAN_POINT('Ctrl Pts',(-5.85223917469671,5.32308809728988,76.3998648727266));
#60667=CARTESIAN_POINT('Ctrl Pts',(-5.84389012029176,5.33225076184958,76.3993685140027));
#60668=CARTESIAN_POINT('Ctrl Pts',(-5.84026368171439,5.33622245164899,76.3991533332963));
#60669=CARTESIAN_POINT('Ctrl Pts',(-5.83195031299158,5.34530866014916,76.398660992285));
#60670=CARTESIAN_POINT('Ctrl Pts',(-5.82726069680937,5.35042072151442,76.398383946943));
#60671=CARTESIAN_POINT('Ctrl Pts',(-5.8143349469063,5.36447368325589,76.3976222255312));
#60672=CARTESIAN_POINT('Ctrl Pts',(-5.80608490426132,5.37340179582522,76.3971381455345));
#60673=CARTESIAN_POINT('Ctrl Pts',(-5.76220351911996,5.42067073428612,76.3945744343269));
#60674=CARTESIAN_POINT('Ctrl Pts',(-5.72621251195026,5.45867667180154,76.3925103242929));
#60675=CARTESIAN_POINT('Ctrl Pts',(-5.28202823152216,5.9185005093116,76.3674949553914));
#60676=CARTESIAN_POINT('Ctrl Pts',(-4.82846832864452,6.29400039735428,76.3468243301362));
#60677=CARTESIAN_POINT('Ctrl Pts',(-4.26928906247498,6.66061181377203,76.3238096190381));
#60678=CARTESIAN_POINT('Ctrl Pts',(-4.2003635546563,6.70429152609681,76.3210078212627));
#60679=CARTESIAN_POINT('Ctrl Pts',(-3.71428837588567,7.00189010659934,76.3014260536155));
#60680=CARTESIAN_POINT('Ctrl Pts',(-3.27512396270644,7.21774716902434,76.284685054587));
#60681=CARTESIAN_POINT('Ctrl Pts',(-2.75310897012774,7.41682365016354,76.2630381751009));
#60682=CARTESIAN_POINT('Ctrl Pts',(-2.68696702781521,7.44104090217362,76.2602638890925));
#60683=CARTESIAN_POINT('Ctrl Pts',(-2.61153521098281,7.46752270597455,76.2570552456935));
#60684=CARTESIAN_POINT('Ctrl Pts',(-2.60255238830475,7.47065810937037,76.2566724280423));
#60685=CARTESIAN_POINT('Ctrl Pts',(-2.58942588361466,7.47521329321921,76.2561119477288));
#60686=CARTESIAN_POINT('Ctrl Pts',(-2.58528661520565,7.47664585913675,76.2559350521128));
#60687=CARTESIAN_POINT('Ctrl Pts',(-2.57795814105536,7.47917536880392,76.255621583945));
#60688=CARTESIAN_POINT('Ctrl Pts',(-2.57476942792706,7.4802737093875,76.2554850964492));
#60689=CARTESIAN_POINT('Ctrl Pts',(-2.56812103566069,7.48255896897828,76.2552003274779));
#60690=CARTESIAN_POINT('Ctrl Pts',(-2.56466125340506,7.48374552167812,76.2550520253291));
#60691=CARTESIAN_POINT('Ctrl Pts',(-2.55566773967461,7.48682293112151,76.2546662383284));
#60692=CARTESIAN_POINT('Ctrl Pts',(-2.5501327407928,7.4887100492387,76.2544285292496));
#60693=CARTESIAN_POINT('Ctrl Pts',(-2.52647354730777,7.49674720960121,76.2534112732783));
#60694=CARTESIAN_POINT('Ctrl Pts',(-2.50832929238517,7.50283756047676,76.2526281934953));
#60695=CARTESIAN_POINT('Ctrl Pts',(-2.38144177708253,7.54491725658579,76.2471322985383));
#60696=CARTESIAN_POINT('Ctrl Pts',(-2.2719545875228,7.5786055071434,76.2422897076891));
#60697=CARTESIAN_POINT('Ctrl Pts',(-1.99129955984922,7.65833244825229,76.2296939089449));
#60698=CARTESIAN_POINT('Ctrl Pts',(-1.81924749826317,7.7010169899037,76.221802413683));
#60699=CARTESIAN_POINT('Ctrl Pts',(-1.24858961316317,7.82240090960169,76.1953896018029));
#60700=CARTESIAN_POINT('Ctrl Pts',(-0.845346381885203,7.87618717279358,
76.1763808516215));
#60701=CARTESIAN_POINT('Ctrl Pts',(-0.0524279349411913,7.92033205965817,
76.1400141756224));
#60702=CARTESIAN_POINT('Ctrl Pts',(0.335988121549553,7.91337914540182,76.1226709526148));
#60703=CARTESIAN_POINT('Ctrl Pts',(0.730419857845168,7.87721228461404,76.1058418754191));
#60704=CARTESIAN_POINT('Ctrl Pts',(0.738480974833161,7.87646065162174,76.1054982529992));
#60705=CARTESIAN_POINT('Ctrl Pts',(0.747697171325159,7.87558704407975,76.1051057574976));
#60706=CARTESIAN_POINT('Ctrl Pts',(0.748853379456794,7.8754771896668,76.1050565239552));
#60707=CARTESIAN_POINT('Ctrl Pts',(0.751450851169223,7.87522981978477,76.1049459334155));
#60708=CARTESIAN_POINT('Ctrl Pts',(0.752892101442853,7.87509216325358,76.1048845806217));
#60709=CARTESIAN_POINT('Ctrl Pts',(0.756561700810109,7.87474065630967,76.1047283948918));
#60710=CARTESIAN_POINT('Ctrl Pts',(0.758789997768888,7.87452625562743,76.1046335783665));
#60711=CARTESIAN_POINT('Ctrl Pts',(0.768390624197728,7.87359839646967,76.1042251661423));
#60712=CARTESIAN_POINT('Ctrl Pts',(0.775762052464235,7.87287552921991,76.1039118515696));
#60713=CARTESIAN_POINT('Ctrl Pts',(0.783976663102461,7.87205832749158,76.1035629965723));
#60714=CARTESIAN_POINT('Ctrl Pts',(0.784820845080389,7.87197420986925,76.103527149679));
#60715=CARTESIAN_POINT('Ctrl Pts',(0.787937608118689,7.87166313696443,76.1033948140748));
#60716=CARTESIAN_POINT('Ctrl Pts',(0.790210105469669,7.87143533323863,76.1032983508473));
#60717=CARTESIAN_POINT('Ctrl Pts',(0.794601676099962,7.87099318464625,76.1031119861319));
#60718=CARTESIAN_POINT('Ctrl Pts',(0.796720761930482,7.87077896805181,76.1030220807951));
#60719=CARTESIAN_POINT('Ctrl Pts',(0.951891240965182,7.85502960749803,76.0964403657639));
#60720=CARTESIAN_POINT('Ctrl Pts',(1.10446199005023,7.8350337787864,76.090085412071));
#60721=CARTESIAN_POINT('Ctrl Pts',(1.27427718356294,7.80771849112803,76.0831379208332));
#60722=CARTESIAN_POINT('Ctrl Pts',(1.29218571475534,7.80477459389872,76.0824068040235));
#60723=CARTESIAN_POINT('Ctrl Pts',(1.3173499220342,7.80054898482547,76.0813816402843));
#60724=CARTESIAN_POINT('Ctrl Pts',(1.32461411284663,7.79931873525908,76.0810859587343));
#60725=CARTESIAN_POINT('Ctrl Pts',(1.33794107399107,7.79704255044026,76.0805439621214));
#60726=CARTESIAN_POINT('Ctrl Pts',(1.34400435967317,7.79599968780535,76.0802975495607));
#60727=CARTESIAN_POINT('Ctrl Pts',(1.35629231726226,7.79387144329037,76.0797985215067));
#60728=CARTESIAN_POINT('Ctrl Pts',(1.36251691813998,7.7927856747394,76.0795459185151));
#60729=CARTESIAN_POINT('Ctrl Pts',(1.37784156025916,7.79009364676491,76.0789244770313));
#60730=CARTESIAN_POINT('Ctrl Pts',(1.38694011108493,7.78847889639276,76.078555908932));
#60731=CARTESIAN_POINT('Ctrl Pts',(1.42011563729916,7.78253114678753,76.0772134479337));
#60732=CARTESIAN_POINT('Ctrl Pts',(1.44417542353122,7.77810239286138,76.0762426040216));
#60733=CARTESIAN_POINT('Ctrl Pts',(1.79330018745065,7.71216222189318,76.062193984688));
#60734=CARTESIAN_POINT('Ctrl Pts',(2.11422722910587,7.63042869234352,76.0497924107294));
#60735=CARTESIAN_POINT('Ctrl Pts',(2.77367472250375,7.41766322184181,76.0248025824101));
#60736=CARTESIAN_POINT('Ctrl Pts',(3.11020133460932,7.28297033385233,76.0123388024757));
#60737=CARTESIAN_POINT('Ctrl Pts',(3.70035690335582,6.99837174232747,75.9897670428475));
#60738=CARTESIAN_POINT('Ctrl Pts',(3.95710285748966,6.85646953993599,75.9796717739896));
#60739=CARTESIAN_POINT('Ctrl Pts',(4.42447690235314,6.56314261721425,75.9598278449249));
#60740=CARTESIAN_POINT('Ctrl Pts',(4.63668852769994,6.41497747435768,75.9501865415141));
#60741=CARTESIAN_POINT('Ctrl Pts',(4.85386200813806,6.24693517836117,75.9392187924459));
#60742=CARTESIAN_POINT('Ctrl Pts',(4.86644981759778,6.23713409207241,75.9385789798622));
#60743=CARTESIAN_POINT('Ctrl Pts',(4.88348785604352,6.22378500200706,75.9377072701521));
#60744=CARTESIAN_POINT('Ctrl Pts',(4.88796410194713,6.22027011705225,75.9374777178803));
#60745=CARTESIAN_POINT('Ctrl Pts',(4.89503247860295,6.21470747066456,75.9371143805708));
#60746=CARTESIAN_POINT('Ctrl Pts',(4.89762713078323,6.2126629073401,75.9369808246781));
#60747=CARTESIAN_POINT('Ctrl Pts',(4.90265712096098,6.20869420953345,75.9367215606518));
#60748=CARTESIAN_POINT('Ctrl Pts',(4.9050926103238,6.20677026458069,75.9365958660512));
#60749=CARTESIAN_POINT('Ctrl Pts',(4.91082284929944,6.20223811224287,75.9362997539038));
#60750=CARTESIAN_POINT('Ctrl Pts',(4.91411665260809,6.1996287132856,75.9361292518156));
#60751=CARTESIAN_POINT('Ctrl Pts',(4.92378295818904,6.19195838185046,75.9356280216759));
#60752=CARTESIAN_POINT('Ctrl Pts',(4.93014971639758,6.18689025237377,75.9352967867975));
#60753=CARTESIAN_POINT('Ctrl Pts',(4.94458275210689,6.17536469943577,75.9345434280883));
#60754=CARTESIAN_POINT('Ctrl Pts',(4.95264420849895,6.16890128837062,75.9341208887497));
#60755=CARTESIAN_POINT('Ctrl Pts',(5.30872120493341,5.88226259233086,75.9153802750712));
#60756=CARTESIAN_POINT('Ctrl Pts',(5.63236209333266,5.57314642905344,75.895128047366));
#60757=CARTESIAN_POINT('Ctrl Pts',(5.97250322988178,5.18821857395531,75.8715688587952));
#60758=CARTESIAN_POINT('Ctrl Pts',(6.01621341142032,5.1374685356768,75.8684917593541));
#60759=CARTESIAN_POINT('Ctrl Pts',(6.22048375360702,4.89411646452558,75.8538912740486));
#60760=CARTESIAN_POINT('Ctrl Pts',(6.37247529847644,4.69450297824402,75.8423725990371));
#60761=CARTESIAN_POINT('Ctrl Pts',(6.77575330470779,4.10910957999597,75.8102870633667));
#60762=CARTESIAN_POINT('Ctrl Pts',(7.00324531293333,3.70813424096044,75.7903119644353));
#60763=CARTESIAN_POINT('Ctrl Pts',(7.20774183315733,3.26088579358375,75.7703369358526));
#60764=CARTESIAN_POINT('Ctrl Pts',(7.22070291602865,3.23208414503129,75.769059958138));
#60765=CARTESIAN_POINT('Ctrl Pts',(7.23782292867703,3.19342366424338,75.7673582637505));
#60766=CARTESIAN_POINT('Ctrl Pts',(7.24213475135818,3.18363309609588,75.7669283775652));
#60767=CARTESIAN_POINT('Ctrl Pts',(7.24884625958942,3.16830952977511,75.7662571965326));
#60768=CARTESIAN_POINT('Ctrl Pts',(7.25125949266104,3.1627824999397,75.7660154442922));
#60769=CARTESIAN_POINT('Ctrl Pts',(7.25586583459554,3.15219960688778,75.765553187832));
#60770=CARTESIAN_POINT('Ctrl Pts',(7.25805998465954,3.14714420237679,75.7653326485742));
#60771=CARTESIAN_POINT('Ctrl Pts',(7.26318054237733,3.13531240740026,75.764817143518));
#60772=CARTESIAN_POINT('Ctrl Pts',(7.26610275449806,3.1285342006477,75.7645223192532));
#60773=CARTESIAN_POINT('Ctrl Pts',(7.27445161075847,3.10909384558267,75.7636781677722));
#60774=CARTESIAN_POINT('Ctrl Pts',(7.27985468505086,3.09642157092452,75.7631296341863));
#60775=CARTESIAN_POINT('Ctrl Pts',(7.31459032204418,3.01435975243527,75.7595886132279));
#60776=CARTESIAN_POINT('Ctrl Pts',(7.34296399785464,2.94456727066848,75.7566284133959));
#60777=CARTESIAN_POINT('Ctrl Pts',(7.42336899314471,2.7383968500386,75.7480281542163));
#60778=CARTESIAN_POINT('Ctrl Pts',(7.47262896743741,2.60096970177034,75.7424794197113));
#60779=CARTESIAN_POINT('Ctrl Pts',(7.59788202095205,2.21853148042592,75.7274809045449));
#60780=CARTESIAN_POINT('Ctrl Pts',(7.66580767061685,1.97106452192522,75.7182715523887));
#60781=CARTESIAN_POINT('Ctrl Pts',(7.84571908143169,1.16372910922274,75.6892059852111));
#60782=CARTESIAN_POINT('Ctrl Pts',(7.90920345579479,0.59497934499948,75.6703152001558));
#60783=CARTESIAN_POINT('Ctrl Pts',(7.91135931281254,-0.104364926786781,
75.64489712916));
#60784=CARTESIAN_POINT('Ctrl Pts',(7.90861295650032,-0.233103098924084,
75.6401214088781));
#60785=CARTESIAN_POINT('Ctrl Pts',(7.89803930332656,-0.464117396627604,
75.6312935212535));
#60786=CARTESIAN_POINT('Ctrl Pts',(7.89136229312373,-0.566418023908654,
75.6272929952555));
#60787=CARTESIAN_POINT('Ctrl Pts',(7.88179749672174,-0.679193035796358,
75.6227551933064));
#60788=CARTESIAN_POINT('Ctrl Pts',(7.88087381629139,-0.689828129933893,
75.6223260057941));
#60789=CARTESIAN_POINT('Ctrl Pts',(7.87955566729525,-0.704656815517333,
75.6217257919629));
#60790=CARTESIAN_POINT('Ctrl Pts',(7.87917936787542,-0.708852051123079,
75.6215557834132));
#60791=CARTESIAN_POINT('Ctrl Pts',(7.87851545229675,-0.716187974345506,
75.621258148387));
#60792=CARTESIAN_POINT('Ctrl Pts',(7.87822930790469,-0.719328797345784,
75.6211306050201));
#60793=CARTESIAN_POINT('Ctrl Pts',(7.87762499826165,-0.725918302168633,
75.6208627779526));
#60794=CARTESIAN_POINT('Ctrl Pts',(7.87730644645747,-0.729366946869954,
75.6207224723322));
#60795=CARTESIAN_POINT('Ctrl Pts',(7.87655108453428,-0.737486283894132,
75.6203918176643));
#60796=CARTESIAN_POINT('Ctrl Pts',(7.87611238428003,-0.74215680039298,75.6202013604028));
#60797=CARTESIAN_POINT('Ctrl Pts',(7.87462355042127,-0.757857310206448,
75.6195602552951));
#60798=CARTESIAN_POINT('Ctrl Pts',(7.87355440395534,-0.768885432985613,
75.6191085148364));
#60799=CARTESIAN_POINT('Ctrl Pts',(7.8709542304535,-0.795131711828499,75.6180300704666));
#60800=CARTESIAN_POINT('Ctrl Pts',(7.86940223501198,-0.810347699760125,
75.6174021889463));
#60801=CARTESIAN_POINT('Ctrl Pts',(7.85120809196158,-0.983742928767514,
75.6102175097682));
#60802=CARTESIAN_POINT('Ctrl Pts',(7.82984422872752,-1.14138172175509,75.6034052790451));
#60803=CARTESIAN_POINT('Ctrl Pts',(7.75348784949516,-1.60035437304463,75.5829698854906));
#60804=CARTESIAN_POINT('Ctrl Pts',(7.68573296522575,-1.89926302227668,75.5689040332123));
#60805=CARTESIAN_POINT('Ctrl Pts',(7.39357992036319,-2.91163099549431,75.5202142548614));
#60806=CARTESIAN_POINT('Ctrl Pts',(7.08554873456032,-3.59694727208695,75.4858731925408));
#60807=CARTESIAN_POINT('Ctrl Pts',(6.65912607762144,-4.27111910674453,75.4532711949426));
#60808=CARTESIAN_POINT('Ctrl Pts',(6.63201142187113,-4.31310133950437,75.451243911244));
#60809=CARTESIAN_POINT('Ctrl Pts',(6.59831674744036,-4.36420248013499,75.4487795160396));
#60810=CARTESIAN_POINT('Ctrl Pts',(6.59211308495563,-4.37356745274508,75.4483280160249));
#60811=CARTESIAN_POINT('Ctrl Pts',(6.58183495229566,-4.3890116447487,75.4475836411606));
#60812=CARTESIAN_POINT('Ctrl Pts',(6.5777719660684,-4.39509846531191,75.4472903253074));
#60813=CARTESIAN_POINT('Ctrl Pts',(6.5704246709892,-4.40607254985559,75.4467615957527));
#60814=CARTESIAN_POINT('Ctrl Pts',(6.56714334333645,-4.4109617976134,75.4465260674801));
#60815=CARTESIAN_POINT('Ctrl Pts',(6.5601227918356,-4.42139736953882,75.4460234308395));
#60816=CARTESIAN_POINT('Ctrl Pts',(6.55638198478108,-4.42694262592752,75.4457563838443));
#60817=CARTESIAN_POINT('Ctrl Pts',(6.54626591208577,-4.44189743144858,75.4450363107336));
#60818=CARTESIAN_POINT('Ctrl Pts',(6.53987738272898,-4.45129801333657,75.4445837979134));
#60819=CARTESIAN_POINT('Ctrl Pts',(6.50849644328835,-4.49726099675213,75.4423718771911));
#60820=CARTESIAN_POINT('Ctrl Pts',(6.48321733072806,-4.53362719579732,75.4406236141858));
#60821=CARTESIAN_POINT('Ctrl Pts',(6.27526581947524,-4.82748704189991,75.4265084870423));
#60822=CARTESIAN_POINT('Ctrl Pts',(6.07762808678988,-5.07405683920033,75.4147565016945));
#60823=CARTESIAN_POINT('Ctrl Pts',(5.80368840844783,-5.37677241885671,75.4001206645649));
#60824=CARTESIAN_POINT('Ctrl Pts',(5.74041000221317,-5.44427903577735,75.3968409184733));
#60825=CARTESIAN_POINT('Ctrl Pts',(5.62629390718222,-5.56181820721542,75.3910844396402));
#60826=CARTESIAN_POINT('Ctrl Pts',(5.57593688839234,-5.61230192217494,75.3885962975681));
#60827=CARTESIAN_POINT('Ctrl Pts',(5.46668339485634,-5.71890816891238,75.3832972037355));
#60828=CARTESIAN_POINT('Ctrl Pts',(5.40758981018975,-5.77481693021322,75.3804904811321));
#60829=CARTESIAN_POINT('Ctrl Pts',(5.04923642458443,-6.10353229848063,75.3637708875067));
#60830=CARTESIAN_POINT('Ctrl Pts',(4.73026516454419,-6.3539327855739,75.3501501401085));
#60831=CARTESIAN_POINT('Ctrl Pts',(4.17396304345769,-6.72544968805596,75.3262309813327));
#60832=CARTESIAN_POINT('Ctrl Pts',(3.94719468742527,-6.86099648426533,75.3164302476946));
#60833=CARTESIAN_POINT('Ctrl Pts',(3.69953787795537,-6.99268277112885,75.305226755931));
#60834=CARTESIAN_POINT('Ctrl Pts',(3.68495606507433,-7.00037796397623,75.3045653103867));
#60835=CARTESIAN_POINT('Ctrl Pts',(3.66534051668494,-7.01065131641605,75.303672982764));
#60836=CARTESIAN_POINT('Ctrl Pts',(3.66032782689947,-7.01326979253774,75.3034447285799));
#60837=CARTESIAN_POINT('Ctrl Pts',(3.65246907561156,-7.01736424381077,75.303086522711));
#60838=CARTESIAN_POINT('Ctrl Pts',(3.64962490885851,-7.01884387226221,75.3029568112737));
#60839=CARTESIAN_POINT('Ctrl Pts',(3.64417083803523,-7.02167704661222,75.3027079310689));
#60840=CARTESIAN_POINT('Ctrl Pts',(3.64156107665035,-7.02303086770143,75.3025887805192));
#60841=CARTESIAN_POINT('Ctrl Pts',(3.6361888811896,-7.02581390972235,75.302343380466));
#60842=CARTESIAN_POINT('Ctrl Pts',(3.63342636521468,-7.02724295312075,75.30221711961));
#60843=CARTESIAN_POINT('Ctrl Pts',(3.62504065297781,-7.03157459675625,75.3018336391608));
#60844=CARTESIAN_POINT('Ctrl Pts',(3.61941482702038,-7.03447207365111,75.3015760809706));
#60845=CARTESIAN_POINT('Ctrl Pts',(3.59126332088931,-7.04892827109666,75.300285850591));
#60846=CARTESIAN_POINT('Ctrl Pts',(3.56868595416626,-7.06038543869717,75.2992465659487));
#60847=CARTESIAN_POINT('Ctrl Pts',(3.50642266352921,-7.09160677824048,75.2963688763414));
#60848=CARTESIAN_POINT('Ctrl Pts',(3.46662546119993,-7.11114578384441,75.2945166545636));
#60849=CARTESIAN_POINT('Ctrl Pts',(3.33122992056975,-7.17621348561152,75.2881772519894));
#60850=CARTESIAN_POINT('Ctrl Pts',(3.23488528060808,-7.2201556972113,75.2836028038682));
#60851=CARTESIAN_POINT('Ctrl Pts',(2.92015971360336,-7.35613634603328,75.2685262451957));
#60852=CARTESIAN_POINT('Ctrl Pts',(2.69852466385739,-7.44029759439141,75.2577073136242));
#60853=CARTESIAN_POINT('Ctrl Pts',(1.64646644903902,-7.78659670313505,75.2064485383649));
#60854=CARTESIAN_POINT('Ctrl Pts',(0.779935994600486,-7.92049991186082,
75.1653840525867));
#60855=CARTESIAN_POINT('Ctrl Pts',(-0.104235593133335,-7.91032427355923,
75.1291093696334));
#60856=CARTESIAN_POINT('Ctrl Pts',(-0.117431775338263,-7.91013937627933,
75.1285690169856));
#60857=CARTESIAN_POINT('Ctrl Pts',(-0.177726048414574,-7.90914365352843,
75.1261048536175));
#60858=CARTESIAN_POINT('Ctrl Pts',(-0.224817258285966,-7.9079451935394,
75.1241935245935));
#60859=CARTESIAN_POINT('Ctrl Pts',(-0.28398466931383,-7.9059104490268,75.1218083076549));
#60860=CARTESIAN_POINT('Ctrl Pts',(-0.29607288721056,-7.90546697973152,
75.1213218478521));
#60861=CARTESIAN_POINT('Ctrl Pts',(-0.315095389034554,-7.90472542644363,
75.120557667594));
#60862=CARTESIAN_POINT('Ctrl Pts',(-0.322030354513464,-7.90444594027644,
75.1202793518456));
#60863=CARTESIAN_POINT('Ctrl Pts',(-0.33426625666628,-7.90393669143006,
75.1197887872038));
#60864=CARTESIAN_POINT('Ctrl Pts',(-0.33956734171407,-7.90371072174731,
75.1195764170383));
#60865=CARTESIAN_POINT('Ctrl Pts',(-0.351690188410239,-7.90318174151913,
75.1190911254828));
#60866=CARTESIAN_POINT('Ctrl Pts',(-0.358511797594762,-7.90287523116757,
75.118818316255));
#60867=CARTESIAN_POINT('Ctrl Pts',(-0.377241562963671,-7.90200935963912,
75.118070008549));
#60868=CARTESIAN_POINT('Ctrl Pts',(-0.389148887442308,-7.90143191210849,
75.1175950889263));
#60869=CARTESIAN_POINT('Ctrl Pts',(-0.451672982941602,-7.89825811867552,
75.1151055641147));
#60870=CARTESIAN_POINT('Ctrl Pts',(-0.502265787237247,-7.89520227700313,
75.1131056716775));
#60871=CARTESIAN_POINT('Ctrl Pts',(-0.642360652955859,-7.88538835573283,
75.1076064626397));
#60872=CARTESIAN_POINT('Ctrl Pts',(-0.731783370383624,-7.8775929365302,
75.1041401301939));
#60873=CARTESIAN_POINT('Ctrl Pts',(-1.18932543569304,-7.82984835134208,
75.0866057585264));
#60874=CARTESIAN_POINT('Ctrl Pts',(-1.55445774395648,-7.76561068144842,
75.0733116577115));
#60875=CARTESIAN_POINT('Ctrl Pts',(-1.98298535629342,-7.6587713932111,75.0578931998984));
#60876=CARTESIAN_POINT('Ctrl Pts',(-2.05196868312361,-7.64057817223776,
75.0554159152606));
#60877=CARTESIAN_POINT('Ctrl Pts',(-2.17814629308361,-7.60546880220136,
75.0508834753753));
#60878=CARTESIAN_POINT('Ctrl Pts',(-2.23541330157723,-7.58883419133082,
75.0488259019974));
#60879=CARTESIAN_POINT('Ctrl Pts',(-2.34137885466724,-7.55675033467469,
75.0450114055189));
#60880=CARTESIAN_POINT('Ctrl Pts',(-2.39012632043474,-7.54147377792694,
75.0432537547265));
#60881=CARTESIAN_POINT('Ctrl Pts',(-2.48102910153206,-7.51201660025889,
75.0399665480035));
#60882=CARTESIAN_POINT('Ctrl Pts',(-2.52321939565732,-7.49795056559365,
75.038436970822));
#60883=CARTESIAN_POINT('Ctrl Pts',(-2.60234336095535,-7.47082755863067,
75.0355581140971));
#60884=CARTESIAN_POINT('Ctrl Pts',(-2.63930300812443,-7.45785056188197,
75.0342091171041));
#60885=CARTESIAN_POINT('Ctrl Pts',(-2.70894169459582,-7.43281703365264,
75.0316572351446));
#60886=CARTESIAN_POINT('Ctrl Pts',(-2.74164045856353,-7.42081813198745,
75.030454751985));
#60887=CARTESIAN_POINT('Ctrl Pts',(-2.80353748768815,-7.39763989381527,
75.0281689269075));
#60888=CARTESIAN_POINT('Ctrl Pts',(-2.83275080869563,-7.38650264271761,
75.0270860128218));
#60889=CARTESIAN_POINT('Ctrl Pts',(-3.13260035774982,-7.27014790305459,
75.0159227205949));
#60890=CARTESIAN_POINT('Ctrl Pts',(-3.39730119123685,-7.15028406115013,
75.0056691052768));
#60891=CARTESIAN_POINT('Ctrl Pts',(-3.68077168369177,-7.00262082970465,
74.9936781594259));
#60892=CARTESIAN_POINT('Ctrl Pts',(-3.70666949180692,-6.98894698226858,
74.9925730224812));
#60893=CARTESIAN_POINT('Ctrl Pts',(-3.74013292644046,-6.97104022530597,
74.9911317850525));
#60894=CARTESIAN_POINT('Ctrl Pts',(-3.74776855564842,-6.96693813541936,
74.9908020274796));
#60895=CARTESIAN_POINT('Ctrl Pts',(-3.8503748658589,-6.91159744346697,74.9863585123374));
#60896=CARTESIAN_POINT('Ctrl Pts',(-3.94428248660473,-6.85844012443397,
74.9821458431518));
#60897=CARTESIAN_POINT('Ctrl Pts',(-4.04775740123271,-6.79703870023905,
74.9773250776704));
#60898=CARTESIAN_POINT('Ctrl Pts',(-4.05841710340704,-6.79067932418798,
74.9768264024764));
#60899=CARTESIAN_POINT('Ctrl Pts',(-4.07393093269104,-6.78137449146389,
74.9760976950002));
#60900=CARTESIAN_POINT('Ctrl Pts',(-4.07879696111116,-6.77844883344216,
74.9758687063703));
#60901=CARTESIAN_POINT('Ctrl Pts',(-4.08738891322262,-6.77327039395603,
74.9754636365002));
#60902=CARTESIAN_POINT('Ctrl Pts',(-4.09111613864862,-6.77101976791924,
74.9752876675537));
#60903=CARTESIAN_POINT('Ctrl Pts',(-4.09828881182738,-6.76668057825193,
74.974948557979));
#60904=CARTESIAN_POINT('Ctrl Pts',(-4.10173452665601,-6.76459245675534,
74.9747854401871));
#60905=CARTESIAN_POINT('Ctrl Pts',(-4.1108183713586,-6.75907810617024,74.9743548624282));
#60906=CARTESIAN_POINT('Ctrl Pts',(-4.11645380526456,-6.75564745944821,
74.9740871764412));
#60907=CARTESIAN_POINT('Ctrl Pts',(-4.1370857341212,-6.74305209203146,74.9731050978656));
#60908=CARTESIAN_POINT('Ctrl Pts',(-4.15205589551518,-6.73384449781604,
74.9723885428181));
#60909=CARTESIAN_POINT('Ctrl Pts',(-4.18873808529172,-6.71111380758679,
74.9706231659168));
#60910=CARTESIAN_POINT('Ctrl Pts',(-4.21041536223115,-6.69753519902802,
74.9695716522344));
#60911=CARTESIAN_POINT('Ctrl Pts',(-4.29302091828066,-6.64523169352483,
74.9655339961701));
#60912=CARTESIAN_POINT('Ctrl Pts',(-4.35348291586055,-6.60577920840755,
74.9625146294311));
#60913=CARTESIAN_POINT('Ctrl Pts',(-4.56908180229136,-6.46085158897698,
74.9515367832989));
#60914=CARTESIAN_POINT('Ctrl Pts',(-4.72099179277314,-6.35069630305085,
74.9434031101507));
#60915=CARTESIAN_POINT('Ctrl Pts',(-5.55097487494354,-5.70259842359616,
74.8971918493891));
#60916=CARTESIAN_POINT('Ctrl Pts',(-6.14124528887608,-5.06147289441774,
74.8582868142302));
#60917=CARTESIAN_POINT('Ctrl Pts',(-6.64278342095406,-4.29648135388938,
74.8210643351798));
#60918=CARTESIAN_POINT('Ctrl Pts',(-6.66927693366555,-4.25524016472949,
74.819079406937));
#60919=CARTESIAN_POINT('Ctrl Pts',(-6.70411899956952,-4.19987836421536,
74.8164430323171));
#60920=CARTESIAN_POINT('Ctrl Pts',(-6.71280920198177,-4.18597449289266,
74.8157832659632));
#60921=CARTESIAN_POINT('Ctrl Pts',(-6.72631012120633,-4.16422356131286,
74.8147547644515));
#60922=CARTESIAN_POINT('Ctrl Pts',(-6.73115045926393,-4.15639497767591,
74.8143853165966));
#60923=CARTESIAN_POINT('Ctrl Pts',(-6.74080623654395,-4.14071697686919,
74.8136468879669));
#60924=CARTESIAN_POINT('Ctrl Pts',(-6.7456216577009,-4.13286755810954,74.8132779073677));
#60925=CARTESIAN_POINT('Ctrl Pts',(-6.75638826830701,-4.11524840460448,
74.8124512964852));
#60926=CARTESIAN_POINT('Ctrl Pts',(-6.76233199963502,-4.10547412503793,
74.8119938451033));
#60927=CARTESIAN_POINT('Ctrl Pts',(-6.77962761495663,-4.07689256413663,
74.8106594256318));
#60928=CARTESIAN_POINT('Ctrl Pts',(-6.79092241522967,-4.05805080474741,
74.809783827594));
#60929=CARTESIAN_POINT('Ctrl Pts',(-6.87311044619286,-3.91964230434996,
74.8033815789275));
#60930=CARTESIAN_POINT('Ctrl Pts',(-6.94092116008519,-3.79827040802802,
74.7979301556462));
#60931=CARTESIAN_POINT('Ctrl Pts',(-7.15243665818085,-3.39508606202152,
74.780317024785));
#60932=CARTESIAN_POINT('Ctrl Pts',(-7.28244750168348,-3.1064339610442,74.7684931771233));
#60933=CARTESIAN_POINT('Ctrl Pts',(-7.58368703654001,-2.31390287227634,
74.7374098427156));
#60934=CARTESIAN_POINT('Ctrl Pts',(-7.72197650334821,-1.79930232279479,
74.7187080685195));
#60935=CARTESIAN_POINT('Ctrl Pts',(-7.81209422176409,-1.24734752017167,
74.6977405539795));
#60936=CARTESIAN_POINT('Ctrl Pts',(-7.81642405686987,-1.21992086371801,
74.6966960964807));
#60937=CARTESIAN_POINT('Ctrl Pts',(-7.83194396905852,-1.11813637000325,
74.6928088706968));
#60938=CARTESIAN_POINT('Ctrl Pts',(-7.842217939224,-1.04364395560218,74.6899420640016));
#60939=CARTESIAN_POINT('Ctrl Pts',(-7.86412117576441,-0.866173827354949,
74.6830403611618));
#60940=CARTESIAN_POINT('Ctrl Pts',(-7.87479181495238,-0.763093431508333,
74.6789743761494));
#60941=CARTESIAN_POINT('Ctrl Pts',(-7.88449381396879,-0.647178220215648,
74.6743125158825));
#60942=CARTESIAN_POINT('Ctrl Pts',(-7.88552279664459,-0.634517590096962,
74.6738021341312));
#60943=CARTESIAN_POINT('Ctrl Pts',(-7.8869724488813,-0.616132724246009,
74.6730591926453));
#60944=CARTESIAN_POINT('Ctrl Pts',(-7.88741739167083,-0.610410380493285,
74.6728276966247));
#60945=CARTESIAN_POINT('Ctrl Pts',(-7.8881902706487,-0.600328549014301,
74.672419385478));
#60946=CARTESIAN_POINT('Ctrl Pts',(-7.88852082168823,-0.595969259606479,
74.6722426863553));
#60947=CARTESIAN_POINT('Ctrl Pts',(-7.88914847521694,-0.587599783764911,
74.6719031488454));
#60948=CARTESIAN_POINT('Ctrl Pts',(-7.88944613408017,-0.583589639435366,
74.6717403354051));
#60949=CARTESIAN_POINT('Ctrl Pts',(-7.89007359526751,-0.575048088177602,
74.6713932702122));
#60950=CARTESIAN_POINT('Ctrl Pts',(-7.89040255158785,-0.570516622210531,
74.6712089803689));
#60951=CARTESIAN_POINT('Ctrl Pts',(-7.89117955925274,-0.559683902082172,
74.6707680268791));
#60952=CARTESIAN_POINT('Ctrl Pts',(-7.89162396655545,-0.553382396496017,
74.6705111974594));
#60953=CARTESIAN_POINT('Ctrl Pts',(-7.89278970467752,-0.53656571560085,
74.6698249290095));
#60954=CARTESIAN_POINT('Ctrl Pts',(-7.89349756814213,-0.52604964544283,
74.6693948694301));
#60955=CARTESIAN_POINT('Ctrl Pts',(-7.90537857213335,-0.34411953389681,
74.6619385649561));
#60956=CARTESIAN_POINT('Ctrl Pts',(-7.91098514682664,-0.172414955914368,
74.6546275518882));
#60957=CARTESIAN_POINT('Ctrl Pts',(-7.91099997052785,-0.000682867722154,
74.6471121226888));
#60958=CARTESIAN_POINT('',(-7.91099996455606,-0.000133956286235481,72.642331508237));
#60959=CARTESIAN_POINT('Ctrl Pts',(-7.91099994932565,-0.00089541584189321,
74.6422459153707));
#60960=CARTESIAN_POINT('Ctrl Pts',(-7.91102194644307,0.193449140794186,
74.6343900678167));
#60961=CARTESIAN_POINT('Ctrl Pts',(-7.90387815483653,0.388049300595132,
74.6265342202626));
#60962=CARTESIAN_POINT('Ctrl Pts',(-7.88953808641908,0.582331334330231,
74.6186783727085));
#60963=CARTESIAN_POINT('Ctrl Pts',(-7.87521209893698,0.776422596816661,
74.6108302390425));
#60964=CARTESIAN_POINT('Ctrl Pts',(-7.8537039329886,0.970196009224877,74.6029821053764));
#60965=CARTESIAN_POINT('Ctrl Pts',(-7.82503509210339,1.16307644088875,74.5951339717104));
#60966=CARTESIAN_POINT('Ctrl Pts',(-7.79638889121586,1.35580455343575,74.5872920357741));
#60967=CARTESIAN_POINT('Ctrl Pts',(-7.76059332992449,1.54764074561036,74.5794500998377));
#60968=CARTESIAN_POINT('Ctrl Pts',(-7.71772184260884,1.73801339468901,74.5716081639014));
#60969=CARTESIAN_POINT('Ctrl Pts',(-7.67487597314194,1.92827228662892,74.5637709139124));
#60970=CARTESIAN_POINT('Ctrl Pts',(-7.6249626772959,2.11706903739895,74.5559336639233));
#60971=CARTESIAN_POINT('Ctrl Pts',(-7.56810678752856,2.3038404138664,74.5480964139343));
#60972=CARTESIAN_POINT('Ctrl Pts',(-7.51127394917922,2.49053606651551,74.5402623414476));
#60973=CARTESIAN_POINT('Ctrl Pts',(-7.44750422697393,2.67520764683579,74.532428268961));
#60974=CARTESIAN_POINT('Ctrl Pts',(-7.37697285163034,2.8573051195679,74.5245941964743));
#60975=CARTESIAN_POINT('Ctrl Pts',(-7.30644453438772,3.03939469691365,74.5167604636575));
#60976=CARTESIAN_POINT('Ctrl Pts',(-7.22915526570112,3.21891005951464,74.5089267308408));
#60977=CARTESIAN_POINT('Ctrl Pts',(-7.1453293354841,3.39531879025673,74.501092998024));
#60978=CARTESIAN_POINT('Ctrl Pts',(-7.06150186723957,3.57173075772376,74.4932591214749));
#60979=CARTESIAN_POINT('Ctrl Pts',(-6.9711376478802,3.74503566313881,74.4854252449258));
#60980=CARTESIAN_POINT('Ctrl Pts',(-6.87450807130635,3.91472346118392,74.4775913683767));
#60981=CARTESIAN_POINT('Ctrl Pts',(-6.7778599042609,4.08444390530183,74.4697559846756));
#60982=CARTESIAN_POINT('Ctrl Pts',(-6.67494415161497,4.25054555136554,74.4619206009745));
#60983=CARTESIAN_POINT('Ctrl Pts',(-6.56607697610846,4.41254508688788,74.4540852172734));
#60984=CARTESIAN_POINT('Ctrl Pts',(-6.45716990750051,4.57460398524273,74.4462469623877));
#60985=CARTESIAN_POINT('Ctrl Pts',(-6.34230726650615,4.73255748814937,74.438408707502));
#60986=CARTESIAN_POINT('Ctrl Pts',(-6.22184723591979,4.88595312839545,74.4305704526164));
#60987=CARTESIAN_POINT('Ctrl Pts',(-6.10125341770897,5.03951913584309,74.422723492258));
#60988=CARTESIAN_POINT('Ctrl Pts',(-5.97505000736939,5.18851689268872,74.4148765318997));
#60989=CARTESIAN_POINT('Ctrl Pts',(-5.84363476146546,5.33252789721652,74.4070295715414));
#60990=CARTESIAN_POINT('Ctrl Pts',(-5.71214195379757,5.47662389757161,74.399177979878));
#60991=CARTESIAN_POINT('Ctrl Pts',(-5.57543142418788,5.61572703025123,74.3913263882147));
#60992=CARTESIAN_POINT('Ctrl Pts',(-5.43393623575889,5.74945719052734,74.3834747965513));
#60993=CARTESIAN_POINT('Ctrl Pts',(-5.29223343387657,5.88338357076468,74.3756116843827));
#60994=CARTESIAN_POINT('Ctrl Pts',(-5.14573220875179,6.01192099649521,74.3677485722141));
#60995=CARTESIAN_POINT('Ctrl Pts',(-4.99489806692352,6.13473017345047,74.3598854600455));
#60996=CARTESIAN_POINT('Ctrl Pts',(-4.8744750196751,6.23277863343284,74.3536077041163));
#60997=CARTESIAN_POINT('Ctrl Pts',(-4.75129077201187,6.32717663391295,74.347329948187));
#60998=CARTESIAN_POINT('Ctrl Pts',(-4.62559424657141,6.41777211079401,74.3410521922577));
#60999=CARTESIAN_POINT('Ctrl Pts',(-4.46854943026035,6.53096179503982,74.3332087851047));
#61000=CARTESIAN_POINT('Ctrl Pts',(-4.30710127573518,6.63856101387509,74.3253653779516));
#61001=CARTESIAN_POINT('Ctrl Pts',(-4.14168797058622,6.74020339116717,74.3175219707985));
#61002=CARTESIAN_POINT('Ctrl Pts',(-3.97646886206965,6.84172643944058,74.3096877718724));
#61003=CARTESIAN_POINT('Ctrl Pts',(-3.80729416822044,6.93730638928325,74.3018535729463));
#61004=CARTESIAN_POINT('Ctrl Pts',(-3.63463451777544,7.02661745950321,74.2940193740201));
#61005=CARTESIAN_POINT('Ctrl Pts',(-3.462143997643,7.11584104426155,74.286192849154));
#61006=CARTESIAN_POINT('Ctrl Pts',(-3.28617562885373,7.19880781798418,74.2783663242879));
#61007=CARTESIAN_POINT('Ctrl Pts',(-3.10722851531469,7.27523552564556,74.2705397994217));
#61008=CARTESIAN_POINT('Ctrl Pts',(-2.92842191524121,7.3516032204805,74.2627194201262));
#61009=CARTESIAN_POINT('Ctrl Pts',(-2.74664155057281,7.42144193847331,74.2548990408307));
#61010=CARTESIAN_POINT('Ctrl Pts',(-2.56241076835612,7.48451548560177,74.2470786615353));
#61011=CARTESIAN_POINT('Ctrl Pts',(-2.37828886025944,7.54755175841125,74.2392629038177));
#61012=CARTESIAN_POINT('Ctrl Pts',(-2.19171975084654,7.60383071078097,74.2314471461001));
#61013=CARTESIAN_POINT('Ctrl Pts',(-2.00324657220252,7.65316432405308,74.2236313883826));
#61014=CARTESIAN_POINT('Ctrl Pts',(-1.81484817241031,7.70247836365968,74.2158187316547));
#61015=CARTESIAN_POINT('Ctrl Pts',(-1.62454754815614,7.74485246558273,74.2080060749269));
#61016=CARTESIAN_POINT('Ctrl Pts',(-1.43290297449505,7.78014846038835,74.200193418199));
#61017=CARTESIAN_POINT('Ctrl Pts',(-1.24126560417739,7.81544312852363,74.1923810551254));
#61018=CARTESIAN_POINT('Ctrl Pts',(-1.04828472912884,7.84366014701759,74.1845686920519));
#61019=CARTESIAN_POINT('Ctrl Pts',(-0.854529267370442,7.86471237434703,
74.1767563289783));
#61020=CARTESIAN_POINT('Ctrl Pts',(-0.660768106299891,7.88576522092723,
74.1689437361043));
#61021=CARTESIAN_POINT('Ctrl Pts',(-0.466232662795107,7.89965281774444,
74.1611311432302));
#61022=CARTESIAN_POINT('Ctrl Pts',(-0.27149740643086,7.90633987116044,74.1533185503562));
#61023=CARTESIAN_POINT('Ctrl Pts',(-0.076722163289667,7.91302829769048,
74.1455043532507));
#61024=CARTESIAN_POINT('Ctrl Pts',(0.118252622912289,7.91251322335745,74.1376901561453));
#61025=CARTESIAN_POINT('Ctrl Pts',(0.312851893044608,7.90481149003684,74.1298759590399));
#61026=CARTESIAN_POINT('Ctrl Pts',(0.507525359154526,7.89710682023227,74.1220587825708));
#61027=CARTESIAN_POINT('Ctrl Pts',(0.70182267285472,7.88221004719473,74.1142416061017));
#61028=CARTESIAN_POINT('Ctrl Pts',(0.89517315124006,7.86018994867802,74.1064244296327));
#61029=CARTESIAN_POINT('Ctrl Pts',(1.08873337038756,7.83814596342317,74.0985987733265));
#61030=CARTESIAN_POINT('Ctrl Pts',(1.28134435330082,7.80896325924617,74.0907731170204));
#61031=CARTESIAN_POINT('Ctrl Pts',(1.47244382938962,7.77276206822854,74.0829474607143));
#61032=CARTESIAN_POINT('Ctrl Pts',(1.66365945679525,7.7365388739271,74.075117047931));
#61033=CARTESIAN_POINT('Ctrl Pts',(1.85336140466193,7.6932887691761,74.0672866351478));
#61034=CARTESIAN_POINT('Ctrl Pts',(2.04100176571583,7.6431821116826,74.0594562223645));
#61035=CARTESIAN_POINT('Ctrl Pts',(2.22889857301095,7.5930069739117,74.0516151078329));
#61036=CARTESIAN_POINT('Ctrl Pts',(2.41472783098999,7.53595666990954,74.0437739933013));
#61037=CARTESIAN_POINT('Ctrl Pts',(2.59795976063738,7.4722504027976,74.0359328787697));
#61038=CARTESIAN_POINT('Ctrl Pts',(2.69675872130326,7.43789987780628,74.0317049367966));
#61039=CARTESIAN_POINT('Ctrl Pts',(2.7948029183207,7.40161502359304,74.0274769948233));
#61040=CARTESIAN_POINT('Ctrl Pts',(2.89201224625962,7.3634357583593,74.0232490528502));
#61041=CARTESIAN_POINT('Ctrl Pts',(3.07390617094678,7.29199635493702,74.0153379091857));
#61042=CARTESIAN_POINT('Ctrl Pts',(3.25339594683619,7.21371711665667,74.0074267655212));
#61043=CARTESIAN_POINT('Ctrl Pts',(3.42993046795433,7.12877955789058,73.9995156218567));
#61044=CARTESIAN_POINT('Ctrl Pts',(3.60627360478942,7.04393408147578,73.9916130548069));
#61045=CARTESIAN_POINT('Ctrl Pts',(3.77966756050509,6.95244481072383,73.983710487757));
#61046=CARTESIAN_POINT('Ctrl Pts',(3.94957870478955,6.85454222064996,73.9758079207072));
#61047=CARTESIAN_POINT('Ctrl Pts',(4.1193371863076,6.75672759467228,73.9679124540024));
#61048=CARTESIAN_POINT('Ctrl Pts',(4.28561879324678,6.65251129941072,73.9600169872976));
#61049=CARTESIAN_POINT('Ctrl Pts',(4.44791186724698,6.54217097156621,73.9521215205928));
#61050=CARTESIAN_POINT('Ctrl Pts',(4.61008924068536,6.43190930658517,73.9442316826551));
#61051=CARTESIAN_POINT('Ctrl Pts',(4.76828346234788,6.315532500463,73.9363418447176));
#61052=CARTESIAN_POINT('Ctrl Pts',(4.92200915181058,6.19336313399214,73.9284520067799));
#61053=CARTESIAN_POINT('Ctrl Pts',(5.07565376969686,6.07125819698108,73.9205663297708));
#61054=CARTESIAN_POINT('Ctrl Pts',(5.2248342819248,5.94336700090116,73.9126806527617));
#61055=CARTESIAN_POINT('Ctrl Pts',(5.36909566265947,5.81005445458227,73.9047949757526));
#61056=CARTESIAN_POINT('Ctrl Pts',(5.51330772398102,5.67678748453967,73.8969119946622));
#61057=CARTESIAN_POINT('Ctrl Pts',(5.65260375261238,5.53810309195948,73.8890290135718));
#61058=CARTESIAN_POINT('Ctrl Pts',(5.78656288774104,5.39440552296711,73.8811460324815));
#61059=CARTESIAN_POINT('Ctrl Pts',(5.92052402967655,5.25070580127895,73.8732629332982));
#61060=CARTESIAN_POINT('Ctrl Pts',(6.04914787705711,5.10199299955927,73.8653798341149));
#61061=CARTESIAN_POINT('Ctrl Pts',(6.17205105019653,4.9487075922677,73.8574967349317));
#61062=CARTESIAN_POINT('Ctrl Pts',(6.29496182703056,4.79541270161295,73.8496131480419));
#61063=CARTESIAN_POINT('Ctrl Pts',(6.41215100808309,4.6375449105039,73.8417295611521));
#61064=CARTESIAN_POINT('Ctrl Pts',(6.52327606147301,4.4755771053366,73.8338459742624));
#61065=CARTESIAN_POINT('Ctrl Pts',(6.63442666983935,4.31357205309211,73.8259605744162));
#61066=CARTESIAN_POINT('Ctrl Pts',(6.73951017654278,4.1474653924283,73.81807517457));
#61067=CARTESIAN_POINT('Ctrl Pts',(6.83822774164264,3.97775845840707,73.8101897747239));
#61068=CARTESIAN_POINT('Ctrl Pts',(6.9369846029145,3.80798396971245,73.8023012359629));
#61069=CARTESIAN_POINT('Ctrl Pts',(7.02937029991796,3.63460664989781,73.7944126972019));
#61070=CARTESIAN_POINT('Ctrl Pts',(7.11513213477735,3.45815206499928,73.7865241584409));
#61071=CARTESIAN_POINT('Ctrl Pts',(7.2009852462306,3.28150967892427,73.7786272238829));
#61072=CARTESIAN_POINT('Ctrl Pts',(7.28020026341932,3.10178379628958,73.770730289325));
#61073=CARTESIAN_POINT('Ctrl Pts',(7.35257237048228,2.91952060051313,73.7628333547671));
#61074=CARTESIAN_POINT('Ctrl Pts',(7.42498861809563,2.73714624039307,73.7549316037813));
#61075=CARTESIAN_POINT('Ctrl Pts',(7.4905535200444,2.55223180610671,73.7470298527954));
#61076=CARTESIAN_POINT('Ctrl Pts',(7.54911218770278,2.36533849109959,73.7391281018096));
#61077=CARTESIAN_POINT('Ctrl Pts',(7.6077465975999,2.17820344043406,73.7312161303673));
#61078=CARTESIAN_POINT('Ctrl Pts',(7.65935658192268,1.98908472824269,73.7233041589251));
#61079=CARTESIAN_POINT('Ctrl Pts',(7.70383813669256,1.79855468742024,73.7153921874828));
#61080=CARTESIAN_POINT('Ctrl Pts',(7.72247764336563,1.71871516774285,73.7120767628027));
#61081=CARTESIAN_POINT('Ctrl Pts',(7.73986606790911,1.63862790595284,73.7087613381226));
#61082=CARTESIAN_POINT('Ctrl Pts',(7.75599846688739,1.5583352597052,73.7054459134424));
#61083=CARTESIAN_POINT('Ctrl Pts',(7.79449283298146,1.36674475146895,73.6975348041545));
#61084=CARTESIAN_POINT('Ctrl Pts',(7.82593565520974,1.17346951254426,73.6896236948665));
#61085=CARTESIAN_POINT('Ctrl Pts',(7.85018093930971,0.979071100634962,73.6817125855785));
#61086=CARTESIAN_POINT('Ctrl Pts',(7.87439993954777,0.784883432431188,73.6738100525771));
#61087=CARTESIAN_POINT('Ctrl Pts',(7.89143690121566,0.589575355637895,73.6659075195756));
#61088=CARTESIAN_POINT('Ctrl Pts',(7.90119645078819,0.393720263705267,73.6580049865742));
#61089=CARTESIAN_POINT('Ctrl Pts',(7.91094723194043,0.198041136836178,73.6501095535655));
#61090=CARTESIAN_POINT('Ctrl Pts',(7.9134336089223,0.00181631610688981,
73.6422141205568));
#61091=CARTESIAN_POINT('Ctrl Pts',(7.90861175274931,-0.194373723212607,
73.634318687548));
#61092=CARTESIAN_POINT('Ctrl Pts',(7.9037933339166,-0.390423905203012,73.6264288829299));
#61093=CARTESIAN_POINT('Ctrl Pts',(7.8916770700637,-0.586439011857354,73.6185390783117));
#61094=CARTESIAN_POINT('Ctrl Pts',(7.87227114556442,-0.781836306853166,
73.6106492736936));
#61095=CARTESIAN_POINT('Ctrl Pts',(7.85287545438328,-0.977130563074305,
73.6027636296029));
#61096=CARTESIAN_POINT('Ctrl Pts',(7.82619779635584,-1.17180731448945,73.5948779855122));
#61097=CARTESIAN_POINT('Ctrl Pts',(7.79229837886304,-1.36528640759678,73.5869923414214));
#61098=CARTESIAN_POINT('Ctrl Pts',(7.75841054896432,-1.55869936513715,73.5791093928237));
#61099=CARTESIAN_POINT('Ctrl Pts',(7.71730593897962,-1.75091514104126,73.571226444226));
#61100=CARTESIAN_POINT('Ctrl Pts',(7.66909632977393,-1.94136098772175,73.5633434956283));
#61101=CARTESIAN_POINT('Ctrl Pts',(7.62088599392436,-2.13180970491528,73.555460428214));
#61102=CARTESIAN_POINT('Ctrl Pts',(7.56557052129184,-2.3204881032442,73.5475773607998));
#61103=CARTESIAN_POINT('Ctrl Pts',(7.50331244954073,-2.50683531261373,73.5396942933856));
#61104=CARTESIAN_POINT('Ctrl Pts',(7.44105052245668,-2.69319406153968,73.5318107378122));
#61105=CARTESIAN_POINT('Ctrl Pts',(7.37184524835379,-2.87722100640294,73.5239271822388));
#61106=CARTESIAN_POINT('Ctrl Pts',(7.29590853774536,-3.05837205206535,73.5160436266654));
#61107=CARTESIAN_POINT('Ctrl Pts',(7.21995435962968,-3.2395647673916,73.50815825766));
#61108=CARTESIAN_POINT('Ctrl Pts',(7.13726579291068,-3.41787994716892,73.5002728886546));
#61109=CARTESIAN_POINT('Ctrl Pts',(7.04810233046337,-3.59279480896374,73.4923875196491));
#61110=CARTESIAN_POINT('Ctrl Pts',(6.9589033692351,-3.76777930987076,73.4844990112301));
#61111=CARTESIAN_POINT('Ctrl Pts',(6.86322453218225,-3.9393604882114,73.476610502811));
#61112=CARTESIAN_POINT('Ctrl Pts',(6.76137067674087,-4.10704121865226,73.468721994392));
#61113=CARTESIAN_POINT('Ctrl Pts',(6.6594084060418,-4.27490043177816,73.4608250892886));
#61114=CARTESIAN_POINT('Ctrl Pts',(6.55125816750903,-4.43885060946561,73.4529281841853));
#61115=CARTESIAN_POINT('Ctrl Pts',(6.43726808841204,-4.59842370360888,73.4450312790819));
#61116=CARTESIAN_POINT('Ctrl Pts',(6.32320847851897,-4.7580941329269,73.4371295570848));
#61117=CARTESIAN_POINT('Ctrl Pts',(6.20330213666765,-4.91338188362191,73.4292278350876));
#61118=CARTESIAN_POINT('Ctrl Pts',(6.0779368546735,-5.06385274179667,73.4213261130905));
#61119=CARTESIAN_POINT('Ctrl Pts',(5.9524094045112,-5.21451824383967,73.4134141697007));
#61120=CARTESIAN_POINT('Ctrl Pts',(5.82140913931665,-5.36035415185085,73.4055022263108));
#61121=CARTESIAN_POINT('Ctrl Pts',(5.68536078078645,-5.50096298772272,73.397590282921));
#61122=CARTESIAN_POINT('Ctrl Pts',(5.62834393133281,-5.55989109911908,73.3942744466256));
#61123=CARTESIAN_POINT('Ctrl Pts',(5.57044084668786,-5.61790161832553,73.3909586103302));
#61124=CARTESIAN_POINT('Ctrl Pts',(5.51168446450331,-5.67496743283633,73.3876427740348));
#61125=CARTESIAN_POINT('Ctrl Pts',(5.37275346019076,-5.80990104561383,73.3798023922834));
#61126=CARTESIAN_POINT('Ctrl Pts',(5.22865548944522,-5.93993266925251,73.371962010532));
#61127=CARTESIAN_POINT('Ctrl Pts',(5.07977286725619,-6.06463755034774,73.3641216287806));
#61128=CARTESIAN_POINT('Ctrl Pts',(4.93105669264826,-6.18920301405829,73.3562900124081));
#61129=CARTESIAN_POINT('Ctrl Pts',(4.77756678462485,-6.30845336992658,73.3484583960355));
#61130=CARTESIAN_POINT('Ctrl Pts',(4.61972327526206,-6.42199952195592,73.3406267796629));
#61131=CARTESIAN_POINT('Ctrl Pts',(4.46202554069436,-6.53544080957168,73.3328023961013));
#61132=CARTESIAN_POINT('Ctrl Pts',(4.2999824952884,-6.64318818069257,73.3249780125397));
#61133=CARTESIAN_POINT('Ctrl Pts',(4.13404857025015,-6.74489165360072,73.3171536289781));
#61134=CARTESIAN_POINT('Ctrl Pts',(3.9682356448381,-6.84652096396374,73.3093349509857));
#61135=CARTESIAN_POINT('Ctrl Pts',(3.79853778921688,-6.94211497125855,73.3015162729933));
#61136=CARTESIAN_POINT('Ctrl Pts',(3.62543989696728,-7.03136590951416,73.2936975950009));
#61137=CARTESIAN_POINT('Ctrl Pts',(3.45243460117617,-7.12056910414509,73.2858830995082));
#61138=CARTESIAN_POINT('Ctrl Pts',(3.27603320358031,-7.20343582829939,73.2780686040155));
#61139=CARTESIAN_POINT('Ctrl Pts',(3.096746940803,-7.27970324839051,73.2702541085229));
#61140=CARTESIAN_POINT('Ctrl Pts',(2.91752176390836,-7.35594468287289,73.2624422755619));
#61141=CARTESIAN_POINT('Ctrl Pts',(2.73541400341827,-7.4255911558716,73.2546304426009));
#61142=CARTESIAN_POINT('Ctrl Pts',(2.55095687597675,-7.4884270722834,73.2468186096399));
#61143=CARTESIAN_POINT('Ctrl Pts',(2.36649110968891,-7.55126593154611,73.2390064108204));
#61144=CARTESIAN_POINT('Ctrl Pts',(2.17967608651558,-7.60729347493693,73.2311942120008));
#61145=CARTESIAN_POINT('Ctrl Pts',(1.99106275853056,-7.65634312786416,73.2233820131813));
#61146=CARTESIAN_POINT('Ctrl Pts',(1.80243400734703,-7.70539679165605,73.2155691755463));
#61147=CARTESIAN_POINT('Ctrl Pts',(1.61200699876838,-7.74747133899127,73.2077563379113));
#61148=CARTESIAN_POINT('Ctrl Pts',(1.42034544108779,-7.78245075975307,73.1999435002764));
#61149=CARTESIAN_POINT('Ctrl Pts',(1.22863448724491,-7.81743919562028,73.1921286490702));
#61150=CARTESIAN_POINT('Ctrl Pts',(1.03568869647809,-7.84532879890732,73.1843137978641));
#61151=CARTESIAN_POINT('Ctrl Pts',(0.842079659009908,-7.86605510074025,
73.1764989466579));
#61152=CARTESIAN_POINT('Ctrl Pts',(0.648386654184466,-7.88679039147584,
73.1686807061864));
#61153=CARTESIAN_POINT('Ctrl Pts',(0.454030179016691,-7.90035615466375,
73.160862465715));
#61154=CARTESIAN_POINT('Ctrl Pts',(0.259584759797906,-7.90673995730735,
73.1530442252434));
#61155=CARTESIAN_POINT('Ctrl Pts',(0.0649130088055798,-7.91313119060877,
73.1452168844484));
#61156=CARTESIAN_POINT('Ctrl Pts',(-0.129847541460096,-7.91232375521652,
73.1373895436533));
#61157=CARTESIAN_POINT('Ctrl Pts',(-0.32412344744981,-7.90435734204959,
73.1295622028582));
#61158=CARTESIAN_POINT('Ctrl Pts',(-0.518526178365934,-7.89638572834192,
73.12172975231));
#61159=CARTESIAN_POINT('Ctrl Pts',(-0.712443285170314,-7.8812458507839,
73.1138973017618));
#61160=CARTESIAN_POINT('Ctrl Pts',(-0.905308544782102,-7.85902903918445,
73.1060648512135));
#61161=CARTESIAN_POINT('Ctrl Pts',(-1.09845058537667,-7.83678034423307,
73.0982211603136));
#61162=CARTESIAN_POINT('Ctrl Pts',(-1.29053741764301,-7.80743448352382,
73.0903774694136));
#61163=CARTESIAN_POINT('Ctrl Pts',(-1.48101390737776,-7.77113368860385,
73.0825337785136));
#61164=CARTESIAN_POINT('Ctrl Pts',(-1.58376893255215,-7.75155075161753,
73.0783023972181));
#61165=CARTESIAN_POINT('Ctrl Pts',(-1.68605557863687,-7.72994464739893,
73.0740710159226));
#61166=CARTESIAN_POINT('Ctrl Pts',(-1.78778884638401,-7.7063436233239,73.0698396346272));
#61167=CARTESIAN_POINT('Ctrl Pts',(-1.97815190839978,-7.66218144010575,
73.061921883455));
#61168=CARTESIAN_POINT('Ctrl Pts',(-2.1671452454434,-7.61089943386916,73.0540041322827));
#61169=CARTESIAN_POINT('Ctrl Pts',(-2.35419659870376,-7.55259421488085,
73.0460863811105));
#61170=CARTESIAN_POINT('Ctrl Pts',(-2.54103304357766,-7.4943559843442,73.0381777268579));
#61171=CARTESIAN_POINT('Ctrl Pts',(-2.72593162325107,-7.42911071492126,
73.0302690726053));
#61172=CARTESIAN_POINT('Ctrl Pts',(-2.90832993989894,-7.35700604598687,
73.0223604183527));
#61173=CARTESIAN_POINT('Ctrl Pts',(-3.09055245868333,-7.28497087246768,
73.0144593865637));
#61174=CARTESIAN_POINT('Ctrl Pts',(-3.27027919682617,-7.20608959507233,
73.0065583547746));
#61175=CARTESIAN_POINT('Ctrl Pts',(-3.44696232993268,-7.12055978810831,
72.9986573229856));
#61176=CARTESIAN_POINT('Ctrl Pts',(-3.62350786865408,-7.03509658864096,
72.9907624442322));
#61177=CARTESIAN_POINT('Ctrl Pts',(-3.79701421605697,-6.94299532447365,
72.9828675654788));
#61178=CARTESIAN_POINT('Ctrl Pts',(-3.96695270934947,-6.84450196886413,
72.9749726867254));
#61179=CARTESIAN_POINT('Ctrl Pts',(-4.13679029977623,-6.7460670947772,72.9670824956438));
#61180=CARTESIAN_POINT('Ctrl Pts',(-4.30306396017696,-6.64124786415838,
72.9591923045622));
#61181=CARTESIAN_POINT('Ctrl Pts',(-4.46526861175117,-6.53033668541751,
72.9513021134806));
#61182=CARTESIAN_POINT('Ctrl Pts',(-4.62740695520858,-6.41947084638376,
72.9434151478535));
#61183=CARTESIAN_POINT('Ctrl Pts',(-4.78547932102437,-6.30251821654022,
72.9355281822263));
#61184=CARTESIAN_POINT('Ctrl Pts',(-4.93900843104948,-6.17981526568733,
72.9276412165992));
#61185=CARTESIAN_POINT('Ctrl Pts',(-5.09252420868523,-6.05712297029592,
72.9197549358721));
#61186=CARTESIAN_POINT('Ctrl Pts',(-5.24149724359643,-5.92868155869958,
72.911868655145));
#61187=CARTESIAN_POINT('Ctrl Pts',(-5.38548185032401,-5.79486895795157,
72.9039823744179));
#61188=CARTESIAN_POINT('Ctrl Pts',(-5.52946620431588,-5.66105659208437,
72.8960961075336));
#61189=CARTESIAN_POINT('Ctrl Pts',(-5.66846189478627,-5.52187329002544,
72.8882098406493));
#61190=CARTESIAN_POINT('Ctrl Pts',(-5.80205867807116,-5.37773521998054,
72.8803235737649));
#61191=CARTESIAN_POINT('Ctrl Pts',(-5.93567761840211,-5.23357324461563,
72.8724359989421));
#61192=CARTESIAN_POINT('Ctrl Pts',(-6.06389563317599,-5.08445511660056,
72.8645484241192));
#61193=CARTESIAN_POINT('Ctrl Pts',(-6.18634133258751,-4.93083176722949,
72.8566608492964));
#61194=CARTESIAN_POINT('Ctrl Pts',(-6.30882786228494,-4.77715719118971,
72.8487706443123));
#61195=CARTESIAN_POINT('Ctrl Pts',(-6.42553802684242,-4.61897466976535,
72.8408804393282));
#61196=CARTESIAN_POINT('Ctrl Pts',(-6.53614235278993,-4.45676610829711,
72.8329902343441));
#61197=CARTESIAN_POINT('Ctrl Pts',(-6.64685348565564,-4.29440090741709,
72.8250924100515));
#61198=CARTESIAN_POINT('Ctrl Pts',(-6.75144680858466,-4.12800218571056,
72.8171945857589));
#61199=CARTESIAN_POINT('Ctrl Pts',(-6.84963706251331,-3.95807947265389,
72.8092967614663));
#61200=CARTESIAN_POINT('Ctrl Pts',(-6.9478816865164,-3.78806266970347,72.8013945639771));
#61201=CARTESIAN_POINT('Ctrl Pts',(-7.03971601159217,-3.61451828871069,
72.7934923664878));
#61202=CARTESIAN_POINT('Ctrl Pts',(-7.1249018280747,-3.43797832167363,72.7855901689985));
#61203=CARTESIAN_POINT('Ctrl Pts',(-7.21019047081311,-3.26122525644048,
72.7776784329098));
#61204=CARTESIAN_POINT('Ctrl Pts',(-7.28881443710697,-3.08146969736468,
72.7697666968211));
#61205=CARTESIAN_POINT('Ctrl Pts',(-7.36058412422407,-2.8992623803686,72.7618549607323));
#61206=CARTESIAN_POINT('Ctrl Pts',(-7.39027285456639,-2.82388927902195,
72.7585821388947));
#61207=CARTESIAN_POINT('Ctrl Pts',(-7.41878927289718,-2.74809680284435,
72.755309317057));
#61208=CARTESIAN_POINT('Ctrl Pts',(-7.44612248664829,-2.6719245711342,72.7520364952194));
#61209=CARTESIAN_POINT('Ctrl Pts',(-7.52247326301973,-2.45915013919315,
72.7428944129709));
#61210=CARTESIAN_POINT('Ctrl Pts',(-7.58973959628872,-2.24298999729443,
72.7337523307223));
#61211=CARTESIAN_POINT('Ctrl Pts',(-7.64765336366459,-2.02418354632915,
72.7246102484738));
#61212=CARTESIAN_POINT('Ctrl Pts',(-7.70439061686576,-1.80982213326664,
72.7156538869932));
#61213=CARTESIAN_POINT('Ctrl Pts',(-7.75215150291776,-1.59292105319892,
72.7066975255126));
#61214=CARTESIAN_POINT('Ctrl Pts',(-7.79073219648633,-1.37419534369438,
72.697741164032));
#61215=CARTESIAN_POINT('Ctrl Pts',(-7.83051291464963,-1.14866632904863,
72.6885062213995));
#61216=CARTESIAN_POINT('Ctrl Pts',(-7.8605330812214,-0.921197480203638,
72.679271278767));
#61217=CARTESIAN_POINT('Ctrl Pts',(-7.88062417100901,-0.692591997722056,
72.6700363361345));
#61218=CARTESIAN_POINT('Ctrl Pts',(-7.90071526079662,-0.463986515240399,
72.660801393502));
#61219=CARTESIAN_POINT('Ctrl Pts',(-7.91087714858086,-0.234244582106221,
72.6515664508695));
#61220=CARTESIAN_POINT('Ctrl Pts',(-7.9109988923078,-0.00418639519816283,
72.642331508237));
#61221=CARTESIAN_POINT('',(-7.90354147324386,0.00220337357936208,70.6423315082369));
#61222=CARTESIAN_POINT('Ctrl Pts',(-7.911,1.85740312019789E-12,72.642331508237));
#61223=CARTESIAN_POINT('Ctrl Pts',(-7.91099999999948,2.20167589666843,72.5537440725042));
#61224=CARTESIAN_POINT('Ctrl Pts',(-6.94214576672286,4.38610418338808,72.4651566367715));
#61225=CARTESIAN_POINT('Ctrl Pts',(-3.67820201488183,7.34180684107678,72.2879817653061));
#61226=CARTESIAN_POINT('Ctrl Pts',(-1.40868175871654,8.08992666571347,72.1993943295734));
#61227=CARTESIAN_POINT('Ctrl Pts',(2.97309270521321,7.65454228025233,72.0222194581079));
#61228=CARTESIAN_POINT('Ctrl Pts',(5.05102072675622,6.47444880834203,71.9336320223752));
#61229=CARTESIAN_POINT('Ctrl Pts',(7.66951518847864,2.93425195367713,71.7564571509098));
#61230=CARTESIAN_POINT('Ctrl Pts',(8.18956872247064,0.601881960099487,71.6678697151771));
#61231=CARTESIAN_POINT('Ctrl Pts',(7.3230668976137,-3.71537198232385,71.4906948437116));
#61232=CARTESIAN_POINT('Ctrl Pts',(5.94329958850262,-5.66643518936439,71.4021074079789));
#61233=CARTESIAN_POINT('Ctrl Pts',(2.16154501637973,-7.92205913232958,71.2249325365135));
#61234=CARTESIAN_POINT('Ctrl Pts',(-0.210816529298817,-8.20894963713001,
71.1363451007807));
#61235=CARTESIAN_POINT('Ctrl Pts',(-4.42123908576272,-6.91982244717931,
70.9591702293153));
#61236=CARTESIAN_POINT('Ctrl Pts',(-6.22631625634043,-5.35390358803681,
70.8705827935826));
#61237=CARTESIAN_POINT('Ctrl Pts',(-7.65317280859478,-2.31334857514619,
70.7354407413122));
#61238=CARTESIAN_POINT('Ctrl Pts',(-7.91100000000025,-1.15702837836482,
70.6888861247746));
#61239=CARTESIAN_POINT('Ctrl Pts',(-7.911,1.68642877440561E-12,70.642331508237));
#61240=CARTESIAN_POINT('',(-7.92318561732542,0.00259301387528471,68.6424391999658));
#61241=CARTESIAN_POINT('Ctrl Pts',(-7.89823755503975,0.00377023974625967,
70.6423315082369));
#61242=CARTESIAN_POINT('Ctrl Pts',(-7.90350964776257,0.958128817974856,
70.6040258452798));
#61243=CARTESIAN_POINT('Ctrl Pts',(-7.52228863784238,3.22866395001779,70.5127529924218));
#61244=CARTESIAN_POINT('Ctrl Pts',(-5.36383164184186,6.23324328561409,70.3685129496619));
#61245=CARTESIAN_POINT('Ctrl Pts',(-0.5271358810351,8.71026298249118,70.1566441900566));
#61246=CARTESIAN_POINT('Ctrl Pts',(6.62174075612686,6.61018822700539,69.8918082405504));
#61247=CARTESIAN_POINT('Ctrl Pts',(9.14004810553684,-1.99688238525928,69.5740051011428));
#61248=CARTESIAN_POINT('Ctrl Pts',(3.27357265470031,-8.75711389441476,69.256201961735));
#61249=CARTESIAN_POINT('Ctrl Pts',(-5.3858310801681,-7.53156686276361,68.945679994676));
#61250=CARTESIAN_POINT('Ctrl Pts',(-7.91004429377716,-2.43849120782205,
68.7410924074197));
#61251=CARTESIAN_POINT('Ctrl Pts',(-7.92318561732542,0.00259301387528471,
68.6424391999658));
#61252=CARTESIAN_POINT('',(-7.91099653591344,4.8067954642318E-5,64.635061427433));
#61253=CARTESIAN_POINT('Ctrl Pts',(-7.91099947655417,0.00287783939459638,
68.6494532539836));
#61254=CARTESIAN_POINT('Ctrl Pts',(-7.91094092592253,0.163829842891923,
68.6434681772393));
#61255=CARTESIAN_POINT('Ctrl Pts',(-7.90597044551911,0.324735313140411,
68.6372897700822));
#61256=CARTESIAN_POINT('Ctrl Pts',(-7.89567872179959,0.492163448253284,
68.6305561724352));
#61257=CARTESIAN_POINT('Ctrl Pts',(-7.89525230816442,0.498957240198783,
68.6302824165131));
#61258=CARTESIAN_POINT('Ctrl Pts',(-7.89454362150085,0.510019912661784,
68.6298357800155));
#61259=CARTESIAN_POINT('Ctrl Pts',(-7.89426665256145,0.514289141639768,
68.6296632071228));
#61260=CARTESIAN_POINT('Ctrl Pts',(-7.8937735402111,0.521795767861521,68.629359397902));
#61261=CARTESIAN_POINT('Ctrl Pts',(-7.89355886777265,0.525033264128524,
68.6292282476011));
#61262=CARTESIAN_POINT('Ctrl Pts',(-7.89313532577422,0.531361766581175,
68.6289716414006));
#61263=CARTESIAN_POINT('Ctrl Pts',(-7.89292663206871,0.534452784346573,
68.6288461958661));
#61264=CARTESIAN_POINT('Ctrl Pts',(-7.89250850430255,0.540592125052581,
68.6285968138893));
#61265=CARTESIAN_POINT('Ctrl Pts',(-7.89229912056636,0.543640439625881,
68.6284728806887));
#61266=CARTESIAN_POINT('Ctrl Pts',(-7.89180048221448,0.550838865707491,
68.6281799603841));
#61267=CARTESIAN_POINT('Ctrl Pts',(-7.89150972073084,0.554988859827049,
68.6280108846847));
#61268=CARTESIAN_POINT('Ctrl Pts',(-7.89048718821528,0.569420030229027,
68.6274222403401));
#61269=CARTESIAN_POINT('Ctrl Pts',(-7.88973860067586,0.57969996486082,68.6270016860655));
#61270=CARTESIAN_POINT('Ctrl Pts',(-7.8808503797559,0.698549930152759,68.6221254326864));
#61271=CARTESIAN_POINT('Ctrl Pts',(-7.87049072626236,0.806937635924736,
68.617542643153));
#61272=CARTESIAN_POINT('Ctrl Pts',(-7.85348961277053,0.952929441680667,
68.6112187738668));
#61273=CARTESIAN_POINT('Ctrl Pts',(-7.8488075570822,0.99075399211787,68.6095665836419));
#61274=CARTESIAN_POINT('Ctrl Pts',(-7.84124407009167,1.0484345092539,68.6070275917584));
#61275=CARTESIAN_POINT('Ctrl Pts',(-7.83856007311695,1.06831617814717,68.6061488957539));
#61276=CARTESIAN_POINT('Ctrl Pts',(-7.74238415395425,1.76085809806045,68.5754226798741));
#61277=CARTESIAN_POINT('Ctrl Pts',(-7.56274349562382,2.4187002454741,68.5426153192326));
#61278=CARTESIAN_POINT('Ctrl Pts',(-7.1907306448635,3.31055477745236,68.4986216735679));
#61279=CARTESIAN_POINT('Ctrl Pts',(-7.06582890206217,3.56937856281599,68.4858752252229));
#61280=CARTESIAN_POINT('Ctrl Pts',(-6.86690645513325,3.93002029751216,68.4682765040594));
#61281=CARTESIAN_POINT('Ctrl Pts',(-6.80411917675493,4.03775035884632,68.4630395629916));
#61282=CARTESIAN_POINT('Ctrl Pts',(-6.69853392034159,4.20945081593222,68.4547244392056));
#61283=CARTESIAN_POINT('Ctrl Pts',(-6.65730457636518,4.27435715415497,68.4515885722328));
#61284=CARTESIAN_POINT('Ctrl Pts',(-6.607713072547,4.34996920439848,68.4479429023018));
#61285=CARTESIAN_POINT('Ctrl Pts',(-6.60026236071995,4.3612659745087,68.447398419022));
#61286=CARTESIAN_POINT('Ctrl Pts',(-6.58881091488455,4.37853210160864,68.4465665106012));
#61287=CARTESIAN_POINT('Ctrl Pts',(-6.58483099114974,4.38451519044823,68.4462782891154));
#61288=CARTESIAN_POINT('Ctrl Pts',(-6.57788085544039,4.39493264306798,68.4457765422278));
#61289=CARTESIAN_POINT('Ctrl Pts',(-6.57491430095284,4.39936943444712,68.4455628767698));
#61290=CARTESIAN_POINT('Ctrl Pts',(-6.5687073268532,4.40863231007383,68.445116856689));
#61291=CARTESIAN_POINT('Ctrl Pts',(-6.56546607255558,4.41345783276506,68.4448845343044));
#61292=CARTESIAN_POINT('Ctrl Pts',(-6.55650168684509,4.42677212465107,68.4442436136742));
#61293=CARTESIAN_POINT('Ctrl Pts',(-6.55076738198565,4.43525337735473,68.443835445305));
#61294=CARTESIAN_POINT('Ctrl Pts',(-6.52830970369499,4.46833056536898,68.4422439493382));
#61295=CARTESIAN_POINT('Ctrl Pts',(-6.51146403846622,4.49284339028041,68.441065337577));
#61296=CARTESIAN_POINT('Ctrl Pts',(-6.24337421164096,4.87827699777393,68.4225441216345));
#61297=CARTESIAN_POINT('Ctrl Pts',(-5.96259051514637,5.21774623364937,68.4064461721521));
#61298=CARTESIAN_POINT('Ctrl Pts',(-5.27195462574641,5.92372307891987,68.3717041088256));
#61299=CARTESIAN_POINT('Ctrl Pts',(-4.84927165961036,6.27443315496323,68.3535185018485));
#61300=CARTESIAN_POINT('Ctrl Pts',(-4.31040847135696,6.63433116497635,68.3301794111759));
#61301=CARTESIAN_POINT('Ctrl Pts',(-4.22599274790826,6.68841951200458,68.3265158864006));
#61302=CARTESIAN_POINT('Ctrl Pts',(-4.01605792533861,6.81737146994626,68.3173340019242));
#61303=CARTESIAN_POINT('Ctrl Pts',(-3.88944820503646,6.89038953698008,68.3117333619421));
#61304=CARTESIAN_POINT('Ctrl Pts',(-3.7386136246717,6.97189573185971,68.3049167503924));
#61305=CARTESIAN_POINT('Ctrl Pts',(-3.71628338822199,6.98382414483279,68.3039043536631));
#61306=CARTESIAN_POINT('Ctrl Pts',(-3.68715147319466,6.99920661171946,68.302579742826));
#61307=CARTESIAN_POINT('Ctrl Pts',(-3.68040133394519,7.00275839939544,68.3022725505751));
#61308=CARTESIAN_POINT('Ctrl Pts',(-3.67005198614956,7.00818492106894,68.3018011637879));
#61309=CARTESIAN_POINT('Ctrl Pts',(-3.66645644142063,7.01006666387812,68.3016373222652));
#61310=CARTESIAN_POINT('Ctrl Pts',(-3.65937162888443,7.01376758712125,68.3013143395282));
#61311=CARTESIAN_POINT('Ctrl Pts',(-3.65588244830939,7.01558693257347,68.3011552066138));
#61312=CARTESIAN_POINT('Ctrl Pts',(-3.64798373953,7.01969802286378,68.300794814471));
#61313=CARTESIAN_POINT('Ctrl Pts',(-3.6435734089288,7.02198821628573,68.3005934788109));
#61314=CARTESIAN_POINT('Ctrl Pts',(-3.63145270505106,7.02826775356491,68.3000398699717));
#61315=CARTESIAN_POINT('Ctrl Pts',(-3.62373793315425,7.03224855617166,68.2996871812363));
#61316=CARTESIAN_POINT('Ctrl Pts',(-3.58613112125047,7.05157525755354,68.2979664460232));
#61317=CARTESIAN_POINT('Ctrl Pts',(-3.5561483611739,7.066743154887,68.2965899441491));
#61318=CARTESIAN_POINT('Ctrl Pts',(-3.392672769792,7.14813954724615,68.2890631914091));
#61319=CARTESIAN_POINT('Ctrl Pts',(-3.257429899254,7.21077490044745,68.2827587768466));
#61320=CARTESIAN_POINT('Ctrl Pts',(-3.08340777210517,7.28547508743618,68.2746137800077));
#61321=CARTESIAN_POINT('Ctrl Pts',(-3.04619000394575,7.30111478814185,68.272869916936));
#61322=CARTESIAN_POINT('Ctrl Pts',(-2.8310518646966,7.38958907319875,68.2627838571465));
#61323=CARTESIAN_POINT('Ctrl Pts',(-2.65064613646246,7.45620235622921,68.2543057865524));
#61324=CARTESIAN_POINT('Ctrl Pts',(-1.77928398254101,7.742321154766,68.2136785728615));
#61325=CARTESIAN_POINT('Ctrl Pts',(-1.06265114629847,7.87276354414527,68.1816371486636));
#61326=CARTESIAN_POINT('Ctrl Pts',(-0.270300186127443,7.90667344668757,
68.14923013952));
#61327=CARTESIAN_POINT('Ctrl Pts',(-0.20231096037545,7.90870518227394,68.1464694220199));
#61328=CARTESIAN_POINT('Ctrl Pts',(-0.116476910722555,7.91016257725009,
68.1430077333634));
#61329=CARTESIAN_POINT('Ctrl Pts',(-0.0986495706354486,7.91040499184555,
68.1422900397425));
#61330=CARTESIAN_POINT('Ctrl Pts',(-0.0702371149717731,7.91069527847364,
68.1411482101363));
#61331=CARTESIAN_POINT('Ctrl Pts',(-0.0596524929844704,7.91078217510751,
68.1407232813959));
#61332=CARTESIAN_POINT('Ctrl Pts',(-0.0397079781150411,7.91090588266893,
68.1399234132388));
#61333=CARTESIAN_POINT('Ctrl Pts',(-0.0303481306473132,7.91094732629901,
68.1395483800319));
#61334=CARTESIAN_POINT('Ctrl Pts',(-0.00939958587563894,7.9110029038809,
68.1387097647156));
#61335=CARTESIAN_POINT('Ctrl Pts',(0.00218912402489875,7.91100818518859,
68.1382463629129));
#61336=CARTESIAN_POINT('Ctrl Pts',(0.0314747774394929,7.91095718111787,
68.1370766141461));
#61337=CARTESIAN_POINT('Ctrl Pts',(0.0491716247692127,7.91086697763484,
68.1363709599773));
#61338=CARTESIAN_POINT('Ctrl Pts',(0.14487613256771,7.9100580022514,68.1325612589977));
#61339=CARTESIAN_POINT('Ctrl Pts',(0.222871048765295,7.9082447787756,68.1294798470457));
#61340=CARTESIAN_POINT('Ctrl Pts',(1.01103895469475,7.87825184796659,68.098564582206));
#61341=CARTESIAN_POINT('Ctrl Pts',(1.71434228040871,7.75564970723329,68.0732099874292));
#61342=CARTESIAN_POINT('Ctrl Pts',(2.58816134928532,7.47848717820106,68.0399228065226));
#61343=CARTESIAN_POINT('Ctrl Pts',(2.78199194130245,7.40856709915989,68.0323879451451));
#61344=CARTESIAN_POINT('Ctrl Pts',(3.14351509859778,7.26196550146311,68.0177501349705));
#61345=CARTESIAN_POINT('Ctrl Pts',(3.31168733223126,7.18683179006791,68.0106899685778));
#61346=CARTESIAN_POINT('Ctrl Pts',(3.50203226266947,7.09369176927395,68.0022628779281));
#61347=CARTESIAN_POINT('Ctrl Pts',(3.52692294393694,7.08134926455154,68.0011521103001));
#61348=CARTESIAN_POINT('Ctrl Pts',(3.55879786564547,7.06533375018621,67.999717781326));
#61349=CARTESIAN_POINT('Ctrl Pts',(3.56584253903808,7.06178095356809,67.9994000319825));
#61350=CARTESIAN_POINT('Ctrl Pts',(3.57653255425188,7.05636964953916,67.9989167069012));
#61351=CARTESIAN_POINT('Ctrl Pts',(3.58018180196981,7.05451883598822,67.9987515099943));
#61352=CARTESIAN_POINT('Ctrl Pts',(3.5875888710558,7.05075491514986,67.9984157831869));
#61353=CARTESIAN_POINT('Ctrl Pts',(3.5913466016845,7.04884163304157,67.998245244622));
#61354=CARTESIAN_POINT('Ctrl Pts',(3.59955010369944,7.04465648397866,67.9978724605965));
#61355=CARTESIAN_POINT('Ctrl Pts',(3.60399525556892,7.04238341216738,67.9976701547008));
#61356=CARTESIAN_POINT('Ctrl Pts',(3.61625134649596,7.03610149732554,67.997111500546));
#61357=CARTESIAN_POINT('Ctrl Pts',(3.62405775201769,7.03208386545488,67.9967547062395));
#61358=CARTESIAN_POINT('Ctrl Pts',(3.66252085681063,7.0122074490791,67.9949919068444));
#61359=CARTESIAN_POINT('Ctrl Pts',(3.69307986320553,6.99616133308654,67.993576206816));
#61360=CARTESIAN_POINT('Ctrl Pts',(4.14022183771854,6.7576272763702,67.97262566497));
#61361=CARTESIAN_POINT('Ctrl Pts',(4.53611858641511,6.49849833620121,67.9510108263184));
#61362=CARTESIAN_POINT('Ctrl Pts',(4.92750917515386,6.18904613259168,67.9280224711265));
#61363=CARTESIAN_POINT('Ctrl Pts',(4.94843960648932,6.17232404868004,67.926787684642));
#61364=CARTESIAN_POINT('Ctrl Pts',(4.99136920263822,6.13766731506257,67.924244324779));
#61365=CARTESIAN_POINT('Ctrl Pts',(5.01335761670537,6.11971992777455,67.9229357473975));
#61366=CARTESIAN_POINT('Ctrl Pts',(5.05855151511288,6.08242471110209,67.9202345565047));
#61367=CARTESIAN_POINT('Ctrl Pts',(5.08174372550052,6.06306147979911,67.9188419850648));
#61368=CARTESIAN_POINT('Ctrl Pts',(5.12963562442472,6.02260858448557,67.9159536586792));
#61369=CARTESIAN_POINT('Ctrl Pts',(5.15431753289776,6.00149869424389,67.9144580219927));
#61370=CARTESIAN_POINT('Ctrl Pts',(5.20686400143601,5.95599360007591,67.9112594598269));
#61371=CARTESIAN_POINT('Ctrl Pts',(5.23468870592389,5.93155347768586,67.9095569259487));
#61372=CARTESIAN_POINT('Ctrl Pts',(5.29446382939873,5.87830116751628,67.9058814038093));
#61373=CARTESIAN_POINT('Ctrl Pts',(5.32635296647424,5.84942184848483,67.9039092549819));
#61374=CARTESIAN_POINT('Ctrl Pts',(5.45704000537359,5.72911468680025,67.8957832267198));
#61375=CARTESIAN_POINT('Ctrl Pts',(5.55373361440389,5.63543121791988,67.8896666623384));
#61376=CARTESIAN_POINT('Ctrl Pts',(5.86952825081222,5.31344151356259,67.8693987595086));
#61377=CARTESIAN_POINT('Ctrl Pts',(6.0773280810714,5.07445904661621,67.8555830484987));
#61378=CARTESIAN_POINT('Ctrl Pts',(6.34452287154075,4.72713235174881,67.8372646471534));
#61379=CARTESIAN_POINT('Ctrl Pts',(6.41653884601722,4.62890718712765,67.8322613868703));
#61380=CARTESIAN_POINT('Ctrl Pts',(6.49493251040166,4.51663615140824,67.8267363506803));
#61381=CARTESIAN_POINT('Ctrl Pts',(6.503568665259,4.50419194290465,67.8261265667568));
#61382=CARTESIAN_POINT('Ctrl Pts',(6.51643972383408,4.4855312841497,67.8252160611097));
#61383=CARTESIAN_POINT('Ctrl Pts',(6.52070156495297,4.47933350808965,67.8249142944688));
#61384=CARTESIAN_POINT('Ctrl Pts',(6.52799683755423,4.46869189338354,67.8243972545249));
#61385=CARTESIAN_POINT('Ctrl Pts',(6.53103458229434,4.46425102722952,67.8241818142289));
#61386=CARTESIAN_POINT('Ctrl Pts',(6.53726325389339,4.45512539421982,67.823739769952));
#61387=CARTESIAN_POINT('Ctrl Pts',(6.54045368154829,4.4504402893004,67.8235131853382));
#61388=CARTESIAN_POINT('Ctrl Pts',(6.54898239257343,4.43788700026679,67.8229070384149));
#61389=CARTESIAN_POINT('Ctrl Pts',(6.5543115385856,4.43001260284519,67.8225278292217));
#61390=CARTESIAN_POINT('Ctrl Pts',(6.57353409713771,4.40149855097581,67.8211583215554));
#61391=CARTESIAN_POINT('Ctrl Pts',(6.58734438804481,4.38080288857381,67.8201712276785));
#61392=CARTESIAN_POINT('Ctrl Pts',(6.62019746402077,4.33106368670392,67.8178152375516));
#61393=CARTESIAN_POINT('Ctrl Pts',(6.6391471491737,4.3019591225542,67.8164499059574));
#61394=CARTESIAN_POINT('Ctrl Pts',(7.07985123176592,3.61523998330174,67.7845411723833));
#61395=CARTESIAN_POINT('Ctrl Pts',(7.40205778277287,2.89893642478682,67.7584110984444));
#61396=CARTESIAN_POINT('Ctrl Pts',(7.66813724775287,1.95531463424542,67.7250073861231));
#61397=CARTESIAN_POINT('Ctrl Pts',(7.71492825677698,1.7616646867055,67.718167678931));
#61398=CARTESIAN_POINT('Ctrl Pts',(7.78818608759195,1.39902066469634,67.7050928322685));
#61399=CARTESIAN_POINT('Ctrl Pts',(7.81657720664827,1.23053536838248,67.6989130312334));
#61400=CARTESIAN_POINT('Ctrl Pts',(7.85564106579971,0.941974937944957,67.6879655591328));
#61401=CARTESIAN_POINT('Ctrl Pts',(7.86906490094676,0.822331064325059,67.6833208780761));
#61402=CARTESIAN_POINT('Ctrl Pts',(7.88090175287269,0.689547614685502,67.6780060991761));
#61403=CARTESIAN_POINT('Ctrl Pts',(7.88201878972633,0.676659549575808,67.6774885771304));
#61404=CARTESIAN_POINT('Ctrl Pts',(7.88366781144431,0.657075307923078,67.6766995653631));
#61405=CARTESIAN_POINT('Ctrl Pts',(7.88422289231788,0.650381046159154,67.6764294043016));
#61406=CARTESIAN_POINT('Ctrl Pts',(7.88511372540038,0.639468874199588,67.6759882564822));
#61407=CARTESIAN_POINT('Ctrl Pts',(7.88545462185806,0.635251375480635,67.6758175691101));
#61408=CARTESIAN_POINT('Ctrl Pts',(7.88610414603498,0.627134513656483,67.6754887085127));
#61409=CARTESIAN_POINT('Ctrl Pts',(7.88641326574405,0.623235190050995,67.6753305641751));
#61410=CARTESIAN_POINT('Ctrl Pts',(7.88696889193816,0.616159756937043,67.6750433133565));
#61411=CARTESIAN_POINT('Ctrl Pts',(7.88721637215501,0.612983725060461,67.6749142644107));
#61412=CARTESIAN_POINT('Ctrl Pts',(7.88771278116616,0.606562999094773,67.6746531609388));
#61413=CARTESIAN_POINT('Ctrl Pts',(7.88796162657585,0.603318297128218,67.6745211014534));
#61414=CARTESIAN_POINT('Ctrl Pts',(7.88865743512677,0.594171611950547,67.6741485191722));
#61415=CARTESIAN_POINT('Ctrl Pts',(7.88909977595405,0.588269290292336,67.6739077272334));
#61416=CARTESIAN_POINT('Ctrl Pts',(7.89089870740357,0.563898496850559,67.6729119990488));
#61417=CARTESIAN_POINT('Ctrl Pts',(7.89219706296108,0.545425919393756,67.6721537153381));
#61418=CARTESIAN_POINT('Ctrl Pts',(7.91204488063971,0.248115668916403,67.6598944346911));
#61419=CARTESIAN_POINT('Ctrl Pts',(7.91586998213839,-0.0314863387240819,
67.6475929125248));
#61420=CARTESIAN_POINT('Ctrl Pts',(7.88580753096586,-0.796397804043023,
67.6129341639281));
#61421=CARTESIAN_POINT('Ctrl Pts',(7.82199184228816,-1.27932658237856,67.5900057008226));
#61422=CARTESIAN_POINT('Ctrl Pts',(7.70473192668626,-1.79523577118004,67.5659425830425));
#61423=CARTESIAN_POINT('Ctrl Pts',(7.69487217659428,-1.83703777119662,67.5639953181844));
#61424=CARTESIAN_POINT('Ctrl Pts',(7.67308528544332,-1.92615257412625,67.5598506312191));
#61425=CARTESIAN_POINT('Ctrl Pts',(7.66105982218207,-1.97343964210881,67.5576553014596));
#61426=CARTESIAN_POINT('Ctrl Pts',(7.63404754080314,-2.07568885271387,67.552918584164));
#61427=CARTESIAN_POINT('Ctrl Pts',(7.61890289850263,-2.13060668341339,67.5503809778475));
#61428=CARTESIAN_POINT('Ctrl Pts',(7.58390209904289,-2.25237942939429,67.5447708382287));
#61429=CARTESIAN_POINT('Ctrl Pts',(7.56375231647056,-2.31914538870215,67.5417061621037));
#61430=CARTESIAN_POINT('Ctrl Pts',(7.46759581862002,-2.62316551521308,67.5278090480241));
#61431=CARTESIAN_POINT('Ctrl Pts',(7.38128796122879,-2.85702431425384,67.5172879759508));
#61432=CARTESIAN_POINT('Ctrl Pts',(7.26879472569624,-3.12251170775818,67.505551997522));
#61433=CARTESIAN_POINT('Ctrl Pts',(7.25324062684075,-3.15847377668298,67.5039666414827));
#61434=CARTESIAN_POINT('Ctrl Pts',(7.23303085979246,-3.20426336802984,67.501953435656));
#61435=CARTESIAN_POINT('Ctrl Pts',(7.22862136846004,-3.21419854133358,67.5015169467027));
#61436=CARTESIAN_POINT('Ctrl Pts',(7.22151536459081,-3.23012073358205,67.5008179416756));
#61437=CARTESIAN_POINT('Ctrl Pts',(7.21883185799487,-3.23611352100214,67.5005549679327));
#61438=CARTESIAN_POINT('Ctrl Pts',(7.21372808772702,-3.24747328522235,67.5000567031605));
#61439=CARTESIAN_POINT('Ctrl Pts',(7.21130928872717,-3.25284091286537,67.4998213607178));
#61440=CARTESIAN_POINT('Ctrl Pts',(7.20581143745926,-3.26500508439965,67.499288236394));
#61441=CARTESIAN_POINT('Ctrl Pts',(7.20272875509302,-3.27179998690852,67.4989905829124));
#61442=CARTESIAN_POINT('Ctrl Pts',(7.19477524597916,-3.28926553305072,67.4982258786636));
#61443=CARTESIAN_POINT('Ctrl Pts',(7.18989028386523,-3.29992974086019,67.4977593278664));
#61444=CARTESIAN_POINT('Ctrl Pts',(7.16128061824754,-3.36202149829367,67.4950449636154));
#61445=CARTESIAN_POINT('Ctrl Pts',(7.13702762745633,-3.41320457427152,67.4928159100865));
#61446=CARTESIAN_POINT('Ctrl Pts',(6.72876861081588,-4.25140526080209,67.4564375544603));
#61447=CARTESIAN_POINT('Ctrl Pts',(6.21733959113934,-4.96943763013283,67.4280391085575));
#61448=CARTESIAN_POINT('Ctrl Pts',(5.43485615499623,-5.75326456697196,67.3892094787069));
#61449=CARTESIAN_POINT('Ctrl Pts',(5.26386324736674,-5.91011395545199,67.3808774830197));
#61450=CARTESIAN_POINT('Ctrl Pts',(5.00540980646068,-6.12706539534449,67.3680950536652));
#61451=CARTESIAN_POINT('Ctrl Pts',(4.92323511246187,-6.19328765606045,67.3640046901931));
#61452=CARTESIAN_POINT('Ctrl Pts',(4.83028269945863,-6.26517627037266,67.3593187354782));
#61453=CARTESIAN_POINT('Ctrl Pts',(4.8207850884402,-6.27248720872898,67.3588392634721));
#61454=CARTESIAN_POINT('Ctrl Pts',(4.80621128289297,-6.28365297669245,67.3581024345928));
#61455=CARTESIAN_POINT('Ctrl Pts',(4.80114694836999,-6.28752332854597,67.3578461882604));
#61456=CARTESIAN_POINT('Ctrl Pts',(4.79173898605905,-6.29469524735209,67.3573697772519));
#61457=CARTESIAN_POINT('Ctrl Pts',(4.78739663434703,-6.29799843066742,67.3571497316832));
#61458=CARTESIAN_POINT('Ctrl Pts',(4.78023993206646,-6.30343078375762,67.356786819352));
#61459=CARTESIAN_POINT('Ctrl Pts',(4.77742758846653,-6.30556255148006,67.3566441434874));
#61460=CARTESIAN_POINT('Ctrl Pts',(4.77189906032785,-6.30974737614529,67.3563635470208));
#61461=CARTESIAN_POINT('Ctrl Pts',(4.76918297458713,-6.31180056303822,67.3562256357615));
#61462=CARTESIAN_POINT('Ctrl Pts',(4.76290964748358,-6.31653643547735,67.3559069701905));
#61463=CARTESIAN_POINT('Ctrl Pts',(4.75935146644038,-6.31921786849791,67.3557261272015));
#61464=CARTESIAN_POINT('Ctrl Pts',(4.74796071436577,-6.32778682218729,67.3551468879168));
#61465=CARTESIAN_POINT('Ctrl Pts',(4.7401194953676,-6.33366277758992,67.3547476811499));
#61466=CARTESIAN_POINT('Ctrl Pts',(4.67105454749812,-6.3852177201588,67.3512275456467));
#61467=CARTESIAN_POINT('Ctrl Pts',(4.60918491314709,-6.43002096771147,67.3480469189616));
#61468=CARTESIAN_POINT('Ctrl Pts',(4.52461019155802,-6.48941837247957,67.3436738738866));
#61469=CARTESIAN_POINT('Ctrl Pts',(4.50246333112469,-6.50480377274657,67.3425264436965));
#61470=CARTESIAN_POINT('Ctrl Pts',(4.44617049445471,-6.54348512428783,67.3396050177943));
#61471=CARTESIAN_POINT('Ctrl Pts',(4.41192003930784,-6.56662707253893,67.3378230043631));
#61472=CARTESIAN_POINT('Ctrl Pts',(3.70830047627113,-7.03405072634773,67.3011485962119));
#61473=CARTESIAN_POINT('Ctrl Pts',(2.97527940937981,-7.37409894589128,67.2623019455133));
#61474=CARTESIAN_POINT('Ctrl Pts',(2.13123365980928,-7.61888637607336,67.223575162696));
#61475=CARTESIAN_POINT('Ctrl Pts',(2.05864615567481,-7.63881947014498,67.2202849282014));
#61476=CARTESIAN_POINT('Ctrl Pts',(1.76022682084135,-7.71620501250749,67.2069282617555));
#61477=CARTESIAN_POINT('Ctrl Pts',(1.53218528114985,-7.76470466796158,67.1971226213925));
#61478=CARTESIAN_POINT('Ctrl Pts',(1.26463299644139,-7.80935876665833,67.1860809016005));
#61479=CARTESIAN_POINT('Ctrl Pts',(1.22689943862315,-7.81537579279685,67.1845341286885));
#61480=CARTESIAN_POINT('Ctrl Pts',(1.17820120134105,-7.82277987557015,67.1825511676504));
#61481=CARTESIAN_POINT('Ctrl Pts',(1.1672754894649,-7.82441761317952,67.1821071392955));
#61482=CARTESIAN_POINT('Ctrl Pts',(1.14964662436026,-7.82702239075837,67.1813920691294));
#61483=CARTESIAN_POINT('Ctrl Pts',(1.14294561559971,-7.82800371655567,67.1811205808547));
#61484=CARTESIAN_POINT('Ctrl Pts',(1.13016997693378,-7.82985788414935,67.1806035916863));
#61485=CARTESIAN_POINT('Ctrl Pts',(1.12409557731458,-7.83073226435541,67.1803580428891));
#61486=CARTESIAN_POINT('Ctrl Pts',(1.11023200305203,-7.8327113945868,67.1797982254109));
#61487=CARTESIAN_POINT('Ctrl Pts',(1.10244218013375,-7.83381159662447,67.1794840989437));
#61488=CARTESIAN_POINT('Ctrl Pts',(1.07918307475748,-7.83706123551461,67.1785474482309));
#61489=CARTESIAN_POINT('Ctrl Pts',(1.06370901392733,-7.83917649088735,67.1779259907163));
#61490=CARTESIAN_POINT('Ctrl Pts',(0.955453308429607,-7.85364826518484,
67.1735899930467));
#61491=CARTESIAN_POINT('Ctrl Pts',(0.862463304555911,-7.86440333918357,
67.1699255647607));
#61492=CARTESIAN_POINT('Ctrl Pts',(0.719489402636579,-7.87837299262084,
67.1643769300196));
#61493=CARTESIAN_POINT('Ctrl Pts',(0.669630958021547,-7.88276731213581,
67.162457857266));
#61494=CARTESIAN_POINT('Ctrl Pts',(0.563476439129206,-7.89110890281257,
67.1584038618069));
#61495=CARTESIAN_POINT('Ctrl Pts',(0.507172964847898,-7.89492755762467,
67.156272727584));
#61496=CARTESIAN_POINT('Ctrl Pts',(0.399609179556531,-7.90106739068111,
67.1522350412394));
#61497=CARTESIAN_POINT('Ctrl Pts',(0.348357864035457,-7.90349291811474,
67.1503257662165));
#61498=CARTESIAN_POINT('Ctrl Pts',(-0.383391119345756,-7.9309920828275,
67.1232564823845));
#61499=CARTESIAN_POINT('Ctrl Pts',(-1.06426157097136,-7.86860256756077,
67.1007311374372));
#61500=CARTESIAN_POINT('Ctrl Pts',(-1.9080332944433,-7.67965476527742,67.069961695459));
#61501=CARTESIAN_POINT('Ctrl Pts',(-2.0858910055835,-7.6332654696956,67.063287981003));
#61502=CARTESIAN_POINT('Ctrl Pts',(-2.37897639460787,-7.54581361684718,
67.05175294653));
#61503=CARTESIAN_POINT('Ctrl Pts',(-2.49515957289562,-7.50819605923408,
67.0470359396797));
#61504=CARTESIAN_POINT('Ctrl Pts',(-2.62939890116315,-7.46127245208345,
67.0413688874191));
#61505=CARTESIAN_POINT('Ctrl Pts',(-2.64835171619549,-7.45456627576543,
67.0405636820065));
#61506=CARTESIAN_POINT('Ctrl Pts',(-2.67298954034492,-7.44574272420475,
67.0395100726196));
#61507=CARTESIAN_POINT('Ctrl Pts',(-2.67869810482986,-7.44369090308348,
67.0392654704491));
#61508=CARTESIAN_POINT('Ctrl Pts',(-2.68795649606905,-7.44035114328275,
67.0388679742034));
#61509=CARTESIAN_POINT('Ctrl Pts',(-2.69150777934348,-7.43906722202124,
67.0387153159681));
#61510=CARTESIAN_POINT('Ctrl Pts',(-2.6983244821171,-7.43659720967967,67.038421922945));
#61511=CARTESIAN_POINT('Ctrl Pts',(-2.70159003394883,-7.43541151235972,
67.0382812114222));
#61512=CARTESIAN_POINT('Ctrl Pts',(-2.70908376487301,-7.43268500654611,
67.0379579404018));
#61513=CARTESIAN_POINT('Ctrl Pts',(-2.71331140991337,-7.4311427414865,67.0377752951474));
#61514=CARTESIAN_POINT('Ctrl Pts',(-2.72455117517701,-7.42703155124166,
67.0372889958287));
#61515=CARTESIAN_POINT('Ctrl Pts',(-2.73156096208925,-7.42445630864336,
67.0369849728667));
#61516=CARTESIAN_POINT('Ctrl Pts',(-2.77828163959225,-7.40721702946232,
67.0349537707147));
#61517=CARTESIAN_POINT('Ctrl Pts',(-2.81787727934781,-7.39224461898516,
67.0332088572557));
#61518=CARTESIAN_POINT('Ctrl Pts',(-3.58184127039359,-7.09633492288994,
66.9991141327769));
#61519=CARTESIAN_POINT('Ctrl Pts',(-4.26104161191115,-6.71052669220169,
66.961774082844));
#61520=CARTESIAN_POINT('Ctrl Pts',(-5.12736918834453,-6.03308995772376,
66.9124971469583));
#61521=CARTESIAN_POINT('Ctrl Pts',(-5.36922694756987,-5.81889345126023,
66.8984474872653));
#61522=CARTESIAN_POINT('Ctrl Pts',(-5.67762462484864,-5.51011858376345,
66.880263990129));
#61523=CARTESIAN_POINT('Ctrl Pts',(-5.75617084761759,-5.42801315025172,
66.8756046517084));
#61524=CARTESIAN_POINT('Ctrl Pts',(-5.84324540770193,-5.33297642586478,
66.8704044451791));
#61525=CARTESIAN_POINT('Ctrl Pts',(-5.85353457242243,-5.32168088730323,
66.8697893870546));
#61526=CARTESIAN_POINT('Ctrl Pts',(-5.86895261327634,-5.30465600680504,
66.8688668556361));
#61527=CARTESIAN_POINT('Ctrl Pts',(-5.87410593765565,-5.29894891096811,
66.8685583595507));
#61528=CARTESIAN_POINT('Ctrl Pts',(-5.88295845250713,-5.28911632972766,
66.8680281573179));
#61529=CARTESIAN_POINT('Ctrl Pts',(-5.88666163967655,-5.28499446011311,
66.86780628445));
#61530=CARTESIAN_POINT('Ctrl Pts',(-5.89428234049941,-5.27649421561489,
66.8673495345632));
#61531=CARTESIAN_POINT('Ctrl Pts',(-5.89819931372861,-5.27211536033217,
66.8671146800983));
#61532=CARTESIAN_POINT('Ctrl Pts',(-5.90762172562808,-5.26155823189152,
66.8665495134014));
#61533=CARTESIAN_POINT('Ctrl Pts',(-5.91312236067572,-5.25537566962838,
66.8662194008167));
#61534=CARTESIAN_POINT('Ctrl Pts',(-5.93322814389547,-5.23270579463592,
66.8650121200683));
#61535=CARTESIAN_POINT('Ctrl Pts',(-5.9477741817461,-5.21616606652942,66.8641374004957));
#61536=CARTESIAN_POINT('Ctrl Pts',(-6.18469580862659,-4.94449218256167,
66.8498684916393));
#61537=CARTESIAN_POINT('Ctrl Pts',(-6.3905521852358,-4.67539698622458,66.8371780757865));
#61538=CARTESIAN_POINT('Ctrl Pts',(-6.80283504860003,-4.05812943447416,
66.8104316711447));
#61539=CARTESIAN_POINT('Ctrl Pts',(-7.00108142342318,-3.70565090907486,
66.7966332241711));
#61540=CARTESIAN_POINT('Ctrl Pts',(-7.38973486476031,-2.8710402448608,66.7649668980283));
#61541=CARTESIAN_POINT('Ctrl Pts',(-7.56145389410808,-2.38229830374398,
66.7471165660588));
#61542=CARTESIAN_POINT('Ctrl Pts',(-7.68964230681711,-1.85844878422692,
66.7256628567245));
#61543=CARTESIAN_POINT('Ctrl Pts',(-7.69491456177336,-1.83649681686598,
66.7247596143042));
#61544=CARTESIAN_POINT('Ctrl Pts',(-7.70152331106617,-1.80845198727906,
66.723599957476));
#61545=CARTESIAN_POINT('Ctrl Pts',(-7.70294670845239,-1.80237951262106,
66.7233485184985));
#61546=CARTESIAN_POINT('Ctrl Pts',(-7.70521690975511,-1.79264260766185,
66.7229447928263));
#61547=CARTESIAN_POINT('Ctrl Pts',(-7.70606828674644,-1.78897923551097,
66.7227927706842));
#61548=CARTESIAN_POINT('Ctrl Pts',(-7.70767704262457,-1.78203449675327,
66.7225043375755));
#61549=CARTESIAN_POINT('Ctrl Pts',(-7.70843493955274,-1.77875324978937,
66.7223679568046));
#61550=CARTESIAN_POINT('Ctrl Pts',(-7.71014712446851,-1.77131885283397,
66.7220587226871));
#61551=CARTESIAN_POINT('Ctrl Pts',(-7.71110015168522,-1.76716541667691,
66.7218857955945));
#61552=CARTESIAN_POINT('Ctrl Pts',(-7.71355383413197,-1.75643212067998,
66.7214384879769));
#61553=CARTESIAN_POINT('Ctrl Pts',(-7.71504942081288,-1.74985113086354,
66.721163808711));
#61554=CARTESIAN_POINT('Ctrl Pts',(-7.72414175752318,-1.7096041130958,66.7194814480187));
#61555=CARTESIAN_POINT('Ctrl Pts',(-7.73152644974159,-1.67589104674753,
66.7180614423544));
#61556=CARTESIAN_POINT('Ctrl Pts',(-7.85334861415972,-1.10179321287086,
66.6937110512951));
#61557=CARTESIAN_POINT('Ctrl Pts',(-7.91109258458655,-0.550968866681914,
66.6679033779296));
#61558=CARTESIAN_POINT('Ctrl Pts',(-7.91089005426597,0.655736935955637,
66.6120946576746));
#61559=CARTESIAN_POINT('Ctrl Pts',(-7.82958133489435,1.30770847290239,66.5825653318638));
#61560=CARTESIAN_POINT('Ctrl Pts',(-7.65798626123248,1.98522778643018,66.5540587658793));
#61561=CARTESIAN_POINT('Ctrl Pts',(-7.64675081407073,2.02807421328028,66.5522641190122));
#61562=CARTESIAN_POINT('Ctrl Pts',(-7.63207438100254,2.08218640665378,66.5500076188406));
#61563=CARTESIAN_POINT('Ctrl Pts',(-7.62896741199729,2.09354145349253,66.5495346687731));
#61564=CARTESIAN_POINT('Ctrl Pts',(-7.62401570662342,2.1114810591777,66.5487883424342));
#61565=CARTESIAN_POINT('Ctrl Pts',(-7.62218776572446,2.11807021188144,66.5485144068926));
#61566=CARTESIAN_POINT('Ctrl Pts',(-7.61879302936558,2.13024586357164,66.5480085645146));
#61567=CARTESIAN_POINT('Ctrl Pts',(-7.61722862772925,2.13583302171916,66.5477765780554));
#61568=CARTESIAN_POINT('Ctrl Pts',(-7.61374842710794,2.1482098730685,66.547262970415));
#61569=CARTESIAN_POINT('Ctrl Pts',(-7.6118296885436,2.15499873851126,66.5469814475543));
#61570=CARTESIAN_POINT('Ctrl Pts',(-7.6063264186957,2.17437131382389,66.5461786602874));
#61571=CARTESIAN_POINT('Ctrl Pts',(-7.60271973838712,2.18694873735875,66.5456581360065));
#61572=CARTESIAN_POINT('Ctrl Pts',(-7.579714404026,2.26642955223683,66.5423730000273));
#61573=CARTESIAN_POINT('Ctrl Pts',(-7.55946372008898,2.33308421321055,66.539636993923));
#61574=CARTESIAN_POINT('Ctrl Pts',(-7.49733577381843,2.52827001211136,66.5316765246582));
#61575=CARTESIAN_POINT('Ctrl Pts',(-7.45304096448978,2.6560074304315,66.5265334227416));
#61576=CARTESIAN_POINT('Ctrl Pts',(-7.33980074703697,2.95738542198601,66.5145183578765));
#61577=CARTESIAN_POINT('Ctrl Pts',(-7.26793571848666,3.12984317430211,66.5077404830479));
#61578=CARTESIAN_POINT('Ctrl Pts',(-7.01715963707973,3.67629946893593,66.486366981675));
#61579=CARTESIAN_POINT('Ctrl Pts',(-6.81494828728814,4.03883532749926,66.4723817100936));
#61580=CARTESIAN_POINT('Ctrl Pts',(-6.33613707954847,4.75808855139636,66.4426852165574));
#61581=CARTESIAN_POINT('Ctrl Pts',(-6.05558270157148,5.11036893659748,66.4269680597869));
#61582=CARTESIAN_POINT('Ctrl Pts',(-5.72661530530558,5.45808117848825,66.4080035600071));
#61583=CARTESIAN_POINT('Ctrl Pts',(-5.70643796006051,5.47917318322084,66.4068383239828));
#61584=CARTESIAN_POINT('Ctrl Pts',(-5.68173905485941,5.50470730057592,66.4054087861052));
#61585=CARTESIAN_POINT('Ctrl Pts',(-5.67732804936663,5.50925651716915,66.4051533607586));
#61586=CARTESIAN_POINT('Ctrl Pts',(-5.6700654376369,5.51672870534834,66.4047325980703));
#61587=CARTESIAN_POINT('Ctrl Pts',(-5.66721701904365,5.51965478398972,66.4045675203916));
#61588=CARTESIAN_POINT('Ctrl Pts',(-5.66209247050693,5.52491090111962,66.4042704329761));
#61589=CARTESIAN_POINT('Ctrl Pts',(-5.65981716280006,5.52724174371747,66.4041384908344));
#61590=CARTESIAN_POINT('Ctrl Pts',(-5.65496254460128,5.53220871092019,66.4038569018087));
#61591=CARTESIAN_POINT('Ctrl Pts',(-5.65238283594739,5.53484443121317,66.4037072215481));
#61592=CARTESIAN_POINT('Ctrl Pts',(-5.64538557486457,5.54198362567672,66.4033011032379));
#61593=CARTESIAN_POINT('Ctrl Pts',(-5.64096448309388,5.54648361542504,66.4030443731792));
#61594=CARTESIAN_POINT('Ctrl Pts',(-5.6189437067743,5.56884380788051,66.4017650100703));
#61595=CARTESIAN_POINT('Ctrl Pts',(-5.60126474090482,5.58662536876952,66.4007358983747));
#61596=CARTESIAN_POINT('Ctrl Pts',(-5.45079467668902,5.73653642085184,66.3919625437275));
#61597=CARTESIAN_POINT('Ctrl Pts',(-5.31344183571156,5.86398662616408,66.3838607627234));
#61598=CARTESIAN_POINT('Ctrl Pts',(-5.01696805963021,6.12011161225012,66.366435329072));
#61599=CARTESIAN_POINT('Ctrl Pts',(-4.857111369941,6.24773536539808,66.3570747924512));
#61600=CARTESIAN_POINT('Ctrl Pts',(-4.55102381369818,6.47325132871581,66.339471771655));
#61601=CARTESIAN_POINT('Ctrl Pts',(-4.40611723015186,6.57274148427782,66.3312615985282));
#61602=CARTESIAN_POINT('Ctrl Pts',(-3.80684380750867,6.95546147392947,66.2980877482013));
#61603=CARTESIAN_POINT('Ctrl Pts',(-3.32753611475839,7.19709205084432,66.2734288323677));
#61604=CARTESIAN_POINT('Ctrl Pts',(-2.63674050532818,7.46144874001913,66.2417255529085));
#61605=CARTESIAN_POINT('Ctrl Pts',(-2.44326791912679,7.5270225287051,66.2332162504104));
#61606=CARTESIAN_POINT('Ctrl Pts',(-2.22926265058221,7.59043275440089,66.2241927791821));
#61607=CARTESIAN_POINT('Ctrl Pts',(-2.21104212489442,7.59576027090131,66.2234275277023));
#61608=CARTESIAN_POINT('Ctrl Pts',(-2.18547415538237,7.60313631934836,66.2223578727714));
#61609=CARTESIAN_POINT('Ctrl Pts',(-2.17814273001472,7.60523986620684,66.2220516385642));
#61610=CARTESIAN_POINT('Ctrl Pts',(-2.16543288040593,7.6088667150911,66.2215215782053));
#61611=CARTESIAN_POINT('Ctrl Pts',(-2.16005586860403,7.61039492354056,66.2212975890711));
#61612=CARTESIAN_POINT('Ctrl Pts',(-2.14888239489348,7.61355775729978,66.2208326712037));
#61613=CARTESIAN_POINT('Ctrl Pts',(-2.1430856757498,7.61519146557947,66.2205917730263));
#61614=CARTESIAN_POINT('Ctrl Pts',(-2.12946442220123,7.6190136032769,66.2200264029842));
#61615=CARTESIAN_POINT('Ctrl Pts',(-2.12163836407965,7.62119660321936,66.2197021113083));
#61616=CARTESIAN_POINT('Ctrl Pts',(-2.096188811041,7.62825326058703,66.2186492958385));
#61617=CARTESIAN_POINT('Ctrl Pts',(-2.07855171896932,7.63307789142871,66.2179223951527));
#61618=CARTESIAN_POINT('Ctrl Pts',(-1.56914799898355,7.77052891315829,66.1970054069954));
#61619=CARTESIAN_POINT('Ctrl Pts',(-1.06570584867169,7.85542426181188,66.1785325924315));
#61620=CARTESIAN_POINT('Ctrl Pts',(0.159150779709888,7.94196668774283,66.1356988099988));
#61621=CARTESIAN_POINT('Ctrl Pts',(0.879317484782621,7.89472518917485,66.1122960571025));
#61622=CARTESIAN_POINT('Ctrl Pts',(1.62666303722671,7.74208407100822,66.0822990366393));
#61623=CARTESIAN_POINT('Ctrl Pts',(1.67015494030046,7.73281842086246,66.0805314033459));
#61624=CARTESIAN_POINT('Ctrl Pts',(1.72218932271921,7.72127340314833,66.0783920044124));
#61625=CARTESIAN_POINT('Ctrl Pts',(1.73080980152335,7.71934559787622,66.0780367618677));
#61626=CARTESIAN_POINT('Ctrl Pts',(1.74484411557498,7.71618240117225,66.0774571177898));
#61627=CARTESIAN_POINT('Ctrl Pts',(1.75025992691864,7.71495573699591,66.0772331183432));
#61628=CARTESIAN_POINT('Ctrl Pts',(1.75990338118739,7.71276084805908,66.0768337044654));
#61629=CARTESIAN_POINT('Ctrl Pts',(1.76413153199991,7.71179484608876,66.0766583911976));
#61630=CARTESIAN_POINT('Ctrl Pts',(1.77302913844042,7.70975431727278,66.076289067136));
#61631=CARTESIAN_POINT('Ctrl Pts',(1.77769841529951,7.70867902448658,66.0760950218924));
#61632=CARTESIAN_POINT('Ctrl Pts',(1.78999339410308,7.70583583564691,66.0755834629921));
#61633=CARTESIAN_POINT('Ctrl Pts',(1.79761744174322,7.70406086485422,66.0752656342688));
#61634=CARTESIAN_POINT('Ctrl Pts',(1.83170418218451,7.69607170444554,66.0738419265431));
#61635=CARTESIAN_POINT('Ctrl Pts',(1.85813716877952,7.68973251338095,66.0727305828458));
#61636=CARTESIAN_POINT('Ctrl Pts',(2.05696284217316,7.64096487874032,66.0643185323845));
#61637=CARTESIAN_POINT('Ctrl Pts',(2.22790946943088,7.59288182224325,66.0567883031286));
#61638=CARTESIAN_POINT('Ctrl Pts',(2.83381579837784,7.40023137470824,66.029327806374));
#61639=CARTESIAN_POINT('Ctrl Pts',(3.2576505771805,7.22368672858054,66.0087263139449));
#61640=CARTESIAN_POINT('Ctrl Pts',(4.12640949275155,6.76971866602819,65.9655569451721));
#61641=CARTESIAN_POINT('Ctrl Pts',(4.56397830033079,6.48278791626769,65.9432578712934));
#61642=CARTESIAN_POINT('Ctrl Pts',(4.99569295035043,6.13417094442863,65.9207741625339));
#61643=CARTESIAN_POINT('Ctrl Pts',(5.02113481454038,6.11336293919424,65.9194467149308));
#61644=CARTESIAN_POINT('Ctrl Pts',(5.05696115562571,6.08368731010578,65.917573751928));
#61645=CARTESIAN_POINT('Ctrl Pts',(5.06745336739912,6.0749505172856,65.9170247768184));
#61646=CARTESIAN_POINT('Ctrl Pts',(5.08527653798075,6.0600309817093,65.9160914343758));
#61647=CARTESIAN_POINT('Ctrl Pts',(5.0926189567968,6.05386200110572,65.9157067042587));
#61648=CARTESIAN_POINT('Ctrl Pts',(5.10732085843323,6.04146402874386,65.9149358762265));
#61649=CARTESIAN_POINT('Ctrl Pts',(5.11468020910902,6.03523490186752,65.9145497825033));
#61650=CARTESIAN_POINT('Ctrl Pts',(5.13228823731932,6.02027571606978,65.9136254353891));
#61651=CARTESIAN_POINT('Ctrl Pts',(5.14252606429163,6.01153290999979,65.9130875226745));
#61652=CARTESIAN_POINT('Ctrl Pts',(5.17735099927239,5.98163936605093,65.9112561443866));
#61653=CARTESIAN_POINT('Ctrl Pts',(5.20183043415213,5.96036349819083,65.9099660587199));
#61654=CARTESIAN_POINT('Ctrl Pts',(5.56223936653641,5.6432088938309,65.8909302454142));
#61655=CARTESIAN_POINT('Ctrl Pts',(5.87260253269959,5.31948245807064,65.8740605656661));
#61656=CARTESIAN_POINT('Ctrl Pts',(6.55426582120358,4.47564338644807,65.8343161857849));
#61657=CARTESIAN_POINT('Ctrl Pts',(6.89323408049747,3.93357050236585,65.8121469050521));
#61658=CARTESIAN_POINT('Ctrl Pts',(7.20358061721953,3.27127866018645,65.783826096306));
#61659=CARTESIAN_POINT('Ctrl Pts',(7.24211326519641,3.18506393607554,65.7801131023004));
#61660=CARTESIAN_POINT('Ctrl Pts',(7.28394685596344,3.08677709767737,65.7758312406306));
#61661=CARTESIAN_POINT('Ctrl Pts',(7.28877451360614,3.07536026158793,65.7753331258333));
#61662=CARTESIAN_POINT('Ctrl Pts',(7.2957785875294,3.05868732704689,65.7746045508147));
#61663=CARTESIAN_POINT('Ctrl Pts',(7.29797621400613,3.05344011607293,65.7743750937799));
#61664=CARTESIAN_POINT('Ctrl Pts',(7.30185194375157,3.04415805890376,65.7739688988962));
#61665=CARTESIAN_POINT('Ctrl Pts',(7.30353236902722,3.04012418011427,65.7737922721432));
#61666=CARTESIAN_POINT('Ctrl Pts',(7.30700637991229,3.03176527566995,65.7734260619754));
#61667=CARTESIAN_POINT('Ctrl Pts',(7.3087994695217,3.02744004680772,65.773236454759));
#61668=CARTESIAN_POINT('Ctrl Pts',(7.31339302995311,3.01633175266325,65.7727491929033));
#61669=CARTESIAN_POINT('Ctrl Pts',(7.31618790003867,3.00954638832292,65.7724512661382));
#61670=CARTESIAN_POINT('Ctrl Pts',(7.32763941219574,2.98163427042889,65.7712245006141));
#61671=CARTESIAN_POINT('Ctrl Pts',(7.33621395232553,2.96047413537408,65.7702916187018));
#61672=CARTESIAN_POINT('Ctrl Pts',(7.3905962671344,2.82458304382312,65.7642806379654));
#61673=CARTESIAN_POINT('Ctrl Pts',(7.43379768561378,2.70884272530146,65.7590603389057));
#61674=CARTESIAN_POINT('Ctrl Pts',(7.52030217422378,2.45941321864593,65.7476522567079));
#61675=CARTESIAN_POINT('Ctrl Pts',(7.56278976212658,2.3254819431823,65.7414353092094));
#61676=CARTESIAN_POINT('Ctrl Pts',(7.68937808901607,1.88618192752425,65.7209018695115));
#61677=CARTESIAN_POINT('Ctrl Pts',(7.75871444421833,1.57688309699188,65.7062362304532));
#61678=CARTESIAN_POINT('Ctrl Pts',(7.90835065262444,0.65258773733756,65.6631082614545));
#61679=CARTESIAN_POINT('Ctrl Pts',(7.93518243310435,0.0313038399315663,
65.6352078284755));
#61680=CARTESIAN_POINT('Ctrl Pts',(7.88471613501784,-0.647175869606253,
65.6072831967041));
#61681=CARTESIAN_POINT('Ctrl Pts',(7.87953331836288,-0.707488542760406,
65.6048207161513));
#61682=CARTESIAN_POINT('Ctrl Pts',(7.87248723459751,-0.779750892207637,
65.6018937001239));
#61683=CARTESIAN_POINT('Ctrl Pts',(7.87128826838524,-0.791762407855548,
65.601407942929));
#61684=CARTESIAN_POINT('Ctrl Pts',(7.86928982409767,-0.811330017020597,
65.6006178645159));
#61685=CARTESIAN_POINT('Ctrl Pts',(7.86850694620996,-0.818887764005264,
65.6003130115811));
#61686=CARTESIAN_POINT('Ctrl Pts',(7.86709215416323,-0.832356520317786,
65.5997702710113));
#61687=CARTESIAN_POINT('Ctrl Pts',(7.86646446399809,-0.838267961854198,
65.5995322480565));
#61688=CARTESIAN_POINT('Ctrl Pts',(7.86514231737033,-0.850587368597784,
65.5990365962943));
#61689=CARTESIAN_POINT('Ctrl Pts',(7.86444669143068,-0.85699520536097,65.5987790052243));
#61690=CARTESIAN_POINT('Ctrl Pts',(7.86260600020357,-0.87375995679363,65.5981056411469));
#61691=CARTESIAN_POINT('Ctrl Pts',(7.86144830055577,-0.884115487543032,
65.5976902743716));
#61692=CARTESIAN_POINT('Ctrl Pts',(7.85887777857409,-0.906704312140545,
65.5967854541167));
#61693=CARTESIAN_POINT('Ctrl Pts',(7.85745684398556,-0.918936665346535,
65.5962962622859));
#61694=CARTESIAN_POINT('Ctrl Pts',(7.85322258853049,-0.95465999839684,65.5948699130692));
#61695=CARTESIAN_POINT('Ctrl Pts',(7.85033243329407,-0.978141828640588,
65.5939352272318));
#61696=CARTESIAN_POINT('Ctrl Pts',(7.7744338475608,-1.57278594691258,65.5703375843208));
#61697=CARTESIAN_POINT('Ctrl Pts',(7.63939349205951,-2.13430009453654,65.5499193941914));
#61698=CARTESIAN_POINT('Ctrl Pts',(7.21837545121001,-3.30546001013523,65.507372771856));
#61699=CARTESIAN_POINT('Ctrl Pts',(6.91334759674717,-3.90338366838295,65.4856411473921));
#61700=CARTESIAN_POINT('Ctrl Pts',(6.50150692742712,-4.50757851728124,65.4572120729399));
#61701=CARTESIAN_POINT('Ctrl Pts',(6.46555920906736,-4.55899113076703,65.4547351512214));
#61702=CARTESIAN_POINT('Ctrl Pts',(6.42427971641129,-4.61655898623468,65.4518895875639));
#61703=CARTESIAN_POINT('Ctrl Pts',(6.41954453482423,-4.62314121702876,65.4515631537998));
#61704=CARTESIAN_POINT('Ctrl Pts',(6.41237754463379,-4.63307158900949,65.4510690302293));
#61705=CARTESIAN_POINT('Ctrl Pts',(6.40995320392804,-4.63642513657832,65.4509018777105));
#61706=CARTESIAN_POINT('Ctrl Pts',(6.40573740872022,-4.64224714477417,65.4506111921949));
#61707=CARTESIAN_POINT('Ctrl Pts',(6.40394716042954,-4.64471646809879,65.450487746564));
#61708=CARTESIAN_POINT('Ctrl Pts',(6.40019871686216,-4.64988048023665,65.4502292632825));
#61709=CARTESIAN_POINT('Ctrl Pts',(6.3982402551412,-4.65257495729345,65.4500942064135));
#61710=CARTESIAN_POINT('Ctrl Pts',(6.3935827714855,-4.65897428140715,65.4497730100365));
#61711=CARTESIAN_POINT('Ctrl Pts',(6.39088223283296,-4.66267801767797,65.4495867610095));
#61712=CARTESIAN_POINT('Ctrl Pts',(6.38186200845938,-4.6750265213773,65.4489646315706));
#61713=CARTESIAN_POINT('Ctrl Pts',(6.375528013643,-4.68366077077349,65.4485277264112));
#61714=CARTESIAN_POINT('Ctrl Pts',(6.18880852938391,-4.93710873807688,65.4356475814128));
#61715=CARTESIAN_POINT('Ctrl Pts',(5.99448912529731,-5.17131124723761,65.4222327115985));
#61716=CARTESIAN_POINT('Ctrl Pts',(5.74316731692485,-5.44096685953509,65.4054992728906));
#61717=CARTESIAN_POINT('Ctrl Pts',(5.69856228120195,-5.48766607509887,65.4025505532815));
#61718=CARTESIAN_POINT('Ctrl Pts',(5.5677386741146,-5.62131658754398,65.3939752088805));
#61719=CARTESIAN_POINT('Ctrl Pts',(5.48006713143088,-5.70681853381715,65.3883182276661));
#61720=CARTESIAN_POINT('Ctrl Pts',(5.33823003196128,-5.83886212341088,65.3793474398773));
#61721=CARTESIAN_POINT('Ctrl Pts',(5.28535748264227,-5.88676541437934,65.3760413591992));
#61722=CARTESIAN_POINT('Ctrl Pts',(5.21068701387108,-5.95260089724688,65.3714310969771));
#61723=CARTESIAN_POINT('Ctrl Pts',(5.18943013167645,-5.97114155832867,65.3701251721931));
#61724=CARTESIAN_POINT('Ctrl Pts',(5.14793064829591,-6.00694921883984,65.3675887389204));
#61725=CARTESIAN_POINT('Ctrl Pts',(5.1276991866357,-6.02422857571521,65.3663581711255));
#61726=CARTESIAN_POINT('Ctrl Pts',(5.08815054670785,-6.05766284306286,65.3639646379976));
#61727=CARTESIAN_POINT('Ctrl Pts',(5.06884263369266,-6.07382823804599,65.3628015940133));
#61728=CARTESIAN_POINT('Ctrl Pts',(4.77458884005739,-6.31780955657994,65.3451624517865));
#61729=CARTESIAN_POINT('Ctrl Pts',(4.484588708145,-6.5268609883565,65.3289373829094));
#61730=CARTESIAN_POINT('Ctrl Pts',(3.95414389393391,-6.85713921173142,65.3017365025117));
#61731=CARTESIAN_POINT('Ctrl Pts',(3.71980025115205,-6.9870392305715,65.2904739226519));
#61732=CARTESIAN_POINT('Ctrl Pts',(3.46113863895642,-7.11370855157737,65.2788343496852));
#61733=CARTESIAN_POINT('Ctrl Pts',(3.44294092627836,-7.12253380624951,65.2780195049568));
#61734=CARTESIAN_POINT('Ctrl Pts',(3.41767737679023,-7.13466629936368,65.2768938229362));
#61735=CARTESIAN_POINT('Ctrl Pts',(3.41064027064769,-7.13803297833426,65.2765808616145));
#61736=CARTESIAN_POINT('Ctrl Pts',(3.39853738267738,-7.14380123519055,65.2760436288176));
#61737=CARTESIAN_POINT('Ctrl Pts',(3.39347401288705,-7.14620784426314,65.2758191778843));
#61738=CARTESIAN_POINT('Ctrl Pts',(3.38315054362597,-7.15110112158841,65.2753621774131));
#61739=CARTESIAN_POINT('Ctrl Pts',(3.37789024985902,-7.15358737362752,65.2751296427917));
#61740=CARTESIAN_POINT('Ctrl Pts',(3.36574600419395,-7.15931090984744,65.2745935550495));
#61741=CARTESIAN_POINT('Ctrl Pts',(3.35886011099411,-7.16254407482488,65.2742901486567));
#61742=CARTESIAN_POINT('Ctrl Pts',(3.34438858056131,-7.16931350052565,65.2736536757385));
#61743=CARTESIAN_POINT('Ctrl Pts',(3.33680197100886,-7.1728476669622,65.2733206838029));
#61744=CARTESIAN_POINT('Ctrl Pts',(3.31667107998892,-7.18218664483193,65.2724388800504));
#61745=CARTESIAN_POINT('Ctrl Pts',(3.3041171434833,-7.18797064258925,65.2718908058595));
#61746=CARTESIAN_POINT('Ctrl Pts',(3.26629029106942,-7.20527863805732,65.2702448533724));
#61747=CARTESIAN_POINT('Ctrl Pts',(3.24097165838254,-7.21670251898742,65.2691505075324));
#61748=CARTESIAN_POINT('Ctrl Pts',(3.15086644352229,-7.25678857354164,65.2652815453654));
#61749=CARTESIAN_POINT('Ctrl Pts',(3.08575481346521,-7.28471394799858,65.2625326866272));
#61750=CARTESIAN_POINT('Ctrl Pts',(2.72633876021872,-7.43317825486152,65.2476041381684));
#61751=CARTESIAN_POINT('Ctrl Pts',(2.42533573231901,-7.53676521957365,65.2360135070626));
#61752=CARTESIAN_POINT('Ctrl Pts',(1.36251957969407,-7.83222711536702,65.1970980564306));
#61753=CARTESIAN_POINT('Ctrl Pts',(0.579198370295354,-7.92870708804797,
65.1722442929536));
#61754=CARTESIAN_POINT('Ctrl Pts',(-0.273564968773696,-7.90656299248594,
65.139186186722));
#61755=CARTESIAN_POINT('Ctrl Pts',(-0.341743006582916,-7.90390962495232,
65.1364986228612));
#61756=CARTESIAN_POINT('Ctrl Pts',(-0.419168056529104,-7.89989276568388,
65.1333874507478));
#61757=CARTESIAN_POINT('Ctrl Pts',(-0.428458909871383,-7.89939431413478,
65.1330131483934));
#61758=CARTESIAN_POINT('Ctrl Pts',(-0.442072842881279,-7.8986398421575,
65.1324632353069));
#61759=CARTESIAN_POINT('Ctrl Pts',(-0.446396652284255,-7.89839665901994,
65.1322883681955));
#61760=CARTESIAN_POINT('Ctrl Pts',(-0.454100171094432,-7.89795704569675,
65.1319764379677));
#61761=CARTESIAN_POINT('Ctrl Pts',(-0.457479961458077,-7.8977619960249,
65.1318394540992));
#61762=CARTESIAN_POINT('Ctrl Pts',(-0.464539172974304,-7.89735005821463,
65.1315530728924));
#61763=CARTESIAN_POINT('Ctrl Pts',(-0.468218568974029,-7.89713276808683,
65.1314036526732));
#61764=CARTESIAN_POINT('Ctrl Pts',(-0.477788768900233,-7.89656087924876,
65.1310146118375));
#61765=CARTESIAN_POINT('Ctrl Pts',(-0.483679321172297,-7.89620226066201,
65.1307747639001));
#61766=CARTESIAN_POINT('Ctrl Pts',(-0.508920606365858,-7.89463721289469,
65.1297453521007));
#61767=CARTESIAN_POINT('Ctrl Pts',(-0.528267126489259,-7.89336624878868,
65.1289521834084));
#61768=CARTESIAN_POINT('Ctrl Pts',(-0.663818456408564,-7.88396066731016,
65.1233666373127));
#61769=CARTESIAN_POINT('Ctrl Pts',(-0.779831116300489,-7.87333168455961,
65.1184409503652));
#61770=CARTESIAN_POINT('Ctrl Pts',(-1.17246918751565,-7.82859567815469,
65.1013755944532));
#61771=CARTESIAN_POINT('Ctrl Pts',(-1.44750189101963,-7.78243633116659,
65.0887596766703));
#61772=CARTESIAN_POINT('Ctrl Pts',(-1.89984988559776,-7.6817073234516,65.0674905476054));
#61773=CARTESIAN_POINT('Ctrl Pts',(-2.07872891234743,-7.63524344915277,
65.0589395686552));
#61774=CARTESIAN_POINT('Ctrl Pts',(-2.47380800169171,-7.51770718545703,
65.0399191989619));
#61775=CARTESIAN_POINT('Ctrl Pts',(-2.68890722311049,-7.44348242729305,
65.029473221703));
#61776=CARTESIAN_POINT('Ctrl Pts',(-3.03351346715425,-7.30767767287447,
65.0127617540415));
#61777=CARTESIAN_POINT('Ctrl Pts',(-3.16507080476889,-7.25166780482523,
65.0063868193198));
#61778=CARTESIAN_POINT('Ctrl Pts',(-3.57928239931427,-7.06189842947632,
64.9863800906994));
#61779=CARTESIAN_POINT('Ctrl Pts',(-3.8555697467116,-6.91493188095261,64.9731473074963));
#61780=CARTESIAN_POINT('Ctrl Pts',(-4.14090003389964,-6.74072213798318,
64.9596202169897));
#61781=CARTESIAN_POINT('Ctrl Pts',(-4.15929868149795,-6.72938500309702,
64.9587485252625));
#61782=CARTESIAN_POINT('Ctrl Pts',(-4.18462115509304,-6.71363792322352,
64.9575495294879));
#61783=CARTESIAN_POINT('Ctrl Pts',(-4.19158483518406,-6.70929243257123,
64.9572198824613));
#61784=CARTESIAN_POINT('Ctrl Pts',(-4.20350583180728,-6.70182766314031,
64.9566556942475));
#61785=CARTESIAN_POINT('Ctrl Pts',(-4.2084664642725,-6.69871370665778,64.956420959278));
#61786=CARTESIAN_POINT('Ctrl Pts',(-4.21853670316011,-6.69237667650353,
64.9559445161954));
#61787=CARTESIAN_POINT('Ctrl Pts',(-4.22364608556527,-6.68915325285777,
64.95570282108));
#61788=CARTESIAN_POINT('Ctrl Pts',(-4.23537692500638,-6.68173366383357,
64.9551479934072));
#61789=CARTESIAN_POINT('Ctrl Pts',(-4.24199585220415,-6.67753349984981,
64.9548350073082));
#61790=CARTESIAN_POINT('Ctrl Pts',(-4.25586587566238,-6.66870307223613,
64.9541792767325));
#61791=CARTESIAN_POINT('Ctrl Pts',(-4.26311568601348,-6.66407080286021,
64.9538366061956));
#61792=CARTESIAN_POINT('Ctrl Pts',(-4.28225469898228,-6.65179790917247,
64.9529321770542));
#61793=CARTESIAN_POINT('Ctrl Pts',(-4.2941310323446,-6.64413722097158,64.9523711540824));
#61794=CARTESIAN_POINT('Ctrl Pts',(-4.32967017335749,-6.62107802603943,
64.950692902182));
#61795=CARTESIAN_POINT('Ctrl Pts',(-4.35327125492157,-6.60558456448919,
64.9495791607741));
#61796=CARTESIAN_POINT('Ctrl Pts',(-4.43635414165144,-6.5504042609527,64.9456607916105));
#61797=CARTESIAN_POINT('Ctrl Pts',(-4.49538100309093,-6.51003717433462,
64.9428812497779));
#61798=CARTESIAN_POINT('Ctrl Pts',(-4.8223070819249,-6.27989305886382,64.9274989605675));
#61799=CARTESIAN_POINT('Ctrl Pts',(-5.07874741751383,-6.07437642427691,
64.9154991433005));
#61800=CARTESIAN_POINT('Ctrl Pts',(-5.89656955768259,-5.33085736647997,
64.8762930818178));
#61801=CARTESIAN_POINT('Ctrl Pts',(-6.39122418823901,-4.72646437585342,
64.8512485770037));
#61802=CARTESIAN_POINT('Ctrl Pts',(-6.81167331635576,-4.02328720890917,
64.8190194679026));
#61803=CARTESIAN_POINT('Ctrl Pts',(-6.83322482880398,-3.98657392411261,
64.8173277527226));
#61804=CARTESIAN_POINT('Ctrl Pts',(-6.85821413568586,-3.94320629057885,
64.8153168083088));
#61805=CARTESIAN_POINT('Ctrl Pts',(-6.86194045197115,-3.93671820351944,
64.815015628031));
#61806=CARTESIAN_POINT('Ctrl Pts',(-6.86789534632451,-3.92631567775764,
64.814532194738));
#61807=CARTESIAN_POINT('Ctrl Pts',(-6.87012980160444,-3.92240459391802,
64.8143503134739));
#61808=CARTESIAN_POINT('Ctrl Pts',(-6.87408205203401,-3.91547302584095,
64.8140277465171));
#61809=CARTESIAN_POINT('Ctrl Pts',(-6.87580120185589,-3.91245331048732,
64.8138871470073));
#61810=CARTESIAN_POINT('Ctrl Pts',(-6.87938353052511,-3.90615123685815,
64.813593562851));
#61811=CARTESIAN_POINT('Ctrl Pts',(-6.88124634581206,-3.90286868513731,
64.8134405560029));
#61812=CARTESIAN_POINT('Ctrl Pts',(-6.88609266291181,-3.89431451337888,
64.8130416007666));
#61813=CARTESIAN_POINT('Ctrl Pts',(-6.88907245585836,-3.88904080576171,
64.8127954179079));
#61814=CARTESIAN_POINT('Ctrl Pts',(-6.901877448275,-3.86631733285549,64.8117337132005));
#61815=CARTESIAN_POINT('Ctrl Pts',(-6.91164235389926,-3.84883384778569,
64.8109144350583));
#61816=CARTESIAN_POINT('Ctrl Pts',(-6.98010767235342,-3.72514995203476,
64.8051027533573));
#61817=CARTESIAN_POINT('Ctrl Pts',(-7.0364217919288,-3.61765270278702,64.7999695735854));
#61818=CARTESIAN_POINT('Ctrl Pts',(-7.16446578323156,-3.35892192035464,
64.7874999820108));
#61819=CARTESIAN_POINT('Ctrl Pts',(-7.23391204766382,-3.20662414353978,
64.7800697395181));
#61820=CARTESIAN_POINT('Ctrl Pts',(-7.64464833544654,-2.22447909682973,
64.7320922283271));
#61821=CARTESIAN_POINT('Ctrl Pts',(-7.84758214064166,-1.34354495997937,
64.6897923431192));
#61822=CARTESIAN_POINT('Ctrl Pts',(-7.90045102068861,-0.410105426828256,
64.6514788716379));
#61823=CARTESIAN_POINT('Ctrl Pts',(-7.90229716424221,-0.372843625238695,
64.6499581785528));
#61824=CARTESIAN_POINT('Ctrl Pts',(-7.90500619706137,-0.309036130821233,
64.6473689126054));
#61825=CARTESIAN_POINT('Ctrl Pts',(-7.90599910803566,-0.28249677385192,
64.6462963373018));
#61826=CARTESIAN_POINT('Ctrl Pts',(-7.90718029755614,-0.246007624109232,
64.6448275929709));
#61827=CARTESIAN_POINT('Ctrl Pts',(-7.90748346825854,-0.2360618760573,64.6444278684035));
#61828=CARTESIAN_POINT('Ctrl Pts',(-7.90793582102612,-0.220242085950251,
64.6437930241016));
#61829=CARTESIAN_POINT('Ctrl Pts',(-7.90809722415668,-0.214368419699298,
64.643557525978));
#61830=CARTESIAN_POINT('Ctrl Pts',(-7.90840775836396,-0.202589778265901,
64.6430856956073));
#61831=CARTESIAN_POINT('Ctrl Pts',(-7.90855682021521,-0.196684804787421,
64.6428493656472));
#61832=CARTESIAN_POINT('Ctrl Pts',(-7.90884298812438,-0.184821821521475,
64.6423750081454));
#61833=CARTESIAN_POINT('Ctrl Pts',(-7.90897997552525,-0.17886381258873,
64.6421369844309));
#61834=CARTESIAN_POINT('Ctrl Pts',(-7.9092775596066,-0.165251617995553,
64.6415936647936));
#61835=CARTESIAN_POINT('Ctrl Pts',(-7.90943377820633,-0.157597337334214,
64.6412885046623));
#61836=CARTESIAN_POINT('Ctrl Pts',(-7.90997103444742,-0.12925673130627,
64.6401599298155));
#61837=CARTESIAN_POINT('Ctrl Pts',(-7.91028203238736,-0.108569078050581,
64.6393386854051));
#61838=CARTESIAN_POINT('Ctrl Pts',(-7.91083749197123,-0.0585696182767007,
64.6373599847449));
#61839=CARTESIAN_POINT('Ctrl Pts',(-7.91100020597333,-0.0292571747042206,
64.6362050642762));
#61840=CARTESIAN_POINT('Ctrl Pts',(-7.91099999980433,5.56412939415241E-5,
64.6350551235107));
#61841=CARTESIAN_POINT('',(-7.91099918378876,-0.00359361845736577,60.642331508237));
#61842=CARTESIAN_POINT('Ctrl Pts',(-7.91099999985539,4.78326250410999E-5,
64.6350554298447));
#61843=CARTESIAN_POINT('Ctrl Pts',(-7.91099386948979,1.01394414802377,64.5952802815208));
#61844=CARTESIAN_POINT('Ctrl Pts',(-7.7161184369875,2.01823940527957,64.5634430191512));
#61845=CARTESIAN_POINT('Ctrl Pts',(-7.25761683982437,3.15530437559156,64.5189314313957));
#61846=CARTESIAN_POINT('Ctrl Pts',(-7.17038029084581,3.34881812174155,64.5109668091539));
#61847=CARTESIAN_POINT('Ctrl Pts',(-7.06342309757213,3.56268177758636,64.5014792860627));
#61848=CARTESIAN_POINT('Ctrl Pts',(-7.05124543716367,3.5867234429763,64.5004027211427));
#61849=CARTESIAN_POINT('Ctrl Pts',(-7.03591889424989,3.61660203525023,64.4990517188644));
#61850=CARTESIAN_POINT('Ctrl Pts',(-7.03288507577004,3.62249809915078,64.4987844836784));
#61851=CARTESIAN_POINT('Ctrl Pts',(-7.02807848656479,3.63181065060439,64.4983613815403));
#61852=CARTESIAN_POINT('Ctrl Pts',(-7.02631062344652,3.63522968158852,64.4982058259261));
#61853=CARTESIAN_POINT('Ctrl Pts',(-7.02315352268604,3.64132457864591,64.4979281371314));
#61854=CARTESIAN_POINT('Ctrl Pts',(-7.02176524848077,3.64400094476363,64.4978060655629));
#61855=CARTESIAN_POINT('Ctrl Pts',(-7.01878532974652,3.64973771583157,64.4975441173107));
#61856=CARTESIAN_POINT('Ctrl Pts',(-7.01719321307264,3.65279787420183,64.4974042102566));
#61857=CARTESIAN_POINT('Ctrl Pts',(-7.01262510613737,3.66156408333416,64.4970029207348));
#61858=CARTESIAN_POINT('Ctrl Pts',(-7.0096441787391,3.66726749803442,64.4967412172963));
#61859=CARTESIAN_POINT('Ctrl Pts',(-6.99580720391803,3.69366330284882,64.4955271808382));
#61860=CARTESIAN_POINT('Ctrl Pts',(-6.98486657172159,3.71431097007132,64.4945693983454));
#61861=CARTESIAN_POINT('Ctrl Pts',(-6.97076287027303,3.7406454445837,64.4933377328772));
#61862=CARTESIAN_POINT('Ctrl Pts',(-6.96768394019634,3.74637742956143,64.493069034115));
#61863=CARTESIAN_POINT('Ctrl Pts',(-6.95902591614555,3.76244831430947,64.4923139709411));
#61864=CARTESIAN_POINT('Ctrl Pts',(-6.95343087665174,3.77277855967851,64.491826637168));
#61865=CARTESIAN_POINT('Ctrl Pts',(-6.6382015856957,4.3517102018188,64.4644055592839));
#61866=CARTESIAN_POINT('Ctrl Pts',(-6.259974352022,4.88014042433532,64.4336344177656));
#61867=CARTESIAN_POINT('Ctrl Pts',(-5.60018827487086,5.5972097939344,64.3888481638421));
#61868=CARTESIAN_POINT('Ctrl Pts',(-5.36403780128666,5.82391548487136,64.3740785313534));
#61869=CARTESIAN_POINT('Ctrl Pts',(-4.9814295865403,6.14814703894353,64.3523077657414));
#61870=CARTESIAN_POINT('Ctrl Pts',(-4.8446437454756,6.25649941217763,64.3448995196463));
#61871=CARTESIAN_POINT('Ctrl Pts',(-4.65535150571118,6.39651017091543,64.3351476978341));
#61872=CARTESIAN_POINT('Ctrl Pts',(-4.60590376953269,6.43220729606451,64.3326442639539));
#61873=CARTESIAN_POINT('Ctrl Pts',(-4.53574987897492,6.4816286910602,64.3291534043964));
#61874=CARTESIAN_POINT('Ctrl Pts',(-4.51538499854268,6.4958321855982,64.3281471566339));
#61875=CARTESIAN_POINT('Ctrl Pts',(-4.48448030128063,6.51717112009017,64.3266307881946));
#61876=CARTESIAN_POINT('Ctrl Pts',(-4.47398967261001,6.52437731837421,64.326117901354));
#61877=CARTESIAN_POINT('Ctrl Pts',(-4.45695009307533,6.53602168387213,64.3252878150125));
#61878=CARTESIAN_POINT('Ctrl Pts',(-4.45041181553591,6.54047538462121,64.3249700101159));
#61879=CARTESIAN_POINT('Ctrl Pts',(-4.43784598216374,6.54900732948644,64.3243605808945));
#61880=CARTESIAN_POINT('Ctrl Pts',(-4.43181945982286,6.55308707701844,64.3240688982204));
#61881=CARTESIAN_POINT('Ctrl Pts',(-4.42100270444228,6.56038790077899,64.3235464365189));
#61882=CARTESIAN_POINT('Ctrl Pts',(-4.41621456346552,6.5636120582339,64.3233155379782));
#61883=CARTESIAN_POINT('Ctrl Pts',(-4.40666604234861,6.57002650148381,64.3228558233716));
#61884=CARTESIAN_POINT('Ctrl Pts',(-4.40190571616421,6.57321686126165,64.3226270045019));
#61885=CARTESIAN_POINT('Ctrl Pts',(-4.3888457062231,6.5819491006779,64.3220002424179));
#61886=CARTESIAN_POINT('Ctrl Pts',(-4.38053898250101,6.58748046074524,64.3216027061369));
#61887=CARTESIAN_POINT('Ctrl Pts',(-4.34865491658069,6.60862474867806,64.3200810652362));
#61888=CARTESIAN_POINT('Ctrl Pts',(-4.32500425530015,6.62412702668795,64.3189612272794));
#61889=CARTESIAN_POINT('Ctrl Pts',(-3.95800998285834,6.86187704030903,64.3017196204905));
#61890=CARTESIAN_POINT('Ctrl Pts',(-3.59800988637363,7.05730621796375,64.2866786028816));
#61891=CARTESIAN_POINT('Ctrl Pts',(-3.0306461341968,7.31055131590422,64.2647779435393));
#61892=CARTESIAN_POINT('Ctrl Pts',(-2.83340924322063,7.38923347269942,64.2574628252671));
#61893=CARTESIAN_POINT('Ctrl Pts',(-2.2403075253277,7.59859069643404,64.2359111276538));
#61894=CARTESIAN_POINT('Ctrl Pts',(-1.83704719089428,7.70602235390341,64.221852051876));
#61895=CARTESIAN_POINT('Ctrl Pts',(-1.21199585755554,7.82066944486034,64.1987407775701));
#61896=CARTESIAN_POINT('Ctrl Pts',(-0.995232906795697,7.85119750111191,
64.1904832831767));
#61897=CARTESIAN_POINT('Ctrl Pts',(-0.767004874880943,7.87373708962187,
64.1812821128865));
#61898=CARTESIAN_POINT('Ctrl Pts',(-0.756507140700339,7.87475264237463,
64.1808577688203));
#61899=CARTESIAN_POINT('Ctrl Pts',(-0.741472438960316,7.8761767611683,64.1802483854263));
#61900=CARTESIAN_POINT('Ctrl Pts',(-0.736937061144705,7.87660240958293,
64.1800643442921));
#61901=CARTESIAN_POINT('Ctrl Pts',(-0.729089730281855,7.87733205004603,
64.1797455330635));
#61902=CARTESIAN_POINT('Ctrl Pts',(-0.725777944227535,7.87763787166503,
64.1796108707708));
#61903=CARTESIAN_POINT('Ctrl Pts',(-0.719422389391531,7.87822072342102,
64.1793522212239));
#61904=CARTESIAN_POINT('Ctrl Pts',(-0.716378661517996,7.87849807733375,
64.1792282535316));
#61905=CARTESIAN_POINT('Ctrl Pts',(-0.709188186183988,7.87914909439321,
64.1789351613605));
#61906=CARTESIAN_POINT('Ctrl Pts',(-0.705041314906496,7.87952124682976,
64.1787659480275));
#61907=CARTESIAN_POINT('Ctrl Pts',(-0.690608202694697,7.88080503174254,
64.178176375359));
#61908=CARTESIAN_POINT('Ctrl Pts',(-0.680320511570052,7.88169979366968,
64.1777550262929));
#61909=CARTESIAN_POINT('Ctrl Pts',(-0.560797236933118,7.89185945884062,
64.1728470945995));
#61910=CARTESIAN_POINT('Ctrl Pts',(-0.451386860279121,7.89887251617531,
64.168231657301));
#61911=CARTESIAN_POINT('Ctrl Pts',(-0.335740740402612,7.90387479707518,
64.1632496920286));
#61912=CARTESIAN_POINT('Ctrl Pts',(-0.329610007988939,7.90413283636504,
64.1629852767757));
#61913=CARTESIAN_POINT('Ctrl Pts',(-0.285202427143589,7.90595017217556,
64.1610678083962));
#61914=CARTESIAN_POINT('Ctrl Pts',(-0.246915485981296,7.90723853279353,
64.1594028240778));
#61915=CARTESIAN_POINT('Ctrl Pts',(0.530469085518871,7.9277460963672,64.1253779099398));
#61916=CARTESIAN_POINT('Ctrl Pts',(1.26865250408552,7.84354558166536,64.0894448731624));
#61917=CARTESIAN_POINT('Ctrl Pts',(2.21460367329774,7.59841963969145,64.0453188475074));
#61918=CARTESIAN_POINT('Ctrl Pts',(2.44196588209815,7.52843046875656,64.0348285139961));
#61919=CARTESIAN_POINT('Ctrl Pts',(2.78341406173769,7.40622176143864,64.019322518065));
#61920=CARTESIAN_POINT('Ctrl Pts',(2.89997527433777,7.36136264321405,64.0140736570269));
#61921=CARTESIAN_POINT('Ctrl Pts',(3.0632417961441,7.29404862251231,64.0067839341006));
#61922=CARTESIAN_POINT('Ctrl Pts',(3.11086022325393,7.27386722576488,64.0046653782119));
#61923=CARTESIAN_POINT('Ctrl Pts',(3.17845399733532,7.24443479096087,64.0016685019175));
#61924=CARTESIAN_POINT('Ctrl Pts',(3.19859339992578,7.235565321805,64.0007769128658));
#61925=CARTESIAN_POINT('Ctrl Pts',(3.23397108687755,7.21980828259798,63.9992129871672));
#61926=CARTESIAN_POINT('Ctrl Pts',(3.24922498244686,7.21295623487672,63.9985394128938));
#61927=CARTESIAN_POINT('Ctrl Pts',(3.27157105676704,7.20283311030566,63.9975537406742));
#61928=CARTESIAN_POINT('Ctrl Pts',(3.27868025021575,7.19959983691455,63.9972403183809));
#61929=CARTESIAN_POINT('Ctrl Pts',(3.29091426047964,7.1940139093937,63.996701231573));
#61930=CARTESIAN_POINT('Ctrl Pts',(3.29604136447162,7.19166629664088,63.9964753904016));
#61931=CARTESIAN_POINT('Ctrl Pts',(3.30622575751362,7.18698985944788,63.9960269462288));
#61932=CARTESIAN_POINT('Ctrl Pts',(3.31128310630907,7.18466117429932,63.9958043385356));
#61933=CARTESIAN_POINT('Ctrl Pts',(3.32318366999913,7.17916625729532,63.9952807019857));
#61934=CARTESIAN_POINT('Ctrl Pts',(3.33002483079712,7.17599557421387,63.9949798296979));
#61935=CARTESIAN_POINT('Ctrl Pts',(3.35361728734951,7.16502014018583,63.9939427367428));
#61936=CARTESIAN_POINT('Ctrl Pts',(3.37034582186741,7.1571664481374,63.9932082376562));
#61937=CARTESIAN_POINT('Ctrl Pts',(3.55477904334699,7.06978894979585,63.985119598948));
#61938=CARTESIAN_POINT('Ctrl Pts',(3.71966841235432,6.98444287871347,63.9779748539739));
#61939=CARTESIAN_POINT('Ctrl Pts',(4.28072169493017,6.66853389689715,63.9538265410862));
#61940=CARTESIAN_POINT('Ctrl Pts',(4.65975669480649,6.40941670241914,63.9378595921906));
#61941=CARTESIAN_POINT('Ctrl Pts',(5.28939977977875,5.89344817366404,63.9098137064711));
#61942=CARTESIAN_POINT('Ctrl Pts',(5.54903177527296,5.6496646169731,63.89767430744));
#61943=CARTESIAN_POINT('Ctrl Pts',(5.90859553882458,5.26327202000188,63.8786808015062));
#61944=CARTESIAN_POINT('Ctrl Pts',(6.02167792494257,5.13350984659474,63.8723354901088));
#61945=CARTESIAN_POINT('Ctrl Pts',(6.17076104171189,4.95072722260881,63.863290463233));
#61946=CARTESIAN_POINT('Ctrl Pts',(6.21048817200704,4.9007987631877,63.860809073322));
#61947=CARTESIAN_POINT('Ctrl Pts',(6.27218267299865,4.8213070086398,63.8568335614568));
#61948=CARTESIAN_POINT('Ctrl Pts',(6.29455447052026,4.7920622597193,63.8553661385901));
#61949=CARTESIAN_POINT('Ctrl Pts',(6.32195478545519,4.75572121436434,63.8535377267592));
#61950=CARTESIAN_POINT('Ctrl Pts',(6.32717711541763,4.74877103336481,63.8531878246028));
#61951=CARTESIAN_POINT('Ctrl Pts',(6.33537587813,4.73782210851243,63.8526362789881));
#61952=CARTESIAN_POINT('Ctrl Pts',(6.33836001645364,4.73382912141493,63.8524350658728));
#61953=CARTESIAN_POINT('Ctrl Pts',(6.3436580537528,4.72672598362314,63.852077008739));
#61954=CARTESIAN_POINT('Ctrl Pts',(6.34597344650699,4.72361694502721,63.8519202471015));
#61955=CARTESIAN_POINT('Ctrl Pts',(6.35131405905895,4.71643471979036,63.8515580195688));
#61956=CARTESIAN_POINT('Ctrl Pts',(6.35433764538506,4.71236032483842,63.8513524647364));
#61957=CARTESIAN_POINT('Ctrl Pts',(6.36262652433077,4.70116826931233,63.850787642565));
#61958=CARTESIAN_POINT('Ctrl Pts',(6.36788378119336,4.69404468798553,63.8504279435061));
#61959=CARTESIAN_POINT('Ctrl Pts',(6.39365515127953,4.65900151748875,63.8486575540353));
#61960=CARTESIAN_POINT('Ctrl Pts',(6.4139974556738,4.63095647999794,63.8472378647344));
#61961=CARTESIAN_POINT('Ctrl Pts',(6.86841664702163,3.99573081911279,63.8150330203316));
#61962=CARTESIAN_POINT('Ctrl Pts',(7.21459132249159,3.33027937341748,63.7807128586842));
#61963=CARTESIAN_POINT('Ctrl Pts',(7.59689770166168,2.24393909209498,63.7306458109734));
#61964=CARTESIAN_POINT('Ctrl Pts',(7.70185451943391,1.85191714279034,63.7135659762062));
#61965=CARTESIAN_POINT('Ctrl Pts',(7.78212536859619,1.42247849583244,63.6958736931847));
#61966=CARTESIAN_POINT('Ctrl Pts',(7.7877474341483,1.39136991685154,63.6945974400299));
#61967=CARTESIAN_POINT('Ctrl Pts',(7.79547377165128,1.34710325910973,63.6927887913858));
#61968=CARTESIAN_POINT('Ctrl Pts',(7.7977314736105,1.33397240681414,63.6922532171616));
#61969=CARTESIAN_POINT('Ctrl Pts',(7.80156138916666,1.31135553735924,63.6913323059691));
#61970=CARTESIAN_POINT('Ctrl Pts',(7.80314949768616,1.30187225624173,63.690946642583));
#61971=CARTESIAN_POINT('Ctrl Pts',(7.80629371567735,1.28288432205146,63.6901753893163));
#61972=CARTESIAN_POINT('Ctrl Pts',(7.80784976573041,1.27337967453623,63.6897898014468));
#61973=CARTESIAN_POINT('Ctrl Pts',(7.8113066844272,1.25201958680365,63.6889243169866));
#61974=CARTESIAN_POINT('Ctrl Pts',(7.81319792899082,1.24016260522442,63.6884446191057));
#61975=CARTESIAN_POINT('Ctrl Pts',(7.81967402108194,1.19895849624785,63.686780159549));
#61976=CARTESIAN_POINT('Ctrl Pts',(7.82412059200975,1.16958977833616,63.685598261645));
#61977=CARTESIAN_POINT('Ctrl Pts',(7.87937518285511,0.790220869603066,63.6703881259816));
#61978=CARTESIAN_POINT('Ctrl Pts',(7.9068244351229,0.437210266177055,63.6568858817682));
#61979=CARTESIAN_POINT('Ctrl Pts',(7.91624864564317,-0.455304595667546,
63.62374615972));
#61980=CARTESIAN_POINT('Ctrl Pts',(7.86687042817707,-0.993287822590111,
63.6047467466212));
#61981=CARTESIAN_POINT('Ctrl Pts',(7.70774213273537,-1.8049134457731,63.5742555361342));
#61982=CARTESIAN_POINT('Ctrl Pts',(7.63687206082662,-2.08450597952448,63.5633783022865));
#61983=CARTESIAN_POINT('Ctrl Pts',(7.54700868196269,-2.37207761037149,63.5513062634907));
#61984=CARTESIAN_POINT('Ctrl Pts',(7.54307469003259,-2.38455791561117,63.5507805668073));
#61985=CARTESIAN_POINT('Ctrl Pts',(7.53732814477398,-2.40263189271311,63.5500165994312));
#61986=CARTESIAN_POINT('Ctrl Pts',(7.53554027822042,-2.40823343738295,63.549779458266));
#61987=CARTESIAN_POINT('Ctrl Pts',(7.53240825660417,-2.41800870192283,63.549364969387));
#61988=CARTESIAN_POINT('Ctrl Pts',(7.53106687187501,-2.42218331221409,63.549187750132));
#61989=CARTESIAN_POINT('Ctrl Pts',(7.52846819721708,-2.4302477888818,63.5488449936077));
#61990=CARTESIAN_POINT('Ctrl Pts',(7.52721136117553,-2.43413780135328,63.5486794776092));
#61991=CARTESIAN_POINT('Ctrl Pts',(7.52422388434788,-2.44335985151692,63.5482866523986));
#61992=CARTESIAN_POINT('Ctrl Pts',(7.52249059184378,-2.44869102198768,63.5480592180016));
#61993=CARTESIAN_POINT('Ctrl Pts',(7.51729972731645,-2.46459928580051,63.5473795066422));
#61994=CARTESIAN_POINT('Ctrl Pts',(7.51382551381067,-2.47517089831649,63.5469264341903));
#61995=CARTESIAN_POINT('Ctrl Pts',(7.47739818319091,-2.58523139427013,63.5421948355159));
#61996=CARTESIAN_POINT('Ctrl Pts',(7.44249770121712,-2.6840510691432,63.5378148009425));
#61997=CARTESIAN_POINT('Ctrl Pts',(7.40096487679848,-2.79460497503083,63.5327724174956));
#61998=CARTESIAN_POINT('Ctrl Pts',(7.39625368563849,-2.80704996201716,63.532202813432));
#61999=CARTESIAN_POINT('Ctrl Pts',(7.3825742744057,-2.84291168628154,63.5305558186826));
#62000=CARTESIAN_POINT('Ctrl Pts',(7.3735261457789,-2.86629759954752,63.5294748755323));
#62001=CARTESIAN_POINT('Ctrl Pts',(7.10216940202607,-3.55786150962325,63.4973124365846));
#62002=CARTESIAN_POINT('Ctrl Pts',(6.75024813504183,-4.18729509146563,63.4629170636766));
#62003=CARTESIAN_POINT('Ctrl Pts',(6.07543787764888,-5.0828894855077,63.4127532224534));
#62004=CARTESIAN_POINT('Ctrl Pts',(5.80832422935133,-5.38610652872779,63.3954243789023));
#62005=CARTESIAN_POINT('Ctrl Pts',(5.50913175319859,-5.67746300934643,63.3785323732826));
#62006=CARTESIAN_POINT('Ctrl Pts',(5.49902717940968,-5.6872505641499,63.3779645582292));
#62007=CARTESIAN_POINT('Ctrl Pts',(5.48278067953501,-5.70290357136074,63.3770558740115));
#62008=CARTESIAN_POINT('Ctrl Pts',(5.47665534457708,-5.70878615481774,63.3767142451668));
#62009=CARTESIAN_POINT('Ctrl Pts',(5.46495112424964,-5.71999035423805,63.3760633050793));
#62010=CARTESIAN_POINT('Ctrl Pts',(5.45937391111856,-5.72531369813512,63.3757539174831));
#62011=CARTESIAN_POINT('Ctrl Pts',(5.44984044537626,-5.73438661330298,63.3752264136606));
#62012=CARTESIAN_POINT('Ctrl Pts',(5.44588808866382,-5.73814025942146,63.3750081176793));
#62013=CARTESIAN_POINT('Ctrl Pts',(5.43789256014338,-5.74571809923725,63.3745673064618));
#62014=CARTESIAN_POINT('Ctrl Pts',(5.43384922621532,-5.74954211728927,63.3743447989949));
#62015=CARTESIAN_POINT('Ctrl Pts',(5.42432528555825,-5.75853044651465,63.3738216537178));
#62016=CARTESIAN_POINT('Ctrl Pts',(5.4188413288419,-5.76369120965395,63.3735211718836));
#62017=CARTESIAN_POINT('Ctrl Pts',(5.40265994777439,-5.77887544362545,63.3726367479052));
#62018=CARTESIAN_POINT('Ctrl Pts',(5.3919419943126,-5.78887704457624,63.372053764352));
#62019=CARTESIAN_POINT('Ctrl Pts',(5.30031123459827,-5.87390824924702,63.3670936249897));
#62020=CARTESIAN_POINT('Ctrl Pts',(5.21786276207866,-5.947268847781,63.362789508506));
#62021=CARTESIAN_POINT('Ctrl Pts',(4.41624326512983,-6.63102330214115,63.3223712004803));
#62022=CARTESIAN_POINT('Ctrl Pts',(3.59505534477739,-7.10977555305068,63.2928519502779));
#62023=CARTESIAN_POINT('Ctrl Pts',(2.44847729209401,-7.52766630663646,63.2494133018637));
#62024=CARTESIAN_POINT('Ctrl Pts',(2.18317760616102,-7.60884422009957,63.2391360996766));
#62025=CARTESIAN_POINT('Ctrl Pts',(1.9030926786154,-7.67869064814262,63.2275628635226));
#62026=CARTESIAN_POINT('Ctrl Pts',(1.89198924616834,-7.68143401345262,63.2271028956903));
#62027=CARTESIAN_POINT('Ctrl Pts',(1.87632441958178,-7.68526835372855,63.2264522738007));
#62028=CARTESIAN_POINT('Ctrl Pts',(1.87176789857552,-7.6863793771852,63.2262628215316));
#62029=CARTESIAN_POINT('Ctrl Pts',(1.86396266427317,-7.68827518733989,63.2259379434895));
#62030=CARTESIAN_POINT('Ctrl Pts',(1.86071444492254,-7.68906196648387,63.2258026385819));
#62031=CARTESIAN_POINT('Ctrl Pts',(1.85451332557606,-7.69055983336048,63.2255441322447));
#62032=CARTESIAN_POINT('Ctrl Pts',(1.85156052017422,-7.69127127757958,63.2254209529526));
#62033=CARTESIAN_POINT('Ctrl Pts',(1.84466740737854,-7.69292789356277,63.2251332013336));
#62034=CARTESIAN_POINT('Ctrl Pts',(1.84072678530712,-7.69387173802188,63.224968549599));
#62035=CARTESIAN_POINT('Ctrl Pts',(1.82681955226321,-7.69719145544059,63.2243869322008));
#62036=CARTESIAN_POINT('Ctrl Pts',(1.81684909027408,-7.69955098427875,63.2239689971357));
#62037=CARTESIAN_POINT('Ctrl Pts',(1.71229761515064,-7.72407890233106,63.2195766644576));
#62038=CARTESIAN_POINT('Ctrl Pts',(1.61732403433772,-7.74452190314256,63.2155026220458));
#62039=CARTESIAN_POINT('Ctrl Pts',(1.38592891000282,-7.78988765208269,63.2054166934043));
#62040=CARTESIAN_POINT('Ctrl Pts',(1.2491833889571,-7.81298190173457,63.1993228071755));
#62041=CARTESIAN_POINT('Ctrl Pts',(0.726161255954787,-7.88723082450871,
63.1756956064618));
#62042=CARTESIAN_POINT('Ctrl Pts',(0.336905156081771,-7.91341924702081,
63.1574804741885));
#62043=CARTESIAN_POINT('Ctrl Pts',(-0.417462906007593,-7.90839513239287,
63.1226286602222));
#62044=CARTESIAN_POINT('Ctrl Pts',(-0.781656927756021,-7.88073833424636,
63.1060071737824));
#62045=CARTESIAN_POINT('Ctrl Pts',(-1.39371326583922,-7.7913960768418,63.0790164059279));
#62046=CARTESIAN_POINT('Ctrl Pts',(-1.64286666338273,-7.74269299004363,
63.068292933197));
#62047=CARTESIAN_POINT('Ctrl Pts',(-1.9277192577267,-7.67263889127527,63.0563515270936));
#62048=CARTESIAN_POINT('Ctrl Pts',(-1.96610142180214,-7.66289334083986,
63.0547491010746));
#62049=CARTESIAN_POINT('Ctrl Pts',(-2.01496393843085,-7.65009544855771,
63.0527173631103));
#62050=CARTESIAN_POINT('Ctrl Pts',(-2.02551299594876,-7.64730914438126,
63.0522792165842));
#62051=CARTESIAN_POINT('Ctrl Pts',(-2.04241015141029,-7.64280871204743,
63.0515781872817));
#62052=CARTESIAN_POINT('Ctrl Pts',(-2.04876191680676,-7.6411084826779,63.0513148421149));
#62053=CARTESIAN_POINT('Ctrl Pts',(-2.06079522574288,-7.63787134477648,
63.0508162728669));
#62054=CARTESIAN_POINT('Ctrl Pts',(-2.06647718619806,-7.6363360115257,63.0505809965113));
#62055=CARTESIAN_POINT('Ctrl Pts',(-2.07934327170509,-7.63284403078826,
63.0500485608063));
#62056=CARTESIAN_POINT('Ctrl Pts',(-2.08652636320027,-7.63088357767284,
63.0497515285542));
#62057=CARTESIAN_POINT('Ctrl Pts',(-2.10496928071966,-7.62582203615739,
63.0489894583112));
#62058=CARTESIAN_POINT('Ctrl Pts',(-2.11622504508396,-7.62270614414721,
63.0485249144724));
#62059=CARTESIAN_POINT('Ctrl Pts',(-2.18136083557474,-7.60451945130429,
63.0458398035159));
#62060=CARTESIAN_POINT('Ctrl Pts',(-2.23508732211326,-7.58890216100012,
63.0436375293616));
#62061=CARTESIAN_POINT('Ctrl Pts',(-3.20395181154837,-7.29608961704842,
63.0041357442748));
#62062=CARTESIAN_POINT('Ctrl Pts',(-4.06132829524855,-6.85590793380312,
62.9739122953314));
#62063=CARTESIAN_POINT('Ctrl Pts',(-4.94136981320677,-6.17984006139831,
62.9341996321728));
#62064=CARTESIAN_POINT('Ctrl Pts',(-5.06053099202144,-6.08264590409552,
62.9285731183903));
#62065=CARTESIAN_POINT('Ctrl Pts',(-5.25598298303272,-5.91350445812071,
62.9187780032969));
#62066=CARTESIAN_POINT('Ctrl Pts',(-5.33381422272958,-5.84339937378735,
62.9147170813021));
#62067=CARTESIAN_POINT('Ctrl Pts',(-5.4233394050688,-5.75948206639975,62.9098235529183));
#62068=CARTESIAN_POINT('Ctrl Pts',(-5.43640919932414,-5.74714702990013,
62.9091034507351));
#62069=CARTESIAN_POINT('Ctrl Pts',(-5.45353595967742,-5.73087240418694,
62.9081521337923));
#62070=CARTESIAN_POINT('Ctrl Pts',(-5.45763095582354,-5.72697278903235,
62.907924092695));
#62071=CARTESIAN_POINT('Ctrl Pts',(-5.46434583781644,-5.72056454569913,
62.9075491989302));
#62072=CARTESIAN_POINT('Ctrl Pts',(-5.46696816190752,-5.71805852308085,
62.9074025540742));
#62073=CARTESIAN_POINT('Ctrl Pts',(-5.4720497004845,-5.71319566248862,62.9071179222737));
#62074=CARTESIAN_POINT('Ctrl Pts',(-5.47450911867186,-5.7108390374761,62.9069799521728));
#62075=CARTESIAN_POINT('Ctrl Pts',(-5.48018816696163,-5.70539030933474,
62.9066608792007));
#62076=CARTESIAN_POINT('Ctrl Pts',(-5.48340670085129,-5.70229707048499,
62.9064796869394));
#62077=CARTESIAN_POINT('Ctrl Pts',(-5.49371482737696,-5.69237343401278,
62.9058982213199));
#62078=CARTESIAN_POINT('Ctrl Pts',(-5.50079426524045,-5.68553254908063,
62.905497128717));
#62079=CARTESIAN_POINT('Ctrl Pts',(-5.56359780145813,-5.62461817598976,
62.9019234905728));
#62080=CARTESIAN_POINT('Ctrl Pts',(-5.6185340923889,-5.56974182785456,62.8986892485283));
#62081=CARTESIAN_POINT('Ctrl Pts',(-5.67534262057534,-5.51129948746517,
62.8952386707162));
#62082=CARTESIAN_POINT('Ctrl Pts',(-5.67803122667456,-5.50852950344129,
62.8950751097641));
#62083=CARTESIAN_POINT('Ctrl Pts',(-5.69261932790654,-5.4934778260836,62.8941862719127));
#62084=CARTESIAN_POINT('Ctrl Pts',(-5.70448093400352,-5.48115961311917,
62.8934585910519));
#62085=CARTESIAN_POINT('Ctrl Pts',(-6.24308788190891,-4.91817715748503,
62.8601935377421));
#62086=CARTESIAN_POINT('Ctrl Pts',(-6.68756186300077,-4.29432807408607,
62.8234329591282));
#62087=CARTESIAN_POINT('Ctrl Pts',(-7.12366409251882,-3.44588679001686,
62.7806759099165));
#62088=CARTESIAN_POINT('Ctrl Pts',(-7.20513390733723,-3.27212120769043,
62.7722276079567));
#62089=CARTESIAN_POINT('Ctrl Pts',(-7.36119616298685,-2.90509018382808,
62.7550709903763));
#62090=CARTESIAN_POINT('Ctrl Pts',(-7.4346810007932,-2.71150969312545,62.7464017701289));
#62091=CARTESIAN_POINT('Ctrl Pts',(-7.51176582974629,-2.48164305530003,
62.7365421595076));
#62092=CARTESIAN_POINT('Ctrl Pts',(-7.52281287159221,-2.44795111802535,
62.735107666452));
#62093=CARTESIAN_POINT('Ctrl Pts',(-7.53691346826921,-2.40394923385608,
62.7332478863943));
#62094=CARTESIAN_POINT('Ctrl Pts',(-7.54017294959365,-2.39370600503139,
62.7328159091998));
#62095=CARTESIAN_POINT('Ctrl Pts',(-7.54543185889127,-2.37706205824172,
62.7321155558766));
#62096=CARTESIAN_POINT('Ctrl Pts',(-7.54744403879132,-2.37066540184412,
62.7318467661456));
#62097=CARTESIAN_POINT('Ctrl Pts',(-7.55128740645077,-2.35839296618936,
62.7313317859079));
#62098=CARTESIAN_POINT('Ctrl Pts',(-7.55311987483477,-2.35251759491574,
62.7310855540372));
#62099=CARTESIAN_POINT('Ctrl Pts',(-7.55727925155486,-2.33912659191759,
62.7305250581618));
#62100=CARTESIAN_POINT('Ctrl Pts',(-7.55960180996909,-2.33160961015453,
62.7302109351507));
#62101=CARTESIAN_POINT('Ctrl Pts',(-7.56678783091468,-2.30822837883013,
62.7292354455046));
#62102=CARTESIAN_POINT('Ctrl Pts',(-7.57161261218675,-2.29235223779771,
62.7285753295871));
#62103=CARTESIAN_POINT('Ctrl Pts',(-7.60785615022647,-2.1717285639451,62.7235768505951));
#62104=CARTESIAN_POINT('Ctrl Pts',(-7.63715052624431,-2.06635262251859,
62.719307344021));
#62105=CARTESIAN_POINT('Ctrl Pts',(-7.68213387188573,-1.89048872157463,
62.7123303695666));
#62106=CARTESIAN_POINT('Ctrl Pts',(-7.69905907623131,-1.82033460666389,
62.7095858501598));
#62107=CARTESIAN_POINT('Ctrl Pts',(-7.84576864342689,-1.17353748112774,
62.6846112895349));
#62108=CARTESIAN_POINT('Ctrl Pts',(-7.91150681219482,-0.584258005828338,
62.6644373132321));
#62109=CARTESIAN_POINT('Ctrl Pts',(-7.91060580399575,0.46049749972319,62.6281482034686));
#62110=CARTESIAN_POINT('Ctrl Pts',(-7.87118945758822,0.913255257185715,
62.6121769119374));
#62111=CARTESIAN_POINT('Ctrl Pts',(-7.78829509126223,1.38823526958181,62.59306333534));
#62112=CARTESIAN_POINT('Ctrl Pts',(-7.78322976338027,1.41635871353383,62.5919225943629));
#62113=CARTESIAN_POINT('Ctrl Pts',(-7.77682397983582,1.45085221115423,62.5905117245318));
#62114=CARTESIAN_POINT('Ctrl Pts',(-7.7756278347614,1.45724916428308,62.5902495764683));
#62115=CARTESIAN_POINT('Ctrl Pts',(-7.77363662771286,1.46782583521355,62.589815310894));
#62116=CARTESIAN_POINT('Ctrl Pts',(-7.77284608319469,1.47200640931157,62.5896434463724));
#62117=CARTESIAN_POINT('Ctrl Pts',(-7.77147477629815,1.47922627612479,62.5893462610977));
#62118=CARTESIAN_POINT('Ctrl Pts',(-7.77089560252826,1.48226586994809,62.5892210300435));
#62119=CARTESIAN_POINT('Ctrl Pts',(-7.76959250367982,1.48908297969179,62.5889399072276));
#62120=CARTESIAN_POINT('Ctrl Pts',(-7.76886760899642,1.49286029736036,62.5887839611286));
#62121=CARTESIAN_POINT('Ctrl Pts',(-7.76693325427897,1.5029003654527,62.5883689885195));
#62122=CARTESIAN_POINT('Ctrl Pts',(-7.76571897624178,1.50916217369208,62.588109691724));
#62123=CARTESIAN_POINT('Ctrl Pts',(-7.76007399132928,1.53808511066186,62.5869097918019));
#62124=CARTESIAN_POINT('Ctrl Pts',(-7.75555169614519,1.56072804379716,62.5859641186058));
#62125=CARTESIAN_POINT('Ctrl Pts',(-7.72029963957853,1.73329641232846,62.5787104949063));
#62126=CARTESIAN_POINT('Ctrl Pts',(-7.68532570494636,1.88231423130748,62.5721798263984));
#62127=CARTESIAN_POINT('Ctrl Pts',(-7.57980728920657,2.27971022146038,62.5542177583192));
#62128=CARTESIAN_POINT('Ctrl Pts',(-7.50139091644964,2.52580288121517,62.5425153881825));
#62129=CARTESIAN_POINT('Ctrl Pts',(-7.18146988446969,3.38248560371697,62.5006625763827));
#62130=CARTESIAN_POINT('Ctrl Pts',(-6.87618048230651,3.96649501451001,62.4703267703));
#62131=CARTESIAN_POINT('Ctrl Pts',(-6.48072918796758,4.5371240398075,62.4409769657717));
#62132=CARTESIAN_POINT('Ctrl Pts',(-6.45901019966186,4.56799000133599,62.4393893559593));
#62133=CARTESIAN_POINT('Ctrl Pts',(-6.36335846992165,4.70187936595585,62.4325026075614));
#62134=CARTESIAN_POINT('Ctrl Pts',(-6.28717385671669,4.80327465678593,62.4272874754914));
#62135=CARTESIAN_POINT('Ctrl Pts',(-6.19891406928886,4.9150410708856,62.4215365002331));
#62136=CARTESIAN_POINT('Ctrl Pts',(-6.18920969064977,4.92725560283619,62.4209079576652));
#62137=CARTESIAN_POINT('Ctrl Pts',(-6.17454211831647,4.94560541293738,62.4199636264361));
#62138=CARTESIAN_POINT('Ctrl Pts',(-6.16960579865482,4.95176206627433,62.4196467753303));
#62139=CARTESIAN_POINT('Ctrl Pts',(-6.16104212414009,4.9624101276146,62.4190987497231));
#62140=CARTESIAN_POINT('Ctrl Pts',(-6.15741905348151,4.96690496487448,62.4188674054333));
#62141=CARTESIAN_POINT('Ctrl Pts',(-6.14988837174393,4.97622674158804,62.4183876066342));
#62142=CARTESIAN_POINT('Ctrl Pts',(-6.14597998966672,4.98105305487234,62.4181391830444));
#62143=CARTESIAN_POINT('Ctrl Pts',(-6.13679599913651,4.99236675164489,62.4175568115567));
#62144=CARTESIAN_POINT('Ctrl Pts',(-6.13151577588889,4.99885038869146,62.417223048027));
#62145=CARTESIAN_POINT('Ctrl Pts',(-6.1143620711042,5.01984551808365,62.4161421966239));
#62146=CARTESIAN_POINT('Ctrl Pts',(-6.10244723556167,5.03432322217302,62.415396764018));
#62147=CARTESIAN_POINT('Ctrl Pts',(-5.78398682149654,5.41849234018072,62.3956130937319));
#62148=CARTESIAN_POINT('Ctrl Pts',(-5.44445470916681,5.75956099169193,62.3780540175138));
#62149=CARTESIAN_POINT('Ctrl Pts',(-4.96336407191662,6.16202252170058,62.3560695677971));
#62150=CARTESIAN_POINT('Ctrl Pts',(-4.84807629523877,6.25313213893486,62.3509848075285));
#62151=CARTESIAN_POINT('Ctrl Pts',(-4.6115995757591,6.42954178443001,62.3408206943881));
#62152=CARTESIAN_POINT('Ctrl Pts',(-4.49041825464805,6.51475264739413,62.3357437288948));
#62153=CARTESIAN_POINT('Ctrl Pts',(-3.96712160646155,6.86117709332413,62.3141275865617));
#62154=CARTESIAN_POINT('Ctrl Pts',(-3.54413330100616,7.08892273531164,62.2974384528388));
#62155=CARTESIAN_POINT('Ctrl Pts',(-3.08724481391446,7.2837587179189,62.2777755919333));
#62156=CARTESIAN_POINT('Ctrl Pts',(-3.07127431262629,7.29050723133412,62.2770862523332));
#62157=CARTESIAN_POINT('Ctrl Pts',(-3.04055341769443,7.30336982970232,62.2757561245411));
#62158=CARTESIAN_POINT('Ctrl Pts',(-3.02580642992365,7.30949186996506,62.2751158084014));
#62159=CARTESIAN_POINT('Ctrl Pts',(-3.00578918095397,7.31773084057933,62.2742440768058));
#62160=CARTESIAN_POINT('Ctrl Pts',(-3.00053494065294,7.31988683827231,62.274015019307));
#62161=CARTESIAN_POINT('Ctrl Pts',(-2.99224898100953,7.32327643536549,62.2736534092099));
#62162=CARTESIAN_POINT('Ctrl Pts',(-2.98921880145346,7.32451381800245,62.273521087041));
#62163=CARTESIAN_POINT('Ctrl Pts',(-2.98337748964284,7.32689490608685,62.2732658501463));
#62164=CARTESIAN_POINT('Ctrl Pts',(-2.98056646495081,7.32803887534106,62.2731429516112));
#62165=CARTESIAN_POINT('Ctrl Pts',(-2.97392781174595,7.33073607721785,62.2728525406626));
#62166=CARTESIAN_POINT('Ctrl Pts',(-2.97009962680472,7.33228792874572,62.2726849433419));
#62167=CARTESIAN_POINT('Ctrl Pts',(-2.95882832237606,7.33684676143428,62.2721910955213));
#62168=CARTESIAN_POINT('Ctrl Pts',(-2.95138188461661,7.33984539425654,62.2718643282391));
#62169=CARTESIAN_POINT('Ctrl Pts',(-2.89220031167994,7.36357281272257,62.2692633722345));
#62170=CARTESIAN_POINT('Ctrl Pts',(-2.8402531463129,7.38376523098079,62.2669565456848));
#62171=CARTESIAN_POINT('Ctrl Pts',(-2.58734664707277,7.47900897408639,62.255627055696));
#62172=CARTESIAN_POINT('Ctrl Pts',(-2.38361528155584,7.54641001514582,62.2462020317969));
#62173=CARTESIAN_POINT('Ctrl Pts',(-1.25651078159794,7.86909604488385,62.1934390942523));
#62174=CARTESIAN_POINT('Ctrl Pts',(-0.294949493266388,7.96338125329544,
62.1475032689685));
#62175=CARTESIAN_POINT('Ctrl Pts',(0.715692789689113,7.87875732724936,62.1059731915442));
#62176=CARTESIAN_POINT('Ctrl Pts',(0.771235192753037,7.87351444020248,62.1037077037033));
#62177=CARTESIAN_POINT('Ctrl Pts',(0.838321498414512,7.86646516463718,62.1009913316676));
#62178=CARTESIAN_POINT('Ctrl Pts',(0.849922035340624,7.86522025480242,62.1005223402112));
#62179=CARTESIAN_POINT('Ctrl Pts',(0.868917657086711,7.863139226174,62.0997555528502));
#62180=CARTESIAN_POINT('Ctrl Pts',(0.876314370984281,7.86231832913185,62.0994572653027));
#62181=CARTESIAN_POINT('Ctrl Pts',(0.889558426021794,7.8608295646086,62.0989236926657));
#62182=CARTESIAN_POINT('Ctrl Pts',(0.895406195920845,7.8601656077742,62.0986882813291));
#62183=CARTESIAN_POINT('Ctrl Pts',(0.907787966926001,7.85874578233914,62.0981902171344));
#62184=CARTESIAN_POINT('Ctrl Pts',(0.914321779268518,7.85798828890454,62.0979276170184));
#62185=CARTESIAN_POINT('Ctrl Pts',(0.931700969017612,7.85595147406421,62.097229730652));
#62186=CARTESIAN_POINT('Ctrl Pts',(0.942544672888111,7.85465784101333,62.0967949076778));
#62187=CARTESIAN_POINT('Ctrl Pts',(0.992795636039444,7.84855743805343,62.0947827476503));
#62188=CARTESIAN_POINT('Ctrl Pts',(1.03216936823762,7.84347649250509,62.0932142942121));
#62189=CARTESIAN_POINT('Ctrl Pts',(1.32398045152804,7.80358459984253,62.0816485923894));
#62190=CARTESIAN_POINT('Ctrl Pts',(1.57465177610998,7.75688997567654,62.0720464924182));
#62191=CARTESIAN_POINT('Ctrl Pts',(2.08916802591955,7.63507126680689,62.0527788769906));
#62192=CARTESIAN_POINT('Ctrl Pts',(2.35223901295436,7.55816889891921,62.0431763295241));
#62193=CARTESIAN_POINT('Ctrl Pts',(2.84348983250134,7.38642332603823,62.0252229098963));
#62194=CARTESIAN_POINT('Ctrl Pts',(3.07225021711206,7.29424171940297,62.0168508495463));
#62195=CARTESIAN_POINT('Ctrl Pts',(3.66538962775336,7.02236844118222,61.9944148772895));
#62196=CARTESIAN_POINT('Ctrl Pts',(4.02084619549653,6.82506233614114,61.9802175514428));
#62197=CARTESIAN_POINT('Ctrl Pts',(4.41322133127512,6.56593744115765,61.9619476235685));
#62198=CARTESIAN_POINT('Ctrl Pts',(4.46645108020621,6.52984466277824,61.959409543361));
#62199=CARTESIAN_POINT('Ctrl Pts',(4.52671311230428,6.48790200643167,61.9564604434949));
#62200=CARTESIAN_POINT('Ctrl Pts',(4.53418372722666,6.48268323864325,61.9560935040183));
#62201=CARTESIAN_POINT('Ctrl Pts',(4.54512042996369,6.47501500313232,61.9555543213263));
#62202=CARTESIAN_POINT('Ctrl Pts',(4.54859361388196,6.47257561943291,61.9553827964435));
#62203=CARTESIAN_POINT('Ctrl Pts',(4.55475263369076,6.46824243872364,61.9550781017596));
#62204=CARTESIAN_POINT('Ctrl Pts',(4.55743925836043,6.46634975906109,61.954945012276));
#62205=CARTESIAN_POINT('Ctrl Pts',(4.56297372485485,6.46244566261971,61.9546704768296));
#62206=CARTESIAN_POINT('Ctrl Pts',(4.56582140753901,6.46043404349387,61.954529015943));
#62207=CARTESIAN_POINT('Ctrl Pts',(4.57319264049173,6.45521965491716,61.9541623206839));
#62208=CARTESIAN_POINT('Ctrl Pts',(4.57771414851098,6.45201401846675,61.9539368793342));
#62209=CARTESIAN_POINT('Ctrl Pts',(4.5875557230671,6.44502103448786,61.9534450742805));
#62210=CARTESIAN_POINT('Ctrl Pts',(4.59287447215981,6.44123184877868,61.9531785790539));
#62211=CARTESIAN_POINT('Ctrl Pts',(4.60831535912621,6.43020259614218,61.9524028785108));
#62212=CARTESIAN_POINT('Ctrl Pts',(4.61842507221944,6.42294525319064,61.951892450943));
#62213=CARTESIAN_POINT('Ctrl Pts',(4.7200848879916,6.3496037824493,61.9467344238851));
#62214=CARTESIAN_POINT('Ctrl Pts',(4.81022346599078,6.28159354561954,61.9419535905088));
#62215=CARTESIAN_POINT('Ctrl Pts',(5.07914361004057,6.06950839979982,61.9271325609015));
#62216=CARTESIAN_POINT('Ctrl Pts',(5.25313147016896,5.91956330116238,61.9167724235427));
#62217=CARTESIAN_POINT('Ctrl Pts',(6.09272473000039,5.12979146979673,61.8638008903368));
#62218=CARTESIAN_POINT('Ctrl Pts',(6.64945863589698,4.38424218008588,61.8198021055462));
#62219=CARTESIAN_POINT('Ctrl Pts',(7.07115389512443,3.54723703613978,61.7813355079288));
#62220=CARTESIAN_POINT('Ctrl Pts',(7.07727501766205,3.53500867410727,61.7807753927345));
#62221=CARTESIAN_POINT('Ctrl Pts',(7.10473691532622,3.47978993010312,61.7782545111206));
#62222=CARTESIAN_POINT('Ctrl Pts',(7.12571811929919,3.4366213039811,61.7763066474846));
#62223=CARTESIAN_POINT('Ctrl Pts',(7.15106927171243,3.38323109207717,61.7739252368066));
#62224=CARTESIAN_POINT('Ctrl Pts',(7.15581200046395,3.37318824950241,61.7734784846607));
#62225=CARTESIAN_POINT('Ctrl Pts',(7.16363659701015,3.35652871034776,61.7727393658837));
#62226=CARTESIAN_POINT('Ctrl Pts',(7.16673047708897,3.34991769250445,61.7724465749429));
#62227=CARTESIAN_POINT('Ctrl Pts',(7.17231511774406,3.33794125818065,61.7719170862362));
#62228=CARTESIAN_POINT('Ctrl Pts',(7.17480901655331,3.33257731605293,61.771680277911));
#62229=CARTESIAN_POINT('Ctrl Pts',(7.18014263837985,3.32107188633906,61.7711730528728));
#62230=CARTESIAN_POINT('Ctrl Pts',(7.18298050430277,3.31492954024937,61.7709027016555));
#62231=CARTESIAN_POINT('Ctrl Pts',(7.19066711075665,3.29823624603744,61.7701691444488));
#62232=CARTESIAN_POINT('Ctrl Pts',(7.19550051601744,3.28767823211026,61.7697064774336));
#62233=CARTESIAN_POINT('Ctrl Pts',(7.21964660206181,3.23462559028851,61.7673880529819));
#62234=CARTESIAN_POINT('Ctrl Pts',(7.23860635575607,3.19197084738868,61.7655446645335));
#62235=CARTESIAN_POINT('Ctrl Pts',(7.40097152010585,2.81780183194893,61.7495497861065));
#62236=CARTESIAN_POINT('Ctrl Pts',(7.52190081977087,2.4769794522955,61.7362055551303));
#62237=CARTESIAN_POINT('Ctrl Pts',(7.75854600509628,1.63011444920188,61.7049235016786));
#62238=CARTESIAN_POINT('Ctrl Pts',(7.8486176987374,1.11869924012562,61.6876223899349));
#62239=CARTESIAN_POINT('Ctrl Pts',(7.91363890963849,0.266949203041437,61.6575337902451));
#62240=CARTESIAN_POINT('Ctrl Pts',(7.91783427997919,-0.0695485862649099,
61.6452876338838));
#62241=CARTESIAN_POINT('Ctrl Pts',(7.89938993817325,-0.429101766765873,
61.6309654440322));
#62242=CARTESIAN_POINT('Ctrl Pts',(7.89806052012822,-0.45291248906759,61.6300115908312));
#62243=CARTESIAN_POINT('Ctrl Pts',(7.89615569121186,-0.484465230673838,
61.6287407452992));
#62244=CARTESIAN_POINT('Ctrl Pts',(7.89567650730703,-0.492213115333169,
61.6284281371634));
#62245=CARTESIAN_POINT('Ctrl Pts',(7.89491426804264,-0.504250113418869,
61.6279416350182));
#62246=CARTESIAN_POINT('Ctrl Pts',(7.89463911856142,-0.508539737088017,
61.6277680947527));
#62247=CARTESIAN_POINT('Ctrl Pts',(7.89410315837529,-0.516790171154996,
61.627434000733));
#62248=CARTESIAN_POINT('Ctrl Pts',(7.89384286242484,-0.520751014724079,
61.6272734698185));
#62249=CARTESIAN_POINT('Ctrl Pts',(7.89324349049632,-0.529767757479902,
61.6269077094448));
#62250=CARTESIAN_POINT('Ctrl Pts',(7.89290253786219,-0.53482352674502,61.6267023977075));
#62251=CARTESIAN_POINT('Ctrl Pts',(7.89218557899021,-0.54530483649764,61.626276292712));
#62252=CARTESIAN_POINT('Ctrl Pts',(7.89180883506443,-0.550730322857615,
61.6260554675534));
#62253=CARTESIAN_POINT('Ctrl Pts',(7.8908310532008,-0.56460431134283,61.6254901216285));
#62254=CARTESIAN_POINT('Ctrl Pts',(7.89022204238863,-0.573052231089277,
61.6251452597735));
#62255=CARTESIAN_POINT('Ctrl Pts',(7.8783849615531,-0.733654064097284,61.6185775413799));
#62256=CARTESIAN_POINT('Ctrl Pts',(7.86277164219871,-0.88544688873738,61.6121723347128));
#62257=CARTESIAN_POINT('Ctrl Pts',(7.8174038127089,-1.2286653070441,61.5973655778602));
#62258=CARTESIAN_POINT('Ctrl Pts',(7.78498756843565,-1.41964264024855,61.5888966547751));
#62259=CARTESIAN_POINT('Ctrl Pts',(7.65721737587657,-2.03462950518168,61.5611886559831));
#62260=CARTESIAN_POINT('Ctrl Pts',(7.53393730256748,-2.45204119837214,61.5417461119891));
#62261=CARTESIAN_POINT('Ctrl Pts',(7.23245424436947,-3.23043532558423,61.5054845859477));
#62262=CARTESIAN_POINT('Ctrl Pts',(7.0597814956763,-3.59216275943425,61.4886267024257));
#62263=CARTESIAN_POINT('Ctrl Pts',(6.84534745355643,-3.96560970148236,61.471190418263));
#62264=CARTESIAN_POINT('Ctrl Pts',(6.8300837192045,-3.9918414886753,61.46996522562));
#62265=CARTESIAN_POINT('Ctrl Pts',(6.80851735931988,-4.02841893095854,61.4682560407387));
#62266=CARTESIAN_POINT('Ctrl Pts',(6.80234141322475,-4.03883882006926,61.467769052098));
#62267=CARTESIAN_POINT('Ctrl Pts',(6.79160764834154,-4.05685407833064,61.4669269115225));
#62268=CARTESIAN_POINT('Ctrl Pts',(6.78706096483878,-4.06445604255309,61.4665714973881));
#62269=CARTESIAN_POINT('Ctrl Pts',(6.77761519835882,-4.08018913024572,61.4658358117663));
#62270=CARTESIAN_POINT('Ctrl Pts',(6.77271422436892,-4.08831911073927,61.4654555848434));
#62271=CARTESIAN_POINT('Ctrl Pts',(6.76126089847395,-4.10724134523986,61.4645704642823));
#62272=CARTESIAN_POINT('Ctrl Pts',(6.7546973140779,-4.11802678496741,61.4640658379744));
#62273=CARTESIAN_POINT('Ctrl Pts',(6.73364692585998,-4.15243155449798,61.4624557287968));
#62274=CARTESIAN_POINT('Ctrl Pts',(6.71906179407703,-4.17599058397504,61.4613526046534));
#62275=CARTESIAN_POINT('Ctrl Pts',(6.68502442888113,-4.23033038742051,61.4588067621071));
#62276=CARTESIAN_POINT('Ctrl Pts',(6.6654828140784,-4.2610545275215,61.4573662430706));
#62277=CARTESIAN_POINT('Ctrl Pts',(6.53569569642452,-4.46203353058331,61.4479353339613));
#62278=CARTESIAN_POINT('Ctrl Pts',(6.41914686498998,-4.62813351139385,61.4401064211871));
#62279=CARTESIAN_POINT('Ctrl Pts',(6.21085389210602,-4.9019538489769,61.4270716921437));
#62280=CARTESIAN_POINT('Ctrl Pts',(6.12237408811986,-5.01202498323201,61.4217934426387));
#62281=CARTESIAN_POINT('Ctrl Pts',(5.9613529236291,-5.20170860658311,61.4125874472854));
#62282=CARTESIAN_POINT('Ctrl Pts',(5.89004438212564,-5.28231755001206,61.4086379537091));
#62283=CARTESIAN_POINT('Ctrl Pts',(5.47865865400861,-5.72866665693717,61.3864803044406));
#62284=CARTESIAN_POINT('Ctrl Pts',(5.10620971446954,-6.06299464460321,61.3688388309151));
#62285=CARTESIAN_POINT('Ctrl Pts',(4.59390058809967,-6.44197263205721,61.3448907802586));
#62286=CARTESIAN_POINT('Ctrl Pts',(4.48092544231186,-6.52106117377738,61.3396218674391));
#62287=CARTESIAN_POINT('Ctrl Pts',(4.31400961149238,-6.63152476371396,61.3317793179069));
#62288=CARTESIAN_POINT('Ctrl Pts',(4.26167106018734,-6.66528012208291,61.3293121390376));
#62289=CARTESIAN_POINT('Ctrl Pts',(4.19985257758221,-6.70412369542239,61.3263829026868));
#62290=CARTESIAN_POINT('Ctrl Pts',(4.19075315020912,-6.70981551380764,61.3259513490234));
#62291=CARTESIAN_POINT('Ctrl Pts',(4.17693855835726,-6.7184176695386,61.3252955542655));
#62292=CARTESIAN_POINT('Ctrl Pts',(4.17223184937826,-6.7213416144,61.3250720129005));
#62293=CARTESIAN_POINT('Ctrl Pts',(4.16391141627536,-6.72649840273857,61.3246766429593));
#62294=CARTESIAN_POINT('Ctrl Pts',(4.16029895481449,-6.72873328726129,61.324504920477));
#62295=CARTESIAN_POINT('Ctrl Pts',(4.15270665852673,-6.73342188400935,61.3241438706768));
#62296=CARTESIAN_POINT('Ctrl Pts',(4.14872644612811,-6.73587497916082,61.323954511186));
#62297=CARTESIAN_POINT('Ctrl Pts',(4.14060388837366,-6.74087116521065,61.3235679082892));
#62298=CARTESIAN_POINT('Ctrl Pts',(4.13646136991116,-6.74341396930759,61.3233706498956));
#62299=CARTESIAN_POINT('Ctrl Pts',(4.12627810102043,-6.74965185601603,61.3228855156285));
#62300=CARTESIAN_POINT('Ctrl Pts',(4.12023473573557,-6.75334264392982,61.3225974113118));
#62301=CARTESIAN_POINT('Ctrl Pts',(4.1036123364545,-6.76346361382753,61.3218044147711));
#62302=CARTESIAN_POINT('Ctrl Pts',(4.09302318346262,-6.7698770653802,61.3212986213026));
#62303=CARTESIAN_POINT('Ctrl Pts',(3.79354731916229,-6.95029885664525,61.3069754204391));
#62304=CARTESIAN_POINT('Ctrl Pts',(3.4938958673471,-7.10565014139569,61.2920483404002));
#62305=CARTESIAN_POINT('Ctrl Pts',(2.38330367620491,-7.59417225138492,61.236897401619));
#62306=CARTESIAN_POINT('Ctrl Pts',(1.52798919228387,-7.8113695664866,61.1956596880325));
#62307=CARTESIAN_POINT('Ctrl Pts',(0.599642799317534,-7.88843294471139,
61.1574956783516));
#62308=CARTESIAN_POINT('Ctrl Pts',(0.544786388673252,-7.89241115018974,
61.1552606651854));
#62309=CARTESIAN_POINT('Ctrl Pts',(0.478245123481413,-7.89653967116389,
61.1525735656734));
#62310=CARTESIAN_POINT('Ctrl Pts',(0.466596437978362,-7.8972365383096,61.1521040527859));
#62311=CARTESIAN_POINT('Ctrl Pts',(0.447484251047435,-7.89833746498598,
61.1513351679276));
#62312=CARTESIAN_POINT('Ctrl Pts',(0.440021663352057,-7.89875672507535,
61.1510353105899));
#62313=CARTESIAN_POINT('Ctrl Pts',(0.426636542794986,-7.89948969458422,
61.1504981267411));
#62314=CARTESIAN_POINT('Ctrl Pts',(0.420714235242946,-7.8998073208754,61.1502606752044));
#62315=CARTESIAN_POINT('Ctrl Pts',(0.408151341442363,-7.90046692902595,
61.1497574552636));
#62316=CARTESIAN_POINT('Ctrl Pts',(0.401510667781274,-7.9008071991472,61.1494917417648));
#62317=CARTESIAN_POINT('Ctrl Pts',(0.383794417911599,-7.90169259146159,
61.1487836205281));
#62318=CARTESIAN_POINT('Ctrl Pts',(0.372718092706051,-7.90222280057098,
61.1483416900395));
#62319=CARTESIAN_POINT('Ctrl Pts',(0.320846568486834,-7.90459651862682,
61.1462757733571));
#62320=CARTESIAN_POINT('Ctrl Pts',(0.280038251950287,-7.9061474363438,61.1446611602098));
#62321=CARTESIAN_POINT('Ctrl Pts',(-0.0259326993814343,-7.91540387151853,
61.132633307875));
#62322=CARTESIAN_POINT('Ctrl Pts',(-0.291330886227619,-7.9100842323467,
61.1226483646982));
#62323=CARTESIAN_POINT('Ctrl Pts',(-0.78599656850133,-7.87523345576896,
61.1046326483856));
#62324=CARTESIAN_POINT('Ctrl Pts',(-1.01520338926843,-7.84897834297204,
61.0965241833831));
#62325=CARTESIAN_POINT('Ctrl Pts',(-1.31194357531869,-7.80176945752871,
61.086150030326));
#62326=CARTESIAN_POINT('Ctrl Pts',(-1.38079627222556,-7.78987832868687,
61.083751286987));
#62327=CARTESIAN_POINT('Ctrl Pts',(-1.50684733463846,-7.76638507354082,
61.0793660548154));
#62328=CARTESIAN_POINT('Ctrl Pts',(-1.56409199861762,-7.75505913973456,
61.0773769175412));
#62329=CARTESIAN_POINT('Ctrl Pts',(-1.66999878403781,-7.73288498133223,
61.0736954606509));
#62330=CARTESIAN_POINT('Ctrl Pts',(-1.71869369956481,-7.72220810733611,
61.0720022032264));
#62331=CARTESIAN_POINT('Ctrl Pts',(-1.80941574484892,-7.7014157102322,61.0688426481332));
#62332=CARTESIAN_POINT('Ctrl Pts',(-1.85146715041356,-7.69141460794823,
61.0673761557768));
#62333=CARTESIAN_POINT('Ctrl Pts',(-1.93020728305919,-7.67200464370164,
61.06462383519));
#62334=CARTESIAN_POINT('Ctrl Pts',(-1.96691449163024,-7.66267595473265,
61.063338147956));
#62335=CARTESIAN_POINT('Ctrl Pts',(-2.03591901926335,-7.64461078701827,
61.0609144736932));
#62336=CARTESIAN_POINT('Ctrl Pts',(-2.06823065595581,-7.63593231283413,
61.0597767729488));
#62337=CARTESIAN_POINT('Ctrl Pts',(-2.12918638008594,-7.61914513125845,
61.0576238848505));
#62338=CARTESIAN_POINT('Ctrl Pts',(-2.15784164755236,-7.61107920012856,
61.0566090335344));
#62339=CARTESIAN_POINT('Ctrl Pts',(-2.43408746857354,-7.53163560743304,
61.0467938395871));
#62340=CARTESIAN_POINT('Ctrl Pts',(-2.67808774422027,-7.44836573925284,
61.0378818421101));
#62341=CARTESIAN_POINT('Ctrl Pts',(-3.0552868471976,-7.2987048299721,61.0231617172854));
#62342=CARTESIAN_POINT('Ctrl Pts',(-3.19142717328143,-7.24021122860647,
61.0176461662436));
#62343=CARTESIAN_POINT('Ctrl Pts',(-3.39392595351592,-7.14638501419299,
61.0090245442973));
#62344=CARTESIAN_POINT('Ctrl Pts',(-3.46155896136129,-7.11387103004195,
61.0060729006649));
#62345=CARTESIAN_POINT('Ctrl Pts',(-3.53721131963036,-7.07616754691953,
61.0026788096852));
#62346=CARTESIAN_POINT('Ctrl Pts',(-3.54569782790225,-7.0719189746135,61.0022967459154));
#62347=CARTESIAN_POINT('Ctrl Pts',(-3.55801694570244,-7.06572394674907,
61.0017401864703));
#62348=CARTESIAN_POINT('Ctrl Pts',(-3.56185567451262,-7.06378960837373,
61.0015664826737));
#62349=CARTESIAN_POINT('Ctrl Pts',(-3.5686286278187,-7.06036978727621,61.0012595141639));
#62350=CARTESIAN_POINT('Ctrl Pts',(-3.57156349981377,-7.05888560489828,
61.0011263350456));
#62351=CARTESIAN_POINT('Ctrl Pts',(-3.57721539444195,-7.05602298069528,
61.000869549538));
#62352=CARTESIAN_POINT('Ctrl Pts',(-3.5799325478822,-7.05464479863411,61.0007459603149));
#62353=CARTESIAN_POINT('Ctrl Pts',(-3.58575297914487,-7.05168835767806,
61.0004809215841));
#62354=CARTESIAN_POINT('Ctrl Pts',(-3.58885601151714,-7.05010961969962,
61.0003394407779));
#62355=CARTESIAN_POINT('Ctrl Pts',(-3.6006589778881,-7.04409478165093,60.99980060489));
#62356=CARTESIAN_POINT('Ctrl Pts',(-3.60935170456554,-7.03964463868951,
60.9994023382798));
#62357=CARTESIAN_POINT('Ctrl Pts',(-3.72039732736456,-6.98253633938219,
60.9942967109243));
#62358=CARTESIAN_POINT('Ctrl Pts',(-3.82159292967034,-6.92766880547784,
60.9894488300577));
#62359=CARTESIAN_POINT('Ctrl Pts',(-4.08079200474085,-6.77972539832798,
60.9765967075683));
#62360=CARTESIAN_POINT('Ctrl Pts',(-4.23681802991186,-6.68333047761783,
60.9684301894143));
#62361=CARTESIAN_POINT('Ctrl Pts',(-4.97848709529102,-6.18870328909454,
60.9280128893947));
#62362=CARTESIAN_POINT('Ctrl Pts',(-5.51232280680041,-5.718384683933,60.8942861970079));
#62363=CARTESIAN_POINT('Ctrl Pts',(-6.1486255251246,-4.98471799443466,60.8520624192308));
#62364=CARTESIAN_POINT('Ctrl Pts',(-6.31084834836532,-4.77767940018079,
60.8410147605737));
#62365=CARTESIAN_POINT('Ctrl Pts',(-6.47408421270489,-4.54648873525531,
60.8295777797758));
#62366=CARTESIAN_POINT('Ctrl Pts',(-6.48563205509533,-4.53000033851557,
60.8287667725967));
#62367=CARTESIAN_POINT('Ctrl Pts',(-6.50155865463927,-4.50707406987797,
60.8276455375746));
#62368=CARTESIAN_POINT('Ctrl Pts',(-6.5059909809571,-4.50067361260898,60.8273332075242));
#62369=CARTESIAN_POINT('Ctrl Pts',(-6.51359638802572,-4.48965638735665,
60.8267967733307));
#62370=CARTESIAN_POINT('Ctrl Pts',(-6.51677402244096,-4.48504277830818,
60.8265724909336));
#62371=CARTESIAN_POINT('Ctrl Pts',(-6.52297403551785,-4.47602047617868,
60.8261345828073));
#62372=CARTESIAN_POINT('Ctrl Pts',(-6.52599685205926,-4.47161208718912,
60.8259209399952));
#62373=CARTESIAN_POINT('Ctrl Pts',(-6.53326003169092,-4.46099662257564,
60.8254072618057));
#62374=CARTESIAN_POINT('Ctrl Pts',(-6.53749602348712,-4.45478655511185,
60.8251073970829));
#62375=CARTESIAN_POINT('Ctrl Pts',(-6.55033035386074,-4.43591338286539,
60.824198001215));
#62376=CARTESIAN_POINT('Ctrl Pts',(-6.55890082210556,-4.42323131819342,
60.8235895550157));
#62377=CARTESIAN_POINT('Ctrl Pts',(-6.64103650996505,-4.30092823208214,
60.817746997335));
#62378=CARTESIAN_POINT('Ctrl Pts',(-6.71188559917261,-4.18950395641703,
60.8126187922149));
#62379=CARTESIAN_POINT('Ctrl Pts',(-6.96513637538515,-3.76828972021598,
60.7938986349276));
#62380=CARTESIAN_POINT('Ctrl Pts',(-7.12915331211552,-3.44794607440122,
60.7809916455826));
#62381=CARTESIAN_POINT('Ctrl Pts',(-7.48001179611938,-2.62966324681593,
60.7499704847939));
#62382=CARTESIAN_POINT('Ctrl Pts',(-7.63955181009023,-2.12200304466565,
60.7324306262417));
#62383=CARTESIAN_POINT('Ctrl Pts',(-7.75159859056179,-1.58023555265639,
60.7125347170563));
#62384=CARTESIAN_POINT('Ctrl Pts',(-7.75605225567748,-1.55822928629906,
60.7117244147999));
#62385=CARTESIAN_POINT('Ctrl Pts',(-7.77264979963041,-1.4743838186034,60.7086280011297));
#62386=CARTESIAN_POINT('Ctrl Pts',(-7.78414811008889,-1.41242008826183,
60.7063208648015));
#62387=CARTESIAN_POINT('Ctrl Pts',(-7.82304913145525,-1.18785978239925,
60.6978714139187));
#62388=CARTESIAN_POINT('Ctrl Pts',(-7.84610574756365,-1.02456182892599,
60.6915605515287));
#62389=CARTESIAN_POINT('Ctrl Pts',(-7.86530173113506,-0.849166449993318,
60.6844939711693));
#62390=CARTESIAN_POINT('Ctrl Pts',(-7.86653577003126,-0.837657422644243,
60.6840289553866));
#62391=CARTESIAN_POINT('Ctrl Pts',(-7.86820691086274,-0.821742423902092,
60.6833840392698));
#62392=CARTESIAN_POINT('Ctrl Pts',(-7.86866558248535,-0.817338702194046,
60.6832053898832));
#62393=CARTESIAN_POINT('Ctrl Pts',(-7.86944910333665,-0.809754303624965,
60.682897365482));
#62394=CARTESIAN_POINT('Ctrl Pts',(-7.86977572177094,-0.806573810145947,
60.6827680930296));
#62395=CARTESIAN_POINT('Ctrl Pts',(-7.87042846414609,-0.800179495977349,
60.682507986923));
#62396=CARTESIAN_POINT('Ctrl Pts',(-7.87075454786571,-0.796965671917656,
60.6823771509921));
#62397=CARTESIAN_POINT('Ctrl Pts',(-7.87141047288421,-0.790461323367632,
60.6821121456393));
#62398=CARTESIAN_POINT('Ctrl Pts',(-7.87174021951579,-0.787170790086976,
60.68197797085));
#62399=CARTESIAN_POINT('Ctrl Pts',(-7.87249334917187,-0.779607531207589,
60.6816693218714));
#62400=CARTESIAN_POINT('Ctrl Pts',(-7.8729153168618,-0.77533466894218,60.6814947676637));
#62401=CARTESIAN_POINT('Ctrl Pts',(-7.87399020034538,-0.764358998692847,
60.6810459253921));
#62402=CARTESIAN_POINT('Ctrl Pts',(-7.87463803491731,-0.757655708433056,
60.6807713526263));
#62403=CARTESIAN_POINT('Ctrl Pts',(-7.88013531242262,-0.700005410187424,
60.6784061558521));
#62404=CARTESIAN_POINT('Ctrl Pts',(-7.88449873614315,-0.649014312055114,
60.6762887246058));
#62405=CARTESIAN_POINT('Ctrl Pts',(-7.90336745621056,-0.400106311807902,
60.6658409886551));
#62406=CARTESIAN_POINT('Ctrl Pts',(-7.91091585282024,-0.201746000078963,
60.6571719939765));
#62407=CARTESIAN_POINT('Ctrl Pts',(-7.9109993003797,-0.00332706956333997,
60.6482969704864));
#62408=CARTESIAN_POINT('',(-7.91186981885086,-0.00113476366102863,58.6438367629128));
#62409=CARTESIAN_POINT('Ctrl Pts',(-7.91099918378876,-0.00359361845736577,
60.642331508237));
#62410=CARTESIAN_POINT('Ctrl Pts',(-7.91108682626939,0.189342721609203,
60.6345315316643));
#62411=CARTESIAN_POINT('Ctrl Pts',(-7.90411218664149,0.382554960580305,
60.6267315550916));
#62412=CARTESIAN_POINT('Ctrl Pts',(-7.89004104426854,0.575476602267969,
60.6189315785189));
#62413=CARTESIAN_POINT('Ctrl Pts',(-7.87598390482651,0.768206257523253,
60.6111393641116));
#62414=CARTESIAN_POINT('Ctrl Pts',(-7.85484434960438,0.960645539965939,
60.6033471497042));
#62415=CARTESIAN_POINT('Ctrl Pts',(-7.82664014023985,1.15222615626722,60.5955549352968));
#62416=CARTESIAN_POINT('Ctrl Pts',(-7.79845839522772,1.34365418064785,60.5877689273052));
#62417=CARTESIAN_POINT('Ctrl Pts',(-7.76322325286589,1.53422455125414,60.5799829193136));
#62418=CARTESIAN_POINT('Ctrl Pts',(-7.72100442904379,1.72337216139934,60.572196911322));
#62419=CARTESIAN_POINT('Ctrl Pts',(-7.67881085024431,1.91240666949041,60.564415559025));
#62420=CARTESIAN_POINT('Ctrl Pts',(-7.62964198436513,2.10001976589426,60.5566342067279));
#62421=CARTESIAN_POINT('Ctrl Pts',(-7.57361898674068,2.28565448913021,60.5488528544309));
#62422=CARTESIAN_POINT('Ctrl Pts',(-7.51628015115184,2.47564930066383,60.5408887379263));
#62423=CARTESIAN_POINT('Ctrl Pts',(-7.45176130606158,2.66357128600721,60.5329246214216));
#62424=CARTESIAN_POINT('Ctrl Pts',(-7.38024728606134,2.84883677956182,60.524960504917));
#62425=CARTESIAN_POINT('Ctrl Pts',(-7.31040575065093,3.02976950475864,60.5171826436687));
#62426=CARTESIAN_POINT('Ctrl Pts',(-7.23389272366826,3.20816826221708,60.5094047824205));
#62427=CARTESIAN_POINT('Ctrl Pts',(-7.15093003176425,3.38350715690276,60.5016269211722));
#62428=CARTESIAN_POINT('Ctrl Pts',(-7.06796419635235,3.55885269528798,60.4938487652159));
#62429=CARTESIAN_POINT('Ctrl Pts',(-6.97854836096569,3.73113781844891,60.4860706092596));
#62430=CARTESIAN_POINT('Ctrl Pts',(-6.88295140546018,3.89985909361783,60.4782924533033));
#62431=CARTESIAN_POINT('Ctrl Pts',(-6.78733364526376,4.06861708746637,60.470512604593));
#62432=CARTESIAN_POINT('Ctrl Pts',(-6.68553226124847,4.23380937952657,60.4627327558827));
#62433=CARTESIAN_POINT('Ctrl Pts',(-6.57786080067544,4.39495941812179,60.4549529071724));
#62434=CARTESIAN_POINT('Ctrl Pts',(-6.46571370897935,4.56280805748254,60.4468496697681));
#62435=CARTESIAN_POINT('Ctrl Pts',(-6.34719832698105,4.72627084304187,60.4387464323637));
#62436=CARTESIAN_POINT('Ctrl Pts',(-6.22271668245228,4.88484575907265,60.4306431949594));
#62437=CARTESIAN_POINT('Ctrl Pts',(-6.10302813294028,5.03731483803252,60.4228519681086));
#62438=CARTESIAN_POINT('Ctrl Pts',(-5.97782445659388,5.18526518610947,60.4150607412579));
#62439=CARTESIAN_POINT('Ctrl Pts',(-5.84750177568918,5.32828715285802,60.4072695144071));
#62440=CARTESIAN_POINT('Ctrl Pts',(-5.71709605754416,5.47140024840582,60.399473323248));
#62441=CARTESIAN_POINT('Ctrl Pts',(-5.58156508413715,5.60957845364282,60.3916771320889));
#62442=CARTESIAN_POINT('Ctrl Pts',(-5.44133979553639,5.74245089047456,60.3838809409298));
#62443=CARTESIAN_POINT('Ctrl Pts',(-5.30094395465509,5.87548493650923,60.3760752674712));
#62444=CARTESIAN_POINT('Ctrl Pts',(-5.15584266786037,6.00320010079997,60.3682695940125));
#62445=CARTESIAN_POINT('Ctrl Pts',(-5.00649830228262,6.12526699411881,60.3604639205539));
#62446=CARTESIAN_POINT('Ctrl Pts',(-4.98896078366883,6.13960131738186,60.3595472998094));
#62447=CARTESIAN_POINT('Ctrl Pts',(-4.97136478452658,6.15385780243507,60.3586306790648));
#62448=CARTESIAN_POINT('Ctrl Pts',(-4.95371107754146,6.16803595646483,60.3577140583202));
#62449=CARTESIAN_POINT('Ctrl Pts',(-4.80134554005385,6.29040470661727,60.3498028919835));
#62450=CARTESIAN_POINT('Ctrl Pts',(-4.64423832116536,6.40728886446966,60.3418917256468));
#62451=CARTESIAN_POINT('Ctrl Pts',(-4.48282075010993,6.51830032465396,60.3339805593101));
#62452=CARTESIAN_POINT('Ctrl Pts',(-4.32157815059095,6.6291914519301,60.3260779684272));
#62453=CARTESIAN_POINT('Ctrl Pts',(-4.15603478696332,6.73422236766679,60.3181753775443));
#62454=CARTESIAN_POINT('Ctrl Pts',(-3.98665579704222,6.83304445733449,60.3102727866614));
#62455=CARTESIAN_POINT('Ctrl Pts',(-3.81742896711696,6.93177777112297,60.3023772949955));
#62456=CARTESIAN_POINT('Ctrl Pts',(-3.64437367100339,7.02431319731362,60.2944818033296));
#62457=CARTESIAN_POINT('Ctrl Pts',(-3.46798506006037,7.11034462056503,60.2865863116636));
#62458=CARTESIAN_POINT('Ctrl Pts',(-3.29172217365904,7.19631472318354,60.2786964476687));
#62459=CARTESIAN_POINT('Ctrl Pts',(-3.11213101467736,7.27578990853649,60.2708065836738));
#62460=CARTESIAN_POINT('Ctrl Pts',(-2.92973268421597,7.34850919568294,60.2629167196788));
#62461=CARTESIAN_POINT('Ctrl Pts',(-2.74743052171536,7.42119014220677,60.2550310155473));
#62462=CARTESIAN_POINT('Ctrl Pts',(-2.56232445649966,7.48712216087777,60.2471453114157));
#62463=CARTESIAN_POINT('Ctrl Pts',(-2.37495724374363,7.54609164338664,60.2392596072841));
#62464=CARTESIAN_POINT('Ctrl Pts',(-2.18765406241649,7.60504097348906,60.2313765980365));
#62465=CARTESIAN_POINT('Ctrl Pts',(-1.99809160216031,7.65703240626555,60.223493588789));
#62466=CARTESIAN_POINT('Ctrl Pts',(-1.80682978364659,7.70190152708587,60.2156105795414));
#62467=CARTESIAN_POINT('Ctrl Pts',(-1.61556506466181,7.74677132834302,60.2077274507486));
#62468=CARTESIAN_POINT('Ctrl Pts',(-1.42260126968149,7.78451851484864,60.1998443219558));
#62469=CARTESIAN_POINT('Ctrl Pts',(-1.22851113939037,7.81502919894697,60.1919611931629));
#62470=CARTESIAN_POINT('Ctrl Pts',(-1.03440897909205,7.84554177414482,60.1840775757616));
#62471=CARTESIAN_POINT('Ctrl Pts',(-0.839180685131621,7.86881689901266,
60.1761939583602));
#62472=CARTESIAN_POINT('Ctrl Pts',(-0.643406833433908,7.88479223865097,
60.1683103409589));
#62473=CARTESIAN_POINT('Ctrl Pts',(-0.447587938824595,7.90077125383535,
60.1604249097245));
#62474=CARTESIAN_POINT('Ctrl Pts',(-0.251223580167572,7.90944710905219,
60.15253947849));
#62475=CARTESIAN_POINT('Ctrl Pts',(-0.054897316110019,7.91080952145126,
60.1446540472556));
#62476=CARTESIAN_POINT('Ctrl Pts',(0.141507119782876,7.91217247632628,60.1367654762547));
#62477=CARTESIAN_POINT('Ctrl Pts',(0.337873086207642,7.90621618352908,60.1288769052538));
#62478=CARTESIAN_POINT('Ctrl Pts',(0.533618919363395,7.89298244321482,60.1209883342528));
#62479=CARTESIAN_POINT('Ctrl Pts',(0.729573112571408,7.87973461635385,60.113091366327));
#62480=CARTESIAN_POINT('Ctrl Pts',(0.92490550979953,7.85919389251085,60.1051943984011));
#62481=CARTESIAN_POINT('Ctrl Pts',(1.11904034249819,7.83145386961205,60.0972974304752));
#62482=CARTESIAN_POINT('Ctrl Pts',(1.31329359668001,7.80369692540856,60.0893956454301));
#62483=CARTESIAN_POINT('Ctrl Pts',(1.50634749149054,7.76873198829577,60.0814938603849));
#62484=CARTESIAN_POINT('Ctrl Pts',(1.69763803616429,7.72670344313591,60.0735920753397));
#62485=CARTESIAN_POINT('Ctrl Pts',(1.88917602195545,7.68462053255931,60.0656800690547));
#62486=CARTESIAN_POINT('Ctrl Pts',(2.07894576880726,7.63545584984425,60.0577680627698));
#62487=CARTESIAN_POINT('Ctrl Pts',(2.26639889844067,7.57940347475624,60.0498560564848));
#62488=CARTESIAN_POINT('Ctrl Pts',(2.34493975122494,7.55591813018714,60.0465410106274));
#62489=CARTESIAN_POINT('Ctrl Pts',(2.42307415975829,7.53122421861491,60.04322596477));
#62490=CARTESIAN_POINT('Ctrl Pts',(2.50076292126058,7.50533848747998,60.0399109189125));
#62491=CARTESIAN_POINT('Ctrl Pts',(2.68450289825263,7.44411671548642,60.0320705770433));
#62492=CARTESIAN_POINT('Ctrl Pts',(2.86626968753469,7.37605151947719,60.0242302351742));
#62493=CARTESIAN_POINT('Ctrl Pts',(3.04551022817515,7.3012867667337,60.016389893305));
#62494=CARTESIAN_POINT('Ctrl Pts',(3.22455037255659,7.22660560320893,60.0085583171713));
#62495=CARTESIAN_POINT('Ctrl Pts',(3.40106957125277,7.14523993174107,60.0007267410377));
#62496=CARTESIAN_POINT('Ctrl Pts',(3.57452900934866,7.05738360593534,59.992895164904));
#62497=CARTESIAN_POINT('Ctrl Pts',(3.74782824265011,6.96960842304562,59.9850708219083));
#62498=CARTESIAN_POINT('Ctrl Pts',(3.91807303175677,6.87535468175213,59.9772464789126));
#62499=CARTESIAN_POINT('Ctrl Pts',(4.08474349608296,6.77486469025087,59.969422135917));
#62500=CARTESIAN_POINT('Ctrl Pts',(4.25129241672361,6.67444798062336,59.9616034987882));
#62501=CARTESIAN_POINT('Ctrl Pts',(4.41427190443657,6.56780425941505,59.9537848616594));
#62502=CARTESIAN_POINT('Ctrl Pts',(4.57318553252301,6.45522231105345,59.9459662245306));
#62503=CARTESIAN_POINT('Ctrl Pts',(4.73201414592293,6.3427005911264,59.9381517701707));
#62504=CARTESIAN_POINT('Ctrl Pts',(4.88678094648591,6.22424717507849,59.9303373158108));
#62505=CARTESIAN_POINT('Ctrl Pts',(5.03701726940283,6.10019491719221,59.9225228614509));
#62506=CARTESIAN_POINT('Ctrl Pts',(5.18720239934277,5.97618493007147,59.9147110698637));
#62507=CARTESIAN_POINT('Ctrl Pts',(5.33285985672674,5.84658012593787,59.9068992782766));
#62508=CARTESIAN_POINT('Ctrl Pts',(5.47355279435779,5.71175461722386,59.8990874866894));
#62509=CARTESIAN_POINT('Ctrl Pts',(5.61425231664508,5.57692279845872,59.8912753294978));
#62510=CARTESIAN_POINT('Ctrl Pts',(5.74998659478077,5.43687002364502,59.8834631723062));
#62511=CARTESIAN_POINT('Ctrl Pts',(5.88035413514493,5.29200871553363,59.8756510151146));
#62512=CARTESIAN_POINT('Ctrl Pts',(6.01073233317344,5.14713556487927,59.8678382192721));
#62513=CARTESIAN_POINT('Ctrl Pts',(6.13574268345728,4.9974533588667,59.8600254234296));
#62514=CARTESIAN_POINT('Ctrl Pts',(6.25502270872204,4.84340912099851,59.8522126275871));
#62515=CARTESIAN_POINT('Ctrl Pts',(6.37433347358118,4.68932518446848,59.8443978183129));
#62516=CARTESIAN_POINT('Ctrl Pts',(6.48791075613094,4.53087725474849,59.8365830090388));
#62517=CARTESIAN_POINT('Ctrl Pts',(6.59543420639039,4.36854307855326,59.8287681997647));
#62518=CARTESIAN_POINT('Ctrl Pts',(6.70300428775412,4.20613850076768,59.8209500013397));
#62519=CARTESIAN_POINT('Ctrl Pts',(6.80451511277483,4.03984461203916,59.8131318029148));
#62520=CARTESIAN_POINT('Ctrl Pts',(6.89969117463817,3.87016571927097,59.8053136044899));
#62521=CARTESIAN_POINT('Ctrl Pts',(6.99497802092188,3.70028932119088,59.7974863057243));
#62522=CARTESIAN_POINT('Ctrl Pts',(7.0839152048176,3.5270203563457,59.7896590069588));
#62523=CARTESIAN_POINT('Ctrl Pts',(7.16627399083047,3.35088616463567,59.7818317081933));
#62524=CARTESIAN_POINT('Ctrl Pts',(7.24868654099437,3.17463699180775,59.7739992997352));
#62525=CARTESIAN_POINT('Ctrl Pts',(7.32451199867448,2.9955191873616,59.7661668912772));
#62526=CARTESIAN_POINT('Ctrl Pts',(7.39357079451981,2.81407745210109,59.7583344828191));
#62527=CARTESIAN_POINT('Ctrl Pts',(7.46272869946862,2.63237532238254,59.7504908337512));
#62528=CARTESIAN_POINT('Ctrl Pts',(7.52510043433205,2.44834293229416,59.7426471846833));
#62529=CARTESIAN_POINT('Ctrl Pts',(7.58055672223744,2.26253857004489,59.7348035356154));
#62530=CARTESIAN_POINT('Ctrl Pts',(7.6104772987424,2.16229071997026,59.7305716169119));
#62531=CARTESIAN_POINT('Ctrl Pts',(7.63838569171401,2.06152721563189,59.7263396982084));
#62532=CARTESIAN_POINT('Ctrl Pts',(7.66426784507321,1.96033655247686,59.7221077795048));
#62533=CARTESIAN_POINT('Ctrl Pts',(7.71269233422802,1.77101280871747,59.714190026352));
#62534=CARTESIAN_POINT('Ctrl Pts',(7.75416568177515,1.57962758394762,59.7062722731992));
#62535=CARTESIAN_POINT('Ctrl Pts',(7.7885102267516,1.38673337299777,59.6983545200463));
#62536=CARTESIAN_POINT('Ctrl Pts',(7.82281531231705,1.19406078361706,59.6904458638221));
#62537=CARTESIAN_POINT('Ctrl Pts',(7.8500078495628,0.999882997071532,59.6825372075979));
#62538=CARTESIAN_POINT('Ctrl Pts',(7.86996001785461,0.80476724422025,59.6746285513738));
#62539=CARTESIAN_POINT('Ctrl Pts',(7.8898929559655,0.609839546680698,59.6667275176239));
#62540=CARTESIAN_POINT('Ctrl Pts',(7.90259939169801,0.413976023955987,59.658826483874));
#62541=CARTESIAN_POINT('Ctrl Pts',(7.90800254266134,0.217753955788902,59.6509254501241));
#62542=CARTESIAN_POINT('Ctrl Pts',(7.91340148584017,0.0216846984879661,
59.6430305694223));
#62543=CARTESIAN_POINT('Ctrl Pts',(7.91150846620884,-0.174742205258469,
59.6351356887204));
#62544=CARTESIAN_POINT('Ctrl Pts',(7.90229848811574,-0.370944207022699,
59.6272408080186));
#62545=CARTESIAN_POINT('Ctrl Pts',(7.89309397856442,-0.567029711349835,
59.6193506150027));
#62546=CARTESIAN_POINT('Ctrl Pts',(7.87658118360316,-0.762890236703942,
59.6114604219868));
#62547=CARTESIAN_POINT('Ctrl Pts',(7.8527871867078,-0.957942795931853,59.6035702289709));
#62548=CARTESIAN_POINT('Ctrl Pts',(7.8290029166758,-1.15291561867838,59.5956832614253));
#62549=CARTESIAN_POINT('Ctrl Pts',(7.79794341847744,-1.34708079217972,59.5877962938796));
#62550=CARTESIAN_POINT('Ctrl Pts',(7.75968768845748,-1.53985972659895,59.579909326334));
#62551=CARTESIAN_POINT('Ctrl Pts',(7.72143528068662,-1.73262191948324,59.5720230437177));
#62552=CARTESIAN_POINT('Ctrl Pts',(7.67598794689021,-1.92399777416498,59.5641367611014));
#62553=CARTESIAN_POINT('Ctrl Pts',(7.62347603004193,-2.11341766325923,59.556250478485));
#62554=CARTESIAN_POINT('Ctrl Pts',(7.5709642054908,-2.30283721942114,59.54836420973));
#62555=CARTESIAN_POINT('Ctrl Pts',(7.5113879141532,-2.49030048463943,59.5404779409749));
#62556=CARTESIAN_POINT('Ctrl Pts',(7.44492776239345,-2.67525169147563,59.5325916722198));
#62557=CARTESIAN_POINT('Ctrl Pts',(7.37845658837979,-2.86023357201797,59.5247040955463));
#62558=CARTESIAN_POINT('Ctrl Pts',(7.30509939563164,-3.04270223978297,59.5168165188729));
#62559=CARTESIAN_POINT('Ctrl Pts',(7.22508553692539,-3.22212041738224,59.5089289421994));
#62560=CARTESIAN_POINT('Ctrl Pts',(7.14504499732114,-3.40159842259356,59.5010387353862));
#62561=CARTESIAN_POINT('Ctrl Pts',(7.05834350931513,-3.57802359641537,59.493148528573));
#62562=CARTESIAN_POINT('Ctrl Pts',(6.96525721812272,-3.75088161441937,59.4852583217598));
#62563=CARTESIAN_POINT('Ctrl Pts',(6.87208103710106,-3.92390655472229,59.4773604956791));
#62564=CARTESIAN_POINT('Ctrl Pts',(6.77250790116481,-4.09335715532156,59.4694626695985));
#62565=CARTESIAN_POINT('Ctrl Pts',(6.66685883195437,-4.25874562691786,59.4615648435179));
#62566=CARTESIAN_POINT('Ctrl Pts',(6.56115126285717,-4.4242256772373,59.4536626442617));
#62567=CARTESIAN_POINT('Ctrl Pts',(6.44936124829765,-4.58563883126795,59.4457604450055));
#62568=CARTESIAN_POINT('Ctrl Pts',(6.33185140915414,-4.74252872762967,59.4378582457493));
#62569=CARTESIAN_POINT('Ctrl Pts',(6.21419972672546,-4.89960800199133,59.4299465079395));
#62570=CARTESIAN_POINT('Ctrl Pts',(6.09081464487292,-5.05215284559114,59.4220347701297));
#62571=CARTESIAN_POINT('Ctrl Pts',(5.96209779950831,-5.1997414194456,59.4141230323198));
#62572=CARTESIAN_POINT('Ctrl Pts',(5.90885233461222,-5.26079343020591,59.4108502349122));
#62573=CARTESIAN_POINT('Ctrl Pts',(5.85469493588517,-5.32099778462534,59.4075774375047));
#62574=CARTESIAN_POINT('Ctrl Pts',(5.79965576047404,-5.38032657559002,59.4043046400971));
#62575=CARTESIAN_POINT('Ctrl Pts',(5.65982344722424,-5.53105706929629,59.3959897838355));
#62576=CARTESIAN_POINT('Ctrl Pts',(5.5139920804601,-5.67646244899675,59.387674927574));
#62577=CARTESIAN_POINT('Ctrl Pts',(5.36258350565656,-5.81606560699415,59.3793600713124));
#62578=CARTESIAN_POINT('Ctrl Pts',(5.21136138525026,-5.95549684855477,59.3710554545073));
#62579=CARTESIAN_POINT('Ctrl Pts',(5.05457596951866,-6.08913992139619,59.3627508377022));
#62580=CARTESIAN_POINT('Ctrl Pts',(4.8926869871892,-6.2165533091408,59.3544462208971));
#62581=CARTESIAN_POINT('Ctrl Pts',(4.73098668713763,-6.34381819605548,59.3461512831572));
#62582=CARTESIAN_POINT('Ctrl Pts',(4.56419491403394,-6.46486769894665,59.3378563454173));
#62583=CARTESIAN_POINT('Ctrl Pts',(4.39280624966499,-6.57929891803863,59.3295614076774));
#62584=CARTESIAN_POINT('Ctrl Pts',(4.22167446503814,-6.69355862600904,59.3212789025069));
#62585=CARTESIAN_POINT('Ctrl Pts',(4.04595978210803,-6.80121968385556,59.3129963973365));
#62586=CARTESIAN_POINT('Ctrl Pts',(3.86618772683885,-6.90192099787013,59.304713892166));
#62587=CARTESIAN_POINT('Ctrl Pts',(3.68658081780607,-7.00252980338562,59.2964389956562));
#62588=CARTESIAN_POINT('Ctrl Pts',(3.50292422415731,-7.0961914719479,59.2881640991463));
#62589=CARTESIAN_POINT('Ctrl Pts',(3.31577171043993,-7.18258859773037,59.2798892026364));
#62590=CARTESIAN_POINT('Ctrl Pts',(3.12883327465321,-7.26888689653191,59.2716237715229));
#62591=CARTESIAN_POINT('Ctrl Pts',(2.93840716391858,-7.34793711142126,59.2633583404094));
#62592=CARTESIAN_POINT('Ctrl Pts',(2.74507121305907,-7.41946797521456,59.2550929092959));
#62593=CARTESIAN_POINT('Ctrl Pts',(2.66951983156124,-7.44742064286531,59.2518629629951));
#62594=CARTESIAN_POINT('Ctrl Pts',(2.59352435622807,-7.4742255494801,59.2486330166942));
#62595=CARTESIAN_POINT('Ctrl Pts',(2.51712021785742,-7.49986845276992,59.2454030703934));
#62596=CARTESIAN_POINT('Ctrl Pts',(2.32157511884167,-7.56549767351361,59.2371365002483));
#62597=CARTESIAN_POINT('Ctrl Pts',(2.12357222812108,-7.62343805701521,59.2288699301033));
#62598=CARTESIAN_POINT('Ctrl Pts',(1.9237325732266,-7.67353725388148,59.2206033599582));
#62599=CARTESIAN_POINT('Ctrl Pts',(1.72371385968645,-7.72368134020848,59.2123293828705));
#62600=CARTESIAN_POINT('Ctrl Pts',(1.52185538124776,-7.76597014237096,59.2040554057828));
#62601=CARTESIAN_POINT('Ctrl Pts',(1.3187880454904,-7.80030249997214,59.1957814286951));
#62602=CARTESIAN_POINT('Ctrl Pts',(1.11552557817975,-7.83466784823743,59.1874995009738));
#62603=CARTESIAN_POINT('Ctrl Pts',(0.91105222372173,-7.86106143930347,59.1792175732524));
#62604=CARTESIAN_POINT('Ctrl Pts',(0.706004523238845,-7.87943390182101,
59.170935645531));
#62605=CARTESIAN_POINT('Ctrl Pts',(0.500616932063557,-7.89783681885714,
59.1626399895399));
#62606=CARTESIAN_POINT('Ctrl Pts',(0.294653384464272,-7.90819199911998,
59.1543443335488));
#62607=CARTESIAN_POINT('Ctrl Pts',(0.0887529832293941,-7.91050212742326,
59.1460486775576));
#62608=CARTESIAN_POINT('Ctrl Pts',(-0.11733351212049,-7.91281434363545,
59.1377455238989));
#62609=CARTESIAN_POINT('Ctrl Pts',(-0.323356453953252,-7.9070669972986,
59.1294423702402));
#62610=CARTESIAN_POINT('Ctrl Pts',(-0.528680035056985,-7.89331479294549,
59.1211392165815));
#62611=CARTESIAN_POINT('Ctrl Pts',(-0.734316660042689,-7.87954162147593,
59.1128234036294));
#62612=CARTESIAN_POINT('Ctrl Pts',(-0.939251500532301,-7.85773922317631,
59.1045075906773));
#62613=CARTESIAN_POINT('Ctrl Pts',(-1.14285525923557,-7.82801397906503,
59.0961917777252));
#62614=CARTESIAN_POINT('Ctrl Pts',(-1.22194060497823,-7.8164678699814,59.09296168538));
#62615=CARTESIAN_POINT('Ctrl Pts',(-1.30082524599181,-7.80372693627788,
59.0897315930347));
#62616=CARTESIAN_POINT('Ctrl Pts',(-1.37947282804922,-7.78979946575481,
59.0865015006895));
#62617=CARTESIAN_POINT('Ctrl Pts',(-1.57209219270116,-7.75568906524173,
59.0785905348463));
#62618=CARTESIAN_POINT('Ctrl Pts',(-1.76368872443122,-7.71438698870522,
59.0706795690031));
#62619=CARTESIAN_POINT('Ctrl Pts',(-1.9536858869878,-7.6659658527145,59.0627686031599));
#62620=CARTESIAN_POINT('Ctrl Pts',(-2.14349078997446,-7.61759371443856,
59.0548656424831));
#62621=CARTESIAN_POINT('Ctrl Pts',(-2.3316992164698,-7.56211695071439,59.0469626818062));
#62622=CARTESIAN_POINT('Ctrl Pts',(-2.51774246360124,-7.49965958473978,
59.0390597211294));
#62623=CARTESIAN_POINT('Ctrl Pts',(-2.70363188161947,-7.43725386138789,
59.0311632949839));
#62624=CARTESIAN_POINT('Ctrl Pts',(-2.88735936205729,-7.36787914342932,
59.0232668688384));
#62625=CARTESIAN_POINT('Ctrl Pts',(-3.0683687865582,-7.29170994963975,59.0153704426929));
#62626=CARTESIAN_POINT('Ctrl Pts',(-3.24926203291897,-7.21558964388623,
59.0074790847482));
#62627=CARTESIAN_POINT('Ctrl Pts',(-3.4274403828353,-7.13268368430048,58.9995877268034));
#62628=CARTESIAN_POINT('Ctrl Pts',(-3.60236494652799,-7.04321572806246,
58.9916963688587));
#62629=CARTESIAN_POINT('Ctrl Pts',(-3.77720959417117,-6.95378864616175,
58.9838086161604));
#62630=CARTESIAN_POINT('Ctrl Pts',(-3.94880311176592,-6.85780569820013,
58.975920863462));
#62631=CARTESIAN_POINT('Ctrl Pts',(-4.11662833311003,-6.75553788880173,
58.9680331107637));
#62632=CARTESIAN_POINT('Ctrl Pts',(-4.28440792071733,-6.65329788727548,
58.9601475028421));
#62633=CARTESIAN_POINT('Ctrl Pts',(-4.44842096051296,-6.54477660959954,
58.9522618949205));
#62634=CARTESIAN_POINT('Ctrl Pts',(-4.60817631522549,-6.43029019934519,
58.9443762869989));
#62635=CARTESIAN_POINT('Ctrl Pts',(-4.76795051169629,-6.31579028641188,
58.9364897490382));
#62636=CARTESIAN_POINT('Ctrl Pts',(-4.92346573571054,-6.19532403030867,
58.9286032110776));
#62637=CARTESIAN_POINT('Ctrl Pts',(-5.07426067561686,-6.06925033228062,
58.9207166731169));
#62638=CARTESIAN_POINT('Ctrl Pts',(-5.22507461283565,-5.94316075134934,
58.9128291416015));
#62639=CARTESIAN_POINT('Ctrl Pts',(-5.37116681609724,-5.81146254138928,
58.9049416100861));
#62640=CARTESIAN_POINT('Ctrl Pts',(-5.51210988437816,-5.67455422236325,
58.8970540785707));
#62641=CARTESIAN_POINT('Ctrl Pts',(-5.65309433250902,-5.53760570806003,
58.889164231334));
#62642=CARTESIAN_POINT('Ctrl Pts',(-5.7889263859168,-5.39544427648208,58.8812743840973));
#62643=CARTESIAN_POINT('Ctrl Pts',(-5.91921609724654,-5.24850471983187,
58.8733845368605));
#62644=CARTESIAN_POINT('Ctrl Pts',(-6.04956589922947,-5.10149739348712,
58.8654910507634));
#62645=CARTESIAN_POINT('Ctrl Pts',(-6.17436803699042,-4.9497078081706,58.8575975646663));
#62646=CARTESIAN_POINT('Ctrl Pts',(-6.29327322210822,-4.79360335779836,
58.8497040785691));
#62647=CARTESIAN_POINT('Ctrl Pts',(-6.41231586145556,-4.63731845089738,
58.841801467613));
#62648=CARTESIAN_POINT('Ctrl Pts',(-6.52544772314626,-4.47670898990953,
58.8338988566568));
#62649=CARTESIAN_POINT('Ctrl Pts',(-6.63236254373327,-4.31227180132282,
58.8259962457006));
#62650=CARTESIAN_POINT('Ctrl Pts',(-6.73934827605431,-4.14772554903365,
58.8180883933023));
#62651=CARTESIAN_POINT('Ctrl Pts',(-6.84010857048051,-3.97934680260961,
58.810180540904));
#62652=CARTESIAN_POINT('Ctrl Pts',(-6.93438330255126,-3.8076566564356,58.8022726885057));
#62653=CARTESIAN_POINT('Ctrl Pts',(-7.02878702919564,-3.63573158944329,
58.7943540159223));
#62654=CARTESIAN_POINT('Ctrl Pts',(-7.11668731464863,-3.46048637948607,
58.786435343339));
#62655=CARTESIAN_POINT('Ctrl Pts',(-7.19787183142198,-3.28246280990692,
58.7785166707556));
#62656=CARTESIAN_POINT('Ctrl Pts',(-7.23142521223477,-3.20888606324205,
58.775243900931));
#62657=CARTESIAN_POINT('Ctrl Pts',(-7.2638320247923,-3.13483492169906,58.7719711311064));
#62658=CARTESIAN_POINT('Ctrl Pts',(-7.29507977676371,-3.06034835446117,
58.7686983612817));
#62659=CARTESIAN_POINT('Ctrl Pts',(-7.37856743028714,-2.86133535911363,
58.7599541843109));
#62660=CARTESIAN_POINT('Ctrl Pts',(-7.4539897791399,-2.6587079227428,58.75121000734));
#62661=CARTESIAN_POINT('Ctrl Pts',(-7.52105080707951,-2.45310329120661,
58.7424658303692));
#62662=CARTESIAN_POINT('Ctrl Pts',(-7.58782306424936,-2.24838401155866,
58.7337593066045));
#62663=CARTESIAN_POINT('Ctrl Pts',(-7.64630574341749,-2.04071331339552,
58.7250527828399));
#62664=CARTESIAN_POINT('Ctrl Pts',(-7.69625194727979,-1.83074492051518,
58.7163462590753));
#62665=CARTESIAN_POINT('Ctrl Pts',(-7.74606533383241,-1.6213348771169,58.7076628877621));
#62666=CARTESIAN_POINT('Ctrl Pts',(-7.78738746955122,-1.40963953497845,
58.698979516449));
#62667=CARTESIAN_POINT('Ctrl Pts',(-7.82002030366252,-1.19632915633863,
58.6902961451359));
#62668=CARTESIAN_POINT('Ctrl Pts',(-7.85250523590745,-0.983985564800771,
58.6816521294858));
#62669=CARTESIAN_POINT('Ctrl Pts',(-7.87637936152144,-0.770041747798524,
58.6730081138357));
#62670=CARTESIAN_POINT('Ctrl Pts',(-7.89149535562621,-0.555177496058689,
58.6643640981856));
#62671=CARTESIAN_POINT('Ctrl Pts',(-7.90433832557822,-0.372622838407328,
58.6570199015361));
#62672=CARTESIAN_POINT('Ctrl Pts',(-7.91085984755608,-0.189404127067722,
58.6496757048866));
#62673=CARTESIAN_POINT('Ctrl Pts',(-7.91099776453137,-0.00594723293680172,
58.642331508237));
#62674=CARTESIAN_POINT('',(-7.911,4.9293902293357E-13,56.642331508237));
#62675=CARTESIAN_POINT('Ctrl Pts',(-7.911,6.63358257213531E-13,58.642331508237));
#62676=CARTESIAN_POINT('Ctrl Pts',(-7.91099999999982,2.20167589666731,58.5537440725043));
#62677=CARTESIAN_POINT('Ctrl Pts',(-6.94214576672346,4.38610418338718,58.4651566367716));
#62678=CARTESIAN_POINT('Ctrl Pts',(-3.67820201488267,7.34180684107638,58.2879817653061));
#62679=CARTESIAN_POINT('Ctrl Pts',(-1.40868175871738,8.08992666571334,58.1993943295734));
#62680=CARTESIAN_POINT('Ctrl Pts',(2.97309270521256,7.6545422802526,58.022219458108));
#62681=CARTESIAN_POINT('Ctrl Pts',(5.05102072675575,6.47444880834243,57.9336320223752));
#62682=CARTESIAN_POINT('Ctrl Pts',(7.66951518847849,2.93425195367758,57.7564571509098));
#62683=CARTESIAN_POINT('Ctrl Pts',(8.18956872247063,0.601881960099865,57.6678697151771));
#62684=CARTESIAN_POINT('Ctrl Pts',(7.32306689761382,-3.71537198232365,57.4906948437116));
#62685=CARTESIAN_POINT('Ctrl Pts',(5.94329958850274,-5.6664351893643,57.4021074079789));
#62686=CARTESIAN_POINT('Ctrl Pts',(2.16154501637974,-7.9220591323296,57.2249325365135));
#62687=CARTESIAN_POINT('Ctrl Pts',(-0.210816529298906,-8.20894963713003,
57.1363451007807));
#62688=CARTESIAN_POINT('Ctrl Pts',(-4.42123908576293,-6.9198224471792,56.9591702293153));
#62689=CARTESIAN_POINT('Ctrl Pts',(-6.22631625634065,-5.35390358803658,
56.8705827935826));
#62690=CARTESIAN_POINT('Ctrl Pts',(-7.65317280859467,-2.31334857514629,
56.7354407413122));
#62691=CARTESIAN_POINT('Ctrl Pts',(-7.91100000000007,-1.15702837836549,
56.6888861247746));
#62692=CARTESIAN_POINT('Ctrl Pts',(-7.911,4.9293902293357E-13,56.642331508237));
#62693=CARTESIAN_POINT('',(-7.911,1.51545442861334E-13,52.642331508237));
#62694=CARTESIAN_POINT('Ctrl Pts',(-7.91099980728415,0.00174618159620388,
56.6387979549077));
#62695=CARTESIAN_POINT('Ctrl Pts',(-7.91084820449805,0.68857601317406,56.6151031213445));
#62696=CARTESIAN_POINT('Ctrl Pts',(-7.82125530223842,1.37238516702683,56.5930307210947));
#62697=CARTESIAN_POINT('Ctrl Pts',(-7.61840630808201,2.1340358358552,56.5631137361859));
#62698=CARTESIAN_POINT('Ctrl Pts',(-7.59039980943151,2.23160318732258,56.5591722855295));
#62699=CARTESIAN_POINT('Ctrl Pts',(-7.55535200479549,2.34539675655594,56.5544191086037));
#62700=CARTESIAN_POINT('Ctrl Pts',(-7.55012304885116,2.36217522631301,56.5537142523069));
#62701=CARTESIAN_POINT('Ctrl Pts',(-7.54316836291411,2.38423213767859,56.5527821986768));
#62702=CARTESIAN_POINT('Ctrl Pts',(-7.54149288624599,2.38952649786587,56.5525580620559));
#62703=CARTESIAN_POINT('Ctrl Pts',(-7.53874602785033,2.39817466492789,56.5521912589115));
#62704=CARTESIAN_POINT('Ctrl Pts',(-7.5376779778534,2.40152953304869,56.5520487973686));
#62705=CARTESIAN_POINT('Ctrl Pts',(-7.5356043339553,2.4080280762334,56.5517725153031));
#62706=CARTESIAN_POINT('Ctrl Pts',(-7.53459901537137,2.41117182534847,56.551638712335));
#62707=CARTESIAN_POINT('Ctrl Pts',(-7.53226961020979,2.41844046589533,56.5513290063651));
#62708=CARTESIAN_POINT('Ctrl Pts',(-7.53094410322701,2.42256489736126,56.5511530163397));
#62709=CARTESIAN_POINT('Ctrl Pts',(-7.52737283904243,2.43364594385742,56.550679507872));
#62710=CARTESIAN_POINT('Ctrl Pts',(-7.52512083150402,2.44060052211482,56.5503816097484));
#62711=CARTESIAN_POINT('Ctrl Pts',(-7.50915335961539,2.48967855821255,56.5482743345795));
#62712=CARTESIAN_POINT('Ctrl Pts',(-7.4950941684472,2.5316885195273,56.5464443878642));
#62713=CARTESIAN_POINT('Ctrl Pts',(-7.22814463990183,3.3076375383237,56.5121901198727));
#62714=CARTESIAN_POINT('Ctrl Pts',(-6.86894496350255,4.00052861050787,56.4745166261569));
#62715=CARTESIAN_POINT('Ctrl Pts',(-6.33139272484424,4.74527014589443,56.4329966167731));
#62716=CARTESIAN_POINT('Ctrl Pts',(-6.24511494801689,4.85825731680045,56.426648399571));
#62717=CARTESIAN_POINT('Ctrl Pts',(-6.02994215817876,5.12483117511727,56.4115888345783));
#62718=CARTESIAN_POINT('Ctrl Pts',(-5.89815979262237,5.27596586528857,56.4029831231325));
#62719=CARTESIAN_POINT('Ctrl Pts',(-5.68150113490863,5.50616413561056,56.3897890670311));
#62720=CARTESIAN_POINT('Ctrl Pts',(-5.60039079547315,5.58864233171825,56.3850422023488));
#62721=CARTESIAN_POINT('Ctrl Pts',(-5.50942505051269,5.6771721421646,56.3799224421398));
#62722=CARTESIAN_POINT('Ctrl Pts',(-5.50133474165043,5.6850122234436,56.3794688224971));
#62723=CARTESIAN_POINT('Ctrl Pts',(-5.48797801151744,5.69790062783065,56.3787227404949));
#62724=CARTESIAN_POINT('Ctrl Pts',(-5.48272131887853,5.70295898279377,56.378429828522));
#62725=CARTESIAN_POINT('Ctrl Pts',(-5.4733390843291,5.71196225916846,56.3779083084703));
#62726=CARTESIAN_POINT('Ctrl Pts',(-5.46921625872517,5.71590999734119,56.3776795745311));
#62727=CARTESIAN_POINT('Ctrl Pts',(-5.46122648705428,5.72354390199454,56.3772371469045));
#62728=CARTESIAN_POINT('Ctrl Pts',(-5.45736007406763,5.72723061898702,56.3770234287103));
#62729=CARTESIAN_POINT('Ctrl Pts',(-5.44942715339064,5.7347795208465,56.376585712194));
#62730=CARTESIAN_POINT('Ctrl Pts',(-5.44536026712633,5.73864130384497,56.376361731779));
#62731=CARTESIAN_POINT('Ctrl Pts',(-5.43562095466984,5.74786976319059,56.3758263472073));
#62732=CARTESIAN_POINT('Ctrl Pts',(-5.42994467687421,5.75323237702149,56.3755151233153));
#62733=CARTESIAN_POINT('Ctrl Pts',(-5.4095039470628,5.77248637984806,56.3743972821306));
#62734=CARTESIAN_POINT('Ctrl Pts',(-5.39469399256677,5.78632946637346,56.3735928002347));
#62735=CARTESIAN_POINT('Ctrl Pts',(-5.18158927956634,5.98399230869551,56.3620939646881));
#62736=CARTESIAN_POINT('Ctrl Pts',(-4.97404324807321,6.1575921851026,56.3518575389367));
#62737=CARTESIAN_POINT('Ctrl Pts',(-4.65321842494282,6.3991156360056,56.3371904487959));
#62738=CARTESIAN_POINT('Ctrl Pts',(-4.54648912519221,6.47538112010362,56.3324853777765));
#62739=CARTESIAN_POINT('Ctrl Pts',(-4.31160821998684,6.63454846901163,56.3224457912904));
#62740=CARTESIAN_POINT('Ctrl Pts',(-4.18285442050865,6.71646701018821,56.3171362598408));
#62741=CARTESIAN_POINT('Ctrl Pts',(-3.94581484207716,6.85782010059937,56.307614806393));
#62742=CARTESIAN_POINT('Ctrl Pts',(-3.8383543163265,6.91853942024402,56.3033881959249));
#62743=CARTESIAN_POINT('Ctrl Pts',(-3.5156802167663,7.09103000341992,56.2908673393033));
#62744=CARTESIAN_POINT('Ctrl Pts',(-3.29670491068004,7.19544623343171,56.2825924325451));
#62745=CARTESIAN_POINT('Ctrl Pts',(-2.858419944565,7.38022555928906,56.2659118569252));
#62746=CARTESIAN_POINT('Ctrl Pts',(-2.6396655276265,7.46126317552849,56.2575302895396));
#62747=CARTESIAN_POINT('Ctrl Pts',(-2.319361546293,7.56406915329006,56.2447726794681));
#62748=CARTESIAN_POINT('Ctrl Pts',(-2.22045331329989,7.59369248779834,56.2407678726379));
#62749=CARTESIAN_POINT('Ctrl Pts',(-2.10383913719518,7.62614575653695,56.2359400614301));
#62750=CARTESIAN_POINT('Ctrl Pts',(-2.08666471780555,7.63086289753016,56.2352263638029));
#62751=CARTESIAN_POINT('Ctrl Pts',(-2.0640349636981,7.63699629647951,56.2342822679548));
#62752=CARTESIAN_POINT('Ctrl Pts',(-2.05859375640707,7.63846480057348,56.2340549831037));
#62753=CARTESIAN_POINT('Ctrl Pts',(-2.049651950738,7.64086781773522,56.233681010764));
#62754=CARTESIAN_POINT('Ctrl Pts',(-2.04615230225382,7.64180573445595,56.2335345290203));
#62755=CARTESIAN_POINT('Ctrl Pts',(-2.03935960652088,7.64362119741479,56.2332499892446));
#62756=CARTESIAN_POINT('Ctrl Pts',(-2.03606663342336,7.64449902076446,56.2331119476084));
#62757=CARTESIAN_POINT('Ctrl Pts',(-2.02844902415641,7.64652441151045,56.2327923827668));
#62758=CARTESIAN_POINT('Ctrl Pts',(-2.02412398308849,7.64767043748335,56.2326107693108));
#62759=CARTESIAN_POINT('Ctrl Pts',(-2.01022576107042,7.65134049733844,56.2320266119199));
#62760=CARTESIAN_POINT('Ctrl Pts',(-2.00064884565773,7.6538502213843,56.2316232380672));
#62761=CARTESIAN_POINT('Ctrl Pts',(-1.91442021617504,7.67627437698169,56.2279838990482));
#62762=CARTESIAN_POINT('Ctrl Pts',(-1.83748052196763,7.69505410092623,56.2246837374486));
#62763=CARTESIAN_POINT('Ctrl Pts',(-1.08233639329698,7.86740167957996,56.1918690604129));
#62764=CARTESIAN_POINT('Ctrl Pts',(-0.386971163054789,7.93206985564289,
56.1586017557931));
#62765=CARTESIAN_POINT('Ctrl Pts',(0.540843078214959,7.8959332211934,56.1164228042473));
#62766=CARTESIAN_POINT('Ctrl Pts',(0.77329510403888,7.87656632993453,56.1060100791956));
#62767=CARTESIAN_POINT('Ctrl Pts',(1.19459226643754,7.82263211511709,56.0875430221281));
#62768=CARTESIAN_POINT('Ctrl Pts',(1.38368227988135,7.7914089784371,56.0794042934287));
#62769=CARTESIAN_POINT('Ctrl Pts',(1.65828317213273,7.7357524261427,56.0678137934268));
#62770=CARTESIAN_POINT('Ctrl Pts',(1.74480491738745,7.71669781337492,56.0641951087904));
#62771=CARTESIAN_POINT('Ctrl Pts',(1.84493711061928,7.69287550797246,56.0600442287473));
#62772=CARTESIAN_POINT('Ctrl Pts',(1.8588749301217,7.68951952466818,56.0594672858678));
#62773=CARTESIAN_POINT('Ctrl Pts',(1.87873080151293,7.68468143731248,56.058646548968));
#62774=CARTESIAN_POINT('Ctrl Pts',(1.88465634121034,7.68323035534389,56.058401768185));
#62775=CARTESIAN_POINT('Ctrl Pts',(1.89660855662261,7.68028876574276,56.057908329374));
#62776=CARTESIAN_POINT('Ctrl Pts',(1.90263516825522,7.6787980152487,56.0576596792959));
#62777=CARTESIAN_POINT('Ctrl Pts',(1.91426583863499,7.67590650454088,56.0571801094962));
#62778=CARTESIAN_POINT('Ctrl Pts',(1.91987012863229,7.67450669794312,56.0569491596193));
#62779=CARTESIAN_POINT('Ctrl Pts',(1.93313891194257,7.6711770554237,56.0564026732089));
#62780=CARTESIAN_POINT('Ctrl Pts',(1.94080206316005,7.66924186739701,56.056087307343));
#62781=CARTESIAN_POINT('Ctrl Pts',(1.96763555511756,7.66242276802149,56.0549838752324));
#62782=CARTESIAN_POINT('Ctrl Pts',(1.98679053717376,7.65747841800647,56.0541977357732));
#62783=CARTESIAN_POINT('Ctrl Pts',(2.21985310861163,7.5963861241652,56.0446510118746));
#62784=CARTESIAN_POINT('Ctrl Pts',(2.43134146712307,7.53136226518839,56.036181076726));
#62785=CARTESIAN_POINT('Ctrl Pts',(2.77083090779123,7.41118926126218,56.0227849629902));
#62786=CARTESIAN_POINT('Ctrl Pts',(2.90058178980716,7.36137603874583,56.0177132520234));
#62787=CARTESIAN_POINT('Ctrl Pts',(3.32410669621311,7.18584119993391,56.0012272631558));
#62788=CARTESIAN_POINT('Ctrl Pts',(3.6115808603374,7.04574267515473,55.9901609389683));
#62789=CARTESIAN_POINT('Ctrl Pts',(4.36862835434026,6.61826197626851,55.9600633063668));
#62790=CARTESIAN_POINT('Ctrl Pts',(4.81790901423686,6.29872335029346,55.9411649348257));
#62791=CARTESIAN_POINT('Ctrl Pts',(5.24656979657568,5.92097057094752,55.9184160237587));
#62792=CARTESIAN_POINT('Ctrl Pts',(5.26270917098474,5.90663011349884,55.9175517850571));
#62793=CARTESIAN_POINT('Ctrl Pts',(5.28342709550625,5.88806911440244,55.9164320875113));
#62794=CARTESIAN_POINT('Ctrl Pts',(5.28805977367231,5.88390887074007,55.9161810486407));
#62795=CARTESIAN_POINT('Ctrl Pts',(5.29552087569938,5.87719271317207,55.9157756567925));
#62796=CARTESIAN_POINT('Ctrl Pts',(5.29835237955799,5.87464020980595,55.9156215573586));
#62797=CARTESIAN_POINT('Ctrl Pts',(5.30375298379715,5.86976467021196,55.9153271549309));
#62798=CARTESIAN_POINT('Ctrl Pts',(5.3063223985772,5.8674419979258,55.915186878865));
#62799=CARTESIAN_POINT('Ctrl Pts',(5.31217295970117,5.86214628367038,55.9148669926695));
#62800=CARTESIAN_POINT('Ctrl Pts',(5.31545313422395,5.85917217554512,55.9146873028564));
#62801=CARTESIAN_POINT('Ctrl Pts',(5.32407911899824,5.85133785847745,55.9142138688774));
#62802=CARTESIAN_POINT('Ctrl Pts',(5.32942075978555,5.84647308758946,55.913919786027));
#62803=CARTESIAN_POINT('Ctrl Pts',(5.36308930692496,5.81572578500935,55.9120604737163));
#62804=CARTESIAN_POINT('Ctrl Pts',(5.39123383724379,5.78964514813365,55.9104807227237));
#62805=CARTESIAN_POINT('Ctrl Pts',(5.8756537307755,5.33415365066025,55.8828638661877));
#62806=CARTESIAN_POINT('Ctrl Pts',(6.27949311272607,4.85225847995284,55.8534082387061));
#62807=CARTESIAN_POINT('Ctrl Pts',(6.78989512557029,4.07126134493764,55.8107953536195));
#62808=CARTESIAN_POINT('Ctrl Pts',(6.94251186674836,3.8051798655182,55.7970010505346));
#62809=CARTESIAN_POINT('Ctrl Pts',(7.16667801156803,3.35573576703768,55.7751570648926));
#62810=CARTESIAN_POINT('Ctrl Pts',(7.24751566716183,3.1773825500198,55.7668367656126));
#62811=CARTESIAN_POINT('Ctrl Pts',(7.35559268135786,2.91328085874929,55.7550296928161));
#62812=CARTESIAN_POINT('Ctrl Pts',(7.38811691399282,2.82978412726945,55.751369050144));
#62813=CARTESIAN_POINT('Ctrl Pts',(7.42420634024071,2.7322679062073,55.7471756010224));
#62814=CARTESIAN_POINT('Ctrl Pts',(7.42915951143515,2.71877116547598,55.7465970073129));
#62815=CARTESIAN_POINT('Ctrl Pts',(7.43616375053874,2.69952346777953,55.7457744264836));
#62816=CARTESIAN_POINT('Ctrl Pts',(7.43824498144354,2.69378356112058,55.7455294451465));
#62817=CARTESIAN_POINT('Ctrl Pts',(7.44242982144057,2.68220020204575,55.7450357123211));
#62818=CARTESIAN_POINT('Ctrl Pts',(7.44453319856616,2.67635667028695,55.7447869686078));
#62819=CARTESIAN_POINT('Ctrl Pts',(7.44857844331403,2.66507664054373,55.7443074480895));
#62820=CARTESIAN_POINT('Ctrl Pts',(7.45052124514183,2.65964048360582,55.7440766406591));
#62821=CARTESIAN_POINT('Ctrl Pts',(7.45510523723345,2.64676956932004,55.74353084638));
#62822=CARTESIAN_POINT('Ctrl Pts',(7.45774126125705,2.63933297102187,55.7432160295765));
#62823=CARTESIAN_POINT('Ctrl Pts',(7.46555432544673,2.61718604773805,55.7422800576544));
#62824=CARTESIAN_POINT('Ctrl Pts',(7.47069901234106,2.60246430623219,55.7416599656982));
#62825=CARTESIAN_POINT('Ctrl Pts',(7.51719198918745,2.46814868853098,55.736021268645));
#62826=CARTESIAN_POINT('Ctrl Pts',(7.55570983343924,2.34759112008196,55.7310961753692));
#62827=CARTESIAN_POINT('Ctrl Pts',(7.5983421122805,2.2022127096188,55.7253061348779));
#62828=CARTESIAN_POINT('Ctrl Pts',(7.60525071758175,2.17823442479767,55.7243559319127));
#62829=CARTESIAN_POINT('Ctrl Pts',(7.6283771171136,2.09651625872132,55.7211335542453));
#62830=CARTESIAN_POINT('Ctrl Pts',(7.64405187247924,2.03862429279536,55.7188777140182));
#62831=CARTESIAN_POINT('Ctrl Pts',(7.68415106515411,1.88355574459934,55.7129027526282));
#62832=CARTESIAN_POINT('Ctrl Pts',(7.70739044450382,1.78608316840343,55.7092174628827));
#62833=CARTESIAN_POINT('Ctrl Pts',(7.82155584536658,1.26341895491585,55.6897809216656));
#62834=CARTESIAN_POINT('Ctrl Pts',(7.87916492944024,0.831707580002971,55.6749176540655));
#62835=CARTESIAN_POINT('Ctrl Pts',(7.92672072185146,-0.11366514564192,55.6423643266124));
#62836=CARTESIAN_POINT('Ctrl Pts',(7.90277216693031,-0.626015841465745,
55.6247047098509));
#62837=CARTESIAN_POINT('Ctrl Pts',(7.82528101283342,-1.16180071787526,55.6032593012995));
#62838=CARTESIAN_POINT('Ctrl Pts',(7.82086231688285,-1.19118277998328,55.6020734922564));
#62839=CARTESIAN_POINT('Ctrl Pts',(7.81522175338531,-1.22730470455429,55.6006029275131));
#62840=CARTESIAN_POINT('Ctrl Pts',(7.81415646726147,-1.23406912165202,55.6003269896369));
#62841=CARTESIAN_POINT('Ctrl Pts',(7.81247112870737,-1.24468110429705,55.5998932239698));
#62842=CARTESIAN_POINT('Ctrl Pts',(7.81185701158553,-1.24852962268448,55.5997357346517));
#62843=CARTESIAN_POINT('Ctrl Pts',(7.81076264030382,-1.25535535658988,55.5994560883905));
#62844=CARTESIAN_POINT('Ctrl Pts',(7.81028352671805,-1.2583327567511,55.599333996981));
#62845=CARTESIAN_POINT('Ctrl Pts',(7.80917653949306,-1.26518702149594,55.599052678061));
#62846=CARTESIAN_POINT('Ctrl Pts',(7.8085474815737,-1.26906369116488,55.5988933821728));
#62847=CARTESIAN_POINT('Ctrl Pts',(7.80681295743093,-1.27970285659211,55.5984556945209));
#62848=CARTESIAN_POINT('Ctrl Pts',(7.80570159982083,-1.28646433563965,55.5981769594429));
#62849=CARTESIAN_POINT('Ctrl Pts',(7.80005370564234,-1.32054925730895,55.5967689789163));
#62850=CARTESIAN_POINT('Ctrl Pts',(7.79538253039404,-1.34784988784197,55.5956319684102));
#62851=CARTESIAN_POINT('Ctrl Pts',(7.78963031808254,-1.38043819715496,55.5942641433041));
#62852=CARTESIAN_POINT('Ctrl Pts',(7.78868706162772,-1.38575032539242,55.594040841202));
#62853=CARTESIAN_POINT('Ctrl Pts',(7.69839780702839,-1.89122697518797,55.5727607158837));
#62854=CARTESIAN_POINT('Ctrl Pts',(7.56108723122098,-2.38158539426013,55.5492259732346));
#62855=CARTESIAN_POINT('Ctrl Pts',(7.26975362807105,-3.13434227944995,55.5118692456279));
#62856=CARTESIAN_POINT('Ctrl Pts',(7.1460330732033,-3.40699911797003,55.4980459094883));
#62857=CARTESIAN_POINT('Ctrl Pts',(6.87882754887679,-3.91689899996896,55.4721219402893));
#62858=CARTESIAN_POINT('Ctrl Pts',(6.73773519694541,-4.15491393276698,55.4599867327234));
#62859=CARTESIAN_POINT('Ctrl Pts',(6.50374156720802,-4.50627029680868,55.4421399394595));
#62860=CARTESIAN_POINT('Ctrl Pts',(6.41969039350662,-4.62522482468499,55.4361082705959));
#62861=CARTESIAN_POINT('Ctrl Pts',(6.31573783490234,-4.76404758226554,55.4290787944988));
#62862=CARTESIAN_POINT('Ctrl Pts',(6.29895824101679,-4.78621132675783,55.4279567753096));
#62863=CARTESIAN_POINT('Ctrl Pts',(6.27625922212665,-4.81586776477866,55.4264557325126));
#62864=CARTESIAN_POINT('Ctrl Pts',(6.27044265640776,-4.82343871576265,55.4260725585723));
#62865=CARTESIAN_POINT('Ctrl Pts',(6.26075616423924,-4.83599970306573,55.4254368709044));
#62866=CARTESIAN_POINT('Ctrl Pts',(6.25689395081798,-4.84099565839245,55.4251840449573));
#62867=CARTESIAN_POINT('Ctrl Pts',(6.24937209811012,-4.85070149102846,55.4246928878978));
#62868=CARTESIAN_POINT('Ctrl Pts',(6.24571310664411,-4.85541186362224,55.4244545307481));
#62869=CARTESIAN_POINT('Ctrl Pts',(6.23721541806494,-4.86632579319855,55.4239022744056));
#62870=CARTESIAN_POINT('Ctrl Pts',(6.23237278316318,-4.87252628408058,55.4235885357871));
#62871=CARTESIAN_POINT('Ctrl Pts',(6.21668772134498,-4.89254773626665,55.4225755059916));
#62872=CARTESIAN_POINT('Ctrl Pts',(6.20580847202311,-4.90633985677398,55.4218777181546));
#62873=CARTESIAN_POINT('Ctrl Pts',(6.10395458900891,-5.03458389145896,55.4153897574647));
#62874=CARTESIAN_POINT('Ctrl Pts',(6.00986696252896,-5.14653266939225,55.4097293684111));
#62875=CARTESIAN_POINT('Ctrl Pts',(5.90796260437688,-5.26117385195258,55.4039176977383));
#62876=CARTESIAN_POINT('Ctrl Pts',(5.90319057552617,-5.26652764775033,55.4036462524957));
#62877=CARTESIAN_POINT('Ctrl Pts',(5.89337042810843,-5.2775148712053,55.4030891014652));
#62878=CARTESIAN_POINT('Ctrl Pts',(5.88832149611894,-5.28314756347061,55.4028034284323));
#62879=CARTESIAN_POINT('Ctrl Pts',(5.8770420733321,-5.29569486457616,55.4021669600065));
#62880=CARTESIAN_POINT('Ctrl Pts',(5.87080743907096,-5.30260574099432,55.401816329154));
#62881=CARTESIAN_POINT('Ctrl Pts',(5.83984553269885,-5.33680440087251,55.4000808297787));
#62882=CARTESIAN_POINT('Ctrl Pts',(5.81493996889262,-5.36393048591619,55.3987030061713));
#62883=CARTESIAN_POINT('Ctrl Pts',(5.72405437049743,-5.4615422688328,55.3937389888923));
#62884=CARTESIAN_POINT('Ctrl Pts',(5.65697394735353,-5.53099347393197,55.3901957522666));
#62885=CARTESIAN_POINT('Ctrl Pts',(5.13709506540786,-6.04989160703775,55.3635699516005));
#62886=CARTESIAN_POINT('Ctrl Pts',(4.63273366873903,-6.4442731164629,55.3426791621788));
#62887=CARTESIAN_POINT('Ctrl Pts',(3.8924164676964,-6.89089218349173,55.312254666605));
#62888=CARTESIAN_POINT('Ctrl Pts',(3.69339570909893,-6.99957984611477,55.3040694496615));
#62889=CARTESIAN_POINT('Ctrl Pts',(3.40410149492052,-7.14179072188917,55.2917915188516));
#62890=CARTESIAN_POINT('Ctrl Pts',(3.31745094337936,-7.18245080889313,55.2880670801005));
#62891=CARTESIAN_POINT('Ctrl Pts',(3.21460597424199,-7.22845191248364,55.2835676450676));
#62892=CARTESIAN_POINT('Ctrl Pts',(3.19910254904616,-7.23532663346636,55.2828872863945));
#62893=CARTESIAN_POINT('Ctrl Pts',(3.17854109133271,-7.24436524443233,55.2819820443794));
#62894=CARTESIAN_POINT('Ctrl Pts',(3.17350263495465,-7.2465738311059,55.2817599892528));
#62895=CARTESIAN_POINT('Ctrl Pts',(3.16523460645284,-7.25018781076949,55.2813952146852));
#62896=CARTESIAN_POINT('Ctrl Pts',(3.16200638500934,-7.25159630884115,55.281252693481));
#62897=CARTESIAN_POINT('Ctrl Pts',(3.15575419107739,-7.25431922082423,55.2809764799473));
#62898=CARTESIAN_POINT('Ctrl Pts',(3.1527303366362,-7.2556339003957,55.2808428047618));
#62899=CARTESIAN_POINT('Ctrl Pts',(3.14571336446607,-7.25867945079962,55.2805324071035));
#62900=CARTESIAN_POINT('Ctrl Pts',(3.14171965223378,-7.26040891186302,55.2803555950225));
#62901=CARTESIAN_POINT('Ctrl Pts',(3.12908647037998,-7.26586728520703,55.2797958245416));
#62902=CARTESIAN_POINT('Ctrl Pts',(3.12044180225646,-7.26958406668447,55.2794120938581));
#62903=CARTESIAN_POINT('Ctrl Pts',(3.04172521177515,-7.30326204433802,55.2759117958871));
#62904=CARTESIAN_POINT('Ctrl Pts',(2.97123256422584,-7.33222374590426,55.272733090728));
#62905=CARTESIAN_POINT('Ctrl Pts',(2.43191404305138,-7.5447468374978,55.2481434555556));
#62906=CARTESIAN_POINT('Ctrl Pts',(1.94697302397703,-7.68418104906985,55.2245559813647));
#62907=CARTESIAN_POINT('Ctrl Pts',(1.00887152905044,-7.85935212631907,55.1800277190929));
#62908=CARTESIAN_POINT('Ctrl Pts',(0.559325978150801,-7.90407850563647,
55.1591525951807));
#62909=CARTESIAN_POINT('Ctrl Pts',(0.00925545095834248,-7.91161581539457,
55.1350186138469));
#62910=CARTESIAN_POINT('Ctrl Pts',(-0.0898978754489525,-7.91111052715705,
55.1307208119828));
#62911=CARTESIAN_POINT('Ctrl Pts',(-0.3253246899419,-7.90548385530522,55.1206455361017));
#62912=CARTESIAN_POINT('Ctrl Pts',(-0.461528531496933,-7.89870274656284,
55.1149198563143));
#62913=CARTESIAN_POINT('Ctrl Pts',(-0.666568296919142,-7.88317235246538,
55.1064545426749));
#62914=CARTESIAN_POINT('Ctrl Pts',(-0.735572017726542,-7.87703331012308,
55.1036319376856));
#62915=CARTESIAN_POINT('Ctrl Pts',(-0.818239526009785,-7.86858285679967,
55.1002809385554));
#62916=CARTESIAN_POINT('Ctrl Pts',(-0.831987956484899,-7.86714103973553,
55.0997246470571));
#62917=CARTESIAN_POINT('Ctrl Pts',(-0.852997722175903,-7.86488202571483,
55.0988760808557));
#62918=CARTESIAN_POINT('Ctrl Pts',(-0.860261787491571,-7.86409079613217,
55.0985829721546));
#62919=CARTESIAN_POINT('Ctrl Pts',(-0.873404999756046,-7.86264075896253,
55.0980531421119));
#62920=CARTESIAN_POINT('Ctrl Pts',(-0.879284519257728,-7.86198541924955,
55.0978163095551));
#62921=CARTESIAN_POINT('Ctrl Pts',(-0.891018681482649,-7.86066418499986,
55.0973440102623));
#62922=CARTESIAN_POINT('Ctrl Pts',(-0.896873326236978,-7.8599983433187,
55.0971085419958));
#62923=CARTESIAN_POINT('Ctrl Pts',(-0.913289997807218,-7.85811271387323,
55.096448783869));
#62924=CARTESIAN_POINT('Ctrl Pts',(-0.923850335808975,-7.85687817152676,
55.0960249680496));
#62925=CARTESIAN_POINT('Ctrl Pts',(-0.966829367758204,-7.85176591468876,
55.0943024661485));
#62926=CARTESIAN_POINT('Ctrl Pts',(-0.999226614946151,-7.84770878731557,
55.0930095431726));
#62927=CARTESIAN_POINT('Ctrl Pts',(-1.50340318242531,-7.78139772556402,
55.0729716394644));
#62928=CARTESIAN_POINT('Ctrl Pts',(-1.96867227984588,-7.67689802705709,
55.0556970234804));
#62929=CARTESIAN_POINT('Ctrl Pts',(-2.64383141451025,-7.45979175542451,
55.0309089999737));
#62930=CARTESIAN_POINT('Ctrl Pts',(-2.86264026685125,-7.37859266160762,
55.0229059714501));
#62931=CARTESIAN_POINT('Ctrl Pts',(-3.55695528195361,-7.08539436583882,
54.9969469010359));
#62932=CARTESIAN_POINT('Ctrl Pts',(-4.01520842627125,-6.83613969233397,
54.9789572998664));
#62933=CARTESIAN_POINT('Ctrl Pts',(-4.46705360645275,-6.52916711821197,
54.9572455646012));
#62934=CARTESIAN_POINT('Ctrl Pts',(-4.48839543329875,-6.51451437869448,
54.9562105098672));
#62935=CARTESIAN_POINT('Ctrl Pts',(-4.51598331356562,-6.49537334221285,
54.9548604752397));
#62936=CARTESIAN_POINT('Ctrl Pts',(-4.52229545808426,-6.49098019811319,
54.9545507625569));
#62937=CARTESIAN_POINT('Ctrl Pts',(-4.53250468772385,-6.48385262942805,
54.9540485134785));
#62938=CARTESIAN_POINT('Ctrl Pts',(-4.5364057384734,-6.48112387168912,54.9538562858985));
#62939=CARTESIAN_POINT('Ctrl Pts',(-4.54386221993309,-6.47589808463257,
54.9534882657051));
#62940=CARTESIAN_POINT('Ctrl Pts',(-4.54741806257322,-6.47340164367663,
54.9533125048534));
#62941=CARTESIAN_POINT('Ctrl Pts',(-4.55556269303644,-6.46767354235411,
54.9529093338039));
#62942=CARTESIAN_POINT('Ctrl Pts',(-4.56015009855247,-6.46443992771909,
54.9526818191273));
#62943=CARTESIAN_POINT('Ctrl Pts',(-4.57427488508008,-6.45446099506771,
54.9519799718867));
#62944=CARTESIAN_POINT('Ctrl Pts',(-4.58380074190543,-6.44769945155181,
54.9515047820107));
#62945=CARTESIAN_POINT('Ctrl Pts',(-4.65590750633217,-6.39627682941083,
54.9478938751817));
#62946=CARTESIAN_POINT('Ctrl Pts',(-4.71784799825,-6.35072765210209,54.9447124525033));
#62947=CARTESIAN_POINT('Ctrl Pts',(-5.30843764849882,-5.9030170426427,54.9136730013443));
#62948=CARTESIAN_POINT('Ctrl Pts',(-5.78511889449883,-5.43668609128565,
54.8833606481556));
#62949=CARTESIAN_POINT('Ctrl Pts',(-6.32077581368699,-4.76138607988594,
54.8457241851147));
#62950=CARTESIAN_POINT('Ctrl Pts',(-6.43778686188287,-4.60194621603398,
54.8371982221568));
#62951=CARTESIAN_POINT('Ctrl Pts',(-6.66582480445574,-4.26547547627779,
54.8199650076297));
#62952=CARTESIAN_POINT('Ctrl Pts',(-6.77606153115479,-4.08809214991765,
54.8112814047331));
#62953=CARTESIAN_POINT('Ctrl Pts',(-6.90762868687323,-3.85641172438153,
54.8004205113061));
#62954=CARTESIAN_POINT('Ctrl Pts',(-6.93555226552375,-3.80596378835723,
54.7980834234914));
#62955=CARTESIAN_POINT('Ctrl Pts',(-6.9709058180247,-3.74041120160998,54.7950812787241));
#62956=CARTESIAN_POINT('Ctrl Pts',(-6.97884232755549,-3.7255823237436,54.794404423413));
#62957=CARTESIAN_POINT('Ctrl Pts',(-6.99159056556223,-3.70157934882366,
54.793312445532));
#62958=CARTESIAN_POINT('Ctrl Pts',(-6.99643165665369,-3.69242093843017,
54.7928966471493));
#62959=CARTESIAN_POINT('Ctrl Pts',(-7.00563055017833,-3.67493536345932,
54.7921043962801));
#62960=CARTESIAN_POINT('Ctrl Pts',(-7.00999153089272,-3.66660988769852,
54.7917278709205));
#62961=CARTESIAN_POINT('Ctrl Pts',(-7.0198696855995,-3.64766962722157,54.7908728526065));
#62962=CARTESIAN_POINT('Ctrl Pts',(-7.02537764467635,-3.63705004954421,
54.7903945710845));
#62963=CARTESIAN_POINT('Ctrl Pts',(-7.03952710152867,-3.60961722974583,
54.7891619324868));
#62964=CARTESIAN_POINT('Ctrl Pts',(-7.04813247566949,-3.59278540522781,
54.7884084055063));
#62965=CARTESIAN_POINT('Ctrl Pts',(-7.09913965331621,-3.49212853534224,
54.7839186813037));
#62966=CARTESIAN_POINT('Ctrl Pts',(-7.14010652271412,-3.40758343678757,
54.7802157934016));
#62967=CARTESIAN_POINT('Ctrl Pts',(-7.46585600995661,-2.70363793335301,
54.7499235717611));
#62968=CARTESIAN_POINT('Ctrl Pts',(-7.67097718628547,-2.05055992411536,
54.7255615778351));
#62969=CARTESIAN_POINT('Ctrl Pts',(-7.82622536317759,-1.17374586088003,
54.6932538320962));
#62970=CARTESIAN_POINT('Ctrl Pts',(-7.85446598018569,-0.966872766718426,
54.6856307079517));
#62971=CARTESIAN_POINT('Ctrl Pts',(-7.89284770347138,-0.568737706153017,
54.6706510248433));
#62972=CARTESIAN_POINT('Ctrl Pts',(-7.90429036087689,-0.377749577358185,
54.6633297457561));
#62973=CARTESIAN_POINT('Ctrl Pts',(-7.90947036055082,-0.158136250474576,
54.6545964830001));
#62974=CARTESIAN_POINT('Ctrl Pts',(-7.90998734532517,-0.129725193635088,
54.653460612989));
#62975=CARTESIAN_POINT('Ctrl Pts',(-7.91045310642648,-0.0933590609501438,
54.6519983368111));
#62976=CARTESIAN_POINT('Ctrl Pts',(-7.9105429723662,-0.0854057662753664,
54.6516780241876));
#62977=CARTESIAN_POINT('Ctrl Pts',(-7.9106680307464,-0.0726328915355494,
54.65116276784));
#62978=CARTESIAN_POINT('Ctrl Pts',(-7.91071081352397,-0.0678133781019686,
54.6509681573814));
#62979=CARTESIAN_POINT('Ctrl Pts',(-7.91078367967065,-0.0586628668222935,
54.6505982939529));
#62980=CARTESIAN_POINT('Ctrl Pts',(-7.91081461074806,-0.0543318760141865,
54.6504230786353));
#62981=CARTESIAN_POINT('Ctrl Pts',(-7.91087676061146,-0.0444988918204385,
54.6500249139243));
#62982=CARTESIAN_POINT('Ctrl Pts',(-7.91090579612882,-0.0389968909106522,
54.6498018669501));
#62983=CARTESIAN_POINT('Ctrl Pts',(-7.91097620417129,-0.0223676890769472,
54.6491269481663));
#62984=CARTESIAN_POINT('Ctrl Pts',(-7.91099983988053,-0.0112404600942861,
54.648674274225));
#62985=CARTESIAN_POINT('Ctrl Pts',(-7.91100139378223,0.0972945637295643,
54.6442482693096));
#62986=CARTESIAN_POINT('Ctrl Pts',(-7.90920388637905,0.194682414279019,
54.6401883349836));
#62987=CARTESIAN_POINT('Ctrl Pts',(-7.89916025783172,0.466590621048157,
54.628612833795));
#62988=CARTESIAN_POINT('Ctrl Pts',(-7.88693120459857,0.640897614751237,
54.620928536967));
#62989=CARTESIAN_POINT('Ctrl Pts',(-7.80809395681931,1.40241207555216,54.5866014928774));
#62990=CARTESIAN_POINT('Ctrl Pts',(-7.6815849677591,1.98151717405071,54.5586767167013));
#62991=CARTESIAN_POINT('Ctrl Pts',(-7.42074431963833,2.75051765220838,54.5223541201694));
#62992=CARTESIAN_POINT('Ctrl Pts',(-7.34098473291401,2.95681351732233,54.5126687284206));
#62993=CARTESIAN_POINT('Ctrl Pts',(-7.17904591430735,3.32854580044242,54.4954035306613));
#62994=CARTESIAN_POINT('Ctrl Pts',(-7.0995176153692,3.4949639688742,54.4877456364344));
#62995=CARTESIAN_POINT('Ctrl Pts',(-7.00571124286028,3.67481581921132,54.4795473328018));
#62996=CARTESIAN_POINT('Ctrl Pts',(-6.99712276538628,3.69114268698732,54.4788037945686));
#62997=CARTESIAN_POINT('Ctrl Pts',(-6.98494621866495,3.71409532607323,54.4777594796682));
#62998=CARTESIAN_POINT('Ctrl Pts',(-6.98140570698104,3.72074617835415,54.4774569892371));
#62999=CARTESIAN_POINT('Ctrl Pts',(-6.97523305518618,3.73230167714746,54.4769316257539));
#63000=CARTESIAN_POINT('Ctrl Pts',(-6.9726052329809,3.73720861721454,54.4767085968184));
#63001=CARTESIAN_POINT('Ctrl Pts',(-6.96711529483525,3.74743404830302,54.4762439615806));
#63002=CARTESIAN_POINT('Ctrl Pts',(-6.96425226205133,3.75275204465178,54.476002388677));
#63003=CARTESIAN_POINT('Ctrl Pts',(-6.95747641027568,3.76530352477339,54.4754324005983));
#63004=CARTESIAN_POINT('Ctrl Pts',(-6.9535583929155,3.77253420263692,54.4751041742924));
#63005=CARTESIAN_POINT('Ctrl Pts',(-6.94063027685553,3.79630439988731,54.4740255936312));
#63006=CARTESIAN_POINT('Ctrl Pts',(-6.93157235509077,3.81281791188241,54.473276979358));
#63007=CARTESIAN_POINT('Ctrl Pts',(-6.79315143912481,4.06304977760698,54.4619432880323));
#63008=CARTESIAN_POINT('Ctrl Pts',(-6.6520856600882,4.29011100597494,54.4518029210906));
#63009=CARTESIAN_POINT('Ctrl Pts',(-6.30205851439357,4.79461171703886,54.4293335472646));
#63010=CARTESIAN_POINT('Ctrl Pts',(-6.08578840830188,5.06630437406255,54.4172875773013));
#63011=CARTESIAN_POINT('Ctrl Pts',(-5.54891953301019,5.65657266600778,54.3900555011515));
#63012=CARTESIAN_POINT('Ctrl Pts',(-5.21750374315478,5.96363479823766,54.3750734310482));
#63013=CARTESIAN_POINT('Ctrl Pts',(-4.78790630533758,6.29830432492145,54.3555834466411));
#63014=CARTESIAN_POINT('Ctrl Pts',(-4.71304484278565,6.35451742239266,54.3521830055718));
#63015=CARTESIAN_POINT('Ctrl Pts',(-4.61844990458297,6.42295705860252,54.3478587710352));
#63016=CARTESIAN_POINT('Ctrl Pts',(-4.59963516703533,6.43644414359359,54.3469973593468));
#63017=CARTESIAN_POINT('Ctrl Pts',(-4.55845615084983,6.46568998733497,54.3451085296948));
#63018=CARTESIAN_POINT('Ctrl Pts',(-4.53606883258644,6.48141566419631,54.3440794215045));
#63019=CARTESIAN_POINT('Ctrl Pts',(-4.50113396791089,6.50568554640207,54.3424693579879));
#63020=CARTESIAN_POINT('Ctrl Pts',(-4.48864251060131,6.51431038815002,54.3418928350978));
#63021=CARTESIAN_POINT('Ctrl Pts',(-4.47246666620241,6.52541053268169,54.3411451041064));
#63022=CARTESIAN_POINT('Ctrl Pts',(-4.46880485544798,6.52791880036227,54.3409757596515));
#63023=CARTESIAN_POINT('Ctrl Pts',(-4.38439703140805,6.58563217884506,54.3370704168385));
#63024=CARTESIAN_POINT('Ctrl Pts',(-4.30263918899262,6.63933604256428,54.333249549241));
#63025=CARTESIAN_POINT('Ctrl Pts',(-4.21212501950866,6.69641758896424,54.3289552114098));
#63026=CARTESIAN_POINT('Ctrl Pts',(-4.2043316587103,6.70131337933255,54.3285849506606));
#63027=CARTESIAN_POINT('Ctrl Pts',(-4.19278990924557,6.70853584926152,54.3280358193725));
#63028=CARTESIAN_POINT('Ctrl Pts',(-4.18904806790678,6.71087302431279,54.3278576688444));
#63029=CARTESIAN_POINT('Ctrl Pts',(-4.18265607223728,6.71485807148709,54.3275531321573));
#63030=CARTESIAN_POINT('Ctrl Pts',(-4.18000689312152,6.71650750854074,54.3274268541708));
#63031=CARTESIAN_POINT('Ctrl Pts',(-4.17484480726642,6.71971729945578,54.3271806724549));
#63032=CARTESIAN_POINT('Ctrl Pts',(-4.17233200835366,6.72127780718651,54.3270607803698));
#63033=CARTESIAN_POINT('Ctrl Pts',(-4.16629971214822,6.7250193198404,54.3267728313904));
#63034=CARTESIAN_POINT('Ctrl Pts',(-4.16277937927967,6.72719897007644,54.3266046815977));
#63035=CARTESIAN_POINT('Ctrl Pts',(-4.15215023733279,6.73376857440024,54.326096655016));
#63036=CARTESIAN_POINT('Ctrl Pts',(-4.14503620344684,6.73815001896247,54.3257562005799));
#63037=CARTESIAN_POINT('Ctrl Pts',(-4.08034280503776,6.77785265155747,54.3226563459042));
#63038=CARTESIAN_POINT('Ctrl Pts',(-4.02232174770383,6.81244531857652,54.3198486142397));
#63039=CARTESIAN_POINT('Ctrl Pts',(-3.86989094279651,6.90069974314022,54.3124166351989));
#63040=CARTESIAN_POINT('Ctrl Pts',(-3.77480844072638,6.95316707137615,54.307726125373));
#63041=CARTESIAN_POINT('Ctrl Pts',(-3.5125096643223,7.09093981235793,54.2947053308149));
#63042=CARTESIAN_POINT('Ctrl Pts',(-3.34329192713029,7.17227613945592,54.2862181017761));
#63043=CARTESIAN_POINT('Ctrl Pts',(-2.71430949998211,7.44750473671709,54.2547718989931));
#63044=CARTESIAN_POINT('Ctrl Pts',(-2.239339324259,7.60382884953763,54.231304310802));
#63045=CARTESIAN_POINT('Ctrl Pts',(-1.56151033566278,7.75784059404436,54.2001202101018));
#63046=CARTESIAN_POINT('Ctrl Pts',(-1.36865451119107,7.79417710300998,54.1914845072642));
#63047=CARTESIAN_POINT('Ctrl Pts',(-0.963286642336671,7.85504146375148,
54.1738878755487));
#63048=CARTESIAN_POINT('Ctrl Pts',(-0.750726622021704,7.87819882917556,
54.1649747842295));
#63049=CARTESIAN_POINT('Ctrl Pts',(-0.518440318842779,7.89401702015003,
54.1555702635607));
#63050=CARTESIAN_POINT('Ctrl Pts',(-0.4993988475509,7.89524451024308,54.1548017542104));
#63051=CARTESIAN_POINT('Ctrl Pts',(-0.472758356611746,7.89686510134103,
54.1537299031472));
#63052=CARTESIAN_POINT('Ctrl Pts',(-0.465163005852263,7.89731614353443,
54.153424693541));
#63053=CARTESIAN_POINT('Ctrl Pts',(-0.452020716693898,7.89807755952089,
54.1528972439245));
#63054=CARTESIAN_POINT('Ctrl Pts',(-0.446474086565619,7.89839304888848,
54.1526748390884));
#63055=CARTESIAN_POINT('Ctrl Pts',(-0.43497060420794,7.89903520463919,54.1522139990201));
#63056=CARTESIAN_POINT('Ctrl Pts',(-0.429013704269862,7.89936097620649,
54.1519755927668));
#63057=CARTESIAN_POINT('Ctrl Pts',(-0.415053910109282,7.90010857366783,
54.1514174390923));
#63058=CARTESIAN_POINT('Ctrl Pts',(-0.407050725320346,7.90052497822478,
54.1510978665853));
#63059=CARTESIAN_POINT('Ctrl Pts',(-0.381176740330629,7.9018317781422,54.1500660474147));
#63060=CARTESIAN_POINT('Ctrl Pts',(-0.363303488125574,7.9026737082129,54.1493553625864));
#63061=CARTESIAN_POINT('Ctrl Pts',(0.0630626495372903,7.92130841543808,
54.1324509563313));
#63062=CARTESIAN_POINT('Ctrl Pts',(0.472336952076169,7.9074679656097,54.1173449989784));
#63063=CARTESIAN_POINT('Ctrl Pts',(1.3219132479206,7.81251035575637,54.087116533106));
#63064=CARTESIAN_POINT('Ctrl Pts',(1.76008875075446,7.72559743536786,54.0721723812568));
#63065=CARTESIAN_POINT('Ctrl Pts',(2.56974624454654,7.492505065984,54.0430045594239));
#63066=CARTESIAN_POINT('Ctrl Pts',(2.94205885645191,7.35428138251562,54.0289021492482));
#63067=CARTESIAN_POINT('Ctrl Pts',(3.32536579388838,7.17819631233874,54.0121623010053));
#63068=CARTESIAN_POINT('Ctrl Pts',(3.34828475148504,7.1675343847979,54.0111525553832));
#63069=CARTESIAN_POINT('Ctrl Pts',(3.37714670378542,7.15393912831975,54.0098693391469));
#63070=CARTESIAN_POINT('Ctrl Pts',(3.38313786960205,7.15110782088136,54.0096023332876));
#63071=CARTESIAN_POINT('Ctrl Pts',(3.39262832704831,7.14660822086276,54.0091783599521));
#63072=CARTESIAN_POINT('Ctrl Pts',(3.3961299375109,7.14494488960087,54.0090217113406));
#63073=CARTESIAN_POINT('Ctrl Pts',(3.40265850190072,7.14183781433899,54.008729242071));
#63074=CARTESIAN_POINT('Ctrl Pts',(3.40568576466494,7.14039471732286,54.0085934624138));
#63075=CARTESIAN_POINT('Ctrl Pts',(3.41240562783139,7.13718611103132,54.0082917004765));
#63076=CARTESIAN_POINT('Ctrl Pts',(3.41609777544479,7.13541966115768,54.0081256589838));
#63077=CARTESIAN_POINT('Ctrl Pts',(3.42677648790989,7.13030041129808,54.0076447242336));
#63078=CARTESIAN_POINT('Ctrl Pts',(3.43375948253413,7.12694021784625,54.0073293690345));
#63079=CARTESIAN_POINT('Ctrl Pts',(3.48122845167115,7.10401235057283,54.0051798296094));
#63080=CARTESIAN_POINT('Ctrl Pts',(3.5215511694137,7.08411040434333,54.0033250721157));
#63081=CARTESIAN_POINT('Ctrl Pts',(3.64159235850062,7.0235839383093,53.9977220212574));
#63082=CARTESIAN_POINT('Ctrl Pts',(3.72079180005881,6.98195055737766,53.9939170533948));
#63083=CARTESIAN_POINT('Ctrl Pts',(3.95807439182758,6.85203247401155,53.9822268946967));
#63084=CARTESIAN_POINT('Ctrl Pts',(4.11384480221491,6.75965805012074,53.9741564195072));
#63085=CARTESIAN_POINT('Ctrl Pts',(4.66141019158781,6.40900211585848,53.9446984926822));
#63086=CARTESIAN_POINT('Ctrl Pts',(5.03322842158587,6.12133028790897,53.9226780181487));
#63087=CARTESIAN_POINT('Ctrl Pts',(5.72872561091578,5.47677844320272,53.8796468509303));
#63088=CARTESIAN_POINT('Ctrl Pts',(6.04981130166447,5.11989115546819,53.8587703798929));
#63089=CARTESIAN_POINT('Ctrl Pts',(6.35667546462409,4.70932218796625,53.8379354926226));
#63090=CARTESIAN_POINT('Ctrl Pts',(6.376518142503,4.68241976401718,53.8365833034318));
#63091=CARTESIAN_POINT('Ctrl Pts',(6.4026258039801,4.64654962589455,53.8347974171092));
#63092=CARTESIAN_POINT('Ctrl Pts',(6.40904341252182,4.63769373173109,53.8343578719279));
#63093=CARTESIAN_POINT('Ctrl Pts',(6.41899593857839,4.62389976315787,53.8336753527245));
#63094=CARTESIAN_POINT('Ctrl Pts',(6.42254355787134,4.61897089476357,53.8334318937847));
#63095=CARTESIAN_POINT('Ctrl Pts',(6.42961224410748,4.60912615946927,53.8329464524287));
#63096=CARTESIAN_POINT('Ctrl Pts',(6.43313335727791,4.60421033090008,53.8327044683241));
#63097=CARTESIAN_POINT('Ctrl Pts',(6.4410235796382,4.59316806449455,53.8321618341848));
#63098=CARTESIAN_POINT('Ctrl Pts',(6.44538959361138,4.58703941656409,53.831861301918));
#63099=CARTESIAN_POINT('Ctrl Pts',(6.45813461694831,4.56909488756851,53.8309832134038));
#63100=CARTESIAN_POINT('Ctrl Pts',(6.46648994586387,4.55726218305472,53.8304065550506));
#63101=CARTESIAN_POINT('Ctrl Pts',(6.52719175045507,4.47079405004421,53.8262096622014));
#63102=CARTESIAN_POINT('Ctrl Pts',(6.57827811890939,4.39528033877656,53.822637098113));
#63103=CARTESIAN_POINT('Ctrl Pts',(6.73780986071604,4.15045307413853,53.8113351755653));
#63104=CARTESIAN_POINT('Ctrl Pts',(6.84111286162604,3.97787925983614,53.803792237628));
#63105=CARTESIAN_POINT('Ctrl Pts',(7.17577841544393,3.36712299310398,53.7782987806675));
#63106=CARTESIAN_POINT('Ctrl Pts',(7.37249837230412,2.91128668839764,53.7614063117358));
#63107=CARTESIAN_POINT('Ctrl Pts',(7.6617425154968,2.01923996278327,53.7288011478788));
#63108=CARTESIAN_POINT('Ctrl Pts',(7.7626401538392,1.58775562584783,53.7131765404564));
#63109=CARTESIAN_POINT('Ctrl Pts',(7.83102565803567,1.12238408748307,53.6945249145642));
#63110=CARTESIAN_POINT('Ctrl Pts',(7.83495871367955,1.0945916207366,53.6934042014381));
#63111=CARTESIAN_POINT('Ctrl Pts',(7.83970063798375,1.05974773550727,53.6919899806515));
#63112=CARTESIAN_POINT('Ctrl Pts',(7.84064807983595,1.0527150819112,53.6917040767372));
#63113=CARTESIAN_POINT('Ctrl Pts',(7.84212129303695,1.04166742391493,53.6912542013861));
#63114=CARTESIAN_POINT('Ctrl Pts',(7.84265344815074,1.03765326041308,53.6910905845958));
#63115=CARTESIAN_POINT('Ctrl Pts',(7.84358621813709,1.03057546304203,53.6908018191059));
#63116=CARTESIAN_POINT('Ctrl Pts',(7.84398811960136,1.02751200765785,53.6906767427893));
#63117=CARTESIAN_POINT('Ctrl Pts',(7.84490749495456,1.0204721822949,53.6903891077557));
#63118=CARTESIAN_POINT('Ctrl Pts',(7.84542373860193,1.01649566693804,53.6902264809888));
#63119=CARTESIAN_POINT('Ctrl Pts',(7.84684738297746,1.00546394646195,53.6897748971894));
#63120=CARTESIAN_POINT('Ctrl Pts',(7.84774828983688,0.998407921708941,53.6894855802659));
#63121=CARTESIAN_POINT('Ctrl Pts',(7.85263788064273,0.959696458744219,53.6878957150061));
#63122=CARTESIAN_POINT('Ctrl Pts',(7.85644450044818,0.928018715253356,53.6865852392076));
#63123=CARTESIAN_POINT('Ctrl Pts',(7.92026897711992,0.368325073013722,53.6632747814623));
#63124=CARTESIAN_POINT('Ctrl Pts',(7.92712024046717,-0.164357049041584,
53.6387148386669));
#63125=CARTESIAN_POINT('Ctrl Pts',(7.85654579817689,-0.966144067404371,
53.6017567592807));
#63126=CARTESIAN_POINT('Ctrl Pts',(7.81844345881557,-1.23721369436539,53.5892470523026));
#63127=CARTESIAN_POINT('Ctrl Pts',(7.72253631184899,-1.73187737823185,53.5667313754097));
#63128=CARTESIAN_POINT('Ctrl Pts',(7.66884339775479,-1.95596973967448,53.5566511928367));
#63129=CARTESIAN_POINT('Ctrl Pts',(7.55492458046071,-2.35387496549663,53.5390551539159));
#63130=CARTESIAN_POINT('Ctrl Pts',(7.49827564471101,-2.52853337112462,53.5314385790942));
#63131=CARTESIAN_POINT('Ctrl Pts',(7.42969323098445,-2.71732933217363,53.5233204662122));
#63132=CARTESIAN_POINT('Ctrl Pts',(7.42373394927293,-2.73356808244131,53.5226231363781));
#63133=CARTESIAN_POINT('Ctrl Pts',(7.41483133141846,-2.7575834457663,53.5215932140294));
#63134=CARTESIAN_POINT('Ctrl Pts',(7.41192893743517,-2.76537512115204,53.5212592718277));
#63135=CARTESIAN_POINT('Ctrl Pts',(7.4069510193809,-2.7786745471853,53.5206896322138));
#63136=CARTESIAN_POINT('Ctrl Pts',(7.40488162544707,-2.78418457649695,53.5204537324379));
#63137=CARTESIAN_POINT('Ctrl Pts',(7.4008534483558,-2.79487386071654,53.5199962973385));
#63138=CARTESIAN_POINT('Ctrl Pts',(7.3988953730365,-2.80005337813129,53.51977473875));
#63139=CARTESIAN_POINT('Ctrl Pts',(7.39421482738385,-2.81239520638055,53.5192470254165));
#63140=CARTESIAN_POINT('Ctrl Pts',(7.39148738407393,-2.81955563198677,53.5189410356066));
#63141=CARTESIAN_POINT('Ctrl Pts',(7.38333736115095,-2.84085899647557,53.5180311902216));
#63142=CARTESIAN_POINT('Ctrl Pts',(7.37788454782948,-2.85499037276248,53.5174283379661));
#63143=CARTESIAN_POINT('Ctrl Pts',(7.33271992907483,-2.97104437362298,53.5124829437925));
#63144=CARTESIAN_POINT('Ctrl Pts',(7.29093783803178,-3.07215117576059,53.5082098766322));
#63145=CARTESIAN_POINT('Ctrl Pts',(7.11722107459119,-3.46899678306391,53.4915539112372));
#63146=CARTESIAN_POINT('Ctrl Pts',(6.96927564021247,-3.75739183977866,53.4797247739583));
#63147=CARTESIAN_POINT('Ctrl Pts',(6.64558138941399,-4.30309985339854,53.4572738053077));
#63148=CARTESIAN_POINT('Ctrl Pts',(6.47150008237445,-4.56071392238005,53.4466391962093));
#63149=CARTESIAN_POINT('Ctrl Pts',(6.01997632535334,-5.15080069639834,53.4210911927234));
#63150=CARTESIAN_POINT('Ctrl Pts',(5.72954266995674,-5.47203302482016,53.4061854269505));
#63151=CARTESIAN_POINT('Ctrl Pts',(5.40201028312265,-5.77948894587036,53.3890880750929));
#63152=CARTESIAN_POINT('Ctrl Pts',(5.38963063290485,-5.79103524501524,53.3884414177846));
#63153=CARTESIAN_POINT('Ctrl Pts',(5.3678184195355,-5.81124861838055,53.3873010956351));
#63154=CARTESIAN_POINT('Ctrl Pts',(5.35840165976526,-5.81993270919212,53.3868084874449));
#63155=CARTESIAN_POINT('Ctrl Pts',(5.28992254482219,-5.88277673681315,53.3832236397932));
#63156=CARTESIAN_POINT('Ctrl Pts',(5.23006311297005,-5.93605775906779,53.3800761611036));
#63157=CARTESIAN_POINT('Ctrl Pts',(5.16198390594688,-5.99482604457503,53.3764680886912));
#63158=CARTESIAN_POINT('Ctrl Pts',(5.15454944248595,-6.00121964215105,53.3760737019837));
#63159=CARTESIAN_POINT('Ctrl Pts',(5.14397392694059,-6.01028037771302,53.375512126942));
#63160=CARTESIAN_POINT('Ctrl Pts',(5.14084262287012,-6.01295893105309,53.3753457806313));
#63161=CARTESIAN_POINT('Ctrl Pts',(5.13509905765693,-6.01786427651866,53.3750405311192));
#63162=CARTESIAN_POINT('Ctrl Pts',(5.13248743573662,-6.02009181860882,53.374901683641));
#63163=CARTESIAN_POINT('Ctrl Pts',(5.12719691676145,-6.02459833906063,53.3746203103493));
#63164=CARTESIAN_POINT('Ctrl Pts',(5.12451794823885,-6.02687723189729,53.374477778232));
#63165=CARTESIAN_POINT('Ctrl Pts',(5.11792432965599,-6.0324785883757,53.3741268387473));
#63166=CARTESIAN_POINT('Ctrl Pts',(5.11400798976526,-6.03579900624991,53.373918280347));
#63167=CARTESIAN_POINT('Ctrl Pts',(5.09944612203629,-6.04812074933684,53.3731423803979));
#63168=CARTESIAN_POINT('Ctrl Pts',(5.08878012974753,-6.05709766608196,53.3725732160128));
#63169=CARTESIAN_POINT('Ctrl Pts',(4.82807335440149,-6.27534404011813,53.3586418954421));
#63170=CARTESIAN_POINT('Ctrl Pts',(4.56537686471979,-6.46896667355995,53.3441806890438));
#63171=CARTESIAN_POINT('Ctrl Pts',(4.01111413607448,-6.82688029823039,53.3141243232239));
#63172=CARTESIAN_POINT('Ctrl Pts',(3.71953711401065,-6.9900196176755,53.2985455209948));
#63173=CARTESIAN_POINT('Ctrl Pts',(2.89880342900438,-7.38329152675879,53.2566522391708));
#63174=CARTESIAN_POINT('Ctrl Pts',(2.35335763240726,-7.57482331444368,53.2310240059406));
#63175=CARTESIAN_POINT('Ctrl Pts',(1.75265460559258,-7.71451513144251,53.2059054740924));
#63176=CARTESIAN_POINT('Ctrl Pts',(1.71337138506902,-7.72333480052468,53.2042756314812));
#63177=CARTESIAN_POINT('Ctrl Pts',(1.66292521790088,-7.73425688957956,53.2021988056117));
#63178=CARTESIAN_POINT('Ctrl Pts',(1.65182309670722,-7.73663559778787,53.2017427413106));
#63179=CARTESIAN_POINT('Ctrl Pts',(1.63412205955062,-7.74038833179083,53.2010171866495));
#63180=CARTESIAN_POINT('Ctrl Pts',(1.62752646252181,-7.74177783500172,53.2007471878776));
#63181=CARTESIAN_POINT('Ctrl Pts',(1.61518925979152,-7.7443604671018,53.2002428032749));
#63182=CARTESIAN_POINT('Ctrl Pts',(1.60944809036837,-7.74555564397812,53.2000083503237));
#63183=CARTESIAN_POINT('Ctrl Pts',(1.59665533552149,-7.74820395806832,53.19948651846));
#63184=CARTESIAN_POINT('Ctrl Pts',(1.58960308055271,-7.7496538556851,53.199199246041));
#63185=CARTESIAN_POINT('Ctrl Pts',(1.56906269175149,-7.75384760794976,53.1983636901308));
#63186=CARTESIAN_POINT('Ctrl Pts',(1.55556933227962,-7.75656589689976,53.1978162454392));
#63187=CARTESIAN_POINT('Ctrl Pts',(1.45991495959644,-7.77557619468792,53.1939455916218));
#63188=CARTESIAN_POINT('Ctrl Pts',(1.37750540830707,-7.79059793923101,53.1906641501927));
#63189=CARTESIAN_POINT('Ctrl Pts',(1.11931529864668,-7.83343618984169,53.1805403464521));
#63190=CARTESIAN_POINT('Ctrl Pts',(0.942821423590777,-7.85663297225901,
53.1738474455045));
#63191=CARTESIAN_POINT('Ctrl Pts',(0.698487286303601,-7.88039308502629,
53.1648346432874));
#63192=CARTESIAN_POINT('Ctrl Pts',(0.631204760605771,-7.88606748810711,
53.1623788327571));
#63193=CARTESIAN_POINT('Ctrl Pts',(0.512766192067003,-7.89453072918604,
53.1580960525916));
#63194=CARTESIAN_POINT('Ctrl Pts',(0.461640722211808,-7.89768526391019,
53.1562604792607));
#63195=CARTESIAN_POINT('Ctrl Pts',(0.102699998759804,-7.91633518719077,
53.1434546825544));
#63196=CARTESIAN_POINT('Ctrl Pts',(-0.205765113024291,-7.9143273820681,
53.1328829458629));
#63197=CARTESIAN_POINT('Ctrl Pts',(-1.07041971224426,-7.85810306177393,
53.1032396024818));
#63198=CARTESIAN_POINT('Ctrl Pts',(-1.62204423100101,-7.76301502540086,
53.0843670750515));
#63199=CARTESIAN_POINT('Ctrl Pts',(-2.19360315738441,-7.60087632333886,
53.0609227427606));
#63200=CARTESIAN_POINT('Ctrl Pts',(-2.22815122294207,-7.59082062390545,
53.0594897195736));
#63201=CARTESIAN_POINT('Ctrl Pts',(-2.26916432534553,-7.57857907398771,
53.0577682496949));
#63202=CARTESIAN_POINT('Ctrl Pts',(-2.27569714609764,-7.57661995977173,
53.0574934294246));
#63203=CARTESIAN_POINT('Ctrl Pts',(-2.28627967858125,-7.5734314642,53.0570472400486));
#63204=CARTESIAN_POINT('Ctrl Pts',(-2.29033096223412,-7.57220727363559,
53.0568761870642));
#63205=CARTESIAN_POINT('Ctrl Pts',(-2.29751496473137,-7.57003016565,53.0565724366728));
#63206=CARTESIAN_POINT('Ctrl Pts',(-2.30064808102345,-7.56907855219083,
53.0564398193403));
#63207=CARTESIAN_POINT('Ctrl Pts',(-2.30722503698683,-7.56707648912086,
53.0561611273542));
#63208=CARTESIAN_POINT('Ctrl Pts',(-2.3106687403075,-7.56602563674595,53.0560150278176));
#63209=CARTESIAN_POINT('Ctrl Pts',(-2.31976697874516,-7.56324250166316,
53.0556285703246));
#63210=CARTESIAN_POINT('Ctrl Pts',(-2.32542028228102,-7.56150623123615,
53.0553879669446));
#63211=CARTESIAN_POINT('Ctrl Pts',(-2.35099484507061,-7.5536202522019,53.0542973946147));
#63212=CARTESIAN_POINT('Ctrl Pts',(-2.37089352503012,-7.54739819758797,
53.0534430216105));
#63213=CARTESIAN_POINT('Ctrl Pts',(-2.51800736355599,-7.50075844345554,
53.0470845300441));
#63214=CARTESIAN_POINT('Ctrl Pts',(-2.64419985437063,-7.45720737089999,
53.0413976549571));
#63215=CARTESIAN_POINT('Ctrl Pts',(-3.01779869987117,-7.31759730086645,
53.0239919044625));
#63216=CARTESIAN_POINT('Ctrl Pts',(-3.26152976506177,-7.21226365561203,
53.0118803527195));
#63217=CARTESIAN_POINT('Ctrl Pts',(-3.59508680838912,-7.04773959719167,
52.9946563558052));
#63218=CARTESIAN_POINT('Ctrl Pts',(-3.68971812254812,-6.99866147430354,
52.9896926528854));
#63219=CARTESIAN_POINT('Ctrl Pts',(-3.88616914120351,-6.89168505301032,
52.9792598173926));
#63220=CARTESIAN_POINT('Ctrl Pts',(-3.98775433606687,-6.83340683129726,
52.9737904063483));
#63221=CARTESIAN_POINT('Ctrl Pts',(-4.48409256518029,-6.53382520938955,
52.946788641531));
#63222=CARTESIAN_POINT('Ctrl Pts',(-4.85847679960628,-6.26045056837409,
52.9256034945241));
#63223=CARTESIAN_POINT('Ctrl Pts',(-5.3769776025157,-5.80715928738465,52.8959088128475));
#63224=CARTESIAN_POINT('Ctrl Pts',(-5.54066492631449,-5.65119728822662,
52.886459357009));
#63225=CARTESIAN_POINT('Ctrl Pts',(-5.71098955644581,-5.47438577363508,
52.8765319542371));
#63226=CARTESIAN_POINT('Ctrl Pts',(-5.7244673050893,-5.46029077912868,52.8757456889945));
#63227=CARTESIAN_POINT('Ctrl Pts',(-5.74320502269232,-5.44054929301917,
52.8746515346896));
#63228=CARTESIAN_POINT('Ctrl Pts',(-5.74850900211401,-5.43494478311402,
52.8743417022937));
#63229=CARTESIAN_POINT('Ctrl Pts',(-5.75765706129074,-5.42525001003886,
52.8738071134581));
#63230=CARTESIAN_POINT('Ctrl Pts',(-5.76150499894516,-5.42116340411987,
52.8735821873183));
#63231=CARTESIAN_POINT('Ctrl Pts',(-5.76946234814722,-5.41269445889231,
52.8731169196789));
#63232=CARTESIAN_POINT('Ctrl Pts',(-5.77357112450705,-5.40831152602033,
52.8728766060831));
#63233=CARTESIAN_POINT('Ctrl Pts',(-5.78316402911962,-5.39805514839312,
52.8723153653332));
#63234=CARTESIAN_POINT('Ctrl Pts',(-5.78864421347987,-5.39217801477691,
52.8719946107387));
#63235=CARTESIAN_POINT('Ctrl Pts',(-5.80623464543317,-5.37325572400189,
52.870964613048));
#63236=CARTESIAN_POINT('Ctrl Pts',(-5.81830986357289,-5.36017799799626,
52.8702568959081));
#63237=CARTESIAN_POINT('Ctrl Pts',(-6.0688096175932,-5.08703741676485,52.8555610459253));
#63238=CARTESIAN_POINT('Ctrl Pts',(-6.28962674410215,-4.81134367714607,
52.8423619123879));
#63239=CARTESIAN_POINT('Ctrl Pts',(-6.61278549892338,-4.34743028797965,
52.8220501574856));
#63240=CARTESIAN_POINT('Ctrl Pts',(-6.72718047041968,-4.1682285009271,52.8146070437094));
#63241=CARTESIAN_POINT('Ctrl Pts',(-6.88317394012459,-3.9006771859441,52.8038761104926));
#63242=CARTESIAN_POINT('Ctrl Pts',(-6.93057345379505,-3.8158246466999,52.8005258083642));
#63243=CARTESIAN_POINT('Ctrl Pts',(-7.01962318096328,-3.64927603782986,
52.7940227074274));
#63244=CARTESIAN_POINT('Ctrl Pts',(-7.06144007828467,-3.56768681235174,
52.7908699696546));
#63245=CARTESIAN_POINT('Ctrl Pts',(-7.31670804373829,-3.04755280095899,
52.7708917995774));
#63246=CARTESIAN_POINT('Ctrl Pts',(-7.4906257351634,-2.59080444162496,52.7539208301729));
#63247=CARTESIAN_POINT('Ctrl Pts',(-7.62995306471455,-2.09015823298453,
52.7333427922374));
#63248=CARTESIAN_POINT('Ctrl Pts',(-7.63834607804533,-2.05927520108679,
52.7320660303111));
#63249=CARTESIAN_POINT('Ctrl Pts',(-7.64875762255149,-2.02002521652862,
52.7304347182502));
#63250=CARTESIAN_POINT('Ctrl Pts',(-7.65095029426418,-2.01170441113285,
52.7300883962383));
#63251=CARTESIAN_POINT('Ctrl Pts',(-7.65439977852426,-1.99852700673814,
52.7295391753409));
#63252=CARTESIAN_POINT('Ctrl Pts',(-7.65566555909101,-1.99367274478783,
52.7293366912091));
#63253=CARTESIAN_POINT('Ctrl Pts',(-7.65799945232955,-1.98468727911223,
52.7289615851987));
#63254=CARTESIAN_POINT('Ctrl Pts',(-7.65906884212541,-1.98055640647481,
52.7287890217172));
#63255=CARTESIAN_POINT('Ctrl Pts',(-7.66143437093945,-1.97138819985877,
52.7284057722394));
#63256=CARTESIAN_POINT('Ctrl Pts',(-7.66272888445041,-1.96635045146487,
52.7281950128939));
#63257=CARTESIAN_POINT('Ctrl Pts',(-7.66641950164567,-1.9519289997621,52.7275911932014));
#63258=CARTESIAN_POINT('Ctrl Pts',(-7.66880333801117,-1.9425421892554,52.7271975860729));
#63259=CARTESIAN_POINT('Ctrl Pts',(-7.67410921618356,-1.92148729396025,
52.7263134348816));
#63260=CARTESIAN_POINT('Ctrl Pts',(-7.67702189196768,-1.90981688933012,
52.725822484112));
#63261=CARTESIAN_POINT('Ctrl Pts',(-7.68610790668835,-1.87305471216532,
52.7242732952206));
#63262=CARTESIAN_POINT('Ctrl Pts',(-7.69218489282864,-1.84793946362036,
52.7232109958669));
#63263=CARTESIAN_POINT('Ctrl Pts',(-7.83953709636964,-1.22563271150984,
52.6967992752754));
#63264=CARTESIAN_POINT('Ctrl Pts',(-7.91096660799007,-0.61407003492305,
52.6689754571467));
#63265=CARTESIAN_POINT('Ctrl Pts',(-7.91099998829544,-0.000430336557561556,
52.6419314571579));
#63266=CARTESIAN_POINT('',(-7.911,2.06501482580279E-13,50.642331508237));
#63267=CARTESIAN_POINT('Ctrl Pts',(-7.911,1.51545442861334E-13,52.642331508237));
#63268=CARTESIAN_POINT('Ctrl Pts',(-7.91099999999996,2.20167589666687,52.5537440725043));
#63269=CARTESIAN_POINT('Ctrl Pts',(-6.94214576672367,4.38610418338687,52.4651566367716));
#63270=CARTESIAN_POINT('Ctrl Pts',(-3.67820201488288,7.3418068410763,52.2879817653061));
#63271=CARTESIAN_POINT('Ctrl Pts',(-1.40868175871752,8.08992666571334,52.1993943295734));
#63272=CARTESIAN_POINT('Ctrl Pts',(2.97309270521258,7.65454228025262,52.022219458108));
#63273=CARTESIAN_POINT('Ctrl Pts',(5.05102072675584,6.47444880834238,51.9336320223752));
#63274=CARTESIAN_POINT('Ctrl Pts',(7.66951518847859,2.93425195367736,51.7564571509098));
#63275=CARTESIAN_POINT('Ctrl Pts',(8.18956872247067,0.601881960099537,51.6678697151771));
#63276=CARTESIAN_POINT('Ctrl Pts',(7.32306689761363,-3.71537198232408,51.4906948437116));
#63277=CARTESIAN_POINT('Ctrl Pts',(5.94329958850236,-5.66643518936472,51.4021074079789));
#63278=CARTESIAN_POINT('Ctrl Pts',(2.16154501637906,-7.9220591323298,51.2249325365134));
#63279=CARTESIAN_POINT('Ctrl Pts',(-0.210816529299704,-8.20894963713003,
51.1363451007807));
#63280=CARTESIAN_POINT('Ctrl Pts',(-4.42123908576373,-6.91982244717871,
50.9591702293153));
#63281=CARTESIAN_POINT('Ctrl Pts',(-6.22631625634134,-5.35390358803581,
50.8705827935825));
#63282=CARTESIAN_POINT('Ctrl Pts',(-7.65317280859479,-2.31334857514567,
50.7354407413122));
#63283=CARTESIAN_POINT('Ctrl Pts',(-7.91100000000003,-1.15702837836533,
50.6888861247746));
#63284=CARTESIAN_POINT('Ctrl Pts',(-7.911,2.06501482580279E-13,50.642331508237));
#63285=CARTESIAN_POINT('',(-7.91099943894101,0.00297944206225246,48.6425309018316));
#63286=CARTESIAN_POINT('Ctrl Pts',(-7.91099989537763,0.00128659828464795,
50.642331508237));
#63287=CARTESIAN_POINT('Ctrl Pts',(-7.91096572008773,0.211422674174465,
50.6339190564692));
#63288=CARTESIAN_POINT('Ctrl Pts',(-7.90255468055934,0.421350259379313,
50.6255066047014));
#63289=CARTESIAN_POINT('Ctrl Pts',(-7.88584196755081,0.630410551001773,
50.6170941529337));
#63290=CARTESIAN_POINT('Ctrl Pts',(-7.86909991135218,0.839837898282741,
50.6086669310821));
#63291=CARTESIAN_POINT('Ctrl Pts',(-7.84402707863192,1.048394644105,50.6002397092305));
#63292=CARTESIAN_POINT('Ctrl Pts',(-7.81075000739738,1.25543033336855,50.591812487379));
#63293=CARTESIAN_POINT('Ctrl Pts',(-7.77738440477785,1.46301682700379,50.5833628454767));
#63294=CARTESIAN_POINT('Ctrl Pts',(-7.73577093775734,1.66907390387563,50.5749132035745));
#63295=CARTESIAN_POINT('Ctrl Pts',(-7.68608714525271,1.87296166420486,50.5664635616723));
#63296=CARTESIAN_POINT('Ctrl Pts',(-7.63633259403002,2.07713979762805,50.5580018859499));
#63297=CARTESIAN_POINT('Ctrl Pts',(-7.57848482854346,2.27914218659757,50.5495402102274));
#63298=CARTESIAN_POINT('Ctrl Pts',(-7.5127706875228,2.47834573792646,50.5410785345049));
#63299=CARTESIAN_POINT('Ctrl Pts',(-7.4469154620526,2.67797696772681,50.5325986920554));
#63300=CARTESIAN_POINT('Ctrl Pts',(-7.37316017474965,2.87479709133008,50.5241188496059));
#63301=CARTESIAN_POINT('Ctrl Pts',(-7.29178003110565,3.06820223876603,50.5156390071564));
#63302=CARTESIAN_POINT('Ctrl Pts',(-7.26035893702876,3.14287649049904,50.5123649169984));
#63303=CARTESIAN_POINT('Ctrl Pts',(-7.2278016498811,3.21704191783815,50.5090908268404));
#63304=CARTESIAN_POINT('Ctrl Pts',(-7.19412580975778,3.29066480112711,50.5058167366824));
#63305=CARTESIAN_POINT('Ctrl Pts',(-7.10860288381246,3.47763695601159,50.4975018804206));
#63306=CARTESIAN_POINT('Ctrl Pts',(-7.01571379924195,3.66143339218067,50.4891870241587));
#63307=CARTESIAN_POINT('Ctrl Pts',(-6.91570954292541,3.84146879694349,50.4808721678969));
#63308=CARTESIAN_POINT('Ctrl Pts',(-6.81582843837433,4.02128249436345,50.4725675510915));
#63309=CARTESIAN_POINT('Ctrl Pts',(-6.70884977933363,4.19734414270669,50.4642629342861));
#63310=CARTESIAN_POINT('Ctrl Pts',(-6.59507168477514,4.36909034842234,50.4559583174807));
#63311=CARTESIAN_POINT('Ctrl Pts',(-6.48142619905779,4.54063638322284,50.4476633797407));
#63312=CARTESIAN_POINT('Ctrl Pts',(-6.36099724542115,4.70787676367204,50.4393684420007));
#63313=CARTESIAN_POINT('Ctrl Pts',(-6.23412814604646,4.87027383816058,50.4310735042606));
#63314=CARTESIAN_POINT('Ctrl Pts',(-6.10744919986194,5.03242750963024,50.4227909990899));
#63315=CARTESIAN_POINT('Ctrl Pts',(-5.9743495511192,5.1897521316094,50.4145084939192));
#63316=CARTESIAN_POINT('Ctrl Pts',(-5.83521501341863,5.34174004863339,50.4062259887485));
#63317=CARTESIAN_POINT('Ctrl Pts',(-5.69620829060746,5.4935883431084,50.3979510922385));
#63318=CARTESIAN_POINT('Ctrl Pts',(-5.55117793158211,5.64010949349851,50.3896761957284));
#63319=CARTESIAN_POINT('Ctrl Pts',(-5.40055026219762,5.78082847570114,50.3814012992183));
#63320=CARTESIAN_POINT('Ctrl Pts',(-5.25009489111149,5.92138649384398,50.3731358681046));
#63321=CARTESIAN_POINT('Ctrl Pts',(-5.09405519942159,6.05615538767114,50.3648704369908));
#63322=CARTESIAN_POINT('Ctrl Pts',(-4.9328948354957,6.18469639852595,50.3566050058771));
#63323=CARTESIAN_POINT('Ctrl Pts',(-4.86991695643135,6.23492736127152,50.3533750595776));
#63324=CARTESIAN_POINT('Ctrl Pts',(-4.80615751659977,6.28420767292708,50.350145113278));
#63325=CARTESIAN_POINT('Ctrl Pts',(-4.74164569489685,6.33251270066363,50.3469151669785));
#63326=CARTESIAN_POINT('Ctrl Pts',(-4.57653722254991,6.45614227933196,50.3386485968336));
#63327=CARTESIAN_POINT('Ctrl Pts',(-4.40668419390388,6.57324130337467,50.3303820266887));
#63328=CARTESIAN_POINT('Ctrl Pts',(-4.23262855662394,6.68347039356438,50.3221154565438));
#63329=CARTESIAN_POINT('Ctrl Pts',(-4.05841696347715,6.79379825029553,50.3138414794564));
#63330=CARTESIAN_POINT('Ctrl Pts',(-3.87999549225706,6.89724372729374,50.3055675023689));
#63331=CARTESIAN_POINT('Ctrl Pts',(-3.6979315218611,6.99351295556289,50.2972935252814));
#63332=CARTESIAN_POINT('Ctrl Pts',(-3.5156926024737,7.08987469090172,50.2890115975602));
#63333=CARTESIAN_POINT('Ctrl Pts',(-3.32980445543751,7.17904627338473,50.280729669839));
#63334=CARTESIAN_POINT('Ctrl Pts',(-3.14085604662888,7.26078124545526,50.2724477421177));
#63335=CARTESIAN_POINT('Ctrl Pts',(-2.95159443359853,7.34265170285999,50.2641520861268));
#63336=CARTESIAN_POINT('Ctrl Pts',(-2.75926268708295,7.41706078818231,50.2558564301358));
#63337=CARTESIAN_POINT('Ctrl Pts',(-2.56446852670033,7.48381067208167,50.2475607741448));
#63338=CARTESIAN_POINT('Ctrl Pts',(-2.36949831009525,7.55062088495796,50.2392576204863));
#63339=CARTESIAN_POINT('Ctrl Pts',(-2.17206151672117,7.60975798982195,50.2309544668278));
#63340=CARTESIAN_POINT('Ctrl Pts',(-1.97277904660427,7.66107458737214,50.2226513131692));
#63341=CARTESIAN_POINT('Ctrl Pts',(-1.77319274310542,7.71246942409397,50.2143355002173));
#63342=CARTESIAN_POINT('Ctrl Pts',(-1.57175542403136,7.7560198534894,50.2060196872654));
#63343=CARTESIAN_POINT('Ctrl Pts',(-1.36909800993088,7.79162958816725,50.1977038743134));
#63344=CARTESIAN_POINT('Ctrl Pts',(-1.29038025064674,7.80546139656658,50.1944737819672));
#63345=CARTESIAN_POINT('Ctrl Pts',(-1.21147846111171,7.81809569875332,50.1912436896209));
#63346=CARTESIAN_POINT('Ctrl Pts',(-1.13242976097967,7.82952896644795,50.1880135972746));
#63347=CARTESIAN_POINT('Ctrl Pts',(-0.938827999898432,7.85753070154159,
50.1801026314314));
#63348=CARTESIAN_POINT('Ctrl Pts',(-0.743942682173932,7.87838269023725,
50.1721916655883));
#63349=CARTESIAN_POINT('Ctrl Pts',(-0.548344041427492,7.89197312541236,
50.1642806997451));
#63350=CARTESIAN_POINT('Ctrl Pts',(-0.352943328428411,7.90554980832309,
50.1563777390682));
#63351=CARTESIAN_POINT('Ctrl Pts',(-0.156831071094351,7.91187955087205,
50.1484747783913));
#63352=CARTESIAN_POINT('Ctrl Pts',(0.0394138177652493,7.91090181654211,
50.1405718177144));
#63353=CARTESIAN_POINT('Ctrl Pts',(0.235496442323643,7.90992489064788,50.132675391569));
#63354=CARTESIAN_POINT('Ctrl Pts',(0.431711137372738,7.90165252663699,50.1247789654235));
#63355=CARTESIAN_POINT('Ctrl Pts',(0.627475108132371,7.88607608311474,50.1168825392781));
#63356=CARTESIAN_POINT('Ctrl Pts',(0.823113430771456,7.87050963709532,50.1089911813333));
#63357=CARTESIAN_POINT('Ctrl Pts',(1.01830126333165,7.84764847933911,50.1010998233886));
#63358=CARTESIAN_POINT('Ctrl Pts',(1.2124567644762,7.8175360308908,50.0932084654439));
#63359=CARTESIAN_POINT('Ctrl Pts',(1.40652356372339,7.78743733961804,50.0853207127456));
#63360=CARTESIAN_POINT('Ctrl Pts',(1.59955863166727,7.75009401192119,50.0774329600473));
#63361=CARTESIAN_POINT('Ctrl Pts',(1.79098591028883,7.70560123995181,50.069545207349));
#63362=CARTESIAN_POINT('Ctrl Pts',(1.98236113748558,7.66112056611281,50.0616595994274));
#63363=CARTESIAN_POINT('Ctrl Pts',(2.17212911153887,7.60949440070085,50.0537739915058));
#63364=CARTESIAN_POINT('Ctrl Pts',(2.35972433844907,7.55086895969802,50.0458883835842));
#63365=CARTESIAN_POINT('Ctrl Pts',(2.54734169058909,7.49223660433294,50.0380018456236));
#63366=CARTESIAN_POINT('Ctrl Pts',(2.73278545268314,7.42660342019414,50.0301153076629));
#63367=CARTESIAN_POINT('Ctrl Pts',(2.91550504660686,7.35416557627104,50.0222287697023));
#63368=CARTESIAN_POINT('Ctrl Pts',(3.09824765974582,7.28171860654875,50.0143412381869));
#63369=CARTESIAN_POINT('Ctrl Pts',(3.27826510016409,7.20246539522135,50.0064537066716));
#63370=CARTESIAN_POINT('Ctrl Pts',(3.45502656880677,7.11665036438065,49.9985661751562));
#63371=CARTESIAN_POINT('Ctrl Pts',(3.63183993331962,7.03081013887659,49.9906763279194));
#63372=CARTESIAN_POINT('Ctrl Pts',(3.80539511113926,6.93840440521484,49.9827864806827));
#63373=CARTESIAN_POINT('Ctrl Pts',(3.97518549589906,6.83972377170261,49.9748966334459));
#63374=CARTESIAN_POINT('Ctrl Pts',(4.14505418933691,6.74099762589608,49.9670031473488));
#63375=CARTESIAN_POINT('Ctrl Pts',(4.31115433203221,6.6359909861206,49.9591096612516));
#63376=CARTESIAN_POINT('Ctrl Pts',(4.47300770478048,6.52503816639983,49.9512161751545));
#63377=CARTESIAN_POINT('Ctrl Pts',(4.6350481798038,6.41395708537291,49.9433135641983));
#63378=CARTESIAN_POINT('Ctrl Pts',(4.79283179476898,6.29691628933584,49.9354109532422));
#63379=CARTESIAN_POINT('Ctrl Pts',(4.94591195799857,6.17429153050993,49.927508342286));
#63380=CARTESIAN_POINT('Ctrl Pts',(5.09909365233387,6.05158544026207,49.9196004898876));
#63381=CARTESIAN_POINT('Ctrl Pts',(5.24756541598531,5.92328822837078,49.9116926374893));
#63382=CARTESIAN_POINT('Ctrl Pts',(5.39091686108726,5.78981315733463,49.9037847850909));
#63383=CARTESIAN_POINT('Ctrl Pts',(5.53446445162516,5.65615545454349,49.8958661125076));
#63384=CARTESIAN_POINT('Ctrl Pts',(5.67287748753951,5.51730598466832,49.8879474399242));
#63385=CARTESIAN_POINT('Ctrl Pts',(5.80578448127278,5.37371264183452,49.8800287673408));
#63386=CARTESIAN_POINT('Ctrl Pts',(5.86071464715428,5.31436583155929,49.8767559975162));
#63387=CARTESIAN_POINT('Ctrl Pts',(5.91470479491093,5.25420906129168,49.8734832276917));
#63388=CARTESIAN_POINT('Ctrl Pts',(5.96773084404036,5.19327541856673,49.8702104578671));
#63389=CARTESIAN_POINT('Ctrl Pts',(6.09480679920306,5.04724906024012,49.8623673249482));
#63390=CARTESIAN_POINT('Ctrl Pts',(6.21671907405414,4.89632666671056,49.8545241920293));
#63391=CARTESIAN_POINT('Ctrl Pts',(6.33306274314762,4.74091101913499,49.8466810591104));
#63392=CARTESIAN_POINT('Ctrl Pts',(6.44926977898489,4.58567789069569,49.8388471371163));
#63393=CARTESIAN_POINT('Ctrl Pts',(6.55992102252503,4.42596229358886,49.8310132151222));
#63394=CARTESIAN_POINT('Ctrl Pts',(6.66464900251338,4.26220303051103,49.8231792931282));
#63395=CARTESIAN_POINT('Ctrl Pts',(6.76927435842586,4.09860423689934,49.8153530476786));
#63396=CARTESIAN_POINT('Ctrl Pts',(6.86798782162776,3.93096996202489,49.8075268022291));
#63397=CARTESIAN_POINT('Ctrl Pts',(6.96046265731882,3.7597713489081,49.7997005567796));
#63398=CARTESIAN_POINT('Ctrl Pts',(7.05286485010405,3.58870721956345,49.7918804591779));
#63399=CARTESIAN_POINT('Ctrl Pts',(7.139038009825,3.41408463631659,49.7840603615761));
#63400=CARTESIAN_POINT('Ctrl Pts',(7.21869904997974,3.23640310002039,49.7762402639743));
#63401=CARTESIAN_POINT('Ctrl Pts',(7.29831299034876,3.05882661836908,49.7684247900245));
#63402=CARTESIAN_POINT('Ctrl Pts',(7.37142233751846,2.87819510625526,49.7606093160747));
#63403=CARTESIAN_POINT('Ctrl Pts',(7.43779016705609,2.69503217621678,49.7527938421248));
#63404=CARTESIAN_POINT('Ctrl Pts',(7.50413164753822,2.51194196469634,49.7449814710391));
#63405=CARTESIAN_POINT('Ctrl Pts',(7.56373682338245,2.32632266768829,49.7371690999534));
#63406=CARTESIAN_POINT('Ctrl Pts',(7.61641702412088,2.13871753971432,49.7293567288676));
#63407=CARTESIAN_POINT('Ctrl Pts',(7.66909523072578,1.95111951326369,49.721544653508));
#63408=CARTESIAN_POINT('Ctrl Pts',(7.71484888073255,1.76153614158864,49.7137325781484));
#63409=CARTESIAN_POINT('Ctrl Pts',(7.75353914339565,1.57052594751931,49.7059205027888));
#63410=CARTESIAN_POINT('Ctrl Pts',(7.79223053762832,1.37951016699727,49.6981081989504));
#63411=CARTESIAN_POINT('Ctrl Pts',(7.82385806239047,1.18706782562856,49.6902958951119));
#63412=CARTESIAN_POINT('Ctrl Pts',(7.84833400920573,0.993767719311079,49.6824835912734));
#63413=CARTESIAN_POINT('Ctrl Pts',(7.87281497848729,0.800427947795876,49.6746696843496));
#63414=CARTESIAN_POINT('Ctrl Pts',(7.89014140225767,0.606230409680675,49.6668557774257));
#63415=CARTESIAN_POINT('Ctrl Pts',(7.90027743487255,0.41174925870444,49.6590418705019));
#63416=CARTESIAN_POINT('Ctrl Pts',(7.91041733099552,0.217193978181619,49.6512249851846));
#63417=CARTESIAN_POINT('Ctrl Pts',(7.91336135827729,0.0223552204291192,
49.6434080998674));
#63418=CARTESIAN_POINT('Ctrl Pts',(7.90912578952055,-0.172192466562872,
49.6355912145501));
#63419=CARTESIAN_POINT('Ctrl Pts',(7.90488562606776,-0.36695119663747,49.627765849566));
#63420=CARTESIAN_POINT('Ctrl Pts',(7.89345031880717,-0.561417873584109,
49.6199404845819));
#63421=CARTESIAN_POINT('Ctrl Pts',(7.87488814875403,-0.755021618639716,
49.6121151195978));
#63422=CARTESIAN_POINT('Ctrl Pts',(7.85631469743633,-0.948743027473951,
49.6042849987036));
#63423=CARTESIAN_POINT('Ctrl Pts',(7.83060579755964,-1.14160011168952,49.5964548778093));
#63424=CARTESIAN_POINT('Ctrl Pts',(7.79788095963174,-1.33303170983018,49.5886247569151));
#63425=CARTESIAN_POINT('Ctrl Pts',(7.7651113890189,-1.52472498228031,49.5807839327644));
#63426=CARTESIAN_POINT('Ctrl Pts',(7.72530679730214,-1.71498853379204,49.5729431086138));
#63427=CARTESIAN_POINT('Ctrl Pts',(7.67863699410016,-1.9032747864763,49.5651022844631));
#63428=CARTESIAN_POINT('Ctrl Pts',(7.65344952427684,-2.00489197751325,49.5608706291285));
#63429=CARTESIAN_POINT('Ctrl Pts',(7.62626326518703,-2.10593354250732,49.5566389737939));
#63430=CARTESIAN_POINT('Ctrl Pts',(7.59711072894231,-2.20631583690769,49.5524073184593));
#63431=CARTESIAN_POINT('Ctrl Pts',(7.54260941011058,-2.39398278246085,49.544496144123));
#63432=CARTESIAN_POINT('Ctrl Pts',(7.48107696304029,-2.57988131185113,49.5365849697867));
#63433=CARTESIAN_POINT('Ctrl Pts',(7.41264373094572,-2.76344602228288,49.5286737954504));
#63434=CARTESIAN_POINT('Ctrl Pts',(7.34428468935969,-2.94681172473563,49.5207711978543));
#63435=CARTESIAN_POINT('Ctrl Pts',(7.26903988384833,-3.12784832774792,49.5128686002581));
#63436=CARTESIAN_POINT('Ctrl Pts',(7.18709001154408,-3.30600335238234,49.5049660026619));
#63437=CARTESIAN_POINT('Ctrl Pts',(7.10521377135276,-3.48399830439527,49.4970705055644));
#63438=CARTESIAN_POINT('Ctrl Pts',(7.01664460893177,-3.65911652444873,49.4891750084669));
#63439=CARTESIAN_POINT('Ctrl Pts',(6.92161219521525,-3.83082309941969,49.4812795113694));
#63440=CARTESIAN_POINT('Ctrl Pts',(6.82664753310625,-4.0024072593533,49.473389643221));
#63441=CARTESIAN_POINT('Ctrl Pts',(6.72522896642979,-4.17058431964628,49.4654997750726));
#63442=CARTESIAN_POINT('Ctrl Pts',(6.617633325523,-4.33484142373483,49.4576099069242));
#63443=CARTESIAN_POINT('Ctrl Pts',(6.51009443085917,-4.49901189816572,49.4497241999144));
#63444=CARTESIAN_POINT('Ctrl Pts',(6.39638514208911,-4.65926624819583,49.4418384929046));
#63445=CARTESIAN_POINT('Ctrl Pts',(6.27682721679446,-4.81511797264701,49.4339527858948));
#63446=CARTESIAN_POINT('Ctrl Pts',(6.15731016886918,-4.97091641072265,49.4260697750422));
#63447=CARTESIAN_POINT('Ctrl Pts',(6.03194867947861,-5.12231495002544,49.4181867641895));
#63448=CARTESIAN_POINT('Ctrl Pts',(5.901106803828,-5.2688575127645,49.4103037533369));
#63449=CARTESIAN_POINT('Ctrl Pts',(5.77026297555807,-5.41540226243214,49.4024206248421));
#63450=CARTESIAN_POINT('Ctrl Pts',(5.63393882094205,-5.55709062790542,49.3945374963474));
#63451=CARTESIAN_POINT('Ctrl Pts',(5.49253790022358,-5.69350054137237,49.3866543678526));
#63452=CARTESIAN_POINT('Ctrl Pts',(5.35112823654482,-5.82991888920067,49.3787707519361));
#63453=CARTESIAN_POINT('Ctrl Pts',(5.20464142918148,-5.96105789470025,49.3708871360196));
#63454=CARTESIAN_POINT('Ctrl Pts',(5.05351705104708,-6.08653320164907,49.3630035201031));
#63455=CARTESIAN_POINT('Ctrl Pts',(4.90235792553739,-6.21203735859306,49.3551180915409));
#63456=CARTESIAN_POINT('Ctrl Pts',(4.74655936988931,-6.33187500173534,49.3472326629787));
#63457=CARTESIAN_POINT('Ctrl Pts',(4.58659328324015,-6.44570268117731,49.3393472344164));
#63458=CARTESIAN_POINT('Ctrl Pts',(4.42656352648673,-6.55957566659862,49.3314586672761));
#63459=CARTESIAN_POINT('Ctrl Pts',(4.26236321429242,-6.66743372201613,49.3235701001357));
#63460=CARTESIAN_POINT('Ctrl Pts',(4.09449259617966,-6.76897712951004,49.3156815329954));
#63461=CARTESIAN_POINT('Ctrl Pts',(3.92644332723753,-6.87062860126302,49.3077845707048));
#63462=CARTESIAN_POINT('Ctrl Pts',(3.75471624571798,-6.96595182364409,49.2998876084142));
#63463=CARTESIAN_POINT('Ctrl Pts',(3.57983651224036,-7.05469287394078,49.2919906461236));
#63464=CARTESIAN_POINT('Ctrl Pts',(3.40485012539054,-7.14348804447243,49.2840888677366));
#63465=CARTESIAN_POINT('Ctrl Pts',(3.22670756574118,-7.22569289582836,49.2761870893496));
#63466=CARTESIAN_POINT('Ctrl Pts',(3.04595350836448,-7.30110185005538,49.2682853109625));
#63467=CARTESIAN_POINT('Ctrl Pts',(2.86496567357744,-7.37660833409884,49.2603733128476));
#63468=CARTESIAN_POINT('Ctrl Pts',(2.68135991670849,-7.44530124449316,49.2524613147326));
#63469=CARTESIAN_POINT('Ctrl Pts',(2.49569666048523,-7.50702465553716,49.2445493166177));
#63470=CARTESIAN_POINT('Ctrl Pts',(2.41790566520306,-7.53288613009597,49.2412342707623));
#63471=CARTESIAN_POINT('Ctrl Pts',(2.3397536061309,-7.55752470766804,49.237919224907));
#63472=CARTESIAN_POINT('Ctrl Pts',(2.26128219665213,-7.58093159361724,49.2346041790516));
#63473=CARTESIAN_POINT('Ctrl Pts',(2.07401468960909,-7.63679078116675,49.2266930127149));
#63474=CARTESIAN_POINT('Ctrl Pts',(1.88442447998909,-7.68578197425321,49.2187818463782));
#63475=CARTESIAN_POINT('Ctrl Pts',(1.69305742689917,-7.72770842806725,49.2108706800415));
#63476=CARTESIAN_POINT('Ctrl Pts',(1.50189780963638,-7.76958943493268,49.2029680891586));
#63477=CARTESIAN_POINT('Ctrl Pts',(1.30896551909382,-7.80442088290069,49.1950654982757));
#63478=CARTESIAN_POINT('Ctrl Pts',(1.11482283013101,-7.83205535331682,49.1871629073929));
#63479=CARTESIAN_POINT('Ctrl Pts',(0.920854547395602,-7.85966499857082,
49.1792674157269));
#63480=CARTESIAN_POINT('Ctrl Pts',(0.725678371578291,-7.88009049750577,
49.171371924061));
#63481=CARTESIAN_POINT('Ctrl Pts',(0.529868343850086,-7.89323511230887,
49.163476432395));
#63482=CARTESIAN_POINT('Ctrl Pts',(0.334197883670724,-7.9063703580225,49.1555865684001));
#63483=CARTESIAN_POINT('Ctrl Pts',(0.137894814354981,-7.9122350360598,49.1476967044051));
#63484=CARTESIAN_POINT('Ctrl Pts',(-0.0584598142239484,-7.91078399718517,
49.1398068404102));
#63485=CARTESIAN_POINT('Ctrl Pts',(-0.254710916503281,-7.90933372335838,
49.1319211362786));
#63486=CARTESIAN_POINT('Ctrl Pts',(-0.451013179879313,-7.90057542106007,
49.1240354321471));
#63487=CARTESIAN_POINT('Ctrl Pts',(-0.646783368387427,-7.88451598225138,
49.1161497280155));
#63488=CARTESIAN_POINT('Ctrl Pts',(-0.842486653808792,-7.86846203164309,
49.1082667187679));
#63489=CARTESIAN_POINT('Ctrl Pts',(-1.03765788350082,-7.84511194553864,
49.1003837095203));
#63490=CARTESIAN_POINT('Ctrl Pts',(-1.23171647932104,-7.81452465058298,
49.0925007002727));
#63491=CARTESIAN_POINT('Ctrl Pts',(-1.42577801802487,-7.78393689177335,
49.0846175714799));
#63492=CARTESIAN_POINT('Ctrl Pts',(-1.61872654723241,-7.74611175014959,
49.0767344426871));
#63493=CARTESIAN_POINT('Ctrl Pts',(-1.80998867403695,-7.70115978277675,
49.0688513138943));
#63494=CARTESIAN_POINT('Ctrl Pts',(-2.00126265556515,-7.65620502921115,
49.0609676964929));
#63495=CARTESIAN_POINT('Ctrl Pts',(-2.19084969038866,-7.60412264805146,
49.0530840790915));
#63496=CARTESIAN_POINT('Ctrl Pts',(-2.37818857432778,-7.54507389658556,
49.0452004616902));
#63497=CARTESIAN_POINT('Ctrl Pts',(-2.56557056049255,-7.48601155940506,
49.0373150304558));
#63498=CARTESIAN_POINT('Ctrl Pts',(-2.7507030360838,-7.41997976179219,49.0294295992214));
#63499=CARTESIAN_POINT('Ctrl Pts',(-2.933041668067,-7.34718909334602,49.021544167987));
#63500=CARTESIAN_POINT('Ctrl Pts',(-3.11545290238636,-7.27436944161462,
49.013655596986));
#63501=CARTESIAN_POINT('Ctrl Pts',(-3.29506775638119,-7.19478568436457,
49.0057670259851));
#63502=CARTESIAN_POINT('Ctrl Pts',(-3.47136329712847,-7.10869593240204,
48.9978784549842));
#63503=CARTESIAN_POINT('Ctrl Pts',(-3.64784649422363,-7.02251454290646,
48.9899814870584));
#63504=CARTESIAN_POINT('Ctrl Pts',(-3.82100301078051,-6.92981347755794,
48.9820845191325));
#63505=CARTESIAN_POINT('Ctrl Pts',(-3.99033491131733,-6.83089659528836,
48.9741875512066));
#63506=CARTESIAN_POINT('Ctrl Pts',(-4.15977010364698,-6.73191937410994,
48.9662857661614));
#63507=CARTESIAN_POINT('Ctrl Pts',(-4.32537573844868,-6.62671896132088,
48.9583839811162));
#63508=CARTESIAN_POINT('Ctrl Pts',(-4.48668394442731,-6.51564180897156,
48.950482196071));
#63509=CARTESIAN_POINT('Ctrl Pts',(-4.64820080830229,-6.40442097437867,
48.942570189786));
#63510=CARTESIAN_POINT('Ctrl Pts',(-4.80540886433323,-6.28730842182488,
48.9346581835011));
#63511=CARTESIAN_POINT('Ctrl Pts',(-4.95787344496143,-6.16469073869455,
48.9267461772161));
#63512=CARTESIAN_POINT('Ctrl Pts',(-5.02175447060904,-6.11331524329342,
48.9234311313587));
#63513=CARTESIAN_POINT('Ctrl Pts',(-5.08480321349437,-6.06097375796805,
48.9201160855013));
#63514=CARTESIAN_POINT('Ctrl Pts',(-5.14698968350636,-6.00769658004456,
48.9168010396439));
#63515=CARTESIAN_POINT('Ctrl Pts',(-5.29194049870996,-5.8835124871017,48.9090739794108));
#63516=CARTESIAN_POINT('Ctrl Pts',(-5.43264100632112,-5.75386768989842,
48.9013469191777));
#63517=CARTESIAN_POINT('Ctrl Pts',(-5.56863976892367,-5.61908997293705,
48.8936198589445));
#63518=CARTESIAN_POINT('Ctrl Pts',(-5.70448562424255,-5.48446379040295,
48.8859014864654));
#63519=CARTESIAN_POINT('Ctrl Pts',(-5.83564000193244,-5.34471642644837,
48.8781831139862));
#63520=CARTESIAN_POINT('Ctrl Pts',(-5.96168298045172,-5.20021701860531,
48.8704647415071));
#63521=CARTESIAN_POINT('Ctrl Pts',(-6.08761020370407,-5.0558503160325,48.8627534574217));
#63522=CARTESIAN_POINT('Ctrl Pts',(-6.2084351360824,-4.90674052780092,48.8550421733363));
#63523=CARTESIAN_POINT('Ctrl Pts',(-6.32377328171775,-4.75329490789628,
48.847330889251));
#63524=CARTESIAN_POINT('Ctrl Pts',(-6.43902921392429,-4.59995866455981,
48.8396251017956));
#63525=CARTESIAN_POINT('Ctrl Pts',(-6.54880592956319,-4.4422930309143,48.8319193143402));
#63526=CARTESIAN_POINT('Ctrl Pts',(-6.65275792867704,-4.28073976579105,
48.8242135268847));
#63527=CARTESIAN_POINT('Ctrl Pts',(-6.75666117229831,-4.11926227226513,
48.8165113535923));
#63528=CARTESIAN_POINT('Ctrl Pts',(-6.85474494229913,-3.95390108078876,
48.8088091802998));
#63529=CARTESIAN_POINT('Ctrl Pts',(-6.94670589464532,-3.7851285596793,48.8011070070073));
#63530=CARTESIAN_POINT('Ctrl Pts',(-7.0386446643698,-3.61639674951179,48.7934066916164));
#63531=CARTESIAN_POINT('Ctrl Pts',(-7.12446338239918,-3.44425556495067,
48.7857063762255));
#63532=CARTESIAN_POINT('Ctrl Pts',(-7.20390364148951,-3.26920377525388,
48.7780060608346));
#63533=CARTESIAN_POINT('Ctrl Pts',(-7.28333949548774,-3.0941616924647,48.7703061724387));
#63534=CARTESIAN_POINT('Ctrl Pts',(-7.35639744499141,-2.91620965562223,
48.7626062840429));
#63535=CARTESIAN_POINT('Ctrl Pts',(-7.42286640105598,-2.73586830678567,
48.754906395647));
#63536=CARTESIAN_POINT('Ctrl Pts',(-7.489344020102,-2.55550345383751,48.7472055037152));
#63537=CARTESIAN_POINT('Ctrl Pts',(-7.54923081163289,-2.37274900903136,
48.7395046117833));
#63538=CARTESIAN_POINT('Ctrl Pts',(-7.602364917705,-2.18814274169858,48.7318037198515));
#63539=CARTESIAN_POINT('Ctrl Pts',(-7.65554123721299,-2.003389810285,48.7240967097945));
#63540=CARTESIAN_POINT('Ctrl Pts',(-7.70195405461654,-1.81678246596557,
48.7163896997376));
#63541=CARTESIAN_POINT('Ctrl Pts',(-7.74149201967497,-1.62887148336163,
48.7086826896806));
#63542=CARTESIAN_POINT('Ctrl Pts',(-7.78104603419266,-1.44088422294079,
48.7009725511535));
#63543=CARTESIAN_POINT('Ctrl Pts',(-7.81371957484111,-1.25159262641768,
48.6932624126264));
#63544=CARTESIAN_POINT('Ctrl Pts',(-7.83945298081485,-1.06155450241292,
48.6855522740993));
#63545=CARTESIAN_POINT('Ctrl Pts',(-7.86521824036993,-0.871281143521426,
48.6778325917316));
#63546=CARTESIAN_POINT('Ctrl Pts',(-7.88402616789796,-0.680259771110366,
48.6701129093639));
#63547=CARTESIAN_POINT('Ctrl Pts',(-7.89586916802662,-0.489051205301197,
48.6623932269962));
#63548=CARTESIAN_POINT('Ctrl Pts',(-7.90602630093594,-0.325061439598059,
48.6557724519413));
#63549=CARTESIAN_POINT('Ctrl Pts',(-7.91106117209866,-0.160934124743805,
48.6491516768865));
#63550=CARTESIAN_POINT('Ctrl Pts',(-7.91099943894101,0.00297944206225246,
48.6425309018316));
#63551=CARTESIAN_POINT('',(-7.89861493486562,-0.000610740782857052,44.6422669711751));
#63552=CARTESIAN_POINT('Ctrl Pts',(-7.91099937608635,0.00314190409447718,
48.6471968050444));
#63553=CARTESIAN_POINT('Ctrl Pts',(-7.91088721046558,0.285563686941826,
48.6372769727183));
#63554=CARTESIAN_POINT('Ctrl Pts',(-7.89565139589759,0.567761009271943,
48.6270474731004));
#63555=CARTESIAN_POINT('Ctrl Pts',(-7.85923996448297,0.905277399101737,
48.6138200189015));
#63556=CARTESIAN_POINT('Ctrl Pts',(-7.85250280932996,0.961966380417291,
48.6115642746992));
#63557=CARTESIAN_POINT('Ctrl Pts',(-7.84425755833575,1.02547194602397,48.6089941122671));
#63558=CARTESIAN_POINT('Ctrl Pts',(-7.84335315319302,1.03236653728107,48.608714506237));
#63559=CARTESIAN_POINT('Ctrl Pts',(-7.84186956477895,1.04356195870714,48.608259540743));
#63560=CARTESIAN_POINT('Ctrl Pts',(-7.84129592913883,1.04786353319166,48.6080845051546));
#63561=CARTESIAN_POINT('Ctrl Pts',(-7.84028428023256,1.05540232927292,48.6077773442198));
#63562=CARTESIAN_POINT('Ctrl Pts',(-7.83984780029141,1.058639759172,48.6076453091428));
#63563=CARTESIAN_POINT('Ctrl Pts',(-7.83896453275709,1.06516056742372,48.6073791032273));
#63564=CARTESIAN_POINT('Ctrl Pts',(-7.83851768725474,1.06844393710996,48.6072449289816));
#63565=CARTESIAN_POINT('Ctrl Pts',(-7.83765246954365,1.07477170136458,48.606986086716));
#63566=CARTESIAN_POINT('Ctrl Pts',(-7.83723438754337,1.07781612440499,48.6068614361949));
#63567=CARTESIAN_POINT('Ctrl Pts',(-7.8362366696263,1.08505011221129,48.6065649733085));
#63568=CARTESIAN_POINT('Ctrl Pts',(-7.8356554490285,1.08923944675882,48.6063930669918));
#63569=CARTESIAN_POINT('Ctrl Pts',(-7.83359068371568,1.10403473098796,48.6057851838064));
#63570=CARTESIAN_POINT('Ctrl Pts',(-7.83208896872543,1.11463808969363,48.6053481345194));
#63571=CARTESIAN_POINT('Ctrl Pts',(-7.8127078075982,1.24951214628098,48.5997714147074));
#63572=CARTESIAN_POINT('Ctrl Pts',(-7.79189486900127,1.37333720840431,48.594462778753));
#63573=CARTESIAN_POINT('Ctrl Pts',(-7.76496296691875,1.51312726990638,48.5882966040542));
#63574=CARTESIAN_POINT('Ctrl Pts',(-7.76172771917633,1.52963617241184,48.5875656365673));
#63575=CARTESIAN_POINT('Ctrl Pts',(-7.7543746149077,1.56653374870656,48.585925942423));
#63576=CARTESIAN_POINT('Ctrl Pts',(-7.75022896540084,1.58691670400343,48.5850160565843));
#63577=CARTESIAN_POINT('Ctrl Pts',(-7.71473713820974,1.75796300598614,48.5773476381108));
#63578=CARTESIAN_POINT('Ctrl Pts',(-7.67908238742702,1.90769311658165,48.5704201986618));
#63579=CARTESIAN_POINT('Ctrl Pts',(-7.63278398310707,2.07969165962441,48.5622841826174));
#63580=CARTESIAN_POINT('Ctrl Pts',(-7.62637497954438,2.1030723698496,48.5611743431005));
#63581=CARTESIAN_POINT('Ctrl Pts',(-7.42692231684401,2.81779422459459,48.5271362686909));
#63582=CARTESIAN_POINT('Ctrl Pts',(-7.14074121909561,3.47983008713342,48.4928118545262));
#63583=CARTESIAN_POINT('Ctrl Pts',(-6.63083032079658,4.32290000599168,48.4499025809316));
#63584=CARTESIAN_POINT('Ctrl Pts',(-6.48097897180199,4.54448080227559,48.4386618443156));
#63585=CARTESIAN_POINT('Ctrl Pts',(-6.30896901439826,4.77296330526061,48.4271035690781));
#63586=CARTESIAN_POINT('Ctrl Pts',(-6.29770065654915,4.787821548977,48.4263520433476));
#63587=CARTESIAN_POINT('Ctrl Pts',(-6.28140751667153,4.80914833346166,48.4252734678862));
#63588=CARTESIAN_POINT('Ctrl Pts',(-6.2764251030701,4.81564907461297,48.4249447180951));
#63589=CARTESIAN_POINT('Ctrl Pts',(-6.26775467847249,4.82692538761249,48.424374488408));
#63590=CARTESIAN_POINT('Ctrl Pts',(-6.26407128762613,4.83170449332727,48.4241328229148));
#63591=CARTESIAN_POINT('Ctrl Pts',(-6.25697464745524,4.84089044820499,48.4236683299806));
#63592=CARTESIAN_POINT('Ctrl Pts',(-6.25356220216553,4.84529791181364,48.423445470393));
#63593=CARTESIAN_POINT('Ctrl Pts',(-6.24550736329436,4.85567873811038,48.4229205860536));
#63594=CARTESIAN_POINT('Ctrl Pts',(-6.24086104988281,4.86164906067754,48.4226187197296));
#63595=CARTESIAN_POINT('Ctrl Pts',(-6.22474727712517,4.88229343295764,48.421574946252));
#63596=CARTESIAN_POINT('Ctrl Pts',(-6.21323652875118,4.89693370115999,48.4208347904964));
#63597=CARTESIAN_POINT('Ctrl Pts',(-6.08305399232213,5.06131203842615,48.4125247209952));
#63598=CARTESIAN_POINT('Ctrl Pts',(-5.95904278837199,5.20674951721812,48.4051769750983));
#63599=CARTESIAN_POINT('Ctrl Pts',(-5.58633867340523,5.61306949347952,48.3845315118996));
#63600=CARTESIAN_POINT('Ctrl Pts',(-5.3249341083309,5.86164033785009,48.3717704744258));
#63601=CARTESIAN_POINT('Ctrl Pts',(-4.72289078532052,6.36049727373689,48.3446445744573));
#63602=CARTESIAN_POINT('Ctrl Pts',(-4.37732995373802,6.60307375551591,48.330421893523));
#63603=CARTESIAN_POINT('Ctrl Pts',(-3.89722039962396,6.88578192154127,48.3105195163111));
#63604=CARTESIAN_POINT('Ctrl Pts',(-3.77859021653241,6.95158782467247,48.3055879704141));
#63605=CARTESIAN_POINT('Ctrl Pts',(-3.58982729169156,7.05003760696387,48.2976356971118));
#63606=CARTESIAN_POINT('Ctrl Pts',(-3.52080559709052,7.08475953216976,48.2947064126986));
#63607=CARTESIAN_POINT('Ctrl Pts',(-3.40243411480107,7.14215029536211,48.2896291077993));
#63608=CARTESIAN_POINT('Ctrl Pts',(-3.3533385107872,7.16533248214319,48.2875075028415));
#63609=CARTESIAN_POINT('Ctrl Pts',(-3.27449862031682,7.20157167018213,48.2840714610069));
#63610=CARTESIAN_POINT('Ctrl Pts',(-3.24490709516551,7.21495347386696,48.2827756273708));
#63611=CARTESIAN_POINT('Ctrl Pts',(-3.20761990210326,7.23153960203846,48.2811358016783));
#63612=CARTESIAN_POINT('Ctrl Pts',(-3.20000011862806,7.23491462922697,48.2808003313775));
#63613=CARTESIAN_POINT('Ctrl Pts',(-3.18860146669585,7.23994189868385,48.2802979601863));
#63614=CARTESIAN_POINT('Ctrl Pts',(-3.18482659944905,7.24160324383208,48.2801315039591));
#63615=CARTESIAN_POINT('Ctrl Pts',(-3.17712425666305,7.24498591066743,48.2797916870253));
#63616=CARTESIAN_POINT('Ctrl Pts',(-3.17319667763026,7.24670699235288,48.2796183147993));
#63617=CARTESIAN_POINT('Ctrl Pts',(-3.16472024820349,7.25041318707886,48.2792439488039));
#63618=CARTESIAN_POINT('Ctrl Pts',(-3.16017092694726,7.25239721368527,48.2790429032041));
#63619=CARTESIAN_POINT('Ctrl Pts',(-3.14793694902274,7.25771893636277,48.2785019303997));
#63620=CARTESIAN_POINT('Ctrl Pts',(-3.14024886584955,7.26104870208256,48.2781616291837));
#63621=CARTESIAN_POINT('Ctrl Pts',(-3.10509030739884,7.27620985076921,48.276603868408));
#63622=CARTESIAN_POINT('Ctrl Pts',(-3.07755839665891,7.28789749452489,48.275379780911));
#63623=CARTESIAN_POINT('Ctrl Pts',(-2.99276416413623,7.32332754355644,48.2715981228162));
#63624=CARTESIAN_POINT('Ctrl Pts',(-2.93528925475976,7.34655295842242,48.2690186171086));
#63625=CARTESIAN_POINT('Ctrl Pts',(-2.79197971761151,7.40251367595795,48.262556081804));
#63626=CARTESIAN_POINT('Ctrl Pts',(-2.70583728182034,7.43443362697497,48.2586444768703));
#63627=CARTESIAN_POINT('Ctrl Pts',(-2.25282967941924,7.59337859246078,48.2379943958161));
#63628=CARTESIAN_POINT('Ctrl Pts',(-1.87754123797349,7.69476896676719,48.2206460470832));
#63629=CARTESIAN_POINT('Ctrl Pts',(-1.4500534414654,7.77711305912955,48.2013623308277));
#63630=CARTESIAN_POINT('Ctrl Pts',(-1.40369240250953,7.78561430968249,48.1992767220109));
#63631=CARTESIAN_POINT('Ctrl Pts',(-1.30264374679526,7.80321173937491,48.194745025025));
#63632=CARTESIAN_POINT('Ctrl Pts',(-1.24793075909471,7.81214842748517,48.1923002837688));
#63633=CARTESIAN_POINT('Ctrl Pts',(-1.12686412053039,7.83061883731462,48.1869128409071));
#63634=CARTESIAN_POINT('Ctrl Pts',(-1.06047387089712,7.83988580345395,48.1839731525093));
#63635=CARTESIAN_POINT('Ctrl Pts',(-0.909683116964655,7.85898316850082,
48.1773330869217));
#63636=CARTESIAN_POINT('Ctrl Pts',(-0.825225463909605,7.86829988341015,
48.1736400511637));
#63637=CARTESIAN_POINT('Ctrl Pts',(-0.621717635841421,7.88743647435205,
48.1648094599451));
#63638=CARTESIAN_POINT('Ctrl Pts',(-0.502562140077705,7.89592421825133,
48.1596950893038));
#63639=CARTESIAN_POINT('Ctrl Pts',(-0.17637824849564,7.91174516962143,48.1458553765805));
#63640=CARTESIAN_POINT('Ctrl Pts',(0.030821625607908,7.91365129023093,48.1372426468061));
#63641=CARTESIAN_POINT('Ctrl Pts',(0.294789407222997,7.90571081779369,48.1264791180981));
#63642=CARTESIAN_POINT('Ctrl Pts',(0.351694234569414,7.90338380774433,48.1241709485929));
#63643=CARTESIAN_POINT('Ctrl Pts',(0.42529106922276,7.89957776498674,48.1212004553319));
#63644=CARTESIAN_POINT('Ctrl Pts',(0.442009892778786,7.89865992534494,48.1205266387112));
#63645=CARTESIAN_POINT('Ctrl Pts',(0.469050676289211,7.89708930096658,48.1194383704988));
#63646=CARTESIAN_POINT('Ctrl Pts',(0.479374462665852,7.89646934329486,48.1190232514962));
#63647=CARTESIAN_POINT('Ctrl Pts',(0.499081288172488,7.89524713172535,48.1182315291213));
#63648=CARTESIAN_POINT('Ctrl Pts',(0.508464530459459,7.89464839147685,48.1178548544885));
#63649=CARTESIAN_POINT('Ctrl Pts',(0.529815503356921,7.89324777270262,48.1169984284899));
#63650=CARTESIAN_POINT('Ctrl Pts',(0.541782533979159,7.89243540080057,48.1165188911918));
#63651=CARTESIAN_POINT('Ctrl Pts',(0.577321298024332,7.88994167088033,48.1150962230125));
#63652=CARTESIAN_POINT('Ctrl Pts',(0.600887457167115,7.88818190225193,48.1141546980934));
#63653=CARTESIAN_POINT('Ctrl Pts',(0.764257205336719,7.8752461422618,48.1076404492136));
#63654=CARTESIAN_POINT('Ctrl Pts',(0.903752443465567,7.86045953334619,48.1021436763652));
#63655=CARTESIAN_POINT('Ctrl Pts',(1.6469122255149,7.76163807512629,48.0731613590942));
#63656=CARTESIAN_POINT('Ctrl Pts',(2.23972135571986,7.61176833761153,48.0513151149297));
#63657=CARTESIAN_POINT('Ctrl Pts',(3.07314921220822,7.29515198038458,48.0190101585542));
#63658=CARTESIAN_POINT('Ctrl Pts',(3.33128403201259,7.1809486785566,48.0087243526581));
#63659=CARTESIAN_POINT('Ctrl Pts',(3.68152602898821,7.00303929452204,47.9938125844243));
#63660=CARTESIAN_POINT('Ctrl Pts',(3.77922709314576,6.95080099906397,47.9895433387148));
#63661=CARTESIAN_POINT('Ctrl Pts',(3.90639103690575,6.87933585053109,47.9838050285108));
#63662=CARTESIAN_POINT('Ctrl Pts',(3.93687077707966,6.86193858256721,47.9824156055327));
#63663=CARTESIAN_POINT('Ctrl Pts',(3.98027494489441,6.83677991367922,47.9804156408983));
#63664=CARTESIAN_POINT('Ctrl Pts',(3.99329477109151,6.8291833400393,47.9798129471165));
#63665=CARTESIAN_POINT('Ctrl Pts',(4.01329072887739,6.81743972387717,47.9788829475732));
#63666=CARTESIAN_POINT('Ctrl Pts',(4.0202823674889,6.81331905521461,47.9785569446317));
#63667=CARTESIAN_POINT('Ctrl Pts',(4.03326832778059,6.80563855934635,47.9779498832717));
#63668=CARTESIAN_POINT('Ctrl Pts',(4.03926431318597,6.80208154994561,47.9776689668664));
#63669=CARTESIAN_POINT('Ctrl Pts',(4.04917210228179,6.79618621405542,47.9772037434508));
#63670=CARTESIAN_POINT('Ctrl Pts',(4.05308660919297,6.79385242025956,47.9770196685798));
#63671=CARTESIAN_POINT('Ctrl Pts',(4.06076152322341,6.78926771153022,47.9766582354467));
#63672=CARTESIAN_POINT('Ctrl Pts',(4.06452208130228,6.78701705153371,47.9764808904026));
#63673=CARTESIAN_POINT('Ctrl Pts',(4.07322480718344,6.78179872174675,47.9760698936315));
#63674=CARTESIAN_POINT('Ctrl Pts',(4.07816560109326,6.77882877508604,47.9758361228778));
#63675=CARTESIAN_POINT('Ctrl Pts',(4.09407120719461,6.76924411822539,47.9750821409098));
#63676=CARTESIAN_POINT('Ctrl Pts',(4.10502316462872,6.76260820959545,47.9745608065324));
#63677=CARTESIAN_POINT('Ctrl Pts',(4.22080459428456,6.69207010530995,47.9690258830486));
#63678=CARTESIAN_POINT('Ctrl Pts',(4.32413488139296,6.62577136506182,47.9638711596446));
#63679=CARTESIAN_POINT('Ctrl Pts',(4.85884722843049,6.26485385073044,47.9361350953094));
#63680=CARTESIAN_POINT('Ctrl Pts',(5.26178922828531,5.93045751736016,47.9116917965391));
#63681=CARTESIAN_POINT('Ctrl Pts',(5.64834048177626,5.53903808415139,47.8864166317572));
#63682=CARTESIAN_POINT('Ctrl Pts',(5.6677609939118,5.51916464859386,47.88514114323));
#63683=CARTESIAN_POINT('Ctrl Pts',(5.70801223592311,5.47753816892919,47.8824861568855));
#63684=CARTESIAN_POINT('Ctrl Pts',(5.72882427929581,5.45576763295687,47.881106931163));
#63685=CARTESIAN_POINT('Ctrl Pts',(5.79928634076314,5.38121270498719,47.8764161431193));
#63686=CARTESIAN_POINT('Ctrl Pts',(5.84833556943622,5.32786481566565,47.8731145856143));
#63687=CARTESIAN_POINT('Ctrl Pts',(5.96593172055449,5.19638159423117,47.8651174537263));
#63688=CARTESIAN_POINT('Ctrl Pts',(6.0336858454794,5.11755398914653,47.8604399195119));
#63689=CARTESIAN_POINT('Ctrl Pts',(6.22219747362919,4.8892828247905,47.8472439583703));
#63690=CARTESIAN_POINT('Ctrl Pts',(6.33909478434824,4.73674059261592,47.8388396148963));
#63691=CARTESIAN_POINT('Ctrl Pts',(6.55282235508251,4.43573912994225,47.8230806209574));
#63692=CARTESIAN_POINT('Ctrl Pts',(6.65044670928969,4.2879862905131,47.8156995897879));
#63693=CARTESIAN_POINT('Ctrl Pts',(6.75959729366131,4.11008131149444,47.8072206700339));
#63694=CARTESIAN_POINT('Ctrl Pts',(6.77599683018701,4.08298799262269,47.8059402054002));
#63695=CARTESIAN_POINT('Ctrl Pts',(6.79741421437031,4.04712034894147,47.8042591540958));
#63696=CARTESIAN_POINT('Ctrl Pts',(6.80257845141105,4.03843404476803,47.8038531269772));
#63697=CARTESIAN_POINT('Ctrl Pts',(6.81100107311602,4.0242051040034,47.803189785819));
#63698=CARTESIAN_POINT('Ctrl Pts',(6.81426936213079,4.01866836124332,47.802932104313));
#63699=CARTESIAN_POINT('Ctrl Pts',(6.82056844848896,4.00796742674824,47.8024349213729));
#63700=CARTESIAN_POINT('Ctrl Pts',(6.82360013882355,4.00280376736772,47.8021953869255));
#63701=CARTESIAN_POINT('Ctrl Pts',(6.8305557051682,3.99092598711178,47.801645260455));
#63702=CARTESIAN_POINT('Ctrl Pts',(6.83447555244873,3.98420950747386,47.8013348177207));
#63703=CARTESIAN_POINT('Ctrl Pts',(6.84489011194071,3.96630403897546,47.8005088942975));
#63704=CARTESIAN_POINT('Ctrl Pts',(6.85136730420453,3.95510485816732,47.7999940614729));
#63705=CARTESIAN_POINT('Ctrl Pts',(6.87215546145045,3.91895745406219,47.7983379551569));
#63706=CARTESIAN_POINT('Ctrl Pts',(6.88635793025572,3.89394692981299,47.7972006811843));
#63707=CARTESIAN_POINT('Ctrl Pts',(7.15142878931303,3.42117159650883,47.7758624602311));
#63708=CARTESIAN_POINT('Ctrl Pts',(7.35827922229107,2.95011072057071,47.7574079628831));
#63709=CARTESIAN_POINT('Ctrl Pts',(7.60649418201631,2.19223900328639,47.7299201064291));
#63710=CARTESIAN_POINT('Ctrl Pts',(7.68032382267733,1.91762675162704,47.7203536042651));
#63711=CARTESIAN_POINT('Ctrl Pts',(7.79577654976965,1.37268149497652,47.7013822521474));
#63712=CARTESIAN_POINT('Ctrl Pts',(7.83848185921121,1.10298549138838,47.691996410984));
#63713=CARTESIAN_POINT('Ctrl Pts',(7.88968194476937,0.618638925296452,47.6744061477431));
#63714=CARTESIAN_POINT('Ctrl Pts',(7.90353688832454,0.40483022463031,47.6663870864262));
#63715=CARTESIAN_POINT('Ctrl Pts',(7.90933487662088,0.164425106429818,47.6568407385094));
#63716=CARTESIAN_POINT('Ctrl Pts',(7.90983816036681,0.138108840181999,47.6557886089252));
#63717=CARTESIAN_POINT('Ctrl Pts',(7.91030052551998,0.105392338829513,47.6544712285875));
#63718=CARTESIAN_POINT('Ctrl Pts',(7.91038318847114,0.0989937382490356,
47.654213133667));
#63719=CARTESIAN_POINT('Ctrl Pts',(7.91049451209835,0.0894832863733912,
47.6538288478653));
#63720=CARTESIAN_POINT('Ctrl Pts',(7.91052910048243,0.0863714932411258,
47.6537030038978));
#63721=CARTESIAN_POINT('Ctrl Pts',(7.9105927543886,0.0803236903608817,47.6534582160627));
#63722=CARTESIAN_POINT('Ctrl Pts',(7.91062202150291,0.0773876854483604,
47.6533392841217));
#63723=CARTESIAN_POINT('Ctrl Pts',(7.91067963600495,0.0712660210728465,
47.6530911087428));
#63724=CARTESIAN_POINT('Ctrl Pts',(7.91070769362919,0.068080358112815,47.6529618482937));
#63725=CARTESIAN_POINT('Ctrl Pts',(7.91077959104164,0.0593159838862543,
47.6526059213124));
#63726=CARTESIAN_POINT('Ctrl Pts',(7.9108194538566,0.0537372511366036,47.6523790236603));
#63727=CARTESIAN_POINT('Ctrl Pts',(7.91095083274186,0.0321560304680096,
47.6514999661282));
#63728=CARTESIAN_POINT('Ctrl Pts',(7.91099969336156,0.0161534191598449,
47.6508453567158));
#63729=CARTESIAN_POINT('Ctrl Pts',(7.91100477424842,-0.250248746012721,
47.6399028293494));
#63730=CARTESIAN_POINT('Ctrl Pts',(7.8991209536246,-0.500488600898607,47.6289658715112));
#63731=CARTESIAN_POINT('Ctrl Pts',(7.81910148450312,-1.34104792581877,47.5909963376035));
#63732=CARTESIAN_POINT('Ctrl Pts',(7.69639076454295,-1.9241624603802,47.5627575848675));
#63733=CARTESIAN_POINT('Ctrl Pts',(7.40981353914708,-2.78911340422794,47.5218229379346));
#63734=CARTESIAN_POINT('Ctrl Pts',(7.29205781415525,-3.08389578830358,47.5080168173924));
#63735=CARTESIAN_POINT('Ctrl Pts',(7.11104079998649,-3.46822852514133,47.4903388075217));
#63736=CARTESIAN_POINT('Ctrl Pts',(7.06318571930844,-3.56467657678949,47.4859291204014));
#63737=CARTESIAN_POINT('Ctrl Pts',(7.00660087830228,-3.6731021699837,47.4809998663061));
#63738=CARTESIAN_POINT('Ctrl Pts',(6.99979003808101,-3.68606495396276,47.4804110082937));
#63739=CARTESIAN_POINT('Ctrl Pts',(6.9894912852694,-3.70553465451106,47.4795272360412));
#63740=CARTESIAN_POINT('Ctrl Pts',(6.98603020962882,-3.71205568562662,47.4792313462821));
#63741=CARTESIAN_POINT('Ctrl Pts',(6.98005691548964,-3.723272057439,47.4787226011407));
#63742=CARTESIAN_POINT('Ctrl Pts',(6.97754907830417,-3.72796971784579,47.4785095863675));
#63743=CARTESIAN_POINT('Ctrl Pts',(6.97237019710205,-3.73764722355843,47.4780708812793));
#63744=CARTESIAN_POINT('Ctrl Pts',(6.96969855624922,-3.74262674713997,47.4778452129005));
#63745=CARTESIAN_POINT('Ctrl Pts',(6.96248399017405,-3.7560390621629,47.4772375518502));
#63746=CARTESIAN_POINT('Ctrl Pts',(6.95793107428815,-3.76446648493944,47.4768559243261));
#63747=CARTESIAN_POINT('Ctrl Pts',(6.94114731557598,-3.79539866141476,47.4754558668672));
#63748=CARTESIAN_POINT('Ctrl Pts',(6.92882244076337,-3.81785236174675,47.4744408805198));
#63749=CARTESIAN_POINT('Ctrl Pts',(6.73308272085197,-4.17038498500779,47.4585248608936));
#63750=CARTESIAN_POINT('Ctrl Pts',(6.52636836969631,-4.48698880418757,47.4445391321518));
#63751=CARTESIAN_POINT('Ctrl Pts',(6.16255302411474,-4.96556252384246,47.4231909295439));
#63752=CARTESIAN_POINT('Ctrl Pts',(6.01981544687402,-5.13767424317418,47.4154568440733));
#63753=CARTESIAN_POINT('Ctrl Pts',(5.65474529316149,-5.5417373434592,47.3967652757463));
#63754=CARTESIAN_POINT('Ctrl Pts',(5.42521398064285,-5.76663174778966,47.3858976714903));
#63755=CARTESIAN_POINT('Ctrl Pts',(4.93373373572088,-6.19279789274453,47.3630361657022));
#63756=CARTESIAN_POINT('Ctrl Pts',(4.67158810927335,-6.39286311395369,47.3510373574941));
#63757=CARTESIAN_POINT('Ctrl Pts',(4.3889127272084,-6.58190545892171,47.3374574438699));
#63758=CARTESIAN_POINT('Ctrl Pts',(4.38004904190869,-6.58780728206612,47.3370309989742));
#63759=CARTESIAN_POINT('Ctrl Pts',(4.36439557378502,-6.59818447800528,47.3362767326171));
#63760=CARTESIAN_POINT('Ctrl Pts',(4.35761072934331,-6.60266732929056,47.3359494216729));
#63761=CARTESIAN_POINT('Ctrl Pts',(4.34731421420031,-6.60944761178649,47.3354521059797));
#63762=CARTESIAN_POINT('Ctrl Pts',(4.34380760277923,-6.61175272676108,47.3352826342853));
#63763=CARTESIAN_POINT('Ctrl Pts',(4.33774287577367,-6.61573254389019,47.3349893529826));
#63764=CARTESIAN_POINT('Ctrl Pts',(4.33518561665835,-6.61740855756204,47.3348656330602));
#63765=CARTESIAN_POINT('Ctrl Pts',(4.32994350924534,-6.6208398633572,47.334611909692));
#63766=CARTESIAN_POINT('Ctrl Pts',(4.32725856496361,-6.62259500508461,47.3344818961613));
#63767=CARTESIAN_POINT('Ctrl Pts',(4.32083508546776,-6.62678844434955,47.3341707101968));
#63768=CARTESIAN_POINT('Ctrl Pts',(4.31709555650466,-6.62922520947093,47.3339894345693));
#63769=CARTESIAN_POINT('Ctrl Pts',(4.30574988725227,-6.63660464333036,47.3334391073623));
#63770=CARTESIAN_POINT('Ctrl Pts',(4.29813733114477,-6.64153737960748,47.3330693938454));
#63771=CARTESIAN_POINT('Ctrl Pts',(4.2197393895256,-6.69214594442403,47.3292572874959));
#63772=CARTESIAN_POINT('Ctrl Pts',(4.14823946307442,-6.73669995384896,47.3257420135045));
#63773=CARTESIAN_POINT('Ctrl Pts',(3.97009734239516,-6.84379497042627,47.3169169727176));
#63774=CARTESIAN_POINT('Ctrl Pts',(3.86267611333562,-6.90499336531258,47.3115378381864));
#63775=CARTESIAN_POINT('Ctrl Pts',(3.11232979114476,-7.30948000298624,47.2738045112072));
#63776=CARTESIAN_POINT('Ctrl Pts',(2.42606091939876,-7.56501890904921,47.238893713967));
#63777=CARTESIAN_POINT('Ctrl Pts',(1.41079622591448,-7.79039905737326,47.1929630832285));
#63778=CARTESIAN_POINT('Ctrl Pts',(1.10342509319658,-7.8398434252781,47.1796982723357));
#63779=CARTESIAN_POINT('Ctrl Pts',(0.74925910478261,-7.87556640918489,47.1651751942411));
#63780=CARTESIAN_POINT('Ctrl Pts',(0.704564844888434,-7.87969059906658,
47.163355856108));
#63781=CARTESIAN_POINT('Ctrl Pts',(0.648182891380866,-7.88440972545541,
47.1610773389292));
#63782=CARTESIAN_POINT('Ctrl Pts',(0.63652618443597,-7.88535935754181,47.1606071581899));
#63783=CARTESIAN_POINT('Ctrl Pts',(0.617971488106171,-7.88682953358245,
47.1598601536594));
#63784=CARTESIAN_POINT('Ctrl Pts',(0.611074869267015,-7.88736688359064,
47.1595828087022));
#63785=CARTESIAN_POINT('Ctrl Pts',(0.598084553654909,-7.88836188375041,
47.1590609898046));
#63786=CARTESIAN_POINT('Ctrl Pts',(0.591991016696638,-7.88882152027104,
47.1588164544426));
#63787=CARTESIAN_POINT('Ctrl Pts',(0.578294728702754,-7.8898386751054,47.1582673583399));
#63788=CARTESIAN_POINT('Ctrl Pts',(0.570691687346488,-7.89039226596766,
47.157962919541));
#63789=CARTESIAN_POINT('Ctrl Pts',(0.551362985804402,-7.89177153940778,
47.1571899108786));
#63790=CARTESIAN_POINT('Ctrl Pts',(0.539636245587326,-7.89258208042732,
47.1567218102988));
#63791=CARTESIAN_POINT('Ctrl Pts',(0.474917751151294,-7.89691044808477,
47.1541432621886));
#63792=CARTESIAN_POINT('Ctrl Pts',(0.421892837630961,-7.899920763264,47.152048544574));
#63793=CARTESIAN_POINT('Ctrl Pts',(-0.472329576491392,-7.94165820869696,
47.1170129571966));
#63794=CARTESIAN_POINT('Ctrl Pts',(-1.31426262356121,-7.84637854832496,
47.0891281908939));
#63795=CARTESIAN_POINT('Ctrl Pts',(-2.39647098960759,-7.54453962645387,
47.0495012253935));
#63796=CARTESIAN_POINT('Ctrl Pts',(-2.6633563306627,-7.4545063047418,47.0393229717895));
#63797=CARTESIAN_POINT('Ctrl Pts',(-3.00094434289365,-7.32017485820054,
47.0252963779983));
#63798=CARTESIAN_POINT('Ctrl Pts',(-3.07655450506013,-7.2887199470262,47.0220774014341));
#63799=CARTESIAN_POINT('Ctrl Pts',(-3.15998510632024,-7.25248216148423,
47.0184251693154));
#63800=CARTESIAN_POINT('Ctrl Pts',(-3.16830355362299,-7.24885204468059,
47.0180599065823));
#63801=CARTESIAN_POINT('Ctrl Pts',(-3.18066630040037,-7.24343167613642,
47.0175153710854));
#63802=CARTESIAN_POINT('Ctrl Pts',(-3.18471539910629,-7.24165232442901,
47.0173367528613));
#63803=CARTESIAN_POINT('Ctrl Pts',(-3.1916294392087,-7.23860707133666,47.0170312890721));
#63804=CARTESIAN_POINT('Ctrl Pts',(-3.19449512913079,-7.23734286049725,
47.0169045458854));
#63805=CARTESIAN_POINT('Ctrl Pts',(-3.20037665482123,-7.23474402751933,
47.0166441377637));
#63806=CARTESIAN_POINT('Ctrl Pts',(-3.20339240057618,-7.23340922417114,
47.0165104621253));
#63807=CARTESIAN_POINT('Ctrl Pts',(-3.21063986389414,-7.23019599321715,
47.0161888487613));
#63808=CARTESIAN_POINT('Ctrl Pts',(-3.21487076458554,-7.22831573762523,
47.0160008006189));
#63809=CARTESIAN_POINT('Ctrl Pts',(-3.2302523669204,-7.22146381987513,47.0153160679354));
#63810=CARTESIAN_POINT('Ctrl Pts',(-3.24139315815675,-7.21647008217896,
47.0148180618169));
#63811=CARTESIAN_POINT('Ctrl Pts',(-3.41380489813097,-7.13870860837326,
47.0070796647416));
#63812=CARTESIAN_POINT('Ctrl Pts',(-3.57259250770177,-7.06058068783148,
46.9995273596727));
#63813=CARTESIAN_POINT('Ctrl Pts',(-4.39908478511926,-6.61890309859251,
46.9584633062142));
#63814=CARTESIAN_POINT('Ctrl Pts',(-5.01443691017841,-6.16583135000306,
46.9221278095568));
#63815=CARTESIAN_POINT('Ctrl Pts',(-5.71043494809567,-5.47924058558368,
46.8793431069405));
#63816=CARTESIAN_POINT('Ctrl Pts',(-5.85879097719294,-5.32031224824233,
46.870063123635));
#63817=CARTESIAN_POINT('Ctrl Pts',(-6.06284906827188,-5.08281009042416,
46.8570838693297));
#63818=CARTESIAN_POINT('Ctrl Pts',(-6.12395204180475,-5.00902280567634,
46.8531663871853));
#63819=CARTESIAN_POINT('Ctrl Pts',(-6.19285003734239,-4.92267656618556,
46.8487110122654));
#63820=CARTESIAN_POINT('Ctrl Pts',(-6.20196690305786,-4.91118546754688,
46.848120662449));
#63821=CARTESIAN_POINT('Ctrl Pts',(-6.21573598630445,-4.89373112758165,
46.847227840397));
#63822=CARTESIAN_POINT('Ctrl Pts',(-6.22041167539806,-4.88778649180598,
46.846924441389));
#63823=CARTESIAN_POINT('Ctrl Pts',(-6.22881219868047,-4.8770745529271,46.8463789520101));
#63824=CARTESIAN_POINT('Ctrl Pts',(-6.23254009964859,-4.87230966870131,
46.8461367408754));
#63825=CARTESIAN_POINT('Ctrl Pts',(-6.24053214640193,-4.86207030824909,
46.8456171764835));
#63826=CARTESIAN_POINT('Ctrl Pts',(-6.24479456414573,-4.85659448632093,
46.8453398912662));
#63827=CARTESIAN_POINT('Ctrl Pts',(-6.25628100697458,-4.84179801544654,
46.8445921555585));
#63828=CARTESIAN_POINT('Ctrl Pts',(-6.26349141812948,-4.8324667942123,46.8441222394033));
#63829=CARTESIAN_POINT('Ctrl Pts',(-6.28976975759651,-4.79830154404987,
46.8424076360185));
#63830=CARTESIAN_POINT('Ctrl Pts',(-6.30871118790363,-4.77337034884639,
46.8411678937925));
#63831=CARTESIAN_POINT('Ctrl Pts',(-6.61209269558256,-4.36909159813067,
46.8212464697403));
#63832=CARTESIAN_POINT('Ctrl Pts',(-6.86202066896686,-3.9650303849528,46.8039940377157));
#63833=CARTESIAN_POINT('Ctrl Pts',(-7.30284478223114,-3.08433829828622,
46.7695523461206));
#63834=CARTESIAN_POINT('Ctrl Pts',(-7.4866504296468,-2.6066659584237,46.752543446868));
#63835=CARTESIAN_POINT('Ctrl Pts',(-7.66522043561788,-1.96293201441549,
46.7286005782283));
#63836=CARTESIAN_POINT('Ctrl Pts',(-7.70276356087339,-1.81000997970422,
46.7228336843915));
#63837=CARTESIAN_POINT('Ctrl Pts',(-7.75817318410624,-1.55118540512928,
46.7127978269462));
#63838=CARTESIAN_POINT('Ctrl Pts',(-7.77849185530214,-1.44585269489026,
46.7086379478401));
#63839=CARTESIAN_POINT('Ctrl Pts',(-7.79978152516121,-1.32199406141429,
46.7036256519453));
#63840=CARTESIAN_POINT('Ctrl Pts',(-7.80283778688522,-1.30383380835545,
46.7028877164963));
#63841=CARTESIAN_POINT('Ctrl Pts',(-7.80677141519388,-1.27995100885669,
46.7019130834933));
#63842=CARTESIAN_POINT('Ctrl Pts',(-7.80770596995518,-1.27423781161715,
46.701679620768));
#63843=CARTESIAN_POINT('Ctrl Pts',(-7.80922124737563,-1.26491023813689,
46.7012979432075));
#63844=CARTESIAN_POINT('Ctrl Pts',(-7.80980573529075,-1.26129646710877,
46.7011499434841));
#63845=CARTESIAN_POINT('Ctrl Pts',(-7.81092719964687,-1.25433201237616,
46.7008644721098));
#63846=CARTESIAN_POINT('Ctrl Pts',(-7.81146452904037,-1.25098138552524,
46.7007270207855));
#63847=CARTESIAN_POINT('Ctrl Pts',(-7.81269113813946,-1.24330101017495,
46.7004116981351));
#63848=CARTESIAN_POINT('Ctrl Pts',(-7.81337897442365,-1.23897103427697,
46.7002337433392));
#63849=CARTESIAN_POINT('Ctrl Pts',(-7.81556134363772,-1.22515877795945,
46.6996654868646));
#63850=CARTESIAN_POINT('Ctrl Pts',(-7.81704221201616,-1.2156743813109,46.6992743898585));
#63851=CARTESIAN_POINT('Ctrl Pts',(-7.8300968239229,-1.13105439358331,46.6957771884164));
#63852=CARTESIAN_POINT('Ctrl Pts',(-7.84060388370665,-1.05576054745434,
46.6926104264097));
#63853=CARTESIAN_POINT('Ctrl Pts',(-7.890692489434,-0.65467418587675,46.675494812044));
#63854=CARTESIAN_POINT('Ctrl Pts',(-7.91105429201082,-0.326825594517507,
46.6606534484356));
#63855=CARTESIAN_POINT('Ctrl Pts',(-7.91086344611451,0.824330149796626,
46.6077205462351));
#63856=CARTESIAN_POINT('Ctrl Pts',(-7.78228473438266,1.64252519945692,46.5693162931647));
#63857=CARTESIAN_POINT('Ctrl Pts',(-7.51327293775616,2.47740673728522,46.5334218007386));
#63858=CARTESIAN_POINT('Ctrl Pts',(-7.49625419425399,2.52843579870849,46.5312382504718));
#63859=CARTESIAN_POINT('Ctrl Pts',(-7.4749613761652,2.59017490666403,46.5286086037491));
#63860=CARTESIAN_POINT('Ctrl Pts',(-7.47118288529898,2.60105361693812,46.5281457092195));
#63861=CARTESIAN_POINT('Ctrl Pts',(-7.46493895531249,2.61890474916414,46.527386884856));
#63862=CARTESIAN_POINT('Ctrl Pts',(-7.46248747642138,2.62588201494009,46.527090480468));
#63863=CARTESIAN_POINT('Ctrl Pts',(-7.45806913171659,2.63840110798912,46.5265589874387));
#63864=CARTESIAN_POINT('Ctrl Pts',(-7.45610586545242,2.643944194469,46.5263237764266));
#63865=CARTESIAN_POINT('Ctrl Pts',(-7.45192400210159,2.65570956728015,46.5258247839785));
#63866=CARTESIAN_POINT('Ctrl Pts',(-7.44970378740904,2.66193127615737,46.5255610579146));
#63867=CARTESIAN_POINT('Ctrl Pts',(-7.44374982469739,2.67855027795454,46.5248570059581));
#63868=CARTESIAN_POINT('Ctrl Pts',(-7.44000208008678,2.68894256052886,46.5244171580344));
#63869=CARTESIAN_POINT('Ctrl Pts',(-7.42223573341392,2.73788612550479,46.5223475743764));
#63870=CARTESIAN_POINT('Ctrl Pts',(-7.40793906652687,2.77633617762917,46.5207273565077));
#63871=CARTESIAN_POINT('Ctrl Pts',(-7.297212151716,3.06718415758546,46.5085122452187));
#63872=CARTESIAN_POINT('Ctrl Pts',(-7.18820392417193,3.3146136978331,46.498363355946));
#63873=CARTESIAN_POINT('Ctrl Pts',(-6.98485245377564,3.71872894532755,46.4819508092894));
#63874=CARTESIAN_POINT('Ctrl Pts',(-6.89736631882546,3.87858863735505,46.4755013145465));
#63875=CARTESIAN_POINT('Ctrl Pts',(-6.44059589898921,4.64880988279558,46.4442768187746));
#63876=CARTESIAN_POINT('Ctrl Pts',(-5.99551034410751,5.21021025676115,46.4213247839597));
#63877=CARTESIAN_POINT('Ctrl Pts',(-5.42483124581693,5.75858182976693,46.3907942880829));
#63878=CARTESIAN_POINT('Ctrl Pts',(-5.36753929600187,5.81202029270604,46.3877157275242));
#63879=CARTESIAN_POINT('Ctrl Pts',(-5.30302508156673,5.87042770581425,46.3842217127422));
#63880=CARTESIAN_POINT('Ctrl Pts',(-5.29657560216107,5.87624738710179,46.3838721174856));
#63881=CARTESIAN_POINT('Ctrl Pts',(-5.28692053861367,5.88493081482364,46.3833482935992));
#63882=CARTESIAN_POINT('Ctrl Pts',(-5.28372216886451,5.88780260529554,46.3831746931267));
#63883=CARTESIAN_POINT('Ctrl Pts',(-5.278212903992,5.89274122562593,46.382875527095));
#63884=CARTESIAN_POINT('Ctrl Pts',(-5.27590312885451,5.89480930878551,46.3827500600273));
#63885=CARTESIAN_POINT('Ctrl Pts',(-5.27138136491089,5.89885313447831,46.3825043563886));
#63886=CARTESIAN_POINT('Ctrl Pts',(-5.26916947852634,5.90082899286552,46.3823841288657));
#63887=CARTESIAN_POINT('Ctrl Pts',(-5.2638057828561,5.90561491385036,46.3820924908241));
#63888=CARTESIAN_POINT('Ctrl Pts',(-5.26065284231471,5.90842369019273,46.381920979579));
#63889=CARTESIAN_POINT('Ctrl Pts',(-5.25088495113326,5.91711133482769,46.3813893973857));
#63890=CARTESIAN_POINT('Ctrl Pts',(-5.24426240363179,5.92298161059053,46.3810286546541));
#63891=CARTESIAN_POINT('Ctrl Pts',(-5.1679372087861,5.9904084738627,46.3768673837861));
#63892=CARTESIAN_POINT('Ctrl Pts',(-5.09716683176234,6.05074025532961,46.3729736168872));
#63893=CARTESIAN_POINT('Ctrl Pts',(-4.88192826333345,6.22777521300063,46.3610720092556));
#63894=CARTESIAN_POINT('Ctrl Pts',(-4.73440247048313,6.34064927503365,46.352837676472));
#63895=CARTESIAN_POINT('Ctrl Pts',(-4.46337130879253,6.53328374006013,46.3377777014192));
#63896=CARTESIAN_POINT('Ctrl Pts',(-4.34134906041434,6.61499555204926,46.3310204994258));
#63897=CARTESIAN_POINT('Ctrl Pts',(-3.49298096863515,7.14951456207522,46.2845324041616));
#63898=CARTESIAN_POINT('Ctrl Pts',(-2.69936282276075,7.48535612077804,46.2442984558652));
#63899=CARTESIAN_POINT('Ctrl Pts',(-1.85649704577245,7.69008862549486,46.2087296599851));
#63900=CARTESIAN_POINT('Ctrl Pts',(-1.84569906945247,7.69268739097793,46.2082749694832));
#63901=CARTESIAN_POINT('Ctrl Pts',(-1.78849040537241,7.70632850003853,46.2058711600591));
#63902=CARTESIAN_POINT('Ctrl Pts',(-1.74198552169552,7.71697372224957,46.2039351611053));
#63903=CARTESIAN_POINT('Ctrl Pts',(-1.68456262408075,7.72957259908383,46.2015664568519));
#63904=CARTESIAN_POINT('Ctrl Pts',(-1.67373361219453,7.73192470188996,46.2011207108942));
#63905=CARTESIAN_POINT('Ctrl Pts',(-1.65577123031196,7.73578669538184,46.2003829104312));
#63906=CARTESIAN_POINT('Ctrl Pts',(-1.64864066816913,7.73730948787828,46.2000904342727));
#63907=CARTESIAN_POINT('Ctrl Pts',(-1.63572194474264,7.74004972233167,46.1995612832223));
#63908=CARTESIAN_POINT('Ctrl Pts',(-1.62993450839717,7.74127053417047,46.1993244984206));
#63909=CARTESIAN_POINT('Ctrl Pts',(-1.61751803436322,7.74387514538855,46.1988170702665));
#63910=CARTESIAN_POINT('Ctrl Pts',(-1.61088857549813,7.74525692643482,46.1985464929168));
#63911=CARTESIAN_POINT('Ctrl Pts',(-1.5928618230011,7.74899010451011,46.1978116923082));
#63912=CARTESIAN_POINT('Ctrl Pts',(-1.58146108140003,7.75132487233656,46.1973480111531));
#63913=CARTESIAN_POINT('Ctrl Pts',(-1.52400651907369,7.76295900783842,46.1950164322002));
#63914=CARTESIAN_POINT('Ctrl Pts',(-1.47787519801554,7.77187322495033,46.1931610734125));
#63915=CARTESIAN_POINT('Ctrl Pts',(-0.861703263717836,7.88525499710756,
46.1685949703723));
#63916=CARTESIAN_POINT('Ctrl Pts',(-0.281909987949086,7.92719266148348,
46.1481175039457));
#63917=CARTESIAN_POINT('Ctrl Pts',(0.913190984529806,7.88225130730059,46.1068526519513));
#63918=CARTESIAN_POINT('Ctrl Pts',(1.52422085831935,7.78719430407909,46.0862059904786));
#63919=CARTESIAN_POINT('Ctrl Pts',(2.15698672618239,7.61137118503577,46.0603227078197));
#63920=CARTESIAN_POINT('Ctrl Pts',(2.19594527966792,7.6002228444951,46.0587101162482));
#63921=CARTESIAN_POINT('Ctrl Pts',(2.24301494424486,7.58636131584293,46.056740100674));
#63922=CARTESIAN_POINT('Ctrl Pts',(2.25121006411208,7.58393349793206,46.0563963101428));
#63923=CARTESIAN_POINT('Ctrl Pts',(2.26463828169596,7.57993168279835,46.0558316950643));
#63924=CARTESIAN_POINT('Ctrl Pts',(2.2698737245545,7.57836553203345,46.0556112383551));
#63925=CARTESIAN_POINT('Ctrl Pts',(2.2792517449345,7.57554956463676,46.05521577069));
#63926=CARTESIAN_POINT('Ctrl Pts',(2.28339493388027,7.57430176972607,46.0550408533146));
#63927=CARTESIAN_POINT('Ctrl Pts',(2.29217189898423,7.57165057480612,46.0546698845663));
#63928=CARTESIAN_POINT('Ctrl Pts',(2.29680541333091,7.5702463192816,46.054473794013));
#63929=CARTESIAN_POINT('Ctrl Pts',(2.30914104328809,7.56649545506043,46.0539510896322));
#63930=CARTESIAN_POINT('Ctrl Pts',(2.31684085753181,7.56414134382935,46.0536241356687));
#63931=CARTESIAN_POINT('Ctrl Pts',(2.35264932870897,7.55313359599738,46.0521004647042));
#63932=CARTESIAN_POINT('Ctrl Pts',(2.38071294319059,7.54433508220576,46.0508973021609));
#63933=CARTESIAN_POINT('Ctrl Pts',(2.60197850094645,7.47360630634047,46.041342815864));
#63934=CARTESIAN_POINT('Ctrl Pts',(2.79277414490122,7.4044235575911,46.0326938461278));
#63935=CARTESIAN_POINT('Ctrl Pts',(3.22446827900906,7.22883016791315,46.0124586444502));
#63936=CARTESIAN_POINT('Ctrl Pts',(3.46314286350154,7.11757107945948,46.0007791008091));
#63937=CARTESIAN_POINT('Ctrl Pts',(4.19763249220316,6.72948117965616,45.9639180252363));
#63938=CARTESIAN_POINT('Ctrl Pts',(4.669495826522,6.41108034137121,45.9389874647248));
#63939=CARTESIAN_POINT('Ctrl Pts',(5.20715117939874,5.95717971262762,45.9097967707891));
#63940=CARTESIAN_POINT('Ctrl Pts',(5.30878376596204,5.8667904422558,45.9042300245248));
#63941=CARTESIAN_POINT('Ctrl Pts',(5.42499351155148,5.75794287037197,45.8977967636495));
#63942=CARTESIAN_POINT('Ctrl Pts',(5.4418789296379,5.74198697507092,45.8968602493102));
#63943=CARTESIAN_POINT('Ctrl Pts',(5.46653378574503,5.71848290140706,45.8954901481128));
#63944=CARTESIAN_POINT('Ctrl Pts',(5.47435834592267,5.71099282310811,45.8950549297332));
#63945=CARTESIAN_POINT('Ctrl Pts',(5.48888579158408,5.69702910319105,45.8942461291335));
#63946=CARTESIAN_POINT('Ctrl Pts',(5.4955926655259,5.69055964653082,45.893872430287));
#63947=CARTESIAN_POINT('Ctrl Pts',(5.50947502443996,5.67712127823062,45.8930982893552));
#63948=CARTESIAN_POINT('Ctrl Pts',(5.51664875741477,5.67015057477277,45.8926978988815));
#63949=CARTESIAN_POINT('Ctrl Pts',(5.53469668729099,5.6525467613961,45.8916896910601));
#63950=CARTESIAN_POINT('Ctrl Pts',(5.54555349162488,5.64189585013542,45.8910823805571));
#63951=CARTESIAN_POINT('Ctrl Pts',(5.5877592145323,5.60025100607808,45.8887182447351));
#63952=CARTESIAN_POINT('Ctrl Pts',(5.61887974011862,5.56902638615567,45.8869680838066));
#63953=CARTESIAN_POINT('Ctrl Pts',(6.10597322674262,5.07206401770137,45.8594613266564));
#63954=CARTESIAN_POINT('Ctrl Pts',(6.50293373993015,4.55199442557474,45.8357478942767));
#63955=CARTESIAN_POINT('Ctrl Pts',(7.01167929093169,3.68073219414796,45.7992666486995));
#63956=CARTESIAN_POINT('Ctrl Pts',(7.17064921264867,3.36053635601431,45.7863750327625));
#63957=CARTESIAN_POINT('Ctrl Pts',(7.36571052391028,2.89021870949779,45.7670193450199));
#63958=CARTESIAN_POINT('Ctrl Pts',(7.41991438851238,2.74807614357545,45.7611148644146));
#63959=CARTESIAN_POINT('Ctrl Pts',(7.474518538081,2.59146353117678,45.7544729172857));
#63960=CARTESIAN_POINT('Ctrl Pts',(7.47901789270622,2.57844952766289,45.7539199755146));
#63961=CARTESIAN_POINT('Ctrl Pts',(7.48528323891336,2.56017316670389,45.7531419433922));
#63962=CARTESIAN_POINT('Ctrl Pts',(7.48707772137369,2.55492054752367,45.7529181634396));
#63963=CARTESIAN_POINT('Ctrl Pts',(7.49017971754867,2.54580937952081,45.7525296883565));
#63964=CARTESIAN_POINT('Ctrl Pts',(7.49148978289561,2.5419516971622,45.7523651119298));
#63965=CARTESIAN_POINT('Ctrl Pts',(7.4942069597042,2.53393022048807,45.7520226983557));
#63966=CARTESIAN_POINT('Ctrl Pts',(7.49561358201777,2.5297662631423,45.7518448383831));
#63967=CARTESIAN_POINT('Ctrl Pts',(7.49891342968008,2.51997096620334,45.7514261712736));
#63968=CARTESIAN_POINT('Ctrl Pts',(7.50080378112076,2.51433866716033,45.7511852284825));
#63969=CARTESIAN_POINT('Ctrl Pts',(7.50694333966711,2.4959773195483,45.7503990574407));
#63970=CARTESIAN_POINT('Ctrl Pts',(7.51116648660083,2.48323963640294,45.7498525846053));
#63971=CARTESIAN_POINT('Ctrl Pts',(7.58591865523912,2.25583983112144,45.7400763699094));
#63972=CARTESIAN_POINT('Ctrl Pts',(7.64723913392699,2.03830237605796,45.7303502927874));
#63973=CARTESIAN_POINT('Ctrl Pts',(7.76152100632742,1.55444819737674,45.7082807016921));
#63974=CARTESIAN_POINT('Ctrl Pts',(7.81025641844645,1.28740138768795,45.6958361691029));
#63975=CARTESIAN_POINT('Ctrl Pts',(7.92593911433649,0.396238513383225,45.654435083206));
#63976=CARTESIAN_POINT('Ctrl Pts',(7.93241723087277,-0.233403940133185,
45.6256025219132));
#63977=CARTESIAN_POINT('Ctrl Pts',(7.84898678516317,-0.998801405390404,
45.5932007595034));
#63978=CARTESIAN_POINT('Ctrl Pts',(7.8297368825879,-1.1399214798817,45.5873262442997));
#63979=CARTESIAN_POINT('Ctrl Pts',(7.80413312575725,-1.29602322332292,45.5809365107599));
#63980=CARTESIAN_POINT('Ctrl Pts',(7.80153225977172,-1.31158851912749,45.5803005694811));
#63981=CARTESIAN_POINT('Ctrl Pts',(7.79757372224525,-1.33485060069996,45.579351938966));
#63982=CARTESIAN_POINT('Ctrl Pts',(7.79625119987939,-1.34255327971313,45.5790381137884));
#63983=CARTESIAN_POINT('Ctrl Pts',(7.79395476609153,-1.35581042345275,45.5784984856089));
#63984=CARTESIAN_POINT('Ctrl Pts',(7.79298632719306,-1.36136582320463,45.5782725055903));
#63985=CARTESIAN_POINT('Ctrl Pts',(7.79102944821688,-1.37252084488801,45.5778190488207));
#63986=CARTESIAN_POINT('Ctrl Pts',(7.79004090927039,-1.37812044637269,45.5775915754188));
#63987=CARTESIAN_POINT('Ctrl Pts',(7.78771526711517,-1.39121164097026,45.5770601264804));
#63988=CARTESIAN_POINT('Ctrl Pts',(7.78637338861701,-1.39870238617536,45.5767563060061));
#63989=CARTESIAN_POINT('Ctrl Pts',(7.78222143640404,-1.42168861592112,45.5758248316491));
#63990=CARTESIAN_POINT('Ctrl Pts',(7.77937589209213,-1.43717769922888,45.575198329775));
#63991=CARTESIAN_POINT('Ctrl Pts',(7.77273428597815,-1.47273206631784,45.5737628740745));
#63992=CARTESIAN_POINT('Ctrl Pts',(7.76890673687844,-1.49279139245896,45.5729549464495));
#63993=CARTESIAN_POINT('Ctrl Pts',(7.75605221739652,-1.55877037406356,45.5703037979563));
#63994=CARTESIAN_POINT('Ctrl Pts',(7.74669538087286,-1.60462514319323,45.5684713097729));
#63995=CARTESIAN_POINT('Ctrl Pts',(7.70809557262344,-1.78557827825945,45.5612778532947));
#63996=CARTESIAN_POINT('Ctrl Pts',(7.67572027569065,-1.91998637657885,45.5560191575296));
#63997=CARTESIAN_POINT('Ctrl Pts',(7.5572423811868,-2.36077534942246,45.5389984784802));
#63998=CARTESIAN_POINT('Ctrl Pts',(7.45617839012619,-2.66281700518543,45.5277125431495));
#63999=CARTESIAN_POINT('Ctrl Pts',(7.05081962363052,-3.66830421336438,45.4902524071992));
#64000=CARTESIAN_POINT('Ctrl Pts',(6.66286385744881,-4.33317394317613,45.4659487454483));
#64001=CARTESIAN_POINT('Ctrl Pts',(6.1570504070919,-4.96756882408057,45.4341102630803));
#64002=CARTESIAN_POINT('Ctrl Pts',(6.1282500762851,-5.00305512475781,45.4322959701446));
#64003=CARTESIAN_POINT('Ctrl Pts',(6.09400688259133,-5.04450851810304,45.4301345773901));
#64004=CARTESIAN_POINT('Ctrl Pts',(6.08885983706439,-5.05071994451675,45.4298095908552));
#64005=CARTESIAN_POINT('Ctrl Pts',(6.08106912539896,-5.06009251634561,45.429317497388));
#64006=CARTESIAN_POINT('Ctrl Pts',(6.07843246151705,-5.06325950278151,45.4291509229686));
#64007=CARTESIAN_POINT('Ctrl Pts',(6.07370712396299,-5.06892625550477,45.4288523342598));
#64008=CARTESIAN_POINT('Ctrl Pts',(6.07161938063593,-5.07142679213555,45.4287203911295));
#64009=CARTESIAN_POINT('Ctrl Pts',(6.06717589532666,-5.07674217664295,45.428439524317));
#64010=CARTESIAN_POINT('Ctrl Pts',(6.06481973653262,-5.07955667713375,45.4282905688284));
#64011=CARTESIAN_POINT('Ctrl Pts',(6.05850097178466,-5.08709396236088,45.4278910323727));
#64012=CARTESIAN_POINT('Ctrl Pts',(6.054534809528,-5.09181374824342,45.4276401813974));
#64013=CARTESIAN_POINT('Ctrl Pts',(6.03564059798249,-5.11424482294583,45.426444854311));
#64014=CARTESIAN_POINT('Ctrl Pts',(6.02064046423679,-5.13189496344394,45.4254949642154));
#64015=CARTESIAN_POINT('Ctrl Pts',(5.90179979410298,-5.2704925151697,45.4179640613292));
#64016=CARTESIAN_POINT('Ctrl Pts',(5.79440809085358,-5.38833566026056,45.4111276596962));
#64017=CARTESIAN_POINT('Ctrl Pts',(5.51159632250249,-5.68043374446661,45.3932448792176));
#64018=CARTESIAN_POINT('Ctrl Pts',(5.33143392529485,-5.84985666971853,45.381966115217));
#64019=CARTESIAN_POINT('Ctrl Pts',(4.90968882997884,-6.21077272332795,45.3563698009899));
#64020=CARTESIAN_POINT('Ctrl Pts',(4.66423628909521,-6.39715936237836,45.3420144150289));
#64021=CARTESIAN_POINT('Ctrl Pts',(4.25220900332335,-6.67368628899001,45.3193078912122));
#64022=CARTESIAN_POINT('Ctrl Pts',(4.09217402739796,-6.77299686490314,45.3107950521843));
#64023=CARTESIAN_POINT('Ctrl Pts',(3.62838649368195,-7.03835770825675,45.2871052565214));
#64024=CARTESIAN_POINT('Ctrl Pts',(3.31705913369678,-7.19032873371709,45.2723645640927));
#64025=CARTESIAN_POINT('Ctrl Pts',(2.97634459470573,-7.32978716892991,45.2574746943218));
#64026=CARTESIAN_POINT('Ctrl Pts',(2.95590532800878,-7.33805361050666,45.2565859602549));
#64027=CARTESIAN_POINT('Ctrl Pts',(2.92791593522201,-7.34923770069508,45.2553750337002));
#64028=CARTESIAN_POINT('Ctrl Pts',(2.92039559333514,-7.35222932748834,45.2550502755954));
#64029=CARTESIAN_POINT('Ctrl Pts',(2.90758469989985,-7.35730280310246,45.2544980688529));
#64030=CARTESIAN_POINT('Ctrl Pts',(2.9022964782286,-7.35939049624918,45.2542704178399));
#64031=CARTESIAN_POINT('Ctrl Pts',(2.89162195904045,-7.36359130610247,45.2538114874263));
#64032=CARTESIAN_POINT('Ctrl Pts',(2.88623558428345,-7.36570421816687,45.2535802151997));
#64033=CARTESIAN_POINT('Ctrl Pts',(2.87396777603052,-7.37050098564255,45.2530541697056));
#64034=CARTESIAN_POINT('Ctrl Pts',(2.86708488741413,-7.37318111847072,45.2527595252431));
#64035=CARTESIAN_POINT('Ctrl Pts',(2.85268227748764,-7.37876614400655,45.2521440059178));
#64036=CARTESIAN_POINT('Ctrl Pts',(2.84516184709727,-7.38166919121668,45.251823194944));
#64037=CARTESIAN_POINT('Ctrl Pts',(2.82542251125756,-7.38925435047484,45.2509826764563));
#64038=CARTESIAN_POINT('Ctrl Pts',(2.81319638024109,-7.39391765923138,45.2504636166194));
#64039=CARTESIAN_POINT('Ctrl Pts',(2.77684453014169,-7.40767981830832,45.2489248429259));
#64040=CARTESIAN_POINT('Ctrl Pts',(2.75268573096859,-7.41669111653112,45.2479081335978));
#64041=CARTESIAN_POINT('Ctrl Pts',(2.66827793293182,-7.44770621905748,45.2443762648857));
#64042=CARTESIAN_POINT('Ctrl Pts',(2.60780505751807,-7.46909553284978,45.2418820329771));
#64043=CARTESIAN_POINT('Ctrl Pts',(2.4419024015777,-7.52551492229622,45.2351336541947));
#64044=CARTESIAN_POINT('Ctrl Pts',(2.3359830622578,-7.55906386269258,45.2309285433124));
#64045=CARTESIAN_POINT('Ctrl Pts',(2.05200853661971,-7.64247082593702,45.2199011537339));
#64046=CARTESIAN_POINT('Ctrl Pts',(1.87285108944981,-7.68833742397841,45.2132001200689));
#64047=CARTESIAN_POINT('Ctrl Pts',(1.28506628606805,-7.81704999288738,45.1918267063637));
#64048=CARTESIAN_POINT('Ctrl Pts',(0.871470791927446,-7.87389405945192,
45.1777695756254));
#64049=CARTESIAN_POINT('Ctrl Pts',(0.0127080435581117,-7.92340366721502,
45.1481782554769));
#64050=CARTESIAN_POINT('Ctrl Pts',(-0.431233234309826,-7.91166491045866,
45.1326436203546));
#64051=CARTESIAN_POINT('Ctrl Pts',(-0.899818011444226,-7.85971013223619,
45.1139671089807));
#64052=CARTESIAN_POINT('Ctrl Pts',(-0.927821650962073,-7.85645357414792,
45.1128421240603));
#64053=CARTESIAN_POINT('Ctrl Pts',(-0.962050147412785,-7.85228756915941,
45.1114556154184));
#64054=CARTESIAN_POINT('Ctrl Pts',(-0.968292429254012,-7.85152025574219,
45.1112022900556));
#64055=CARTESIAN_POINT('Ctrl Pts',(-0.978625524780857,-7.85023758127673,
45.1107821692991));
#64056=CARTESIAN_POINT('Ctrl Pts',(-0.982716850587435,-7.84972646604264,
45.1106156226619));
#64057=CARTESIAN_POINT('Ctrl Pts',(-0.989803761351205,-7.84883549527352,
45.1103267856339));
#64058=CARTESIAN_POINT('Ctrl Pts',(-0.992799535337517,-7.84845712229003,
45.1102045807844));
#64059=CARTESIAN_POINT('Ctrl Pts',(-0.99950588677319,-7.84760619386737,
45.1099307722018));
#64060=CARTESIAN_POINT('Ctrl Pts',(-1.00321634597973,-7.84713272187991,
45.1097791159097));
#64061=CARTESIAN_POINT('Ctrl Pts',(-1.01302232219203,-7.84587436466876,
45.109377886866));
#64062=CARTESIAN_POINT('Ctrl Pts',(-1.01911725193471,-7.84508500896157,
45.1091280597903));
#64063=CARTESIAN_POINT('Ctrl Pts',(-1.04669353182927,-7.84148092021652,
45.107995745496));
#64064=CARTESIAN_POINT('Ctrl Pts',(-1.06816400425993,-7.83858507732715,
45.1071087016272));
#64065=CARTESIAN_POINT('Ctrl Pts',(-1.22762586692925,-7.81641024104995,
45.1004815696595));
#64066=CARTESIAN_POINT('Ctrl Pts',(-1.36509184669648,-7.7935777830643,45.0945514412104));
#64067=CARTESIAN_POINT('Ctrl Pts',(-1.64282285221011,-7.73987486413295,
45.0822285833282));
#64068=CARTESIAN_POINT('Ctrl Pts',(-1.78299715113025,-7.70879031179902,
45.0758295594722));
#64069=CARTESIAN_POINT('Ctrl Pts',(-2.2850066613363,-7.58304163453388,45.0524424394893));
#64070=CARTESIAN_POINT('Ctrl Pts',(-2.64086672672486,-7.46656523303081,
45.0349969617625));
#64071=CARTESIAN_POINT('Ctrl Pts',(-3.17638800541315,-7.24818914115788,
45.0084324763907));
#64072=CARTESIAN_POINT('Ctrl Pts',(-3.36256915990343,-7.16371553180975,
44.9991296066186));
#64073=CARTESIAN_POINT('Ctrl Pts',(-3.89622209013668,-6.89619383659496,
44.9724562400596));
#64074=CARTESIAN_POINT('Ctrl Pts',(-4.23361160688387,-6.69437270348464,
44.9556128660747));
#64075=CARTESIAN_POINT('Ctrl Pts',(-4.57622662745964,-6.45312071604315,
44.9386252568006));
#64076=CARTESIAN_POINT('Ctrl Pts',(-4.59772321238927,-6.43782248911711,
44.9375597377885));
#64077=CARTESIAN_POINT('Ctrl Pts',(-4.62719905411467,-6.41662281773909,
44.9360990903914));
#64078=CARTESIAN_POINT('Ctrl Pts',(-4.63524421934644,-6.41081355987418,
44.9357004588083));
#64079=CARTESIAN_POINT('Ctrl Pts',(-4.64803139755435,-6.40154353185536,
44.935066921038));
#64080=CARTESIAN_POINT('Ctrl Pts',(-4.65278051294209,-6.3980926033829,44.934831639726));
#64081=CARTESIAN_POINT('Ctrl Pts',(-4.66240442312029,-6.39108303987759,
44.9343548745983));
#64082=CARTESIAN_POINT('Ctrl Pts',(-4.66727899598378,-6.3875241057237,44.9341134024499));
#64083=CARTESIAN_POINT('Ctrl Pts',(-4.67844563869341,-6.37935171312257,
44.9335602662545));
#64084=CARTESIAN_POINT('Ctrl Pts',(-4.68473497043451,-6.37473451456304,
44.9332487456852));
#64085=CARTESIAN_POINT('Ctrl Pts',(-4.69790243907058,-6.36503784610155,
44.9325965772672));
#64086=CARTESIAN_POINT('Ctrl Pts',(-4.70477919435659,-6.35995651260747,
44.9322560014181));
#64087=CARTESIAN_POINT('Ctrl Pts',(-4.72289860424831,-6.34652235009006,
44.9313586753923));
#64088=CARTESIAN_POINT('Ctrl Pts',(-4.73412736029245,-6.33815077962664,
44.9308026453174));
#64089=CARTESIAN_POINT('Ctrl Pts',(-4.76764816537428,-6.31302065184092,
44.9291428655593));
#64090=CARTESIAN_POINT('Ctrl Pts',(-4.78987399083888,-6.29617391366351,
44.9280425119272));
#64091=CARTESIAN_POINT('Ctrl Pts',(-4.86784613495153,-6.23642073199929,
44.924182470146));
#64092=CARTESIAN_POINT('Ctrl Pts',(-4.9231094534904,-6.19288811105501,44.9214470261026));
#64093=CARTESIAN_POINT('Ctrl Pts',(-5.23434407602938,-5.9409196417508,44.9060323172904));
#64094=CARTESIAN_POINT('Ctrl Pts',(-5.47766144267767,-5.71735353500339,
44.8939648016532));
#64095=CARTESIAN_POINT('Ctrl Pts',(-6.24443266890608,-4.91880369379686,
44.8546951624153));
#64096=CARTESIAN_POINT('Ctrl Pts',(-6.6969699804357,-4.2822659340079,44.8296507195791));
#64097=CARTESIAN_POINT('Ctrl Pts',(-7.06877571347331,-3.55220259280201,
44.7974216999255));
#64098=CARTESIAN_POINT('Ctrl Pts',(-7.08778856981776,-3.51411246498051,
44.7957299784945));
#64099=CARTESIAN_POINT('Ctrl Pts',(-7.10978015125898,-3.46915021033776,
44.7937190273155));
#64100=CARTESIAN_POINT('Ctrl Pts',(-7.11305800903638,-3.46242440214129,
44.793417846661));
#64101=CARTESIAN_POINT('Ctrl Pts',(-7.1182939215366,-3.45164206373017,44.7929344128781));
#64102=CARTESIAN_POINT('Ctrl Pts',(-7.12025806742463,-3.44758848219771,
44.792752531502));
#64103=CARTESIAN_POINT('Ctrl Pts',(-7.12373126898598,-3.44040490080144,
44.7924299644162));
#64104=CARTESIAN_POINT('Ctrl Pts',(-7.12524172834748,-3.43727557620928,
44.7922893648894));
#64105=CARTESIAN_POINT('Ctrl Pts',(-7.12838853690268,-3.43074512492742,
44.7919957807693));
#64106=CARTESIAN_POINT('Ctrl Pts',(-7.13002451025928,-3.4273438298877,44.7918427739743));
#64107=CARTESIAN_POINT('Ctrl Pts',(-7.13427970521626,-3.41848077060412,
44.791443819028));
#64108=CARTESIAN_POINT('Ctrl Pts',(-7.13689508495794,-3.41301717504889,
44.7911976364068));
#64109=CARTESIAN_POINT('Ctrl Pts',(-7.14812995048461,-3.38947787103691,
44.7901359340581));
#64110=CARTESIAN_POINT('Ctrl Pts',(-7.15668699532723,-3.37137260843522,
44.7893166580578));
#64111=CARTESIAN_POINT('Ctrl Pts',(-7.21660884791525,-3.24333191274209,
44.7835049994685));
#64112=CARTESIAN_POINT('Ctrl Pts',(-7.26550494932593,-3.13226442378221,
44.778371841829));
#64113=CARTESIAN_POINT('Ctrl Pts',(-7.70724254340192,-2.06280148467221,
44.7283908523604));
#64114=CARTESIAN_POINT('Ctrl Pts',(-7.91088113128406,-1.03708363487558,
44.6779412040058));
#64115=CARTESIAN_POINT('Ctrl Pts',(-7.91099994798975,-0.000907141745418172,
44.6351174622069));
#64116=CARTESIAN_POINT('',(-7.90852312217059,0.00709379171421498,42.6423315082371));
#64117=CARTESIAN_POINT('Ctrl Pts',(-7.89861493486562,-0.000610740782857052,
44.6422669711751));
#64118=CARTESIAN_POINT('Ctrl Pts',(-7.8954795751415,1.45177507856196,44.5840303434289));
#64119=CARTESIAN_POINT('Ctrl Pts',(-6.81619969976293,5.55073973453917,44.4198593358802));
#64120=CARTESIAN_POINT('Ctrl Pts',(-0.210945049882454,9.354012036458,44.1497539485288));
#64121=CARTESIAN_POINT('Ctrl Pts',(6.40488750778627,5.92654785945168,43.8849179990226));
#64122=CARTESIAN_POINT('Ctrl Pts',(8.18512056268212,0.79234657492906,43.6730492394173));
#64123=CARTESIAN_POINT('Ctrl Pts',(7.4227292473118,-4.58798910622404,43.4611804798124));
#64124=CARTESIAN_POINT('Ctrl Pts',(1.58715686282455,-9.22079020936372,43.1963445303059));
#64125=CARTESIAN_POINT('Ctrl Pts',(-6.17232811875731,-6.56794650215052,
42.9057391431469));
#64126=CARTESIAN_POINT('Ctrl Pts',(-7.89172359999745,-1.9501472650058,42.7210681357908));
#64127=CARTESIAN_POINT('Ctrl Pts',(-7.90852312217059,0.00709379171421498,
42.6423315082371));
#64128=CARTESIAN_POINT('',(-7.92071738904598,-0.000648184374720526,40.6423303528761));
#64129=CARTESIAN_POINT('Ctrl Pts',(-7.91099681685684,0.00709673735080949,
42.6423314790088));
#64130=CARTESIAN_POINT('Ctrl Pts',(-7.9107752173155,0.254121980005545,42.6323970776905));
#64131=CARTESIAN_POINT('Ctrl Pts',(-7.89897987247902,0.500645992443577,
42.6224626763721));
#64132=CARTESIAN_POINT('Ctrl Pts',(-7.87577275734792,0.745737537352352,
42.6125282750538));
#64133=CARTESIAN_POINT('Ctrl Pts',(-7.85215362603152,0.995180406534389,
42.6024174996316));
#64134=CARTESIAN_POINT('Ctrl Pts',(-7.81671393357025,1.24313964973455,42.5923067242094));
#64135=CARTESIAN_POINT('Ctrl Pts',(-7.76967306550624,1.488657601716,42.5821959487873));
#64136=CARTESIAN_POINT('Ctrl Pts',(-7.73639540989157,1.66234193598769,42.5750433830217));
#64137=CARTESIAN_POINT('Ctrl Pts',(-7.69731303644139,1.8348050543254,42.5678908172562));
#64138=CARTESIAN_POINT('Ctrl Pts',(-7.6525179617014,2.00571429815851,42.5607382514906));
#64139=CARTESIAN_POINT('Ctrl Pts',(-7.60297192480338,2.19475016315747,42.5528270851539));
#64140=CARTESIAN_POINT('Ctrl Pts',(-7.54635066681069,2.38220313786713,42.5449159188171));
#64141=CARTESIAN_POINT('Ctrl Pts',(-7.48276962060389,2.5675045871366,42.5370047524803));
#64142=CARTESIAN_POINT('Ctrl Pts',(-7.41925749423832,2.75260517550139,42.5291021615975));
#64143=CARTESIAN_POINT('Ctrl Pts',(-7.3488007174694,2.93555856057317,42.5211995707145));
#64144=CARTESIAN_POINT('Ctrl Pts',(-7.2715653994801,3.11580770284107,42.5132969798316));
#64145=CARTESIAN_POINT('Ctrl Pts',(-7.19439946509978,3.29589492001654,42.5054014881656));
#64146=CARTESIAN_POINT('Ctrl Pts',(-7.1104672551568,3.47328241886557,42.4975059964996));
#64147=CARTESIAN_POINT('Ctrl Pts',(-7.01998429752439,3.64742943214957,42.4896105048336));
#64148=CARTESIAN_POINT('Ctrl Pts',(-6.92956583344602,3.82145231863552,42.4817206408387));
#64149=CARTESIAN_POINT('Ctrl Pts',(-6.83260608261984,3.99223901657015,42.4738307768437));
#64150=CARTESIAN_POINT('Ctrl Pts',(-6.72936829589034,4.15926956787679,42.4659409128487));
#64151=CARTESIAN_POINT('Ctrl Pts',(-6.62618494040187,4.32621205375229,42.4580552087171));
#64152=CARTESIAN_POINT('Ctrl Pts',(-6.51673032558461,4.48940204658587,42.4501695045855));
#64153=CARTESIAN_POINT('Ctrl Pts',(-6.4013133068748,4.64834475348243,42.442283800454));
#64154=CARTESIAN_POINT('Ctrl Pts',(-6.28593573112009,4.80723314282581,42.4344007912063));
#64155=CARTESIAN_POINT('Ctrl Pts',(-6.16460001487929,4.9618768604002,42.4265177819587));
#64156=CARTESIAN_POINT('Ctrl Pts',(-6.03765809640805,5.11181041421513,42.4186347727111));
#64157=CARTESIAN_POINT('Ctrl Pts',(-5.91071425287239,5.26174624176087,42.4107516439183));
#64158=CARTESIAN_POINT('Ctrl Pts',(-5.77816425357656,5.40697149421105,42.4028685151254));
#64159=CARTESIAN_POINT('Ctrl Pts',(-5.64040042235492,5.54705363914019,42.3949853863326));
#64160=CARTESIAN_POINT('Ctrl Pts',(-5.50262805231716,5.68714446657814,42.3871017689311));
#64161=CARTESIAN_POINT('Ctrl Pts',(-5.35964144792159,5.82209130486687,42.3792181515297));
#64162=CARTESIAN_POINT('Ctrl Pts',(-5.21186992463021,5.95149837341279,42.3713345341283));
#64163=CARTESIAN_POINT('Ctrl Pts',(-5.06406440262239,6.08093521545046,42.3634491028939));
#64164=CARTESIAN_POINT('Ctrl Pts',(-4.91147202751804,6.2048295207068,42.3555636716594));
#64165=CARTESIAN_POINT('Ctrl Pts',(-4.75455550521427,6.32282555095716,42.347678240425));
#64166=CARTESIAN_POINT('Ctrl Pts',(-4.59757650297498,6.44086856405071,42.3397896694241));
#64167=CARTESIAN_POINT('Ctrl Pts',(-4.43627019823336,6.55300841532703,42.3319010984231));
#64168=CARTESIAN_POINT('Ctrl Pts',(-4.27112878713447,6.65893233812383,42.3240125274222));
#64169=CARTESIAN_POINT('Ctrl Pts',(-4.10581159260935,6.76496901077509,42.3161155594963));
#64170=CARTESIAN_POINT('Ctrl Pts',(-3.93665142823722,6.86477635285342,42.3082185915704));
#64171=CARTESIAN_POINT('Ctrl Pts',(-3.76416659665973,6.95808672212348,42.3003216236445));
#64172=CARTESIAN_POINT('Ctrl Pts',(-3.59157655001415,7.05145401035138,42.2924198385993));
#64173=CARTESIAN_POINT('Ctrl Pts',(-3.41565810142144,7.13831627243318,42.284518053554));
#64174=CARTESIAN_POINT('Ctrl Pts',(-3.23695033211913,7.21845368118365,42.2766162685088));
#64175=CARTESIAN_POINT('Ctrl Pts',(-3.05801139796657,7.29869475052016,42.2687042622238));
#64176=CARTESIAN_POINT('Ctrl Pts',(-2.8762762550339,7.37219346255176,42.2607922559388));
#64177=CARTESIAN_POINT('Ctrl Pts',(-2.69230103212412,7.4387792111625,42.2528802496538));
#64178=CARTESIAN_POINT('Ctrl Pts',(-2.6152173850023,7.46667792637031,42.2495652037968));
#64179=CARTESIAN_POINT('Ctrl Pts',(-2.53774063856249,7.4933636683486,42.2462501579398));
#64180=CARTESIAN_POINT('Ctrl Pts',(-2.45991226034516,7.51882654883085,42.2429351120828));
#64181=CARTESIAN_POINT('Ctrl Pts',(-2.27584207891438,7.5790482460764,42.2350947702136));
#64182=CARTESIAN_POINT('Ctrl Pts',(-2.08928226693087,7.63259703827931,42.2272544283444));
#64183=CARTESIAN_POINT('Ctrl Pts',(-1.90076281645489,7.67925919054582,42.2194140864752));
#64184=CARTESIAN_POINT('Ctrl Pts',(-1.71245413633543,7.7258691731373,42.2115825103416));
#64185=CARTESIAN_POINT('Ctrl Pts',(-1.52219051807484,7.76560776355152,42.203750934208));
#64186=CARTESIAN_POINT('Ctrl Pts',(-1.33052027264029,7.7983098684326,42.1959193580743));
#64187=CARTESIAN_POINT('Ctrl Pts',(-1.13902705125604,7.83098177009122,42.1880950150786));
#64188=CARTESIAN_POINT('Ctrl Pts',(-0.946130133980474,7.85663006967012,
42.180270672083));
#64189=CARTESIAN_POINT('Ctrl Pts',(-0.752391472052713,7.87513987639473,
42.1724463290873));
#64190=CARTESIAN_POINT('Ctrl Pts',(-0.558794093171459,7.89363618492616,
42.1646276919585));
#64191=CARTESIAN_POINT('Ctrl Pts',(-0.364356540635688,7.90500433570941,
42.1568090548297));
#64192=CARTESIAN_POINT('Ctrl Pts',(-0.169649596957392,7.90918074229261,
42.1489904177009));
#64193=CARTESIAN_POINT('Ctrl Pts',(0.0249531835348763,7.91335491460615,
42.141175963341));
#64194=CARTESIAN_POINT('Ctrl Pts',(0.219824717474835,7.91034499936617,42.1333615089811));
#64195=CARTESIAN_POINT('Ctrl Pts',(0.414390284975091,7.90013934634816,42.1255470546213));
#64196=CARTESIAN_POINT('Ctrl Pts',(0.608889554322827,7.88993717090302,42.1177352630341));
#64197=CARTESIAN_POINT('Ctrl Pts',(0.80308271426759,7.87254416148577,42.109923471447));
#64198=CARTESIAN_POINT('Ctrl Pts',(0.996396040113872,7.84800076014557,42.1021116798598));
#64199=CARTESIAN_POINT('Ctrl Pts',(1.18971841333569,7.82345621013458,42.0942995226683));
#64200=CARTESIAN_POINT('Ctrl Pts',(1.38216052021535,7.79176063483256,42.0864873654767));
#64201=CARTESIAN_POINT('Ctrl Pts',(1.57315422730095,7.75300630575812,42.0786752082851));
#64202=CARTESIAN_POINT('Ctrl Pts',(1.76416354829495,7.7142488084822,42.0708624124426));
#64203=CARTESIAN_POINT('Ctrl Pts',(1.95372388860504,7.66843147708458,42.0630496166001));
#64204=CARTESIAN_POINT('Ctrl Pts',(2.14127785751969,7.6156976132785,42.0552368207576));
#64205=CARTESIAN_POINT('Ctrl Pts',(2.32888016087265,7.5629501594551,42.0474220114834));
#64206=CARTESIAN_POINT('Ctrl Pts',(2.5144747241418,7.50328271750232,42.0396072022092));
#64207=CARTESIAN_POINT('Ctrl Pts',(2.69751970754075,7.43688835652582,42.031792392935));
#64208=CARTESIAN_POINT('Ctrl Pts',(2.88064407445718,7.37046520143643,42.0239741945101));
#64209=CARTESIAN_POINT('Ctrl Pts',(3.06121632856204,7.29730943561723,42.0161559960851));
#64210=CARTESIAN_POINT('Ctrl Pts',(3.23871484176716,7.21766216816201,42.0083377976602));
#64211=CARTESIAN_POINT('Ctrl Pts',(3.41641996227953,7.13792219171919,42.0005104988946));
#64212=CARTESIAN_POINT('Ctrl Pts',(3.59104387509404,7.051675766105,41.9926832001291));
#64213=CARTESIAN_POINT('Ctrl Pts',(3.7620888131397,6.95921035477799,41.9848559013636));
#64214=CARTESIAN_POINT('Ctrl Pts',(3.93324541001745,6.86668458165392,41.9770234929055));
#64215=CARTESIAN_POINT('Ctrl Pts',(4.10081807426051,6.76793191029551,41.9691910844475));
#64216=CARTESIAN_POINT('Ctrl Pts',(4.26433820122678,6.66328302757417,41.9613586759894));
#64217=CARTESIAN_POINT('Ctrl Pts',(4.42809300261807,6.55848395895928,41.9535150269215));
#64218=CARTESIAN_POINT('Ctrl Pts',(4.58778336278074,6.44777197775258,41.9456713778536));
#64219=CARTESIAN_POINT('Ctrl Pts',(4.74297299130483,6.3315186332943,41.9378277287857));
#64220=CARTESIAN_POINT('Ctrl Pts',(4.826703138568,6.26879595173432,41.9335958100822));
#64221=CARTESIAN_POINT('Ctrl Pts',(4.90912374903964,6.20446085109633,41.9293638913787));
#64222=CARTESIAN_POINT('Ctrl Pts',(4.99017083595707,6.1385760586608,41.9251319726753));
#64223=CARTESIAN_POINT('Ctrl Pts',(5.14180674225222,6.01530820793337,41.9172142195224));
#64224=CARTESIAN_POINT('Ctrl Pts',(5.28908562653389,5.88624514946329,41.9092964663696));
#64225=CARTESIAN_POINT('Ctrl Pts',(5.43153577643814,5.75172496815282,41.9013787132167));
#64226=CARTESIAN_POINT('Ctrl Pts',(5.57382226136985,5.61735934085155,41.8934700569926));
#64227=CARTESIAN_POINT('Ctrl Pts',(5.71129081437693,5.47754931330097,41.8855614007684));
#64228=CARTESIAN_POINT('Ctrl Pts',(5.84350099013029,5.3326744864417,41.8776527445442));
#64229=CARTESIAN_POINT('Ctrl Pts',(5.97558373985316,5.18793929198214,41.8697517107943));
#64230=CARTESIAN_POINT('Ctrl Pts',(6.10241797775633,5.03814927516368,41.8618506770445));
#64231=CARTESIAN_POINT('Ctrl Pts',(6.22359827888221,4.88372250062332,41.8539496432946));
#64232=CARTESIAN_POINT('Ctrl Pts',(6.3446842090389,4.72941598823981,41.8460547625928));
#64233=CARTESIAN_POINT('Ctrl Pts',(6.4601247631334,4.57048018198781,41.8381598818909));
#64234=CARTESIAN_POINT('Ctrl Pts',(6.56955298426317,4.40736821549538,41.8302650011891));
#64235=CARTESIAN_POINT('Ctrl Pts',(6.67891623099291,4.24435309881052,41.8223748081732));
#64236=CARTESIAN_POINT('Ctrl Pts',(6.78227406681057,4.07716704806391,41.8144846151574));
#64237=CARTESIAN_POINT('Ctrl Pts',(6.87930111374699,3.90629455960497,41.8065944221415));
#64238=CARTESIAN_POINT('Ctrl Pts',(6.97628849652655,3.73549192293891,41.7987074545959));
#64239=CARTESIAN_POINT('Ctrl Pts',(7.06695007841203,3.56100615102911,41.7908204870503));
#64240=CARTESIAN_POINT('Ctrl Pts',(7.15100480639265,3.3833491186913,41.7829335195047));
#64241=CARTESIAN_POINT('Ctrl Pts',(7.2350522347939,3.20570751465408,41.7750472368884));
#64242=CARTESIAN_POINT('Ctrl Pts',(7.31249379934101,3.02489550735143,41.767160954272));
#64243=CARTESIAN_POINT('Ctrl Pts',(7.38309503535332,2.84144834528823,41.7592746716557));
#64244=CARTESIAN_POINT('Ctrl Pts',(7.45369614727388,2.65800150565959,41.7513884029007));
#64245=CARTESIAN_POINT('Ctrl Pts',(7.51745683033518,2.4719198418899,41.7435021341456));
#64246=CARTESIAN_POINT('Ctrl Pts',(7.57419125410534,2.28375739653628,41.7356158653906));
#64247=CARTESIAN_POINT('Ctrl Pts',(7.63093508714138,2.09556374489981,41.7277282887171));
#64248=CARTESIAN_POINT('Ctrl Pts',(7.68065023952765,1.90528895396002,41.7198407120436));
#64249=CARTESIAN_POINT('Ctrl Pts',(7.72320105331794,1.71350123724164,41.7119531353701));
#64250=CARTESIAN_POINT('Ctrl Pts',(7.76576605582388,1.52164956824752,41.7040629285569));
#64251=CARTESIAN_POINT('Ctrl Pts',(7.80116188516549,1.32828430444575,41.6961727217438));
#64252=CARTESIAN_POINT('Ctrl Pts',(7.82930414348475,1.13398308136079,41.6882825149306));
#64253=CARTESIAN_POINT('Ctrl Pts',(7.85747357769407,0.939494229102066,41.68038468885));
#64254=CARTESIAN_POINT('Ctrl Pts',(7.87837540062114,0.744067953381702,41.6724868627694));
#64255=CARTESIAN_POINT('Ctrl Pts',(7.8919770681622,0.548287292942333,41.6645890366888));
#64256=CARTESIAN_POINT('Ctrl Pts',(7.90558626720361,0.352398225051473,41.6566868374326));
#64257=CARTESIAN_POINT('Ctrl Pts',(7.91188724033619,0.15615472481144,41.6487846381765));
#64258=CARTESIAN_POINT('Ctrl Pts',(7.91089957771789,-0.0398606480500094,
41.6408824389203));
#64259=CARTESIAN_POINT('Ctrl Pts',(7.90991072291592,-0.236112626328689,
41.6329707011105));
#64260=CARTESIAN_POINT('Ctrl Pts',(7.90161567342775,-0.432135583878224,
41.6250589633007));
#64261=CARTESIAN_POINT('Ctrl Pts',(7.88608592012398,-0.627351464828427,
41.6171472254909));
#64262=CARTESIAN_POINT('Ctrl Pts',(7.87966182751903,-0.708105155672722,
41.6138744280831));
#64263=CARTESIAN_POINT('Ctrl Pts',(7.87200035814089,-0.78872084903206,41.6106016306753));
#64264=CARTESIAN_POINT('Ctrl Pts',(7.86310912297639,-0.869158167519254,
41.6073288332675));
#64265=CARTESIAN_POINT('Ctrl Pts',(7.84052008578004,-1.07351690347274,41.5990139770059));
#64266=CARTESIAN_POINT('Ctrl Pts',(7.80994062011707,-1.27716956920081,41.5906991207443));
#64267=CARTESIAN_POINT('Ctrl Pts',(7.77142554366926,-1.47948167248024,41.5823842644827));
#64268=CARTESIAN_POINT('Ctrl Pts',(7.73295789719928,-1.68154463543707,41.5740796476776));
#64269=CARTESIAN_POINT('Ctrl Pts',(7.68657418514291,-1.88227004180361,41.5657750308724));
#64270=CARTESIAN_POINT('Ctrl Pts',(7.63238085311091,-2.0810294358961,41.5574704140673));
#64271=CARTESIAN_POINT('Ctrl Pts',(7.57825068363204,-2.27955717509084,41.5491754763274));
#64272=CARTESIAN_POINT('Ctrl Pts',(7.51632912558697,-2.47612319039856,41.5408805385876));
#64273=CARTESIAN_POINT('Ctrl Pts',(7.44677361945884,-2.670109297488,41.5325856008478));
#64274=CARTESIAN_POINT('Ctrl Pts',(7.3773223641015,-2.86380465547201,41.5243030956773));
#64275=CARTESIAN_POINT('Ctrl Pts',(7.30026009332459,-3.05492754681884,41.5160205905068));
#64276=CARTESIAN_POINT('Ctrl Pts',(7.21579400125396,-3.24287494847817,41.5077380853363));
#64277=CARTESIAN_POINT('Ctrl Pts',(7.13140550331944,-3.43064969367965,41.4994631888265));
#64278=CARTESIAN_POINT('Ctrl Pts',(7.03962686708011,-3.61525449989592,41.4911882923166));
#64279=CARTESIAN_POINT('Ctrl Pts',(6.94071398715704,-3.79610462823177,41.4829133958068));
#64280=CARTESIAN_POINT('Ctrl Pts',(6.84191425059518,-3.97674788774112,41.4746479646933));
#64281=CARTESIAN_POINT('Ctrl Pts',(6.73599669479649,-4.15364478284566,41.4663825335797));
#64282=CARTESIAN_POINT('Ctrl Pts',(6.62326402536842,-4.32623330973498,41.4581171024662));
#64283=CARTESIAN_POINT('Ctrl Pts',(6.57921061017469,-4.39367706025826,41.4548871561654));
#64284=CARTESIAN_POINT('Ctrl Pts',(6.53411698324595,-4.46046313740019,41.4516572098646));
#64285=CARTESIAN_POINT('Ctrl Pts',(6.48800312905023,-4.52655900187266,41.4484272635638));
#64286=CARTESIAN_POINT('Ctrl Pts',(6.36998153523263,-4.69572159749272,41.4401606934187));
#64287=CARTESIAN_POINT('Ctrl Pts',(6.24540708208217,-4.86017049045324,41.4318941232737));
#64288=CARTESIAN_POINT('Ctrl Pts',(6.11468798505374,-5.01941349616062,41.4236275531286));
#64289=CARTESIAN_POINT('Ctrl Pts',(5.98385176220058,-5.17879918544523,41.415353576041));
#64290=CARTESIAN_POINT('Ctrl Pts',(5.84686009039699,-5.3329694483423,41.4070795989534));
#64291=CARTESIAN_POINT('Ctrl Pts',(5.70415960291809,-5.48146734227591,41.3988056218657));
#64292=CARTESIAN_POINT('Ctrl Pts',(5.56132199162359,-5.6301079308715,41.3905236941444));
#64293=CARTESIAN_POINT('Ctrl Pts',(5.41276481606496,-5.77306505704043,41.382241766423));
#64294=CARTESIAN_POINT('Ctrl Pts',(5.25897007300826,-5.90992003086366,41.3739598387017));
#64295=CARTESIAN_POINT('Ctrl Pts',(5.1049203970669,-6.04700185791062,41.3656641827106));
#64296=CARTESIAN_POINT('Ctrl Pts',(4.94561601610714,-6.17796111457056,41.3573685267194));
#64297=CARTESIAN_POINT('Ctrl Pts',(4.78157198150445,-6.30241940731427,41.3490728707283));
#64298=CARTESIAN_POINT('Ctrl Pts',(4.6173796828416,-6.42699018626846,41.3407697170696));
#64299=CARTESIAN_POINT('Ctrl Pts',(4.44843941738418,-6.54504810111771,41.3324665634109));
#64300=CARTESIAN_POINT('Ctrl Pts',(4.27529456373084,-6.65625851310881,41.3241634097521));
#64301=CARTESIAN_POINT('Ctrl Pts',(4.10188572706688,-6.76763848058337,41.3158475968));
#64302=CARTESIAN_POINT('Ctrl Pts',(3.92425973916612,-6.87214992416895,41.3075317838479));
#64303=CARTESIAN_POINT('Ctrl Pts',(3.74298551908125,-6.96950359810138,41.2992159708959));
#64304=CARTESIAN_POINT('Ctrl Pts',(3.67257358532567,-7.00731846464215,41.2959858785505));
#64305=CARTESIAN_POINT('Ctrl Pts',(3.60161144474516,-7.0440539050805,41.2927557862051));
#64306=CARTESIAN_POINT('Ctrl Pts',(3.53013323911411,-7.07969493086402,41.2895256938598));
#64307=CARTESIAN_POINT('Ctrl Pts',(3.35507271984093,-7.16698498558781,41.2816147280166));
#64308=CARTESIAN_POINT('Ctrl Pts',(3.17655169375813,-7.24788823486347,41.2737037621734));
#64309=CARTESIAN_POINT('Ctrl Pts',(2.99507658703413,-7.32211972299006,41.2657927963303));
#64310=CARTESIAN_POINT('Ctrl Pts',(2.81378511634647,-7.39627609571102,41.2578898356534));
#64311=CARTESIAN_POINT('Ctrl Pts',(2.6295458357032,-7.46377402594048,41.2499868749765));
#64312=CARTESIAN_POINT('Ctrl Pts',(2.44288948778114,-7.52437452221036,41.2420839142997));
#64313=CARTESIAN_POINT('Ctrl Pts',(2.25638747591343,-7.58492491120241,41.2341874881542));
#64314=CARTESIAN_POINT('Ctrl Pts',(2.06747270404295,-7.63858912207468,41.2262910620088));
#64315=CARTESIAN_POINT('Ctrl Pts',(1.87669587182935,-7.68517622469769,41.2183946358633));
#64316=CARTESIAN_POINT('Ctrl Pts',(1.68604148681759,-7.73173342609899,41.2105032779186));
#64317=CARTESIAN_POINT('Ctrl Pts',(1.49352775615284,-7.77122248811454,41.2026119199739));
#64318=CARTESIAN_POINT('Ctrl Pts',(1.29972079733459,-7.803502216888,41.1947205620293));
#64319=CARTESIAN_POINT('Ctrl Pts',(1.10600238117861,-7.83576719834207,41.186832809331));
#64320=CARTESIAN_POINT('Ctrl Pts',(0.910992253337599,-7.86082935345353,
41.1789450566327));
#64321=CARTESIAN_POINT('Ctrl Pts',(0.715267271467289,-7.87859846231344,
41.1710573039344));
#64322=CARTESIAN_POINT('Ctrl Pts',(0.519595509620023,-7.89636273953472,
41.1631716960128));
#64323=CARTESIAN_POINT('Ctrl Pts',(0.323209623895253,-7.90683789200927,
41.1552860880912));
#64324=CARTESIAN_POINT('Ctrl Pts',(0.126692438162148,-7.90998546307846,
41.1474004801696));
#64325=CARTESIAN_POINT('Ctrl Pts',(-0.0698479250685975,-7.91313340537636,
41.139513942209));
#64326=CARTESIAN_POINT('Ctrl Pts',(-0.266519274877356,-7.90895202712437,
41.1316274042483));
#64327=CARTESIAN_POINT('Ctrl Pts',(-0.462737289344198,-7.89745498252762,
41.1237408662877));
#64328=CARTESIAN_POINT('Ctrl Pts',(-0.65898002357199,-7.88595648952058,
41.1158533347723));
#64329=CARTESIAN_POINT('Ctrl Pts',(-0.854768964509576,-7.86714051314872,
41.107965803257));
#64330=CARTESIAN_POINT('Ctrl Pts',(-1.0495234431412,-7.8410727290529,41.1000782717416));
#64331=CARTESIAN_POINT('Ctrl Pts',(-1.24433510025892,-7.81499729164691,
41.0921884245049));
#64332=CARTESIAN_POINT('Ctrl Pts',(-1.43811134833977,-7.78166584941576,
41.0842985772681));
#64333=CARTESIAN_POINT('Ctrl Pts',(-1.63028001038072,-7.74119552057388,
41.0764087300314));
#64334=CARTESIAN_POINT('Ctrl Pts',(-1.82253730213947,-7.70070652649393,
41.0685152439342));
#64335=CARTESIAN_POINT('Ctrl Pts',(-2.0131851935778,-7.65307215560085,41.0606217578371));
#64336=CARTESIAN_POINT('Ctrl Pts',(-2.20166476039912,-7.598459928355,41.0527282717399));
#64337=CARTESIAN_POINT('Ctrl Pts',(-2.39036220933888,-7.54378456945003,
41.0448256607838));
#64338=CARTESIAN_POINT('Ctrl Pts',(-2.57688599598329,-7.48211533802818,
41.0369230498276));
#64339=CARTESIAN_POINT('Ctrl Pts',(-2.76069423665923,-7.41366901956626,
41.0290204388715));
#64340=CARTESIAN_POINT('Ctrl Pts',(-2.94462438897629,-7.34517730377622,
41.0211125864731));
#64341=CARTESIAN_POINT('Ctrl Pts',(-3.12583508758474,-7.26989967170283,
41.0132047340748));
#64342=CARTESIAN_POINT('Ctrl Pts',(-3.30380706649977,-7.18809987878203,
41.0052968816764));
#64343=CARTESIAN_POINT('Ctrl Pts',(-3.48202256156049,-7.10618816054347,
40.997378209093));
#64344=CARTESIAN_POINT('Ctrl Pts',(-3.65699017924273,-7.01773661133071,
40.9894595365097));
#64345=CARTESIAN_POINT('Ctrl Pts',(-3.82821673433037,-6.92305406847245,
40.9815408639263));
#64346=CARTESIAN_POINT('Ctrl Pts',(-3.89898428997597,-6.88392198339978,
40.9782680941016));
#64347=CARTESIAN_POINT('Ctrl Pts',(-3.96911317311707,-6.84372605308623,
40.9749953242769));
#64348=CARTESIAN_POINT('Ctrl Pts',(-4.03857014346165,-6.80249014672863,
40.9717225544521));
#64349=CARTESIAN_POINT('Ctrl Pts',(-4.20502250025122,-6.70366905269699,
40.9638794215333));
#64350=CARTESIAN_POINT('Ctrl Pts',(-4.36810660132914,-6.59857981631457,
40.9560362886144));
#64351=CARTESIAN_POINT('Ctrl Pts',(-4.52731165393276,-6.4874779528076,40.9481931556955));
#64352=CARTESIAN_POINT('Ctrl Pts',(-4.68632973714723,-6.37650656661408,
40.9403592337015));
#64353=CARTESIAN_POINT('Ctrl Pts',(-4.8414775577109,-6.25953681227435,40.9325253117074));
#64354=CARTESIAN_POINT('Ctrl Pts',(-4.99226859464812,-6.13687015333469,
40.9246913897133));
#64355=CARTESIAN_POINT('Ctrl Pts',(-5.14291186982358,-6.01432369677576,
40.9168651442639));
#64356=CARTESIAN_POINT('Ctrl Pts',(-5.28920659270855,-5.88609167275004,
40.9090388988143));
#64357=CARTESIAN_POINT('Ctrl Pts',(-5.4306947850553,-5.75251902661548,40.9012126533649));
#64358=CARTESIAN_POINT('Ctrl Pts',(-5.57207183242556,-5.61905130746013,
40.8933925557631));
#64359=CARTESIAN_POINT('Ctrl Pts',(-5.70864961500615,-5.48025156199503,
40.8855724581614));
#64360=CARTESIAN_POINT('Ctrl Pts',(-5.84000271093576,-5.33650534865871,
40.8777523605597));
#64361=CARTESIAN_POINT('Ctrl Pts',(-5.97127814402506,-5.19284412562377,
40.8699368866099));
#64362=CARTESIAN_POINT('Ctrl Pts',(-6.0973348074805,-5.0442425192713,40.86212141266));
#64363=CARTESIAN_POINT('Ctrl Pts',(-6.21778355414878,-4.8911234572189,40.8543059387102));
#64364=CARTESIAN_POINT('Ctrl Pts',(-6.33818448079993,-4.73806518580462,
40.8464935676245));
#64365=CARTESIAN_POINT('Ctrl Pts',(-6.45298170951549,-4.58049330795824,
40.8386811965388));
#64366=CARTESIAN_POINT('Ctrl Pts',(-6.56182575565952,-4.41886453202216,
40.8308688254532));
#64367=CARTESIAN_POINT('Ctrl Pts',(-6.67066568166833,-4.25724187431152,
40.8230567500936));
#64368=CARTESIAN_POINT('Ctrl Pts',(-6.77355267021599,-4.09156291097583,
40.815244674734));
#64369=CARTESIAN_POINT('Ctrl Pts',(-6.87017977626858,-3.92231447512183,
40.8074325993744));
#64370=CARTESIAN_POINT('Ctrl Pts',(-6.96680970836285,-3.7530610892786,40.799620295536));
#64371=CARTESIAN_POINT('Ctrl Pts',(-7.0571792181417,-3.58023832811498,40.7918079916975));
#64372=CARTESIAN_POINT('Ctrl Pts',(-7.14102668421596,-3.40435880825092,
40.7839956878591));
#64373=CARTESIAN_POINT('Ctrl Pts',(-7.22489135579719,-3.22844319789484,
40.7761817809353));
#64374=CARTESIAN_POINT('Ctrl Pts',(-7.30223116625825,-3.04946989684581,
40.7683678740114));
#64375=CARTESIAN_POINT('Ctrl Pts',(-7.37283206215466,-2.86797287003629,
40.7605539670876));
#64376=CARTESIAN_POINT('Ctrl Pts',(-7.44345986869196,-2.68640666278299,
40.7527370817704));
#64377=CARTESIAN_POINT('Ctrl Pts',(-7.50734351665096,-2.50231514113536,
40.7449201964531));
#64378=CARTESIAN_POINT('Ctrl Pts',(-7.56431831949938,-2.31624898516677,
40.7371033111359));
#64379=CARTESIAN_POINT('Ctrl Pts',(-7.62135492795542,-2.12998098678269,
40.7292779461518));
#64380=CARTESIAN_POINT('Ctrl Pts',(-7.67146761948069,-1.94173441219844,
40.7214525811677));
#64381=CARTESIAN_POINT('Ctrl Pts',(-7.71454224380687,-1.75207276347737,
40.7136272161836));
#64382=CARTESIAN_POINT('Ctrl Pts',(-7.75764304698127,-1.56229584680925,
40.7057970952894));
#64383=CARTESIAN_POINT('Ctrl Pts',(-7.7936971934392,-1.37110248660038,40.6979669743952));
#64384=CARTESIAN_POINT('Ctrl Pts',(-7.82264222598379,-1.17906301962849,
40.690136853501));
#64385=CARTESIAN_POINT('Ctrl Pts',(-7.85162682446981,-0.986761047430777,
40.6822960293504));
#64386=CARTESIAN_POINT('Ctrl Pts',(-7.87348286043591,-0.793611006666677,
40.6744552051998));
#64387=CARTESIAN_POINT('Ctrl Pts',(-7.88819989848087,-0.600186105809256,
40.6666143810492));
#64388=CARTESIAN_POINT('Ctrl Pts',(-7.8961426136037,-0.49579561089576,40.6623827257143));
#64389=CARTESIAN_POINT('Ctrl Pts',(-7.90200684590501,-0.391325034556162,
40.6581510703794));
#64390=CARTESIAN_POINT('Ctrl Pts',(-7.90579724297386,-0.286863997369564,
40.6539194150445));
#64391=CARTESIAN_POINT('Ctrl Pts',(-7.90925710005275,-0.191512441210014,
40.650056779442));
#64392=CARTESIAN_POINT('Ctrl Pts',(-7.91099181751041,-0.0961026461293392,
40.6461941438395));
#64393=CARTESIAN_POINT('Ctrl Pts',(-7.91099997112236,-0.000675945236853683,
40.642331508237));
#64394=CARTESIAN_POINT('',(-7.90652959962495,-0.00529323366394208,38.6423315082371));
#64395=CARTESIAN_POINT('Ctrl Pts',(-7.92426962316665,-0.000638036300153408,
40.6423299305302));
#64396=CARTESIAN_POINT('Ctrl Pts',(-7.91681046214448,2.5252695445412,40.5402587122325));
#64397=CARTESIAN_POINT('Ctrl Pts',(-5.23832781156842,7.68132265384459,40.332253114132));
#64398=CARTESIAN_POINT('Ctrl Pts',(3.54974568342456,8.65605708304547,40.0183131362292));
#64399=CARTESIAN_POINT('Ctrl Pts',(9.20185311915298,1.69349879413918,39.7005099968215));
#64400=CARTESIAN_POINT('Ctrl Pts',(6.86833150499802,-5.3826179369575,39.435674047315));
#64401=CARTESIAN_POINT('Ctrl Pts',(2.08192809636596,-7.95547529202212,39.2238052877101));
#64402=CARTESIAN_POINT('Ctrl Pts',(-3.35120507934021,-8.05704524214747,
39.0119365281047));
#64403=CARTESIAN_POINT('Ctrl Pts',(-7.37691166608612,-4.37872292798657,
38.8181119349473));
#64404=CARTESIAN_POINT('Ctrl Pts',(-7.91046959319798,-0.878292219197368,
38.6772545316909));
#64405=CARTESIAN_POINT('Ctrl Pts',(-7.90405025860222,-0.00822892851515322,
38.6423315082371));
#64406=CARTESIAN_POINT('',(-7.91214355523022,0.00146147383487005,36.6443103639743));
#64407=CARTESIAN_POINT('Ctrl Pts',(-7.911,-8.17679257636428E-13,38.6423315082371));
#64408=CARTESIAN_POINT('Ctrl Pts',(-7.91100000000023,2.2016758966659,38.5537440725043));
#64409=CARTESIAN_POINT('Ctrl Pts',(-6.94214576672421,4.38610418338602,38.4651566367716));
#64410=CARTESIAN_POINT('Ctrl Pts',(-3.67820201488378,7.34180684107585,38.2879817653062));
#64411=CARTESIAN_POINT('Ctrl Pts',(-1.40868175871851,8.08992666571317,38.1993943295734));
#64412=CARTESIAN_POINT('Ctrl Pts',(2.97309270521164,7.65454228025298,38.022219458108));
#64413=CARTESIAN_POINT('Ctrl Pts',(5.05102072675505,6.474448808343,37.9336320223753));
#64414=CARTESIAN_POINT('Ctrl Pts',(7.66951518847823,2.9342519536783,37.7564571509098));
#64415=CARTESIAN_POINT('Ctrl Pts',(8.1895687224706,0.60188196010054,37.6678697151771));
#64416=CARTESIAN_POINT('Ctrl Pts',(7.32306689761408,-3.71537198232318,37.4906948437117));
#64417=CARTESIAN_POINT('Ctrl Pts',(5.94329958850306,-5.666435189364,37.4021074079789));
#64418=CARTESIAN_POINT('Ctrl Pts',(2.16154501638003,-7.92205913232954,37.2249325365135));
#64419=CARTESIAN_POINT('Ctrl Pts',(-0.210816529298698,-8.20894963713006,
37.1363451007808));
#64420=CARTESIAN_POINT('Ctrl Pts',(-4.42123908576288,-6.91982244717925,
36.9591702293153));
#64421=CARTESIAN_POINT('Ctrl Pts',(-6.22631625634069,-5.35390358803658,
36.8705827935826));
#64422=CARTESIAN_POINT('Ctrl Pts',(-7.65317280859451,-2.31334857514661,
36.7354407413123));
#64423=CARTESIAN_POINT('Ctrl Pts',(-7.91099999999989,-1.1570283783663,36.6888861247747));
#64424=CARTESIAN_POINT('Ctrl Pts',(-7.911,-7.63833440942108E-13,36.6423315082371));
#64425=CARTESIAN_POINT('',(-7.91099997583771,0.000602220688781498,34.642307277048));
#64426=CARTESIAN_POINT('Ctrl Pts',(-7.91099771853781,0.00600810199810929,
36.6423315082371));
#64427=CARTESIAN_POINT('Ctrl Pts',(-7.91082701748352,0.230773868533368,
36.6333181043834));
#64428=CARTESIAN_POINT('Ctrl Pts',(-7.90107349095901,0.455147217331988,
36.6243047005298));
#64429=CARTESIAN_POINT('Ctrl Pts',(-7.88186061629211,0.678376168024303,
36.6152912966761));
#64430=CARTESIAN_POINT('Ctrl Pts',(-7.86249103411946,0.903425858854828,
36.606204376076));
#64431=CARTESIAN_POINT('Ctrl Pts',(-7.83350723763257,1.12731227582692,36.5971174554758));
#64432=CARTESIAN_POINT('Ctrl Pts',(-7.79508525974753,1.34928380753155,36.5880305348757));
#64433=CARTESIAN_POINT('Ctrl Pts',(-7.75650928789974,1.57214499348267,36.5789071942111));
#64434=CARTESIAN_POINT('Ctrl Pts',(-7.70841942193409,1.79307580146918,36.5697838535464));
#64435=CARTESIAN_POINT('Ctrl Pts',(-7.65104221992903,2.01133635895725,36.5606605128818));
#64436=CARTESIAN_POINT('Ctrl Pts',(-7.59339181638938,2.23063616404131,36.5514937314327));
#64437=CARTESIAN_POINT('Ctrl Pts',(-7.52636550019852,2.44724011743129,36.5423269499835));
#64438=CARTESIAN_POINT('Ctrl Pts',(-7.45024055696212,2.66042038847185,36.5331601685343));
#64439=CARTESIAN_POINT('Ctrl Pts',(-7.42067243304598,2.74322295491882,36.5295996466045));
#64440=CARTESIAN_POINT('Ctrl Pts',(-7.38973212761027,2.82550925150776,36.5260391246746));
#64441=CARTESIAN_POINT('Ctrl Pts',(-7.35743777047115,2.90723759841616,36.5224786027448));
#64442=CARTESIAN_POINT('Ctrl Pts',(-7.28629962259197,3.08726915015888,36.5146354698259));
#64443=CARTESIAN_POINT('Ctrl Pts',(-7.20843803850659,3.26497043139147,36.506792336907));
#64444=CARTESIAN_POINT('Ctrl Pts',(-7.12402418831121,3.439796558571,36.4989492039881));
#64445=CARTESIAN_POINT('Ctrl Pts',(-7.03970947319829,3.61441737107176,36.491115281994));
#64446=CARTESIAN_POINT('Ctrl Pts',(-6.94885796507703,3.78616943984571,36.48328136));
#64447=CARTESIAN_POINT('Ctrl Pts',(-6.85169005333668,3.95452454955171,36.4754474380059));
#64448=CARTESIAN_POINT('Ctrl Pts',(-6.75461735747975,4.12271468627217,36.4676211925564));
#64449=CARTESIAN_POINT('Ctrl Pts',(-6.65124075828519,4.28751419072813,36.4597949471069));
#64450=CARTESIAN_POINT('Ctrl Pts',(-6.54182810735693,4.44841612417216,36.4519687016574));
#64451=CARTESIAN_POINT('Ctrl Pts',(-6.43250140470697,4.60919166232245,36.4441486040556));
#64452=CARTESIAN_POINT('Ctrl Pts',(-6.31714829073141,4.76607543819526,36.4363285064539));
#64453=CARTESIAN_POINT('Ctrl Pts',(-6.19608188419913,4.91858620787512,36.4285084088522));
#64454=CARTESIAN_POINT('Ctrl Pts',(-6.07508705847705,5.07100680518784,36.4206929349023));
#64455=CARTESIAN_POINT('Ctrl Pts',(-5.94838588706709,5.21905927215613,36.4128774609525));
#64456=CARTESIAN_POINT('Ctrl Pts',(-5.81633414354872,5.362292245914,36.4050619870027));
#64457=CARTESIAN_POINT('Ctrl Pts',(-5.6843348266164,5.50546835396435,36.397249615917));
#64458=CARTESIAN_POINT('Ctrl Pts',(-5.54698940788077,5.6438285229488,36.3894372448313));
#64459=CARTESIAN_POINT('Ctrl Pts',(-5.40469331071708,5.77695518565706,36.3816248737456));
#64460=CARTESIAN_POINT('Ctrl Pts',(-5.26240259996817,5.91007680904635,36.373812798386));
#64461=CARTESIAN_POINT('Ctrl Pts',(-5.11516183465845,6.03796507408886,36.3660007230264));
#64462=CARTESIAN_POINT('Ctrl Pts',(-4.96340293520149,6.1602396303093,36.3581886476668));
#64463=CARTESIAN_POINT('Ctrl Pts',(-4.81163959726983,6.28251776267932,36.3503763438283));
#64464=CARTESIAN_POINT('Ctrl Pts',(-4.65535813544312,6.39918163782201,36.3425640399899));
#64465=CARTESIAN_POINT('Ctrl Pts',(-4.49502312304542,6.50989156002518,36.3347517361514));
#64466=CARTESIAN_POINT('Ctrl Pts',(-4.33465520989007,6.62062419991343,36.3269378292276));
#64467=CARTESIAN_POINT('Ctrl Pts',(-4.17023237864531,6.7254002531701,36.3191239223037));
#64468=CARTESIAN_POINT('Ctrl Pts',(-4.00224783295993,6.82392359889584,36.3113100153799));
#64469=CARTESIAN_POINT('Ctrl Pts',(-3.83419925732518,6.92248449834304,36.3034931300627));
#64470=CARTESIAN_POINT('Ctrl Pts',(-3.66258656612503,7.0147877650145,36.2956762447454));
#64471=CARTESIAN_POINT('Ctrl Pts',(-3.48792730457781,7.10058336462439,36.2878593594282));
#64472=CARTESIAN_POINT('Ctrl Pts',(-3.31307857468228,7.18647203430915,36.2800339944441));
#64473=CARTESIAN_POINT('Ctrl Pts',(-3.13517698946395,7.26583878220487,36.27220862946));
#64474=CARTESIAN_POINT('Ctrl Pts',(-2.95476077761802,7.33848143331099,36.2643832644759));
#64475=CARTESIAN_POINT('Ctrl Pts',(-2.77423491679197,7.41116823340198,36.2565531435816));
#64476=CARTESIAN_POINT('Ctrl Pts',(-2.59119171346333,7.47712267358661,36.2487230226874));
#64477=CARTESIAN_POINT('Ctrl Pts',(-2.40618435216095,7.53619253094132,36.2408929017932));
#64478=CARTESIAN_POINT('Ctrl Pts',(-2.22092409805519,7.59534313287678,36.2330520776425));
#64479=CARTESIAN_POINT('Ctrl Pts',(-2.03369466101054,7.647590261596,36.2252112534919));
#64480=CARTESIAN_POINT('Ctrl Pts',(-1.84506032084028,7.69283260005447,36.2173704293413));
#64481=CARTESIAN_POINT('Ctrl Pts',(-1.74325526864717,7.71724967397614,36.2131387740066));
#64482=CARTESIAN_POINT('Ctrl Pts',(-1.64104112949169,7.73962734805209,36.2089071186719));
#64483=CARTESIAN_POINT('Ctrl Pts',(-1.53850712496967,7.75995598095876,36.2046754633371));
#64484=CARTESIAN_POINT('Ctrl Pts',(-1.34681750920186,7.79796081505384,36.1967642890008));
#64485=CARTESIAN_POINT('Ctrl Pts',(-1.15346117883056,7.82890972097021,36.1888531146645));
#64486=CARTESIAN_POINT('Ctrl Pts',(-0.959000070226024,7.85265814010176,
36.1809419403282));
#64487=CARTESIAN_POINT('Ctrl Pts',(-0.764749782710718,7.87638081286365,
36.173039342732));
#64488=CARTESIAN_POINT('Ctrl Pts',(-0.569397441845241,7.8929185063317,36.1651367451358));
#64489=CARTESIAN_POINT('Ctrl Pts',(-0.373516690169528,7.90217731275152,
36.1572341475396));
#64490=CARTESIAN_POINT('Ctrl Pts',(-0.177811937714245,7.91142780011651,
36.1493386504421));
#64491=CARTESIAN_POINT('Ctrl Pts',(0.0184199374734158,7.91341241269837,
36.1414431533446));
#64492=CARTESIAN_POINT('Ctrl Pts',(0.214598342881783,7.90808880521915,36.1335476562471));
#64493=CARTESIAN_POINT('Ctrl Pts',(0.410636886512517,7.90276899310774,36.1256577880986));
#64494=CARTESIAN_POINT('Ctrl Pts',(0.606621693015979,7.89015135087714,36.1177679199502));
#64495=CARTESIAN_POINT('Ctrl Pts',(0.801970041781192,7.87024555221027,36.1098780518018));
#64496=CARTESIAN_POINT('Ctrl Pts',(0.997215363279053,7.85035025191748,36.101992344792));
#64497=CARTESIAN_POINT('Ctrl Pts',(1.19182455367119,7.82317448934777,36.0941066377822));
#64498=CARTESIAN_POINT('Ctrl Pts',(1.38521760805087,7.78877995441814,36.0862209307724));
#64499=CARTESIAN_POINT('Ctrl Pts',(1.57854454051247,7.75439717912811,36.0783379199197));
#64500=CARTESIAN_POINT('Ctrl Pts',(1.77065582657825,7.7128006108626,36.0704549090671));
#64501=CARTESIAN_POINT('Ctrl Pts',(1.96097899889779,7.66410349394382,36.0625718982145));
#64502=CARTESIAN_POINT('Ctrl Pts',(2.15130501150619,7.61540565029336,36.0546887697197));
#64503=CARTESIAN_POINT('Ctrl Pts',(2.33984252091461,7.55960712353441,36.0468056412249));
#64504=CARTESIAN_POINT('Ctrl Pts',(2.52603106682682,7.49687188428786,36.0389225127301));
#64505=CARTESIAN_POINT('Ctrl Pts',(2.71223112496288,7.43413276605877,36.0310388968136));
#64506=CARTESIAN_POINT('Ctrl Pts',(2.89608160303152,7.36445619030373,36.0231552808971));
#64507=CARTESIAN_POINT('Ctrl Pts',(3.07703894152665,7.28805545755029,36.0152716649806));
#64508=CARTESIAN_POINT('Ctrl Pts',(3.25803788676078,7.21163715830646,36.0073862364184));
#64509=CARTESIAN_POINT('Ctrl Pts',(3.43614204910383,7.12849175547434,35.9995008078561));
#64510=CARTESIAN_POINT('Ctrl Pts',(3.61082930293514,7.03888007747432,35.9916153792939));
#64511=CARTESIAN_POINT('Ctrl Pts',(3.78558608622667,6.9492327320088,35.9837268121535));
#64512=CARTESIAN_POINT('Ctrl Pts',(3.95692294440953,6.85311414030414,35.9758382450131));
#64513=CARTESIAN_POINT('Ctrl Pts',(4.12434352441048,6.75083042985479,35.9679496778728));
#64514=CARTESIAN_POINT('Ctrl Pts',(4.29194227630253,6.64843786730302,35.9600527155822));
#64515=CARTESIAN_POINT('Ctrl Pts',(4.45561613086508,6.53986726085201,35.9521557532915));
#64516=CARTESIAN_POINT('Ctrl Pts',(4.61489792240152,6.42546793360718,35.9442587910009));
#64517=CARTESIAN_POINT('Ctrl Pts',(4.77427685464063,6.31099883799192,35.9363570126139));
#64518=CARTESIAN_POINT('Ctrl Pts',(4.92925811202304,6.19069414562624,35.9284552342268));
#64519=CARTESIAN_POINT('Ctrl Pts',(5.07940846381662,6.06494275799105,35.9205534558398));
#64520=CARTESIAN_POINT('Ctrl Pts',(5.22975301186175,5.93902873038989,35.9126414577248));
#64521=CARTESIAN_POINT('Ctrl Pts',(5.37525391931462,5.80765416731018,35.9047294596099));
#64522=CARTESIAN_POINT('Ctrl Pts',(5.51551478509475,5.67124480651305,35.8968174614949));
#64523=CARTESIAN_POINT('Ctrl Pts',(5.57428264562653,5.61409068696611,35.8935024156397));
#64524=CARTESIAN_POINT('Ctrl Pts',(5.63213108832611,5.55605309984752,35.8901873697846));
#64525=CARTESIAN_POINT('Ctrl Pts',(5.68903310393153,5.49716502775487,35.8868723239294));
#64526=CARTESIAN_POINT('Ctrl Pts',(5.82482649262485,5.35663202944195,35.8789611575927));
#64527=CARTESIAN_POINT('Ctrl Pts',(5.95559203093924,5.21087552504861,35.871049991256));
#64528=CARTESIAN_POINT('Ctrl Pts',(6.08090378471279,5.06028953332373,35.8631388249193));
#64529=CARTESIAN_POINT('Ctrl Pts',(6.20607970451243,4.90986677204655,35.8552362340364));
#64530=CARTESIAN_POINT('Ctrl Pts',(6.32581339647896,4.75462521346952,35.8473336431536));
#64531=CARTESIAN_POINT('Ctrl Pts',(6.43971515906603,4.59499615561266,35.8394310522707));
#64532=CARTESIAN_POINT('Ctrl Pts',(6.55351459909433,4.43551049899284,35.8315355606048));
#64533=CARTESIAN_POINT('Ctrl Pts',(6.66149234738,4.27164547377879,35.8236400689388));
#64534=CARTESIAN_POINT('Ctrl Pts',(6.76329827788125,4.10386615332524,35.8157445772729));
#64535=CARTESIAN_POINT('Ctrl Pts',(6.86503164415108,3.93620642096816,35.807854713278));
#64536=CARTESIAN_POINT('Ctrl Pts',(6.96060177897564,3.76463824559535,35.7999648492831));
#64537=CARTESIAN_POINT('Ctrl Pts',(7.04970112771916,3.5896566701894,35.7920749852881));
#64538=CARTESIAN_POINT('Ctrl Pts',(7.13875349959255,3.41476735232358,35.7841892811566));
#64539=CARTESIAN_POINT('Ctrl Pts',(7.22134172750293,3.2364685270999,35.776303577025));
#64540=CARTESIAN_POINT('Ctrl Pts',(7.29720345001519,3.05528113421439,35.7684178728935));
#64541=CARTESIAN_POINT('Ctrl Pts',(7.37303924731667,2.87415566084767,35.7605348636459));
#64542=CARTESIAN_POINT('Ctrl Pts',(7.44215298767534,2.69014390493507,35.7526518543984));
#64543=CARTESIAN_POINT('Ctrl Pts',(7.50432972686331,2.50378839970865,35.7447688451508));
#64544=CARTESIAN_POINT('Ctrl Pts',(7.56650740895673,2.31743006841541,35.736885716358));
#64545=CARTESIAN_POINT('Ctrl Pts',(7.62174776253362,2.12872824118862,35.7290025875652));
#64546=CARTESIAN_POINT('Ctrl Pts',(7.66988498578327,1.9382428394957,35.7211194587724));
#64547=CARTESIAN_POINT('Ctrl Pts',(7.71802519265272,1.74774563122195,35.7132358413711));
#64548=CARTESIAN_POINT('Ctrl Pts',(7.75906130680061,1.55546496257375,35.7053522239697));
#64549=CARTESIAN_POINT('Ctrl Pts',(7.79287814629815,1.36197327321381,35.6974686065684));
#64550=CARTESIAN_POINT('Ctrl Pts',(7.82670276624695,1.16843706601361,35.689583175334));
#64551=CARTESIAN_POINT('Ctrl Pts',(7.85330474238622,0.973689622693154,35.6816977440996));
#64552=CARTESIAN_POINT('Ctrl Pts',(7.87262045375448,0.778311114610711,35.6738123128652));
#64553=CARTESIAN_POINT('Ctrl Pts',(7.89194385611916,0.582854812064674,35.6659237418643));
#64554=CARTESIAN_POINT('Ctrl Pts',(7.90397517890498,0.386767287052605,35.6580351708634));
#64555=CARTESIAN_POINT('Ctrl Pts',(7.90870283912137,0.190631588341385,35.6501465998625));
#64556=CARTESIAN_POINT('Ctrl Pts',(7.91343553165706,-0.00571288541193959,
35.6422496319367));
#64557=CARTESIAN_POINT('Ctrl Pts',(7.91084902483556,-0.202105290369741,
35.6343526640108));
#64558=CARTESIAN_POINT('Ctrl Pts',(7.90098385553714,-0.397963710081122,
35.626455696085));
#64559=CARTESIAN_POINT('Ctrl Pts',(7.89111266852429,-0.593941602657351,
35.6185539110398));
#64560=CARTESIAN_POINT('Ctrl Pts',(7.87395399744757,-0.789384517943676,
35.6106521259946));
#64561=CARTESIAN_POINT('Ctrl Pts',(7.84960003056775,-0.983717622140998,
35.6027503409495));
#64562=CARTESIAN_POINT('Ctrl Pts',(7.82521456096634,-1.17830210311438,35.5948383346645));
#64563=CARTESIAN_POINT('Ctrl Pts',(7.79361526042141,-1.37177356625965,35.5869263283796));
#64564=CARTESIAN_POINT('Ctrl Pts',(7.75494523190075,-1.56356817894833,35.5790143220947));
#64565=CARTESIAN_POINT('Ctrl Pts',(7.73874290429313,-1.64392806661943,35.5756992762371));
#64566=CARTESIAN_POINT('Ctrl Pts',(7.72129989716543,-1.7239937681947,35.5723842303794));
#64567=CARTESIAN_POINT('Ctrl Pts',(7.70262930165425,-1.80372471328009,35.5690691845218));
#64568=CARTESIAN_POINT('Ctrl Pts',(7.65847188785192,-1.99229461362846,35.5612288426526));
#64569=CARTESIAN_POINT('Ctrl Pts',(7.60731924415892,-2.17952560368335,35.5533885007834));
#64570=CARTESIAN_POINT('Ctrl Pts',(7.54926404323549,-2.36485378100038,35.5455481589142));
#64571=CARTESIAN_POINT('Ctrl Pts',(7.49127374975459,-2.54997475589924,35.5377165827805));
#64572=CARTESIAN_POINT('Ctrl Pts',(7.42639636982972,-2.73319682218983,35.5298850066469));
#64573=CARTESIAN_POINT('Ctrl Pts',(7.35477565602851,-2.91396569119994,35.5220534305132));
#64574=CARTESIAN_POINT('Ctrl Pts',(7.28322109015136,-3.09456760452386,35.5142290875176));
#64575=CARTESIAN_POINT('Ctrl Pts',(7.20493572193786,-3.27272050820327,35.5064047445219));
#64576=CARTESIAN_POINT('Ctrl Pts',(7.12011328741707,-3.44788453611005,35.4985804015262));
#64577=CARTESIAN_POINT('Ctrl Pts',(7.03535270927447,-3.62292082643872,35.4907617643974));
#64578=CARTESIAN_POINT('Ctrl Pts',(6.94406471220099,-3.79497226723115,35.4829431272686));
#64579=CARTESIAN_POINT('Ctrl Pts',(6.84649145905047,-3.96351809648309,35.4751244901398));
#64580=CARTESIAN_POINT('Ctrl Pts',(6.74897040507044,-4.13197375806928,35.4673100357799));
#64581=CARTESIAN_POINT('Ctrl Pts',(6.64517096884488,-4.29692724050937,35.45949558142));
#64582=CARTESIAN_POINT('Ctrl Pts',(6.53538173784099,-4.45788139598784,35.4516811270601));
#64583=CARTESIAN_POINT('Ctrl Pts',(6.42562991748111,-4.61878070639128,35.443869335473));
#64584=CARTESIAN_POINT('Ctrl Pts',(6.30989256689027,-4.77568311499015,35.4360575438859));
#64585=CARTESIAN_POINT('Ctrl Pts',(6.1885022692311,-4.92811938407762,35.4282457522987));
#64586=CARTESIAN_POINT('Ctrl Pts',(6.06710629031017,-5.08056278742839,35.4204335951071));
#64587=CARTESIAN_POINT('Ctrl Pts',(5.94005704764244,-5.22853935290935,35.4126214379155));
#64588=CARTESIAN_POINT('Ctrl Pts',(5.8077285080673,-5.37161154371595,35.4048092807239));
#64589=CARTESIAN_POINT('Ctrl Pts',(5.67538915051427,-5.51469543080364,35.3969964848814));
#64590=CARTESIAN_POINT('Ctrl Pts',(5.53776987464694,-5.65287388565324,35.3891836890389));
#64591=CARTESIAN_POINT('Ctrl Pts',(5.39528267202063,-5.78574505910811,35.3813708931964));
#64592=CARTESIAN_POINT('Ctrl Pts',(5.25275874908957,-5.91865047472573,35.3735560839222));
#64593=CARTESIAN_POINT('Ctrl Pts',(5.10536465747417,-6.04624564430942,35.3657412746481));
#64594=CARTESIAN_POINT('Ctrl Pts',(4.9535468367383,-6.16816785895455,35.3579264653739));
#64595=CARTESIAN_POINT('Ctrl Pts',(4.80166317517817,-6.2901429492046,35.350108266949));
#64596=CARTESIAN_POINT('Ctrl Pts',(4.6453522367111,-6.40643996352781,35.342290068524));
#64597=CARTESIAN_POINT('Ctrl Pts',(4.48509101177552,-6.51673841857186,35.3344718700991));
#64598=CARTESIAN_POINT('Ctrl Pts',(4.32464324364248,-6.62716526041994,35.3266445713336));
#64599=CARTESIAN_POINT('Ctrl Pts',(4.16023629511131,-6.73157939802848,35.318817272568));
#64600=CARTESIAN_POINT('Ctrl Pts',(3.99237437147008,-6.82970481631739,35.3109899738025));
#64601=CARTESIAN_POINT('Ctrl Pts',(3.82440286688135,-6.92789429127904,35.3031575653444));
#64602=CARTESIAN_POINT('Ctrl Pts',(3.65297220136262,-7.01978670022458,35.2953251568864));
#64603=CARTESIAN_POINT('Ctrl Pts',(3.47860836580684,-7.10515339998643,35.2874927484283));
#64604=CARTESIAN_POINT('Ctrl Pts',(3.30399429357627,-7.19064261299202,35.2796490993604));
#64605=CARTESIAN_POINT('Ctrl Pts',(3.12643896376706,-7.26958726935294,35.2718054502925));
#64606=CARTESIAN_POINT('Ctrl Pts',(2.94648649823127,-7.34180756460838,35.2639618012246));
#64607=CARTESIAN_POINT('Ctrl Pts',(2.84939594789554,-7.38077290020899,35.2597298825211));
#64608=CARTESIAN_POINT('Ctrl Pts',(2.75160784009182,-7.4177816583206,35.2554979638176));
#64609=CARTESIAN_POINT('Ctrl Pts',(2.65320901345151,-7.45281174664567,35.2512660451141));
#64610=CARTESIAN_POINT('Ctrl Pts',(2.46910868581014,-7.51835166168475,35.2433482919612));
#64611=CARTESIAN_POINT('Ctrl Pts',(2.28231966222409,-7.57715815354364,35.2354305388084));
#64612=CARTESIAN_POINT('Ctrl Pts',(2.09337586950565,-7.62900376648036,35.2275127856555));
#64613=CARTESIAN_POINT('Ctrl Pts',(1.90464915961008,-7.68078981253822,35.2196041294313));
#64614=CARTESIAN_POINT('Ctrl Pts',(1.71377294057433,-7.72563081917493,35.2116954732072));
#64615=CARTESIAN_POINT('Ctrl Pts',(1.52130037261706,-7.76334761403064,35.203786816983));
#64616=CARTESIAN_POINT('Ctrl Pts',(1.32901331243296,-7.80102805690799,35.1958857832331));
#64617=CARTESIAN_POINT('Ctrl Pts',(1.13513330392061,-7.83159790058237,35.1879847494832));
#64618=CARTESIAN_POINT('Ctrl Pts',(0.940228182791328,-7.8549278777265,35.1800837157334));
#64619=CARTESIAN_POINT('Ctrl Pts',(0.745474846935986,-7.87823968630249,
35.1721888350316));
#64620=CARTESIAN_POINT('Ctrl Pts',(0.549698329371412,-7.89432282060209,
35.1642939543297));
#64621=CARTESIAN_POINT('Ctrl Pts',(0.353476449613453,-7.90309910095835,
35.1563990736279));
#64622=CARTESIAN_POINT('Ctrl Pts',(0.157371079095513,-7.91187017028638,
35.148508880612));
#64623=CARTESIAN_POINT('Ctrl Pts',(-0.0391787835774433,-7.91334301531703,
35.1406186875962));
#64624=CARTESIAN_POINT('Ctrl Pts',(-0.235590118047823,-7.90749127702827,
35.1327284945803));
#64625=CARTESIAN_POINT('Ctrl Pts',(-0.431921160576763,-7.90164193089997,
35.1248415270347));
#64626=CARTESIAN_POINT('Ctrl Pts',(-0.628113444003138,-7.88847397916084,
35.116954559489));
#64627=CARTESIAN_POINT('Ctrl Pts',(-0.823583578101995,-7.86801316025086,
35.1090675919434));
#64628=CARTESIAN_POINT('Ctrl Pts',(-1.01903673695377,-7.84755411822336,
35.1011813093271));
#64629=CARTESIAN_POINT('Ctrl Pts',(-1.21376752832503,-7.81980350027923,
35.0932950267108));
#64630=CARTESIAN_POINT('Ctrl Pts',(-1.40719678991613,-7.78483899605186,
35.0854087440944));
#64631=CARTESIAN_POINT('Ctrl Pts',(-1.60062571152781,-7.74987455327958,
35.0775224753394));
#64632=CARTESIAN_POINT('Ctrl Pts',(-1.7927527687319,-7.70769631023993,35.0696362065843));
#64633=CARTESIAN_POINT('Ctrl Pts',(-1.98300800320462,-7.65843327706303,
35.0617499378293));
#64634=CARTESIAN_POINT('Ctrl Pts',(-2.17329479104399,-7.60916207373223,
35.0538623611558));
#64635=CARTESIAN_POINT('Ctrl Pts',(-2.36170880402906,-7.55280382540219,
35.0459747844823));
#64636=CARTESIAN_POINT('Ctrl Pts',(-2.54769403726926,-7.48953777562158,
35.0380872078088));
#64637=CARTESIAN_POINT('Ctrl Pts',(-2.73374128792723,-7.42625062955838,
35.0301970009956));
#64638=CARTESIAN_POINT('Ctrl Pts',(-2.91735781917053,-7.35605120339168,
35.0223067941825));
#64639=CARTESIAN_POINT('Ctrl Pts',(-3.09800620248061,-7.27916743655424,
35.0144165873693));
#64640=CARTESIAN_POINT('Ctrl Pts',(-3.27882903094525,-7.20220942603777,
35.0065187612887));
#64641=CARTESIAN_POINT('Ctrl Pts',(-3.4566776692938,-7.11855431692191,34.9986209352081));
#64642=CARTESIAN_POINT('Ctrl Pts',(-3.63103700779795,-7.02847716422282,
34.9907231091275));
#64643=CARTESIAN_POINT('Ctrl Pts',(-3.80549289236293,-6.93835013410198,
34.9828209098713));
#64644=CARTESIAN_POINT('Ctrl Pts',(-3.97645532548991,-6.84179413942413,
34.9749187106152));
#64645=CARTESIAN_POINT('Ctrl Pts',(-4.14343668829894,-6.73912853491149,
34.967016511359));
#64646=CARTESIAN_POINT('Ctrl Pts',(-4.31061961027366,-6.63633900522994,
34.9591047735492));
#64647=CARTESIAN_POINT('Ctrl Pts',(-4.47381157744548,-6.52742532572589,
34.9511930357394));
#64648=CARTESIAN_POINT('Ctrl Pts',(-4.63255577967717,-6.41274886052617,
34.9432812979295));
#64649=CARTESIAN_POINT('Ctrl Pts',(-4.69822246707736,-6.36531138887956,
34.9400085005218));
#64650=CARTESIAN_POINT('Ctrl Pts',(-4.7631284715238,-6.31688826717927,34.9367357031141));
#64651=CARTESIAN_POINT('Ctrl Pts',(-4.82724324427238,-6.26750697332094,
34.9334629057065));
#64652=CARTESIAN_POINT('Ctrl Pts',(-4.9901329845309,-6.14204905176277,34.9251480494447));
#64653=CARTESIAN_POINT('Ctrl Pts',(-5.14826870260402,-6.01013011207214,
34.916833193183));
#64654=CARTESIAN_POINT('Ctrl Pts',(-5.30113670268692,-5.87212658748308,
34.9085183369213));
#64655=CARTESIAN_POINT('Ctrl Pts',(-5.45381645114158,-5.73429300943739,
34.900213720116));
#64656=CARTESIAN_POINT('Ctrl Pts',(-5.60124120300028,-5.59038998637751,
34.8919091033107));
#64657=CARTESIAN_POINT('Ctrl Pts',(-5.7429292391724,-5.44083493168638,34.8836044865055));
#64658=CARTESIAN_POINT('Ctrl Pts',(-5.88445213735088,-5.29145418403159,
34.8753095487655));
#64659=CARTESIAN_POINT('Ctrl Pts',(-6.02025145469556,-5.13643475578282,
34.8670146110256));
#64660=CARTESIAN_POINT('Ctrl Pts',(-6.14988073861615,-4.97623229972216,
34.8587196732856));
#64661=CARTESIAN_POINT('Ctrl Pts',(-6.27931573234284,-4.8162699573558,34.850437168115));
#64662=CARTESIAN_POINT('Ctrl Pts',(-6.40259896399246,-4.65114031746882,
34.8421546629444));
#64663=CARTESIAN_POINT('Ctrl Pts',(-6.51932278113482,-4.48133367150635,
34.8338721577738));
#64664=CARTESIAN_POINT('Ctrl Pts',(-6.63593937082608,-4.31168301713387,
34.8255972612639));
#64665=CARTESIAN_POINT('Ctrl Pts',(-6.74600839679552,-4.13736416539555,
34.8173223647539));
#64666=CARTESIAN_POINT('Ctrl Pts',(-6.84916312819214,-3.95889952428869,
34.809047468244));
#64667=CARTESIAN_POINT('Ctrl Pts',(-6.95219986410578,-3.7806390233239,34.8007820371304));
#64668=CARTESIAN_POINT('Ctrl Pts',(-7.04833794108248,-3.5982424491227,34.7925166060167));
#64669=CARTESIAN_POINT('Ctrl Pts',(-7.13725437163391,-3.41226039958745,
34.7842511749031));
#64670=CARTESIAN_POINT('Ctrl Pts',(-7.17200093136426,-3.33958275887612,
34.7810212286029));
#64671=CARTESIAN_POINT('Ctrl Pts',(-7.20564516586145,-3.26635789443598,
34.7777912823027));
#64672=CARTESIAN_POINT('Ctrl Pts',(-7.23816965150534,-3.1926197856975,34.7745613360024));
#64673=CARTESIAN_POINT('Ctrl Pts',(-7.31840746268982,-3.01070808659052,
34.7665930679041));
#64674=CARTESIAN_POINT('Ctrl Pts',(-7.39175938613969,-2.82582452526994,
34.7586247998057));
#64675=CARTESIAN_POINT('Ctrl Pts',(-7.45802138349776,-2.63852952291427,
34.7506565317073));
#64676=CARTESIAN_POINT('Ctrl Pts',(-7.52431377894204,-2.45114859785996,
34.7426846081184));
#64677=CARTESIAN_POINT('Ctrl Pts',(-7.58350965261639,-2.26135434108176,
34.7347126845296));
#64678=CARTESIAN_POINT('Ctrl Pts',(-7.63545481655088,-2.06972238341522,
34.7267407609407));
#64679=CARTESIAN_POINT('Ctrl Pts',(-7.68745901341395,-1.87787264617471,
34.7187597776828));
#64680=CARTESIAN_POINT('Ctrl Pts',(-7.73219595004951,-1.68418135819225,
34.7107787944248));
#64681=CARTESIAN_POINT('Ctrl Pts',(-7.76956228279999,-1.48923568775792,
34.7027978111669));
#64682=CARTESIAN_POINT('Ctrl Pts',(-7.80695234487526,-1.29416621793553,
34.6948117596207));
#64683=CARTESIAN_POINT('Ctrl Pts',(-7.83696241662768,-1.09784110643337,
34.6868257080745));
#64684=CARTESIAN_POINT('Ctrl Pts',(-7.85954098251039,-0.900853231242278,
34.6788396565284));
#64685=CARTESIAN_POINT('Ctrl Pts',(-7.882149948988,-0.70360012447599,34.6708428522745));
#64686=CARTESIAN_POINT('Ctrl Pts',(-7.89730739062614,-0.505682803529445,
34.6628460480207));
#64687=CARTESIAN_POINT('Ctrl Pts',(-7.90501385848876,-0.307696111611117,
34.6548492437669));
#64688=CARTESIAN_POINT('Ctrl Pts',(-7.90901433267791,-0.204920019511226,
34.6506980541969));
#64689=CARTESIAN_POINT('Ctrl Pts',(-7.91100784171156,-0.102125195674259,
34.6465468646269));
#64690=CARTESIAN_POINT('Ctrl Pts',(-7.91099997681615,0.000605652426356633,
34.6423956750568));
#64691=CARTESIAN_POINT('',(-7.91099996767813,-0.000709561171833796,32.6423600584031));
#64692=CARTESIAN_POINT('Ctrl Pts',(-7.9109999758377,0.000602220688781498,
34.642307277048));
#64693=CARTESIAN_POINT('Ctrl Pts',(-7.91082332165325,2.20207422639699,34.5537279183783));
#64694=CARTESIAN_POINT('Ctrl Pts',(-6.94199696978074,4.38623892820854,34.4651485597086));
#64695=CARTESIAN_POINT('Ctrl Pts',(-3.67820201488358,7.34180684107595,34.2879817653062));
#64696=CARTESIAN_POINT('Ctrl Pts',(-1.40868175871828,8.08992666571321,34.1993943295734));
#64697=CARTESIAN_POINT('Ctrl Pts',(2.97309270521185,7.6545422802529,34.022219458108));
#64698=CARTESIAN_POINT('Ctrl Pts',(5.05102072675523,6.47444880834286,33.9336320223753));
#64699=CARTESIAN_POINT('Ctrl Pts',(7.66951518847832,2.93425195367808,33.7564571509098));
#64700=CARTESIAN_POINT('Ctrl Pts',(8.18956872247062,0.601881960100311,33.6678697151771));
#64701=CARTESIAN_POINT('Ctrl Pts',(7.32306689761398,-3.71537198232339,33.4906948437116));
#64702=CARTESIAN_POINT('Ctrl Pts',(5.9432995885029,-5.66643518936416,33.4021074079789));
#64703=CARTESIAN_POINT('Ctrl Pts',(2.16154501637981,-7.9220591323296,33.2249325365135));
#64704=CARTESIAN_POINT('Ctrl Pts',(-0.210816529298928,-8.20894963713005,
33.1363451007807));
#64705=CARTESIAN_POINT('Ctrl Pts',(-4.42123908576307,-6.91982244717912,
32.9591702293153));
#64706=CARTESIAN_POINT('Ctrl Pts',(-6.22631625634084,-5.3539035880364,32.8705827935826));
#64707=CARTESIAN_POINT('Ctrl Pts',(-7.6530723291585,-2.31356269145162,32.7354502580342));
#64708=CARTESIAN_POINT('Ctrl Pts',(-7.91089457986223,-1.15750112512268,
32.6889051582187));
#64709=CARTESIAN_POINT('Ctrl Pts',(-7.91099996767813,-0.000709561171833796,
32.6423600584031));
#64710=CARTESIAN_POINT('',(-7.89985414996542,-0.000443308007164689,30.6422883933054));
#64711=CARTESIAN_POINT('Ctrl Pts',(-7.91099996745743,-0.000717557340472534,
32.6421607581184));
#64712=CARTESIAN_POINT('Ctrl Pts',(-7.91101730405701,0.190416768768663,
32.6344617805176));
#64713=CARTESIAN_POINT('Ctrl Pts',(-7.90410346812666,0.381778287241483,
32.6267628029168));
#64714=CARTESIAN_POINT('Ctrl Pts',(-7.89023511416832,0.572809604620282,
32.619063825316));
#64715=CARTESIAN_POINT('Ctrl Pts',(-7.87637563695231,0.763718648239245,
32.6113697756137));
#64716=CARTESIAN_POINT('Ctrl Pts',(-7.85557052456921,0.95429755069337,32.6036757259114));
#64717=CARTESIAN_POINT('Ctrl Pts',(-7.82784848039218,1.14398827267673,32.595981676209));
#64718=CARTESIAN_POINT('Ctrl Pts',(-7.80013838581885,1.33359722836102,32.5882909430314));
#64719=CARTESIAN_POINT('Ctrl Pts',(-7.76551734357096,1.52231840649562,32.5806002098538));
#64720=CARTESIAN_POINT('Ctrl Pts',(-7.72406595920795,1.70959821531406,32.5729094766762));
#64721=CARTESIAN_POINT('Ctrl Pts',(-7.68279797660037,1.89604940414253,32.5652527711671));
#64722=CARTESIAN_POINT('Ctrl Pts',(-7.63476005599379,2.08107160339361,32.557596065658));
#64723=CARTESIAN_POINT('Ctrl Pts',(-7.58008228976945,2.2641275318152,32.5499393601489));
#64724=CARTESIAN_POINT('Ctrl Pts',(-7.52104938203463,2.46176405720806,32.5416727900037));
#64725=CARTESIAN_POINT('Ctrl Pts',(-7.45431613058651,2.65697908205414,32.5334062198586));
#64726=CARTESIAN_POINT('Ctrl Pts',(-7.38011585245908,2.84917725041498,32.5251396497135));
#64727=CARTESIAN_POINT('Ctrl Pts',(-7.3058490900229,3.04154763056111,32.5168656726258));
#64728=CARTESIAN_POINT('Ctrl Pts',(-7.22410204983201,3.23089548380066,32.508591695538));
#64729=CARTESIAN_POINT('Ctrl Pts',(-7.13515557910966,3.41664687404191,32.5003177184503));
#64730=CARTESIAN_POINT('Ctrl Pts',(-7.04612363790539,3.60257675659107,32.4920357907289));
#64731=CARTESIAN_POINT('Ctrl Pts',(-6.94987858139909,3.78490301205503,32.4837538630074));
#64732=CARTESIAN_POINT('Ctrl Pts',(-6.84674683060963,3.96307694065318,32.475471935286));
#64733=CARTESIAN_POINT('Ctrl Pts',(-6.7434441268069,4.14154621350514,32.4671762792947));
#64734=CARTESIAN_POINT('Ctrl Pts',(-6.63323205361478,4.31584914412215,32.4588806233035));
#64735=CARTESIAN_POINT('Ctrl Pts',(-6.51648105415954,4.48546493362503,32.4505849673123));
#64736=CARTESIAN_POINT('Ctrl Pts',(-6.39962453439545,4.6552340229761,32.4422818136535));
#64737=CARTESIAN_POINT('Ctrl Pts',(-6.27621746330108,4.82030727749149,32.4339786599947));
#64738=CARTESIAN_POINT('Ctrl Pts',(-6.14667090140141,4.98019656538426,32.4256755063359));
#64739=CARTESIAN_POINT('Ctrl Pts',(-6.01692682805005,5.14032962636446,32.4173596933837));
#64740=CARTESIAN_POINT('Ctrl Pts',(-5.88102474355538,5.29526269852458,32.4090438804315));
#64741=CARTESIAN_POINT('Ctrl Pts',(-5.73941419321809,5.44454274652029,32.4007280674793));
#64742=CARTESIAN_POINT('Ctrl Pts',(-5.6844087286637,5.50252725663729,32.3974979751346));
#64743=CARTESIAN_POINT('Ctrl Pts',(-5.62854236594452,5.55965927475457,32.3942678827898));
#64744=CARTESIAN_POINT('Ctrl Pts',(-5.57184282595133,5.61591386355726,32.391037790445));
#64745=CARTESIAN_POINT('Ctrl Pts',(-5.43297740777338,5.75368953156892,32.3831268246019));
#64746=CARTESIAN_POINT('Ctrl Pts',(-5.28882350508073,5.88648540814427,32.3752158587587));
#64747=CARTESIAN_POINT('Ctrl Pts',(-5.13977266638553,6.0138721251683,32.3673048929155));
#64748=CARTESIAN_POINT('Ctrl Pts',(-4.99087265336391,6.14112993860767,32.3594019322387));
#64749=CARTESIAN_POINT('Ctrl Pts',(-4.83708583466091,6.26298927354107,32.3514989715618));
#64750=CARTESIAN_POINT('Ctrl Pts',(-4.67884126043563,6.37905678448194,32.343596010885));
#64751=CARTESIAN_POINT('Ctrl Pts',(-4.5207275301032,6.49502832546594,32.3356995847395));
#64752=CARTESIAN_POINT('Ctrl Pts',(-4.35816366340133,6.60521738028724,32.3278031585941));
#64753=CARTESIAN_POINT('Ctrl Pts',(-4.19161272993564,6.70926998430094,32.3199067324486));
#64754=CARTESIAN_POINT('Ctrl Pts',(-4.02516869464782,6.81325580373685,32.3120153745039));
#64755=CARTESIAN_POINT('Ctrl Pts',(-3.85474298242594,6.91111283785862,32.3041240165592));
#64756=CARTESIAN_POINT('Ctrl Pts',(-3.68082889719706,7.00252951650752,32.2962326586145));
#64757=CARTESIAN_POINT('Ctrl Pts',(-3.50699426637195,7.09390443052485,32.2883449059163));
#64758=CARTESIAN_POINT('Ctrl Pts',(-3.32967474266194,7.1788446924165,32.280457153218));
#64759=CARTESIAN_POINT('Ctrl Pts',(-3.14938981054062,7.25708376837851,32.2725694005198));
#64760=CARTESIAN_POINT('Ctrl Pts',(-2.9691539001017,7.33530157017697,32.2646837925982));
#64761=CARTESIAN_POINT('Ctrl Pts',(-2.7859545041022,7.40682168089425,32.2567981846765));
#64762=CARTESIAN_POINT('Ctrl Pts',(-2.60033300180316,7.47142484936664,32.2489125767549));
#64763=CARTESIAN_POINT('Ctrl Pts',(-2.41468960705884,7.5360356372221,32.2410260387943));
#64764=CARTESIAN_POINT('Ctrl Pts',(-2.22662385836511,7.59372773310941,32.2331395008336));
#64765=CARTESIAN_POINT('Ctrl Pts',(-2.03669489588992,7.64433089950036,32.225252962873));
#64766=CARTESIAN_POINT('Ctrl Pts',(-1.84674200595547,7.69494044093378,32.2173654313576));
#64767=CARTESIAN_POINT('Ctrl Pts',(-1.6549257674043,7.73845918388771,32.2094778998423));
#64768=CARTESIAN_POINT('Ctrl Pts',(-1.46181816204011,7.77476743453653,32.2015903683269));
#64769=CARTESIAN_POINT('Ctrl Pts',(-1.26865386169985,7.81108634502134,32.1937005210902));
#64770=CARTESIAN_POINT('Ctrl Pts',(-1.07419777761833,7.84019048089693,32.1858106738534));
#64771=CARTESIAN_POINT('Ctrl Pts',(-0.879029956633336,7.86201165957805,
32.1779208266167));
#64772=CARTESIAN_POINT('Ctrl Pts',(-0.683772122693678,7.8838429023607,32.1700273405195));
#64773=CARTESIAN_POINT('Ctrl Pts',(-0.487802239768998,7.89838445616257,
32.1621338544224));
#64774=CARTESIAN_POINT('Ctrl Pts',(-0.291703572906515,7.90562015439356,
32.1542403683252));
#64775=CARTESIAN_POINT('Ctrl Pts',(-0.0953782162571706,7.91286421708166,
32.146337757369));
#64776=CARTESIAN_POINT('Ctrl Pts',(0.101075877358963,7.91278554207477,32.1384351464129));
#64777=CARTESIAN_POINT('Ctrl Pts',(0.297076178164408,7.90542008652084,32.1305325354567));
#64778=CARTESIAN_POINT('Ctrl Pts',(0.493206477049126,7.89804974579546,32.1226246830584));
#64779=CARTESIAN_POINT('Ctrl Pts',(0.688882040664565,7.88338301527019,32.11471683066));
#64780=CARTESIAN_POINT('Ctrl Pts',(0.883527089932634,7.86150754508034,32.1068089782617));
#64781=CARTESIAN_POINT('Ctrl Pts',(1.07843846883588,7.83960214304268,32.0988903056783));
#64782=CARTESIAN_POINT('Ctrl Pts',(1.27231617759625,7.81046835095796,32.090971633095));
#64783=CARTESIAN_POINT('Ctrl Pts',(1.46459506826753,7.77424480486732,32.0830529605116));
#64784=CARTESIAN_POINT('Ctrl Pts',(1.54406350754329,7.75927369356743,32.0797801906868));
#64785=CARTESIAN_POINT('Ctrl Pts',(1.62325902643033,7.74309213452968,32.0765074208621));
#64786=CARTESIAN_POINT('Ctrl Pts',(1.70214257694173,7.72571237153974,32.0732346510373));
#64787=CARTESIAN_POINT('Ctrl Pts',(1.89118556037584,7.68406208798004,32.0653915181184));
#64788=CARTESIAN_POINT('Ctrl Pts',(2.0789953821601,7.63540366148418,32.0575483851995));
#64789=CARTESIAN_POINT('Ctrl Pts',(2.26500689276479,7.57981957408803,32.0497052522807));
#64790=CARTESIAN_POINT('Ctrl Pts',(2.45079995264848,7.5243007642864,32.0418713302866));
#64791=CARTESIAN_POINT('Ctrl Pts',(2.63479857353871,7.46187258822571,32.0340374082926));
#64792=CARTESIAN_POINT('Ctrl Pts',(2.81644624761652,7.3926687694152,32.0262034862985));
#64793=CARTESIAN_POINT('Ctrl Pts',(2.99791592318182,7.3235327641722,32.0183772408491));
#64794=CARTESIAN_POINT('Ctrl Pts',(3.17703891368189,7.24763446245187,32.0105509953995));
#64795=CARTESIAN_POINT('Ctrl Pts',(3.3532721819272,7.16515782616916,32.0027247499501));
#64796=CARTESIAN_POINT('Ctrl Pts',(3.52936701146528,7.08274597878255,31.9949046523483));
#64797=CARTESIAN_POINT('Ctrl Pts',(3.70257632308965,6.99376623725406,31.9870845547466));
#64798=CARTESIAN_POINT('Ctrl Pts',(3.87237526095857,6.89845133622874,31.9792644571449));
#64799=CARTESIAN_POINT('Ctrl Pts',(4.04207380478795,6.80319279037302,31.9714489831951));
#64800=CARTESIAN_POINT('Ctrl Pts',(4.20836568583172,6.70160671794843,31.9636335092453));
#64801=CARTESIAN_POINT('Ctrl Pts',(4.37074877749668,6.59397271180366,31.9558180352955));
#64802=CARTESIAN_POINT('Ctrl Pts',(4.53306740055944,6.48638143802624,31.9480056642099));
#64803=CARTESIAN_POINT('Ctrl Pts',(4.69148003350514,6.37274720845049,31.9401932931243));
#64804=CARTESIAN_POINT('Ctrl Pts',(4.84551162107078,6.25339412879662,31.9323809220387));
#64805=CARTESIAN_POINT('Ctrl Pts',(4.99953737799311,6.13404556708123,31.9245688466791));
#64806=CARTESIAN_POINT('Ctrl Pts',(5.14918213653042,6.0089787947287,31.9167567713195));
#64807=CARTESIAN_POINT('Ctrl Pts',(5.2940017910241,5.87855986076808,31.9089446959599));
#64808=CARTESIAN_POINT('Ctrl Pts',(5.4388256810409,5.7481371124605,31.9011323921215));
#64809=CARTESIAN_POINT('Ctrl Pts',(5.57882392393806,5.61236212559122,31.8933200882831));
#64810=CARTESIAN_POINT('Ctrl Pts',(5.71358736844511,5.47163964302699,31.8855077844447));
#64811=CARTESIAN_POINT('Ctrl Pts',(5.8483784664225,5.33088828419729,31.8776938775209));
#64812=CARTESIAN_POINT('Ctrl Pts',(5.97793238286326,5.18518766132498,31.8698799705971));
#64813=CARTESIAN_POINT('Ctrl Pts',(6.10187844259713,5.03497770320469,31.8620660636732));
#64814=CARTESIAN_POINT('Ctrl Pts',(6.22587174632039,4.88471049019722,31.8542491783559));
#64815=CARTESIAN_POINT('Ctrl Pts',(6.34425271182407,4.72993078924735,31.8464322930386));
#64816=CARTESIAN_POINT('Ctrl Pts',(6.4566923009425,4.57110987955331,31.8386154077213));
#64817=CARTESIAN_POINT('Ctrl Pts',(6.5692538632265,4.41211668277367,31.8307900427373));
#64818=CARTESIAN_POINT('Ctrl Pts',(6.67586097316177,4.24907380864018,31.8229646777532));
#64819=CARTESIAN_POINT('Ctrl Pts',(6.77622856060272,4.08248055653324,31.8151393127691));
#64820=CARTESIAN_POINT('Ctrl Pts',(6.87665714701675,3.91578605642824,31.8073091918749));
#64821=CARTESIAN_POINT('Ctrl Pts',(6.97083848387219,3.74553718491091,31.7994790709807));
#64822=CARTESIAN_POINT('Ctrl Pts',(7.05853444472115,3.57225593885505,31.7916489500865));
#64823=CARTESIAN_POINT('Ctrl Pts',(7.14635028013734,3.39873782881844,31.7838081259359));
#64824=CARTESIAN_POINT('Ctrl Pts',(7.22766288666815,3.22217938360985,31.7759673017853));
#64825=CARTESIAN_POINT('Ctrl Pts',(7.30228263624338,3.04312163746677,31.7681264776346));
#64826=CARTESIAN_POINT('Ctrl Pts',(7.34255455859735,2.94648502731197,31.7638948222997));
#64827=CARTESIAN_POINT('Ctrl Pts',(7.38087790776481,2.84912070401904,31.7596631669647));
#64828=CARTESIAN_POINT('Ctrl Pts',(7.41722899812936,2.75111522646889,31.7554315116297));
#64829=CARTESIAN_POINT('Ctrl Pts',(7.48518817495826,2.5678917932173,31.7475203372934));
#64830=CARTESIAN_POINT('Ctrl Pts',(7.54644557606945,2.38190244921842,31.7396091629571));
#64831=CARTESIAN_POINT('Ctrl Pts',(7.60076925248574,2.19367904910163,31.7316979886208));
#64832=CARTESIAN_POINT('Ctrl Pts',(7.6550340349838,2.00565970758809,31.7237953910246));
#64833=CARTESIAN_POINT('Ctrl Pts',(7.70237997089292,1.81541146255084,31.7158927934285));
#64834=CARTESIAN_POINT('Ctrl Pts',(7.74262326082517,1.62348576862533,31.7079901958323));
#64835=CARTESIAN_POINT('Ctrl Pts',(7.7828303920864,1.43173252029361,31.7000946987347));
#64836=CARTESIAN_POINT('Ctrl Pts',(7.81594752004121,1.23830516089803,31.6921992016372));
#64837=CARTESIAN_POINT('Ctrl Pts',(7.84184065013985,1.04377019396713,31.6843037045397));
#64838=CARTESIAN_POINT('Ctrl Pts',(7.86771532020873,0.849373917154589,31.6764138363913));
#64839=CARTESIAN_POINT('Ctrl Pts',(7.88637620810694,0.653871946477836,31.6685239682429));
#64840=CARTESIAN_POINT('Ctrl Pts',(7.89774034043308,0.457841146136858,31.6606341000945));
#64841=CARTESIAN_POINT('Ctrl Pts',(7.90909847928391,0.261913732990894,31.6527483930847));
#64842=CARTESIAN_POINT('Ctrl Pts',(7.91316751097663,0.0654583893702774,
31.6448626860749));
#64843=CARTESIAN_POINT('Ctrl Pts',(7.90991624966504,-0.130942442641423,
31.6369769790651));
#64844=CARTESIAN_POINT('Ctrl Pts',(7.90666609997367,-0.327276124364865,
31.6290939682124));
#64845=CARTESIAN_POINT('Ctrl Pts',(7.89610065123511,-0.523554987258206,
31.6212109573598));
#64846=CARTESIAN_POINT('Ctrl Pts',(7.8782408148018,-0.719195845365574,31.6133279465071));
#64847=CARTESIAN_POINT('Ctrl Pts',(7.86038071183727,-0.914839623118703,
31.6054448180123));
#64848=CARTESIAN_POINT('Ctrl Pts',(7.83522602659116,-1.10984503292152,31.5975616895176));
#64849=CARTESIAN_POINT('Ctrl Pts',(7.80284965968011,-1.30363268923034,31.5896785610228));
#64850=CARTESIAN_POINT('Ctrl Pts',(7.77047129090595,-1.4974323276236,31.5817949451063));
#64851=CARTESIAN_POINT('Ctrl Pts',(7.73087040698091,-1.69001372207064,31.5739113291898));
#64852=CARTESIAN_POINT('Ctrl Pts',(7.68417129613581,-1.88080634081302,31.5660277132734));
#64853=CARTESIAN_POINT('Ctrl Pts',(7.63746144796589,-2.07164282767804,31.5581422847111));
#64854=CARTESIAN_POINT('Ctrl Pts',(7.58365020274053,-2.26068938422741,31.5502568561489));
#64855=CARTESIAN_POINT('Ctrl Pts',(7.52291217691596,-2.44738909420009,31.5423714275867));
#64856=CARTESIAN_POINT('Ctrl Pts',(7.46214997598967,-2.63416311486068,31.5344828604464));
#64857=CARTESIAN_POINT('Ctrl Pts',(7.39445560748082,-2.81858809992278,31.526594293306));
#64858=CARTESIAN_POINT('Ctrl Pts',(7.32005250441971,-3.00012538613618,31.5187057261657));
#64859=CARTESIAN_POINT('Ctrl Pts',(7.24557022028299,-3.18185586748518,31.5108087638751));
#64860=CARTESIAN_POINT('Ctrl Pts',(7.16436507186001,-3.36069219243615,31.5029118015845));
#64861=CARTESIAN_POINT('Ctrl Pts',(7.07670777418312,-3.53611765624621,31.4950148392939));
#64862=CARTESIAN_POINT('Ctrl Pts',(6.98899701721613,-3.71165010625147,31.4871130609069));
#64863=CARTESIAN_POINT('Ctrl Pts',(6.89482643122074,-3.88376724624117,31.4792112825198));
#64864=CARTESIAN_POINT('Ctrl Pts',(6.79451119570603,-4.05197959168422,31.4713095041328));
#64865=CARTESIAN_POINT('Ctrl Pts',(6.69406621795305,-4.22040949377348,31.4633975060178));
#64866=CARTESIAN_POINT('Ctrl Pts',(6.58746090398517,-4.38492422541705,31.4554855079029));
#64867=CARTESIAN_POINT('Ctrl Pts',(6.47505265009752,-4.5450648156506,31.4475735097879));
#64868=CARTESIAN_POINT('Ctrl Pts',(6.42795474755298,-4.61216207631781,31.4442584639326));
#64869=CARTESIAN_POINT('Ctrl Pts',(6.37983859997287,-4.67849185985307,31.4409434180773));
#64870=CARTESIAN_POINT('Ctrl Pts',(6.33073248300737,-4.74402226265807,31.4376283722221));
#64871=CARTESIAN_POINT('Ctrl Pts',(6.2135435582011,-4.90040680131411,31.4297172058853));
#64872=CARTESIAN_POINT('Ctrl Pts',(6.09039907079601,-5.05265666110265,31.4218060395486));
#64873=CARTESIAN_POINT('Ctrl Pts',(5.96162041120069,-5.20028874897879,31.4138948732119));
#64874=CARTESIAN_POINT('Ctrl Pts',(5.83298134359543,-5.34776080834547,31.405992282329));
#64875=CARTESIAN_POINT('Ctrl Pts',(5.69872049319156,-5.49062480853605,31.3980896914461));
#64876=CARTESIAN_POINT('Ctrl Pts',(5.55920180975748,-5.62842751027222,31.3901871005632));
#64877=CARTESIAN_POINT('Ctrl Pts',(5.41980846159799,-5.76610641826955,31.3822916088972));
#64878=CARTESIAN_POINT('Ctrl Pts',(5.27516693347967,-5.89873284458451,31.3743961172313));
#64879=CARTESIAN_POINT('Ctrl Pts',(5.12568080582907,-6.02588726054142,31.3665006255653));
#64880=CARTESIAN_POINT('Ctrl Pts',(4.97630122743358,-6.15295104462155,31.3586107615704));
#64881=CARTESIAN_POINT('Ctrl Pts',(4.82208419082698,-6.27455036654056,31.3507208975755));
#64882=CARTESIAN_POINT('Ctrl Pts',(4.66346962535559,-6.39030297039082,31.3428310335807));
#64883=CARTESIAN_POINT('Ctrl Pts',(4.50493868805716,-6.50599454467078,31.3349453294491));
#64884=CARTESIAN_POINT('Ctrl Pts',(4.34201511982195,-6.61584534065912,31.3270596253175));
#64885=CARTESIAN_POINT('Ctrl Pts',(4.17517159395903,-6.71951361044813,31.3191739211859));
#64886=CARTESIAN_POINT('Ctrl Pts',(4.00838508569865,-6.82314645233442,31.3112909119383));
#64887=CARTESIAN_POINT('Ctrl Pts',(3.8376815822631,-6.92060079721286,31.3034079026907));
#64888=CARTESIAN_POINT('Ctrl Pts',(3.66356260546471,-7.01157828422679,31.2955248934431));
#64889=CARTESIAN_POINT('Ctrl Pts',(3.48944098816572,-7.10255715090715,31.2876417646503));
#64890=CARTESIAN_POINT('Ctrl Pts',(3.31190409569383,-7.18705879629818,31.2797586358574));
#64891=CARTESIAN_POINT('Ctrl Pts',(3.13147842034112,-7.26483061763575,31.2718755070646));
#64892=CARTESIAN_POINT('Ctrl Pts',(2.95104156192538,-7.34260725939136,31.2639918896632));
#64893=CARTESIAN_POINT('Ctrl Pts',(2.76771588046419,-7.41365310879269,31.2561082722619));
#64894=CARTESIAN_POINT('Ctrl Pts',(2.58204826506268,-7.47776355315457,31.2482246548605));
#64895=CARTESIAN_POINT('Ctrl Pts',(2.39633793195291,-7.54188874780692,31.240339223626));
#64896=CARTESIAN_POINT('Ctrl Pts',(2.20828491727192,-7.59907524520427,31.2324537923915));
#64897=CARTESIAN_POINT('Ctrl Pts',(2.01845193058505,-7.64916811188756,31.2245683611571));
#64898=CARTESIAN_POINT('Ctrl Pts',(1.8285433575136,-7.69928092420175,31.2166797901562));
#64899=CARTESIAN_POINT('Ctrl Pts',(1.63685373345786,-7.74229438980108,31.2087912191553));
#64900=CARTESIAN_POINT('Ctrl Pts',(1.44395687147668,-7.77810449616841,31.2009026481544));
#64901=CARTESIAN_POINT('Ctrl Pts',(1.25085468200666,-7.81395272031091,31.1930056802285));
#64902=CARTESIAN_POINT('Ctrl Pts',(1.05654302709883,-7.84258220703017,31.1851087123026));
#64903=CARTESIAN_POINT('Ctrl Pts',(0.861602877452391,-7.8639405822759,31.1772117443768));
#64904=CARTESIAN_POINT('Ctrl Pts',(0.666543815081898,-7.88531198604647,
31.1693099593316));
#64905=CARTESIAN_POINT('Ctrl Pts',(0.470855836739858,-7.89940341115062,
31.1614081742864));
#64906=CARTESIAN_POINT('Ctrl Pts',(0.275121121529162,-7.90621460425206,
31.1535063892411));
#64907=CARTESIAN_POINT('Ctrl Pts',(0.0791332165088265,-7.91303460787381,
31.1455943829562));
#64908=CARTESIAN_POINT('Ctrl Pts',(-0.116901202330898,-7.91255557032341,
31.1376823766712));
#64909=CARTESIAN_POINT('Ctrl Pts',(-0.312402733260923,-7.90482925383282,
31.1297703703863));
#64910=CARTESIAN_POINT('Ctrl Pts',(-0.394315779947933,-7.9015920100097,
31.1264553245289));
#64911=CARTESIAN_POINT('Ctrl Pts',(-0.47613536764902,-7.89708311507568,
31.1231402786716));
#64912=CARTESIAN_POINT('Ctrl Pts',(-0.557819362036135,-7.89130905232697,
31.1198252328143));
#64913=CARTESIAN_POINT('Ctrl Pts',(-0.751008376246334,-7.87765294382273,
31.1119848909451));
#64914=CARTESIAN_POINT('Ctrl Pts',(-0.943986168014457,-7.8568777548247,
31.1041445490759));
#64915=CARTESIAN_POINT('Ctrl Pts',(-1.13618127400415,-7.82898544593118,
31.0963042072067));
#64916=CARTESIAN_POINT('Ctrl Pts',(-1.32816150014477,-7.80112432146921,
31.0884726310731));
#64917=CARTESIAN_POINT('Ctrl Pts',(-1.51936043865765,-7.76616197153333,
31.0806410549395));
#64918=CARTESIAN_POINT('Ctrl Pts',(-1.70920800755183,-7.72415231510363,
31.0728094788059));
#64919=CARTESIAN_POINT('Ctrl Pts',(-1.89888023579474,-7.68218145822538,
31.0649851358102));
#64920=CARTESIAN_POINT('Ctrl Pts',(-2.08720323917296,-7.63317633233087,
31.0571607928146));
#64921=CARTESIAN_POINT('Ctrl Pts',(-2.27361323890234,-7.57724249578222,
31.049336449819));
#64922=CARTESIAN_POINT('Ctrl Pts',(-2.4598872999808,-7.52134944873142,31.0415178126901));
#64923=CARTESIAN_POINT('Ctrl Pts',(-2.64425080075974,-7.45853785530182,
31.0336991755613));
#64924=CARTESIAN_POINT('Ctrl Pts',(-2.82615113501385,-7.38896411968958,
31.0258805384325));
#64925=CARTESIAN_POINT('Ctrl Pts',(-3.00795415728584,-7.31942760422947,
31.0180660840726));
#64926=CARTESIAN_POINT('Ctrl Pts',(-3.18729631045722,-7.24313627821234,
31.0102516297128));
#64927=CARTESIAN_POINT('Ctrl Pts',(-3.3636409316227,-7.160296130965,31.0024371753529));
#64928=CARTESIAN_POINT('Ctrl Pts',(-3.53992546341619,-7.07748421147075,
30.9946253837659));
#64929=CARTESIAN_POINT('Ctrl Pts',(-3.71321418047056,-6.98812806626,30.9868135921788));
#64930=CARTESIAN_POINT('Ctrl Pts',(-3.88299099028596,-6.89248155379164,
30.9790018005917));
#64931=CARTESIAN_POINT('Ctrl Pts',(-4.05277574593132,-6.79683056491143,
30.9711896434001));
#64932=CARTESIAN_POINT('Ctrl Pts',(-4.21904795512081,-6.69488878522707,
30.9633774862085));
#64933=CARTESIAN_POINT('Ctrl Pts',(-4.3813162531998,-6.58695596534904,30.9555653290169));
#64934=CARTESIAN_POINT('Ctrl Pts',(-4.54359781685918,-6.47901432186519,
30.9477525331744));
#64935=CARTESIAN_POINT('Ctrl Pts',(-4.70187452392754,-6.36508085674399,
30.9399397373319));
#64936=CARTESIAN_POINT('Ctrl Pts',(-4.85568420710096,-6.24549852941383,
30.9321269414894));
#64937=CARTESIAN_POINT('Ctrl Pts',(-5.00953352848999,-6.12588538458261,
30.9243121322152));
#64938=CARTESIAN_POINT('Ctrl Pts',(-5.15891325492716,-6.00062069333281,
30.916497322941));
#64939=CARTESIAN_POINT('Ctrl Pts',(-5.30339439317307,-5.8700876407819,30.9086825136668));
#64940=CARTESIAN_POINT('Ctrl Pts',(-5.44793819044681,-5.73949797825219,
30.9008643152419));
#64941=CARTESIAN_POINT('Ctrl Pts',(-5.58757890682345,-5.60363563853184,
30.893046116817));
#64942=CARTESIAN_POINT('Ctrl Pts',(-5.72192438807513,-5.46292067461637,
30.8852279183922));
#64943=CARTESIAN_POINT('Ctrl Pts',(-5.85642624673967,-5.32204191924472,
30.8774006196266));
#64944=CARTESIAN_POINT('Ctrl Pts',(-5.98562031693983,-5.17629951264028,
30.8695733208611));
#64945=CARTESIAN_POINT('Ctrl Pts',(-6.10915402742201,-5.02614743807157,
30.8617460220956));
#64946=CARTESIAN_POINT('Ctrl Pts',(-6.23276838121355,-4.87589734361702,
30.8539136136375));
#64947=CARTESIAN_POINT('Ctrl Pts',(-6.35071479910128,-4.72123212319134,
30.8460812051795));
#64948=CARTESIAN_POINT('Ctrl Pts',(-6.46268402166588,-4.56263479100667,
30.8382487967214));
#64949=CARTESIAN_POINT('Ctrl Pts',(-6.57481393584329,-4.40380984930117,
30.8304051476535));
#64950=CARTESIAN_POINT('Ctrl Pts',(-6.68094933047527,-4.24104181829432,
30.8225614985856));
#64951=CARTESIAN_POINT('Ctrl Pts',(-6.78082628644783,-4.07483936775649,
30.8147178495177));
#64952=CARTESIAN_POINT('Ctrl Pts',(-6.8347133426367,-3.98516742387666,30.810485930814));
#64953=CARTESIAN_POINT('Ctrl Pts',(-6.88677940065042,-3.89449610642381,
30.8062540121104));
#64954=CARTESIAN_POINT('Ctrl Pts',(-6.93698886021879,-3.8029076445794,30.8020220934067));
#64955=CARTESIAN_POINT('Ctrl Pts',(-7.03702128819584,-3.62043573008878,
30.7935908315175));
#64956=CARTESIAN_POINT('Ctrl Pts',(-7.12994872693167,-3.43383525325003,
30.7851595696284));
#64957=CARTESIAN_POINT('Ctrl Pts',(-7.2154380065385,-3.24366696407009,30.7767283077393));
#64958=CARTESIAN_POINT('Ctrl Pts',(-7.30078206904377,-3.05382170589345,
30.7683113676859));
#64959=CARTESIAN_POINT('Ctrl Pts',(-7.37871306135141,-2.86042097340825,
30.7598944276324));
#64960=CARTESIAN_POINT('Ctrl Pts',(-7.44894322862298,-2.66405063329356,
30.751477487579));
#64961=CARTESIAN_POINT('Ctrl Pts',(-7.5190551931533,-2.46801079947557,30.7430747138792));
#64962=CARTESIAN_POINT('Ctrl Pts',(-7.58149209220624,-2.26901158538908,
30.7346719401795));
#64963=CARTESIAN_POINT('Ctrl Pts',(-7.63601347913692,-2.06766030731337,
30.7262691664797));
#64964=CARTESIAN_POINT('Ctrl Pts',(-7.69040594310445,-1.86678515071707,
30.7178862622393));
#64965=CARTESIAN_POINT('Ctrl Pts',(-7.73692016983713,-1.66356929268312,
30.7095033579989));
#64966=CARTESIAN_POINT('Ctrl Pts',(-7.77536500274913,-1.45863637484604,
30.7011204537585));
#64967=CARTESIAN_POINT('Ctrl Pts',(-7.81375381875048,-1.25400205913772,
30.6927497640178));
#64968=CARTESIAN_POINT('Ctrl Pts',(-7.84409663700915,-1.04765594202256,
30.6843790742771));
#64969=CARTESIAN_POINT('Ctrl Pts',(-7.86625228079528,-0.840235713882164,
30.6760083845363));
#64970=CARTESIAN_POINT('Ctrl Pts',(-7.88836370980692,-0.633229422646547,
30.6676543997112));
#64971=CARTESIAN_POINT('Ctrl Pts',(-7.90232053262437,-0.425153570025834,
30.6593004148861));
#64972=CARTESIAN_POINT('Ctrl Pts',(-7.90803273194084,-0.216654818899259,
30.6509464300609));
#64973=CARTESIAN_POINT('Ctrl Pts',(-7.90999627195931,-0.144984413341794,
30.648074789453));
#64974=CARTESIAN_POINT('Ctrl Pts',(-7.91098606472354,-0.0732641305949829,
30.645203148845));
#64975=CARTESIAN_POINT('Ctrl Pts',(-7.91099985387987,-0.00152049748538701,
30.6423315082371));
#64976=CARTESIAN_POINT('',(-7.91184153648199,4.99451412439681E-5,28.6437895940631));
#64977=CARTESIAN_POINT('Ctrl Pts',(-7.89546650976364,-1.92594324088665E-5,
30.6422714205947));
#64978=CARTESIAN_POINT('Ctrl Pts',(-7.89546412269911,0.00218135211731857,
30.6421831647693));
#64979=CARTESIAN_POINT('Ctrl Pts',(-7.89546128372232,0.00411991532010145,
30.6421054184775));
#64980=CARTESIAN_POINT('Ctrl Pts',(-7.89545723413254,0.00631726536019909,
30.6420172935349));
#64981=CARTESIAN_POINT('Ctrl Pts',(-7.89502030649362,0.243398801313106,
30.632509114881));
#64982=CARTESIAN_POINT('Ctrl Pts',(-7.88409107758035,0.480852628331748,
30.6232175521955));
#64983=CARTESIAN_POINT('Ctrl Pts',(-7.86274775425919,0.717537746077602,
30.6140618702597));
#64984=CARTESIAN_POINT('Ctrl Pts',(-7.84133330654603,0.955011592216039,
30.6048756779718));
#64985=CARTESIAN_POINT('Ctrl Pts',(-7.80943596256734,1.1917110943165,30.5958262735592));
#64986=CARTESIAN_POINT('Ctrl Pts',(-7.76716639284816,1.42652545074094,30.5868321119856));
#64987=CARTESIAN_POINT('Ctrl Pts',(-7.72491866505277,1.66121847171497,30.5778425979586));
#64988=CARTESIAN_POINT('Ctrl Pts',(-7.67231018451083,1.8940279712867,30.568908269694));
#64989=CARTESIAN_POINT('Ctrl Pts',(-7.60947191037755,2.12389257139215,30.5599477085005));
#64990=CARTESIAN_POINT('Ctrl Pts',(-7.54678661352194,2.35319757527631,30.5510089614365));
#64991=CARTESIAN_POINT('Ctrl Pts',(-7.4739220288526,2.57957185345583,30.5420441090141));
#64992=CARTESIAN_POINT('Ctrl Pts',(-7.39101717471166,2.80201274063794,30.5329723257269));
#64993=CARTESIAN_POINT('Ctrl Pts',(-7.30838812292402,3.02371362627498,30.5239307218448));
#64994=CARTESIAN_POINT('Ctrl Pts',(-7.21578623579024,3.24150726677263,30.5147828973754));
#64995=CARTESIAN_POINT('Ctrl Pts',(-7.11334689049767,3.45445261467261,30.5054488307867));
#64996=CARTESIAN_POINT('Ctrl Pts',(-7.06218249042566,3.56081039099685,30.5007868338178));
#64997=CARTESIAN_POINT('Ctrl Pts',(-7.00856392603403,3.66595951555365,30.4960783767544));
#64998=CARTESIAN_POINT('Ctrl Pts',(-6.95250697360272,3.76978749396466,30.4913134892526));
#64999=CARTESIAN_POINT('Ctrl Pts',(-6.84121380227646,3.97592329850941,30.4818534772809));
#65000=CARTESIAN_POINT('Ctrl Pts',(-6.72031101138611,4.17684884004786,30.4721710362662));
#65001=CARTESIAN_POINT('Ctrl Pts',(-6.59068832436126,4.37211674975882,30.4621881423824));
#65002=CARTESIAN_POINT('Ctrl Pts',(-6.47029688634264,4.55347840016564,30.452916193329));
#65003=CARTESIAN_POINT('Ctrl Pts',(-6.34238358593672,4.72996025928655,30.4433850618682));
#65004=CARTESIAN_POINT('Ctrl Pts',(-6.20763774264494,4.90123666969266,30.433532234907));
#65005=CARTESIAN_POINT('Ctrl Pts',(-6.09888078764801,5.03947841729326,30.4255797561349));
#65006=CARTESIAN_POINT('Ctrl Pts',(-5.98543685338641,5.17396077302761,30.4176635528211));
#65007=CARTESIAN_POINT('Ctrl Pts',(-5.86747184415262,5.30437293182994,30.4098965082411));
#65008=CARTESIAN_POINT('Ctrl Pts',(-5.74963212763683,5.43464657757706,30.4021377131763));
#65009=CARTESIAN_POINT('Ctrl Pts',(-5.62728033527176,5.56085838282157,30.3945277601652));
#65010=CARTESIAN_POINT('Ctrl Pts',(-5.50060359947352,5.68265147185828,30.3871791731794));
#65011=CARTESIAN_POINT('Ctrl Pts',(-5.43746134417914,5.74335946431315,30.3835162562863));
#65012=CARTESIAN_POINT('Ctrl Pts',(-5.3732449336438,5.80296890158039,30.3799182768963));
#65013=CARTESIAN_POINT('Ctrl Pts',(-5.30798024592445,5.86143156577821,30.3763991702581));
#65014=CARTESIAN_POINT('Ctrl Pts',(-5.08331837819765,6.06267869941112,30.3642852829831));
#65015=CARTESIAN_POINT('Ctrl Pts',(-4.84690886434787,6.2514706121673,30.3523459441257));
#65016=CARTESIAN_POINT('Ctrl Pts',(-4.60054071673013,6.42659030156861,30.3405140373188));
#65017=CARTESIAN_POINT('Ctrl Pts',(-4.50088145039366,6.49742859757221,30.3357278701005));
#65018=CARTESIAN_POINT('Ctrl Pts',(-4.39959251112845,6.56603028009268,30.3309592821233));
#65019=CARTESIAN_POINT('Ctrl Pts',(-4.29679155596662,6.63231708308071,30.326203830883));
#65020=CARTESIAN_POINT('Ctrl Pts',(-4.04082351634497,6.79736713526092,30.3143630505171));
#65021=CARTESIAN_POINT('Ctrl Pts',(-3.77548350392549,6.94806249708131,30.3026037152006));
#65022=CARTESIAN_POINT('Ctrl Pts',(-3.5026855417861,7.08340682054121,30.2908572455461));
#65023=CARTESIAN_POINT('Ctrl Pts',(-3.22956687612411,7.21891025589828,30.2790969666455));
#65024=CARTESIAN_POINT('Ctrl Pts',(-2.94897345341156,7.33902731325784,30.2673495836747));
#65025=CARTESIAN_POINT('Ctrl Pts',(-2.66278861089816,7.44279415657953,30.2555462750944));
#65026=CARTESIAN_POINT('Ctrl Pts',(-2.37764267387871,7.54618430649331,30.2437858147727));
#65027=CARTESIAN_POINT('Ctrl Pts',(-2.08694631195099,7.63334365571279,30.2319698341457));
#65028=CARTESIAN_POINT('Ctrl Pts',(-1.79251626616018,7.70334184067585,30.2200302584625));
#65029=CARTESIAN_POINT('Ctrl Pts',(-1.5006846181593,7.7727222791429,30.2081960516692));
#65030=CARTESIAN_POINT('Ctrl Pts',(-1.20518508910376,7.82524412846403,30.1962404216906));
#65031=CARTESIAN_POINT('Ctrl Pts',(-0.907736453985132,7.86000968883437,
30.1840970802323));
#65032=CARTESIAN_POINT('Ctrl Pts',(-0.805063307239477,7.87201004472833,
30.1799054486956));
#65033=CARTESIAN_POINT('Ctrl Pts',(-0.702157472595626,7.8818947616983,30.1756914515555));
#65034=CARTESIAN_POINT('Ctrl Pts',(-0.599088191656171,7.88962680232436,
30.1714523625255));
#65035=CARTESIAN_POINT('Ctrl Pts',(-0.306040219117324,7.91161064473019,
30.1593997273045));
#65036=CARTESIAN_POINT('Ctrl Pts',(-0.0116744980615128,7.9161938128868,
30.1471442526803));
#65037=CARTESIAN_POINT('Ctrl Pts',(0.28236443491014,7.90424368096634,30.1346232772743));
#65038=CARTESIAN_POINT('Ctrl Pts',(0.449042743781442,7.89746965359806,30.127525662734));
#65039=CARTESIAN_POINT('Ctrl Pts',(0.615616935621651,7.88538273710484,30.1203427353734));
#65040=CARTESIAN_POINT('Ctrl Pts',(0.781794208160822,7.86813767748803,30.1130630815916));
#65041=CARTESIAN_POINT('Ctrl Pts',(0.990485363128304,7.84648073635568,30.1039210410931));
#65042=CARTESIAN_POINT('Ctrl Pts',(1.19810556530782,7.81614683836484,30.0949825327481));
#65043=CARTESIAN_POINT('Ctrl Pts',(1.40410903431245,7.77756160137206,30.0861910988723));
#65044=CARTESIAN_POINT('Ctrl Pts',(1.61232268313516,7.7385623892531,30.0773053430425));
#65045=CARTESIAN_POINT('Ctrl Pts',(1.81888521446852,7.69113406978758,30.0685698344904));
#65046=CARTESIAN_POINT('Ctrl Pts',(2.02326640029138,7.63567381629991,30.059926278788));
#65047=CARTESIAN_POINT('Ctrl Pts',(2.23031076776408,7.57949088998504,30.0511700935456));
#65048=CARTESIAN_POINT('Ctrl Pts',(2.43511714741324,7.51506559391288,30.0425082731425));
#65049=CARTESIAN_POINT('Ctrl Pts',(2.63716020931853,7.44276395616095,30.0338802145172));
#65050=CARTESIAN_POINT('Ctrl Pts',(2.7593900790063,7.39902367783961,30.0286605030781));
#65051=CARTESIAN_POINT('Ctrl Pts',(2.88060907249666,7.35239983002036,30.0234531480436));
#65052=CARTESIAN_POINT('Ctrl Pts',(3.00070395312335,7.30296474165692,30.0182447311977));
#65053=CARTESIAN_POINT('Ctrl Pts',(3.25343976420335,7.19893018924178,30.0072837855759));
#65054=CARTESIAN_POINT('Ctrl Pts',(3.50117487065036,7.08200517932002,29.9965506364678));
#65055=CARTESIAN_POINT('Ctrl Pts',(3.74248687266088,6.95291237079717,29.9859497658109));
#65056=CARTESIAN_POINT('Ctrl Pts',(3.99168009790156,6.81960340546115,29.9750026718937));
#65057=CARTESIAN_POINT('Ctrl Pts',(4.23402402383837,6.67332010383523,29.964196637924));
#65058=CARTESIAN_POINT('Ctrl Pts',(4.46800670144774,6.51483954969744,29.9534264780255));
#65059=CARTESIAN_POINT('Ctrl Pts',(4.69448803737438,6.36143978529503,29.9430016028729));
#65060=CARTESIAN_POINT('Ctrl Pts',(4.91313658488023,6.19661310307585,29.9326103384614));
#65061=CARTESIAN_POINT('Ctrl Pts',(5.12262184026173,6.02103222294843,29.9221572946339));
#65062=CARTESIAN_POINT('Ctrl Pts',(5.32917845457106,5.84790599470614,29.9118503862153));
#65063=CARTESIAN_POINT('Ctrl Pts',(5.52682713705019,5.66432485566542,29.9014834136807));
#65064=CARTESIAN_POINT('Ctrl Pts',(5.71431895097915,5.4708910518928,29.8909649319167));
#65065=CARTESIAN_POINT('Ctrl Pts',(5.89586083992772,5.28359573810009,29.8807802470055));
#65066=CARTESIAN_POINT('Ctrl Pts',(6.06788130357792,5.08706353728799,29.8704535163693));
#65067=CARTESIAN_POINT('Ctrl Pts',(6.22925714558252,4.88179344435557,29.8599017273886));
#65068=CARTESIAN_POINT('Ctrl Pts',(6.25606745649414,4.84769072523719,29.8581486970729));
#65069=CARTESIAN_POINT('Ctrl Pts',(6.28258396788685,4.81334671390474,29.8563894548956));
#65070=CARTESIAN_POINT('Ctrl Pts',(6.30880152702889,4.77876355552774,29.8546236201992));
#65071=CARTESIAN_POINT('Ctrl Pts',(6.32705822238815,4.75468144385483,29.8533939746044));
#65072=CARTESIAN_POINT('Ctrl Pts',(6.34516995295352,4.73048336668523,29.852161132241));
#65073=CARTESIAN_POINT('Ctrl Pts',(6.36313657566678,4.70617129738668,29.8509249645731));
#65074=CARTESIAN_POINT('Ctrl Pts',(6.50761186100613,4.51067027278374,29.8409845500948));
#65075=CARTESIAN_POINT('Ctrl Pts',(6.6423066129919,4.30831997422948,29.8308633426248));
#65076=CARTESIAN_POINT('Ctrl Pts',(6.76708109523822,4.10009238934386,29.8206455720084));
#65077=CARTESIAN_POINT('Ctrl Pts',(6.89684698153664,3.8835349922062,29.8100190557835));
#65078=CARTESIAN_POINT('Ctrl Pts',(7.01588253952261,3.66061966769824,29.7992880961758));
#65079=CARTESIAN_POINT('Ctrl Pts',(7.12397765144178,3.43245841341115,29.7885474412361));
#65080=CARTESIAN_POINT('Ctrl Pts',(7.23329173525428,3.20172421987469,29.7776856655885));
#65081=CARTESIAN_POINT('Ctrl Pts',(7.33141638311738,2.96562429015909,29.7668139747105));
#65082=CARTESIAN_POINT('Ctrl Pts',(7.41809190885471,2.72534141341218,29.7560303583132));
#65083=CARTESIAN_POINT('Ctrl Pts',(7.50509960111561,2.48413770085651,29.7452054158744));
#65084=CARTESIAN_POINT('Ctrl Pts',(7.58056929512689,2.23871832786616,29.7344692242652));
#65085=CARTESIAN_POINT('Ctrl Pts',(7.64420956899104,1.99032320316301,29.7239209040971));
#65086=CARTESIAN_POINT('Ctrl Pts',(7.66729558128016,1.9002159086266,29.7200944175934));
#65087=CARTESIAN_POINT('Ctrl Pts',(7.68882471931851,1.80971747965483,29.7162926537119));
#65088=CARTESIAN_POINT('Ctrl Pts',(7.70878252342339,1.71888871380841,29.7125203441244));
#65089=CARTESIAN_POINT('Ctrl Pts',(7.75911040891409,1.48984449116967,29.7030076560574));
#65090=CARTESIAN_POINT('Ctrl Pts',(7.79971784227922,1.25872499840184,29.6935267004336));
#65091=CARTESIAN_POINT('Ctrl Pts',(7.83045312881348,1.026338145523,29.6841043965909));
#65092=CARTESIAN_POINT('Ctrl Pts',(7.86091227707832,0.796039150303125,29.6747667465443));
#65093=CARTESIAN_POINT('Ctrl Pts',(7.88167563920507,0.564494664909313,29.6654866991103));
#65094=CARTESIAN_POINT('Ctrl Pts',(7.8925465890629,0.33250349080512,29.6562904545633));
#65095=CARTESIAN_POINT('Ctrl Pts',(7.90327280642752,0.10360097606082,29.6472166459965));
#65096=CARTESIAN_POINT('Ctrl Pts',(7.90436801653756,-0.125737091559307,
29.6382244237192));
#65097=CARTESIAN_POINT('Ctrl Pts',(7.89559906329219,-0.354720295755568,
29.629338955409));
#65098=CARTESIAN_POINT('Ctrl Pts',(7.88705954372156,-0.57771231075014,29.6206859693107));
#65099=CARTESIAN_POINT('Ctrl Pts',(7.86916497631032,-0.800368274466062,
29.6121342239709));
#65100=CARTESIAN_POINT('Ctrl Pts',(7.84166199009046,-1.02192777059955,29.6037069628183));
#65101=CARTESIAN_POINT('Ctrl Pts',(7.81942455580808,-1.20106885351757,29.5968931330558));
#65102=CARTESIAN_POINT('Ctrl Pts',(7.79090490783725,-1.37949267680095,29.5901606844468));
#65103=CARTESIAN_POINT('Ctrl Pts',(7.75595211371944,-1.55677895632439,29.5835219031088));
#65104=CARTESIAN_POINT('Ctrl Pts',(7.70384921105463,-1.82105338699455,29.5736257049194));
#65105=CARTESIAN_POINT('Ctrl Pts',(7.63855814103414,-2.08232461837313,29.5633880391846));
#65106=CARTESIAN_POINT('Ctrl Pts',(7.55971905996207,-2.33919985628434,29.552885756511));
#65107=CARTESIAN_POINT('Ctrl Pts',(7.52069221803405,-2.46635797594862,29.5476869271968));
#65108=CARTESIAN_POINT('Ctrl Pts',(7.47834551663021,-2.59243806069412,29.5424232551434));
#65109=CARTESIAN_POINT('Ctrl Pts',(7.43263583996337,-2.71726648701272,29.5371040624316));
#65110=CARTESIAN_POINT('Ctrl Pts',(7.33891971869409,-2.97319557668874,29.5261984042521));
#65111=CARTESIAN_POINT('Ctrl Pts',(7.23106599937438,-3.22386638812884,29.5150593643078));
#65112=CARTESIAN_POINT('Ctrl Pts',(7.11010579502649,-3.46826954382605,29.5037672825078));
#65113=CARTESIAN_POINT('Ctrl Pts',(6.98844648158592,-3.71408526714707,29.492409936292));
#65114=CARTESIAN_POINT('Ctrl Pts',(6.85352793073787,-3.95356014371426,29.480897774048));
#65115=CARTESIAN_POINT('Ctrl Pts',(6.70642559643767,-4.18562160434378,29.4693125367638));
#65116=CARTESIAN_POINT('Ctrl Pts',(6.55852595528369,-4.41894085733898,29.4576645065327));
#65117=CARTESIAN_POINT('Ctrl Pts',(6.39830942902776,-4.64476540451055,29.4459426069692));
#65118=CARTESIAN_POINT('Ctrl Pts',(6.22690683037516,-4.86196855604495,29.4342299154074));
#65119=CARTESIAN_POINT('Ctrl Pts',(6.05573084914591,-5.07888453562902,29.4225327096085));
#65120=CARTESIAN_POINT('Ctrl Pts',(5.87339790505756,-5.28720100457781,29.410844687479));
#65121=CARTESIAN_POINT('Ctrl Pts',(5.68108025345432,-5.48577147790493,29.3992485972701));
#65122=CARTESIAN_POINT('Ctrl Pts',(5.49060621566564,-5.6824383960215,29.3877636706071));
#65123=CARTESIAN_POINT('Ctrl Pts',(5.29033779390495,-5.86954426748541,29.37636892174));
#65124=CARTESIAN_POINT('Ctrl Pts',(5.0814635797187,-6.04596572059475,29.3651447419124));
#65125=CARTESIAN_POINT('Ctrl Pts',(4.93417895129952,-6.17036675433466,29.3572301739909));
#65126=CARTESIAN_POINT('Ctrl Pts',(4.78261643501547,-6.28945508417574,29.3494004157432));
#65127=CARTESIAN_POINT('Ctrl Pts',(4.62720834647535,-6.4028382635155,29.3416836527204));
#65128=CARTESIAN_POINT('Ctrl Pts',(4.49779169203943,-6.49725852102785,29.3352574900742));
#65129=CARTESIAN_POINT('Ctrl Pts',(4.36561329795816,-6.58795204972318,29.328827803173));
#65130=CARTESIAN_POINT('Ctrl Pts',(4.23071911293456,-6.67459997598174,29.3224932309414));
#65131=CARTESIAN_POINT('Ctrl Pts',(4.17061489451043,-6.7132073176172,29.3196707629977));
#65132=CARTESIAN_POINT('Ctrl Pts',(4.10997185339344,-6.75101089244237,29.3168671780523));
#65133=CARTESIAN_POINT('Ctrl Pts',(4.04879584613982,-6.78797967381976,29.3140912014682));
#65134=CARTESIAN_POINT('Ctrl Pts',(3.85886069759447,-6.90275785725601,29.3054725362673));
#65135=CARTESIAN_POINT('Ctrl Pts',(3.66390030777603,-7.00972981581459,29.2969636370112));
#65136=CARTESIAN_POINT('Ctrl Pts',(3.46469529601492,-7.10828847885071,29.2885038963771));
#65137=CARTESIAN_POINT('Ctrl Pts',(3.26624601390199,-7.20647323711867,29.2800762496986));
#65138=CARTESIAN_POINT('Ctrl Pts',(3.06358500976317,-7.29630844349399,29.2716973893607));
#65139=CARTESIAN_POINT('Ctrl Pts',(2.85748136980523,-7.377245344131,29.2633073952103));
#65140=CARTESIAN_POINT('Ctrl Pts',(2.65321619915542,-7.45746027785976,29.2549922408188));
#65141=CARTESIAN_POINT('Ctrl Pts',(2.44557017836928,-7.52893509243917,29.2466661503588));
#65142=CARTESIAN_POINT('Ctrl Pts',(2.23527897503751,-7.59118481739772,29.2382707929012));
#65143=CARTESIAN_POINT('Ctrl Pts',(2.07251993239705,-7.63936422518255,29.2317730396867));
#65144=CARTESIAN_POINT('Ctrl Pts',(1.90817615877255,-7.68201854366409,29.2252337935135));
#65145=CARTESIAN_POINT('Ctrl Pts',(1.74257982759338,-7.71894247785003,29.2186260103798));
#65146=CARTESIAN_POINT('Ctrl Pts',(1.52726421289925,-7.76695259697258,29.2100342808586));
#65147=CARTESIAN_POINT('Ctrl Pts',(1.30983244520213,-7.80527365789384,29.2013266804133));
#65148=CARTESIAN_POINT('Ctrl Pts',(1.09115861770332,-7.83424991552118,29.192443759928));
#65149=CARTESIAN_POINT('Ctrl Pts',(0.872125635103007,-7.86327376444405,
29.1835462499225));
#65150=CARTESIAN_POINT('Ctrl Pts',(0.651847066314613,-7.88292277445575,
29.1744728435044));
#65151=CARTESIAN_POINT('Ctrl Pts',(0.4311625345861,-7.89357782348103,29.1651637981544));
#65152=CARTESIAN_POINT('Ctrl Pts',(0.211743315076415,-7.90417178093991,
29.1559081269524));
#65153=CARTESIAN_POINT('Ctrl Pts',(-0.00807683931881509,-7.90587528930512,
29.146419511181));
#65154=CARTESIAN_POINT('Ctrl Pts',(-0.227517940637586,-7.89908699077107,
29.1366392300558));
#65155=CARTESIAN_POINT('Ctrl Pts',(-0.268085759595382,-7.89783204598495,
29.1348311609582));
#65156=CARTESIAN_POINT('Ctrl Pts',(-0.308640757788562,-7.89628693235663,
29.1330131237645));
#65157=CARTESIAN_POINT('Ctrl Pts',(-0.34917819275588,-7.89445423238116,
29.1311847474671));
#65158=CARTESIAN_POINT('Ctrl Pts',(-0.538828059795782,-7.88588015000639,
29.1226308929378));
#65159=CARTESIAN_POINT('Ctrl Pts',(-0.728031810797408,-7.87015139420761,
29.1143509327306));
#65160=CARTESIAN_POINT('Ctrl Pts',(-0.916358502593095,-7.84757804624816,
29.1062655195673));
#65161=CARTESIAN_POINT('Ctrl Pts',(-1.10611378864828,-7.8248334631069,29.0981187726934));
#65162=CARTESIAN_POINT('Ctrl Pts',(-1.29497906805076,-7.79514041704204,
29.0901695356186));
#65163=CARTESIAN_POINT('Ctrl Pts',(-1.48255483525554,-7.75878252323287,
29.082336641613));
#65164=CARTESIAN_POINT('Ctrl Pts',(-1.67162478348115,-7.72213501165647,
29.074441352759));
#65165=CARTESIAN_POINT('Ctrl Pts',(-1.85938507411905,-7.67871641847901,
29.0666642678754));
#65166=CARTESIAN_POINT('Ctrl Pts',(-2.04546167796984,-7.62877763964518,
29.0589222650794));
#65167=CARTESIAN_POINT('Ctrl Pts',(-2.13475364070083,-7.60481368347776,
29.0552071358756));
#65168=CARTESIAN_POINT('Ctrl Pts',(-2.22365836859117,-7.57934769442297,
29.0515000850955));
#65169=CARTESIAN_POINT('Ctrl Pts',(-2.31213684239565,-7.55240382264388,
29.0477919277812));
#65170=CARTESIAN_POINT('Ctrl Pts',(-2.52253784614527,-7.48833154129159,
29.0389739635077));
#65171=CARTESIAN_POINT('Ctrl Pts',(-2.7306355300909,-7.41541124061954,29.0303909052055));
#65172=CARTESIAN_POINT('Ctrl Pts',(-2.93552934277737,-7.33397728379057,
29.0219582481968));
#65173=CARTESIAN_POINT('Ctrl Pts',(-3.14073584780823,-7.25241904905129,
29.0135127219499));
#65174=CARTESIAN_POINT('Ctrl Pts',(-3.34272841978637,-7.16232190482128,
29.0052180564073));
#65175=CARTESIAN_POINT('Ctrl Pts',(-3.54065085396848,-7.0640410666409,28.9969893594079));
#65176=CARTESIAN_POINT('Ctrl Pts',(-3.73824838897254,-6.9659215611749,28.9887741702097));
#65177=CARTESIAN_POINT('Ctrl Pts',(-3.93178901997251,-6.85964594418846,
28.9806247331514));
#65178=CARTESIAN_POINT('Ctrl Pts',(-4.12047194257944,-6.74557574391328,
28.9724565734496));
#65179=CARTESIAN_POINT('Ctrl Pts',(-4.30869741496518,-6.63178209987131,
28.9643082169521));
#65180=CARTESIAN_POINT('Ctrl Pts',(-4.49208872615072,-6.51023231954899,
28.9561412284849));
#65181=CARTESIAN_POINT('Ctrl Pts',(-4.66990257513552,-6.38128259761895,
28.947871746188));
#65182=CARTESIAN_POINT('Ctrl Pts',(-4.84722625193836,-6.25268834612568,
28.9396250600356));
#65183=CARTESIAN_POINT('Ctrl Pts',(-5.01900332658137,-6.11673554487985,
28.9312764443558));
#65184=CARTESIAN_POINT('Ctrl Pts',(-5.18454679116245,-5.97376467352253,
28.9227427289143));
#65185=CARTESIAN_POINT('Ctrl Pts',(-5.30722346042526,-5.86781551784852,
28.9164187837833));
#65186=CARTESIAN_POINT('Ctrl Pts',(-5.42647794164635,-5.75801208869698,
28.9099931890388));
#65187=CARTESIAN_POINT('Ctrl Pts',(-5.54204749344127,-5.64448530799503,
28.9034320978716));
#65188=CARTESIAN_POINT('Ctrl Pts',(-5.7020121852652,-5.4873481018131,28.8943506148142));
#65189=CARTESIAN_POINT('Ctrl Pts',(-5.85491566406144,-5.3230794649538,28.8850095409915));
#65190=CARTESIAN_POINT('Ctrl Pts',(-6.00067576598747,-5.15259419213927,
28.8753191211564));
#65191=CARTESIAN_POINT('Ctrl Pts',(-6.14643586791348,-4.98210891932477,
28.8656287013213));
#65192=CARTESIAN_POINT('Ctrl Pts',(-6.28505318089336,-4.80540767793714,
28.8555889354738));
#65193=CARTESIAN_POINT('Ctrl Pts',(-6.41648389579647,-4.62336032226345,
28.8451100683667));
#65194=CARTESIAN_POINT('Ctrl Pts',(-6.53962515289976,-4.45279486314295,
28.8352921131838));
#65195=CARTESIAN_POINT('Ctrl Pts',(-6.65528280494462,-4.27697500599435,
28.8258401557342));
#65196=CARTESIAN_POINT('Ctrl Pts',(-6.7633938673275,-4.09665303851573,28.8166951548517));
#65197=CARTESIAN_POINT('Ctrl Pts',(-6.87365135597915,-3.91275097664805,
28.8073685900322));
#65198=CARTESIAN_POINT('Ctrl Pts',(-6.97606016824697,-3.72416611941421,
28.7983612913453));
#65199=CARTESIAN_POINT('Ctrl Pts',(-7.07054837617649,-3.53164260475705,
28.7896106307524));
#65200=CARTESIAN_POINT('Ctrl Pts',(-7.09892101577191,-3.47383221323089,
28.7869830082726));
#65201=CARTESIAN_POINT('Ctrl Pts',(-7.12657941808578,-3.41566633441897,
28.7843785259008));
#65202=CARTESIAN_POINT('Ctrl Pts',(-7.15352143167685,-3.3571642301761,28.7817954879908));
#65203=CARTESIAN_POINT('Ctrl Pts',(-7.25230039082061,-3.14267480661102,
28.7723251566322));
#65204=CARTESIAN_POINT('Ctrl Pts',(-7.3418497446533,-2.92397966063852,28.762864035899));
#65205=CARTESIAN_POINT('Ctrl Pts',(-7.42196251902932,-2.70188901454886,
28.7534152726674));
#65206=CARTESIAN_POINT('Ctrl Pts',(-7.5024061150049,-2.47888125650843,28.7439274912519));
#65207=CARTESIAN_POINT('Ctrl Pts',(-7.57333523304903,-2.25244906459848,
28.734452169608));
#65208=CARTESIAN_POINT('Ctrl Pts',(-7.63449089954376,-2.02339652599593,
28.7249924937579));
#65209=CARTESIAN_POINT('Ctrl Pts',(-7.69505982794055,-1.79654155727583,
28.7156235756826));
#65210=CARTESIAN_POINT('Ctrl Pts',(-7.74604202587532,-1.56711546990253,
28.7062700046243));
#65211=CARTESIAN_POINT('Ctrl Pts',(-7.78713558864553,-1.33589585848278,
28.6969348757802));
#65212=CARTESIAN_POINT('Ctrl Pts',(-7.8270789797213,-1.11114787508277,28.6878610287582));
#65213=CARTESIAN_POINT('Ctrl Pts',(-7.85767946192405,-0.884704685624519,
28.678804606036));
#65214=CARTESIAN_POINT('Ctrl Pts',(-7.87861219250326,-0.657287840938538,
28.6697684501219));
#65215=CARTESIAN_POINT('Ctrl Pts',(-7.89871791238911,-0.438855785011747,
28.661089294817));
#65216=CARTESIAN_POINT('Ctrl Pts',(-7.90990453771594,-0.219525002565944,
28.6524288365514));
#65217=CARTESIAN_POINT('Ctrl Pts',(-7.91184153648199,4.99451412436924E-5,
28.6437895940631));
#65218=CARTESIAN_POINT('',(-7.91808516897138,-0.00159779970073705,26.6422647402301));
#65219=CARTESIAN_POINT('Ctrl Pts',(-7.911,-5.4678483962789E-13,28.642331508237));
#65220=CARTESIAN_POINT('Ctrl Pts',(-7.91100000000015,2.20167589666618,28.5537440725043));
#65221=CARTESIAN_POINT('Ctrl Pts',(-6.94214576672406,4.38610418338626,28.4651566367716));
#65222=CARTESIAN_POINT('Ctrl Pts',(-3.67820201488353,7.34180684107597,28.2879817653062));
#65223=CARTESIAN_POINT('Ctrl Pts',(-1.40868175871823,8.08992666571321,28.1993943295734));
#65224=CARTESIAN_POINT('Ctrl Pts',(2.9730927052119,7.65454228025288,28.022219458108));
#65225=CARTESIAN_POINT('Ctrl Pts',(5.05102072675527,6.47444880834283,27.9336320223753));
#65226=CARTESIAN_POINT('Ctrl Pts',(7.66951518847833,2.93425195367804,27.7564571509098));
#65227=CARTESIAN_POINT('Ctrl Pts',(8.18956872247062,0.601881960100259,27.6678697151771));
#65228=CARTESIAN_POINT('Ctrl Pts',(7.32306689761395,-3.71537198232343,27.4906948437116));
#65229=CARTESIAN_POINT('Ctrl Pts',(5.94329958850286,-5.6664351893642,27.4021074079789));
#65230=CARTESIAN_POINT('Ctrl Pts',(2.16154501637976,-7.92205913232961,27.2249325365135));
#65231=CARTESIAN_POINT('Ctrl Pts',(-0.210816529298981,-8.20894963713005,
27.1363451007807));
#65232=CARTESIAN_POINT('Ctrl Pts',(-4.42123908576312,-6.9198224471791,26.9591702293153));
#65233=CARTESIAN_POINT('Ctrl Pts',(-6.22631625634087,-5.35390358803636,
26.8705827935826));
#65234=CARTESIAN_POINT('Ctrl Pts',(-7.6529404869374,-2.3138436401746,26.7354627452239));
#65235=CARTESIAN_POINT('Ctrl Pts',(-7.9107562251631,-1.15812141717204,26.6889301325979));
#65236=CARTESIAN_POINT('Ctrl Pts',(-7.9109998272103,-0.00164059837198713,
26.642397519972));
#65237=CARTESIAN_POINT('',(-7.90279014835528,-0.00473842408097357,24.6423332821822));
#65238=CARTESIAN_POINT('Ctrl Pts',(-7.92184818564761,-0.00157506937677171,
26.6421942210654));
#65239=CARTESIAN_POINT('Ctrl Pts',(-7.90527866078965,2.38817114548611,26.5457221946099));
#65240=CARTESIAN_POINT('Ctrl Pts',(-5.47644787019391,7.43173693689856,26.3433157883521));
#65241=CARTESIAN_POINT('Ctrl Pts',(1.61672921772412,8.57512333172727,26.0879421921928));
#65242=CARTESIAN_POINT('Ctrl Pts',(6.10409558131502,5.51035650884788,25.8760734325877));
#65243=CARTESIAN_POINT('Ctrl Pts',(8.69528679823428,0.733853537314583,25.6642046729827));
#65244=CARTESIAN_POINT('Ctrl Pts',(6.76558824356892,-6.46288284829038,25.3993687234762));
#65245=CARTESIAN_POINT('Ctrl Pts',(-1.77924551132568,-9.18489542958251,
25.0815655840685));
#65246=CARTESIAN_POINT('Ctrl Pts',(-7.25618309704257,-4.65554030243547,
24.8292205841656));
#65247=CARTESIAN_POINT('Ctrl Pts',(-7.90576535995413,-1.01347673874075,
24.6828099640653));
#65248=CARTESIAN_POINT('Ctrl Pts',(-7.90074683040818,-0.00474821529727623,
24.6423337237675));
#65249=CARTESIAN_POINT('',(-7.90432432633472,0.00627944674389112,22.6423294472501));
#65250=CARTESIAN_POINT('Ctrl Pts',(-7.91099860438285,-0.00469909061914475,
24.642331508237));
#65251=CARTESIAN_POINT('Ctrl Pts',(-7.91111988382393,0.199476901486499,
24.6341493331127));
#65252=CARTESIAN_POINT('Ctrl Pts',(-7.90333194721171,0.403663036123113,
24.6259671579884));
#65253=CARTESIAN_POINT('Ctrl Pts',(-7.88766198850874,0.60721442261722,24.617784982864));
#65254=CARTESIAN_POINT('Ctrl Pts',(-7.87238375930625,0.805677277324782,
24.6098073519529));
#65255=CARTESIAN_POINT('Ctrl Pts',(-7.84961292323444,1.00353639927101,24.6018297210419));
#65256=CARTESIAN_POINT('Ctrl Pts',(-7.81942730419529,1.20019899783543,24.5938520901308));
#65257=CARTESIAN_POINT('Ctrl Pts',(-7.78923239663649,1.39692211211797,24.5858720043957));
#65258=CARTESIAN_POINT('Ctrl Pts',(-7.75161820732367,1.592447639378,24.5778919186606));
#65259=CARTESIAN_POINT('Ctrl Pts',(-7.70671387622014,1.78619210335169,24.5699118329255));
#65260=CARTESIAN_POINT('Ctrl Pts',(-7.66178892353793,1.98002554129762,24.5619280824668));
#65261=CARTESIAN_POINT('Ctrl Pts',(-7.6095672292207,2.17207596064996,24.553944332008));
#65262=CARTESIAN_POINT('Ctrl Pts',(-7.55022817545046,2.36177380344395,24.5459605815493));
#65263=CARTESIAN_POINT('Ctrl Pts',(-7.48829006397143,2.55978043462141,24.5376271418579));
#65264=CARTESIAN_POINT('Ctrl Pts',(-7.41859721950583,2.75522337689826,24.5292937021666));
#65265=CARTESIAN_POINT('Ctrl Pts',(-7.34140975810823,2.94747752553829,24.5209602624752));
#65266=CARTESIAN_POINT('Ctrl Pts',(-7.26731873141991,3.13201925031989,24.5129611251621));
#65267=CARTESIAN_POINT('Ctrl Pts',(-7.18632283809609,3.31362275397686,24.5049619878489));
#65268=CARTESIAN_POINT('Ctrl Pts',(-7.09869945867559,3.49175987080997,24.4969628505357));
#65269=CARTESIAN_POINT('Ctrl Pts',(-7.01100849759306,3.67003438022603,24.4889575436933));
#65270=CARTESIAN_POINT('Ctrl Pts',(-6.91668001319148,3.84483687849186,24.4809522368509));
#65271=CARTESIAN_POINT('Ctrl Pts',(-6.81603576199685,4.01566650646939,24.4729469300086));
#65272=CARTESIAN_POINT('Ctrl Pts',(-6.71525529087635,4.18672734883804,24.4649307881479));
#65273=CARTESIAN_POINT('Ctrl Pts',(-6.60814215854351,4.3538043018684,24.4569146462873));
#65274=CARTESIAN_POINT('Ctrl Pts',(-6.49506023788673,4.51642707305485,24.4488985044266));
#65275=CARTESIAN_POINT('Ctrl Pts',(-6.48123936272855,4.53630283219823,24.4479187713688));
#65276=CARTESIAN_POINT('Ctrl Pts',(-6.46732937497621,4.55611209863451,24.446939038311));
#65277=CARTESIAN_POINT('Ctrl Pts',(-6.45333097816966,4.5758540499229,24.4459593052532));
#65278=CARTESIAN_POINT('Ctrl Pts',(-6.34130840660208,4.7338395808127,24.438118963384));
#65279=CARTESIAN_POINT('Ctrl Pts',(-6.22331232814448,4.88794656333586,24.4302786215148));
#65280=CARTESIAN_POINT('Ctrl Pts',(-6.09964126902208,5.03768770263131,24.4224382796456));
#65281=CARTESIAN_POINT('Ctrl Pts',(-5.97610847782461,5.18726142687627,24.414606703512));
#65282=CARTESIAN_POINT('Ctrl Pts',(-5.84691356140695,5.33247875908419,24.4067751273783));
#65283=CARTESIAN_POINT('Ctrl Pts',(-5.71239872668933,5.47288057491831,24.3989435512447));
#65284=CARTESIAN_POINT('Ctrl Pts',(-5.57800812805659,5.61315271753127,24.391119208249));
#65285=CARTESIAN_POINT('Ctrl Pts',(-5.43830763749175,5.74861794886992,24.3832948652533));
#65286=CARTESIAN_POINT('Ctrl Pts',(-5.29368031332814,5.87884935512742,24.3754705222576));
#65287=CARTESIAN_POINT('Ctrl Pts',(-5.14915845798907,6.00898579071866,24.3676518851288));
#65288=CARTESIAN_POINT('Ctrl Pts',(-4.99971718517095,6.13389576897055,24.359833248));
#65289=CARTESIAN_POINT('Ctrl Pts',(-4.84577719711519,6.25318833523495,24.3520146108712));
#65290=CARTESIAN_POINT('Ctrl Pts',(-4.69191956297701,6.37241708305754,24.3442001565113));
#65291=CARTESIAN_POINT('Ctrl Pts',(-4.5335682850339,6.48603419050078,24.3363857021514));
#65292=CARTESIAN_POINT('Ctrl Pts',(-4.3711781539614,6.59368808379124,24.3285712477916));
#65293=CARTESIAN_POINT('Ctrl Pts',(-4.20884335727195,6.70130529405344,24.3207594562044));
#65294=CARTESIAN_POINT('Ctrl Pts',(-4.04247274225547,6.80296314473486,24.3129476646172));
#65295=CARTESIAN_POINT('Ctrl Pts',(-3.87255131813304,6.89835250537591,24.3051358730301));
#65296=CARTESIAN_POINT('Ctrl Pts',(-3.70262194141433,6.99374633039264,24.2973237158385));
#65297=CARTESIAN_POINT('Ctrl Pts',(-3.5291417257168,7.08287089914626,24.2895115586469));
#65298=CARTESIAN_POINT('Ctrl Pts',(-3.35262204987139,7.16546205005066,24.2816994014553));
#65299=CARTESIAN_POINT('Ctrl Pts',(-3.17608794338219,7.24805995285664,24.2738866056127));
#65300=CARTESIAN_POINT('Ctrl Pts',(-2.99651420014128,7.32412322397701,24.2660738097702));
#65301=CARTESIAN_POINT('Ctrl Pts',(-2.81443395397274,7.39343509599735,24.2582610139277));
#65302=CARTESIAN_POINT('Ctrl Pts',(-2.6323067839967,7.46276483034493,24.2504462046535));
#65303=CARTESIAN_POINT('Ctrl Pts',(-2.44767215300058,7.52533957430112,24.2426313953793));
#65304=CARTESIAN_POINT('Ctrl Pts',(-2.26108033499531,7.58099180310186,24.2348165861052));
#65305=CARTESIAN_POINT('Ctrl Pts',(-2.07440759527138,7.63666816733388,24.2269983876803));
#65306=CARTESIAN_POINT('Ctrl Pts',(-1.88577631439626,7.68541593548877,24.2191801892554));
#65307=CARTESIAN_POINT('Ctrl Pts',(-1.69574913354654,7.72711821289646,24.2113619908304));
#65308=CARTESIAN_POINT('Ctrl Pts',(-1.50550076208681,7.76886903152934,24.2035346920649));
#65309=CARTESIAN_POINT('Ctrl Pts',(-1.31385358901552,7.80355790455573,24.1957073932993));
#65310=CARTESIAN_POINT('Ctrl Pts',(-1.12137868713031,7.83111938614461,24.1878800945338));
#65311=CARTESIAN_POINT('Ctrl Pts',(-0.92877813684542,7.8586988599809,24.1800476860757));
#65312=CARTESIAN_POINT('Ctrl Pts',(-0.73534912940628,7.87914163335445,24.1722152776176));
#65313=CARTESIAN_POINT('Ctrl Pts',(-0.541665045788452,7.8924343505772,24.1643828691595));
#65314=CARTESIAN_POINT('Ctrl Pts',(-0.347702998217335,7.90574614472233,
24.1565392200916));
#65315=CARTESIAN_POINT('Ctrl Pts',(-0.15348549339493,7.91188737686632,24.1486955710237));
#65316=CARTESIAN_POINT('Ctrl Pts',(0.040415717483983,7.91089676141588,24.1408519219558));
#65317=CARTESIAN_POINT('Ctrl Pts',(0.1450320961399,7.91036229027671,24.1366200032524));
#65318=CARTESIAN_POINT('Ctrl Pts',(0.249556504707496,7.90775265085662,24.1323880845489));
#65319=CARTESIAN_POINT('Ctrl Pts',(0.353900185828802,7.90308013741923,24.1281561658455));
#65320=CARTESIAN_POINT('Ctrl Pts',(0.549123101975789,7.89433804887892,24.1202384126927));
#65321=CARTESIAN_POINT('Ctrl Pts',(0.744296330346685,7.87834574622237,24.1123206595398));
#65322=CARTESIAN_POINT('Ctrl Pts',(0.938839588114405,7.85509396683383,24.104402906387));
#65323=CARTESIAN_POINT('Ctrl Pts',(1.13315932967706,7.83186890206675,24.0964942501628));
#65324=CARTESIAN_POINT('Ctrl Pts',(1.32685020368346,7.80140101411378,24.0885855939386));
#65325=CARTESIAN_POINT('Ctrl Pts',(1.51933232660837,7.76373301198095,24.0806769377144));
#65326=CARTESIAN_POINT('Ctrl Pts',(1.71162893255038,7.72610131479947,24.0727759039646));
#65327=CARTESIAN_POINT('Ctrl Pts',(1.90271877253867,7.68128339320356,24.0648748702147));
#65328=CARTESIAN_POINT('Ctrl Pts',(2.09202719526749,7.62937371048642,24.0569738364649));
#65329=CARTESIAN_POINT('Ctrl Pts',(2.28118819123502,7.57750445320989,24.049078955763));
#65330=CARTESIAN_POINT('Ctrl Pts',(2.46857020327513,7.51855452867736,24.0411840750612));
#65331=CARTESIAN_POINT('Ctrl Pts',(2.65360860351722,7.45266948008158,24.0332891943594));
#65332=CARTESIAN_POINT('Ctrl Pts',(2.83853713485194,7.38682355157272,24.0253990013435));
#65333=CARTESIAN_POINT('Ctrl Pts',(3.02112450363762,7.31405081939341,24.0175088083277));
#65334=CARTESIAN_POINT('Ctrl Pts',(3.2008208115859,7.23454678138987,24.0096186153118));
#65335=CARTESIAN_POINT('Ctrl Pts',(3.38044366061104,7.15507524422669,24.0017316477662));
#65336=CARTESIAN_POINT('Ctrl Pts',(3.55717748969029,7.06887802450121,23.9938446802205));
#65337=CARTESIAN_POINT('Ctrl Pts',(3.73049170866777,6.9761990088845,23.9859577126748));
#65338=CARTESIAN_POINT('Ctrl Pts',(3.90379087648731,6.88352804180823,23.9780714300585));
#65339=CARTESIAN_POINT('Ctrl Pts',(4.07367071921496,6.78437655700258,23.9701851474422));
#65340=CARTESIAN_POINT('Ctrl Pts',(4.23962415783559,6.67903496025413,23.9622988648259));
#65341=CARTESIAN_POINT('Ctrl Pts',(4.40557730476928,6.57369354865862,23.9544125960708));
#65342=CARTESIAN_POINT('Ctrl Pts',(4.56760377012997,6.46216223100105,23.9465263273158));
#65343=CARTESIAN_POINT('Ctrl Pts',(4.72522435664793,6.34477547115271,23.9386400585607));
#65344=CARTESIAN_POINT('Ctrl Pts',(4.88287108415609,6.2273692429963,23.9307524818872));
#65345=CARTESIAN_POINT('Ctrl Pts',(5.03611020051353,6.10410584347305,23.9228649052137));
#65346=CARTESIAN_POINT('Ctrl Pts',(5.18449437880163,5.97536099630594,23.9149773285402));
#65347=CARTESIAN_POINT('Ctrl Pts',(5.33292803630578,5.84657321872548,23.9070871217271));
#65348=CARTESIAN_POINT('Ctrl Pts',(5.47650327003698,5.7123005772867,23.8991969149139));
#65349=CARTESIAN_POINT('Ctrl Pts',(5.61480832495223,5.57295688786906,23.8913067081008));
#65350=CARTESIAN_POINT('Ctrl Pts',(5.75324693570809,5.43347863964165,23.8834088820202));
#65351=CARTESIAN_POINT('Ctrl Pts',(5.88640495959489,5.28891980691886,23.8755110559396));
#65352=CARTESIAN_POINT('Ctrl Pts',(6.0139090833572,5.13972942255852,23.867613229859));
#65353=CARTESIAN_POINT('Ctrl Pts',(6.14148380856284,4.99045642866246,23.8597110306028));
#65354=CARTESIAN_POINT('Ctrl Pts',(6.26339817817814,4.83654703931126,23.8518088313466));
#65355=CARTESIAN_POINT('Ctrl Pts',(6.37932104863958,4.67848094560446,23.8439066320904));
#65356=CARTESIAN_POINT('Ctrl Pts',(6.49538384679467,4.52022405413836,23.8359948942806));
#65357=CARTESIAN_POINT('Ctrl Pts',(6.60544050707392,4.35780072065255,23.8280831564708));
#65358=CARTESIAN_POINT('Ctrl Pts',(6.70920426454532,4.19171792187963,23.820171418661));
#65359=CARTESIAN_POINT('Ctrl Pts',(6.75212754696815,4.12301552471299,23.8168986212532));
#65360=CARTESIAN_POINT('Ctrl Pts',(6.79397455576169,4.05368720450044,23.8136258238455));
#65361=CARTESIAN_POINT('Ctrl Pts',(6.83472736305399,3.98376993220254,23.8103530264378));
#65362=CARTESIAN_POINT('Ctrl Pts',(6.93826378547244,3.80613838434233,23.8020381701762));
#65363=CARTESIAN_POINT('Ctrl Pts',(7.03496030254178,3.6243162306715,23.7937233139146));
#65364=CARTESIAN_POINT('Ctrl Pts',(7.12448314941557,3.43884586070582,23.7854084576529));
#65365=CARTESIAN_POINT('Ctrl Pts',(7.21389575201512,3.25360389105408,23.7771038408477));
#65366=CARTESIAN_POINT('Ctrl Pts',(7.2961521767793,3.06472292830131,23.7687992240426));
#65367=CARTESIAN_POINT('Ctrl Pts',(7.37096373096742,2.87277125381797,23.7604946072374));
#65368=CARTESIAN_POINT('Ctrl Pts',(7.44568809197913,2.68104329980665,23.7521996694975));
#65369=CARTESIAN_POINT('Ctrl Pts',(7.51298478295705,2.48625204459096,23.7439047317576));
#65370=CARTESIAN_POINT('Ctrl Pts',(7.57261219626893,2.28898788221323,23.7356097940178));
#65371=CARTESIAN_POINT('Ctrl Pts',(7.63215023917516,2.09201938213637,23.7273272888472));
#65372=CARTESIAN_POINT('Ctrl Pts',(7.68404185948036,1.89258565149747,23.7190447836767));
#65373=CARTESIAN_POINT('Ctrl Pts',(7.72809444914455,1.69129452937721,23.7107622785062));
#65374=CARTESIAN_POINT('Ctrl Pts',(7.7721065702309,1.49018832182164,23.7024873819963));
#65375=CARTESIAN_POINT('Ctrl Pts',(7.8082939586741,1.28722841083785,23.6942124854864));
#65376=CARTESIAN_POINT('Ctrl Pts',(7.83651401943129,1.08303694454844,23.6859375889765));
#65377=CARTESIAN_POINT('Ctrl Pts',(7.86470180014006,0.879079046516573,23.677672157863));
#65378=CARTESIAN_POINT('Ctrl Pts',(7.884940398717,0.673892694018034,23.6694067267494));
#65379=CARTESIAN_POINT('Ctrl Pts',(7.89713836537564,0.468109643259195,23.6611412956359));
#65380=CARTESIAN_POINT('Ctrl Pts',(7.90190505893862,0.387694212485036,23.6579113493353));
#65381=CARTESIAN_POINT('Ctrl Pts',(7.90544444214007,0.307187765194219,23.6546814030347));
#65382=CARTESIAN_POINT('Ctrl Pts',(7.9077531950713,0.226628342975039,23.651451456734));
#65383=CARTESIAN_POINT('Ctrl Pts',(7.91366210694694,0.0204484091214447,
23.6431848865891));
#65384=CARTESIAN_POINT('Ctrl Pts',(7.91149972666629,-0.185846420877929,
23.6349183164441));
#65385=CARTESIAN_POINT('Ctrl Pts',(7.90130094414447,-0.391617658005469,
23.6266517462991));
#65386=CARTESIAN_POINT('Ctrl Pts',(7.89109302339534,-0.597573268545718,
23.6183777692115));
#65387=CARTESIAN_POINT('Ctrl Pts',(7.8728343396224,-0.803004056335675,23.6101037921239));
#65388=CARTESIAN_POINT('Ctrl Pts',(7.84661163214932,-1.00727696996359,23.6018298150363));
#65389=CARTESIAN_POINT('Ctrl Pts',(7.82036372674066,-1.21174617360933,23.593547887315));
#65390=CARTESIAN_POINT('Ctrl Pts',(7.78613655671095,-1.41505499083991,23.5852659595937));
#65391=CARTESIAN_POINT('Ctrl Pts',(7.74406804962572,-1.61658004527027,23.5769840318724));
#65392=CARTESIAN_POINT('Ctrl Pts',(7.70192980903953,-1.81843915119313,23.5686883758813));
#65393=CARTESIAN_POINT('Ctrl Pts',(7.6519243053614,-2.01850829498922,23.5603927198903));
#65394=CARTESIAN_POINT('Ctrl Pts',(7.59424001638265,-2.21617679203903,23.5520970638992));
#65395=CARTESIAN_POINT('Ctrl Pts',(7.53650359197021,-2.41402394315571,23.5437939102405));
#65396=CARTESIAN_POINT('Ctrl Pts',(7.47107461759645,-2.60946583698416,23.5354907565819));
#65397=CARTESIAN_POINT('Ctrl Pts',(7.39819038259295,-2.80191007402257,23.5271876029232));
#65398=CARTESIAN_POINT('Ctrl Pts',(7.32519502560454,-2.99464771862167,23.5188717899711));
#65399=CARTESIAN_POINT('Ctrl Pts',(7.24472179802206,-3.18437829881425,23.5105559770191));
#65400=CARTESIAN_POINT('Ctrl Pts',(7.15705553730343,-3.37053067571774,23.502240164067));
#65401=CARTESIAN_POINT('Ctrl Pts',(7.12300353068101,-3.44283742085703,23.4990100717214));
#65402=CARTESIAN_POINT('Ctrl Pts',(7.08786675124449,-3.51460457707592,23.4957799793758));
#65403=CARTESIAN_POINT('Ctrl Pts',(7.05166370350665,-3.58579977308366,23.4925498870302));
#65404=CARTESIAN_POINT('Ctrl Pts',(6.96299717529939,-3.76016716062393,23.484638921187));
#65405=CARTESIAN_POINT('Ctrl Pts',(6.86774749850498,-3.93146395442826,23.4767279553439));
#65406=CARTESIAN_POINT('Ctrl Pts',(6.76615185853524,-4.0991596733038,23.4688169895007));
#65407=CARTESIAN_POINT('Ctrl Pts',(6.66465902396409,-4.26668569960961,23.4609140288238));
#65408=CARTESIAN_POINT('Ctrl Pts',(6.55683319458905,-4.43061761729703,23.453011068147));
#65409=CARTESIAN_POINT('Ctrl Pts',(6.44295846077933,-4.59044739351973,23.4451081074701));
#65410=CARTESIAN_POINT('Ctrl Pts',(6.3291778838376,-4.7501450151315,23.4372116813247));
#65411=CARTESIAN_POINT('Ctrl Pts',(6.20935856514258,-4.90574697343133,23.4293152551793));
#65412=CARTESIAN_POINT('Ctrl Pts',(6.08382924630566,-5.05677196458333,23.4214188290338));
#65413=CARTESIAN_POINT('Ctrl Pts',(5.95838049654882,-5.20770002264655,23.4135274710892));
#65414=CARTESIAN_POINT('Ctrl Pts',(5.82722926808575,-5.35405670266394,23.4056361131445));
#65415=CARTESIAN_POINT('Ctrl Pts',(5.69074630437131,-5.4953914782556,23.3977447551998));
#65416=CARTESIAN_POINT('Ctrl Pts',(5.5543256942733,-5.63666168363172,23.3898570025015));
#65417=CARTESIAN_POINT('Ctrl Pts',(5.4125784417489,-5.7729143092266,23.3819692498032));
#65418=CARTESIAN_POINT('Ctrl Pts',(5.2659142710303,-5.90373338576188,23.3740814971049));
#65419=CARTESIAN_POINT('Ctrl Pts',(5.11928998009721,-6.03451689098696,23.3661958891832));
#65420=CARTESIAN_POINT('Ctrl Pts',(4.96775169261106,-6.15986956290902,23.3583102812615));
#65421=CARTESIAN_POINT('Ctrl Pts',(4.81174474820048,-6.2794134660942,23.3504246733398));
#65422=CARTESIAN_POINT('Ctrl Pts',(4.65571940412607,-6.39897146844424,23.3425381353792));
#65423=CARTESIAN_POINT('Ctrl Pts',(4.49522461937134,-6.51271911820504,23.3346515974186));
#65424=CARTESIAN_POINT('Ctrl Pts',(4.33073796624141,-6.62031945360307,23.3267650594579));
#65425=CARTESIAN_POINT('Ctrl Pts',(4.16623059090162,-6.72793334460995,23.3188775279425));
#65426=CARTESIAN_POINT('Ctrl Pts',(3.99773063316515,-6.82939818878412,23.3109899964272));
#65427=CARTESIAN_POINT('Ctrl Pts',(3.82574370650676,-6.92442099327618,23.3031024649118));
#65428=CARTESIAN_POINT('Ctrl Pts',(3.65370628574886,-7.0194716957663,23.295212617675));
#65429=CARTESIAN_POINT('Ctrl Pts',(3.47818015752651,-7.10807642291331,23.2873227704383));
#65430=CARTESIAN_POINT('Ctrl Pts',(3.29969474408242,-7.18998856715884,23.2794329232015));
#65431=CARTESIAN_POINT('Ctrl Pts',(3.12112701174214,-7.27193848993859,23.2715394371043));
#65432=CARTESIAN_POINT('Ctrl Pts',(2.93959758720813,-7.34718953530905,23.2636459510071));
#65433=CARTESIAN_POINT('Ctrl Pts',(2.75565525731032,-7.41554347993847,23.2557524649098));
#65434=CARTESIAN_POINT('Ctrl Pts',(2.57150029033558,-7.4839764416326,23.2478498539537));
#65435=CARTESIAN_POINT('Ctrl Pts',(2.384927169524,-7.54549625696796,23.2399472429976));
#65436=CARTESIAN_POINT('Ctrl Pts',(2.19650032593727,-7.59995442868952,23.2320446320414));
#65437=CARTESIAN_POINT('Ctrl Pts',(2.00794850740072,-7.65444872003793,23.2241367796431));
#65438=CARTESIAN_POINT('Ctrl Pts',(1.81754084822449,-7.7018719475486,23.2162289272447));
#65439=CARTESIAN_POINT('Ctrl Pts',(1.62585157652943,-7.74212681703786,23.2083210748464));
#65440=CARTESIAN_POINT('Ctrl Pts',(1.43390001954144,-7.78243676660616,23.2004024022631));
#65441=CARTESIAN_POINT('Ctrl Pts',(1.24066368569655,-7.8155587091444,23.1924837296797));
#65442=CARTESIAN_POINT('Ctrl Pts',(1.04672269370989,-7.84144709874859,23.1845650570964));
#65443=CARTESIAN_POINT('Ctrl Pts',(0.966567311649314,-7.85214671278274,
23.1812922872718));
#65444=CARTESIAN_POINT('Ctrl Pts',(0.886291575390236,-7.86161134336304,
23.1780195174471));
#65445=CARTESIAN_POINT('Ctrl Pts',(0.805936402846742,-7.86984037414778,
23.1747467476225));
#65446=CARTESIAN_POINT('Ctrl Pts',(0.613366704165532,-7.8895610956458,23.1669036147036));
#65447=CARTESIAN_POINT('Ctrl Pts',(0.419770715722492,-7.90224040504155,
23.1590604817847));
#65448=CARTESIAN_POINT('Ctrl Pts',(0.225710951693573,-7.90777943333561,
23.1512173488658));
#65449=CARTESIAN_POINT('Ctrl Pts',(0.0318790902025709,-7.91331195663048,
23.1433834268718));
#65450=CARTESIAN_POINT('Ctrl Pts',(-0.162415114935045,-7.91172088590572,
23.1355495048777));
#65451=CARTESIAN_POINT('Ctrl Pts',(-0.35660128971044,-7.90295871937699,
23.1277155828836));
#65452=CARTESIAN_POINT('Ctrl Pts',(-0.55059717936082,-7.89420513898966,
23.1198893374341));
#65453=CARTESIAN_POINT('Ctrl Pts',(-0.744484901034405,-7.87829447231448,
23.1120630919846));
#65454=CARTESIAN_POINT('Ctrl Pts',(-0.93769112081678,-7.8552311463089,23.1042368465351));
#65455=CARTESIAN_POINT('Ctrl Pts',(-1.13074556891857,-7.83218593752414,
23.0964167489334));
#65456=CARTESIAN_POINT('Ctrl Pts',(-1.32311923407877,-7.80199930159378,
23.0885966513316));
#65457=CARTESIAN_POINT('Ctrl Pts',(-1.51424075520649,-7.76472767940201,
23.0807765537299));
#65458=CARTESIAN_POINT('Ctrl Pts',(-1.70524927526403,-7.72747809414867,
23.0729610797801));
#65459=CARTESIAN_POINT('Ctrl Pts',(-1.89500678198136,-7.68315193419874,
23.0651456058303));
#65460=CARTESIAN_POINT('Ctrl Pts',(-2.08294880594098,-7.63185726228086,
23.0573301318806));
#65461=CARTESIAN_POINT('Ctrl Pts',(-2.27081621400834,-7.5805829551416,23.0495177607949));
#65462=CARTESIAN_POINT('Ctrl Pts',(-2.45686923670015,-7.52234574061494,
23.0417053897093));
#65463=CARTESIAN_POINT('Ctrl Pts',(-2.64055515475202,-7.45730443757747,
23.0338930186236));
#65464=CARTESIAN_POINT('Ctrl Pts',(-2.82423411963755,-7.392265596585,23.026080943264));
#65465=CARTESIAN_POINT('Ctrl Pts',(-3.00554582402382,-7.3204232890152,23.0182688679044));
#65466=CARTESIAN_POINT('Ctrl Pts',(-3.18395378716133,-7.24198586585344,
23.0104567925449));
#65467=CARTESIAN_POINT('Ctrl Pts',(-3.36236696817639,-7.16354614864123,
23.0026444887064));
#65468=CARTESIAN_POINT('Ctrl Pts',(-3.53787591637705,-7.07851107249217,
22.9948321848679));
#65469=CARTESIAN_POINT('Ctrl Pts',(-3.70996521119385,-6.98713669050001,
22.9870198810295));
#65470=CARTESIAN_POINT('Ctrl Pts',(-3.8820898187468,-6.89574355847783,22.9792059741057));
#65471=CARTESIAN_POINT('Ctrl Pts',(-4.0507930643653,-6.79800869423773,22.9713920671819));
#65472=CARTESIAN_POINT('Ctrl Pts',(-4.21558503163935,-6.69423362611571,
22.9635781602581));
#65473=CARTESIAN_POINT('Ctrl Pts',(-4.38043981196355,-6.59041900249431,
22.9557612749407));
#65474=CARTESIAN_POINT('Ctrl Pts',(-4.54138004686675,-6.48055977616732,
22.9479443896234));
#65475=CARTESIAN_POINT('Ctrl Pts',(-4.69794552818048,-6.36500029962679,
22.9401275043061));
#65476=CARTESIAN_POINT('Ctrl Pts',(-4.8546808499172,-6.24931546550287,22.932302139322));
#65477=CARTESIAN_POINT('Ctrl Pts',(-5.00703165659419,-6.12791823983644,
22.9244767743379));
#65478=CARTESIAN_POINT('Ctrl Pts',(-5.15457070589401,-6.00119336781772,
22.9166514093538));
#65479=CARTESIAN_POINT('Ctrl Pts',(-5.30219942289215,-5.87439147803558,
22.9088212884596));
#65480=CARTESIAN_POINT('Ctrl Pts',(-5.44501029713251,-5.74225572714289,
22.9009911675653));
#65481=CARTESIAN_POINT('Ctrl Pts',(-5.58261354661621,-5.605207131689,22.893161046671));
#65482=CARTESIAN_POINT('Ctrl Pts',(-5.72040489062322,-5.4679711998871,22.8853202225204));
#65483=CARTESIAN_POINT('Ctrl Pts',(-5.85297415308385,-5.32580926684511,
22.8774793983697));
#65484=CARTESIAN_POINT('Ctrl Pts',(-5.97997163617299,-5.17917563233441,
22.8696385742191));
#65485=CARTESIAN_POINT('Ctrl Pts',(-6.04851157106872,-5.10003816032772,
22.8654069188843));
#65486=CARTESIAN_POINT('Ctrl Pts',(-6.11542934495411,-5.01959872920869,
22.8611752635496));
#65487=CARTESIAN_POINT('Ctrl Pts',(-6.18067532756721,-4.93793210718839,
22.8569436082148));
#65488=CARTESIAN_POINT('Ctrl Pts',(-6.30271867379094,-4.78517376978624,
22.849028249193));
#65489=CARTESIAN_POINT('Ctrl Pts',(-6.41926470017325,-4.62767631910825,
22.8411128901711));
#65490=CARTESIAN_POINT('Ctrl Pts',(-6.52992445675855,-4.46587142549207,
22.8331975311492));
#65491=CARTESIAN_POINT('Ctrl Pts',(-6.64110696691312,-4.30330217012168,
22.8252447801945));
#65492=CARTESIAN_POINT('Ctrl Pts',(-6.74634718042822,-4.13638489684024,
22.8172920292398));
#65493=CARTESIAN_POINT('Ctrl Pts',(-6.84528955920018,-3.96559350547998,
22.8093392782852));
#65494=CARTESIAN_POINT('Ctrl Pts',(-6.94352912354301,-3.79601529148324,
22.8014430178676));
#65495=CARTESIAN_POINT('Ctrl Pts',(-7.03555983439679,-3.62261810730013,
22.7935467574501));
#65496=CARTESIAN_POINT('Ctrl Pts',(-7.12107525983665,-3.44589729152545,
22.7856504970326));
#65497=CARTESIAN_POINT('Ctrl Pts',(-7.20652914612961,-3.26930364869278,
22.7777599189715));
#65498=CARTESIAN_POINT('Ctrl Pts',(-7.28547693697055,-3.08939144689937,
22.7698693409104));
#65499=CARTESIAN_POINT('Ctrl Pts',(-7.35765725544608,-2.90668207951638,
22.7619787628493));
#65500=CARTESIAN_POINT('Ctrl Pts',(-7.42979771891297,-2.72407359674528,
22.7540925416415));
#65501=CARTESIAN_POINT('Ctrl Pts',(-7.49517802851293,-2.53867134475953,
22.7462063204337));
#65502=CARTESIAN_POINT('Ctrl Pts',(-7.55358412795725,-2.35101846480887,
22.7383200992259));
#65503=CARTESIAN_POINT('Ctrl Pts',(-7.61282584253642,-2.16068083809245,
22.7303210499768));
#65504=CARTESIAN_POINT('Ctrl Pts',(-7.66489210879814,-1.96802801737583,
22.7223220007277));
#65505=CARTESIAN_POINT('Ctrl Pts',(-7.70961103913861,-1.773645574852,22.7143229514787));
#65506=CARTESIAN_POINT('Ctrl Pts',(-7.75367631114435,-1.58210442801016,
22.7064408246419));
#65507=CARTESIAN_POINT('Ctrl Pts',(-7.79060750583644,-1.38888422606102,
22.6985586978051));
#65508=CARTESIAN_POINT('Ctrl Pts',(-7.82029101971393,-1.19455823088774,
22.6906765709684));
#65509=CARTESIAN_POINT('Ctrl Pts',(-7.8506350154868,-0.995908327091516,
22.6826190605132));
#65510=CARTESIAN_POINT('Ctrl Pts',(-7.87340495139189,-0.796103210318132,
22.6745615500579));
#65511=CARTESIAN_POINT('Ctrl Pts',(-7.88853513891433,-0.595763679753899,
22.6665040396027));
#65512=CARTESIAN_POINT('Ctrl Pts',(-7.90366532643677,-0.395424149189665,
22.6584465291475));
#65513=CARTESIAN_POINT('Ctrl Pts',(-7.91115575002603,-0.194550588700236,
22.6503890186922));
#65514=CARTESIAN_POINT('Ctrl Pts',(-7.91099754422913,0.00623339398873903,
22.642331508237));
#65515=CARTESIAN_POINT('',(-7.91848594748034,0.000888686695662845,20.6423541988083));
#65516=CARTESIAN_POINT('Ctrl Pts',(-7.90381617034521,0.00628295359526841,
22.6423292903089));
#65517=CARTESIAN_POINT('Ctrl Pts',(-7.90984156749653,0.86262601629398,22.6079330164751));
#65518=CARTESIAN_POINT('Ctrl Pts',(-7.38540658840461,4.34883843418324,22.4676023628386));
#65519=CARTESIAN_POINT('Ctrl Pts',(-2.30235307566298,9.06792087288601,22.2213373293996));
#65520=CARTESIAN_POINT('Ctrl Pts',(6.38434810196999,6.83974694744736,21.9035341899918));
#65521=CARTESIAN_POINT('Ctrl Pts',(8.72304347646132,-0.234661512707255,
21.6386982404854));
#65522=CARTESIAN_POINT('Ctrl Pts',(6.40966022654009,-5.15172471127276,21.4268294808803));
#65523=CARTESIAN_POINT('Ctrl Pts',(2.10518128385569,-8.46845707787939,21.2149607212753));
#65524=CARTESIAN_POINT('Ctrl Pts',(-5.21263751244591,-7.71560869397964,
20.9534841473543));
#65525=CARTESIAN_POINT('Ctrl Pts',(-7.91649490000832,-2.53781226327639,
20.7449747633346));
#65526=CARTESIAN_POINT('Ctrl Pts',(-7.92424408506929,0.000873706451288429,
20.6423997591175));
#65527=CARTESIAN_POINT('',(-7.911,-2.74780198594726E-13,18.642331508237));
#65528=CARTESIAN_POINT('Ctrl Pts',(-7.91099994505201,0.000908162115281039,
20.6422949670549));
#65529=CARTESIAN_POINT('Ctrl Pts',(-7.9107335608261,2.20227658242684,20.5537197117162));
#65530=CARTESIAN_POINT('Ctrl Pts',(-6.94192137756157,4.38630738163188,20.4651444563776));
#65531=CARTESIAN_POINT('Ctrl Pts',(-3.67820201488333,7.34180684107607,20.2879817653061));
#65532=CARTESIAN_POINT('Ctrl Pts',(-1.40868175871801,8.08992666571325,20.1993943295734));
#65533=CARTESIAN_POINT('Ctrl Pts',(2.97309270521211,7.6545422802528,20.022219458108));
#65534=CARTESIAN_POINT('Ctrl Pts',(5.05102072675545,6.47444880834269,19.9336320223752));
#65535=CARTESIAN_POINT('Ctrl Pts',(7.66951518847842,2.93425195367783,19.7564571509098));
#65536=CARTESIAN_POINT('Ctrl Pts',(8.18956872247064,0.601881960100036,19.6678697151771));
#65537=CARTESIAN_POINT('Ctrl Pts',(7.32306689761385,-3.71537198232363,19.4906948437116));
#65538=CARTESIAN_POINT('Ctrl Pts',(5.94329958850271,-5.66643518936436,19.4021074079789));
#65539=CARTESIAN_POINT('Ctrl Pts',(2.16154501637954,-7.92205913232967,19.2249325365135));
#65540=CARTESIAN_POINT('Ctrl Pts',(-0.210816529299205,-8.20894963713004,
19.1363451007807));
#65541=CARTESIAN_POINT('Ctrl Pts',(-4.42123908576331,-6.91982244717898,
18.9591702293153));
#65542=CARTESIAN_POINT('Ctrl Pts',(-6.22631625634102,-5.35390358803619,
18.8705827935826));
#65543=CARTESIAN_POINT('Ctrl Pts',(-7.65317280859465,-2.31334857514614,
18.7354407413122));
#65544=CARTESIAN_POINT('Ctrl Pts',(-7.91099999999996,-1.15702837836581,
18.6888861247746));
#65545=CARTESIAN_POINT('Ctrl Pts',(-7.911,-2.74780198594726E-13,18.642331508237));
#65546=CARTESIAN_POINT('',(-7.9028343770497,0.00216472906886937,16.642331508237));
#65547=CARTESIAN_POINT('Ctrl Pts',(-7.911,-2.74780198594726E-13,18.642331508237));
#65548=CARTESIAN_POINT('Ctrl Pts',(-7.91100000000008,2.20167589666645,18.5537440725043));
#65549=CARTESIAN_POINT('Ctrl Pts',(-6.94214576672391,4.3861041833865,18.4651566367716));
#65550=CARTESIAN_POINT('Ctrl Pts',(-3.67820201488328,7.3418068410761,18.2879817653061));
#65551=CARTESIAN_POINT('Ctrl Pts',(-1.40868175871795,8.08992666571326,18.1993943295734));
#65552=CARTESIAN_POINT('Ctrl Pts',(2.97309270521216,7.65454228025278,18.022219458108));
#65553=CARTESIAN_POINT('Ctrl Pts',(5.05102072675549,6.47444880834266,17.9336320223752));
#65554=CARTESIAN_POINT('Ctrl Pts',(7.66951518847843,2.93425195367777,17.7564571509098));
#65555=CARTESIAN_POINT('Ctrl Pts',(8.18956872247064,0.601881960099978,17.6678697151771));
#65556=CARTESIAN_POINT('Ctrl Pts',(7.32306689761383,-3.71537198232368,17.4906948437116));
#65557=CARTESIAN_POINT('Ctrl Pts',(5.94329958850267,-5.6664351893644,17.4021074079789));
#65558=CARTESIAN_POINT('Ctrl Pts',(2.16154501637949,-7.92205913232969,17.2249325365135));
#65559=CARTESIAN_POINT('Ctrl Pts',(-0.210816529299263,-8.20894963713004,
17.1363451007807));
#65560=CARTESIAN_POINT('Ctrl Pts',(-4.42123908576336,-6.91982244717894,
16.9591702293153));
#65561=CARTESIAN_POINT('Ctrl Pts',(-6.22631625634105,-5.35390358803615,
16.8705827935826));
#65562=CARTESIAN_POINT('Ctrl Pts',(-7.65317280859467,-2.31334857514607,
16.7354407413122));
#65563=CARTESIAN_POINT('Ctrl Pts',(-7.91099999999997,-1.15702837836572,
16.6888861247746));
#65564=CARTESIAN_POINT('Ctrl Pts',(-7.911,-1.64868119156836E-13,16.642331508237));
#65565=CARTESIAN_POINT('',(-7.91527914730039,0.000969948445309178,14.6424015413963));
#65566=CARTESIAN_POINT('Ctrl Pts',(-7.89668078699942,0.00379606269054533,
16.642331508237));
#65567=CARTESIAN_POINT('Ctrl Pts',(-7.90106252337055,1.17903434357931,16.5951812788451));
#65568=CARTESIAN_POINT('Ctrl Pts',(-7.10778324508014,4.98943963042238,16.4420966696509));
#65569=CARTESIAN_POINT('Ctrl Pts',(-1.19022084510717,9.27962245901281,16.1830776806536));
#65570=CARTESIAN_POINT('Ctrl Pts',(7.1481032504245,6.02560715721669,15.8652745412461));
#65571=CARTESIAN_POINT('Ctrl Pts',(8.94447937923684,-2.74304707876909,15.5474714018383));
#65572=CARTESIAN_POINT('Ctrl Pts',(2.52814114509511,-9.00835952561415,15.2296682624306));
#65573=CARTESIAN_POINT('Ctrl Pts',(-4.73176752524436,-7.33191172920264,
14.9648323129244));
#65574=CARTESIAN_POINT('Ctrl Pts',(-7.50325925665173,-3.14592317945734,
14.7690954788964));
#65575=CARTESIAN_POINT('Ctrl Pts',(-7.91181181028092,-0.91279513892285,
14.679293024671));
#65576=CARTESIAN_POINT('Ctrl Pts',(-7.91746780378482,0.000959046564810386,
14.6424577603469));
#65577=CARTESIAN_POINT('',(-7.91553726929787,-0.000951753929678635,12.6422689007438));
#65578=CARTESIAN_POINT('Ctrl Pts',(-7.91099993453595,0.000991263561006212,
14.6422916233472));
#65579=CARTESIAN_POINT('Ctrl Pts',(-7.91070917900769,2.20233154695537,14.5537174825778));
#65580=CARTESIAN_POINT('Ctrl Pts',(-6.94190084478929,4.38632597532549,14.4651433418083));
#65581=CARTESIAN_POINT('Ctrl Pts',(-3.67820201488291,7.3418068410763,14.2879817653061));
#65582=CARTESIAN_POINT('Ctrl Pts',(-1.40868175871746,8.08992666571337,14.1993943295734));
#65583=CARTESIAN_POINT('Ctrl Pts',(2.97309270521278,7.65454228025256,14.0222194581079));
#65584=CARTESIAN_POINT('Ctrl Pts',(5.05102072675609,6.47444880834222,13.9336320223752));
#65585=CARTESIAN_POINT('Ctrl Pts',(7.66951518847877,2.93425195367695,13.7564571509098));
#65586=CARTESIAN_POINT('Ctrl Pts',(8.18956872247073,0.601881960099008,13.667869715177));
#65587=CARTESIAN_POINT('Ctrl Pts',(7.32306689761334,-3.71537198232469,13.4906948437116));
#65588=CARTESIAN_POINT('Ctrl Pts',(5.94329958850185,-5.66643518936529,13.4021074079789));
#65589=CARTESIAN_POINT('Ctrl Pts',(2.16154501637819,-7.92205913233006,13.2249325365134));
#65590=CARTESIAN_POINT('Ctrl Pts',(-0.210816529300703,-8.20894963713002,
13.1363451007807));
#65591=CARTESIAN_POINT('Ctrl Pts',(-4.4212390857647,-6.91982244717811,12.9591702293152));
#65592=CARTESIAN_POINT('Ctrl Pts',(-6.22631625634216,-5.35390358803489,
12.8705827935825));
#65593=CARTESIAN_POINT('Ctrl Pts',(-7.65303491965023,-2.31364240911259,
12.735453801206));
#65594=CARTESIAN_POINT('Ctrl Pts',(-7.91085532589086,-1.15767713118784,
12.6889122445621));
#65595=CARTESIAN_POINT('Ctrl Pts',(-7.91099993913047,-0.000973737913675424,
12.6423706879183));
#65596=CARTESIAN_POINT('',(-7.89704659861909,-0.00212787115983104,10.6422490387989));
#65597=CARTESIAN_POINT('Ctrl Pts',(-7.91798387824917,-0.000939899775352797,
12.642214015293));
#65598=CARTESIAN_POINT('Ctrl Pts',(-7.91240748074079,0.9404534482577,12.6042565360171));
#65599=CARTESIAN_POINT('Ctrl Pts',(-7.48579772889252,3.20106885968654,12.5133318668401));
#65600=CARTESIAN_POINT('Ctrl Pts',(-4.65416054181148,7.3814187774994,12.3164728178603));
#65601=CARTESIAN_POINT('Ctrl Pts',(2.6230288800739,8.9811891465743,12.051636868354));
#65602=CARTESIAN_POINT('Ctrl Pts',(8.97291786243676,2.64853991397236,11.7338337289462));
#65603=CARTESIAN_POINT('Ctrl Pts',(7.08414191259461,-6.1006766062498,11.4160305895387));
#65604=CARTESIAN_POINT('Ctrl Pts',(-1.28804455293763,-9.26655059186473,
11.0982274501309));
#65605=CARTESIAN_POINT('Ctrl Pts',(-7.13464643336658,-4.93299045016783,
10.8403277563637));
#65606=CARTESIAN_POINT('Ctrl Pts',(-7.90190329265851,-1.1513941715232,10.6883624423991));
#65607=CARTESIAN_POINT('Ctrl Pts',(-7.89705579113888,-0.00418322831448492,
10.642331508237));
#65608=CARTESIAN_POINT('',(-7.90817188740471,-3.24836861786255E-5,8.64270656474482));
#65609=CARTESIAN_POINT('Ctrl Pts',(-7.89703740609931,-7.2514005176659E-5,
10.6421665693608));
#65610=CARTESIAN_POINT('Ctrl Pts',(-7.89702702068455,0.00212803473133817,
10.6420782743881));
#65611=CARTESIAN_POINT('Ctrl Pts',(-7.8970167925981,0.00413170092462163,
10.6419978793563));
#65612=CARTESIAN_POINT('Ctrl Pts',(-7.89700473044708,0.00632931527902227,
10.6419097025558));
#65613=CARTESIAN_POINT('Ctrl Pts',(-7.89555713694605,0.27006770257325,10.631327496845));
#65614=CARTESIAN_POINT('Ctrl Pts',(-7.88121311475603,0.534201069122857,
10.620936877814));
#65615=CARTESIAN_POINT('Ctrl Pts',(-7.85413508916187,0.797232455759467,
10.6106644974064));
#65616=CARTESIAN_POINT('Ctrl Pts',(-7.82687300158976,1.06205178949431,10.6003222908348));
#65617=CARTESIAN_POINT('Ctrl Pts',(-7.78670404858205,1.32575354639783,10.5900999357962));
#65618=CARTESIAN_POINT('Ctrl Pts',(-7.73382622050846,1.58685167858934,10.579922578301));
#65619=CARTESIAN_POINT('Ctrl Pts',(-7.68088919018293,1.84824213741315,10.5697338261911));
#65620=CARTESIAN_POINT('Ctrl Pts',(-7.61521569910729,2.10702279727448,10.5595901724399));
#65621=CARTESIAN_POINT('Ctrl Pts',(-7.5370235017524,2.36175098493019,10.5494165113558));
#65622=CARTESIAN_POINT('Ctrl Pts',(-7.45905535631495,2.6157492744528,10.5392720018796));
#65623=CARTESIAN_POINT('Ctrl Pts',(-7.36864102369296,2.8657181736505,10.5290976567902));
#65624=CARTESIAN_POINT('Ctrl Pts',(-7.26600211153003,3.11027875781575,10.5188190141712));
#65625=CARTESIAN_POINT('Ctrl Pts',(-7.16384440122462,3.35369276896209,10.508588560897));
#65626=CARTESIAN_POINT('Ctrl Pts',(-7.04957730822994,3.59174915994034,10.4982547857566));
#65627=CARTESIAN_POINT('Ctrl Pts',(-6.92341216917452,3.82313929640141,10.4877442692305));
#65628=CARTESIAN_POINT('Ctrl Pts',(-6.84744917416091,3.96245739895959,10.4814159734711));
#65629=CARTESIAN_POINT('Ctrl Pts',(-6.76717276827334,4.09935987343639,10.4750236063915));
#65630=CARTESIAN_POINT('Ctrl Pts',(-6.68262590130838,4.23356965677974,10.4685511429316));
#65631=CARTESIAN_POINT('Ctrl Pts',(-6.54417057120691,4.45335378980207,10.4579517310659));
#65632=CARTESIAN_POINT('Ctrl Pts',(-6.3942646586491,4.66591471059473,10.4471375177489));
#65633=CARTESIAN_POINT('Ctrl Pts',(-6.2341008017312,4.87068285980329,10.436038125106));
#65634=CARTESIAN_POINT('Ctrl Pts',(-6.09355091025868,5.05037471851674,10.4262979848435));
#65635=CARTESIAN_POINT('Ctrl Pts',(-5.94510155572144,5.22406642500045,10.4163382356336));
#65636=CARTESIAN_POINT('Ctrl Pts',(-5.78953492220527,5.39139621295431,10.4061113183207));
#65637=CARTESIAN_POINT('Ctrl Pts',(-5.70004020286178,5.48765806597681,10.4002279545558));
#65638=CARTESIAN_POINT('Ctrl Pts',(-5.60808757673465,5.58164513007581,10.3943687592721));
#65639=CARTESIAN_POINT('Ctrl Pts',(-5.51362768341834,5.67309653812542,10.3886852955563));
#65640=CARTESIAN_POINT('Ctrl Pts',(-5.44683502953349,5.73776189006145,10.3846665145531));
#65641=CARTESIAN_POINT('Ctrl Pts',(-5.37878938090202,5.80115853730033,10.3807355978151));
#65642=CARTESIAN_POINT('Ctrl Pts',(-5.3094837862637,5.8631825275386,10.3769461295963));
#65643=CARTESIAN_POINT('Ctrl Pts',(-5.13111694733864,6.0228092233927,10.3671934469895));
#65644=CARTESIAN_POINT('Ctrl Pts',(-4.94564170770916,6.17430019275652,10.3575033034082));
#65645=CARTESIAN_POINT('Ctrl Pts',(-4.75385236145091,6.31723214046822,10.3478841393255));
#65646=CARTESIAN_POINT('Ctrl Pts',(-4.55885457981442,6.46255519032749,10.3381040566779));
#65647=CARTESIAN_POINT('Ctrl Pts',(-4.3573289131039,6.59903091686291,10.3283973482188));
#65648=CARTESIAN_POINT('Ctrl Pts',(-4.15007692950517,6.72617240645461,10.3187728851479));
#65649=CARTESIAN_POINT('Ctrl Pts',(-4.04720521653535,6.78928042885673,10.3139956811602));
#65650=CARTESIAN_POINT('Ctrl Pts',(-3.94292225070908,6.85008805127412,10.3092387402827));
#65651=CARTESIAN_POINT('Ctrl Pts',(-3.83732397753682,6.90853144666653,10.3045031473766));
#65652=CARTESIAN_POINT('Ctrl Pts',(-3.620076390972,7.0287671874437,10.2947606004685));
#65653=CARTESIAN_POINT('Ctrl Pts',(-3.3972622476175,7.13899997770821,10.2851084087083));
#65654=CARTESIAN_POINT('Ctrl Pts',(-3.16976350958247,7.23873507443482,10.275556018546));
#65655=CARTESIAN_POINT('Ctrl Pts',(-2.94226477154745,7.33847017116143,10.2660036283837));
#65656=CARTESIAN_POINT('Ctrl Pts',(-2.71008049778106,7.42770786090225,10.2565510398193));
#65657=CARTESIAN_POINT('Ctrl Pts',(-2.47409109842804,7.50589469250486,10.2472076993025));
#65658=CARTESIAN_POINT('Ctrl Pts',(-2.19846253296326,7.59721457505867,10.2362949568219));
#65659=CARTESIAN_POINT('Ctrl Pts',(-1.91787860110224,7.67403236286004,10.2251698700566));
#65660=CARTESIAN_POINT('Ctrl Pts',(-1.6340284544711,7.73543001613488,10.213830036402));
#65661=CARTESIAN_POINT('Ctrl Pts',(-1.35036972588251,7.79678626510274,10.202497849912));
#65662=CARTESIAN_POINT('Ctrl Pts',(-1.06345026831751,7.84274278214282,10.1909512060697));
#65663=CARTESIAN_POINT('Ctrl Pts',(-0.774977872832234,7.87242967015964,
10.1791877071281));
#65664=CARTESIAN_POINT('Ctrl Pts',(-0.53831386443594,7.89678492225596,10.1695368814135));
#65665=CARTESIAN_POINT('Ctrl Pts',(-0.300605292751217,7.91019043798737,
10.1597400984903));
#65666=CARTESIAN_POINT('Ctrl Pts',(-0.0627986367552478,7.91219190920741,
10.1497960343608));
#65667=CARTESIAN_POINT('Ctrl Pts',(0.219271870481511,7.91456592182659,10.1380010440092));
#65668=CARTESIAN_POINT('Ctrl Pts',(0.501479517216926,7.90089439683192,10.1259988417638));
#65669=CARTESIAN_POINT('Ctrl Pts',(0.782278769383866,7.87199419134308,10.1137872181538));
#65670=CARTESIAN_POINT('Ctrl Pts',(1.01297476499424,7.84825067483746,10.1037545252425));
#65671=CARTESIAN_POINT('Ctrl Pts',(1.24234299120268,7.81377352999714,10.0938813063388));
#65672=CARTESIAN_POINT('Ctrl Pts',(1.46963759991846,7.76913012586632,10.0841330693608));
#65673=CARTESIAN_POINT('Ctrl Pts',(1.70346444832434,7.72320371102965,10.0741046769455));
#65674=CARTESIAN_POINT('Ctrl Pts',(1.93509725439572,7.66651851932442,10.0642085534158));
#65675=CARTESIAN_POINT('Ctrl Pts',(2.16375259399093,7.59964465304451,10.0544071465934));
#65676=CARTESIAN_POINT('Ctrl Pts',(2.39560012060677,7.53183718124139,10.0444689053385));
#65677=CARTESIAN_POINT('Ctrl Pts',(2.624387123297,7.45355465361222,10.034628043873));
#65678=CARTESIAN_POINT('Ctrl Pts',(2.84931711292389,7.36534096512308,10.0248454151962));
#65679=CARTESIAN_POINT('Ctrl Pts',(3.07724198741346,7.27595273409839,10.0149325333389));
#65680=CARTESIAN_POINT('Ctrl Pts',(3.30120723175786,7.1763671808047,10.0050794453031));
#65681=CARTESIAN_POINT('Ctrl Pts',(3.52039379899349,7.06709768473889,9.99524541947884));
#65682=CARTESIAN_POINT('Ctrl Pts',(3.6483425847122,7.00331230083493,9.98950486850069));
#65683=CARTESIAN_POINT('Ctrl Pts',(3.77466312743019,6.93622606141243,9.98377081309979));
#65684=CARTESIAN_POINT('Ctrl Pts',(3.89919232314342,6.86593288751937,9.97803515116346));
#65685=CARTESIAN_POINT('Ctrl Pts',(4.1684164793643,6.7139635415274,9.96563501691116));
#65686=CARTESIAN_POINT('Ctrl Pts',(4.42910711837882,6.54663212729827,9.9534595189747));
#65687=CARTESIAN_POINT('Ctrl Pts',(4.67936144343141,6.36497348585735,9.94142699231249));
#65688=CARTESIAN_POINT('Ctrl Pts',(4.92193896997612,6.18888740260204,9.92976357528588));
#65689=CARTESIAN_POINT('Ctrl Pts',(5.15471203616973,5.99933981309755,9.91823449250182));
#65690=CARTESIAN_POINT('Ctrl Pts',(5.37594902342265,5.79722587738221,9.90676536619906));
#65691=CARTESIAN_POINT('Ctrl Pts',(5.58221097229248,5.60879258332934,9.89607255948345));
#65692=CARTESIAN_POINT('Ctrl Pts',(5.77844670814061,5.40943631042047,9.88543186730674));
#65693=CARTESIAN_POINT('Ctrl Pts',(5.96323750513471,5.19984156073173,9.87478301605315));
#65694=CARTESIAN_POINT('Ctrl Pts',(6.10325066591985,5.04103482432902,9.86671454431647));
#65695=CARTESIAN_POINT('Ctrl Pts',(6.2366932871527,4.87634952504931,9.85864138856705));
#65696=CARTESIAN_POINT('Ctrl Pts',(6.36293627257074,4.70606719169118,9.85053733121235));
#65697=CARTESIAN_POINT('Ctrl Pts',(6.45160000815178,4.58647347542257,9.84484564073109));
#65698=CARTESIAN_POINT('Ctrl Pts',(6.53673968783333,4.46439922780143,9.83903742432002));
#65699=CARTESIAN_POINT('Ctrl Pts',(6.61812466727398,4.3399314349128,9.83313430227379));
#65700=CARTESIAN_POINT('Ctrl Pts',(6.75370500146756,4.13257886110665,9.82330021169203));
#65701=CARTESIAN_POINT('Ctrl Pts',(6.87886655377201,3.91858118728099,9.81320273256478));
#65702=CARTESIAN_POINT('Ctrl Pts',(6.99344417898774,3.69901002383476,9.80294182320879));
#65703=CARTESIAN_POINT('Ctrl Pts',(7.10858965371848,3.4783506603282,9.79263006053488));
#65704=CARTESIAN_POINT('Ctrl Pts',(7.2130450888691,3.2520621136234,9.7821532436896));
#65705=CARTESIAN_POINT('Ctrl Pts',(7.30662205930488,3.02128078655226,9.77161282455504));
#65706=CARTESIAN_POINT('Ctrl Pts',(7.40058146661728,2.78955628628909,9.76102932810184));
#65707=CARTESIAN_POINT('Ctrl Pts',(7.48357232131068,2.5533021140594,9.75038170842851));
#65708=CARTESIAN_POINT('Ctrl Pts',(7.55539753140135,2.31372078523287,9.73977266636942));
#65709=CARTESIAN_POINT('Ctrl Pts',(7.61423297563002,2.11746832885144,9.73108229565418));
#65710=CARTESIAN_POINT('Ctrl Pts',(7.66557588020918,1.91898436532077,9.72241781062201));
#65711=CARTESIAN_POINT('Ctrl Pts',(7.70932182241582,1.71895566935502,9.71383566080776));
#65712=CARTESIAN_POINT('Ctrl Pts',(7.75822972503801,1.49532386511304,9.70424082923638));
#65713=CARTESIAN_POINT('Ctrl Pts',(7.79765925323227,1.26973381984225,9.69474443889133));
#65714=CARTESIAN_POINT('Ctrl Pts',(7.82759777935467,1.04295255634549,9.68534929909551));
#65715=CARTESIAN_POINT('Ctrl Pts',(7.85781617323768,0.814051323278355,9.67586633277394));
#65716=CARTESIAN_POINT('Ctrl Pts',(7.87836535250214,0.583935620769487,9.66648651884618));
#65717=CARTESIAN_POINT('Ctrl Pts',(7.88918039584671,0.353385737595114,9.65721274615922));
#65718=CARTESIAN_POINT('Ctrl Pts',(7.89991464852466,0.124558110925905,9.64800825052032));
#65719=CARTESIAN_POINT('Ctrl Pts',(7.90105957925932,-0.104698090131597,
9.63890821773866));
#65720=CARTESIAN_POINT('Ctrl Pts',(7.89250110137832,-0.333615219723845,
9.62991547240277));
#65721=CARTESIAN_POINT('Ctrl Pts',(7.88416383567005,-0.556615496306306,
9.62115516381114));
#65722=CARTESIAN_POINT('Ctrl Pts',(7.86661808081932,-0.779294703447366,
9.61249666819413));
#65723=CARTESIAN_POINT('Ctrl Pts',(7.83971248071679,-1.00092736644294,9.60394259673));
#65724=CARTESIAN_POINT('Ctrl Pts',(7.81714654705787,-1.18681238483126,9.59676823122847));
#65725=CARTESIAN_POINT('Ctrl Pts',(7.78799582433962,-1.37196117934447,9.58966732087001));
#65726=CARTESIAN_POINT('Ctrl Pts',(7.75214648273455,-1.55593149415293,9.58264140617834));
#65727=CARTESIAN_POINT('Ctrl Pts',(7.70467843800058,-1.7995262365404,9.57333840595717));
#65728=CARTESIAN_POINT('Ctrl Pts',(7.64595391924143,-2.04102238733024,9.56389437275389));
#65729=CARTESIAN_POINT('Ctrl Pts',(7.57581145299394,-2.27912565841045,9.55431751332156));
#65730=CARTESIAN_POINT('Ctrl Pts',(7.50656737413922,-2.51417929368003,9.54486331467144));
#65731=CARTESIAN_POINT('Ctrl Pts',(7.42619596540761,-2.74592550209097,9.53527967048953));
#65732=CARTESIAN_POINT('Ctrl Pts',(7.33459218539083,-2.97312081782567,9.52557447621325));
#65733=CARTESIAN_POINT('Ctrl Pts',(7.30181172033032,-3.05442279147776,9.5221014668918));
#65734=CARTESIAN_POINT('Ctrl Pts',(7.26759334344641,-3.13514207242139,9.51861289222605));
#65735=CARTESIAN_POINT('Ctrl Pts',(7.23193383328093,-3.21522206971646,9.51510911402665));
#65736=CARTESIAN_POINT('Ctrl Pts',(7.1325267868186,-3.43845889980398,9.50534172685153));
#65737=CARTESIAN_POINT('Ctrl Pts',(7.02191693766909,-3.65672597042445,9.4954561911977));
#65738=CARTESIAN_POINT('Ctrl Pts',(6.90104335864473,-3.86925749793192,9.48546034509179));
#65739=CARTESIAN_POINT('Ctrl Pts',(6.77871191293198,-4.08435238656995,9.47534393822167));
#65740=CARTESIAN_POINT('Ctrl Pts',(6.64586829745989,-4.29357193377647,9.46511454392482));
#65741=CARTESIAN_POINT('Ctrl Pts',(6.50353113152558,-4.49615234994838,9.45478028726757));
#65742=CARTESIAN_POINT('Ctrl Pts',(6.36119286381313,-4.69873433421864,9.44444595061675));
#65743=CARTESIAN_POINT('Ctrl Pts',(6.20936163863106,-4.89467652984285,9.43400674998211));
#65744=CARTESIAN_POINT('Ctrl Pts',(6.0490904654515,-5.08325368747344,9.42347081061866));
#65745=CARTESIAN_POINT('Ctrl Pts',(5.91049103437001,-5.24633159003101,9.41435953269691));
#65746=CARTESIAN_POINT('Ctrl Pts',(5.76558064259386,-5.40390197968804,9.4051759091224));
#65747=CARTESIAN_POINT('Ctrl Pts',(5.61505461253099,-5.55552384739372,9.39592519468185));
#65748=CARTESIAN_POINT('Ctrl Pts',(5.47480690155528,-5.6967925692932,9.38730614371349));
#65749=CARTESIAN_POINT('Ctrl Pts',(5.32928970466327,-5.83266074883043,9.37888526581639));
#65750=CARTESIAN_POINT('Ctrl Pts',(5.17898788440507,-5.96294046145067,9.37060028741146));
#65751=CARTESIAN_POINT('Ctrl Pts',(5.02767409623669,-6.09409733502806,9.36225952703219));
#65752=CARTESIAN_POINT('Ctrl Pts',(4.87151084921231,-6.21959087718161,9.35405650230249));
#65753=CARTESIAN_POINT('Ctrl Pts',(4.71094050224414,-6.33922128397126,9.34592767330901));
#65754=CARTESIAN_POINT('Ctrl Pts',(4.55019310037605,-6.45898360272413,9.33778988096065));
#65755=CARTESIAN_POINT('Ctrl Pts',(4.38502860122831,-6.57287052360287,9.32972644806442));
#65756=CARTESIAN_POINT('Ctrl Pts',(4.21584208175296,-6.68066364004644,9.32167362428589));
#65757=CARTESIAN_POINT('Ctrl Pts',(4.16007671984261,-6.71619319741638,9.31901934288213));
#65758=CARTESIAN_POINT('Ctrl Pts',(4.10387402278031,-6.75106052327771,9.31636621407356));
#65759=CARTESIAN_POINT('Ctrl Pts',(4.04724706045905,-6.78525717371924,9.31371195500284));
#65760=CARTESIAN_POINT('Ctrl Pts',(3.86877282023437,-6.89303659460988,9.3053463840524));
#65761=CARTESIAN_POINT('Ctrl Pts',(3.68574723757595,-6.99386394134694,9.29720584355353));
#65762=CARTESIAN_POINT('Ctrl Pts',(3.49889719965554,-7.08730734369488,9.28920532526346));
#65763=CARTESIAN_POINT('Ctrl Pts',(3.31226265849002,-7.18064297646356,9.28121403408274));
#65764=CARTESIAN_POINT('Ctrl Pts',(3.12181315928759,-7.26661192393304,9.27336244231793));
#65765=CARTESIAN_POINT('Ctrl Pts',(2.92825622783153,-7.34483285249033,9.26556583551076));
#65766=CARTESIAN_POINT('Ctrl Pts',(2.73518574491443,-7.42285719570125,9.25778882318653));
#65767=CARTESIAN_POINT('Ctrl Pts',(2.5390240120457,-7.49317274126278,9.25006651979013));
#65768=CARTESIAN_POINT('Ctrl Pts',(2.34044700890272,-7.55544561978073,9.24231484797419));
#65769=CARTESIAN_POINT('Ctrl Pts',(2.14248387900954,-7.61752599033601,9.23458713937601));
#65770=CARTESIAN_POINT('Ctrl Pts',(1.9421208672976,-7.67161374140195,9.22683024365442));
#65771=CARTESIAN_POINT('Ctrl Pts',(1.73999367948123,-7.7174170398759,9.21896086079442));
#65772=CARTESIAN_POINT('Ctrl Pts',(1.56613390118553,-7.75681476466454,9.21219200810249));
#65773=CARTESIAN_POINT('Ctrl Pts',(1.39096847410628,-7.7900839588043,9.2053399308244));
#65774=CARTESIAN_POINT('Ctrl Pts',(1.21487801380399,-7.81705842571823,9.19835161768601));
#65775=CARTESIAN_POINT('Ctrl Pts',(1.0098590372569,-7.84846431556657,9.19021524956609));
#65776=CARTESIAN_POINT('Ctrl Pts',(0.803587424053422,-7.87133746293345,
9.18189420653297));
#65777=CARTESIAN_POINT('Ctrl Pts',(0.596720111584622,-7.88607584164099,
9.17330482375524));
#65778=CARTESIAN_POINT('Ctrl Pts',(0.39076607409736,-7.9007491535558,9.16475336126711));
#65779=CARTESIAN_POINT('Ctrl Pts',(0.184221793699587,-7.90736010137687,
9.15593592312961));
#65780=CARTESIAN_POINT('Ctrl Pts',(-0.0223140826013648,-7.90631499665483,
9.14676994771359));
#65781=CARTESIAN_POINT('Ctrl Pts',(-0.131389206576435,-7.90576305900039,
9.14192923953853));
#65782=CARTESIAN_POINT('Ctrl Pts',(-0.240462840871124,-7.90307594974536,
9.13699132164999));
#65783=CARTESIAN_POINT('Ctrl Pts',(-0.349452669468577,-7.89831402156496,
9.13194403305901));
#65784=CARTESIAN_POINT('Ctrl Pts',(-0.533994996194332,-7.89025109204741,
9.12339792933334));
#65785=CARTESIAN_POINT('Ctrl Pts',(-0.718108056857789,-7.87516509976259,
9.11517006747972));
#65786=CARTESIAN_POINT('Ctrl Pts',(-0.901368396608811,-7.85341029818643,
9.10717206460129));
#65787=CARTESIAN_POINT('Ctrl Pts',(-1.08568892050605,-7.83152964234323,
9.0991277922689));
#65788=CARTESIAN_POINT('Ctrl Pts',(-1.26914711928099,-7.80290320176188,
9.0913160461308));
#65789=CARTESIAN_POINT('Ctrl Pts',(-1.45135891336227,-7.76786640856552,
9.08364690048055));
#65790=CARTESIAN_POINT('Ctrl Pts',(-1.63498581304967,-7.73255751024708,
9.07591819419066));
#65791=CARTESIAN_POINT('Ctrl Pts',(-1.81734721592646,-7.69073871274669,
9.06833431193674));
#65792=CARTESIAN_POINT('Ctrl Pts',(-1.99809262181031,-7.64272181670799,
9.06080321653726));
#65793=CARTESIAN_POINT('Ctrl Pts',(-2.10335603487673,-7.61475749674548,
9.05641721954883));
#65794=CARTESIAN_POINT('Ctrl Pts',(-2.20807211685569,-7.58469033334239,
9.05204912639857));
#65795=CARTESIAN_POINT('Ctrl Pts',(-2.31217745076366,-7.55257622973733,
9.04768075708763));
#65796=CARTESIAN_POINT('Ctrl Pts',(-2.53339558011493,-7.48433551950067,
9.0383982116982));
#65797=CARTESIAN_POINT('Ctrl Pts',(-2.75200593699641,-7.40633864216497,
9.02935840111635));
#65798=CARTESIAN_POINT('Ctrl Pts',(-2.96702330165383,-7.31902232135849,
9.0204752354755));
#65799=CARTESIAN_POINT('Ctrl Pts',(-3.18265007296923,-7.2314585268313,9.01156689298304));
#65800=CARTESIAN_POINT('Ctrl Pts',(-3.39466327846068,-7.13452322304539,
9.00281608462254));
#65801=CARTESIAN_POINT('Ctrl Pts',(-3.60212000872174,-7.02867003300061,
8.99413598645784));
#65802=CARTESIAN_POINT('Ctrl Pts',(-3.82000675679168,-6.91749500714021,
8.98501949088956));
#65803=CARTESIAN_POINT('Ctrl Pts',(-4.03286685373061,-6.79648380236499,
8.97598099424619));
#65804=CARTESIAN_POINT('Ctrl Pts',(-4.23966966324943,-6.66616269160833,
8.96691990779514));
#65805=CARTESIAN_POINT('Ctrl Pts',(-4.4361580294336,-6.54234144279908,8.95831074974374));
#65806=CARTESIAN_POINT('Ctrl Pts',(-4.62717887254434,-6.41011651956876,
8.94968119905727));
#65807=CARTESIAN_POINT('Ctrl Pts',(-4.81190003464847,-6.26992772426865,
8.94094497962545));
#65808=CARTESIAN_POINT('Ctrl Pts',(-4.99616121317992,-6.13008802022683,
8.93223051469852));
#65809=CARTESIAN_POINT('Ctrl Pts',(-5.17415435597442,-5.98232474636406,
8.92340991160736));
#65810=CARTESIAN_POINT('Ctrl Pts',(-5.34510027977848,-5.82705221848147,
8.91439753715966));
#65811=CARTESIAN_POINT('Ctrl Pts',(-5.51533200361693,-5.67242840822611,
8.90542281577428));
#65812=CARTESIAN_POINT('Ctrl Pts',(-5.67857572524734,-5.51035857045978,
8.89625792209928));
#65813=CARTESIAN_POINT('Ctrl Pts',(-5.83410269058135,-5.34122009760758,
8.88681829177263));
#65814=CARTESIAN_POINT('Ctrl Pts',(-5.86019177437216,-5.31284773284747,
8.88523482805612));
#65815=CARTESIAN_POINT('Ctrl Pts',(-5.88606380104645,-5.28427638023463,
8.88364363356768));
#65816=CARTESIAN_POINT('Ctrl Pts',(-5.91171542817903,-5.25550771479195,
8.88204430914758));
#65817=CARTESIAN_POINT('Ctrl Pts',(-6.06300674317755,-5.085832348661,8.87261161728062));
#65818=CARTESIAN_POINT('Ctrl Pts',(-6.2066291982959,-4.90929692272948,8.86289612173482));
#65819=CARTESIAN_POINT('Ctrl Pts',(-6.34255282084846,-4.72680038854599,
8.85281593003401));
#65820=CARTESIAN_POINT('Ctrl Pts',(-6.42443673137412,-4.61685974985719,
8.8467433614855));
#65821=CARTESIAN_POINT('Ctrl Pts',(-6.50352715000144,-4.50475489559639,
8.84053843851567));
#65822=CARTESIAN_POINT('Ctrl Pts',(-6.57982143804972,-4.39067407350341,
8.83418325692507));
#65823=CARTESIAN_POINT('Ctrl Pts',(-6.66262998064053,-4.26685265964994,
8.82728544925323));
#65824=CARTESIAN_POINT('Ctrl Pts',(-6.74183405868872,-4.14066738188957,
8.82037815828341));
#65825=CARTESIAN_POINT('Ctrl Pts',(-6.81720648710848,-4.01222251231833,
8.81359871654385));
#65826=CARTESIAN_POINT('Ctrl Pts',(-6.89252770279151,-3.88386491621602,
8.80682388118055));
#65827=CARTESIAN_POINT('Ctrl Pts',(-6.96402204106891,-3.75325047507872,
8.80017672136903));
#65828=CARTESIAN_POINT('Ctrl Pts',(-7.0314313039316,-3.62052458635116,8.79379428989082));
#65829=CARTESIAN_POINT('Ctrl Pts',(-7.0752591266859,-3.53422952126631,8.78964459200525));
#65830=CARTESIAN_POINT('Ctrl Pts',(-7.1173594500746,-3.44704274577096,8.78560680210125));
#65831=CARTESIAN_POINT('Ctrl Pts',(-7.15765548612065,-3.35901452181828,
8.78171858872071));
#65832=CARTESIAN_POINT('Ctrl Pts',(-7.25215275396775,-3.1525816447121,8.77260043275997));
#65833=CARTESIAN_POINT('Ctrl Pts',(-7.33793684335818,-2.94228142107834,
8.76349613287821));
#65834=CARTESIAN_POINT('Ctrl Pts',(-7.41492855600244,-2.72885753313259,
8.7543997876551));
#65835=CARTESIAN_POINT('Ctrl Pts',(-7.49370634335228,-2.51048257974443,
8.74509242293966));
#65836=CARTESIAN_POINT('Ctrl Pts',(-7.56327943433531,-2.28883665517175,
8.73579338623242));
#65837=CARTESIAN_POINT('Ctrl Pts',(-7.62351601627474,-2.06468814798325,
8.72649635580341));
#65838=CARTESIAN_POINT('Ctrl Pts',(-7.68355400772679,-1.84127862298557,
8.71722997621388));
#65839=CARTESIAN_POINT('Ctrl Pts',(-7.73431710757442,-1.61538216568751,
8.70796558969562));
#65840=CARTESIAN_POINT('Ctrl Pts',(-7.77562516852486,-1.38774352143513,
8.69869693683797));
#65841=CARTESIAN_POINT('Ctrl Pts',(-7.81713818439863,-1.15897542061162,
8.68938229644199));
#65842=CARTESIAN_POINT('Ctrl Pts',(-7.84910234635378,-0.928446981403521,
8.68006334726568));
#65843=CARTESIAN_POINT('Ctrl Pts',(-7.87128150063596,-0.696910155248286,
8.67073373626488));
#65844=CARTESIAN_POINT('Ctrl Pts',(-7.89346065491813,-0.46537332909306,
8.66140412526407));
#65845=CARTESIAN_POINT('Ctrl Pts',(-7.90585501534277,-0.232827279694014,
8.65206385243877));
#65846=CARTESIAN_POINT('Ctrl Pts',(-7.90817188740471,-3.24836861791286E-5,
8.64270656474482));
#65847=CARTESIAN_POINT('',(-7.91099726676438,-0.00657611181310816,4.63857422362495));
#65848=CARTESIAN_POINT('Ctrl Pts',(-7.91099897267188,0.00403167266891616,
8.64093322807217));
#65849=CARTESIAN_POINT('Ctrl Pts',(-7.91071147929497,0.568154803721865,
8.62151017142005));
#65850=CARTESIAN_POINT('Ctrl Pts',(-7.85008557225209,1.13058901663712,8.60282672000359));
#65851=CARTESIAN_POINT('Ctrl Pts',(-7.70446776992235,1.79992327657939,8.57706428746811));
#65852=CARTESIAN_POINT('Ctrl Pts',(-7.67605254157754,1.91748852523687,8.57239830883372));
#65853=CARTESIAN_POINT('Ctrl Pts',(-7.6399084192444,2.05331572809818,8.56679485636979));
#65854=CARTESIAN_POINT('Ctrl Pts',(-7.6347912945223,2.0722615688514,8.56600840973354));
#65855=CARTESIAN_POINT('Ctrl Pts',(-7.62806804450101,2.09679103890409,8.56498366270866));
#65856=CARTESIAN_POINT('Ctrl Pts',(-7.62652615056634,2.10239235794477,8.56474921959791));
#65857=CARTESIAN_POINT('Ctrl Pts',(-7.62402124448975,2.11145304428912,8.56436926261314));
#65858=CARTESIAN_POINT('Ctrl Pts',(-7.62306204223672,2.11491347217686,8.56422398012812));
#65859=CARTESIAN_POINT('Ctrl Pts',(-7.62122376175076,2.12152777333931,8.56394595733856));
#65860=CARTESIAN_POINT('Ctrl Pts',(-7.62034508045135,2.12468175842142,8.56381324124017));
#65861=CARTESIAN_POINT('Ctrl Pts',(-7.61833566936705,2.13187716354249,8.56351013942218));
#65862=CARTESIAN_POINT('Ctrl Pts',(-7.61720368449931,2.13591821948406,8.56333967710951));
#65863=CARTESIAN_POINT('Ctrl Pts',(-7.61420202700498,2.14660105771514,8.56288842810637));
#65864=CARTESIAN_POINT('Ctrl Pts',(-7.61232688358175,2.15324128371969,8.56260730836368));
#65865=CARTESIAN_POINT('Ctrl Pts',(-7.60015111553249,2.1961432186556,8.56078696564003));
#65866=CARTESIAN_POINT('Ctrl Pts',(-7.58960026718761,2.23233279484788,8.55923271180766));
#65867=CARTESIAN_POINT('Ctrl Pts',(-7.57802455891257,2.2710068109678,8.55755275284633));
#65868=CARTESIAN_POINT('Ctrl Pts',(-7.57725646716247,2.27356824875688,8.55744139715597));
#65869=CARTESIAN_POINT('Ctrl Pts',(-7.39494893255526,2.88041017289333,8.53103848636192));
#65870=CARTESIAN_POINT('Ctrl Pts',(-7.14178172006194,3.46076605949351,8.50098841716276));
#65871=CARTESIAN_POINT('Ctrl Pts',(-6.78930611493616,4.06122111193233,8.46861726726607));
#65872=CARTESIAN_POINT('Ctrl Pts',(-6.75551486324552,4.11718514032574,8.4655848389041));
#65873=CARTESIAN_POINT('Ctrl Pts',(-6.69032316780531,4.2221898212127,8.45987102659698));
#65874=CARTESIAN_POINT('Ctrl Pts',(-6.65906731570989,4.27131520287284,8.45718768349993));
#65875=CARTESIAN_POINT('Ctrl Pts',(-6.55894981573849,4.42490127654341,8.44877142898938));
#65876=CARTESIAN_POINT('Ctrl Pts',(-6.48814977801939,4.52807771686597,8.44307795031505));
#65877=CARTESIAN_POINT('Ctrl Pts',(-6.17375540666743,4.96371945335501,8.41892192422169));
#65878=CARTESIAN_POINT('Ctrl Pts',(-5.90681704168521,5.27857445365528,8.40121017526256));
#65879=CARTESIAN_POINT('Ctrl Pts',(-5.6038122881104,5.5840428638979,8.38382601181636));
#65880=CARTESIAN_POINT('Ctrl Pts',(-5.59105566449164,5.59681547208216,8.38309863132567));
#65881=CARTESIAN_POINT('Ctrl Pts',(-5.5725244527013,5.61524332025531,8.38204844792172));
#65882=CARTESIAN_POINT('Ctrl Pts',(-5.56678478686352,5.62093350422191,8.38172406678175));
#65883=CARTESIAN_POINT('Ctrl Pts',(-5.55675804883858,5.63084338008546,8.38115894861103));
#65884=CARTESIAN_POINT('Ctrl Pts',(-5.55247487036598,5.63506699148698,8.3809180353069));
#65885=CARTESIAN_POINT('Ctrl Pts',(-5.54419430983004,5.64321378516719,8.38045323002627));
#65886=CARTESIAN_POINT('Ctrl Pts',(-5.54019757168485,5.64713761450091,8.38022930906826));
#65887=CARTESIAN_POINT('Ctrl Pts',(-5.53071810214171,5.6564244091298,8.37969921575778));
#65888=CARTESIAN_POINT('Ctrl Pts',(-5.52523172734549,5.66178365721794,8.37939320963027));
#65889=CARTESIAN_POINT('Ctrl Pts',(-5.50596437987271,5.68054987733145,8.37832133040583));
#65890=CARTESIAN_POINT('Ctrl Pts',(-5.49214228102466,5.69391463169782,8.37755733713394));
#65891=CARTESIAN_POINT('Ctrl Pts',(-5.32278698876308,5.85647588315636,8.36825642986655));
#65892=CARTESIAN_POINT('Ctrl Pts',(-5.1612628419349,5.99931208686304,8.36000377675366));
#65893=CARTESIAN_POINT('Ctrl Pts',(-4.66516204581226,6.40312992346567,8.3362209467074));
#65894=CARTESIAN_POINT('Ctrl Pts',(-4.31521484457735,6.64400151538207,8.32145224818872));
#65895=CARTESIAN_POINT('Ctrl Pts',(-3.75707114934672,6.96539253531888,8.29926001363458));
#65896=CARTESIAN_POINT('Ctrl Pts',(-3.5620160801797,7.0671292925896,8.29172391110682));
#65897=CARTESIAN_POINT('Ctrl Pts',(-3.11522632764545,7.27696407111459,8.27450682254273));
#65898=CARTESIAN_POINT('Ctrl Pts',(-2.8616145661547,7.38037851881212,8.26476429999101));
#65899=CARTESIAN_POINT('Ctrl Pts',(-2.49138092852051,7.50939121013662,8.24996743660681));
#65900=CARTESIAN_POINT('Ctrl Pts',(-2.37873420362238,7.54583057561246,8.24538864031097));
#65901=CARTESIAN_POINT('Ctrl Pts',(-2.24400670352834,7.58609578229227,8.23978811780086));
#65902=CARTESIAN_POINT('Ctrl Pts',(-2.22267818384232,7.59237228928891,8.23889815169648));
#65903=CARTESIAN_POINT('Ctrl Pts',(-2.19434584367898,7.60058024723546,8.23771173906431));
#65904=CARTESIAN_POINT('Ctrl Pts',(-2.18736526461459,7.60259212209678,8.23741909063928));
#65905=CARTESIAN_POINT('Ctrl Pts',(-2.1758968110581,7.60588034600524,8.23693775216939));
#65906=CARTESIAN_POINT('Ctrl Pts',(-2.17141055071119,7.607162348093,8.23674932434889));
#65907=CARTESIAN_POINT('Ctrl Pts',(-2.16271412783194,7.60963913430154,8.23638380382866));
#65908=CARTESIAN_POINT('Ctrl Pts',(-2.15850410188849,7.61083439545462,8.23620673307318));
#65909=CARTESIAN_POINT('Ctrl Pts',(-2.14878100683365,7.61358614591791,8.23579751593458));
#65910=CARTESIAN_POINT('Ctrl Pts',(-2.14326723885183,7.61514014048698,8.23556525656888));
#65911=CARTESIAN_POINT('Ctrl Pts',(-2.12847429791216,7.61929202848718,8.23494159587623));
#65912=CARTESIAN_POINT('Ctrl Pts',(-2.11919207693431,7.62187895417693,8.23454970477561));
#65913=CARTESIAN_POINT('Ctrl Pts',(-2.0540618783678,7.63990236087384,8.23179612460157));
#65914=CARTESIAN_POINT('Ctrl Pts',(-1.99805144706895,7.65474156724469,8.22940847016318));
#65915=CARTESIAN_POINT('Ctrl Pts',(-1.35206344752239,7.81831435710219,8.2016817481281));
#65916=CARTESIAN_POINT('Ctrl Pts',(-0.746993376766655,7.89912069534865,
8.17408137396201));
#65917=CARTESIAN_POINT('Ctrl Pts',(0.163515756134235,7.91508183977154,8.13400391078272));
#65918=CARTESIAN_POINT('Ctrl Pts',(0.465755618220304,7.90305921801159,8.12090484267445));
#65919=CARTESIAN_POINT('Ctrl Pts',(0.91591458075945,7.85923240971991,8.10182484749996));
#65920=CARTESIAN_POINT('Ctrl Pts',(1.06480982682816,7.8404474255024,8.09558244888485));
#65921=CARTESIAN_POINT('Ctrl Pts',(1.29560376783461,7.80463357671714,8.08600515604046));
#65922=CARTESIAN_POINT('Ctrl Pts',(1.37791608591314,7.79052257714193,8.08260896460322));
#65923=CARTESIAN_POINT('Ctrl Pts',(1.47869669300443,7.77159824890433,8.07847200904348));
#65924=CARTESIAN_POINT('Ctrl Pts',(1.49739000352375,7.76801817930019,8.07770556191647));
#65925=CARTESIAN_POINT('Ctrl Pts',(1.52494814395747,7.76263717945895,8.07657692017905));
#65926=CARTESIAN_POINT('Ctrl Pts',(1.53382305243678,7.76088845854323,8.07621364400052));
#65927=CARTESIAN_POINT('Ctrl Pts',(1.55102784302016,7.75746774483151,8.07550977210399));
#65928=CARTESIAN_POINT('Ctrl Pts',(1.55935806730456,7.75579754765237,8.0751691397102));
#65929=CARTESIAN_POINT('Ctrl Pts',(1.5764696628885,7.75233801609144,8.07446976777318));
#65930=CARTESIAN_POINT('Ctrl Pts',(1.58525072100077,7.75054717202455,8.07411106014527));
#65931=CARTESIAN_POINT('Ctrl Pts',(1.60627968801366,7.74622120787136,8.07325246477966));
#65932=CARTESIAN_POINT('Ctrl Pts',(1.61852467619761,7.74367195270736,8.07275287096891));
#65933=CARTESIAN_POINT('Ctrl Pts',(1.65576251266275,7.73582731078088,8.07123465667474));
#65934=CARTESIAN_POINT('Ctrl Pts',(1.68073587378208,7.73043987192592,8.07021796221002));
#65935=CARTESIAN_POINT('Ctrl Pts',(1.96176477363138,7.66838803904843,8.0587933920971));
#65936=CARTESIAN_POINT('Ctrl Pts',(2.21488403218841,7.59914437091114,8.04866522825797));
#65937=CARTESIAN_POINT('Ctrl Pts',(2.83684592915637,7.39527472089752,8.0239755458874));
#65938=CARTESIAN_POINT('Ctrl Pts',(3.19999003836993,7.24554065522871,8.00975853284183));
#65939=CARTESIAN_POINT('Ctrl Pts',(3.83226704636499,6.92799005811155,7.98417475481596));
#65940=CARTESIAN_POINT('Ctrl Pts',(4.10528376745843,6.76978218201824,7.97280843355973));
#65941=CARTESIAN_POINT('Ctrl Pts',(4.524343642968,6.49225265196611,7.95399458963835));
#65942=CARTESIAN_POINT('Ctrl Pts',(4.67683302577009,6.38327945724006,7.94683078210738));
#65943=CARTESIAN_POINT('Ctrl Pts',(4.85198578698879,6.24846290926921,7.93806446732156));
#65944=CARTESIAN_POINT('Ctrl Pts',(4.87853720774578,6.22775476960711,7.9367204309245));
#65945=CARTESIAN_POINT('Ctrl Pts',(4.91157533751003,6.20164654719234,7.93502801022562));
#65946=CARTESIAN_POINT('Ctrl Pts',(4.91818695243797,6.19640454557412,7.93468831109778));
#65947=CARTESIAN_POINT('Ctrl Pts',(4.92864675021852,6.1880842347254,7.9341492729188));
#65948=CARTESIAN_POINT('Ctrl Pts',(4.93250047685226,6.18501288035744,7.93395032399543));
#65949=CARTESIAN_POINT('Ctrl Pts',(4.93972326643218,6.17924539655191,7.93357678553511));
#65950=CARTESIAN_POINT('Ctrl Pts',(4.94309299961681,6.17655010639183,7.93340224365291));
#65951=CARTESIAN_POINT('Ctrl Pts',(4.95062267914803,6.17051736343863,7.93301162011654));
#65952=CARTESIAN_POINT('Ctrl Pts',(4.95478145807877,6.16717845909347,7.93279545518975));
#65953=CARTESIAN_POINT('Ctrl Pts',(4.96526805247362,6.15874177051359,7.93224932342807));
#65954=CARTESIAN_POINT('Ctrl Pts',(4.97159138449121,6.15363844677584,7.93191903472614));
#65955=CARTESIAN_POINT('Ctrl Pts',(5.00532151805875,6.12633019788134,7.93015192034964));
#65956=CARTESIAN_POINT('Ctrl Pts',(5.03258710438046,6.103952175792,7.92870484104854));
#65957=CARTESIAN_POINT('Ctrl Pts',(5.4392996066812,5.76556851714933,7.90682426751278));
#65958=CARTESIAN_POINT('Ctrl Pts',(5.78844946786801,5.41493286596525,7.8841274704591));
#65959=CARTESIAN_POINT('Ctrl Pts',(6.30597278406671,4.78756397113375,7.84663887023609));
#65960=CARTESIAN_POINT('Ctrl Pts',(6.4942248692803,4.52892029569258,7.83190454295929));
#65961=CARTESIAN_POINT('Ctrl Pts',(6.84390426293828,3.98166718509391,7.80276521183197));
#65962=CARTESIAN_POINT('Ctrl Pts',(7.00394690589092,3.69289314831301,7.78841660649541));
#65963=CARTESIAN_POINT('Ctrl Pts',(7.16839311585861,3.3467753782507,7.77250025044536));
#65964=CARTESIAN_POINT('Ctrl Pts',(7.19079270161591,3.29837320010106,7.77030188466864));
#65965=CARTESIAN_POINT('Ctrl Pts',(7.23367884508027,3.2031888997531,7.76603192031594));
#65966=CARTESIAN_POINT('Ctrl Pts',(7.25420521718807,3.15642765774219,7.76395900688133));
#65967=CARTESIAN_POINT('Ctrl Pts',(7.27897985240022,3.0984700137937,7.76141991328677));
#65968=CARTESIAN_POINT('Ctrl Pts',(7.28365711946097,3.08745900147985,7.76093886117387));
#65969=CARTESIAN_POINT('Ctrl Pts',(7.29097103463763,3.07013179145667,7.76018395424569));
#65970=CARTESIAN_POINT('Ctrl Pts',(7.29362448407297,3.0638227315688,7.75990951742222));
#65971=CARTESIAN_POINT('Ctrl Pts',(7.2983236661073,3.0526088689214,7.75942249718236));
#65972=CARTESIAN_POINT('Ctrl Pts',(7.30037264874885,3.04770543711758,7.75920980130275));
#65973=CARTESIAN_POINT('Ctrl Pts',(7.30473604574677,3.03723371905589,7.75875612642902));
#65974=CARTESIAN_POINT('Ctrl Pts',(7.30704903818827,3.0316648422801,7.75851519673983));
#65975=CARTESIAN_POINT('Ctrl Pts',(7.31368417655183,3.0156380443322,7.75782278194854));
#65976=CARTESIAN_POINT('Ctrl Pts',(7.31799026257383,3.00517346704651,7.7573718523875));
#65977=CARTESIAN_POINT('Ctrl Pts',(7.33673571501738,2.95933937591365,7.75540194126166));
#65978=CARTESIAN_POINT('Ctrl Pts',(7.35094133533399,2.92387448970292,7.75389103712112));
#65979=CARTESIAN_POINT('Ctrl Pts',(7.5620322506461,2.38561422750803,7.73115787573218));
#65980=CARTESIAN_POINT('Ctrl Pts',(7.70719697583827,1.86405079231759,7.7118797281732));
#65981=CARTESIAN_POINT('Ctrl Pts',(7.86646791400167,0.931407599437989,7.67940979006949));
#65982=CARTESIAN_POINT('Ctrl Pts',(7.90390263768989,0.526446351861149,7.66590036787826));
#65983=CARTESIAN_POINT('Ctrl Pts',(7.91262224721879,-0.0463581511342715,
7.64591947725558));
#65984=CARTESIAN_POINT('Ctrl Pts',(7.9098860977543,-0.213162061307259,7.63999209352008));
#65985=CARTESIAN_POINT('Ctrl Pts',(7.8936979611195,-0.550007916894117,7.62760144786612));
#65986=CARTESIAN_POINT('Ctrl Pts',(7.88001543409475,-0.719948806275036,
7.62113232594531));
#65987=CARTESIAN_POINT('Ctrl Pts',(7.85816077260593,-0.913129314617089,
7.61340312474966));
#65988=CARTESIAN_POINT('Ctrl Pts',(7.8553572149372,-0.936941233684731,7.61244386459863));
#65989=CARTESIAN_POINT('Ctrl Pts',(7.85169101467516,-0.966906306303083,
7.61122809659573));
#65990=CARTESIAN_POINT('Ctrl Pts',(7.85092928579957,-0.973071911035898,
7.61097748014946));
#65991=CARTESIAN_POINT('Ctrl Pts',(7.84970641544429,-0.982875188773056,
7.61057826058596));
#65992=CARTESIAN_POINT('Ctrl Pts',(7.84925000441222,-0.9865134634709,7.61042993651213));
#65993=CARTESIAN_POINT('Ctrl Pts',(7.84838296473613,-0.99338636503417,7.61014943560255));
#65994=CARTESIAN_POINT('Ctrl Pts',(7.84797286655356,-0.99662104993463,7.61001729077698));
#65995=CARTESIAN_POINT('Ctrl Pts',(7.8470405120942,-1.00393881580851,7.60971805183827));
#65996=CARTESIAN_POINT('Ctrl Pts',(7.84651706888449,-1.00802174179599,7.60955088788374));
#65997=CARTESIAN_POINT('Ctrl Pts',(7.84516621765225,-1.01849375181251,7.60912161983706));
#65998=CARTESIAN_POINT('Ctrl Pts',(7.84433419284816,-1.02488222518112,7.6088592463545));
#65999=CARTESIAN_POINT('Ctrl Pts',(7.83950938961043,-1.06157807558204,7.60734932592833));
#66000=CARTESIAN_POINT('Ctrl Pts',(7.83534882271064,-1.09186274666821,7.60609212004813));
#66001=CARTESIAN_POINT('Ctrl Pts',(7.76527231781697,-1.58090934348024,7.58562018664586));
#66002=CARTESIAN_POINT('Ctrl Pts',(7.65934622298113,-2.03299577745273,7.56432048276451));
#66003=CARTESIAN_POINT('Ctrl Pts',(7.42154091190563,-2.75554484602005,7.52911039680101));
#66004=CARTESIAN_POINT('Ctrl Pts',(7.31275807224921,-3.03247020277189,7.51530509923572));
#66005=CARTESIAN_POINT('Ctrl Pts',(7.07222674984201,-3.55602244542797,7.4891368304081));
#66006=CARTESIAN_POINT('Ctrl Pts',(6.94248527659778,-3.80310448702041,7.47675485164227));
#66007=CARTESIAN_POINT('Ctrl Pts',(6.72923071275136,-4.16179392610184,7.45888440052028));
#66008=CARTESIAN_POINT('Ctrl Pts',(6.65539287671006,-4.27888103919119,7.45306665618013));
#66009=CARTESIAN_POINT('Ctrl Pts',(6.53699824154604,-4.45613769102088,7.44428469662259));
#66010=CARTESIAN_POINT('Ctrl Pts',(6.49459830995342,-4.51770985548721,7.44123894550398));
#66011=CARTESIAN_POINT('Ctrl Pts',(6.44334450773971,-4.58992624971152,7.4376713101261));
#66012=CARTESIAN_POINT('Ctrl Pts',(6.43532833567487,-4.60115861907106,7.43711654157955));
#66013=CARTESIAN_POINT('Ctrl Pts',(6.4230807990294,-4.61822541587162,7.43627380038086));
#66014=CARTESIAN_POINT('Ctrl Pts',(6.41887080351395,-4.6240751022041,7.43598498299026));
#66015=CARTESIAN_POINT('Ctrl Pts',(6.41154961035063,-4.63421845718184,7.43548423097848));
#66016=CARTESIAN_POINT('Ctrl Pts',(6.40844208244668,-4.63851476131563,7.43527215109287));
#66017=CARTESIAN_POINT('Ctrl Pts',(6.40196972703011,-4.64744417953311,7.43483140140609));
#66018=CARTESIAN_POINT('Ctrl Pts',(6.39860418325591,-4.65207677214078,7.43460276023524));
#66019=CARTESIAN_POINT('Ctrl Pts',(6.38937233023096,-4.66475523205794,7.4339770697975));
#66020=CARTESIAN_POINT('Ctrl Pts',(6.38349584602102,-4.67279369693589,7.43358042561094));
#66021=CARTESIAN_POINT('Ctrl Pts',(6.36096424233352,-4.70349293709222,7.43206583789562));
#66022=CARTESIAN_POINT('Ctrl Pts',(6.34420341297114,-4.72607606557458,7.43095211592028));
#66023=CARTESIAN_POINT('Ctrl Pts',(6.07855565993108,-5.08004350379971,7.41350126157916));
#66024=CARTESIAN_POINT('Ctrl Pts',(5.80411864030804,-5.39146879504295,7.39827663107649));
#66025=CARTESIAN_POINT('Ctrl Pts',(5.14622568717159,-6.0292696252545,7.3660095330975));
#66026=CARTESIAN_POINT('Ctrl Pts',(4.75353722307944,-6.34346828974936,7.34935014834362));
#66027=CARTESIAN_POINT('Ctrl Pts',(4.13846064785114,-6.74622506733091,7.32352948275121));
#66028=CARTESIAN_POINT('Ctrl Pts',(3.93762125777047,-6.86538681493492,7.31512043375686));
#66029=CARTESIAN_POINT('Ctrl Pts',(3.63637664995337,-7.0265498410981,7.30212492202932));
#66030=CARTESIAN_POINT('Ctrl Pts',(3.5398987143048,-7.07564505802181,7.29790769161243));
#66031=CARTESIAN_POINT('Ctrl Pts',(3.43419631081239,-7.12673141724409,7.2931959927669));
#66032=CARTESIAN_POINT('Ctrl Pts',(3.42593774283983,-7.13070512472645,7.29282726863415));
#66033=CARTESIAN_POINT('Ctrl Pts',(3.41374762366139,-7.13654447892173,7.29228210394887));
#66034=CARTESIAN_POINT('Ctrl Pts',(3.40982138858437,-7.13842125651517,7.29210637706188));
#66035=CARTESIAN_POINT('Ctrl Pts',(3.40312566407425,-7.14161509178855,7.29180646271214));
#66036=CARTESIAN_POINT('Ctrl Pts',(3.40035694879235,-7.14293378280346,7.29168237874522));
#66037=CARTESIAN_POINT('Ctrl Pts',(3.39470754023777,-7.14562046893532,7.29142905501253));
#66038=CARTESIAN_POINT('Ctrl Pts',(3.39182678710229,-7.14698833188202,7.29129980708599));
#66039=CARTESIAN_POINT('Ctrl Pts',(3.38497603078409,-7.15023618955032,7.29099226938482));
#66040=CARTESIAN_POINT('Ctrl Pts',(3.3810052911652,-7.15211461851389,7.29081388182533));
#66041=CARTESIAN_POINT('Ctrl Pts',(3.36908528655124,-7.15774144359293,7.29027796368081));
#66042=CARTESIAN_POINT('Ctrl Pts',(3.36113136277975,-7.16147988912177,7.28991981779205));
#66043=CARTESIAN_POINT('Ctrl Pts',(3.28487925283945,-7.19716433657516,7.28648131511179));
#66044=CARTESIAN_POINT('Ctrl Pts',(3.21613584699936,-7.2281446943565,7.28334261282636));
#66045=CARTESIAN_POINT('Ctrl Pts',(2.75001866550971,-7.43024245417687,7.2618547921381));
#66046=CARTESIAN_POINT('Ctrl Pts',(2.33965115898892,-7.5694839270577,7.24197358517235));
#66047=CARTESIAN_POINT('Ctrl Pts',(1.42928893271001,-7.79723787145641,7.19864974593833));
#66048=CARTESIAN_POINT('Ctrl Pts',(0.927892356212872,-7.87266721608372,
7.17532035901489));
#66049=CARTESIAN_POINT('Ctrl Pts',(0.18230046849807,-7.91256240755643,7.14290499246501));
#66050=CARTESIAN_POINT('Ctrl Pts',(-0.0585698784159418,-7.91444629599931,
7.13276054190036));
#66051=CARTESIAN_POINT('Ctrl Pts',(-0.324829722659474,-7.90437006971546,
7.12191139033257));
#66052=CARTESIAN_POINT('Ctrl Pts',(-0.350488286076147,-7.90327391181675,
7.12086957961653));
#66053=CARTESIAN_POINT('Ctrl Pts',(-0.395192057562846,-7.90114599248355,
7.11906082405882));
#66054=CARTESIAN_POINT('Ctrl Pts',(-0.414239641911428,-7.90017026921181,
7.11829214960519));
#66055=CARTESIAN_POINT('Ctrl Pts',(-0.441769593808843,-7.89866019365127,
7.11718403722202));
#66056=CARTESIAN_POINT('Ctrl Pts',(-0.450254850499073,-7.89818104369389,
7.11684289036724));
#66057=CARTESIAN_POINT('Ctrl Pts',(-0.464962902089955,-7.89732672257769,
7.11625223849874));
#66058=CARTESIAN_POINT('Ctrl Pts',(-0.471186047924912,-7.89695786818719,
7.1160025380797));
#66059=CARTESIAN_POINT('Ctrl Pts',(-0.483138517865475,-7.8962352499575,
7.11552335556403));
#66060=CARTESIAN_POINT('Ctrl Pts',(-0.488867903856261,-7.89588260569163,
7.11529383898065));
#66061=CARTESIAN_POINT('Ctrl Pts',(-0.502343938871402,-7.89503843049926,
7.11475441303453));
#66062=CARTESIAN_POINT('Ctrl Pts',(-0.510090265005628,-7.89454173299364,
7.11444466379778));
#66063=CARTESIAN_POINT('Ctrl Pts',(-0.536763249935253,-7.89279202824524,
7.11337921440185));
#66064=CARTESIAN_POINT('Ctrl Pts',(-0.555686193364753,-7.89148234797809,
7.1126252691143));
#66065=CARTESIAN_POINT('Ctrl Pts',(-0.762587658718213,-7.87641455317025,
7.10440250932966));
#66066=CARTESIAN_POINT('Ctrl Pts',(-0.950027801780292,-7.8560103739309,
7.0971431839287));
#66067=CARTESIAN_POINT('Ctrl Pts',(-1.29009060629585,-7.80664159572602,
7.08424311733428));
#66068=CARTESIAN_POINT('Ctrl Pts',(-1.44292741037141,-7.77984252840712,
7.07854569161725));
#66069=CARTESIAN_POINT('Ctrl Pts',(-2.20016694196386,-7.62398048251643,
7.05063645513779));
#66070=CARTESIAN_POINT('Ctrl Pts',(-2.78872370337274,-7.42891439450698,
7.03015134615013));
#66071=CARTESIAN_POINT('Ctrl Pts',(-3.44521394135837,-7.12220490875548,
7.004144308134));
#66072=CARTESIAN_POINT('Ctrl Pts',(-3.54094160453842,-7.07509953283296,
7.00026228163398));
#66073=CARTESIAN_POINT('Ctrl Pts',(-3.74785418237849,-6.96803134782176,
6.99161641703096));
#66074=CARTESIAN_POINT('Ctrl Pts',(-3.85861301536865,-6.90731315259118,
6.98682298630535));
#66075=CARTESIAN_POINT('Ctrl Pts',(-4.01474589726591,-6.81679343589915,
6.9797623386975));
#66076=CARTESIAN_POINT('Ctrl Pts',(-4.06134383345277,-6.78913421493755,
6.97761542655229));
#66077=CARTESIAN_POINT('Ctrl Pts',(-4.11472255728099,-6.75670390827992,
6.97510596640457));
#66078=CARTESIAN_POINT('Ctrl Pts',(-4.12178539476263,-6.75239769164559,
6.97477290566087));
#66079=CARTESIAN_POINT('Ctrl Pts',(-4.13247418609869,-6.74585770962509,
6.97426729047583));
#66080=CARTESIAN_POINT('Ctrl Pts',(-4.13610512939409,-6.74363207001609,
6.97409526055397));
#66081=CARTESIAN_POINT('Ctrl Pts',(-4.1426642050995,-6.73960429887846,6.97378399993207));
#66082=CARTESIAN_POINT('Ctrl Pts',(-4.14559295448717,-6.73780319372323,
6.9736448360087));
#66083=CARTESIAN_POINT('Ctrl Pts',(-4.15189385609066,-6.73392263863843,
6.97334505037147));
#66084=CARTESIAN_POINT('Ctrl Pts',(-4.15526560547604,-6.73184257415849,
6.97318438892134));
#66085=CARTESIAN_POINT('Ctrl Pts',(-4.16435200880427,-6.72622765740883,
6.97275078507602));
#66086=CARTESIAN_POINT('Ctrl Pts',(-4.1700637133671,-6.72268806196385,6.97247753546295));
#66087=CARTESIAN_POINT('Ctrl Pts',(-4.19638147682942,-6.70633225887918,
6.97121534363996));
#66088=CARTESIAN_POINT('Ctrl Pts',(-4.21693281919563,-6.69342867598355,
6.97022081350512));
#66089=CARTESIAN_POINT('Ctrl Pts',(-4.54489276868713,-6.4854023565472,6.95421158154743));
#66090=CARTESIAN_POINT('Ctrl Pts',(-4.83850588341102,-6.26939466798868,
6.93794134598426));
#66091=CARTESIAN_POINT('Ctrl Pts',(-5.56255141416055,-5.65547924242552,
6.89467056812326));
#66092=CARTESIAN_POINT('Ctrl Pts',(-5.96560570703009,-5.22858421540378,
6.86742087018337));
#66093=CARTESIAN_POINT('Ctrl Pts',(-6.4863507765081,-4.53756879106466,6.82978984664789));
#66094=CARTESIAN_POINT('Ctrl Pts',(-6.64284250436611,-4.30522253935676,
6.81801894587401));
#66095=CARTESIAN_POINT('Ctrl Pts',(-6.79586806638635,-4.04974278978103,
6.80599024775713));
#66096=CARTESIAN_POINT('Ctrl Pts',(-6.80498582709915,-4.03440297162688,
6.80527134013262));
#66097=CARTESIAN_POINT('Ctrl Pts',(-6.81821431821871,-4.01197478160315,
6.80422506498984));
#66098=CARTESIAN_POINT('Ctrl Pts',(-6.8223660321924,-4.00491071819191,6.80389622317893));
#66099=CARTESIAN_POINT('Ctrl Pts',(-6.82963139472718,-3.99250475796903,
6.80331992733872));
#66100=CARTESIAN_POINT('Ctrl Pts',(-6.83274976585024,-3.98716564337876,
6.80307230379194));
#66101=CARTESIAN_POINT('Ctrl Pts',(-6.83879076757475,-3.97679465131281,
6.80259207107961));
#66102=CARTESIAN_POINT('Ctrl Pts',(-6.84171411123687,-3.97176319556593,
6.80235943643488));
#66103=CARTESIAN_POINT('Ctrl Pts',(-6.84867647494627,-3.95974956351787,
6.80180480380491));
#66104=CARTESIAN_POINT('Ctrl Pts',(-6.8527103767237,-3.95276441968311,6.80148298924659));
#66105=CARTESIAN_POINT('Ctrl Pts',(-6.86485964847448,-3.93165212620949,
6.80051232926105));
#66106=CARTESIAN_POINT('Ctrl Pts',(-6.87294209043584,-3.91750602556343,
6.79986466113227));
#66107=CARTESIAN_POINT('Ctrl Pts',(-6.95369601770744,-3.77514924013578,
6.79337402167086));
#66108=CARTESIAN_POINT('Ctrl Pts',(-7.02281711840131,-3.64495303543774,
6.78765862509866));
#66109=CARTESIAN_POINT('Ctrl Pts',(-7.11824231190146,-3.45240573578784,
6.77949794533659));
#66110=CARTESIAN_POINT('Ctrl Pts',(-7.14744630711651,-3.39153217702231,
6.77695922614847));
#66111=CARTESIAN_POINT('Ctrl Pts',(-7.46176102839755,-2.71426984332509,
6.74914170098844));
#66112=CARTESIAN_POINT('Ctrl Pts',(-7.6671252487402,-2.06404914908849,6.72663812453134));
#66113=CARTESIAN_POINT('Ctrl Pts',(-7.82376566730491,-1.19004905646277,
6.69562366334662));
#66114=CARTESIAN_POINT('Ctrl Pts',(-7.85244955238754,-0.983135444346683,
6.68820075373254));
#66115=CARTESIAN_POINT('Ctrl Pts',(-7.88874576839007,-0.61457782966774,
6.67449659629814));
#66116=CARTESIAN_POINT('Ctrl Pts',(-7.89964926935827,-0.453378014245832,
6.66833997739062));
#66117=CARTESIAN_POINT('Ctrl Pts',(-7.90648316265765,-0.268335920070195,
6.66097868722274));
#66118=CARTESIAN_POINT('Ctrl Pts',(-7.90724991391673,-0.244701745842623,
6.66003298460298));
#66119=CARTESIAN_POINT('Ctrl Pts',(-7.90808784598529,-0.214727302504374,
6.65882623507));
#66120=CARTESIAN_POINT('Ctrl Pts',(-7.90825738900562,-0.208389690394877,
6.65857067098738));
#66121=CARTESIAN_POINT('Ctrl Pts',(-7.90851595994916,-0.198269085449415,
6.65816188371518));
#66122=CARTESIAN_POINT('Ctrl Pts',(-7.90860989258907,-0.194486209701014,
6.65800893699114));
#66123=CARTESIAN_POINT('Ctrl Pts',(-7.90878219758714,-0.187340507902215,
6.65771974035148));
#66124=CARTESIAN_POINT('Ctrl Pts',(-7.90886113940516,-0.183977695150078,
6.65758352277971));
#66125=CARTESIAN_POINT('Ctrl Pts',(-7.90903436488574,-0.17639232957355,
6.65727598997111));
#66126=CARTESIAN_POINT('Ctrl Pts',(-7.90912741173672,-0.172169752447682,
6.65710460418133));
#66127=CARTESIAN_POINT('Ctrl Pts',(-7.90939154332332,-0.159730871858649,
6.65659917005622));
#66128=CARTESIAN_POINT('Ctrl Pts',(-7.90955320593334,-0.151514415141959,
6.65626457951751));
#66129=CARTESIAN_POINT('Ctrl Pts',(-7.91055658713074,-0.0961301159729605,
6.65400438583313));
#66130=CARTESIAN_POINT('Ctrl Pts',(-7.91098916588274,-0.0489566925479483,
6.65205564367597));
#66131=CARTESIAN_POINT('Ctrl Pts',(-7.91102344790239,0.103134037520468,
6.64570318947202));
#66132=CARTESIAN_POINT('Ctrl Pts',(-7.90895994131844,0.208037490304112,
6.64121498214525));
#66133=CARTESIAN_POINT('Ctrl Pts',(-7.89734454701748,0.50151101491396,6.62842160014599));
#66134=CARTESIAN_POINT('Ctrl Pts',(-7.88312778758773,0.689821860973479,
6.61993882411635));
#66135=CARTESIAN_POINT('Ctrl Pts',(-7.76369551942669,1.75998621118394,6.57083169253472));
#66136=CARTESIAN_POINT('Ctrl Pts',(-7.51724645926729,2.61997199051387,6.52885975577479));
#66137=CARTESIAN_POINT('Ctrl Pts',(-7.10957271997544,3.46999187554645,6.49027534514519));
#66138=CARTESIAN_POINT('Ctrl Pts',(-7.08559408268638,3.51869642489519,6.48807148846915));
#66139=CARTESIAN_POINT('Ctrl Pts',(-7.05590584847955,3.57746378792904,6.4854203244357));
#66140=CARTESIAN_POINT('Ctrl Pts',(-7.05067339831071,3.58776519973336,6.48495589902699));
#66141=CARTESIAN_POINT('Ctrl Pts',(-7.04204949574865,3.60465182299889,6.48419507458754));
#66142=CARTESIAN_POINT('Ctrl Pts',(-7.03867133844764,3.61124378231878,6.48389819673668));
#66143=CARTESIAN_POINT('Ctrl Pts',(-7.03259413603216,3.623061593723,6.48336618210451));
#66144=CARTESIAN_POINT('Ctrl Pts',(-7.02989851402985,3.62828919419385,6.48313092197821));
#66145=CARTESIAN_POINT('Ctrl Pts',(-7.02416628167898,3.63937530219927,6.4826321689708));
#66146=CARTESIAN_POINT('Ctrl Pts',(-7.02112816522473,3.64523302831263,6.48236873079233));
#66147=CARTESIAN_POINT('Ctrl Pts',(-7.01299910361643,3.66085862898465,6.48166625555504));
#66148=CARTESIAN_POINT('Ctrl Pts',(-7.00789507253669,3.67061970004345,6.4812276926898));
#66149=CARTESIAN_POINT('Ctrl Pts',(-6.98384590010682,3.71637891289789,6.47917295105448));
#66150=CARTESIAN_POINT('Ctrl Pts',(-6.96464350685349,3.75224155238918,6.4775661239629));
#66151=CARTESIAN_POINT('Ctrl Pts',(-6.8177594581398,4.02155151523423,6.46552419682136));
#66152=CARTESIAN_POINT('Ctrl Pts',(-6.6786449454492,4.24858063965722,6.45552117709732));
#66153=CARTESIAN_POINT('Ctrl Pts',(-6.24096730423131,4.88806012939086,6.42737479122158));
#66154=CARTESIAN_POINT('Ctrl Pts',(-5.91374514936757,5.2792452545901,6.41026666768018));
#66155=CARTESIAN_POINT('Ctrl Pts',(-5.23416753709721,5.94856819957873,6.37746628043565));
#66156=CARTESIAN_POINT('Ctrl Pts',(-4.8913456869406,6.23350829206073,6.3618823575361));
#66157=CARTESIAN_POINT('Ctrl Pts',(-4.50322756710697,6.50428039620954,6.34312301587694));
#66158=CARTESIAN_POINT('Ctrl Pts',(-4.47992979496336,6.52034899275809,6.34199284329726));
#66159=CARTESIAN_POINT('Ctrl Pts',(-4.45136932705794,6.53982196841356,6.34060174153448));
#66160=CARTESIAN_POINT('Ctrl Pts',(-4.4461878927256,6.54334574102412,6.34034914273798));
#66161=CARTESIAN_POINT('Ctrl Pts',(-4.43764100856011,6.5491434383596,6.3399320949884));
#66162=CARTESIAN_POINT('Ctrl Pts',(-4.43427797698291,6.5514209389849,6.33976789787987));
#66163=CARTESIAN_POINT('Ctrl Pts',(-4.42821645607803,6.55551909575341,6.33947177189199));
#66164=CARTESIAN_POINT('Ctrl Pts',(-4.42551859195046,6.55734067964341,6.33933990877247));
#66165=CARTESIAN_POINT('Ctrl Pts',(-4.41974936168588,6.56123085192514,6.33905779005097));
#66166=CARTESIAN_POINT('Ctrl Pts',(-4.41667767387697,6.56329894468278,6.33890749967426));
#66167=CARTESIAN_POINT('Ctrl Pts',(-4.40831325910088,6.56892197093703,6.33849802512201));
#66168=CARTESIAN_POINT('Ctrl Pts',(-4.40301769180088,6.57247265919341,6.33823854066548));
#66169=CARTESIAN_POINT('Ctrl Pts',(-4.37620879031418,6.59040113868457,6.33692369092501));
#66170=CARTESIAN_POINT('Ctrl Pts',(-4.3546295283039,6.60467956723946,6.33586140936924));
#66171=CARTESIAN_POINT('Ctrl Pts',(-4.1636277665221,6.72971741569367,6.32642738100648));
#66172=CARTESIAN_POINT('Ctrl Pts',(-3.99009346743656,6.83403505707336,6.31763871742243));
#66173=CARTESIAN_POINT('Ctrl Pts',(-3.63802423351111,7.02769330109621,6.29968584484765));
#66174=CARTESIAN_POINT('Ctrl Pts',(-3.45971831647988,7.11716494505054,6.29053561573333));
#66175=CARTESIAN_POINT('Ctrl Pts',(-2.74278111754678,7.44360245588153,6.25402064440536));
#66176=CARTESIAN_POINT('Ctrl Pts',(-2.18173738972459,7.62694020339394,6.22621450780322));
#66177=CARTESIAN_POINT('Ctrl Pts',(-1.49565644334698,7.76913922536113,6.19533442674687));
#66178=CARTESIAN_POINT('Ctrl Pts',(-1.38530506027283,7.78957275603625,6.19045365597572));
#66179=CARTESIAN_POINT('Ctrl Pts',(-1.07332300422859,7.84050198934743,6.17690545029293));
#66180=CARTESIAN_POINT('Ctrl Pts',(-0.870889506981382,7.86556124031206,
6.16840922762043));
#66181=CARTESIAN_POINT('Ctrl Pts',(-0.648794529560549,7.88437357916863,
6.1593983861036));
#66182=CARTESIAN_POINT('Ctrl Pts',(-0.629880743417078,7.8859071344546,6.15863344098221));
#66183=CARTESIAN_POINT('Ctrl Pts',(-0.603358397050679,7.88796157440263,
6.15756414342877));
#66184=CARTESIAN_POINT('Ctrl Pts',(-0.595754399091126,7.88853952585184,
6.15725796185806));
#66185=CARTESIAN_POINT('Ctrl Pts',(-0.582575416170867,7.88952204688443,
6.15672796766475));
#66186=CARTESIAN_POINT('Ctrl Pts',(-0.577000822407313,7.88993170407207,
6.15650399215719));
#66187=CARTESIAN_POINT('Ctrl Pts',(-0.565418769516555,7.89077048764221,
6.15603907891336));
#66188=CARTESIAN_POINT('Ctrl Pts',(-0.559411243757319,7.89119866269632,
6.15579817177235));
#66189=CARTESIAN_POINT('Ctrl Pts',(-0.545296992296478,7.89218843061656,
6.15523273932184));
#66190=CARTESIAN_POINT('Ctrl Pts',(-0.537189871659079,7.89274439447207,
6.15490839431645));
#66191=CARTESIAN_POINT('Ctrl Pts',(-0.511234745258356,7.89448414951912,
6.15387138250419));
#66192=CARTESIAN_POINT('Ctrl Pts',(-0.493383516506788,7.89561990364859,
6.15316025162415));
#66193=CARTESIAN_POINT('Ctrl Pts',(-0.451659946713336,7.89813244171489,
6.15150297207179));
#66194=CARTESIAN_POINT('Ctrl Pts',(-0.427784855312348,7.89946155790637,
6.15055834497181));
#66195=CARTESIAN_POINT('Ctrl Pts',(-0.185309265694481,7.91185755709024,
6.14100162603336));
#66196=CARTESIAN_POINT('Ctrl Pts',(0.033662794855598,7.91395634601143,6.13267970517584));
#66197=CARTESIAN_POINT('Ctrl Pts',(0.749017906919613,7.89111670623702,6.10625032271572));
#66198=CARTESIAN_POINT('Ctrl Pts',(1.24300245222186,7.82851947334889,6.08926480322795));
#66199=CARTESIAN_POINT('Ctrl Pts',(2.0430668001165,7.64945351220834,6.06101556156691));
#66200=CARTESIAN_POINT('Ctrl Pts',(2.35365483102663,7.55966607977866,6.04982963553433));
#66201=CARTESIAN_POINT('Ctrl Pts',(2.84775816177783,7.3834165937122,6.03057518549417));
#66202=CARTESIAN_POINT('Ctrl Pts',(3.03498640570151,7.30844897378979,6.02291021662726));
#66203=CARTESIAN_POINT('Ctrl Pts',(3.23225750486438,7.22057049262203,6.01426989212432));
#66204=CARTESIAN_POINT('Ctrl Pts',(3.24534636538813,7.214697067876,6.01369409370674));
#66205=CARTESIAN_POINT('Ctrl Pts',(3.26356614932882,7.20646160702582,6.01288913612258));
#66206=CARTESIAN_POINT('Ctrl Pts',(3.26871068462162,7.204129604927,6.01266146508798));
#66207=CARTESIAN_POINT('Ctrl Pts',(3.27758437254653,7.20009572740804,6.012268104008));
#66208=CARTESIAN_POINT('Ctrl Pts',(3.2813147124833,7.19839645758281,6.01210254152987));
#66209=CARTESIAN_POINT('Ctrl Pts',(3.28862764790719,7.19505835377466,6.01177758276833));
#66210=CARTESIAN_POINT('Ctrl Pts',(3.29221034410869,7.19341974104402,6.01161819723236));
#66211=CARTESIAN_POINT('Ctrl Pts',(3.30087138391499,7.18945062767021,6.01123244506941));
#66212=CARTESIAN_POINT('Ctrl Pts',(3.30594848193471,7.18711742323972,6.0110059484111));
#66213=CARTESIAN_POINT('Ctrl Pts',(3.32151743922212,7.17994264747415,6.01031027133182));
#66214=CARTESIAN_POINT('Ctrl Pts',(3.33200113533262,7.17508348050341,6.009840255225));
#66215=CARTESIAN_POINT('Ctrl Pts',(3.44323285405106,7.12323150033678,6.0048370101673));
#66216=CARTESIAN_POINT('Ctrl Pts',(3.5429872951274,7.07414439760871,6.00020718659184));
#66217=CARTESIAN_POINT('Ctrl Pts',(3.8322530047261,6.92414945003292,5.98642274432849));
#66218=CARTESIAN_POINT('Ctrl Pts',(4.01872728951156,6.81761198786974,5.97707687422037));
#66219=CARTESIAN_POINT('Ctrl Pts',(4.90514703219556,6.26216319322926,5.93102501476368));
#66220=CARTESIAN_POINT('Ctrl Pts',(5.53581723435538,5.71229141104296,5.89385793602659));
#66221=CARTESIAN_POINT('Ctrl Pts',(6.10098617330596,5.03630194739823,5.85800112057454));
#66222=CARTESIAN_POINT('Ctrl Pts',(6.1323690200035,4.9980416036641,5.85599719808608));
#66223=CARTESIAN_POINT('Ctrl Pts',(6.17374451740898,4.94662232028513,5.85333715379805));
#66224=CARTESIAN_POINT('Ctrl Pts',(6.18405766507667,4.93372319284318,5.85267259218814));
#66225=CARTESIAN_POINT('Ctrl Pts',(6.20009105885904,4.91354023419417,5.85163700123266));
#66226=CARTESIAN_POINT('Ctrl Pts',(6.20583901581246,4.90627851650074,5.85126525198408));
#66227=CARTESIAN_POINT('Ctrl Pts',(6.21724995299581,4.89181030133763,5.850526262223));
#66228=CARTESIAN_POINT('Ctrl Pts',(6.22291319113226,4.8846040185932,5.8501590147725));
#66229=CARTESIAN_POINT('Ctrl Pts',(6.23548452618911,4.86855006404709,5.84934270250191));
#66230=CARTESIAN_POINT('Ctrl Pts',(6.24238634706428,4.85969749031077,5.84889379989512));
#66231=CARTESIAN_POINT('Ctrl Pts',(6.25667198856353,4.84129346118173,5.84796310739756));
#66232=CARTESIAN_POINT('Ctrl Pts',(6.26405283568117,4.83173973043217,5.84748139482729));
#66233=CARTESIAN_POINT('Ctrl Pts',(6.28299112466769,4.80710977533512,5.84624315873157));
#66234=CARTESIAN_POINT('Ctrl Pts',(6.2945162046897,4.79200872473228,5.84548747163797));
#66235=CARTESIAN_POINT('Ctrl Pts',(6.32780741229175,4.74806068336325,5.84329830717785));
#66236=CARTESIAN_POINT('Ctrl Pts',(6.34943049754676,4.7191057718518,5.84186853036351));
#66237=CARTESIAN_POINT('Ctrl Pts',(6.49042612227705,4.52757870647068,5.83249240352917));
#66238=CARTESIAN_POINT('Ctrl Pts',(6.60374530757276,4.36063674694733,5.82470569087755));
#66239=CARTESIAN_POINT('Ctrl Pts',(6.81375538505173,4.02425478886288,5.80967662482413));
#66240=CARTESIAN_POINT('Ctrl Pts',(6.91080692907022,3.85520943798788,5.80242975799392));
#66241=CARTESIAN_POINT('Ctrl Pts',(7.33824612423678,3.04257640137642,5.76869844499615));
#66242=CARTESIAN_POINT('Ctrl Pts',(7.58554213421754,2.35933032892604,5.74381727703515));
#66243=CARTESIAN_POINT('Ctrl Pts',(7.74404968218386,1.61706515113415,5.71375224029246));
#66244=CARTESIAN_POINT('Ctrl Pts',(7.75129517153371,1.58196974985342,5.71232312961162));
#66245=CARTESIAN_POINT('Ctrl Pts',(7.75989868319961,1.53881776691502,5.71055547441325));
#66246=CARTESIAN_POINT('Ctrl Pts',(7.76148307976106,1.53080635457468,5.7102268566353));
#66247=CARTESIAN_POINT('Ctrl Pts',(7.76408345169298,1.51754989963186,5.70968234354736));
#66248=CARTESIAN_POINT('Ctrl Pts',(7.7651065261497,1.51230624544787,5.70946676469407));
#66249=CARTESIAN_POINT('Ctrl Pts',(7.76686435049282,1.50324790131082,5.70909401439142));
#66250=CARTESIAN_POINT('Ctrl Pts',(7.76760160436761,1.49943369559405,5.70893695579678));
#66251=CARTESIAN_POINT('Ctrl Pts',(7.76923991502855,1.49092421011634,5.70858632310695));
#66252=CARTESIAN_POINT('Ctrl Pts',(7.77013952521912,1.48622865538102,5.70839268341547));
#66253=CARTESIAN_POINT('Ctrl Pts',(7.7724920410848,1.47388907770682,5.70788338675628));
#66254=CARTESIAN_POINT('Ctrl Pts',(7.77393792435386,1.46624373476725,5.70756740831289));
#66255=CARTESIAN_POINT('Ctrl Pts',(7.78030083328137,1.43232483101939,5.70616361034092));
#66256=CARTESIAN_POINT('Ctrl Pts',(7.78509591580113,1.40602881614237,5.70507012487186));
#66257=CARTESIAN_POINT('Ctrl Pts',(7.81772317784502,1.22181720806596,5.69737093919074));
#66258=CARTESIAN_POINT('Ctrl Pts',(7.84087851624784,1.06313023775982,5.69052266048115));
#66259=CARTESIAN_POINT('Ctrl Pts',(7.87075959753136,0.803311390275426,5.67906787879977));
#66260=CARTESIAN_POINT('Ctrl Pts',(7.88039290012531,0.702547185654779,5.67456737271057));
#66261=CARTESIAN_POINT('Ctrl Pts',(7.92853959033575,0.0712849214034552,
5.64611904344095));
#66262=CARTESIAN_POINT('Ctrl Pts',(7.91540312773242,-0.461788922677369,
5.62108359128015));
#66263=CARTESIAN_POINT('Ctrl Pts',(7.79398026758889,-1.42490740654869,5.57730803467653));
#66264=CARTESIAN_POINT('Ctrl Pts',(7.70295655714242,-1.85500137982462,5.55829215853666));
#66265=CARTESIAN_POINT('Ctrl Pts',(7.56818997241208,-2.30375778674544,5.53926796679553));
#66266=CARTESIAN_POINT('Ctrl Pts',(7.5595060046451,-2.33209527885939,5.53806992817338));
#66267=CARTESIAN_POINT('Ctrl Pts',(7.547612705697,-2.37014091472058,5.53646578947383));
#66268=CARTESIAN_POINT('Ctrl Pts',(7.54454356268742,-2.37989242248096,5.53605501548854));
#66269=CARTESIAN_POINT('Ctrl Pts',(7.53970050021364,-2.39517663730959,5.53541177923968));
#66270=CARTESIAN_POINT('Ctrl Pts',(7.53793937862533,-2.40071336922869,5.53517888914768));
#66271=CARTESIAN_POINT('Ctrl Pts',(7.53454859079476,-2.41133303897929,5.53473243237383));
#66272=CARTESIAN_POINT('Ctrl Pts',(7.5329198769411,-2.41641627615211,5.53451883394969));
#66273=CARTESIAN_POINT('Ctrl Pts',(7.52908470320697,-2.42834434377707,5.53401785705166));
#66274=CARTESIAN_POINT('Ctrl Pts',(7.52687405021886,-2.43518782694959,5.53373061937226));
#66275=CARTESIAN_POINT('Ctrl Pts',(7.52055205146019,-2.45466788526552,5.53291352475275));
#66276=CARTESIAN_POINT('Ctrl Pts',(7.51641818475173,-2.46729715678315,5.53238442451228));
#66277=CARTESIAN_POINT('Ctrl Pts',(7.49406862765426,-2.53499925504279,5.52955144002753));
#66278=CARTESIAN_POINT('Ctrl Pts',(7.47527922314624,-2.58988156872399,5.52726692462762));
#66279=CARTESIAN_POINT('Ctrl Pts',(7.419002104162,-2.74854576203569,5.52069516276651));
#66280=CARTESIAN_POINT('Ctrl Pts',(7.37994412608967,-2.85175768996061,5.51646136557125));
#66281=CARTESIAN_POINT('Ctrl Pts',(7.23833043271452,-3.20355970950644,5.50214614670354));
#66282=CARTESIAN_POINT('Ctrl Pts',(7.12526656651669,-3.44772556345542,5.49241976365217));
#66283=CARTESIAN_POINT('Ctrl Pts',(6.89051923623114,-3.89356761827715,5.47470902098286));
#66284=CARTESIAN_POINT('Ctrl Pts',(6.77184723745495,-4.0964878828728,5.46666682230964));
#66285=CARTESIAN_POINT('Ctrl Pts',(6.30382404455578,-4.82071219808375,5.43734913745196));
#66286=CARTESIAN_POINT('Ctrl Pts',(5.9019117183868,-5.30515752190417,5.41662268430215));
#66287=CARTESIAN_POINT('Ctrl Pts',(5.44582022749347,-5.73820234441149,5.39185914061455));
#66288=CARTESIAN_POINT('Ctrl Pts',(5.44454390179606,-5.73941336697351,5.39178983285197));
#66289=CARTESIAN_POINT('Ctrl Pts',(5.41561536434037,-5.76684344414265,5.39021872098501));
#66290=CARTESIAN_POINT('Ctrl Pts',(5.38777491550423,-5.79286237111219,5.38870219151012));
#66291=CARTESIAN_POINT('Ctrl Pts',(5.35465441903023,-5.82337058851257,5.3868912766207));
#66292=CARTESIAN_POINT('Ctrl Pts',(5.34955466991898,-5.82805574710614,5.38661225191621));
#66293=CARTESIAN_POINT('Ctrl Pts',(5.34134909306165,-5.8355743968328,5.38616298304038));
#66294=CARTESIAN_POINT('Ctrl Pts',(5.338247138314,-5.83841212702958,5.38599307403998));
#66295=CARTESIAN_POINT('Ctrl Pts',(5.33272467074675,-5.8434561102553,5.38569045117117));
#66296=CARTESIAN_POINT('Ctrl Pts',(5.33030505154964,-5.84566333137357,5.38555781493821));
#66297=CARTESIAN_POINT('Ctrl Pts',(5.3252323925531,-5.85028493607,5.38527965440236));
#66298=CARTESIAN_POINT('Ctrl Pts',(5.32257907969499,-5.85269901910348,5.38513410637005));
#66299=CARTESIAN_POINT('Ctrl Pts',(5.31563658503624,-5.85900693419021,5.38475313839462));
#66300=CARTESIAN_POINT('Ctrl Pts',(5.31134477333396,-5.8628978549431,5.38451749057208));
#66301=CARTESIAN_POINT('Ctrl Pts',(5.29260841750075,-5.87984662144051,5.3834881715472));
#66302=CARTESIAN_POINT('Ctrl Pts',(5.27812007596994,-5.89285572565744,5.38269074111624));
#66303=CARTESIAN_POINT('Ctrl Pts',(5.17442466057858,-5.98527478853529,5.37697389045674));
#66304=CARTESIAN_POINT('Ctrl Pts',(5.08348121995228,-6.06270574425857,5.37191020654303));
#66305=CARTESIAN_POINT('Ctrl Pts',(4.81481472702408,-6.28115760289221,5.35690458604107));
#66306=CARTESIAN_POINT('Ctrl Pts',(4.63273928641868,-6.4166266617673,5.34668086950046));
#66307=CARTESIAN_POINT('Ctrl Pts',(4.24004379146213,-6.683367551155,5.32494517502725));
#66308=CARTESIAN_POINT('Ctrl Pts',(4.02854954289427,-6.81294063864242,5.31341506509093));
#66309=CARTESIAN_POINT('Ctrl Pts',(3.55014522555859,-7.07596087184507,5.28816772428524));
#66310=CARTESIAN_POINT('Ctrl Pts',(3.28105046358647,-7.20468440826013,5.27450473494476));
#66311=CARTESIAN_POINT('Ctrl Pts',(2.85189109243631,-7.38093148878701,5.25387180039208));
#66312=CARTESIAN_POINT('Ctrl Pts',(2.69651134816254,-7.43910365174001,5.24662331968075));
#66313=CARTESIAN_POINT('Ctrl Pts',(2.51267588593666,-7.50141171983601,5.23832199560696));
#66314=CARTESIAN_POINT('Ctrl Pts',(2.48589190813856,-7.51033017524066,5.23711921479041));
#66315=CARTESIAN_POINT('Ctrl Pts',(2.43917513217959,-7.52560850692108,5.23503298502007));
#66316=CARTESIAN_POINT('Ctrl Pts',(2.41926386294814,-7.53203299881919,5.2341474820606));
#66317=CARTESIAN_POINT('Ctrl Pts',(2.3929366404672,-7.54041246959668,5.23298150078921));
#66318=CARTESIAN_POINT('Ctrl Pts',(2.38654344802886,-7.54243835559213,5.2326987360169));
#66319=CARTESIAN_POINT('Ctrl Pts',(2.24068365330851,-7.58845464176538,5.22625610003152));
#66320=CARTESIAN_POINT('Ctrl Pts',(2.10002202388193,-7.62857900902259,5.22022319384978));
#66321=CARTESIAN_POINT('Ctrl Pts',(1.94130260266432,-7.66913123002159,5.21361163633654));
#66322=CARTESIAN_POINT('Ctrl Pts',(1.92426731585183,-7.6734232856582,5.2129045130747));
#66323=CARTESIAN_POINT('Ctrl Pts',(1.89958218180412,-7.6795553539887,5.21188343177967));
#66324=CARTESIAN_POINT('Ctrl Pts',(1.89194372456656,-7.68144074011864,5.21156796872443));
#66325=CARTESIAN_POINT('Ctrl Pts',(1.87850953909575,-7.68473542080214,5.21101401454212));
#66326=CARTESIAN_POINT('Ctrl Pts',(1.87271501229685,-7.68614956002874,5.21077536295318));
#66327=CARTESIAN_POINT('Ctrl Pts',(1.86078256180256,-7.68904734884855,5.21028449933993));
#66328=CARTESIAN_POINT('Ctrl Pts',(1.85464444891714,-7.69053020561584,5.21003231371852));
#66329=CARTESIAN_POINT('Ctrl Pts',(1.8422654391753,-7.69350506767117,5.2095243569158));
#66330=CARTESIAN_POINT('Ctrl Pts',(1.83602448910071,-7.69499683238017,5.20926859384797));
#66331=CARTESIAN_POINT('Ctrl Pts',(1.81139562774766,-7.70085216292545,5.20826055102294));
#66332=CARTESIAN_POINT('Ctrl Pts',(1.79299384759245,-7.70515744319818,5.20751019909747));
#66333=CARTESIAN_POINT('Ctrl Pts',(1.57810016597318,-7.75462244532385,5.1987802541683));
#66334=CARTESIAN_POINT('Ctrl Pts',(1.37995964699328,-7.79232237260666,5.1910512489065));
#66335=CARTESIAN_POINT('Ctrl Pts',(0.890968020032899,-7.86612265833955,
5.17262840179251));
#66336=CARTESIAN_POINT('Ctrl Pts',(0.599137367636005,-7.89371635379074,
5.16219693247563));
#66337=CARTESIAN_POINT('Ctrl Pts',(-0.428471933227776,-7.93355122247504,
5.12641603759899));
#66338=CARTESIAN_POINT('Ctrl Pts',(-1.16363922138665,-7.85941737862278,
5.10277865502671));
#66339=CARTESIAN_POINT('Ctrl Pts',(-1.91999253216604,-7.67459643573014,
5.07220294834361));
#66340=CARTESIAN_POINT('Ctrl Pts',(-1.96203479673353,-7.66395596914826,
5.07048127575492));
#66341=CARTESIAN_POINT('Ctrl Pts',(-2.01103863132241,-7.65112395424004,
5.06844642171024));
#66342=CARTESIAN_POINT('Ctrl Pts',(-2.01808799430845,-7.64926761110933,
5.06815302008423));
#66343=CARTESIAN_POINT('Ctrl Pts',(-2.02936187150806,-7.64628213682953,
5.06768268524874));
#66344=CARTESIAN_POINT('Ctrl Pts',(-2.03358804624155,-7.64515923833829,
5.06750612489999));
#66345=CARTESIAN_POINT('Ctrl Pts',(-2.04109050360451,-7.64315916749087,
5.06719224995212));
#66346=CARTESIAN_POINT('Ctrl Pts',(-2.04436716138332,-7.64228338998845,
5.06705501810331));
#66347=CARTESIAN_POINT('Ctrl Pts',(-2.05118423540561,-7.64045664023745,
5.06676919991644));
#66348=CARTESIAN_POINT('Ctrl Pts',(-2.05472455511314,-7.63950531392277,
5.06662059272963));
#66349=CARTESIAN_POINT('Ctrl Pts',(-2.0638764039309,-7.63703928056875,5.0662359934031));
#66350=CARTESIAN_POINT('Ctrl Pts',(-2.06948691881879,-7.63552085166107,
5.06599978350611));
#66351=CARTESIAN_POINT('Ctrl Pts',(-2.09305728041989,-7.6291138853219,5.06500563905816));
#66352=CARTESIAN_POINT('Ctrl Pts',(-2.11100139144183,-7.62416818864292,
5.06424439861309));
#66353=CARTESIAN_POINT('Ctrl Pts',(-2.23402160194552,-7.58979416784353,
5.05899615232844));
#66354=CARTESIAN_POINT('Ctrl Pts',(-2.33849244929992,-7.55825900139326,
5.05439205598049));
#66355=CARTESIAN_POINT('Ctrl Pts',(-2.66461291928151,-7.45240912924316,
5.03962993170186));
#66356=CARTESIAN_POINT('Ctrl Pts',(-2.88363371305214,-7.37042798336743,
5.02914512901995));
#66357=CARTESIAN_POINT('Ctrl Pts',(-3.32546959450999,-7.18233403775669,
5.00724378642243));
#66358=CARTESIAN_POINT('Ctrl Pts',(-3.54761102952931,-7.07524728994771,
4.99582061292049));
#66359=CARTESIAN_POINT('Ctrl Pts',(-3.87552666056263,-6.89783887445839,
4.97862181384411));
#66360=CARTESIAN_POINT('Ctrl Pts',(-3.98520935426634,-6.8350563357683,4.97280819635379));
#66361=CARTESIAN_POINT('Ctrl Pts',(-4.22829323390074,-6.68807353137622,
4.95982983710774));
#66362=CARTESIAN_POINT('Ctrl Pts',(-4.36077719442273,-6.60245529898888,
4.95269083661561));
#66363=CARTESIAN_POINT('Ctrl Pts',(-4.80699792251463,-6.2947895277123,4.92851108551677));
#66364=CARTESIAN_POINT('Ctrl Pts',(-5.10708594539538,-6.05386909264616,
4.9120446361679));
#66365=CARTESIAN_POINT('Ctrl Pts',(-5.40765727608774,-5.77424007167193,
4.89540307254504));
#66366=CARTESIAN_POINT('Ctrl Pts',(-5.42672583031313,-5.75632281935096,
4.89434644852284));
#66367=CARTESIAN_POINT('Ctrl Pts',(-5.45287813165452,-5.73150406683766,
4.89289602763517));
#66368=CARTESIAN_POINT('Ctrl Pts',(-5.4600382483855,-5.72468349465123,4.89249879095456));
#66369=CARTESIAN_POINT('Ctrl Pts',(-5.47142371467195,-5.71379715406999,
4.89186691877582));
#66370=CARTESIAN_POINT('Ctrl Pts',(-5.47565735380193,-5.70974009279524,
4.89163191170061));
#66371=CARTESIAN_POINT('Ctrl Pts',(-5.4838859887871,-5.70183709106808,4.89117504964814));
#66372=CARTESIAN_POINT('Ctrl Pts',(-5.48788145906199,-5.69799164991946,
4.89095317348654));
#66373=CARTESIAN_POINT('Ctrl Pts',(-5.49613082791164,-5.69003531776596,
4.89049497853555));
#66374=CARTESIAN_POINT('Ctrl Pts',(-5.50038416581546,-5.68592384961104,
4.89025868476488));
#66375=CARTESIAN_POINT('Ctrl Pts',(-5.51003213202295,-5.67657673407986,
4.88972257637979));
#66376=CARTESIAN_POINT('Ctrl Pts',(-5.51542392066684,-5.6713381568686,4.88942288795969));
#66377=CARTESIAN_POINT('Ctrl Pts',(-5.52908126568421,-5.65803099835766,
4.8886635652447));
#66378=CARTESIAN_POINT('Ctrl Pts',(-5.53733664542472,-5.64995197303344,
4.88820438124126));
#66379=CARTESIAN_POINT('Ctrl Pts',(-5.62953882810789,-5.55932325814271,
4.88307355545819));
#66380=CARTESIAN_POINT('Ctrl Pts',(-5.71165241360203,-5.47492563031201,
4.87848289381951));
#66381=CARTESIAN_POINT('Ctrl Pts',(-5.92513051783187,-5.2454772625069,4.86646638034512));
#66382=CARTESIAN_POINT('Ctrl Pts',(-6.05305100791411,-5.0973309005762,4.859180563585));
#66383=CARTESIAN_POINT('Ctrl Pts',(-6.26408275052058,-4.83377098473046,
4.84689468706409));
#66384=CARTESIAN_POINT('Ctrl Pts',(-6.34981621841605,-4.72058366149653,
4.84181779491729));
#66385=CARTESIAN_POINT('Ctrl Pts',(-6.82622800964603,-4.05513295250188,
4.81289545506634));
#66386=CARTESIAN_POINT('Ctrl Pts',(-7.1477806944428,-3.45695464486397,4.79070779214516));
#66387=CARTESIAN_POINT('Ctrl Pts',(-7.40972639245703,-2.77184859914397,
4.76285418706393));
#66388=CARTESIAN_POINT('Ctrl Pts',(-7.42956501495622,-2.71822613366663,
4.7606573527678));
#66389=CARTESIAN_POINT('Ctrl Pts',(-7.46984340307126,-2.6056202526197,4.75600035716128));
#66390=CARTESIAN_POINT('Ctrl Pts',(-7.49016965978471,-2.54660076678196,
4.75353470644808));
#66391=CARTESIAN_POINT('Ctrl Pts',(-7.51244983040541,-2.47933254075756,
4.75069015977429));
#66392=CARTESIAN_POINT('Ctrl Pts',(-7.51509193466226,-2.47131250849409,
4.75035046899859));
#66393=CARTESIAN_POINT('Ctrl Pts',(-7.51907665262619,-2.45915152888948,
4.74983453246708));
#66394=CARTESIAN_POINT('Ctrl Pts',(-7.52042870319198,-2.45501365986703,
4.74965883118682));
#66395=CARTESIAN_POINT('Ctrl Pts',(-7.5227766250305,-2.44780784661962,4.74935259552582));
#66396=CARTESIAN_POINT('Ctrl Pts',(-7.52377403764787,-2.44474040225809,
4.74922215075859));
#66397=CARTESIAN_POINT('Ctrl Pts',(-7.5258587182061,-2.43831581346585,4.74894876571159));
#66398=CARTESIAN_POINT('Ctrl Pts',(-7.52694561464965,-2.43495855541102,
4.74880580391882));
#66399=CARTESIAN_POINT('Ctrl Pts',(-7.5295368802034,-2.42693621585783,4.74846395090658));
#66400=CARTESIAN_POINT('Ctrl Pts',(-7.53103916009834,-2.42227046282022,
4.74826493833207));
#66401=CARTESIAN_POINT('Ctrl Pts',(-7.53610174353222,-2.40649694980396,
4.74759149341887));
#66402=CARTESIAN_POINT('Ctrl Pts',(-7.53964180203625,-2.39538275701834,
4.74711589951726));
#66403=CARTESIAN_POINT('Ctrl Pts',(-7.6510658372388,-2.04286720655529,4.73199803653185));
#66404=CARTESIAN_POINT('Ctrl Pts',(-7.73566424716292,-1.69456991453052,
4.71608971253339));
#66405=CARTESIAN_POINT('Ctrl Pts',(-7.87227861830664,-0.90077509254703,
4.67947086257571));
#66406=CARTESIAN_POINT('Ctrl Pts',(-7.91062332330754,-0.454110717659903,
4.65865197264493));
#66407=CARTESIAN_POINT('Ctrl Pts',(-7.91099723840516,-0.0066101396285724,
4.63857575021375));
#66408=CARTESIAN_POINT('Ctrl Pts',(-7.91099726676438,-0.00657611181310816,
4.63857422362495));
#66409=CARTESIAN_POINT('Ctrl Pts',(-7.9113461326049,0.413106033086809,4.61974605390583));
#66410=CARTESIAN_POINT('Ctrl Pts',(-7.87829895328532,0.832195301771229,
4.60162986480888));
#66411=CARTESIAN_POINT('Ctrl Pts',(-7.80869075279927,1.26836483588196,4.58368330375488));
#66412=CARTESIAN_POINT('Ctrl Pts',(-7.80514953152656,1.28997729834642,4.58279626632511));
#66413=CARTESIAN_POINT('Ctrl Pts',(-7.79957281418619,1.32314876595044,4.58143819724901));
#66414=CARTESIAN_POINT('Ctrl Pts',(-7.79760128023062,1.33471832860122,4.5809651620792));
#66415=CARTESIAN_POINT('Ctrl Pts',(-7.79431135143178,1.35376853773993,4.58018730769839));
#66416=CARTESIAN_POINT('Ctrl Pts',(-7.79300791898969,1.36125172977364,4.57988201897181));
#66417=CARTESIAN_POINT('Ctrl Pts',(-7.79066592557885,1.3745838366973,4.57933858188826));
#66418=CARTESIAN_POINT('Ctrl Pts',(-7.78963155133526,1.38043347639168,4.57910030208452));
#66419=CARTESIAN_POINT('Ctrl Pts',(-7.78761651413336,1.39175462195172,4.57863945487179));
#66420=CARTESIAN_POINT('Ctrl Pts',(-7.78663667154418,1.39722626815737,4.57841686186114));
#66421=CARTESIAN_POINT('Ctrl Pts',(-7.78461698452675,1.40843651503787,4.57796110166126));
#66422=CARTESIAN_POINT('Ctrl Pts',(-7.78357655964526,1.41417500790755,4.57772795291462));
#66423=CARTESIAN_POINT('Ctrl Pts',(-7.78107324115795,1.42789567922791,4.57717086270932));
#66424=CARTESIAN_POINT('Ctrl Pts',(-7.77960440781211,1.43587677517552,4.57684710843452));
#66425=CARTESIAN_POINT('Ctrl Pts',(-7.77428334955081,1.46454158546665,4.57568537435958));
#66426=CARTESIAN_POINT('Ctrl Pts',(-7.77036088056845,1.48521225724189,4.57484960884818));
#66427=CARTESIAN_POINT('Ctrl Pts',(-7.71297578157759,1.78117004491051,4.56291121538317));
#66428=CARTESIAN_POINT('Ctrl Pts',(-7.64499308453453,2.05345086443624,4.5522847487377));
#66429=CARTESIAN_POINT('Ctrl Pts',(-7.5258993133572,2.44140875890111,4.53744649876811));
#66430=CARTESIAN_POINT('Ctrl Pts',(-7.48626573197478,2.56036399048052,4.53293754984294));
#66431=CARTESIAN_POINT('Ctrl Pts',(-7.43172633737116,2.71194411482492,4.52721686896124));
#66432=CARTESIAN_POINT('Ctrl Pts',(-7.41940394808735,2.74547670049398,4.52595289539375));
#66433=CARTESIAN_POINT('Ctrl Pts',(-7.18938955804791,3.35854948915662,4.50286190390203));
#66434=CARTESIAN_POINT('Ctrl Pts',(-6.90466090853297,3.91059232269851,4.48255338963114));
#66435=CARTESIAN_POINT('Ctrl Pts',(-6.43819736912211,4.60215586547379,4.45209327277847));
#66436=CARTESIAN_POINT('Ctrl Pts',(-6.31064937823296,4.775553967995,4.44395249049151));
#66437=CARTESIAN_POINT('Ctrl Pts',(-6.16947094897371,4.9519355062321,4.43489464959119));
#66438=CARTESIAN_POINT('Ctrl Pts',(-6.16272211331928,4.96033196469787,4.43446154403397));
#66439=CARTESIAN_POINT('Ctrl Pts',(-6.15301521540111,4.97235826190897,4.43383840975184));
#66440=CARTESIAN_POINT('Ctrl Pts',(-6.15007102283519,4.97599933075136,4.43364938163703));
#66441=CARTESIAN_POINT('Ctrl Pts',(-6.14496447784659,4.98230311521361,4.43332147398018));
#66442=CARTESIAN_POINT('Ctrl Pts',(-6.14280362032367,4.98496704582215,4.43318270338037));
#66443=CARTESIAN_POINT('Ctrl Pts',(-6.13865221788584,4.9900781455581,4.43291606916263));
#66444=CARTESIAN_POINT('Ctrl Pts',(-6.13666194005881,4.99252553166319,4.43278822514949));
#66445=CARTESIAN_POINT('Ctrl Pts',(-6.1319800007823,4.99827574506915,4.4324874510393));
#66446=CARTESIAN_POINT('Ctrl Pts',(-6.1292871344986,5.00157758878303,4.43231443178927));
#66447=CARTESIAN_POINT('Ctrl Pts',(-6.11990333844358,5.01306452104573,4.4317114189976));
#66448=CARTESIAN_POINT('Ctrl Pts',(-6.1131987048338,5.02123832905829,4.43128040706413));
#66449=CARTESIAN_POINT('Ctrl Pts',(-6.0323667443222,5.11938099048258,4.42608236925635));
#66450=CARTESIAN_POINT('Ctrl Pts',(-5.95627915950428,5.20771027995432,4.42117238894877));
#66451=CARTESIAN_POINT('Ctrl Pts',(-5.42676746904316,5.79562568742529,4.38709675512741));
#66452=CARTESIAN_POINT('Ctrl Pts',(-4.91299893262688,6.23711222095047,4.35475675985159));
#66453=CARTESIAN_POINT('Ctrl Pts',(-4.1804002909589,6.71930976424148,4.31498152846115));
#66454=CARTESIAN_POINT('Ctrl Pts',(-4.0071570860641,6.82404345354929,4.30595104611405));
#66455=CARTESIAN_POINT('Ctrl Pts',(-3.6596479254456,7.01632657621063,4.28864502927477));
#66456=CARTESIAN_POINT('Ctrl Pts',(-3.48578344059753,7.10430732468601,4.28035966991629));
#66457=CARTESIAN_POINT('Ctrl Pts',(-3.25612831501158,7.21005665594024,4.26990186611492));
#66458=CARTESIAN_POINT('Ctrl Pts',(-3.20315101459247,7.23374815414356,4.26752189287803));
#66459=CARTESIAN_POINT('Ctrl Pts',(-3.1167633037527,7.27124568226868,4.26369288065955));
#66460=CARTESIAN_POINT('Ctrl Pts',(-3.08351105439703,7.28540917776741,4.26223136304086));
#66461=CARTESIAN_POINT('Ctrl Pts',(-3.04294818463583,7.30235910386455,4.26046334279329));
#66462=CARTESIAN_POINT('Ctrl Pts',(-3.03572928254775,7.30536308883576,4.26014925968905));
#66463=CARTESIAN_POINT('Ctrl Pts',(-3.023065936168,7.31061064623256,4.25959929049798));
#66464=CARTESIAN_POINT('Ctrl Pts',(-3.01762342444244,7.31285884888284,4.25936324329587));
#66465=CARTESIAN_POINT('Ctrl Pts',(-3.00664801553082,7.31737825193149,4.25888787440208));
#66466=CARTESIAN_POINT('Ctrl Pts',(-3.00111504272893,7.31964925878599,4.25864855955188));
#66467=CARTESIAN_POINT('Ctrl Pts',(-2.99045810324077,7.32400928123497,4.2581882545279));
#66468=CARTESIAN_POINT('Ctrl Pts',(-2.98533451129728,7.3260991990737,4.25796723311663));
#66469=CARTESIAN_POINT('Ctrl Pts',(-2.97324025818644,7.33101766180571,4.25744617472242));
#66470=CARTESIAN_POINT('Ctrl Pts',(-2.96626774076713,7.33384164548961,4.25714629610532));
#66471=CARTESIAN_POINT('Ctrl Pts',(-2.94205819848575,7.34360673306386,4.25610687189978));
#66472=CARTESIAN_POINT('Ctrl Pts',(-2.92480069062687,7.35049707295204,4.25536908548243));
#66473=CARTESIAN_POINT('Ctrl Pts',(-2.72763869072126,7.42841290996933,4.24697575651684));
#66474=CARTESIAN_POINT('Ctrl Pts',(-2.54520577019872,7.49288096473461,4.23955016034975));
#66475=CARTESIAN_POINT('Ctrl Pts',(-2.1481941124392,7.61700083548056,4.22401648706631));
#66476=CARTESIAN_POINT('Ctrl Pts',(-1.93309052457241,7.67441253341597,4.21598180268807));
#66477=CARTESIAN_POINT('Ctrl Pts',(-1.44406121445967,7.78306627934274,4.19830125171412));
#66478=CARTESIAN_POINT('Ctrl Pts',(-1.16927581143561,7.82906329113373,4.1887726796936));
#66479=CARTESIAN_POINT('Ctrl Pts',(-0.859015539428168,7.86429641872186,
4.17809123347411));
#66480=CARTESIAN_POINT('Ctrl Pts',(-0.825371726146504,7.86789853587983,
4.17693384475849));
#66481=CARTESIAN_POINT('Ctrl Pts',(-0.753203540400699,7.87515732235826,
4.17445154571953));
#66482=CARTESIAN_POINT('Ctrl Pts',(-0.714673374249742,7.87874738691195,
4.17312649065848));
#66483=CARTESIAN_POINT('Ctrl Pts',(-0.63159310311237,7.88587396853312,4.17026750962228));
#66484=CARTESIAN_POINT('Ctrl Pts',(-0.587036277189106,7.8893159707387,4.16873306794271));
#66485=CARTESIAN_POINT('Ctrl Pts',(-0.490170527452116,7.89597367029267,
4.16539098863235));
#66486=CARTESIAN_POINT('Ctrl Pts',(-0.437854062968823,7.89904748185584,
4.16358201762563));
#66487=CARTESIAN_POINT('Ctrl Pts',(-0.322506537285998,7.90467517138215,
4.15957855518861));
#66488=CARTESIAN_POINT('Ctrl Pts',(-0.25946785672346,7.90699540558906,4.15738074223292));
#66489=CARTESIAN_POINT('Ctrl Pts',(0.0328355819333474,7.91425474497045,
4.14711974313601));
#66490=CARTESIAN_POINT('Ctrl Pts',(0.26220761524485,7.909977391763,4.13887034271463));
#66491=CARTESIAN_POINT('Ctrl Pts',(0.594608680693564,7.88930454105963,4.1262376284037));
#66492=CARTESIAN_POINT('Ctrl Pts',(0.698020675745524,7.88082807214791,4.12221139048813));
#66493=CARTESIAN_POINT('Ctrl Pts',(0.818973251966151,7.86851458849383,4.11735879227862));
#66494=CARTESIAN_POINT('Ctrl Pts',(0.83670828271239,7.86664847674009,4.11664364126642));
#66495=CARTESIAN_POINT('Ctrl Pts',(0.860010697111956,7.86411686312228,4.1156990487015));
#66496=CARTESIAN_POINT('Ctrl Pts',(0.865584020258824,7.86350537225923,4.11547275530861));
#66497=CARTESIAN_POINT('Ctrl Pts',(0.874680690835874,7.86249752052174,4.11510278989729));
#66498=CARTESIAN_POINT('Ctrl Pts',(0.878204438470202,7.86210471408913,4.1149593272395));
#66499=CARTESIAN_POINT('Ctrl Pts',(0.884995674509492,7.86134304484092,4.11468254317032));
#66500=CARTESIAN_POINT('Ctrl Pts',(0.888263199406716,7.86097451345243,4.11454924137605));
#66501=CARTESIAN_POINT('Ctrl Pts',(0.895797945565579,7.86011994094739,4.11424155232053));
#66502=CARTESIAN_POINT('Ctrl Pts',(0.900064988862908,7.85963246348314,4.11406708027626));
#66503=CARTESIAN_POINT('Ctrl Pts',(0.91374006954864,7.85805890638206,4.11350721990209));
#66504=CARTESIAN_POINT('Ctrl Pts',(0.923146522803904,7.8569594110432,4.11312104083225));
#66505=CARTESIAN_POINT('Ctrl Pts',(1.00652200016415,7.84706207992535,4.10968867769814));
#66506=CARTESIAN_POINT('Ctrl Pts',(1.08036307204307,7.83723706174253,4.10658316599355));
#66507=CARTESIAN_POINT('Ctrl Pts',(1.80923373930108,7.72976009046038,4.07535546164927));
#66508=CARTESIAN_POINT('Ctrl Pts',(2.4496657420749,7.5512660580536,4.0435378618385));
#66509=CARTESIAN_POINT('Ctrl Pts',(3.36686820783636,7.16649222607155,3.99756935831303));
#66510=CARTESIAN_POINT('Ctrl Pts',(3.66499985560903,7.01870487430802,3.98251432674953));
#66511=CARTESIAN_POINT('Ctrl Pts',(4.11028283307435,6.76183990387279,3.96017117581671));
#66512=CARTESIAN_POINT('Ctrl Pts',(4.26443130901173,6.66569841696209,3.95246058826742));
#66513=CARTESIAN_POINT('Ctrl Pts',(4.46148063829603,6.53316387841869,3.94263896580992));
#66514=CARTESIAN_POINT('Ctrl Pts',(4.50748920022761,6.50150605869257,3.94034815569935));
#66515=CARTESIAN_POINT('Ctrl Pts',(4.58192315704946,6.4491191927419,3.9366453678727));
#66516=CARTESIAN_POINT('Ctrl Pts',(4.61055187983273,6.42868334773626,3.93522202210638));
#66517=CARTESIAN_POINT('Ctrl Pts',(4.6453607668822,6.40348383042291,3.93349225132037));
#66518=CARTESIAN_POINT('Ctrl Pts',(4.65167116992574,6.39890124539521,3.93317869985202));
#66519=CARTESIAN_POINT('Ctrl Pts',(4.66388318123222,6.39000532904415,3.93257197119375));
#66520=CARTESIAN_POINT('Ctrl Pts',(4.66978560637872,6.38569313577089,3.93227874952173));
#66521=CARTESIAN_POINT('Ctrl Pts',(4.68045423842075,6.37787614508806,3.93174879981233));
#66522=CARTESIAN_POINT('Ctrl Pts',(4.68522250303956,6.37437417298724,3.93151196032289));
#66523=CARTESIAN_POINT('Ctrl Pts',(4.69473080512801,6.36737452714166,3.93103971680801));
#66524=CARTESIAN_POINT('Ctrl Pts',(4.69947087304328,6.36387690131776,3.93080431112737));
#66525=CARTESIAN_POINT('Ctrl Pts',(4.71274907888548,6.35405618486938,3.93014492079969));
#66526=CARTESIAN_POINT('Ctrl Pts',(4.72127840683957,6.34772117277358,3.92972140932326));
#66527=CARTESIAN_POINT('Ctrl Pts',(4.75592001619211,6.32188326456845,3.92800151959611));
#66528=CARTESIAN_POINT('Ctrl Pts',(4.78192459528733,6.30223614355705,3.92671088252802));
#66529=CARTESIAN_POINT('Ctrl Pts',(5.18435880848601,5.99426191876322,3.90674200385417));
#66530=CARTESIAN_POINT('Ctrl Pts',(5.53426070615083,5.67280992077122,3.88952291819492));
#66531=CARTESIAN_POINT('Ctrl Pts',(6.19015867324328,4.95142548559815,3.85543642278137));
#66532=CARTESIAN_POINT('Ctrl Pts',(6.49107402614173,4.54979086371607,3.83870690388996));
#66533=CARTESIAN_POINT('Ctrl Pts',(6.7994156173806,4.04476800415872,3.81745028651577));
#66534=CARTESIAN_POINT('Ctrl Pts',(6.84548840490171,3.96629408710438,3.81413927791344));
#66535=CARTESIAN_POINT('Ctrl Pts',(6.9699844044705,3.74561180077756,3.80476118564742));
#66536=CARTESIAN_POINT('Ctrl Pts',(7.04539800874132,3.60175752857554,3.79856984891739));
#66537=CARTESIAN_POINT('Ctrl Pts',(7.12809184909534,3.43146505073849,3.79104984562325));
#66538=CARTESIAN_POINT('Ctrl Pts',(7.13972818106474,3.4071875904325,3.78997378134248));
#66539=CARTESIAN_POINT('Ctrl Pts',(7.15457606103271,3.37579964487902,3.7885778478988));
#66540=CARTESIAN_POINT('Ctrl Pts',(7.15790142996604,3.36874293672058,3.78826370530835));
#66541=CARTESIAN_POINT('Ctrl Pts',(7.16324982095177,3.35734953530132,3.78775602657592));
#66542=CARTESIAN_POINT('Ctrl Pts',(7.16527936098063,3.35301589296802,3.78756281184802));
#66543=CARTESIAN_POINT('Ctrl Pts',(7.16894909997456,3.34516141442336,3.78721242188283));
#66544=CARTESIAN_POINT('Ctrl Pts',(7.17059064186508,3.34164120355616,3.7870553120658));
#66545=CARTESIAN_POINT('Ctrl Pts',(7.17448069898205,3.33328309045065,3.78668211320358));
#66546=CARTESIAN_POINT('Ctrl Pts',(7.17672691206228,3.32844412461362,3.78646591333636));
#66547=CARTESIAN_POINT('Ctrl Pts',(7.18238909130059,3.31621384136436,3.78591914329472));
#66548=CARTESIAN_POINT('Ctrl Pts',(7.18579853796791,3.30881952839231,3.78558826353629));
#66549=CARTESIAN_POINT('Ctrl Pts',(7.20403239091891,3.26911335549267,3.78380989421684));
#66550=CARTESIAN_POINT('Ctrl Pts',(7.21865012854457,3.23670744515868,3.78235280280194));
#66551=CARTESIAN_POINT('Ctrl Pts',(7.5233897602565,2.54879984287543,3.75131737612828));
#66552=CARTESIAN_POINT('Ctrl Pts',(7.72330635234167,1.85697598462248,3.71845160350633));
#66553=CARTESIAN_POINT('Ctrl Pts',(7.85578943479332,0.953435919954922,3.67860894188584));
#66554=CARTESIAN_POINT('Ctrl Pts',(7.87703192123432,0.758182116598835,3.67014968929901));
#66555=CARTESIAN_POINT('Ctrl Pts',(7.90557668066405,0.357626394008536,3.65313974142851));
#66556=CARTESIAN_POINT('Ctrl Pts',(7.91219390578955,0.152422220298308,3.64460897013142));
#66557=CARTESIAN_POINT('Ctrl Pts',(7.91057662893636,-0.0898222997029053,
3.63473730704896));
#66558=CARTESIAN_POINT('Ctrl Pts',(7.91006986536628,-0.12682825148641,3.6332346696947));
#66559=CARTESIAN_POINT('Ctrl Pts',(7.90890315018272,-0.183154517483053,
3.63095540683182));
#66560=CARTESIAN_POINT('Ctrl Pts',(7.9084320354041,-0.202478053636192,3.63017488473024));
#66561=CARTESIAN_POINT('Ctrl Pts',(7.90754770532422,-0.234007330673138,
3.62890359356408));
#66562=CARTESIAN_POINT('Ctrl Pts',(7.90717703974626,-0.246214146701041,
3.62841195298656));
#66563=CARTESIAN_POINT('Ctrl Pts',(7.90640842014516,-0.269731300098618,
3.62746582082769));
#66564=CARTESIAN_POINT('Ctrl Pts',(7.90601445892209,-0.281041734638155,
3.62701124890992));
#66565=CARTESIAN_POINT('Ctrl Pts',(7.90525713516359,-0.301520849151827,
3.62618901105196));
#66566=CARTESIAN_POINT('Ctrl Pts',(7.90490208906579,-0.310689810305537,
3.62582117688634));
#66567=CARTESIAN_POINT('Ctrl Pts',(7.90415890407945,-0.329055854651695,
3.62508497546821));
#66568=CARTESIAN_POINT('Ctrl Pts',(7.90377066320563,-0.338252923671653,
3.62471661119487));
#66569=CARTESIAN_POINT('Ctrl Pts',(7.90265310833152,-0.36367374169184,3.62369927288451));
#66570=CARTESIAN_POINT('Ctrl Pts',(7.90188988704084,-0.379895981475649,
3.62305099009468));
#66571=CARTESIAN_POINT('Ctrl Pts',(7.89869923170493,-0.443538009338258,
3.62051131205509));
#66572=CARTESIAN_POINT('Ctrl Pts',(7.89589483711112,-0.490938189700778,
3.61862767657726));
#66573=CARTESIAN_POINT('Ctrl Pts',(7.83679487522013,-1.3574567574322,3.58433352492923));
#66574=CARTESIAN_POINT('Ctrl Pts',(7.65376146253957,-2.16285430851055,3.55546092757715));
#66575=CARTESIAN_POINT('Ctrl Pts',(7.27933111055042,-3.10353123309247,3.5184128417499));
#66576=CARTESIAN_POINT('Ctrl Pts',(7.2021041731806,-3.27875871758812,3.51132144737967));
#66577=CARTESIAN_POINT('Ctrl Pts',(7.06094892846123,-3.5699281841366,3.49899125446052));
#66578=CARTESIAN_POINT('Ctrl Pts',(7.0003282870638,-3.6873823346244,3.49386019219852));
#66579=CARTESIAN_POINT('Ctrl Pts',(6.92586660625074,-3.82319364130145,3.48768605027054));
#66580=CARTESIAN_POINT('Ctrl Pts',(6.91485096587378,-3.84308131206811,3.48677575580106));
#66581=CARTESIAN_POINT('Ctrl Pts',(6.90017269478158,-3.86931407985933,3.48556652568591));
#66582=CARTESIAN_POINT('Ctrl Pts',(6.89658668702919,-3.87570209564345,3.48527139278894));
#66583=CARTESIAN_POINT('Ctrl Pts',(6.89069575709783,-3.8861619724174,3.4847870238208));
#66584=CARTESIAN_POINT('Ctrl Pts',(6.88839608119013,-3.89023679501067,3.48459805264576));
#66585=CARTESIAN_POINT('Ctrl Pts',(6.88394141698612,-3.89811373199796,3.48423221706504));
#66586=CARTESIAN_POINT('Ctrl Pts',(6.88178688996864,-3.9019161063546,3.48405537622846));
#66587=CARTESIAN_POINT('Ctrl Pts',(6.87681818007794,-3.91066811897232,3.48364777194068));
#66588=CARTESIAN_POINT('Ctrl Pts',(6.87400180460029,-3.91561650429318,3.48341689547405));
#66589=CARTESIAN_POINT('Ctrl Pts',(6.8650220857485,-3.93135436739274,3.48268127459577));
#66590=CARTESIAN_POINT('Ctrl Pts',(6.85883868507879,-3.94213232770218,3.48217548259414));
#66591=CARTESIAN_POINT('Ctrl Pts',(6.79915976145434,-4.04559005024999,3.47730067454748));
#66592=CARTESIAN_POINT('Ctrl Pts',(6.74382121814735,-4.13717834663212,3.47282585299034));
#66593=CARTESIAN_POINT('Ctrl Pts',(6.68044360613762,-4.2374200617693,3.46775773281299));
#66594=CARTESIAN_POINT('Ctrl Pts',(6.67422319014463,-4.24721089194645,3.46726093549891));
#66595=CARTESIAN_POINT('Ctrl Pts',(6.64395662616424,-4.29461926703525,3.46484686177509));
#66596=CARTESIAN_POINT('Ctrl Pts',(6.61961417028502,-4.33204598564868,3.46291499371247));
#66597=CARTESIAN_POINT('Ctrl Pts',(6.55063146943546,-4.43616830599287,3.45747153876109));
#66598=CARTESIAN_POINT('Ctrl Pts',(6.50529177037389,-4.50239273201016,3.4539293167579));
#66599=CARTESIAN_POINT('Ctrl Pts',(6.31854657755343,-4.76644726493357,3.43951512594269));
#66600=CARTESIAN_POINT('Ctrl Pts',(6.16906481531727,-4.95839515373934,3.42837206930145));
#66601=CARTESIAN_POINT('Ctrl Pts',(5.77954837991584,-5.4136373996023,3.40078035347787));
#66602=CARTESIAN_POINT('Ctrl Pts',(5.53010701885256,-5.66820819805886,3.38431470438502));
#66603=CARTESIAN_POINT('Ctrl Pts',(5.03021769156437,-6.11385521820825,3.35426489861763));
#66604=CARTESIAN_POINT('Ctrl Pts',(4.78385255596312,-6.30849415009625,3.34059416401193));
#66605=CARTESIAN_POINT('Ctrl Pts',(4.4351627534636,-6.5517686100401,3.32285292834257));
#66606=CARTESIAN_POINT('Ctrl Pts',(4.34242608550252,-6.61359793295346,3.31827598207366));
#66607=CARTESIAN_POINT('Ctrl Pts',(4.23372817827796,-6.68279654663093,3.31307073470467));
#66608=CARTESIAN_POINT('Ctrl Pts',(4.2190141431131,-6.69209560874318,3.31236943137613));
#66609=CARTESIAN_POINT('Ctrl Pts',(4.1973919216448,-6.70566089020976,3.3113436961367));
#66610=CARTESIAN_POINT('Ctrl Pts',(4.19050771729806,-6.70996512585298,3.31101783150176));
#66611=CARTESIAN_POINT('Ctrl Pts',(4.17850638290732,-6.71744308983454,3.3104509879392));
#66612=CARTESIAN_POINT('Ctrl Pts',(4.17339223927146,-6.72062158394293,3.31020982973519));
#66613=CARTESIAN_POINT('Ctrl Pts',(4.16352237718879,-6.72674019682897,3.30974516830112));
#66614=CARTESIAN_POINT('Ctrl Pts',(4.15876716235496,-6.72968111803709,3.30952163498626));
#66615=CARTESIAN_POINT('Ctrl Pts',(4.1475133713162,-6.73662468059505,3.30899341062463));
#66616=CARTESIAN_POINT('Ctrl Pts',(4.14101210675458,-6.74062296710052,3.30868888316714));
#66617=CARTESIAN_POINT('Ctrl Pts',(4.11829466574378,-6.75454895377204,3.30762694602706));
#66618=CARTESIAN_POINT('Ctrl Pts',(4.10204843214782,-6.76442763208508,3.30687137427375));
#66619=CARTESIAN_POINT('Ctrl Pts',(3.90983996775815,-6.88035473911191,3.29797749803898));
#66620=CARTESIAN_POINT('Ctrl Pts',(3.72984032651347,-6.97957224301875,3.29009823352059));
#66621=CARTESIAN_POINT('Ctrl Pts',(3.3848435529992,-7.15257486092685,3.2757283582639));
#66622=CARTESIAN_POINT('Ctrl Pts',(3.22078882215947,-7.22793306713144,3.26918915231857));
#66623=CARTESIAN_POINT('Ctrl Pts',(2.53976986034529,-7.51296210826921,3.24299384441545));
#66624=CARTESIAN_POINT('Ctrl Pts',(2.00394032043284,-7.67328024046745,3.22468660656596));
#66625=CARTESIAN_POINT('Ctrl Pts',(1.25148051286011,-7.8141468322362,3.19814487975362));
#66626=CARTESIAN_POINT('Ctrl Pts',(1.04582790496657,-7.84431839046821,3.19079256511615));
#66627=CARTESIAN_POINT('Ctrl Pts',(0.682112183144507,-7.88312202441566,
3.17728068105468));
#66628=CARTESIAN_POINT('Ctrl Pts',(0.524529798662349,-7.89517276227876,
3.17125965750425));
#66629=CARTESIAN_POINT('Ctrl Pts',(0.343699301150583,-7.90356388118705,
3.1640584609471));
#66630=CARTESIAN_POINT('Ctrl Pts',(0.320692927856891,-7.90453080572275,
3.1631368749317));
#66631=CARTESIAN_POINT('Ctrl Pts',(0.291561230009582,-7.90562777880492,
3.16196273131111));
#66632=CARTESIAN_POINT('Ctrl Pts',(0.285439321161095,-7.90585118259775,
3.16171558785424));
#66633=CARTESIAN_POINT('Ctrl Pts',(0.275671790169792,-7.90619626429341,
3.16132061998871));
#66634=CARTESIAN_POINT('Ctrl Pts',(0.272026319682302,-7.90632253243103,
3.16117306438117));
#66635=CARTESIAN_POINT('Ctrl Pts',(0.265118274049408,-7.90655702292956,
3.16089317612412));
#66636=CARTESIAN_POINT('Ctrl Pts',(0.261855725732904,-7.90666574700803,
3.16076087369509));
#66637=CARTESIAN_POINT('Ctrl Pts',(0.254447226148604,-7.90690804397598,
3.16046018306959));
#66638=CARTESIAN_POINT('Ctrl Pts',(0.25030123812789,-7.90704037531561,3.16029172241721));
#66639=CARTESIAN_POINT('Ctrl Pts',(0.239613683606313,-7.90737308560492,
3.15985698665332));
#66640=CARTESIAN_POINT('Ctrl Pts',(0.233071981559446,-7.90756860755657,
3.15959043055696));
#66641=CARTESIAN_POINT('Ctrl Pts',(0.194592457241041,-7.90867091383711,
3.15801982194463));
#66642=CARTESIAN_POINT('Ctrl Pts',(0.162650036029058,-7.9093923127789,3.15670519662121));
#66643=CARTESIAN_POINT('Ctrl Pts',(-0.370402013244937,-7.91820053529516,
3.13459676736143));
#66644=CARTESIAN_POINT('Ctrl Pts',(-0.871124245329878,-7.87884268276986,
3.11138836845481));
#66645=CARTESIAN_POINT('Ctrl Pts',(-1.8440331853989,-7.70845386717232,3.0656354948699));
#66646=CARTESIAN_POINT('Ctrl Pts',(-2.31463408691876,-7.58045331384529,
3.04320730346226));
#66647=CARTESIAN_POINT('Ctrl Pts',(-3.01048162545472,-7.32028373929692,
3.01098232744258));
#66648=CARTESIAN_POINT('Ctrl Pts',(-3.24595845126178,-7.21895588338692,
3.00023387229291));
#66649=CARTESIAN_POINT('Ctrl Pts',(-3.49284756836139,-7.09818875858424,
2.98913616852862));
#66650=CARTESIAN_POINT('Ctrl Pts',(-3.50954688055067,-7.08994700176744,
2.98838635547279));
#66651=CARTESIAN_POINT('Ctrl Pts',(-3.53350968651125,-7.07801502292328,
2.98731156375863));
#66652=CARTESIAN_POINT('Ctrl Pts',(-3.54079676104572,-7.07437245746181,
2.98698487470491));
#66653=CARTESIAN_POINT('Ctrl Pts',(-3.55343109242113,-7.06803256498799,
2.98641872627335));
#66654=CARTESIAN_POINT('Ctrl Pts',(-3.55878093003968,-7.06534041363244,
2.98617908097432));
#66655=CARTESIAN_POINT('Ctrl Pts',(-3.56905912182974,-7.06015357459443,
2.98571882820238));
#66656=CARTESIAN_POINT('Ctrl Pts',(-3.57398792890262,-7.05765979600808,
2.9854981882038));
#66657=CARTESIAN_POINT('Ctrl Pts',(-3.58558790359786,-7.05177540667011,
2.98497907366586));
#66658=CARTESIAN_POINT('Ctrl Pts',(-3.59225688589682,-7.04838048538039,
2.98468075475164));
#66659=CARTESIAN_POINT('Ctrl Pts',(-3.61526618961727,-7.03662619886458,
2.98365192933108));
#66660=CARTESIAN_POINT('Ctrl Pts',(-3.63158228865482,-7.02821940259681,
2.98292313647108));
#66661=CARTESIAN_POINT('Ctrl Pts',(-3.81174316116407,-6.93459744695517,
2.97488398113846));
#66662=CARTESIAN_POINT('Ctrl Pts',(-3.97259050695435,-6.84372398100208,
2.96778304378895));
#66663=CARTESIAN_POINT('Ctrl Pts',(-4.76752217581276,-6.35713512157041,
2.932886150135));
#66664=CARTESIAN_POINT('Ctrl Pts',(-5.34635665456707,-5.8786746103773,2.9085708611738));
#66665=CARTESIAN_POINT('Ctrl Pts',(-5.97664321400985,-5.18645732853546,
2.8756797597553));
#66666=CARTESIAN_POINT('Ctrl Pts',(-6.09877210602362,-5.04227892096413,
2.86890288269143));
#66667=CARTESIAN_POINT('Ctrl Pts',(-6.28072062752146,-4.81118951116262,
2.85792050089018));
#66668=CARTESIAN_POINT('Ctrl Pts',(-6.34416416012781,-4.72721648111431,
2.85390618576162));
#66669=CARTESIAN_POINT('Ctrl Pts',(-6.43418790302885,-4.60298481864827,
2.84789425920229));
#66670=CARTESIAN_POINT('Ctrl Pts',(-6.46210668868853,-4.56370684563079,
2.84598312214154));
#66671=CARTESIAN_POINT('Ctrl Pts',(-6.49409156755445,-4.51782642904247,
2.84373575157979));
#66672=CARTESIAN_POINT('Ctrl Pts',(-6.49850947689704,-4.51146932931417,
2.84342402907383));
#66673=CARTESIAN_POINT('Ctrl Pts',(-6.50523745335268,-4.50175779711832,
2.84294730056086));
#66674=CARTESIAN_POINT('Ctrl Pts',(-6.50755426570889,-4.49840805920864,
2.84278277184036));
#66675=CARTESIAN_POINT('Ctrl Pts',(-6.5117735869608,-4.49229751839385,2.84248247257348));
#66676=CARTESIAN_POINT('Ctrl Pts',(-6.51367693090283,-4.48953729034141,
2.84234676004748));
#66677=CARTESIAN_POINT('Ctrl Pts',(-6.51778667962103,-4.48356922077212,
2.84205319345133));
#66678=CARTESIAN_POINT('Ctrl Pts',(-6.51999247127112,-4.48036096011981,
2.84189529722315));
#66679=CARTESIAN_POINT('Ctrl Pts',(-6.52596120398778,-4.4716658673442,2.84146714100703));
#66680=CARTESIAN_POINT('Ctrl Pts',(-6.52971958614786,-4.4661759247586,2.84119657009575));
#66681=CARTESIAN_POINT('Ctrl Pts',(-6.54729453417257,-4.44043424833065,
2.83992679894327));
#66682=CARTESIAN_POINT('Ctrl Pts',(-6.56102370695979,-4.42012329272008,
2.83892173512237));
#66683=CARTESIAN_POINT('Ctrl Pts',(-6.77700847681125,-4.09737169983901,
2.82290499672281));
#66684=CARTESIAN_POINT('Ctrl Pts',(-6.95824084589083,-3.78141978208877,
2.8066064321629));
#66685=CARTESIAN_POINT('Ctrl Pts',(-7.34232088910019,-2.99004645780602,
2.76634140042128));
#66686=CARTESIAN_POINT('Ctrl Pts',(-7.52164893681742,-2.50497779403031,
2.74218312004849));
#66687=CARTESIAN_POINT('Ctrl Pts',(-7.69981614148297,-1.82527241729796,
2.71091799803428));
#66688=CARTESIAN_POINT('Ctrl Pts',(-7.74075411332836,-1.64302144571686,
2.70276385629693));
#66689=CARTESIAN_POINT('Ctrl Pts',(-7.80783294921315,-1.28566805199094,
2.68725779053315));
#66690=CARTESIAN_POINT('Ctrl Pts',(-7.83462354931685,-1.11080009069451,
2.67989048892087));
#66691=CARTESIAN_POINT('Ctrl Pts',(-7.8593221719404,-0.903329603047026,
2.67140403945952));
#66692=CARTESIAN_POINT('Ctrl Pts',(-7.86291938884934,-0.871463189056676,
2.67010755803925));
#66693=CARTESIAN_POINT('Ctrl Pts',(-7.86742142293673,-0.829281810804904,
2.66840053167805));
#66694=CARTESIAN_POINT('Ctrl Pts',(-7.86849987235438,-0.818985914177716,
2.66798458758142));
#66695=CARTESIAN_POINT('Ctrl Pts',(-7.87023453339471,-0.80210546403663,
2.66730380401011));
#66696=CARTESIAN_POINT('Ctrl Pts',(-7.87090269718427,-0.795522166759528,
2.66703859313565));
#66697=CARTESIAN_POINT('Ctrl Pts',(-7.87217935334179,-0.782784437686145,
2.66652601040819));
#66698=CARTESIAN_POINT('Ctrl Pts',(-7.8727888901592,-0.77663011676877,2.66627860627157));
#66699=CARTESIAN_POINT('Ctrl Pts',(-7.87417650102444,-0.762450289938069,
2.66570915865352));
#66700=CARTESIAN_POINT('Ctrl Pts',(-7.87494952392045,-0.754424290507175,
2.66538727226171));
#66701=CARTESIAN_POINT('Ctrl Pts',(-7.8769823814999,-0.732974318159018,
2.6645281539418));
#66702=CARTESIAN_POINT('Ctrl Pts',(-7.87822017326152,-0.719548256502081,
2.6639916063435));
#66703=CARTESIAN_POINT('Ctrl Pts',(-7.88647634114548,-0.627419536763525,
2.6603179848463));
#66704=CARTESIAN_POINT('Ctrl Pts',(-7.89234969238837,-0.548617474275349,
2.65721652641348));
#66705=CARTESIAN_POINT('Ctrl Pts',(-7.89925256520858,-0.432569512619185,
2.65270539816774));
#66706=CARTESIAN_POINT('Ctrl Pts',(-7.90120109106163,-0.395384414709395,
2.65126837136832));
#66707=CARTESIAN_POINT('Ctrl Pts',(-7.90409180081347,-0.331604948878667,
2.64881755839694));
#66708=CARTESIAN_POINT('Ctrl Pts',(-7.90516246252931,-0.30501720377632,
2.64780004328332));
#66709=CARTESIAN_POINT('Ctrl Pts',(-7.90941321556983,-0.184313441106155,
2.64319896469569));
#66710=CARTESIAN_POINT('Ctrl Pts',(-7.91104687283901,-0.090149221173572,
2.6396600503638));
#66711=CARTESIAN_POINT('Ctrl Pts',(-7.91090043088205,0.197783711785378,
2.62897232910267));
#66712=CARTESIAN_POINT('Ctrl Pts',(-7.90368344506989,0.391479553338397,
2.62196911778459));
#66713=CARTESIAN_POINT('Ctrl Pts',(-7.83360410443304,1.33702722556193,2.58830171568523));
#66714=CARTESIAN_POINT('Ctrl Pts',(-7.67054236727053,2.07737074208001,2.56390246919381));
#66715=CARTESIAN_POINT('Ctrl Pts',(-7.38098275117619,2.84776302298358,2.53195489733808));
#66716=CARTESIAN_POINT('Ctrl Pts',(-7.3559215824904,2.91188560715957,2.52924061533081));
#66717=CARTESIAN_POINT('Ctrl Pts',(-7.32639570807193,2.98461725333508,2.52609028782147));
#66718=CARTESIAN_POINT('Ctrl Pts',(-7.32274766067037,2.99355656649625,2.52570184461408));
#66719=CARTESIAN_POINT('Ctrl Pts',(-7.31738022512135,3.00664061305569,2.52513144800519));
#66720=CARTESIAN_POINT('Ctrl Pts',(-7.31567364939421,3.01079062548021,2.52495025584307));
#66721=CARTESIAN_POINT('Ctrl Pts',(-7.31264053572508,3.01814867866673,2.52462851035576));
#66722=CARTESIAN_POINT('Ctrl Pts',(-7.31131541343025,3.02135730700736,2.52448804183294));
#66723=CARTESIAN_POINT('Ctrl Pts',(-7.30854297254269,3.02805794318884,2.52419435281525));
#66724=CARTESIAN_POINT('Ctrl Pts',(-7.30709526607084,3.03154977879059,2.52404110936979));
#66725=CARTESIAN_POINT('Ctrl Pts',(-7.30330907022856,3.04066352943553,2.5236406315867));
#66726=CARTESIAN_POINT('Ctrl Pts',(-7.30096659568248,3.04628377582745,2.52339315911423));
#66727=CARTESIAN_POINT('Ctrl Pts',(-7.29077549824852,3.07065577093975,2.52231782254121));
#66728=CARTESIAN_POINT('Ctrl Pts',(-7.28286116320372,3.08937979100684,2.52148607870905));
#66729=CARTESIAN_POINT('Ctrl Pts',(-7.1875282475584,3.31251967234924,2.51150879781683));
#66730=CARTESIAN_POINT('Ctrl Pts',(-7.09160778362345,3.51318005866237,2.50188465827764));
#66731=CARTESIAN_POINT('Ctrl Pts',(-6.80248448454122,4.05778221343971,2.47446765944818));
#66732=CARTESIAN_POINT('Ctrl Pts',(-6.59182146172717,4.39172769546328,2.45617814284535));
#66733=CARTESIAN_POINT('Ctrl Pts',(-6.00621276690245,5.18237120887278,2.41113207155075));
#66734=CARTESIAN_POINT('Ctrl Pts',(-5.60336842861333,5.61551544528882,2.38493884658187));
#66735=CARTESIAN_POINT('Ctrl Pts',(-5.12639249907694,6.02540888216721,2.35932354004985));
#66736=CARTESIAN_POINT('Ctrl Pts',(-5.09652529637467,6.05069270515896,2.35773870909082));
#66737=CARTESIAN_POINT('Ctrl Pts',(-5.05753268577517,6.08320800186725,2.35569416201859));
#66738=CARTESIAN_POINT('Ctrl Pts',(-5.04857746838279,6.09064216720154,2.35522626205605));
#66739=CARTESIAN_POINT('Ctrl Pts',(-5.03481659835367,6.10201453812305,2.3545098065588));
#66740=CARTESIAN_POINT('Ctrl Pts',(-5.03002267565726,6.10596687553497,2.35426068242709));
#66741=CARTESIAN_POINT('Ctrl Pts',(-5.02099045769576,6.11339560899103,2.35379219067829));
#66742=CARTESIAN_POINT('Ctrl Pts',(-5.01675319759292,6.11687325378643,2.35357277296644));
#66743=CARTESIAN_POINT('Ctrl Pts',(-5.00704401041266,6.1248249964528,2.35307083560828));
#66744=CARTESIAN_POINT('Ctrl Pts',(-5.00156969125374,6.12929617356259,2.35278843311107));
#66745=CARTESIAN_POINT('Ctrl Pts',(-4.98649143065941,6.14157776550707,2.3520122516251));
#66746=CARTESIAN_POINT('Ctrl Pts',(-4.97687511952548,6.14937299927664,2.35151907985435));
#66747=CARTESIAN_POINT('Ctrl Pts',(-4.92582803772797,6.19055492798307,2.34891085951436));
#66748=CARTESIAN_POINT('Ctrl Pts',(-4.88407906257168,6.22354593642434,2.3468115819914));
#66749=CARTESIAN_POINT('Ctrl Pts',(-4.7672221738974,6.31398883347697,2.3410271497152));
#66750=CARTESIAN_POINT('Ctrl Pts',(-4.69141141161012,6.37051975503729,2.33737785952797));
#66751=CARTESIAN_POINT('Ctrl Pts',(-4.47404734589596,6.52661983411752,2.32718936707845));
#66752=CARTESIAN_POINT('Ctrl Pts',(-4.33021297689338,6.6229242418097,2.32076936232157));
#66753=CARTESIAN_POINT('Ctrl Pts',(-3.56005813576383,7.10275784842637,2.28781164904871));
#66754=CARTESIAN_POINT('Ctrl Pts',(-2.8858346125184,7.40236329522394,2.26409867194546));
#66755=CARTESIAN_POINT('Ctrl Pts',(-2.05456376408631,7.64066249596872,2.23273018666935));
#66756=CARTESIAN_POINT('Ctrl Pts',(-1.92823373080248,7.6735173137064,2.22789728491863));
#66757=CARTESIAN_POINT('Ctrl Pts',(-1.79187482110973,7.70540047150329,2.2225581134677));
#66758=CARTESIAN_POINT('Ctrl Pts',(-1.78259225512469,7.70755322081026,2.22219404569177));
#66759=CARTESIAN_POINT('Ctrl Pts',(-1.76496239083467,7.71160826644694,2.22150140456071));
#66760=CARTESIAN_POINT('Ctrl Pts',(-1.75661584453204,7.71351379528824,2.22117298126222));
#66761=CARTESIAN_POINT('Ctrl Pts',(-1.7378146952725,7.7177740267806,2.22043201837602));
#66762=CARTESIAN_POINT('Ctrl Pts',(-1.72735838194081,7.72012103935042,2.22001911755073));
#66763=CARTESIAN_POINT('Ctrl Pts',(-1.64157668157672,7.73919250462231,2.21662487028983));
#66764=CARTESIAN_POINT('Ctrl Pts',(-1.56601723034388,7.75483487634673,2.21359160729075));
#66765=CARTESIAN_POINT('Ctrl Pts',(-1.4805930848233,7.7712200889489,2.21010176978536));
#66766=CARTESIAN_POINT('Ctrl Pts',(-1.47093942835568,7.7730531163893,2.20970651942825));
#66767=CARTESIAN_POINT('Ctrl Pts',(-1.45689889186557,7.77569202791625,2.20913036254567));
#66768=CARTESIAN_POINT('Ctrl Pts',(-1.45251467405962,7.77651220121256,2.20895027174178));
#66769=CARTESIAN_POINT('Ctrl Pts',(-1.44478197119958,7.77795202171177,2.2086323081849));
#66770=CARTESIAN_POINT('Ctrl Pts',(-1.44143377180702,7.77857321607112,2.20849452446221));
#66771=CARTESIAN_POINT('Ctrl Pts',(-1.4345174880602,7.77985178135427,2.20820968349918));
#66772=CARTESIAN_POINT('Ctrl Pts',(-1.43094935118121,7.78050885981514,2.20806260938227));
#66773=CARTESIAN_POINT('Ctrl Pts',(-1.42181068094513,7.78218526234554,2.20768560566028));
#66774=CARTESIAN_POINT('Ctrl Pts',(-1.41623954809576,7.7832010517458,2.20745547124208));
#66775=CARTESIAN_POINT('Ctrl Pts',(-1.39291826733194,7.78742737206569,2.20649083398231));
#66776=CARTESIAN_POINT('Ctrl Pts',(-1.37515840835317,7.79058314353882,2.20575315620827));
#66777=CARTESIAN_POINT('Ctrl Pts',(-1.25363013962849,7.81174914723672,2.20068508373344));
#66778=CARTESIAN_POINT('Ctrl Pts',(-1.14952581524441,7.82774564309514,2.19624284960392));
#66779=CARTESIAN_POINT('Ctrl Pts',(-0.891369157628512,7.86215280926732,
2.18503411193041));
#66780=CARTESIAN_POINT('Ctrl Pts',(-0.737037383336073,7.87811890637888,
2.17816482037906));
#66781=CARTESIAN_POINT('Ctrl Pts',(-0.18858277653159,7.91860149865178,2.15339534770232));
#66782=CARTESIAN_POINT('Ctrl Pts',(0.206795517166995,7.91814653931338,2.1349170390916));
#66783=CARTESIAN_POINT('Ctrl Pts',(1.17516282775335,7.84443012758718,2.09022089405342));
#66784=CARTESIAN_POINT('Ctrl Pts',(1.74341202609434,7.73800952994934,2.06459980023237));
#66785=CARTESIAN_POINT('Ctrl Pts',(2.33278967875018,7.55933612796605,2.03952453445194));
#66786=CARTESIAN_POINT('Ctrl Pts',(2.37037352394977,7.5476353779152,2.03793133286367));
#66787=CARTESIAN_POINT('Ctrl Pts',(2.41872340293825,7.5321861335829,2.03588906901936));
#66788=CARTESIAN_POINT('Ctrl Pts',(2.42957048096277,7.52869431776472,2.03543137258639));
#66789=CARTESIAN_POINT('Ctrl Pts',(2.44677075590514,7.52311628131994,2.03470634970607));
#66790=CARTESIAN_POINT('Ctrl Pts',(2.45312889720443,7.52104542787811,2.03443850513224));
#66791=CARTESIAN_POINT('Ctrl Pts',(2.46501458808005,7.51715757022761,2.03393810814981));
#66792=CARTESIAN_POINT('Ctrl Pts',(2.47054277092266,7.51534252528196,2.03370548978492));
#66793=CARTESIAN_POINT('Ctrl Pts',(2.48296324597073,7.5112493775946,2.03318312711714));
#66794=CARTESIAN_POINT('Ctrl Pts',(2.48985441946781,7.50896788270431,2.03289349770266));
#66795=CARTESIAN_POINT('Ctrl Pts',(2.51005635140208,7.50224866169681,2.0320449826566));
#66796=CARTESIAN_POINT('Ctrl Pts',(2.52335848766041,7.49778499388771,2.0314869751491));
#66797=CARTESIAN_POINT('Ctrl Pts',(2.62192183698695,7.46441904520914,2.0273575211887));
#66798=CARTESIAN_POINT('Ctrl Pts',(2.70669762333801,7.43409809328792,2.02383445619594));
#66799=CARTESIAN_POINT('Ctrl Pts',(2.9788232352709,7.33149723114966,2.01260737217662));
#66800=CARTESIAN_POINT('Ctrl Pts',(3.16394797762751,7.25352873788172,2.00509866171235));
#66801=CARTESIAN_POINT('Ctrl Pts',(3.67797896795766,7.01360684268325,1.9844354395639));
#66802=CARTESIAN_POINT('Ctrl Pts',(3.99888278040356,6.83572690408658,1.97177831166398));
#66803=CARTESIAN_POINT('Ctrl Pts',(4.80589812982396,6.31204843409116,1.93883363853392));
#66804=CARTESIAN_POINT('Ctrl Pts',(5.26722033216891,5.93252200391318,1.91888323186619));
#66805=CARTESIAN_POINT('Ctrl Pts',(5.70277741203841,5.48299029916984,1.89410432302098));
#66806=CARTESIAN_POINT('Ctrl Pts',(5.72389170376333,5.46094465706556,1.89288631522391));
#66807=CARTESIAN_POINT('Ctrl Pts',(5.74930655088799,5.43409943644993,1.89139893042648));
#66808=CARTESIAN_POINT('Ctrl Pts',(5.75372977312431,5.42941582481192,1.89113927675374));
#66809=CARTESIAN_POINT('Ctrl Pts',(5.76097090209258,5.42172963374268,1.89071290170691));
#66810=CARTESIAN_POINT('Ctrl Pts',(5.76379220076254,5.41873024078939,1.89054645153968));
#66811=CARTESIAN_POINT('Ctrl Pts',(5.76884477963886,5.41335030771621,1.89024777440034));
#66812=CARTESIAN_POINT('Ctrl Pts',(5.77107693328892,5.41097058535856,1.89011561768633));
#66813=CARTESIAN_POINT('Ctrl Pts',(5.77576536774285,5.40596599508891,1.88983760041001));
#66814=CARTESIAN_POINT('Ctrl Pts',(5.77822132533042,5.40334084049854,1.88969171453592));
#66815=CARTESIAN_POINT('Ctrl Pts',(5.78478007051951,5.39632066179451,1.88930144978534));
#66816=CARTESIAN_POINT('Ctrl Pts',(5.78887963297001,5.39192263889081,1.88905681210221));
#66817=CARTESIAN_POINT('Ctrl Pts',(5.79788755943404,5.38223679351104,1.88851773595793));
#66818=CARTESIAN_POINT('Ctrl Pts',(5.80279370685935,5.37694692629812,1.88822312253327));
#66819=CARTESIAN_POINT('Ctrl Pts',(5.81737742326499,5.36117938077445,1.88734439219395));
#66820=CARTESIAN_POINT('Ctrl Pts',(5.82703385505538,5.35068228214799,1.88675863296099));
#66821=CARTESIAN_POINT('Ctrl Pts',(6.12759115350671,5.02218059617028,1.86840585500462));
#66822=CARTESIAN_POINT('Ctrl Pts',(6.39202193788916,4.68098840293117,1.84873902271576));
#66823=CARTESIAN_POINT('Ctrl Pts',(7.0010036513548,3.74674900432866,1.7969424353437));
#66824=CARTESIAN_POINT('Ctrl Pts',(7.29878758828355,3.12732228295483,1.76475584871739));
#66825=CARTESIAN_POINT('Ctrl Pts',(7.57441046011432,2.29140249793099,1.72711905801443));
#66826=CARTESIAN_POINT('Ctrl Pts',(7.62877695007623,2.10332806109193,1.71897514442353));
#66827=CARTESIAN_POINT('Ctrl Pts',(7.6806555245116,1.89520556203789,1.71030479795432));
#66828=CARTESIAN_POINT('Ctrl Pts',(7.68513118053164,1.87697420149655,1.70954809981223));
#66829=CARTESIAN_POINT('Ctrl Pts',(7.69132590388351,1.85134666988387,1.70848834289437));
#66830=CARTESIAN_POINT('Ctrl Pts',(7.69309926420538,1.84396376410596,1.7081834992438));
#66831=CARTESIAN_POINT('Ctrl Pts',(7.69615801959283,1.83114824703942,1.70765512933721));
#66832=CARTESIAN_POINT('Ctrl Pts',(7.69744829692394,1.82571681307334,1.70743144284098));
#66833=CARTESIAN_POINT('Ctrl Pts',(7.70012067210099,1.81441423480567,1.70696647050967));
#66834=CARTESIAN_POINT('Ctrl Pts',(7.70150180715093,1.80854286514025,1.70672521637794));
#66835=CARTESIAN_POINT('Ctrl Pts',(7.70473725186795,1.79471768837487,1.70615781159063));
#66836=CARTESIAN_POINT('Ctrl Pts',(7.70658596375103,1.78676257100049,1.70583184454492));
#66837=CARTESIAN_POINT('Ctrl Pts',(7.71258380128167,1.76077103421638,1.7047685190822));
#66838=CARTESIAN_POINT('Ctrl Pts',(7.71668196773315,1.74272285279694,1.70403282834968));
#66839=CARTESIAN_POINT('Ctrl Pts',(7.77957341712086,1.46117926570953,1.69259751136017));
#66840=CARTESIAN_POINT('Ctrl Pts',(7.82490656094049,1.19484758577534,1.68235009178677));
#66841=CARTESIAN_POINT('Ctrl Pts',(7.89337246717776,0.614396892602981,1.66092572130965));
#66842=CARTESIAN_POINT('Ctrl Pts',(7.91155649071522,0.300164557838142,1.64989621615588));
#66843=CARTESIAN_POINT('Ctrl Pts',(7.90981910850575,-0.659320240013322,
1.61671123026394));
#66844=CARTESIAN_POINT('Ctrl Pts',(7.82977573982341,-1.30167271186645,1.59527636254536));
#66845=CARTESIAN_POINT('Ctrl Pts',(7.66264358999745,-1.96710876236341,1.56825099224333));
#66846=CARTESIAN_POINT('Ctrl Pts',(7.65227916836112,-2.00704935099972,1.56660935769269));
#66847=CARTESIAN_POINT('Ctrl Pts',(7.63939039118805,-2.05516631254114,1.56460948267511));
#66848=CARTESIAN_POINT('Ctrl Pts',(7.63716448183387,-2.06342259311515,1.56426553800746));
#66849=CARTESIAN_POINT('Ctrl Pts',(7.63350075683849,-2.07692483803282,1.56370177716505));
#66850=CARTESIAN_POINT('Ctrl Pts',(7.63207090561242,-2.0821729704611,1.56348233532205));
#66851=CARTESIAN_POINT('Ctrl Pts',(7.629527042067,-2.09147215292516,1.56309295027046));
#66852=CARTESIAN_POINT('Ctrl Pts',(7.62841521134831,-2.09552380450841,1.5629231083048));
#66853=CARTESIAN_POINT('Ctrl Pts',(7.62606420325262,-2.10406450829294,1.56256469716655));
#66854=CARTESIAN_POINT('Ctrl Pts',(7.62482428896246,-2.10855335467245,1.56237609415065));
#66855=CARTESIAN_POINT('Ctrl Pts',(7.62157106104263,-2.12029058244908,1.56188235084967));
#66856=CARTESIAN_POINT('Ctrl Pts',(7.61955137380321,-2.12753718039163,1.56157692065343));
#66857=CARTESIAN_POINT('Ctrl Pts',(7.61510995586803,-2.143385456197,1.56090766672895));
#66858=CARTESIAN_POINT('Ctrl Pts',(7.61268398284403,-2.15198592704694,1.560543653489));
#66859=CARTESIAN_POINT('Ctrl Pts',(7.60552401597372,-2.1772055599211,1.55947384907795));
#66860=CARTESIAN_POINT('Ctrl Pts',(7.60075015419546,-2.19381327705722,1.55876631214438));
#66861=CARTESIAN_POINT('Ctrl Pts',(7.58408298194358,-2.25108899448655,1.55631596955899));
#66862=CARTESIAN_POINT('Ctrl Pts',(7.5719175037975,-2.29167658332965,1.55456173652297));
#66863=CARTESIAN_POINT('Ctrl Pts',(7.51736853738067,-2.46849044476569,1.54684697758201));
#66864=CARTESIAN_POINT('Ctrl Pts',(7.47163158996922,-2.60365003391587,1.54076086466285));
#66865=CARTESIAN_POINT('Ctrl Pts',(7.35115954333056,-2.93029025326666,1.52569466993713));
#66866=CARTESIAN_POINT('Ctrl Pts',(7.2725686335105,-3.12023868300716,1.516627475259));
#66867=CARTESIAN_POINT('Ctrl Pts',(6.87354471296583,-3.98740996724609,1.47429809241824));
#66868=CARTESIAN_POINT('Ctrl Pts',(6.46529365065728,-4.62009900714643,1.44117517092932));
#66869=CARTESIAN_POINT('Ctrl Pts',(5.94407549555546,-5.22053519497322,1.40883941943225));
#66870=CARTESIAN_POINT('Ctrl Pts',(5.91373322941831,-5.25488159456848,1.40698422770056));
#66871=CARTESIAN_POINT('Ctrl Pts',(5.87256887603593,-5.30067011224025,1.40450299228025));
#66872=CARTESIAN_POINT('Ctrl Pts',(5.86200880568694,-5.31234614903184,1.40386956960724));
#66873=CARTESIAN_POINT('Ctrl Pts',(5.8453983445093,-5.33060213234659,1.40287804094524));
#66874=CARTESIAN_POINT('Ctrl Pts',(5.83937155426294,-5.33720345790456,1.40251927010259));
#66875=CARTESIAN_POINT('Ctrl Pts',(5.82778764329796,-5.34984855793779,1.40183156962037));
#66876=CARTESIAN_POINT('Ctrl Pts',(5.82223227783044,-5.3558939227364,1.40150259109513));
#66877=CARTESIAN_POINT('Ctrl Pts',(5.80920940520938,-5.37002124461455,1.40073332371105));
#66878=CARTESIAN_POINT('Ctrl Pts',(5.80173442016159,-5.37809629887392,1.40029324620418));
#66879=CARTESIAN_POINT('Ctrl Pts',(5.78033645266236,-5.4011155023088,1.39903766976062));
#66880=CARTESIAN_POINT('Ctrl Pts',(5.76637237913592,-5.4160213963549,1.39822334255135));
#66881=CARTESIAN_POINT('Ctrl Pts',(5.67656728734826,-5.51114245201953,1.39301838556512));
#66882=CARTESIAN_POINT('Ctrl Pts',(5.59911086875452,-5.58981803066453,1.38867520781155));
#66883=CARTESIAN_POINT('Ctrl Pts',(5.36789261565527,-5.81504589609741,1.37611634827837));
#66884=CARTESIAN_POINT('Ctrl Pts',(5.20984355800252,-5.95706011680667,1.36803777709649));
#66885=CARTESIAN_POINT('Ctrl Pts',(4.74733624604546,-6.34014048954591,1.34560570135726));
#66886=CARTESIAN_POINT('Ctrl Pts',(4.43058417981132,-6.5654029178304,1.33164555352016));
#66887=CARTESIAN_POINT('Ctrl Pts',(3.73760325290378,-6.98515223639266,1.30241278465072));
#66888=CARTESIAN_POINT('Ctrl Pts',(3.35973445799983,-7.17454995580319,1.28717411846075));
#66889=CARTESIAN_POINT('Ctrl Pts',(2.90200442161702,-7.35985412200094,1.2679037073622));
#66890=CARTESIAN_POINT('Ctrl Pts',(2.83504904818616,-7.38590406187277,1.26506461942681));
#66891=CARTESIAN_POINT('Ctrl Pts',(2.7571310664331,-7.41500355789432,1.26172849785012));
#66892=CARTESIAN_POINT('Ctrl Pts',(2.74650399639461,-7.41894637242531,1.26127280229689));
#66893=CARTESIAN_POINT('Ctrl Pts',(2.73071053210617,-7.42476741783605,1.26059450114377));
#66894=CARTESIAN_POINT('Ctrl Pts',(2.72555056408974,-7.42666313639438,1.26037272079089));
#66895=CARTESIAN_POINT('Ctrl Pts',(2.71652082347185,-7.42996989104575,1.25998431246967));
#66896=CARTESIAN_POINT('Ctrl Pts',(2.71265191277623,-7.43138328753252,1.25981779712084));
#66897=CARTESIAN_POINT('Ctrl Pts',(2.7044871926356,-7.43435881022194,1.25946618591878));
#66898=CARTESIAN_POINT('Ctrl Pts',(2.70019113089328,-7.43592023563773,1.25928105648296));
#66899=CARTESIAN_POINT('Ctrl Pts',(2.6891100688137,-7.43993683454291,1.25880322557751));
#66900=CARTESIAN_POINT('Ctrl Pts',(2.68232306885573,-7.44238644642539,1.25851025474875));
#66901=CARTESIAN_POINT('Ctrl Pts',(2.66760772934499,-7.44767486668801,1.25787436586238));
#66902=CARTESIAN_POINT('Ctrl Pts',(2.65967819566742,-7.45051030548828,1.25753128269091));
#66903=CARTESIAN_POINT('Ctrl Pts',(2.63684564945331,-7.45863366061509,1.25654213423054));
#66904=CARTESIAN_POINT('Ctrl Pts',(2.62193135279596,-7.46388953814629,1.25589447110958));
#66905=CARTESIAN_POINT('Ctrl Pts',(2.57234896496281,-7.48119568585069,1.25373591182469));
#66906=CARTESIAN_POINT('Ctrl Pts',(2.53761431252072,-7.4930488896003,1.25221481697049));
#66907=CARTESIAN_POINT('Ctrl Pts',(2.38740440631949,-7.54314375160728,1.2455963752325));
#66908=CARTESIAN_POINT('Ctrl Pts',(2.27114407840564,-7.57895900227316,1.24037429642332));
#66909=CARTESIAN_POINT('Ctrl Pts',(2.05287139227233,-7.64072705638989,1.2304463449608));
#66910=CARTESIAN_POINT('Ctrl Pts',(1.95107447212419,-7.66735274599372,1.22576686669231));
#66911=CARTESIAN_POINT('Ctrl Pts',(0.927843377872795,-7.91328927259855,
1.17843672060966));
#66912=CARTESIAN_POINT('Ctrl Pts',(-0.0257557132769284,-7.96751163361469,
1.13318083180045));
#66913=CARTESIAN_POINT('Ctrl Pts',(-1.02127807460617,-7.84499730013908,
1.09208424949607));
#66914=CARTESIAN_POINT('Ctrl Pts',(-1.07620374946437,-7.8376512554759,1.08983249307969));
#66915=CARTESIAN_POINT('Ctrl Pts',(-1.14257068903076,-7.8280641765508,1.08713026245907));
#66916=CARTESIAN_POINT('Ctrl Pts',(-1.15408924000219,-7.8263742920518,1.08666194505183));
#66917=CARTESIAN_POINT('Ctrl Pts',(-1.17295832777921,-7.82356344940469,
1.08589587639087));
#66918=CARTESIAN_POINT('Ctrl Pts',(-1.18031106883719,-7.82245754649716,
1.08559763645871));
#66919=CARTESIAN_POINT('Ctrl Pts',(-1.19348177870301,-7.82045758838228,
1.08506390035953));
#66920=CARTESIAN_POINT('Ctrl Pts',(-1.19930032437965,-7.81956740363072,
1.08482827854389));
#66921=CARTESIAN_POINT('Ctrl Pts',(-1.21162604848919,-7.81766759853267,
1.0843295113037));
#66922=CARTESIAN_POINT('Ctrl Pts',(-1.21813297283708,-7.8166563454773,1.0840664192081));
#66923=CARTESIAN_POINT('Ctrl Pts',(-1.23545458614173,-7.8139422075249,1.08336662881469));
#66924=CARTESIAN_POINT('Ctrl Pts',(-1.24626703363144,-7.81222499286318,
1.08293039753233));
#66925=CARTESIAN_POINT('Ctrl Pts',(-1.29652321065315,-7.80413640082477,
1.08090552123602));
#66926=CARTESIAN_POINT('Ctrl Pts',(-1.33592221084362,-7.7974886538103,1.07932590098434));
#66927=CARTESIAN_POINT('Ctrl Pts',(-1.62809948587043,-7.7459104099924,1.06766791844162));
#66928=CARTESIAN_POINT('Ctrl Pts',(-1.87861681302469,-7.68899531425484,
1.05799268345513));
#66929=CARTESIAN_POINT('Ctrl Pts',(-2.51712944630752,-7.5108536480039,1.03386666648871));
#66930=CARTESIAN_POINT('Ctrl Pts',(-2.89934727401863,-7.37174803807389,
1.01997259875936));
#66931=CARTESIAN_POINT('Ctrl Pts',(-3.42574524311268,-7.13286363509513,
1.00036078557428));
#66932=CARTESIAN_POINT('Ctrl Pts',(-3.5799317212013,-7.05673878914083,0.99454802385252));
#66933=CARTESIAN_POINT('Ctrl Pts',(-3.91319750011234,-6.87846353217755,
0.981627354904344));
#66934=CARTESIAN_POINT('Ctrl Pts',(-4.09100892432498,-6.7742170113582,0.974496716787072));
#66935=CARTESIAN_POINT('Ctrl Pts',(-4.40109634795412,-6.57575525997807,
0.961305585218286));
#66936=CARTESIAN_POINT('Ctrl Pts',(-4.53492561757346,-6.4841846990211,0.955343457574303));
#66937=CARTESIAN_POINT('Ctrl Pts',(-4.74183583189245,-6.33306953341771,
0.945542051319331));
#66938=CARTESIAN_POINT('Ctrl Pts',(-4.81683176177043,-6.27621759073707,
0.941862203444714));
#66939=CARTESIAN_POINT('Ctrl Pts',(-4.89791869603541,-6.21243878340461,
0.937721386082936));
#66940=CARTESIAN_POINT('Ctrl Pts',(-4.90503482280005,-6.20682177739849,
0.937356599447361));
#66941=CARTESIAN_POINT('Ctrl Pts',(-4.91556323266419,-6.19848192409276,
0.936814802780212));
#66942=CARTESIAN_POINT('Ctrl Pts',(-4.91898296271878,-6.19576844870096,
0.936638494441916));
#66943=CARTESIAN_POINT('Ctrl Pts',(-4.92483821928573,-6.19111453705791,
0.936336054851823));
#66944=CARTESIAN_POINT('Ctrl Pts',(-4.92727485126152,-6.18917548928605,
0.936210028530215));
#66945=CARTESIAN_POINT('Ctrl Pts',(-4.93203049294346,-6.18538640806916,
0.935963732861911));
#66946=CARTESIAN_POINT('Ctrl Pts',(-4.93434960847619,-6.18353650767301,
0.935843473508284));
#66947=CARTESIAN_POINT('Ctrl Pts',(-4.93914824708803,-6.17970433522073,
0.935594323276705));
#66948=CARTESIAN_POINT('Ctrl Pts',(-4.94162761886262,-6.17772187411384,
0.935465418269891));
#66949=CARTESIAN_POINT('Ctrl Pts',(-4.94727535728616,-6.17320046847667,
0.935171392606627));
#66950=CARTESIAN_POINT('Ctrl Pts',(-4.95044296122101,-6.17066057828451,
0.935006201648206));
#66951=CARTESIAN_POINT('Ctrl Pts',(-4.96609302198877,-6.15809203266822,
0.93418865538541));
#66952=CARTESIAN_POINT('Ctrl Pts',(-4.9785468850579,-6.1480280002567,0.933533689045903));
#66953=CARTESIAN_POINT('Ctrl Pts',(-5.13541759084523,-6.02047075184343,
0.925229126891528));
#66954=CARTESIAN_POINT('Ctrl Pts',(-5.27566483766739,-5.89796009111895,
0.917220389129484));
#66955=CARTESIAN_POINT('Ctrl Pts',(-5.50066023271181,-5.68696886726174,
0.903577190709815));
#66956=CARTESIAN_POINT('Ctrl Pts',(-5.58791566751331,-5.60125652928248,
0.898072169212023));
#66957=CARTESIAN_POINT('Ctrl Pts',(-6.22182442970545,-4.94899951916871,
0.856684368956515));
#66958=CARTESIAN_POINT('Ctrl Pts',(-6.68329652895918,-4.30553807599008,
0.819208773506188));
#66959=CARTESIAN_POINT('Ctrl Pts',(-7.12258477876593,-3.44730283969861,
0.778240032815006));
#66960=CARTESIAN_POINT('Ctrl Pts',(-7.19776856344398,-3.28743729392084,
0.770917695881308));
#66961=CARTESIAN_POINT('Ctrl Pts',(-7.27415499052423,-3.10980231314302,
0.763108373812415));
#66962=CARTESIAN_POINT('Ctrl Pts',(-7.28071949563079,-3.09440218516111,
0.762433969287101));
#66963=CARTESIAN_POINT('Ctrl Pts',(-7.29036759828207,-3.07156736220434,
0.761437847649765));
#66964=CARTESIAN_POINT('Ctrl Pts',(-7.2934887917746,-3.06414866209062,0.761114824615793));
#66965=CARTESIAN_POINT('Ctrl Pts',(-7.29880023897846,-3.05146989770226,
0.760563794382481));
#66966=CARTESIAN_POINT('Ctrl Pts',(-7.30099613849812,-3.04621221370423,
0.760335591423101));
#66967=CARTESIAN_POINT('Ctrl Pts',(-7.30524696690901,-3.03600337433877,
0.759893071889591));
#66968=CARTESIAN_POINT('Ctrl Pts',(-7.30730254709344,-3.03105249409005,
0.759678732819961));
#66969=CARTESIAN_POINT('Ctrl Pts',(-7.31219067649834,-3.01924552490682,
0.759168203010356));
#66970=CARTESIAN_POINT('Ctrl Pts',(-7.31501861993959,-3.0123875281022,0.758872171771544));
#66971=CARTESIAN_POINT('Ctrl Pts',(-7.32340830906583,-2.99196035961901,
0.757991918077854));
#66972=CARTESIAN_POINT('Ctrl Pts',(-7.32894198962146,-2.97837965521888,
0.757408665433738));
#66973=CARTESIAN_POINT('Ctrl Pts',(-7.37410611594611,-2.86665025942511,
0.752626282645348));
#66974=CARTESIAN_POINT('Ctrl Pts',(-7.41180171080291,-2.76772852961935,
0.748494134567827));
#66975=CARTESIAN_POINT('Ctrl Pts',(-7.55602591054977,-2.36515028115023,
0.732061334349842));
#66976=CARTESIAN_POINT('Ctrl Pts',(-7.64597131931583,-2.05587154157563,
0.720324350296821));
#66977=CARTESIAN_POINT('Ctrl Pts',(-7.84623618187793,-1.1687019970341,0.688197761162855));
#66978=CARTESIAN_POINT('Ctrl Pts',(-7.91134728837762,-0.582879817310929,
0.668873487582277));
#66979=CARTESIAN_POINT('Ctrl Pts',(-7.91099860705843,0.00469458407978809,
0.647721152219829));
#66980=CARTESIAN_POINT('Origin',(0.,0.,183.));
#66981=CARTESIAN_POINT('',(-4.,-4.89858719658941E-16,184.));
#66982=CARTESIAN_POINT('Origin',(0.,0.,184.));
#66983=CARTESIAN_POINT('',(-4.,-4.89858719658941E-16,182.));
#66984=CARTESIAN_POINT('',(-4.,-4.89858719658941E-16,183.));
#66985=CARTESIAN_POINT('Origin',(0.,0.,182.));
#66986=CARTESIAN_POINT('Origin',(8.,0.,182.));
#66987=CARTESIAN_POINT('',(-5.,6.12323399573677E-16,182.));
#66988=CARTESIAN_POINT('Origin',(0.,0.,182.));
#66989=CARTESIAN_POINT('Origin',(4.,0.,184.));
#66990=CARTESIAN_POINT('',(-5.,-6.12323399573677E-16,184.));
#66991=CARTESIAN_POINT('Origin',(0.,0.,184.));
#66992=CARTESIAN_POINT('Origin',(0.,0.,158.));
#66993=CARTESIAN_POINT('',(-5.,-6.12323399573677E-16,185.));
#66994=CARTESIAN_POINT('Origin',(0.,0.,185.));
#66995=CARTESIAN_POINT('',(-5.,-6.12323399573677E-16,158.));
#66996=CARTESIAN_POINT('Origin',(0.,0.,158.));
#66997=CARTESIAN_POINT('',(-5.,-6.12323399573677E-16,158.));
#66998=CARTESIAN_POINT('',(-5.,-6.12323399573677E-16,158.));
#66999=CARTESIAN_POINT('Origin',(0.,0.,158.));
#67000=CARTESIAN_POINT('Origin',(0.,0.,185.));
#67001=CARTESIAN_POINT('Origin',(0.,0.,154.));
#67002=CARTESIAN_POINT('',(-10.,-1.22464679914735E-15,154.));
#67003=CARTESIAN_POINT('Origin',(0.,0.,154.));
#67004=CARTESIAN_POINT('',(6.04416524408958,-3.53101493938209,154.));
#67005=CARTESIAN_POINT('',(-6.07123506171349,-3.48426514564655,154.000000121761));
#67006=CARTESIAN_POINT('Origin',(0.,0.,154.));
#67007=CARTESIAN_POINT('Origin',(-1.40492233861576,-0.171210964340612,153.999999999995));
#67008=CARTESIAN_POINT('Origin',(1.19342779692842,-0.571021005665173,153.999999999995));
#67009=CARTESIAN_POINT('Origin',(0.,0.,154.));
#67010=CARTESIAN_POINT('',(-10.,-1.22464679914735E-15,158.));
#67011=CARTESIAN_POINT('Origin',(0.,0.,158.));
#67012=CARTESIAN_POINT('',(-10.,-1.22464679914735E-15,154.));
#67013=CARTESIAN_POINT('Origin',(0.,0.,158.));
#67014=CARTESIAN_POINT('Origin',(0.,18.,-5.));
#67015=CARTESIAN_POINT('',(-8.,18.,0.));
#67016=CARTESIAN_POINT('Origin',(0.,18.,0.));
#67017=CARTESIAN_POINT('',(-8.,18.,-10.));
#67018=CARTESIAN_POINT('',(-8.,18.,-5.));
#67019=CARTESIAN_POINT('Origin',(0.,18.,-10.));
#67020=CARTESIAN_POINT('Origin',(18.,0.,-5.));
#67021=CARTESIAN_POINT('',(10.,9.79717439317883E-16,0.));
#67022=CARTESIAN_POINT('Origin',(18.,0.,0.));
#67023=CARTESIAN_POINT('',(10.,9.79717439317883E-16,-10.));
#67024=CARTESIAN_POINT('',(10.,9.79717439317883E-16,-5.));
#67025=CARTESIAN_POINT('Origin',(18.,0.,-10.));
#67026=CARTESIAN_POINT('Origin',(-18.,0.,-5.));
#67027=CARTESIAN_POINT('',(-26.,9.79717439317883E-16,0.));
#67028=CARTESIAN_POINT('Origin',(-18.,0.,0.));
#67029=CARTESIAN_POINT('',(-26.,9.79717439317883E-16,-10.));
#67030=CARTESIAN_POINT('',(-26.,9.79717439317883E-16,-5.));
#67031=CARTESIAN_POINT('Origin',(-18.,0.,-10.));
#67032=CARTESIAN_POINT('Origin',(0.,-18.,-5.));
#67033=CARTESIAN_POINT('',(-8.,-18.,0.));
#67034=CARTESIAN_POINT('Origin',(0.,-18.,0.));
#67035=CARTESIAN_POINT('',(-8.,-18.,-10.));
#67036=CARTESIAN_POINT('',(-8.,-18.,-5.));
#67037=CARTESIAN_POINT('Origin',(0.,-18.,-10.));
#67038=CARTESIAN_POINT('Origin',(0.,0.,153.5));
#67039=CARTESIAN_POINT('Ctrl Pts',(-6.07123482803126,-3.48426499407615,
154.000000365283));
#67040=CARTESIAN_POINT('Ctrl Pts',(-6.37729082463053,-2.98510698007377,
153.983009074227));
#67041=CARTESIAN_POINT('Ctrl Pts',(-6.6197085761198,-2.44959580558649,153.965827313444));
#67042=CARTESIAN_POINT('Ctrl Pts',(-6.9846747189001,-1.27750436456966,153.928602162082));
#67043=CARTESIAN_POINT('Ctrl Pts',(-7.0919311032529,-0.639071943781941,
153.908394854784));
#67044=CARTESIAN_POINT('Ctrl Pts',(-7.13926079552257,1.02962958383913,153.860216444196));
#67045=CARTESIAN_POINT('Ctrl Pts',(-6.9390178381147,1.95420836025049,153.839610574055));
#67046=CARTESIAN_POINT('Ctrl Pts',(-6.36073513248416,3.46730423446295,153.798161280371));
#67047=CARTESIAN_POINT('Ctrl Pts',(-5.96341174680285,4.15209317811089,153.775889324813));
#67048=CARTESIAN_POINT('Ctrl Pts',(-4.9660733049039,5.37226764090361,153.726971778021));
#67049=CARTESIAN_POINT('Ctrl Pts',(-4.25430228608747,6.0418766964822,153.69407810596));
#67050=CARTESIAN_POINT('Ctrl Pts',(-2.49085845485886,6.97949242594648,153.642859236));
#67051=CARTESIAN_POINT('Ctrl Pts',(-1.63249269525403,7.24793969981517,153.623916701874));
#67052=CARTESIAN_POINT('Ctrl Pts',(0.0560132140757014,7.46364414088888,
153.580474698423));
#67053=CARTESIAN_POINT('Ctrl Pts',(0.876036956523461,7.43596342213082,153.556771317729));
#67054=CARTESIAN_POINT('Ctrl Pts',(2.26944149094137,7.16065895049613,153.512935028995));
#67055=CARTESIAN_POINT('Ctrl Pts',(3.1051275024235,6.92367809008591,153.484990573071));
#67056=CARTESIAN_POINT('Ctrl Pts',(4.80872094961789,5.91228941939438,153.436000484306));
#67057=CARTESIAN_POINT('Ctrl Pts',(5.51398732222406,5.28896519422956,153.416367441624));
#67058=CARTESIAN_POINT('Ctrl Pts',(6.71662248272036,3.7642603069226,153.367120384876));
#67059=CARTESIAN_POINT('Ctrl Pts',(7.18428961469687,2.85171462781057,153.336756402359));
#67060=CARTESIAN_POINT('Ctrl Pts',(7.6725689600507,1.12984169336891,153.28386581576));
#67061=CARTESIAN_POINT('Ctrl Pts',(7.76711987065858,0.359391098290495,153.263717416961));
#67062=CARTESIAN_POINT('Ctrl Pts',(7.71591129163788,-1.26410811526187,153.226979141127));
#67063=CARTESIAN_POINT('Ctrl Pts',(7.54993713581411,-2.10059887369074,153.208958867732));
#67064=CARTESIAN_POINT('Ctrl Pts',(7.05995918060561,-3.42583218192886,153.173305452414));
#67065=CARTESIAN_POINT('Ctrl Pts',(6.80641914608851,-3.93660409196822,153.157670685671));
#67066=CARTESIAN_POINT('Ctrl Pts',(6.1501911740556,-4.965772420327,153.122315830429));
#67067=CARTESIAN_POINT('Ctrl Pts',(5.73217936663422,-5.47174237691816,153.102402843541));
#67068=CARTESIAN_POINT('Ctrl Pts',(5.25622342069531,-5.91850150513378,153.0844112844));
#67069=CARTESIAN_POINT('Ctrl Pts',(-1.31596378579611,-7.79949774689402,
153.090263860954));
#67070=CARTESIAN_POINT('Ctrl Pts',(-1.1121036545036,-7.81524681765638,153.108651036666));
#67071=CARTESIAN_POINT('Ctrl Pts',(-0.90819989047042,-7.82301474609582,
153.127052284549));
#67072=CARTESIAN_POINT('Ctrl Pts',(-0.704669024892965,-7.82273003893546,
153.145595904417));
#67073=CARTESIAN_POINT('Ctrl Pts',(-0.505071248433598,-7.82245083353834,
153.163781182029));
#67074=CARTESIAN_POINT('Ctrl Pts',(-0.305831889755628,-7.81442791085797,
153.182103714959));
#67075=CARTESIAN_POINT('Ctrl Pts',(-0.107316191403576,-7.79856092090086,
153.200700723659));
#67076=CARTESIAN_POINT('Ctrl Pts',(0.0418228097860945,-7.78664051836476,
153.214672108922));
#67077=CARTESIAN_POINT('Ctrl Pts',(0.190553974279541,-7.77029230854503,
153.228798779438));
#67078=CARTESIAN_POINT('Ctrl Pts',(0.338731670168721,-7.74945715955899,
153.243143329143));
#67079=CARTESIAN_POINT('Ctrl Pts',(0.540870352871086,-7.7210345987635,153.26271164787));
#67080=CARTESIAN_POINT('Ctrl Pts',(0.741986038978563,-7.68426235743513,
153.282684506573));
#67081=CARTESIAN_POINT('Ctrl Pts',(0.941626984869757,-7.63924361945789,
153.302941831059));
#67082=CARTESIAN_POINT('Ctrl Pts',(1.07092990212845,-7.61008600288892,153.316062041145));
#67083=CARTESIAN_POINT('Ctrl Pts',(1.19961276752827,-7.57746829045134,153.329301877301));
#67084=CARTESIAN_POINT('Ctrl Pts',(1.32753676621016,-7.54141321421978,153.342633146228));
#67085=CARTESIAN_POINT('Ctrl Pts',(1.35930484500025,-7.53245945640804,153.34594377446));
#67086=CARTESIAN_POINT('Ctrl Pts',(1.3910260623527,-7.52329370259455,153.349260060887));
#67087=CARTESIAN_POINT('Ctrl Pts',(1.42269816996776,-7.51391628179592,153.35258161386));
#67088=CARTESIAN_POINT('Ctrl Pts',(1.44498487760559,-7.50731767338387,153.354918890587));
#67089=CARTESIAN_POINT('Ctrl Pts',(1.46724583341159,-7.50061464406909,153.357258626739));
#67090=CARTESIAN_POINT('Ctrl Pts',(1.48946890932793,-7.49381093413642,153.359599490312));
#67091=CARTESIAN_POINT('Ctrl Pts',(1.67899517349363,-7.43578648554704,153.379563204141));
#67092=CARTESIAN_POINT('Ctrl Pts',(1.86599674061145,-7.37037383453255,153.399630360127));
#67093=CARTESIAN_POINT('Ctrl Pts',(2.05003895801424,-7.29779065970799,153.419735608681));
#67094=CARTESIAN_POINT('Ctrl Pts',(2.23578121112045,-7.22453701921305,153.440026573539));
#67095=CARTESIAN_POINT('Ctrl Pts',(2.41850899147636,-7.1439790360393,153.460356086658));
#67096=CARTESIAN_POINT('Ctrl Pts',(2.59773797487726,-7.05633057828242,153.480688607584));
#67097=CARTESIAN_POINT('Ctrl Pts',(2.77608539636706,-6.96911323127816,153.500921120264));
#67098=CARTESIAN_POINT('Ctrl Pts',(2.95096799697956,-6.8748745111543,153.521156467461));
#67099=CARTESIAN_POINT('Ctrl Pts',(3.12187594854324,-6.77382454579522,153.54139366803));
#67100=CARTESIAN_POINT('Ctrl Pts',(3.28970994734263,-6.67459206650105,153.56126688203));
#67101=CARTESIAN_POINT('Ctrl Pts',(3.45371058847674,-6.56879099008516,153.581141863008));
#67102=CARTESIAN_POINT('Ctrl Pts',(3.61336928750934,-6.45662439871814,153.60105168054));
#67103=CARTESIAN_POINT('Ctrl Pts',(3.68030089588206,-6.40960227958922,153.609398210469));
#67104=CARTESIAN_POINT('Ctrl Pts',(3.74646915874975,-6.36146152991643,153.617751279783));
#67105=CARTESIAN_POINT('Ctrl Pts',(3.81183546444604,-6.31221736887221,153.626115154147));
#67106=CARTESIAN_POINT('Ctrl Pts',(3.84959742054882,-6.28376913659318,153.630946944061));
#67107=CARTESIAN_POINT('Ctrl Pts',(3.88709173129729,-6.25495266134965,153.635782366191));
#67108=CARTESIAN_POINT('Ctrl Pts',(3.92431278871413,-6.2257709286127,153.640621322474));
#67109=CARTESIAN_POINT('Ctrl Pts',(3.95252988483424,-6.20364840403291,153.644289710855));
#67110=CARTESIAN_POINT('Ctrl Pts',(3.98058993694438,-6.18131596302765,153.647960131348));
#67111=CARTESIAN_POINT('Ctrl Pts',(4.00849044342186,-6.15877490889018,153.651632561352));
#67112=CARTESIAN_POINT('Ctrl Pts',(4.0268583028332,-6.14393536059329,153.654050247858));
#67113=CARTESIAN_POINT('Ctrl Pts',(4.04515052636911,-6.12901062189163,153.65646795302));
#67114=CARTESIAN_POINT('Ctrl Pts',(4.06336326620589,-6.11400400376567,153.658885235115));
#67115=CARTESIAN_POINT('Ctrl Pts',(4.21292912360686,-5.99076731742344,153.67873633233));
#67116=CARTESIAN_POINT('Ctrl Pts',(4.35721037603448,-5.86195109305672,153.698567169177));
#67117=CARTESIAN_POINT('Ctrl Pts',(4.49593593538605,-5.7278629388539,153.71838934154));
#67118=CARTESIAN_POINT('Ctrl Pts',(4.63479042340091,-5.59365016589614,153.73822993622));
#67119=CARTESIAN_POINT('Ctrl Pts',(4.76807887264492,-5.4541553608342,153.758061800089));
#67120=CARTESIAN_POINT('Ctrl Pts',(4.89550039371483,-5.30967073548228,153.777913914657));
#67121=CARTESIAN_POINT('Ctrl Pts',(5.02145670136866,-5.16684753129144,153.797537750798));
#67122=CARTESIAN_POINT('Ctrl Pts',(5.14168023766823,-5.01914842940895,153.817181405182));
#67123=CARTESIAN_POINT('Ctrl Pts',(5.25585219203421,-4.86684331841067,153.836889910767));
#67124=CARTESIAN_POINT('Ctrl Pts',(5.36870538178194,-4.71629743622369,153.856370769554));
#67125=CARTESIAN_POINT('Ctrl Pts',(5.47564609616922,-4.56125128584607,153.875915068782));
#67126=CARTESIAN_POINT('Ctrl Pts',(5.57633788489941,-4.4019549671733,153.895582237819));
#67127=CARTESIAN_POINT('Ctrl Pts',(5.62032802259992,-4.33236173537188,153.904174412862));
#67128=CARTESIAN_POINT('Ctrl Pts',(5.66312508875151,-4.26195716942302,153.912790238856));
#67129=CARTESIAN_POINT('Ctrl Pts',(5.70469916221104,-4.19076149173311,153.921435568427));
#67130=CARTESIAN_POINT('Ctrl Pts',(5.73054731178932,-4.14649648777464,153.926810691751));
#67131=CARTESIAN_POINT('Ctrl Pts',(5.75592268161,-4.10192566619461,153.932197230444));
#67132=CARTESIAN_POINT('Ctrl Pts',(5.78081783980179,-4.05705380882406,153.937596690597));
#67133=CARTESIAN_POINT('Ctrl Pts',(5.79587442276576,-4.02991532518632,153.940862282209));
#67134=CARTESIAN_POINT('Ctrl Pts',(5.81075818838583,-4.00266131967346,153.944133246818));
#67135=CARTESIAN_POINT('Ctrl Pts',(5.82545270270185,-3.97532066537712,153.947406605795));
#67136=CARTESIAN_POINT('Ctrl Pts',(5.90369690306284,-3.82973928808508,153.964836331614));
#67137=CARTESIAN_POINT('Ctrl Pts',(5.97664922546305,-3.6815768948131,153.982348779896));
#67138=CARTESIAN_POINT('Ctrl Pts',(6.04416524408959,-3.53101493938209,154.));
#67139=CARTESIAN_POINT('Ctrl Pts',(4.60531350164922,-6.46554420335129,-0.676259423350488));
#67140=CARTESIAN_POINT('Ctrl Pts',(5.68236987471326,-5.69840091938804,-0.623235491717399));
#67141=CARTESIAN_POINT('Ctrl Pts',(7.42535730630537,-3.61951054181251,-0.517244370183029));
#67142=CARTESIAN_POINT('Ctrl Pts',(8.58296678012314,1.73151873861316,-0.305318868846102));
#67143=CARTESIAN_POINT('Ctrl Pts',(4.71465848402119,8.11444401416975,-0.0404829193397082));
#67144=CARTESIAN_POINT('Ctrl Pts',(-4.27978750802599,8.35543959967712,0.277320220067964));
#67145=CARTESIAN_POINT('Ctrl Pts',(-9.33794990612123,0.932116542185654,
0.595123359475637));
#67146=CARTESIAN_POINT('Ctrl Pts',(-5.83855067917698,-7.35186461183959,
0.912926498883309));
#67147=CARTESIAN_POINT('Ctrl Pts',(1.53223224477109,-8.62179203470423,1.17776244838971));
#67148=CARTESIAN_POINT('Ctrl Pts',(6.06593278951601,-5.59317548027687,1.38963120799482));
#67149=CARTESIAN_POINT('Ctrl Pts',(8.71699111872767,-0.828587516564991,
1.60149996759994));
#67150=CARTESIAN_POINT('Ctrl Pts',(6.8565807090538,6.41311451068115,1.86633591710633));
#67151=CARTESIAN_POINT('Ctrl Pts',(-1.68792736490162,9.23452166984993,2.184139056514));
#67152=CARTESIAN_POINT('Ctrl Pts',(-8.66924682276468,3.58420186719372,2.50194219592167));
#67153=CARTESIAN_POINT('Ctrl Pts',(-7.7163283608382,-5.3465045633832,2.81974533532935));
#67154=CARTESIAN_POINT('Ctrl Pts',(0.326212197437957,-9.38266708925739,
3.13754847473702));
#67155=CARTESIAN_POINT('Ctrl Pts',(6.75680014268004,-5.56896829319403,3.40238442424342));
#67156=CARTESIAN_POINT('Ctrl Pts',(8.24512830401543,-0.323374826084047,
3.61425318384852));
#67157=CARTESIAN_POINT('Ctrl Pts',(7.17220337466533,5.02266100663792,3.82612194345365));
#67158=CARTESIAN_POINT('Ctrl Pts',(1.06007560991606,9.3283081635453,4.09095789296003));
#67159=CARTESIAN_POINT('Ctrl Pts',(-7.27390854203853,5.93440838897662,4.40876103236771));
#67160=CARTESIAN_POINT('Ctrl Pts',(-8.92329103308646,-2.89418249863981,
4.72656417177538));
#67161=CARTESIAN_POINT('Ctrl Pts',(-2.40607174040283,-9.07401688178992,
5.04436731118306));
#67162=CARTESIAN_POINT('Ctrl Pts',(6.33339962621769,-6.93030482747814,5.36217045059073));
#67163=CARTESIAN_POINT('Ctrl Pts',(8.75483483974857,0.143116954380555,5.62700640009711));
#67164=CARTESIAN_POINT('Ctrl Pts',(6.4857259272773,5.10118745343669,5.83887515970225));
#67165=CARTESIAN_POINT('Ctrl Pts',(2.20189237340188,8.47462592794457,6.05074391930734));
#67166=CARTESIAN_POINT('Ctrl Pts',(-5.2429169905794,7.7879971588325,6.31557986881376));
#67167=CARTESIAN_POINT('Ctrl Pts',(-9.38545862533877,-0.200320147439794,
6.63338300822141));
#67168=CARTESIAN_POINT('Ctrl Pts',(-4.91519471530038,-7.99013595043972,
6.95118614762909));
#67169=CARTESIAN_POINT('Ctrl Pts',(4.05345806777821,-8.46737500993547,7.26898928703676));
#67170=CARTESIAN_POINT('Ctrl Pts',(9.3154477429652,-1.16769493639905,7.58679242644443));
#67171=CARTESIAN_POINT('Ctrl Pts',(6.57115862390735,5.78683757551102,7.85162837595083));
#67172=CARTESIAN_POINT('Ctrl Pts',(1.62843632194056,8.08918719373227,8.06349713555594));
#67173=CARTESIAN_POINT('Ctrl Pts',(-3.82014314373728,7.87871316550388,8.27536589516105));
#67174=CARTESIAN_POINT('Ctrl Pts',(-9.04164929613513,2.52777691600338,8.54020184466747));
#67175=CARTESIAN_POINT('Ctrl Pts',(-7.0140760084076,-6.23936692209582,8.85800498407512));
#67176=CARTESIAN_POINT('Ctrl Pts',(1.44062724585838,-9.26962808007599,9.1758081234828));
#67177=CARTESIAN_POINT('Ctrl Pts',(8.57686766441828,-3.81632059811431,9.49361126289047));
#67178=CARTESIAN_POINT('Ctrl Pts',(7.84800405600511,5.15266052317008,9.81141440229815));
#67179=CARTESIAN_POINT('Ctrl Pts',(1.24879103801572,8.66649500826888,10.0762503518046));
#67180=CARTESIAN_POINT('Ctrl Pts',(-4.00667033342535,7.21341438901849,10.2881191114097));
#67181=CARTESIAN_POINT('Ctrl Pts',(-8.01750035760689,3.51956002943052,10.4999878710148));
#67182=CARTESIAN_POINT('Ctrl Pts',(-8.52166878717728,-3.93982730735651,
10.7648238205212));
#67183=CARTESIAN_POINT('Ctrl Pts',(-1.292444002806,-9.29820145726888,11.0826269599288));
#67184=CARTESIAN_POINT('Ctrl Pts',(7.10833853462331,-6.12151410044222,11.4004300993365));
#67185=CARTESIAN_POINT('Ctrl Pts',(9.00356579477459,2.65758627696441,11.7182332387442));
#67186=CARTESIAN_POINT('Ctrl Pts',(2.63198810748128,9.01186533034181,12.0360363781519));
#67187=CARTESIAN_POINT('Ctrl Pts',(-4.67005731023871,7.40663077951727,12.3008723276583));
#67188=CARTESIAN_POINT('Ctrl Pts',(-7.72800462548672,2.89217890471641,12.5127410872634));
#67189=CARTESIAN_POINT('Ctrl Pts',(-8.38532598247424,-2.5206989016241,12.7246098468685));
#67190=CARTESIAN_POINT('Ctrl Pts',(-3.93134236556828,-8.52558650972633,
12.9894457963749));
#67191=CARTESIAN_POINT('Ctrl Pts',(5.04651945463183,-7.91578190922199,13.3072489357826));
#67192=CARTESIAN_POINT('Ctrl Pts',(9.38077626567956,-0.0494798745878378,
13.6250520751902));
#67193=CARTESIAN_POINT('Ctrl Pts',(5.12974155706928,7.86210616807101,13.9428552145979));
#67194=CARTESIAN_POINT('Ctrl Pts',(-3.84118794702279,8.56658352470727,14.2606583540055));
#67195=CARTESIAN_POINT('Ctrl Pts',(-8.35826877743383,2.60901472383387,14.525494303512));
#67196=CARTESIAN_POINT('Ctrl Pts',(-7.75808397367562,-2.81049592880473,
14.7373630631171));
#67197=CARTESIAN_POINT('Ctrl Pts',(-4.74792936837933,-7.35695463475806,
14.9492318227222));
#67198=CARTESIAN_POINT('Ctrl Pts',(2.53677627359465,-9.03912851263144,15.2140677722286));
#67199=CARTESIAN_POINT('Ctrl Pts',(8.97503017698373,-2.75241624079192,15.5318709116363));
#67200=CARTESIAN_POINT('Ctrl Pts',(7.17251833904147,6.0461882439137,15.8496740510439));
#67201=CARTESIAN_POINT('Ctrl Pts',(-1.19428616794719,9.31131797273588,16.1674771904516));
#67202=CARTESIAN_POINT('Ctrl Pts',(-8.4796337332461,4.02950243580197,16.4852803298593));
#67203=CARTESIAN_POINT('Ctrl Pts',(-8.05418178699415,-3.434788279801,16.7501162793657));
#67204=CARTESIAN_POINT('Ctrl Pts',(-4.08254108033916,-7.17074700681693,
16.9619850389708));
#67205=CARTESIAN_POINT('Ctrl Pts',(1.15729944866126,-8.67918618138446,17.1738537985759));
#67206=CARTESIAN_POINT('Ctrl Pts',(7.79321241317349,-5.23516173707155,17.4386897480823));
#67207=CARTESIAN_POINT('Ctrl Pts',(8.61664847138021,3.72563161906873,17.75649288749));
#67208=CARTESIAN_POINT('Ctrl Pts',(1.53833159092038,9.25391525361577,18.0742960268977));
#67209=CARTESIAN_POINT('Ctrl Pts',(-6.9478671948217,6.31301063546267,18.3920991663053));
#67210=CARTESIAN_POINT('Ctrl Pts',(-9.06781150631994,-2.43225669204367,
18.709902305713));
#67211=CARTESIAN_POINT('Ctrl Pts',(-3.90304244852039,-7.83797642443857,
18.9747382552194));
#67212=CARTESIAN_POINT('Ctrl Pts',(1.54301357886363,-8.105915334117,19.1866070148245));
#67213=CARTESIAN_POINT('Ctrl Pts',(6.50974814736132,-5.85583417139971,19.3984757744296));
#67214=CARTESIAN_POINT('Ctrl Pts',(9.32724733240242,1.06936211375347,19.663311723936));
#67215=CARTESIAN_POINT('Ctrl Pts',(4.14255413218105,8.42414429495918,19.9811148633437));
#67216=CARTESIAN_POINT('Ctrl Pts',(-4.83063397340052,8.04154133358492,20.2989180027513));
#67217=CARTESIAN_POINT('Ctrl Pts',(-9.38282324990462,0.299315387832322,
20.6167211421591));
#67218=CARTESIAN_POINT('Ctrl Pts',(-5.32478016722184,-7.73225674049304,
20.9345242815667));
#67219=CARTESIAN_POINT('Ctrl Pts',(2.11237174904617,-8.49738197204518,21.1993602310731));
#67220=CARTESIAN_POINT('Ctrl Pts',(6.4315530863595,-5.16932096176763,21.4112289906782));
#67221=CARTESIAN_POINT('Ctrl Pts',(8.75283793689736,-0.235463023461224,
21.6230977502834));
#67222=CARTESIAN_POINT('Ctrl Pts',(6.40615450560057,6.86310881310455,21.8879336997897));
#67223=CARTESIAN_POINT('Ctrl Pts',(-2.31021700157468,9.09889329786755,22.2057368391974));
#67224=CARTESIAN_POINT('Ctrl Pts',(-8.89226376341935,2.98815273480211,22.5235399786051));
#67225=CARTESIAN_POINT('Ctrl Pts',(-7.33610591228832,-5.85734682975425,
22.8413431180127));
#67226=CARTESIAN_POINT('Ctrl Pts',(0.961614183393465,-9.33897083689823,
23.1591462574204));
#67227=CARTESIAN_POINT('Ctrl Pts',(7.11881881475451,-5.09804212102095,23.4239822069268));
#67228=CARTESIAN_POINT('Ctrl Pts',(8.24808328779048,0.236381865002667,23.6358509665319));
#67229=CARTESIAN_POINT('Ctrl Pts',(6.81516466103088,5.49737623126183,23.8477197261371));
#67230=CARTESIAN_POINT('Ctrl Pts',(0.425183917852744,9.37871509142584,24.1125556756434));
#67231=CARTESIAN_POINT('Ctrl Pts',(-7.65952089614688,5.42758707731466,24.4303588150511));
#67232=CARTESIAN_POINT('Ctrl Pts',(-8.70653421947809,-3.49251678446689,
24.7481619544587));
#67233=CARTESIAN_POINT('Ctrl Pts',(-1.78532270905324,-9.21626739330421,
25.0659650938665));
#67234=CARTESIAN_POINT('Ctrl Pts',(6.78869681247535,-6.48495749549885,25.3837682332741));
#67235=CARTESIAN_POINT('Ctrl Pts',(8.72498645285493,0.736360090244496,25.6486041827805));
#67236=CARTESIAN_POINT('Ctrl Pts',(6.12494475337123,5.52917770347282,25.8604729423856));
#67237=CARTESIAN_POINT('Ctrl Pts',(1.62225132418204,8.60441255555522,26.0723417019908));
#67238=CARTESIAN_POINT('Ctrl Pts',(-5.75887431216354,7.41461022487644,26.3371776514971));
#67239=CARTESIAN_POINT('Ctrl Pts',(-9.35028086563414,-0.836187523286537,
26.6549807909049));
#67240=CARTESIAN_POINT('Ctrl Pts',(-4.36215842218694,-8.30499762218326,
26.9727839303124));
#67241=CARTESIAN_POINT('Ctrl Pts',(4.61821377210678,-8.17306939866945,27.2905870697202));
#67242=CARTESIAN_POINT('Ctrl Pts',(9.37318165779515,-0.533426414898873,
27.6083902091278));
#67243=CARTESIAN_POINT('Ctrl Pts',(6.16369419152492,6.21904242615925,27.8732261586342));
#67244=CARTESIAN_POINT('Ctrl Pts',(1.0762473331214,8.18098074721972,28.0850949182393));
#67245=CARTESIAN_POINT('Ctrl Pts',(-4.34552480206557,7.60158068954343,28.2969636778444));
#67246=CARTESIAN_POINT('Ctrl Pts',(-9.19222594893933,1.90894217664809,28.5617996273508));
#67247=CARTESIAN_POINT('Ctrl Pts',(-6.57491120082365,-6.70056001701554,
28.8796027667585));
#67248=CARTESIAN_POINT('Ctrl Pts',(2.06578740672041,-9.15062478713675,29.1974059061662));
#67249=CARTESIAN_POINT('Ctrl Pts',(8.81587626065388,-3.22603279542901,29.5152090455739));
#67250=CARTESIAN_POINT('Ctrl Pts',(7.48059838386803,5.67289396599397,29.8330121849815));
#67251=CARTESIAN_POINT('Ctrl Pts',(0.658334507932313,8.73122044508511,30.0978481344879));
#67252=CARTESIAN_POINT('Ctrl Pts',(-4.4865159400542,6.92516635381925,30.309716894093));
#67253=CARTESIAN_POINT('Ctrl Pts',(-8.2376758883841,2.96787983970747,30.5215856536982));
#67254=CARTESIAN_POINT('Ctrl Pts',(-8.23494234109841,-4.508525564852,30.7864216032046));
#67255=CARTESIAN_POINT('Ctrl Pts',(-0.659057717521624,-9.36443296549871,
31.1042247426122));
#67256=CARTESIAN_POINT('Ctrl Pts',(7.50701695534774,-5.62548735994027,31.4220278820199));
#67257=CARTESIAN_POINT('Ctrl Pts',(8.80266564433859,3.26190732460705,31.7398310214275));
#67258=CARTESIAN_POINT('Ctrl Pts',(2.01493291010401,9.1695759715441,32.0576341608353));
#67259=CARTESIAN_POINT('Ctrl Pts',(-5.16147639882758,7.07296091954089,32.3224701103416));
#67260=CARTESIAN_POINT('Ctrl Pts',(-7.90631023908158,2.3615699675903,32.5343388699467));
#67261=CARTESIAN_POINT('Ctrl Pts',(-8.19512929753748,-3.08341865169973,
32.7462076295519));
#67262=CARTESIAN_POINT('Ctrl Pts',(-3.34426672559207,-8.77251151029379,
33.0110435790582));
#67263=CARTESIAN_POINT('Ctrl Pts',(5.57159242753132,-7.55541657764941,33.3288467184659));
#67264=CARTESIAN_POINT('Ctrl Pts',(9.36254556394446,0.586644839566965,33.6466498578736));
#67265=CARTESIAN_POINT('Ctrl Pts',(4.58489192880254,8.19180858184234,33.9644529972813));
#67266=CARTESIAN_POINT('Ctrl Pts',(-4.41315836778878,8.28644141661275,34.2822561366889));
#67267=CARTESIAN_POINT('Ctrl Pts',(-8.51592577979034,2.03632583299158,34.5470920861953));
#67268=CARTESIAN_POINT('Ctrl Pts',(-7.54968252853129,-3.33002222617508,
34.7589608458004));
#67269=CARTESIAN_POINT('Ctrl Pts',(-4.2382072629376,-7.66193278366428,34.9708296054056));
#67270=CARTESIAN_POINT('Ctrl Pts',(3.14378643854585,-8.84633737537489,35.235665554912));
#67271=CARTESIAN_POINT('Ctrl Pts',(9.14099053016895,-2.13758133592746,35.5534686943197));
#67272=CARTESIAN_POINT('Ctrl Pts',(6.74608634709743,6.51856814049157,35.8712718337273));
#67273=CARTESIAN_POINT('Ctrl Pts',(-1.82283971500673,9.20892052380395,36.189074973135));
#67274=CARTESIAN_POINT('Ctrl Pts',(-8.73331966470392,3.44531649696147,36.5068781125426));
#67275=CARTESIAN_POINT('Ctrl Pts',(-7.80277237585837,-3.97295331404088,
36.7717140620491));
#67276=CARTESIAN_POINT('Ctrl Pts',(-3.58697481303287,-7.43104070767335,
36.9835828216541));
#67277=CARTESIAN_POINT('Ctrl Pts',(1.74307995654875,-8.58075096073092,37.1954515812593));
#67278=CARTESIAN_POINT('Ctrl Pts',(8.13022077659065,-4.69474048846503,37.4602875307657));
#67279=CARTESIAN_POINT('Ctrl Pts',(8.34422581050367,4.30126231049319,37.7780906701733));
#67280=CARTESIAN_POINT('Ctrl Pts',(0.90738208935135,9.33691969273868,38.0958938095811));
#67281=CARTESIAN_POINT('Ctrl Pts',(-7.35989821147914,5.82742311463735,38.4136969489886));
#67282=CARTESIAN_POINT('Ctrl Pts',(-8.88204073208721,-3.0414520485589,38.7315000883964));
#67283=CARTESIAN_POINT('Ctrl Pts',(-3.36265146813914,-8.08456491648306,
38.9963360379027));
#67284=CARTESIAN_POINT('Ctrl Pts',(2.08903913788005,-7.98264804365293,39.2082047975079));
#67285=CARTESIAN_POINT('Ctrl Pts',(6.89179100417881,-5.40100282722816,39.420073557113));
#67286=CARTESIAN_POINT('Ctrl Pts',(9.23328300362556,1.69928311505142,39.6849095066194));
#67287=CARTESIAN_POINT('Ctrl Pts',(3.56187020826584,8.68562274450209,40.002712646027));
#67288=CARTESIAN_POINT('Ctrl Pts',(-5.36473011593325,7.69552352916454,40.3205157854348));
#67289=CARTESIAN_POINT('Ctrl Pts',(-9.38152653210372,-0.337522988517498,
40.6383189248424));
#67290=CARTESIAN_POINT('Ctrl Pts',(-4.78828546141623,-8.07548143890686,
40.9561220642501));
#67291=CARTESIAN_POINT('Ctrl Pts',(2.68362839752818,-8.33461177314138,41.2209580137564));
#67292=CARTESIAN_POINT('Ctrl Pts',(6.76723069875256,-4.72137087912944,41.4328267733616));
#67293=CARTESIAN_POINT('Ctrl Pts',(8.74866168043804,0.358515810309832,41.6446955329666));
#67294=CARTESIAN_POINT('Ctrl Pts',(5.92609922447768,7.28164995806476,41.9095314824732));
#67295=CARTESIAN_POINT('Ctrl Pts',(-2.92180050089287,8.92132521956945,42.2273346218806));
#67296=CARTESIAN_POINT('Ctrl Pts',(-9.07439735351213,2.37838690614001,42.5451377612886));
#67297=CARTESIAN_POINT('Ctrl Pts',(-6.92210083284602,-6.34125239209545,
42.862940900696));
#67298=CARTESIAN_POINT('Ctrl Pts',(1.59257796183507,-9.25228477542799,43.1807440401039));
#67299=CARTESIAN_POINT('Ctrl Pts',(7.4480823495277,-4.60365985924904,43.4455799896102));
#67300=CARTESIAN_POINT('Ctrl Pts',(8.21307769156944,0.795052916902295,43.6574487492153));
#67301=CARTESIAN_POINT('Ctrl Pts',(6.42676406589048,5.94679059883447,43.8693175088204));
#67302=CARTESIAN_POINT('Ctrl Pts',(-0.211665554595585,9.38596163550319,
44.1341534583268));
#67303=CARTESIAN_POINT('Ctrl Pts',(-8.00988320686094,4.89578725567103,44.4519565977345));
#67304=CARTESIAN_POINT('Ctrl Pts',(-8.44970977156173,-4.07477807752771,
44.7697597371422));
#67305=CARTESIAN_POINT('Ctrl Pts',(-1.15635737635423,-9.31610430697805,
45.0875628765497));
#67306=CARTESIAN_POINT('Ctrl Pts',(7.21275197559268,-6.00976597453871,45.4053660159576));
#67307=CARTESIAN_POINT('Ctrl Pts',(8.65498527413781,1.3262144206215,45.6702019654639));
#67308=CARTESIAN_POINT('Ctrl Pts',(5.73597625169008,5.93172240993103,45.882070725069));
#67309=CARTESIAN_POINT('Ctrl Pts',(1.03514460450429,8.69460122333234,46.0939394846741));
#67310=CARTESIAN_POINT('Ctrl Pts',(-6.24832900639056,7.00710088110893,46.3587754341805));
#67311=CARTESIAN_POINT('Ctrl Pts',(-9.27207262988954,-1.46820672468048,
46.6765785735882));
#67312=CARTESIAN_POINT('Ctrl Pts',(-3.7890472542822,-8.5816392670365,46.9943817129958));
#67313=CARTESIAN_POINT('Ctrl Pts',(5.16171622086671,-7.84115090376312,47.3121848524036));
#67314=CARTESIAN_POINT('Ctrl Pts',(9.38777970915338,0.103296962915415,47.6299879918112));
#67315=CARTESIAN_POINT('Ctrl Pts',(5.72786412260422,6.62262692426425,47.8948239413177));
#67316=CARTESIAN_POINT('Ctrl Pts',(0.51910539873841,8.23512500775983,48.1066927009227));
#67317=CARTESIAN_POINT('Ctrl Pts',(-4.85090813224476,7.28946534922341,48.3185614605278));
#67318=CARTESIAN_POINT('Ctrl Pts',(-9.30049950644462,1.28132238752107,48.5833974100343));
#67319=CARTESIAN_POINT('Ctrl Pts',(-6.10548831459029,-7.13091679104062,
48.9012005494418));
#67320=CARTESIAN_POINT('Ctrl Pts',(2.68144070795267,-8.98950984951128,49.2190036888497));
#67321=CARTESIAN_POINT('Ctrl Pts',(9.0143137421148,-2.62089862433939,49.5368068282571));
#67322=CARTESIAN_POINT('Ctrl Pts',(7.0787666142288,6.167020459786,49.8546099676651));
#67323=CARTESIAN_POINT('Ctrl Pts',(0.0648482886750494,8.75576435752259,
50.1194459171712));
#67324=CARTESIAN_POINT('Ctrl Pts',(-4.9457143701813,6.60504834781795,50.3313146767765));
#67325=CARTESIAN_POINT('Ctrl Pts',(-8.41994121215125,2.40254131471727,50.5431834363815));
#67326=CARTESIAN_POINT('Ctrl Pts',(-7.91031826793559,-5.0564753564221,50.808019385888));
#67327=CARTESIAN_POINT('Ctrl Pts',(-0.022638414813296,-9.38756887285086,
51.1258225252955));
#67328=CARTESIAN_POINT('Ctrl Pts',(7.87114769895336,-5.10357183803536,51.4436256647034));
#67329=CARTESIAN_POINT('Ctrl Pts',(8.56125517505403,3.8512169074144,51.7614288041108));
#67330=CARTESIAN_POINT('Ctrl Pts',(1.38860488811382,9.28508775375044,52.0792319435187));
#67331=CARTESIAN_POINT('Ctrl Pts',(-5.62914210825904,6.70674093058861,52.344067893025));
#67332=CARTESIAN_POINT('Ctrl Pts',(-8.04823060738345,1.82009296433092,52.5559366526302));
#67333=CARTESIAN_POINT('Ctrl Pts',(-7.9672182071849,-3.63194835096917,52.7678054122352));
#67334=CARTESIAN_POINT('Ctrl Pts',(-2.74180059859255,-8.97906496288433,
53.0326413617416));
#67335=CARTESIAN_POINT('Ctrl Pts',(6.07102464627148,-7.16028083141352,53.3504445011493));
#67336=CARTESIAN_POINT('Ctrl Pts',(9.30122794725025,1.2200697840768,53.668247640557));
#67337=CARTESIAN_POINT('Ctrl Pts',(4.01894239268663,8.48381187230187,53.9860507799647));
#67338=CARTESIAN_POINT('Ctrl Pts',(-4.96481920736273,7.96816468004654,54.3038539193723));
#67339=CARTESIAN_POINT('Ctrl Pts',(-8.63439205486384,1.45426566620785,54.5686898688788));
#67340=CARTESIAN_POINT('Ctrl Pts',(-7.30653705711197,-3.83422359043915,
54.7805586284838));
#67341=CARTESIAN_POINT('Ctrl Pts',(-3.70898071026316,-7.93165032486322,
54.992427388089));
#67342=CARTESIAN_POINT('Ctrl Pts',(3.73632873703891,-8.61283493972319,55.2572633375954));
#67343=CARTESIAN_POINT('Ctrl Pts',(9.2648835760257,-1.5129091721029,55.575066477003));
#67344=CARTESIAN_POINT('Ctrl Pts',(6.28860851972772,6.96094925210161,55.8928696164107));
#67345=CARTESIAN_POINT('Ctrl Pts',(-2.44300446019104,9.0641431502283,56.2106727558183));
#67346=CARTESIAN_POINT('Ctrl Pts',(-8.9468144110687,2.84527503486617,56.5284758952261));
#67347=CARTESIAN_POINT('Ctrl Pts',(-7.51545420598724,-4.49283461332772,
56.7933118447323));
#67348=CARTESIAN_POINT('Ctrl Pts',(-3.07490110363451,-7.65713637800046,
57.0051806043376));
#67349=CARTESIAN_POINT('Ctrl Pts',(2.32083872106099,-8.44282668398626,57.2170493639426));
#67350=CARTESIAN_POINT('Ctrl Pts',(8.42981344693531,-4.13271380330264,57.4818853134491));
#67351=CARTESIAN_POINT('Ctrl Pts',(8.03340259441033,4.85709837212146,57.7996884528567));
#67352=CARTESIAN_POINT('Ctrl Pts',(0.272256768860956,9.37695514847626,58.1174915922644));
#67353=CARTESIAN_POINT('Ctrl Pts',(-7.73805859902398,5.31501749370731,58.435294731672));
#67354=CARTESIAN_POINT('Ctrl Pts',(-8.65539435078031,-3.63665048672807,
58.7530978710798));
#67355=CARTESIAN_POINT('Ctrl Pts',(-2.80678539320662,-8.29394782606501,
59.0179338205861));
#67356=CARTESIAN_POINT('Ctrl Pts',(2.62545083162156,-7.82264419740334,59.2298025801913));
#67357=CARTESIAN_POINT('Ctrl Pts',(7.24211748526434,-4.92131579098878,59.4416713397963));
#67358=CARTESIAN_POINT('Ctrl Pts',(9.09682663282309,2.32138392828507,59.7065072893028));
#67359=CARTESIAN_POINT('Ctrl Pts',(2.96479437493774,8.90712951262538,60.0243104287104));
#67360=CARTESIAN_POINT('Ctrl Pts',(-5.87413749527606,7.31409053070298,60.3421135681181));
#67361=CARTESIAN_POINT('Ctrl Pts',(-9.33705554795461,-0.97280806676027,
60.6599167075258));
#67362=CARTESIAN_POINT('Ctrl Pts',(-4.2297548202907,-8.38154235748808,60.9777198469334));
#67363=CARTESIAN_POINT('Ctrl Pts',(3.2425348504619,-8.13348526331403,61.2425557964399));
#67364=CARTESIAN_POINT('Ctrl Pts',(7.07176516832905,-4.25169280551155,61.4544245560449));
#67365=CARTESIAN_POINT('Ctrl Pts',(8.70422363414217,0.95084473593113,61.6662933156501));
#67366=CARTESIAN_POINT('Ctrl Pts',(5.41877173073039,7.66668057638876,61.9311292651565));
#67367=CARTESIAN_POINT('Ctrl Pts',(-3.5199377244256,8.70270074497046,62.2489324045641));
#67368=CARTESIAN_POINT('Ctrl Pts',(-9.21477010149155,1.75767561893064,62.5667355439718));
#67369=CARTESIAN_POINT('Ctrl Pts',(-6.47623989028538,-6.79597518563895,
62.8845386833795));
#67370=CARTESIAN_POINT('Ctrl Pts',(2.21621261480156,-9.12301922480348,63.2023418227871));
#67371=CARTESIAN_POINT('Ctrl Pts',(7.74306942726154,-4.08809131864914,63.4671777722936));
#67372=CARTESIAN_POINT('Ctrl Pts',(8.14027509050269,1.35006509449442,63.6790465318986));
#67373=CARTESIAN_POINT('Ctrl Pts',(6.00878717284279,6.36883753101665,63.8909152915039));
#67374=CARTESIAN_POINT('Ctrl Pts',(-0.847540931303655,9.35001350265893,
64.1557512410101));
#67375=CARTESIAN_POINT('Ctrl Pts',(-8.32338362417113,4.34145676993609,64.4735543804179));
#67376=CARTESIAN_POINT('Ctrl Pts',(-8.15399932582899,-4.63828703285015,
64.7913575198255));
#67377=CARTESIAN_POINT('Ctrl Pts',(-0.522070427691442,-9.37306803073971,
65.1091606592332));
#67378=CARTESIAN_POINT('Ctrl Pts',(7.60361368412317,-5.5069172022788,65.4269637986408));
#67379=CARTESIAN_POINT('Ctrl Pts',(8.54515340921122,1.90996544420299,65.6917997481474));
#67380=CARTESIAN_POINT('Ctrl Pts',(5.32061049305866,6.30696902557715,65.9036685077523));
#67381=CARTESIAN_POINT('Ctrl Pts',(0.443274096256249,8.74477689026912,66.1155372673576));
#67382=CARTESIAN_POINT('Ctrl Pts',(-6.70902857000643,6.56734449964217,66.3803732168638));
#67383=CARTESIAN_POINT('Ctrl Pts',(-9.15119384027104,-2.09346916341428,
66.6981763562716));
#67384=CARTESIAN_POINT('Ctrl Pts',(-3.19849869654243,-8.81878776776366,
67.0159794956792));
#67385=CARTESIAN_POINT('Ctrl Pts',(5.68146418679031,-7.47314703017458,67.333782635087));
#67386=CARTESIAN_POINT('Ctrl Pts',(9.35917471673265,0.739544962821455,67.6515857744945));
#67387=CARTESIAN_POINT('Ctrl Pts',(5.26567412914822,6.99573375351603,67.916421724001));
#67388=CARTESIAN_POINT('Ctrl Pts',(-0.0404254852931306,8.25137080060695,
68.1282904836061));
#67389=CARTESIAN_POINT('Ctrl Pts',(-5.33396733442199,6.94380351535604,68.3401592432112));
#67390=CARTESIAN_POINT('Ctrl Pts',(-9.36597168800007,0.647805887207846,
68.6049951927176));
#67391=CARTESIAN_POINT('Ctrl Pts',(-5.60796765815626,-7.52845672048098,
68.9227983321252));
#67392=CARTESIAN_POINT('Ctrl Pts',(3.28475388189587,-8.78702472589971,69.240601471533));
#67393=CARTESIAN_POINT('Ctrl Pts',(9.1712668885677,-2.00370294432065,69.5584046109406));
#67394=CARTESIAN_POINT('Ctrl Pts',(6.64435799900976,6.63276601102574,69.8762077503483));
#67395=CARTESIAN_POINT('Ctrl Pts',(-0.528936368355967,8.74001378982291,
70.1410436998546));
#67396=CARTESIAN_POINT('Ctrl Pts',(-5.38215236557387,6.25453357505922,70.3529124594599));
#67397=CARTESIAN_POINT('Ctrl Pts',(-8.56345754306331,1.82614616024865,70.5647812190648));
#67398=CARTESIAN_POINT('Ctrl Pts',(-7.54929048622397,-5.58115496543806,
70.8296171685713));
#67399=CARTESIAN_POINT('Ctrl Pts',(0.613885040667023,-9.36750274626135,
71.147420307979));
#67400=CARTESIAN_POINT('Ctrl Pts',(8.19905507261868,-4.55816934438155,71.4652234473866));
#67401=CARTESIAN_POINT('Ctrl Pts',(8.28044526515006,4.42280285549989,71.7830265867943));
#67402=CARTESIAN_POINT('Ctrl Pts',(0.755886643805071,9.35786935756555,72.100829726202));
#67403=CARTESIAN_POINT('Ctrl Pts',(-6.0709025814317,6.30965570102665,72.3656656757083));
#67404=CARTESIAN_POINT('Ctrl Pts',(-8.15311211898698,1.27024043376002,72.5775344353135));
#67405=CARTESIAN_POINT('Ctrl Pts',(-7.70264275461673,-4.16376518087617,
72.7894031949187));
#67406=CARTESIAN_POINT('Ctrl Pts',(-2.12671404881879,-9.14429302064248,
73.054239144425));
#67407=CARTESIAN_POINT('Ctrl Pts',(6.54251347660453,-6.73219860486695,73.3720422838326));
#67408=CARTESIAN_POINT('Ctrl Pts',(9.19711332143845,1.84788996034588,73.6898454232404));
#67409=CARTESIAN_POINT('Ctrl Pts',(3.43448286563956,8.73675319058521,74.007648562648));
#67410=CARTESIAN_POINT('Ctrl Pts',(-5.49360270115903,7.61325580989032,74.3254517020558));
#67411=CARTESIAN_POINT('Ctrl Pts',(-8.71317307193497,0.865446903682397,
74.590287651562));
#67412=CARTESIAN_POINT('Ctrl Pts',(-7.02969889960619,-4.32069156311902,
74.8021564111673));
#67413=CARTESIAN_POINT('Ctrl Pts',(-3.16284988407271,-8.16508048661717,
75.0140251707722));
#67414=CARTESIAN_POINT('Ctrl Pts',(4.31202586543046,-8.33924037179835,75.2788611202788));
#67415=CARTESIAN_POINT('Ctrl Pts',(9.34555270036502,-0.882038459310571,
75.5966642596863));
#67416=CARTESIAN_POINT('Ctrl Pts',(5.80326091633985,7.37269032199734,75.9144673990941));
#67417=CARTESIAN_POINT('Ctrl Pts',(-3.05394033905752,8.87503027579986,76.2322705385017));
#67418=CARTESIAN_POINT('Ctrl Pts',(-9.1152435335431,2.23719675377212,76.5500736779094));
#67419=CARTESIAN_POINT('Ctrl Pts',(-6.81651864177013,-6.44743929429287,
76.8678768173171));
#67420=CARTESIAN_POINT('Ctrl Pts',(1.72522542783871,-9.22718507141483,77.1856799567247));
#67421=CARTESIAN_POINT('Ctrl Pts',(8.69565483555478,-3.53865568029239,77.5034830961325));
#67422=CARTESIAN_POINT('Ctrl Pts',(7.8449010032873,3.88968983220228,77.7683190456387));
#67423=CARTESIAN_POINT('Ctrl Pts',(3.66594536676364,7.39228562561244,77.9801878052441));
#67424=CARTESIAN_POINT('Ctrl Pts',(-1.65140120025543,8.59891024493111,78.1920565648489));
#67425=CARTESIAN_POINT('Ctrl Pts',(-8.07972130758836,4.78115448994417,78.4568925143554));
#67426=CARTESIAN_POINT('Ctrl Pts',(-8.3896089253915,-4.21200557295021,78.7746956537631));
#67427=CARTESIAN_POINT('Ctrl Pts',(-1.00692323689734,-9.32671948478797,
79.0924987931708));
#67428=CARTESIAN_POINT('Ctrl Pts',(7.29733197467081,-5.90558436552824,79.4103019325784));
#67429=CARTESIAN_POINT('Ctrl Pts',(8.91397127598894,2.94654434612107,79.7281050719862));
#67430=CARTESIAN_POINT('Ctrl Pts',(3.44868801762181,8.04824184799615,79.9929410214924));
#67431=CARTESIAN_POINT('Ctrl Pts',(-2.0037815204154,8.00447422400582,80.2048097810977));
#67432=CARTESIAN_POINT('Ctrl Pts',(-6.83379386824274,5.47420081702346,80.4166785407027));
#67433=CARTESIAN_POINT('Ctrl Pts',(-9.25088187844766,-1.6007085938909,80.6815144902092));
#67434=CARTESIAN_POINT('Ctrl Pts',(-3.65430448618155,-8.64713927319536,
80.9993176296168));
#67435=CARTESIAN_POINT('Ctrl Pts',(5.28234787004528,-7.75230371152486,81.3171207690245));
#67436=CARTESIAN_POINT('Ctrl Pts',(9.38459283052847,0.237444624201594,81.6349239084322));
#67437=CARTESIAN_POINT('Ctrl Pts',(4.87414259099121,8.02395236752506,81.9527270478397));
#67438=CARTESIAN_POINT('Ctrl Pts',(-2.59458247415171,8.36276011106766,82.2175629973463));
#67439=CARTESIAN_POINT('Ctrl Pts',(-6.71648974456451,4.79327861061246,82.4294317569514));
#67440=CARTESIAN_POINT('Ctrl Pts',(-8.75198783567674,-0.265186070959599,
82.6413005165564));
#67441=CARTESIAN_POINT('Ctrl Pts',(-6.00342500595349,-7.21803064373623,
82.9061364660629));
#67442=CARTESIAN_POINT('Ctrl Pts',(2.82648341645369,-8.95198041368108,83.2239396054705));
#67443=CARTESIAN_POINT('Ctrl Pts',(9.04851439375484,-2.47503512383449,83.5417427448782));
#67444=CARTESIAN_POINT('Ctrl Pts',(6.98934009826024,6.2670636535728,83.8595458842859));
#67445=CARTESIAN_POINT('Ctrl Pts',(-1.49380661323534,9.26874424774865,84.1773490236935));
#67446=CARTESIAN_POINT('Ctrl Pts',(-7.39855811862921,4.68283595162349,84.4421849732));
#67447=CARTESIAN_POINT('Ctrl Pts',(-8.22109022443365,-0.707410652091151,
84.654053732805));
#67448=CARTESIAN_POINT('Ctrl Pts',(-6.48982435061033,-5.87790733872935,
84.8659224924102));
#67449=CARTESIAN_POINT('Ctrl Pts',(0.111547012188838,-9.38768530546449,
85.1307584419166));
#67450=CARTESIAN_POINT('Ctrl Pts',(7.95721132033966,-4.98093865088163,85.4485615813242));
#67451=CARTESIAN_POINT('Ctrl Pts',(8.49268893873445,3.98442545350508,85.7663647207319));
#67452=CARTESIAN_POINT('Ctrl Pts',(1.2556530401561,9.30324122460166,86.0841678601397));
#67453=CARTESIAN_POINT('Ctrl Pts',(-7.14824422597728,6.08635216003193,86.4019709995472));
#67454=CARTESIAN_POINT('Ctrl Pts',(-8.6686378048306,-1.23382875378166,86.6668069490537));
#67455=CARTESIAN_POINT('Ctrl Pts',(-5.79891511690275,-5.8702076432944,86.8786757086588));
#67456=CARTESIAN_POINT('Ctrl Pts',(-1.12781848653672,-8.68306629287317,
87.0905444682638));
#67457=CARTESIAN_POINT('Ctrl Pts',(6.17323898017392,-7.07334423195992,87.3553804177703));
#67458=CARTESIAN_POINT('Ctrl Pts',(9.28720448840491,1.36923140151558,87.6731835571779));
#67459=CARTESIAN_POINT('Ctrl Pts',(3.88035969589542,8.54073885768649,87.9909866965857));
#67460=CARTESIAN_POINT('Ctrl Pts',(-5.0777923921815,7.8957574850199,88.3087898359931));
#67461=CARTESIAN_POINT('Ctrl Pts',(-9.38834746436722,-0.00316519361544216,
88.6265929754011));
#67462=CARTESIAN_POINT('Ctrl Pts',(-5.79817233028434,-6.56115938027206,
88.8914289249072));
#67463=CARTESIAN_POINT('Ctrl Pts',(-0.606908062902263,-8.229120056945,89.1032976845126));
#67464=CARTESIAN_POINT('Ctrl Pts',(4.77288601530261,-7.34078836842037,89.3151664441175));
#67465=CARTESIAN_POINT('Ctrl Pts',(9.28630449027279,-1.38044450959777,89.580002393624));
#67466=CARTESIAN_POINT('Ctrl Pts',(6.18119623774963,7.06539276408422,89.8978055330316));
#67467=CARTESIAN_POINT('Ctrl Pts',(-2.58541006692869,9.01759759528832,90.2156086724394));
#67468=CARTESIAN_POINT('Ctrl Pts',(-8.98584767790854,2.71689222270035,90.5334118118469));
#67469=CARTESIAN_POINT('Ctrl Pts',(-7.14413868793919,-6.09117070337302,
90.8512149512548));
#67470=CARTESIAN_POINT('Ctrl Pts',(-0.158229698722761,-8.75457469826193,
91.1160509007609));
#67471=CARTESIAN_POINT('Ctrl Pts',(4.87498654891268,-6.65742145701708,91.3279196603662));
#67472=CARTESIAN_POINT('Ctrl Pts',(8.39383785726041,-2.49220801921283,91.5397884199713));
#67473=CARTESIAN_POINT('Ctrl Pts',(7.96379846267019,4.97181980527365,91.8046243694778));
#67474=CARTESIAN_POINT('Ctrl Pts',(0.12276077239064,9.3867934691835,92.1224275088853));
#67475=CARTESIAN_POINT('Ctrl Pts',(-7.81626756533493,5.18723172335875,92.4402306482931));
#67476=CARTESIAN_POINT('Ctrl Pts',(-8.60184359340913,-3.7596873054644,92.7580337877005));
#67477=CARTESIAN_POINT('Ctrl Pts',(-1.48755653318772,-9.26974938661827,
93.0758369271086));
#67478=CARTESIAN_POINT('Ctrl Pts',(5.55729080655709,-6.76639739273147,93.3406728766146));
#67479=CARTESIAN_POINT('Ctrl Pts',(8.02836053062309,-1.9058282972932,93.55254163622));
#67480=CARTESIAN_POINT('Ctrl Pts',(8.00550179241508,3.54676695550274,93.7644103958249));
#67481=CARTESIAN_POINT('Ctrl Pts',(2.83741137236831,8.94931141675683,94.0292463453314));
#67482=CARTESIAN_POINT('Ctrl Pts',(-5.99431095549163,7.22462441994161,94.347049484739));
#67483=CARTESIAN_POINT('Ctrl Pts',(-9.31371162891651,-1.120797616928,94.6648526241468));
#67484=CARTESIAN_POINT('Ctrl Pts',(-4.10919837457598,-8.44046506767997,
94.9826557635543));
#67485=CARTESIAN_POINT('Ctrl Pts',(4.87955190532278,-8.02066402072798,95.3004589029622));
#67486=CARTESIAN_POINT('Ctrl Pts',(8.61839038970218,-1.5462735449124,95.5652948524683));
#67487=CARTESIAN_POINT('Ctrl Pts',(7.3470155989771,3.7560772218923,95.7771636120737));
#67488=CARTESIAN_POINT('Ctrl Pts',(3.79336521223575,7.89164084025658,95.9890323716785));
#67489=CARTESIAN_POINT('Ctrl Pts',(-3.64425554288549,8.65219507803006,96.2538683211854));
#67490=CARTESIAN_POINT('Ctrl Pts',(-9.2482205837292,1.6116382581185,96.5716714605926));
#67491=CARTESIAN_POINT('Ctrl Pts',(-6.36249322888283,-6.89348181379674,
96.8894746000007));
#67492=CARTESIAN_POINT('Ctrl Pts',(2.34619137542456,-9.08968359571602,97.2072777394079));
#67493=CARTESIAN_POINT('Ctrl Pts',(8.91595908687415,-2.94053595307482,97.525080878816));
#67494=CARTESIAN_POINT('Ctrl Pts',(7.56294531793053,4.41242256623269,97.789916828322));
#67495=CARTESIAN_POINT('Ctrl Pts',(3.15639382722669,7.62390531918362,98.0017855879274));
#67496=CARTESIAN_POINT('Ctrl Pts',(-2.23065927072821,8.4670995035443,98.2136543475322));
#67497=CARTESIAN_POINT('Ctrl Pts',(-8.38525627827585,4.22238739077491,98.4784902970391));
#67498=CARTESIAN_POINT('Ctrl Pts',(-8.08474932180308,-4.77114139844422,
98.7962934364465));
#67499=CARTESIAN_POINT('Ctrl Pts',(-0.37225172720383,-9.37351802987116,
99.1140965758541));
#67500=CARTESIAN_POINT('Ctrl Pts',(7.68093084977082,-5.39724588298354,99.4318997152619));
#67501=CARTESIAN_POINT('Ctrl Pts',(8.69368894436464,3.54412904234188,99.7497028546694));
#67502=CARTESIAN_POINT('Ctrl Pts',(2.89508531527422,8.26354014949349,100.014538804176));
#67503=CARTESIAN_POINT('Ctrl Pts',(-2.54186864664432,7.8502011497564,100.226407563781));
#67504=CARTESIAN_POINT('Ctrl Pts',(-7.18921699219222,4.99827708557477,100.438276323386));
#67505=CARTESIAN_POINT('Ctrl Pts',(-9.12106806867608,-2.22422917360528,
100.703112272893));
#67506=CARTESIAN_POINT('Ctrl Pts',(-3.05962523352364,-8.87500170539302,
101.0209154123));
#67507=CARTESIAN_POINT('Ctrl Pts',(5.79579453715258,-7.37632545972848,101.338718551708));
#67508=CARTESIAN_POINT('Ctrl Pts',(9.34690000800457,0.873167842231912,101.656521691115));
#67509=CARTESIAN_POINT('Ctrl Pts',(4.31890805017312,8.3359529379843,101.974324830524));
#67510=CARTESIAN_POINT('Ctrl Pts',(-3.15560227365146,8.16760607984566,102.23916078003));
#67511=CARTESIAN_POINT('Ctrl Pts',(-7.02601626638363,4.32687528511553,102.451029539635));
#67512=CARTESIAN_POINT('Ctrl Pts',(-8.71386983768246,-0.857955265112621,
102.66289829924));
#67513=CARTESIAN_POINT('Ctrl Pts',(-5.50023293227864,-7.60845029035593,
102.927734248746));
#67514=CARTESIAN_POINT('Ctrl Pts',(3.42691836949006,-8.7397478412821,103.245537388154));
#67515=CARTESIAN_POINT('Ctrl Pts',(9.19549938924046,-1.85585629486889,103.563340527562));
#67516=CARTESIAN_POINT('Ctrl Pts',(6.54835438700928,6.72651593787452,103.881143666969));
#67517=CARTESIAN_POINT('Ctrl Pts',(-2.11878448355848,9.14613746028187,104.198946806377));
#67518=CARTESIAN_POINT('Ctrl Pts',(-7.69902724331096,4.17044293711862,104.463782755883));
#67519=CARTESIAN_POINT('Ctrl Pts',(-8.15421127793089,-1.26316774155096,
104.675651515489));
#67520=CARTESIAN_POINT('Ctrl Pts',(-6.07637259690935,-6.3043882215911,104.887520275093));
#67521=CARTESIAN_POINT('Ctrl Pts',(0.7477696280061,-9.35852118198021,105.1523562246));
#67522=CARTESIAN_POINT('Ctrl Pts',(8.27660614921521,-4.4299833511106,105.470159364008));
#67523=CARTESIAN_POINT('Ctrl Pts',(8.20300544916199,4.55105627362975,105.787962503416));
#67524=CARTESIAN_POINT('Ctrl Pts',(0.622009718693708,9.36696673156227,106.105765642823));
#67525=CARTESIAN_POINT('Ctrl Pts',(-7.5444468647533,5.58770074673416,106.423568782231));
#67526=CARTESIAN_POINT('Ctrl Pts',(-8.56503821645671,-1.81871799233499,
106.688404731737));
#67527=CARTESIAN_POINT('Ctrl Pts',(-5.3875751976612,-6.24986302233706,106.900273491342));
#67528=CARTESIAN_POINT('Ctrl Pts',(-0.53651679449818,-8.73955173416969,
107.112142250947));
#67529=CARTESIAN_POINT('Ctrl Pts',(6.6386025863016,-6.63852648042387,107.376978200454));
#67530=CARTESIAN_POINT('Ctrl Pts',(9.17300134601047,1.99574751570282,107.694781339861));
#67531=CARTESIAN_POINT('Ctrl Pts',(3.2923740484798,8.78417239867384,108.012584479269));
#67532=CARTESIAN_POINT('Ctrl Pts',(-5.60143576160796,7.53331794423434,108.330387618677));
#67533=CARTESIAN_POINT('Ctrl Pts',(-9.36653003787306,-0.639682092731105,
108.648190758084));
#67534=CARTESIAN_POINT('Ctrl Pts',(-5.33998801752543,-6.93917450117029,
108.913026707591));
#67535=CARTESIAN_POINT('Ctrl Pts',(-0.0475822746342192,-8.25133263391868,
109.124895467196));
#67536=CARTESIAN_POINT('Ctrl Pts',(5.25960441743795,-7.00029829057828,109.336764226801));
#67537=CARTESIAN_POINT('Ctrl Pts',(9.35852975395092,-0.747662339933337,
109.601600176307));
#67538=CARTESIAN_POINT('Ctrl Pts',(5.6879438639411,7.46821641632047,109.919403315715));
#67539=CARTESIAN_POINT('Ctrl Pts',(-3.19084854132404,8.82155865995665,110.237206455123));
#67540=CARTESIAN_POINT('Ctrl Pts',(-9.14937463317463,2.10140563960524,110.55500959453));
#67541=CARTESIAN_POINT('Ctrl Pts',(-6.71472221522252,-6.56152297127247,
110.872812733938));
#67542=CARTESIAN_POINT('Ctrl Pts',(0.435689170539254,-8.74515807356746,
111.137648683444));
#67543=CARTESIAN_POINT('Ctrl Pts',(5.31513815892038,-6.31158147059979,111.34951744305));
#67544=CARTESIAN_POINT('Ctrl Pts',(8.54349359153895,-1.91737634186406,111.561386202655));
#67545=CARTESIAN_POINT('Ctrl Pts',(7.60838723404739,5.50032015676579,111.826222152161));
#67546=CARTESIAN_POINT('Ctrl Pts',(-0.513940525685185,9.37351732149688,
112.144025291569));
#67547=CARTESIAN_POINT('Ctrl Pts',(-8.14997325281275,4.64535763781033,112.461828430977));
#67548=CARTESIAN_POINT('Ctrl Pts',(-8.32714604435014,-4.33423587226256,
112.779631570384));
#67549=CARTESIAN_POINT('Ctrl Pts',(-0.855650321852643,-9.34927487331794,
113.097434709792));
#67550=CARTESIAN_POINT('Ctrl Pts',(6.00326091836658,-6.37404684098099,113.362270659298));
#67551=CARTESIAN_POINT('Ctrl Pts',(8.13910105320298,-1.35712503262605,113.574139418903));
#67552=CARTESIAN_POINT('Ctrl Pts',(7.74661230987278,4.08137385025368,113.786008178509));
#67553=CARTESIAN_POINT('Ctrl Pts',(2.22412460764706,9.12109356710027,114.050844128015));
#67554=CARTESIAN_POINT('Ctrl Pts',(-6.47034298326984,6.80158977880867,114.368647267423));
#67555=CARTESIAN_POINT('Ctrl Pts',(-9.21629115066875,-1.74968255144495,
114.68645040683));
#67556=CARTESIAN_POINT('Ctrl Pts',(-3.52748466476459,-8.69964446286136,
115.004253546238));
#67557=CARTESIAN_POINT('Ctrl Pts',(5.41212001747173,-7.67137764985019,115.322056685646));
#67558=CARTESIAN_POINT('Ctrl Pts',(8.70339564743194,-0.958393963497642,
115.586892635152));
#67559=CARTESIAN_POINT('Ctrl Pts',(7.0754502027632,4.2455575295418,115.798761394757));
#67560=CARTESIAN_POINT('Ctrl Pts',(3.24958818761061,8.13066979995796,116.010630154362));
#67561=CARTESIAN_POINT('Ctrl Pts',(-4.22248352081092,8.38520787140186,116.275466103869));
#67562=CARTESIAN_POINT('Ctrl Pts',(-9.33620827337083,0.980906171142857,
116.593269243276));
#67563=CARTESIAN_POINT('Ctrl Pts',(-5.88047914271609,-7.30899286200274,
116.911072382684));
#67564=CARTESIAN_POINT('Ctrl Pts',(2.9570676846459,-8.90969766876333,117.228875522091));
#67565=CARTESIAN_POINT('Ctrl Pts',(9.09480976491298,-2.32927316349603,117.546678661499));
#67566=CARTESIAN_POINT('Ctrl Pts',(7.24638325133705,4.91503250851395,117.811514611005));
#67567=CARTESIAN_POINT('Ctrl Pts',(2.63223479371206,7.82036407715153,118.023383370611));
#67568=CARTESIAN_POINT('Ctrl Pts',(-2.79959060385439,8.29637916417864,118.235252130216));
#67569=CARTESIAN_POINT('Ctrl Pts',(-8.65223685596117,3.64415635209118,118.500088079723));
#67570=CARTESIAN_POINT('Ctrl Pts',(-7.74266565467541,-5.30830390993709,
118.81789121913));
#67571=CARTESIAN_POINT('Ctrl Pts',(0.264123589339781,-9.37718776255869,
119.135694358538));
#67572=CARTESIAN_POINT('Ctrl Pts',(8.02918678132282,-4.86406429552229,119.453497497945));
#67573=CARTESIAN_POINT('Ctrl Pts',(8.43339477442419,4.12540067252307,119.771300637353));
#67574=CARTESIAN_POINT('Ctrl Pts',(2.32816071136047,8.44081053495957,120.036136586859));
#67575=CARTESIAN_POINT('Ctrl Pts',(-3.06825855014793,7.6598005050964,120.248005346464));
#67576=CARTESIAN_POINT('Ctrl Pts',(-7.51155453092633,4.49935143258734,120.45987410607));
#67577=CARTESIAN_POINT('Ctrl Pts',(-8.94927888749763,-2.83751396893987,
120.724710055576));
#67578=CARTESIAN_POINT('Ctrl Pts',(-2.45086530172317,-9.06202080736714,
121.042513194984));
#67579=CARTESIAN_POINT('Ctrl Pts',(6.28256859347107,-6.96640104164675,121.360316334391));
#67580=CARTESIAN_POINT('Ctrl Pts',(9.26619230882614,1.50487273089625,121.678119473799));
#67581=CARTESIAN_POINT('Ctrl Pts',(3.7437976511162,8.60959100524735,121.995922613207));
#67582=CARTESIAN_POINT('Ctrl Pts',(-3.70209981932849,7.93486431596248,122.260758562713));
#67583=CARTESIAN_POINT('Ctrl Pts',(-7.30320870515385,3.8405594536989,122.472627322318));
#67584=CARTESIAN_POINT('Ctrl Pts',(-8.63565016053205,-1.44677610220397,
122.684496081923));
#67585=CARTESIAN_POINT('Ctrl Pts',(-4.97172850631308,-7.96385546011813,
122.94933203143));
#67586=CARTESIAN_POINT('Ctrl Pts',(4.01158246931131,-8.4872945001489,123.267135170837));
#67587=CARTESIAN_POINT('Ctrl Pts',(9.30016622434986,-1.22813672047871,123.584938310245));
#67588=CARTESIAN_POINT('Ctrl Pts',(6.07723281321958,7.15501245102138,123.902741449653));
#67589=CARTESIAN_POINT('Ctrl Pts',(-2.73401159915763,8.9814396789051,124.22054458906));
#67590=CARTESIAN_POINT('Ctrl Pts',(-7.96406504960543,3.63885733035252,124.485380538567));
#67591=CARTESIAN_POINT('Ctrl Pts',(-8.04980623286806,-1.81311166829539,
124.697249298172));
#67592=CARTESIAN_POINT('Ctrl Pts',(-5.63495706479247,-6.70185598643782,
124.909118057777));
#67593=CARTESIAN_POINT('Ctrl Pts',(1.38055096962363,-9.28628866396099,125.173954007283));
#67594=CARTESIAN_POINT('Ctrl Pts',(8.55791161203055,-3.85864104070546,125.491757146691));
#67595=CARTESIAN_POINT('Ctrl Pts',(7.87557130771675,5.09674289932255,125.809560286099));
#67596=CARTESIAN_POINT('Ctrl Pts',(-0.0144961233994668,9.38758497712538,
126.127363425506));
#67597=CARTESIAN_POINT('Ctrl Pts',(-7.90592957204853,5.0633344479649,126.445166564914));
#67598=CARTESIAN_POINT('Ctrl Pts',(-8.42202188284641,-2.39523739739133,
126.71000251442));
#67599=CARTESIAN_POINT('Ctrl Pts',(-4.95144138099217,-6.60075621114956,
126.921871274026));
#67600=CARTESIAN_POINT('Ctrl Pts',(0.0572539753503746,-8.75581731006953,
127.13374003363));
#67601=CARTESIAN_POINT('Ctrl Pts',(7.07341500278416,-6.17315788948633,127.398575983137));
#67602=CARTESIAN_POINT('Ctrl Pts',(9.01658358087113,2.61307909744599,127.716379122545));
#67603=CARTESIAN_POINT('Ctrl Pts',(2.68923672680319,8.98718072767756,128.034182261952));
#67604=CARTESIAN_POINT('Ctrl Pts',(-6.09930103632042,7.1362096878304,128.35198540136));
#67605=CARTESIAN_POINT('Ctrl Pts',(-9.30160735966655,-1.273255142042,128.669788540768));
#67606=CARTESIAN_POINT('Ctrl Pts',(-4.85722880598274,-7.28525518505279,
128.934624490274));
#67607=CARTESIAN_POINT('Ctrl Pts',(0.51196248970237,-8.23557215483952,129.146493249879));
#67608=CARTESIAN_POINT('Ctrl Pts',(5.7221178502404,-6.62759248090642,129.358362009484));
#67609=CARTESIAN_POINT('Ctrl Pts',(9.38768658363369,-0.111439389827381,
129.623197958991));
#67610=CARTESIAN_POINT('Ctrl Pts',(5.168515280694,7.8366709535093,129.941001098399));
#67611=CARTESIAN_POINT('Ctrl Pts',(-3.78160256705032,8.58492245914921,130.258804237806));
#67612=CARTESIAN_POINT('Ctrl Pts',(-9.27079569704023,1.4762482799598,130.576607377214));
#67613=CARTESIAN_POINT('Ctrl Pts',(-6.25440424642379,-7.00167877386955,
130.894410516621));
#67614=CARTESIAN_POINT('Ctrl Pts',(1.02760297588888,-8.69549578281488,131.159246466128));
#67615=CARTESIAN_POINT('Ctrl Pts',(5.73082923046837,-5.93669526248734,131.371115225733));
#67616=CARTESIAN_POINT('Ctrl Pts',(8.65383173005065,-1.3337208002335,131.582983985338));
#67617=CARTESIAN_POINT('Ctrl Pts',(7.21796181708323,6.00350775274488,131.847819934845));
#67618=CARTESIAN_POINT('Ctrl Pts',(-1.14827664309823,9.31710376626014,132.165623074252));
#67619=CARTESIAN_POINT('Ctrl Pts',(-8.44617234530928,4.08210537811788,132.48342621366));
#67620=CARTESIAN_POINT('Ctrl Pts',(-8.01412654203442,-4.88883806324193,
132.801229353067));
#67621=CARTESIAN_POINT('Ctrl Pts',(-0.219806363843781,-9.38577451745743,
133.119032492475));
#67622=CARTESIAN_POINT('Ctrl Pts',(6.4216037154782,-5.95236259869669,133.383868441981));
#67623=CARTESIAN_POINT('Ctrl Pts',(8.21238501522175,-0.802176208942004,
133.595737201587));
#67624=CARTESIAN_POINT('Ctrl Pts',(7.45207252009975,4.59719805318194,133.807605961192));
#67625=CARTESIAN_POINT('Ctrl Pts',(1.60060230738995,9.25089997695995,134.072441910698));
#67626=CARTESIAN_POINT('Ctrl Pts',(-6.91659816072736,6.34725387261032,134.390245050106));
#67627=CARTESIAN_POINT('Ctrl Pts',(-9.07645682777433,-2.37051535710585,
134.708048189513));
#67628=CARTESIAN_POINT('Ctrl Pts',(-2.92953728957566,-8.91878764795583,
135.025851328922));
#67629=CARTESIAN_POINT('Ctrl Pts',(5.91978127567269,-7.28678720550658,135.343654468329));
#67630=CARTESIAN_POINT('Ctrl Pts',(8.7483474319312,-0.366103803899804,135.608490417835));
#67631=CARTESIAN_POINT('Ctrl Pts',(6.77132322176431,4.7154995636545,135.82035917744));
#67632=CARTESIAN_POINT('Ctrl Pts',(2.69085639145085,8.33228100015807,136.032227937046));
#67633=CARTESIAN_POINT('Ctrl Pts',(-4.78127941297109,8.07963150801064,136.297063886552));
#67634=CARTESIAN_POINT('Ctrl Pts',(-9.38123025361558,0.345659903649954,
136.61486702596));
#67635=CARTESIAN_POINT('Ctrl Pts',(-5.37140278988185,-7.69086755012565,
136.932670165367));
#67636=CARTESIAN_POINT('Ctrl Pts',(3.55433541669274,-8.68870885609521,137.250473304775));
#67637=CARTESIAN_POINT('Ctrl Pts',(9.23180566187414,-1.70729093933327,137.568276444182));
#67638=CARTESIAN_POINT('Ctrl Pts',(6.89647295730047,5.39502321906315,137.833112393689));
#67639=CARTESIAN_POINT('Ctrl Pts',(2.0959620806498,7.98083311847255,138.044981153294));
#67640=CARTESIAN_POINT('Ctrl Pts',(-3.35563807741036,8.08747846231697,138.256849912899));
#67641=CARTESIAN_POINT('Ctrl Pts',(-8.87939939579868,3.04915471893925,138.521685862406));
#67642=CARTESIAN_POINT('Ctrl Pts',(-7.36494984302657,-5.82103733453466,
138.839489001813));
#67643=CARTESIAN_POINT('Ctrl Pts',(0.89928339557674,-9.33770319613803,139.157292141221));
#67644=CARTESIAN_POINT('Ctrl Pts',(8.34049198343126,-4.30849803465926,139.475095280629));
#67645=CARTESIAN_POINT('Ctrl Pts',(8.13428968912092,4.68768699718746,139.792898420036));
#67646=CARTESIAN_POINT('Ctrl Pts',(1.75052179242454,8.57923587735251,140.057734369543));
#67647=CARTESIAN_POINT('Ctrl Pts',(-3.58052817041019,7.43414906558445,140.269603129148));
#67648=CARTESIAN_POINT('Ctrl Pts',(-7.79932351038639,3.97971953350241,140.481471888753));
#67649=CARTESIAN_POINT('Ctrl Pts',(-8.73630466580453,-3.43774037943266,
140.746307838259));
#67650=CARTESIAN_POINT('Ctrl Pts',(-1.83082636208119,-9.20733602472795,
141.064110977667));
#67651=CARTESIAN_POINT('Ctrl Pts',(6.74042994684304,-6.52441688861351,141.381914117074));
#67652=CARTESIAN_POINT('Ctrl Pts',(9.14284111731162,2.12965211805653,141.699717256482));
#67653=CARTESIAN_POINT('Ctrl Pts',(3.15145810322174,8.84360729305531,142.01752039589));
#67654=CARTESIAN_POINT('Ctrl Pts',(-4.23156011172795,7.66560589945927,142.282356345396));
#67655=CARTESIAN_POINT('Ctrl Pts',(-7.54679140282833,3.33656917066706,142.494225105002));
#67656=CARTESIAN_POINT('Ctrl Pts',(-8.51768877835491,-2.02893880145877,
142.706093864606));
#67657=CARTESIAN_POINT('Ctrl Pts',(-4.42034393072991,-8.28261055852364,
142.970929814113));
#67658=CARTESIAN_POINT('Ctrl Pts',(4.57778506083285,-8.19578219435772,143.288732953521));
#67659=CARTESIAN_POINT('Ctrl Pts',(9.3620332174066,-0.59476519788765,143.606536092929));
#67660=CARTESIAN_POINT('Ctrl Pts',(5.57814350230469,7.55058122980996,143.924339232336));
#67661=CARTESIAN_POINT('Ctrl Pts',(-3.33665665318324,8.77540885145237,144.242142371744));
#67662=CARTESIAN_POINT('Ctrl Pts',(-8.19245181991234,3.09052551540061,144.50697832125));
#67663=CARTESIAN_POINT('Ctrl Pts',(-7.90835556671305,-2.35471156201695,
144.718847080855));
#67664=CARTESIAN_POINT('Ctrl Pts',(-5.1676091709004,-7.06848146653319,144.93071584046));
#67665=CARTESIAN_POINT('Ctrl Pts',(2.00697894421316,-9.17132016854132,145.195551789967));
#67666=CARTESIAN_POINT('Ctrl Pts',(8.79983312769516,-3.2695410673115,145.513354929374));
#67667=CARTESIAN_POINT('Ctrl Pts',(7.51189338113173,5.61897405460601,145.831158068782));
#67668=CARTESIAN_POINT('Ctrl Pts',(-0.650935249830781,9.36500107153992,
146.14896120819));
#67669=CARTESIAN_POINT('Ctrl Pts',(-8.23102879335794,4.51566643132572,146.466764347598));
#67670=CARTESIAN_POINT('Ctrl Pts',(-8.24024695947341,-2.9607338092988,146.731600297104));
#67671=CARTESIAN_POINT('Ctrl Pts',(-4.49252079448732,-6.92127236495981,
146.943469056709));
#67672=CARTESIAN_POINT('Ctrl Pts',(0.650761301820232,-8.73178820528528,
147.155337816314));
#67673=CARTESIAN_POINT('Ctrl Pts',(7.4756751106369,-5.67938002490987,147.420173765821));
#67674=CARTESIAN_POINT('Ctrl Pts',(8.81867118648771,3.21838501357198,147.737976905228));
#67675=CARTESIAN_POINT('Ctrl Pts',(2.0737231238013,9.14882984880614,148.055780044636));
#67676=CARTESIAN_POINT('Ctrl Pts',(-6.56909649240655,6.70625973837498,148.373583184043));
#67677=CARTESIAN_POINT('Ctrl Pts',(-9.193879243756,-1.90096763361108,148.691386323451));
#67678=CARTESIAN_POINT('Ctrl Pts',(-4.35211456730083,-7.59781044961311,
148.956222272958));
#67679=CARTESIAN_POINT('Ctrl Pts',(1.06914875867794,-8.18190888238425,149.168091032563));
#67680=CARTESIAN_POINT('Ctrl Pts',(6.15830368944283,-6.22439167206857,149.379959792168));
#67681=CARTESIAN_POINT('Ctrl Pts',(9.3736282979707,0.525308135358659,149.644795741674));
#67682=CARTESIAN_POINT('Ctrl Pts',(4.62532190065374,8.1690410535072,149.962598881082));
#67683=CARTESIAN_POINT('Ctrl Pts',(-4.35499181730632,8.30881398094853,150.28040202049));
#67684=CARTESIAN_POINT('Ctrl Pts',(-9.34947948145903,0.844229048237673,
150.598205159897));
#67685=CARTESIAN_POINT('Ctrl Pts',(-5.76544724662711,-7.40947736302889,
150.916008299305));
#67686=CARTESIAN_POINT('Ctrl Pts',(1.61503940058015,-8.60605247318171,151.180844248811));
#67687=CARTESIAN_POINT('Ctrl Pts',(6.11981070531535,-5.53417288230174,151.392713008416));
#67688=CARTESIAN_POINT('Ctrl Pts',(8.72516264438353,-0.744694817129546,
151.604581768021));
#67689=CARTESIAN_POINT('Ctrl Pts',(6.79258094058841,6.48069683519393,151.869417717528));
#67690=CARTESIAN_POINT('Ctrl Pts',(-1.77440860364534,9.21507589793784,152.187220856935));
#67691=CARTESIAN_POINT('Ctrl Pts',(-8.70886625593951,3.50508210372682,152.505023996343));
#67692=CARTESIAN_POINT('Ctrl Pts',(-7.6538609868877,-5.43052651898935,152.822827135751));
#67693=CARTESIAN_POINT('Ctrl Pts',(-0.9466795259243,-8.7045547712713,153.087663085258));
#67694=CARTESIAN_POINT('Ctrl Pts',(4.27613052328954,-7.06725396548898,153.299535285551));
#67695=CARTESIAN_POINT('Ctrl Pts',(6.18792442894812,-5.14458818350946,153.405473106043));
#67696=CARTESIAN_POINT('Ctrl Pts',(6.85423122541137,-4.00395918922165,153.458443736632));
#67697=CARTESIAN_POINT('Ctrl Pts',(4.37750802528476,-6.14572094339974,-0.44955678837992));
#67698=CARTESIAN_POINT('Ctrl Pts',(5.40128695262251,-5.41652500898836,-0.396532856746831));
#67699=CARTESIAN_POINT('Ctrl Pts',(7.05805613175304,-3.44046858888462,-0.290541735212461));
#67700=CARTESIAN_POINT('Ctrl Pts',(8.15840353697748,1.64586779412391,-0.078616233875533));
#67701=CARTESIAN_POINT('Ctrl Pts',(4.48144417158412,7.71305662036539,0.186219715630859));
#67702=CARTESIAN_POINT('Ctrl Pts',(-4.06808443251202,7.94213116854575,0.504022855038533));
#67703=CARTESIAN_POINT('Ctrl Pts',(-8.87604082525919,0.88600865987949,0.821825994446204));
#67704=CARTESIAN_POINT('Ctrl Pts',(-5.54974215001441,-6.98819881157078,
1.13962913385388));
#67705=CARTESIAN_POINT('Ctrl Pts',(1.45643916438736,-8.1953082696198,1.40446508336027));
#67706=CARTESIAN_POINT('Ctrl Pts',(5.76587662434617,-5.31650462948363,1.61633384296539));
#67707=CARTESIAN_POINT('Ctrl Pts',(8.28579825562455,-0.787600779429617,
1.8282026025705));
#67708=CARTESIAN_POINT('Ctrl Pts',(6.51741451893584,6.09588472696246,2.0930385520769));
#67709=CARTESIAN_POINT('Ctrl Pts',(-1.60443270220511,8.77772874853394,2.41084169148457));
#67710=CARTESIAN_POINT('Ctrl Pts',(-8.24041566903942,3.40690648579429,2.72864483089224));
#67711=CARTESIAN_POINT('Ctrl Pts',(-7.33463407283986,-5.0820354846744,3.04644797029991));
#67712=CARTESIAN_POINT('Ctrl Pts',(0.310075852972152,-8.91854603754864,
3.36425110970758));
#67713=CARTESIAN_POINT('Ctrl Pts',(6.42256967722955,-5.29349487006409,3.62908705921399));
#67714=CARTESIAN_POINT('Ctrl Pts',(7.83727650840871,-0.30737883443838,3.84095581881909));
#67715=CARTESIAN_POINT('Ctrl Pts',(6.81742465965292,4.77421110570834,4.05282457842421));
#67716=CARTESIAN_POINT('Ctrl Pts',(1.00763813107558,8.86687601910892,4.3176605279306));
#67717=CARTESIAN_POINT('Ctrl Pts',(-6.91409890044602,5.64085818235034,4.63546366733828));
#67718=CARTESIAN_POINT('Ctrl Pts',(-8.48189338148272,-2.75101947129031,
4.95326680674595));
#67719=CARTESIAN_POINT('Ctrl Pts',(-2.28705349793356,-8.62516345681626,
5.27106994615362));
#67720=CARTESIAN_POINT('Ctrl Pts',(6.02011300233425,-6.5874918155073,5.5888730855613));
#67721=CARTESIAN_POINT('Ctrl Pts',(8.32177000704095,0.136037560988745,5.85370903506768));
#67722=CARTESIAN_POINT('Ctrl Pts',(6.16490436238276,4.84885317968135,6.0655777946728));
#67723=CARTESIAN_POINT('Ctrl Pts',(2.09297402488047,8.05542185077758,6.27744655427792));
#67724=CARTESIAN_POINT('Ctrl Pts',(-4.98357195312415,7.40275771703265,6.54228250378431));
#67725=CARTESIAN_POINT('Ctrl Pts',(-8.9211994880889,-0.190411152840623,
6.86008564319199));
#67726=CARTESIAN_POINT('Ctrl Pts',(-4.67206071950657,-7.59489755336788,
7.17788878259965));
#67727=CARTESIAN_POINT('Ctrl Pts',(3.85295055711175,-8.04852960516554,7.49569192200733));
#67728=CARTESIAN_POINT('Ctrl Pts',(8.85465174940877,-1.10993398241913,7.813495061415));
#67729=CARTESIAN_POINT('Ctrl Pts',(6.24611106307449,5.50058707593904,8.07833101092139));
#67730=CARTESIAN_POINT('Ctrl Pts',(1.54788443075806,7.68904914853577,8.29019977052652));
#67731=CARTESIAN_POINT('Ctrl Pts',(-3.63117674040154,7.48898638465389,8.50206853013162));
#67732=CARTESIAN_POINT('Ctrl Pts',(-8.59439695939712,2.40273843072248,8.76690447963802));
#67733=CARTESIAN_POINT('Ctrl Pts',(-6.6671191886872,-5.93073170032617,9.0847076190457));
#67734=CARTESIAN_POINT('Ctrl Pts',(1.3693654792293,-8.81109859239982,9.40251075845336));
#67735=CARTESIAN_POINT('Ctrl Pts',(8.15260611885662,-3.62754328002339,9.72031389786104));
#67736=CARTESIAN_POINT('Ctrl Pts',(7.45979632555549,4.89778009329165,10.0381170372687));
#67737=CARTESIAN_POINT('Ctrl Pts',(1.18701860120112,8.23779997522517,10.3029529867751));
#67738=CARTESIAN_POINT('Ctrl Pts',(-3.80847721506004,6.85659713857236,10.5148217463803));
#67739=CARTESIAN_POINT('Ctrl Pts',(-7.62090835848221,3.34546220768456,10.7266905059854));
#67740=CARTESIAN_POINT('Ctrl Pts',(-8.10013769775553,-3.74494063216588,
10.9915264554918));
#67741=CARTESIAN_POINT('Ctrl Pts',(-1.22851223754719,-8.83825856488072,
11.3093295948994));
#67742=CARTESIAN_POINT('Ctrl Pts',(6.75671894445668,-5.81870856174881,11.6271327343071));
#67743=CARTESIAN_POINT('Ctrl Pts',(8.55819728856564,2.52612666892943,11.9449358737148));
#67744=CARTESIAN_POINT('Ctrl Pts',(2.50179473315566,8.56608628103863,12.2627390131224));
#67745=CARTESIAN_POINT('Ctrl Pts',(-4.43904923015306,7.04025592743055,12.5275749626288));
#67746=CARTESIAN_POINT('Ctrl Pts',(-7.3457327618181,2.74911498672665,12.739443722234));
#67747=CARTESIAN_POINT('Ctrl Pts',(-7.97053919776979,-2.39601053592402,
12.9513124818391));
#67748=CARTESIAN_POINT('Ctrl Pts',(-3.73687540473799,-8.10386162705828,
13.2161484313455));
#67749=CARTESIAN_POINT('Ctrl Pts',(4.79688937669392,-7.52422149363303,13.5339515707531));
#67750=CARTESIAN_POINT('Ctrl Pts',(8.91674874505521,-0.0470323134403838,
13.8517547101608));
#67751=CARTESIAN_POINT('Ctrl Pts',(4.87599483198481,7.47320086548901,14.1695578495685));
#67752=CARTESIAN_POINT('Ctrl Pts',(-3.65118054584055,8.14283069225432,14.4873609889762));
#67753=CARTESIAN_POINT('Ctrl Pts',(-7.94482039878572,2.47995774610828,14.7521969384825));
#67754=CARTESIAN_POINT('Ctrl Pts',(-7.37432421124854,-2.67147252385011,
14.9640656980877));
#67755=CARTESIAN_POINT('Ctrl Pts',(-4.51306928532146,-6.99303705247811,
15.1759344576928));
#67756=CARTESIAN_POINT('Ctrl Pts',(2.41129262796859,-8.59200086844431,15.4407704071992));
#67757=CARTESIAN_POINT('Ctrl Pts',(8.53107320768763,-2.616265793562,15.7585735466068));
#67758=CARTESIAN_POINT('Ctrl Pts',(6.817724044067,5.74710875831507,16.0763766860145));
#67759=CARTESIAN_POINT('Ctrl Pts',(-1.13520985765706,8.85072626153168,16.3941798254222));
#67760=CARTESIAN_POINT('Ctrl Pts',(-8.0601819410273,3.83017990942736,16.7119829648299));
#67761=CARTESIAN_POINT('Ctrl Pts',(-7.65577531194065,-3.26488375972616,
16.9768189143363));
#67762=CARTESIAN_POINT('Ctrl Pts',(-3.88059495544502,-6.81604033219195,
17.1886876739414));
#67763=CARTESIAN_POINT('Ctrl Pts',(1.1000527157068,-8.24986336942072,17.4005564335465));
#67764=CARTESIAN_POINT('Ctrl Pts',(7.40771499469042,-4.97620031936837,17.6653923830529));
#67765=CARTESIAN_POINT('Ctrl Pts',(8.19041913672562,3.54134030308396,17.9831955224606));
#67766=CARTESIAN_POINT('Ctrl Pts',(1.46223680155422,8.79616301333324,18.3009986618682));
#67767=CARTESIAN_POINT('Ctrl Pts',(-6.60418544645305,6.00073256914073,18.6188018012759));
#67768=CARTESIAN_POINT('Ctrl Pts',(-8.61926503515426,-2.31194319022132,
18.9366049406836));
#67769=CARTESIAN_POINT('Ctrl Pts',(-3.70997536547946,-7.45026471871834,
19.20144089019));
#67770=CARTESIAN_POINT('Ctrl Pts',(1.46668719125818,-7.70494981822022,19.4133096497951));
#67771=CARTESIAN_POINT('Ctrl Pts',(6.18773830434186,-5.56617070061853,19.6251784094002));
#67772=CARTESIAN_POINT('Ctrl Pts',(8.86586766281804,1.01646527065157,19.8900143589066));
#67773=CARTESIAN_POINT('Ctrl Pts',(3.93763941419164,8.00743733171186,20.2078174983143));
#67774=CARTESIAN_POINT('Ctrl Pts',(-4.5916828416135,7.6437601285613,20.5256206377219));
#67775=CARTESIAN_POINT('Ctrl Pts',(-8.91869447358585,0.284509515337135,
20.8434237771296));
#67776=CARTESIAN_POINT('Ctrl Pts',(-5.06138570295972,-7.34977454259096,
21.1612269165373));
#67777=CARTESIAN_POINT('Ctrl Pts',(2.00788160904171,-8.07705224915103,21.4260628660437));
#67778=CARTESIAN_POINT('Ctrl Pts',(6.11341122390523,-4.91361641011203,21.6379316256488));
#67779=CARTESIAN_POINT('Ctrl Pts',(8.31987188256932,-0.223815658693506,
21.8498003852539));
#67780=CARTESIAN_POINT('Ctrl Pts',(6.08926900404114,6.52361970515354,22.1146363347603));
#67781=CARTESIAN_POINT('Ctrl Pts',(-2.19594028960663,8.64880934128916,22.432439474168));
#67782=CARTESIAN_POINT('Ctrl Pts',(-8.45240090026003,2.84034139536688,22.7502426135756));
#67783=CARTESIAN_POINT('Ctrl Pts',(-6.97321962856273,-5.56760853412987,
23.0680457529833));
#67784=CARTESIAN_POINT('Ctrl Pts',(0.914047176923553,-8.8770112548876,23.385848892391));
#67785=CARTESIAN_POINT('Ctrl Pts',(6.76668080923863,-4.84586343362311,23.6506848418974));
#67786=CARTESIAN_POINT('Ctrl Pts',(7.8400853215732,0.224689049010087,23.8625536015025));
#67787=CARTESIAN_POINT('Ctrl Pts',(6.47804714849922,5.2254441661226,24.0744223611076));
#67788=CARTESIAN_POINT('Ctrl Pts',(0.404151858925233,8.91478952841686,24.339258310614));
#67789=CARTESIAN_POINT('Ctrl Pts',(-7.28063663433841,5.15910718789769,24.6570614500217));
#67790=CARTESIAN_POINT('Ctrl Pts',(-8.27585861517074,-3.31975667823038,
24.9748645894293));
#67791=CARTESIAN_POINT('Ctrl Pts',(-1.69701030859419,-8.76037743422127,
25.292667728837));
#67792=CARTESIAN_POINT('Ctrl Pts',(6.45288855301478,-6.16417394169035,25.6104708682447));
#67793=CARTESIAN_POINT('Ctrl Pts',(8.2933980942229,0.699935455727023,25.8753068177511));
#67794=CARTESIAN_POINT('Ctrl Pts',(5.82196951471606,5.25567255334745,26.0871755773562));
#67795=CARTESIAN_POINT('Ctrl Pts',(1.54200537880764,8.1787884801584,26.2990443369613));
#67796=CARTESIAN_POINT('Ctrl Pts',(-5.47400703753924,7.04784066321128,26.5638802864678));
#67797=CARTESIAN_POINT('Ctrl Pts',(-8.88776182410288,-0.794824845804046,
26.8816834258753));
#67798=CARTESIAN_POINT('Ctrl Pts',(-4.14638080422807,-7.89418434338091,
27.1994865652831));
#67799=CARTESIAN_POINT('Ctrl Pts',(4.38977017365657,-7.76878205383336,27.5172897046907));
#67800=CARTESIAN_POINT('Ctrl Pts',(8.90952981045906,-0.507040055206927,
27.8350928440984));
#67801=CARTESIAN_POINT('Ctrl Pts',(5.8588021812506,5.91141257166313,28.0999287936048));
#67802=CARTESIAN_POINT('Ctrl Pts',(1.02300990719647,7.77630206126733,28.3117975532099));
#67803=CARTESIAN_POINT('Ctrl Pts',(-4.13056997928662,7.22556248590099,28.523666312815));
#67804=CARTESIAN_POINT('Ctrl Pts',(-8.73752521892493,1.81451484140921,28.7885022623214));
#67805=CARTESIAN_POINT('Ctrl Pts',(-6.24967801580441,-6.36911151388161,
29.1063054017291));
#67806=CARTESIAN_POINT('Ctrl Pts',(1.96360159806944,-8.69798189150852,29.4241085411368));
#67807=CARTESIAN_POINT('Ctrl Pts',(8.37979196576129,-3.06645453056966,29.7419116805444));
#67808=CARTESIAN_POINT('Ctrl Pts',(7.11056466570447,5.39227977722585,30.0597148199521));
#67809=CARTESIAN_POINT('Ctrl Pts',(0.625769470583524,8.29932371709461,30.3245507694585));
#67810=CARTESIAN_POINT('Ctrl Pts',(-4.26458687907389,6.5826075205137,30.5364195290636));
#67811=CARTESIAN_POINT('Ctrl Pts',(-7.83019273241325,2.8210713150692,30.7482882886687));
#67812=CARTESIAN_POINT('Ctrl Pts',(-7.82759440220744,-4.28550778036562,
31.0131242381751));
#67813=CARTESIAN_POINT('Ctrl Pts',(-0.626456906038276,-8.90121387914958,
31.3309273775828));
#67814=CARTESIAN_POINT('Ctrl Pts',(7.13567642164131,-5.34721817645243,31.6487305169904));
#67815=CARTESIAN_POINT('Ctrl Pts',(8.36723482303544,3.10055449777475,31.9665336563982));
#67816=CARTESIAN_POINT('Ctrl Pts',(1.9152626593684,8.7159956405836,32.2843367958058));
#67817=CARTESIAN_POINT('Ctrl Pts',(-4.90615988468414,6.72309131109787,32.5491727453122));
#67818=CARTESIAN_POINT('Ctrl Pts',(-7.51521834715023,2.24475304052566,32.7610415049173));
#67819=CARTESIAN_POINT('Ctrl Pts',(-7.78975074234866,-2.93089490830397,
32.9729102645224));
#67820=CARTESIAN_POINT('Ctrl Pts',(-3.17883992582329,-8.33857228709058,
33.2377462140288));
#67821=CARTESIAN_POINT('Ctrl Pts',(5.2959891995192,-7.18168191832974,33.5555493534365));
#67822=CARTESIAN_POINT('Ctrl Pts',(8.89941983940671,0.557625988388055,33.8733524928441));
#67823=CARTESIAN_POINT('Ctrl Pts',(4.35809662169856,7.7865942884825,34.1911556322519));
#67824=CARTESIAN_POINT('Ctrl Pts',(-4.19485799716548,7.87654603520225,34.5089587716595));
#67825=CARTESIAN_POINT('Ctrl Pts',(-8.09467877277286,1.9355973643979,34.7737947211659));
#67826=CARTESIAN_POINT('Ctrl Pts',(-7.17623150848824,-3.16530004184014,
34.9856634807711));
#67827=CARTESIAN_POINT('Ctrl Pts',(-4.02856098714868,-7.28292921593141,
35.1975322403761));
#67828=CARTESIAN_POINT('Ctrl Pts',(2.98827655480704,-8.40874629734028,35.4623681898826));
#67829=CARTESIAN_POINT('Ctrl Pts',(8.6888242006846,-2.03184418376158,35.7801713292902));
#67830=CARTESIAN_POINT('Ctrl Pts',(6.41238584802353,6.19612200953295,36.0979744686979));
#67831=CARTESIAN_POINT('Ctrl Pts',(-1.73267150616142,8.75339398343433,36.4157776081056));
#67832=CARTESIAN_POINT('Ctrl Pts',(-8.30131909715377,3.27489119029515,36.7335807475132));
#67833=CARTESIAN_POINT('Ctrl Pts',(-7.41680206625722,-3.77642803471834,
36.9984166970196));
#67834=CARTESIAN_POINT('Ctrl Pts',(-3.40954226567329,-7.0634583991753,37.2102854566248));
#67835=CARTESIAN_POINT('Ctrl Pts',(1.65685712726635,-8.15629732484478,37.4221542162298));
#67836=CARTESIAN_POINT('Ctrl Pts',(7.72805297274963,-4.46251143543848,37.6869901657363));
#67837=CARTESIAN_POINT('Ctrl Pts',(7.93147207832679,4.08849696688301,38.0047933051439));
#67838=CARTESIAN_POINT('Ctrl Pts',(0.862497716326057,8.8750615721968,38.3225964445516));
#67839=CARTESIAN_POINT('Ctrl Pts',(-6.9958350228475,5.53916501925954,38.6403995839592));
#67840=CARTESIAN_POINT('Ctrl Pts',(-8.44268355926215,-2.89100421639401,
38.958202723367));
#67841=CARTESIAN_POINT('Ctrl Pts',(-3.19631525253309,-7.68465551588802,
39.2230386728733));
#67842=CARTESIAN_POINT('Ctrl Pts',(1.98570316394913,-7.58778004181559,39.4349074324785));
#67843=CARTESIAN_POINT('Ctrl Pts',(6.55088310895129,-5.13383794877675,39.6467761920836));
#67844=CARTESIAN_POINT('Ctrl Pts',(8.77655135391446,1.6152267311884,39.91161214159));
#67845=CARTESIAN_POINT('Ctrl Pts',(3.38567948004545,8.25598154285045,40.2294152809976));
#67846=CARTESIAN_POINT('Ctrl Pts',(-5.0993594958464,7.314858368627,40.5472184204053));
#67847=CARTESIAN_POINT('Ctrl Pts',(-8.91746189895706,-0.320827146821168,
40.865021559813));
#67848=CARTESIAN_POINT('Ctrl Pts',(-4.55142913228414,-7.67602135971745,
41.1828246992206));
#67849=CARTESIAN_POINT('Ctrl Pts',(2.55088059539345,-7.92233360692975,41.4476606487271));
#67850=CARTESIAN_POINT('Ctrl Pts',(6.43248427759269,-4.487824532757,41.6595294083321));
#67851=CARTESIAN_POINT('Ctrl Pts',(8.31590220794029,0.340781542072778,41.8713981679373));
#67852=CARTESIAN_POINT('Ctrl Pts',(5.63296003724804,6.92145738120303,42.1362341174436));
#67853=CARTESIAN_POINT('Ctrl Pts',(-2.77727132720888,8.48002480848681,42.4540372568513));
#67854=CARTESIAN_POINT('Ctrl Pts',(-8.62552510820369,2.26073811590348,42.771840396259));
#67855=CARTESIAN_POINT('Ctrl Pts',(-6.57969363796116,-6.02757732493426,
43.0896435356667));
#67856=CARTESIAN_POINT('Ctrl Pts',(1.51379983280753,-8.79461318803933,43.4074466750743));
#67857=CARTESIAN_POINT('Ctrl Pts',(7.07965706273086,-4.37593618161517,43.6722826245808));
#67858=CARTESIAN_POINT('Ctrl Pts',(7.80681130486786,0.755724995272883,43.8841513841859));
#67859=CARTESIAN_POINT('Ctrl Pts',(6.10885909612371,5.6526278963992,44.096020143791));
#67860=CARTESIAN_POINT('Ctrl Pts',(-0.201195350454262,8.92167761645756,
44.3608560932973));
#67861=CARTESIAN_POINT('Ctrl Pts',(-7.61366799612502,4.65361326522414,44.6786592327051));
#67862=CARTESIAN_POINT('Ctrl Pts',(-8.03173819178576,-3.87321595570929,
44.9964623721127));
#67863=CARTESIAN_POINT('Ctrl Pts',(-1.09915724375289,-8.8552758359632,45.3142655115205));
#67864=CARTESIAN_POINT('Ctrl Pts',(6.85596749195023,-5.71248814531507,45.632068650928));
#67865=CARTESIAN_POINT('Ctrl Pts',(8.22685957920027,1.26061217492319,45.8969046004345));
#67866=CARTESIAN_POINT('Ctrl Pts',(5.45224164774619,5.6383050673828,46.1087733600396));
#67867=CARTESIAN_POINT('Ctrl Pts',(0.983940357573422,8.26451589412118,46.3206421196447));
#67868=CARTESIAN_POINT('Ctrl Pts',(-5.93925046802993,6.6604890915795,46.5854780691511));
#67869=CARTESIAN_POINT('Ctrl Pts',(-8.81342222062257,-1.3955807173089,46.9032812085587));
#67870=CARTESIAN_POINT('Ctrl Pts',(-3.60161903372427,-8.15714169037575,
47.2210843479665));
#67871=CARTESIAN_POINT('Ctrl Pts',(4.9063878437363,-7.45328216991178,47.5388874873741));
#67872=CARTESIAN_POINT('Ctrl Pts',(8.92340575765604,0.0981872969094068,
47.8566906267818));
#67873=CARTESIAN_POINT('Ctrl Pts',(5.44453079154443,6.29503344322871,48.1215265762882));
#67874=CARTESIAN_POINT('Ctrl Pts',(0.493427439442421,7.82776803311762,48.3333953358933));
#67875=CARTESIAN_POINT('Ctrl Pts',(-4.61095412314837,6.92888617785462,48.5452640954984));
#67876=CARTESIAN_POINT('Ctrl Pts',(-8.84044293923562,1.21794076176243,48.8101000450048));
#67877=CARTESIAN_POINT('Ctrl Pts',(-5.80347550407464,-6.77818034955503,
49.1279031844124));
#67878=CARTESIAN_POINT('Ctrl Pts',(2.54880112161379,-8.5448366317567,49.4457063238202));
#67879=CARTESIAN_POINT('Ctrl Pts',(8.56841358018594,-2.49125380007206,49.7635094632278));
#67880=CARTESIAN_POINT('Ctrl Pts',(6.72860982250429,5.86196391301944,50.0813126026355));
#67881=CARTESIAN_POINT('Ctrl Pts',(0.0616405167643138,8.32265354548276,
50.3461485521419));
#67882=CARTESIAN_POINT('Ctrl Pts',(-4.70107069550896,6.2783244049762,50.558017311747));
#67883=CARTESIAN_POINT('Ctrl Pts',(-8.00344215772086,2.28369770754799,50.7698860713521));
#67884=CARTESIAN_POINT('Ctrl Pts',(-7.51902811568601,-4.8063528019244,51.0347220208585));
#67885=CARTESIAN_POINT('Ctrl Pts',(-0.0215185877121976,-8.92320535053807,
51.3525251602661));
#67886=CARTESIAN_POINT('Ctrl Pts',(7.48179514989205,-4.85111961880997,51.6703282996739));
#67887=CARTESIAN_POINT('Ctrl Pts',(8.13776591363277,3.66071341577086,51.9881314390816));
#67888=CARTESIAN_POINT('Ctrl Pts',(1.31991644857489,8.82579354108318,52.3059345784892));
#67889=CARTESIAN_POINT('Ctrl Pts',(-5.35069213975294,6.37498668367476,52.5707705279956));
#67890=CARTESIAN_POINT('Ctrl Pts',(-7.65011851213803,1.73006062568215,52.7826392876008));
#67891=CARTESIAN_POINT('Ctrl Pts',(-7.57311345441759,-3.45229115196891,
52.9945080472057));
#67892=CARTESIAN_POINT('Ctrl Pts',(-2.60617526250377,-8.53490840971108,
53.2593439967123));
#67893=CARTESIAN_POINT('Ctrl Pts',(5.77071660837816,-6.80609187443695,53.5771471361199));
#67894=CARTESIAN_POINT('Ctrl Pts',(8.84113534714055,1.15971806681325,53.8949502755276));
#67895=CARTESIAN_POINT('Ctrl Pts',(3.82014222720046,8.06415340512867,54.2127534149352));
#67896=CARTESIAN_POINT('Ctrl Pts',(-4.71923049680223,7.57401310925028,54.530556554343));
#67897=CARTESIAN_POINT('Ctrl Pts',(-8.20728501981211,1.38232926432565,54.7953925038493));
#67898=CARTESIAN_POINT('Ctrl Pts',(-6.94511342020426,-3.64456068666602,
55.0072612634544));
#67899=CARTESIAN_POINT('Ctrl Pts',(-3.52551304465861,-7.53930496553799,
55.2191300230596));
#67900=CARTESIAN_POINT('Ctrl Pts',(3.55150827964952,-8.18679424442952,55.4839659725659));
#67901=CARTESIAN_POINT('Ctrl Pts',(8.80658877899636,-1.43807192279932,55.8017691119736));
#67902=CARTESIAN_POINT('Ctrl Pts',(5.97753752336905,6.6166203894183,56.1195722513813));
#67903=CARTESIAN_POINT('Ctrl Pts',(-2.32215931151299,8.61577813719931,56.4373753907889));
#67904=CARTESIAN_POINT('Ctrl Pts',(-8.50425315695961,2.70453125391184,56.7551785301966));
#67905=CARTESIAN_POINT('Ctrl Pts',(-7.14369631700244,-4.27059299417418,
57.020014479703));
#67906=CARTESIAN_POINT('Ctrl Pts',(-2.92279868749432,-7.278370068269,57.2318832393081));
#67907=CARTESIAN_POINT('Ctrl Pts',(2.20603659733405,-8.02519558158345,57.4437519989132));
#67908=CARTESIAN_POINT('Ctrl Pts',(8.0128260545997,-3.92828584496743,57.7085879484197));
#67909=CARTESIAN_POINT('Ctrl Pts',(7.63602397855986,4.61683815791143,58.0263910878273));
#67910=CARTESIAN_POINT('Ctrl Pts',(0.25878937236362,8.91311664243787,58.3441942272349));
#67911=CARTESIAN_POINT('Ctrl Pts',(-7.3552894075989,5.0521059478154,58.6619973666427));
#67912=CARTESIAN_POINT('Ctrl Pts',(-8.22724842054307,-3.45676069286183,
58.9798005060503));
#67913=CARTESIAN_POINT('Ctrl Pts',(-2.66794553283229,-7.88368113417099,
59.2446364555568));
#67914=CARTESIAN_POINT('Ctrl Pts',(2.49558082881807,-7.43569091242558,59.4565052151618));
#67915=CARTESIAN_POINT('Ctrl Pts',(6.88388041345025,-4.67787901134262,59.668373974767));
#67916=CARTESIAN_POINT('Ctrl Pts',(8.64684490546638,2.20655483545132,59.9332099242733));
#67917=CARTESIAN_POINT('Ctrl Pts',(2.81813847525576,8.4665313034189,60.2510130636811));
#67918=CARTESIAN_POINT('Ctrl Pts',(-5.58356863609584,6.95229325524742,60.5688162030886));
#67919=CARTESIAN_POINT('Ctrl Pts',(-8.87519070722709,-0.92468734599234,
60.8866193424964));
#67920=CARTESIAN_POINT('Ctrl Pts',(-4.02052665126542,-7.96694273278701,
61.204422481904));
#67921=CARTESIAN_POINT('Ctrl Pts',(3.08214029839192,-7.73115597905461,61.4692584314104));
#67922=CARTESIAN_POINT('Ctrl Pts',(6.72195470866535,-4.04137945668859,61.6811271910155));
#67923=CARTESIAN_POINT('Ctrl Pts',(8.27366232476659,0.903810448701441,61.8929959506206));
#67924=CARTESIAN_POINT('Ctrl Pts',(5.15072789940744,7.28744215533195,62.1578319001271));
#67925=CARTESIAN_POINT('Ctrl Pts',(-3.3458212196969,8.27221476651291,62.4756350395347));
#67926=CARTESIAN_POINT('Ctrl Pts',(-8.75895420713288,1.67073080366058,62.7934381789424));
#67927=CARTESIAN_POINT('Ctrl Pts',(-6.15588755971667,-6.45980689569075,
63.11124131835));
#67928=CARTESIAN_POINT('Ctrl Pts',(2.10658590420723,-8.67174186015929,63.4290444577578));
#67929=CARTESIAN_POINT('Ctrl Pts',(7.36005237125288,-3.88587064682533,63.693880407264));
#67930=CARTESIAN_POINT('Ctrl Pts',(7.73760994206874,1.28328305634092,63.9057491668694));
#67931=CARTESIAN_POINT('Ctrl Pts',(5.71155776081948,6.05379794313175,64.1176179264742));
#67932=CARTESIAN_POINT('Ctrl Pts',(-0.805616648510092,8.88750768644881,
64.3824538759809));
#67933=CARTESIAN_POINT('Ctrl Pts',(-7.9116608672323,4.1267031755862,64.7002570153883));
#67934=CARTESIAN_POINT('Ctrl Pts',(-7.75065529723538,-4.40885049467406,
65.0180601547962));
#67935=CARTESIAN_POINT('Ctrl Pts',(-0.496245800892245,-8.90942180405585,
65.3358632942037));
#67936=CARTESIAN_POINT('Ctrl Pts',(7.22749491679466,-5.23451318545963,65.6536664336115));
#67937=CARTESIAN_POINT('Ctrl Pts',(8.12246063437796,1.81548749222381,65.9185023831178));
#67938=CARTESIAN_POINT('Ctrl Pts',(5.05742228502824,5.99498981226798,66.1303711427229));
#67939=CARTESIAN_POINT('Ctrl Pts',(0.42134719233992,8.31220958199092,66.3422399023281));
#67940=CARTESIAN_POINT('Ctrl Pts',(-6.37716116319796,6.2424856074841,66.6070758518344));
#67941=CARTESIAN_POINT('Ctrl Pts',(-8.69852279597928,-1.98991405476493,
66.9248789912421));
#67942=CARTESIAN_POINT('Ctrl Pts',(-3.04028242767115,-8.38255945286813,
67.2426821306498));
#67943=CARTESIAN_POINT('Ctrl Pts',(5.4004260652692,-7.10348189911743,67.5604852700574));
#67944=CARTESIAN_POINT('Ctrl Pts',(8.89621573381947,0.702962786061858,67.8782884094652));
#67945=CARTESIAN_POINT('Ctrl Pts',(5.00520339182766,6.64968424794669,68.1431243589715));
#67946=CARTESIAN_POINT('Ctrl Pts',(-0.0384258066755255,7.84321021496693,
68.3549931185767));
#67947=CARTESIAN_POINT('Ctrl Pts',(-5.07011841966402,6.60032278010828,68.5668618781817));
#67948=CARTESIAN_POINT('Ctrl Pts',(-8.90267648752489,0.615761656414104,
68.8316978276883));
#67949=CARTESIAN_POINT('Ctrl Pts',(-5.33056510057982,-7.1560556518278,69.1495009670957));
#67950=CARTESIAN_POINT('Ctrl Pts',(3.12227093202969,-8.35236759500319,69.4673041065036));
#67951=CARTESIAN_POINT('Ctrl Pts',(8.71760291505868,-1.90458819272834,69.7851072459112));
#67952=CARTESIAN_POINT('Ctrl Pts',(6.31568957316768,6.30467099204083,70.1029103853189));
#67953=CARTESIAN_POINT('Ctrl Pts',(-0.502772112368008,8.30768209207719,
70.3677463348252));
#67954=CARTESIAN_POINT('Ctrl Pts',(-5.11591994012307,5.94514812280067,70.5796150944303));
#67955=CARTESIAN_POINT('Ctrl Pts',(-8.1398593397655,1.73581439547418,70.7914838540355));
#67956=CARTESIAN_POINT('Ctrl Pts',(-7.17585885886399,-5.30507871892191,
71.0563198035419));
#67957=CARTESIAN_POINT('Ctrl Pts',(0.583518731386589,-8.90413181077787,
71.3741229429495));
#67958=CARTESIAN_POINT('Ctrl Pts',(7.79348232585873,-4.3326958910605,71.6919260823573));
#67959=CARTESIAN_POINT('Ctrl Pts',(7.87084648811618,4.20402541266067,72.0097292217649));
#67960=CARTESIAN_POINT('Ctrl Pts',(0.718496112866162,8.89497494527636,72.3275323611726));
#67961=CARTESIAN_POINT('Ctrl Pts',(-5.7706005815723,5.99754358919117,72.5923683106789));
#67962=CARTESIAN_POINT('Ctrl Pts',(-7.74981197678148,1.20740698561282,72.8042370702841));
#67963=CARTESIAN_POINT('Ctrl Pts',(-7.32162543595896,-3.95780124157864,
73.0161058298892));
#67964=CARTESIAN_POINT('Ctrl Pts',(-2.02151445560857,-8.69196333085375,
73.2809417793956));
#67965=CARTESIAN_POINT('Ctrl Pts',(6.21888287064807,-6.3991850739513,73.5987449188032));
#67966=CARTESIAN_POINT('Ctrl Pts',(8.74217083367641,1.75648262129356,73.916548058211));
#67967=CARTESIAN_POINT('Ctrl Pts',(3.26459345311881,8.30458278096055,74.2343511976185));
#67968=CARTESIAN_POINT('Ctrl Pts',(-5.22185729667213,7.23666008718191,74.5521543370264));
#67969=CARTESIAN_POINT('Ctrl Pts',(-8.28216907153752,0.822636887797858,
74.8169902865326));
#67970=CARTESIAN_POINT('Ctrl Pts',(-6.68196928121076,-4.10696513615418,
75.0288590461378));
#67971=CARTESIAN_POINT('Ctrl Pts',(-3.00639701191772,-7.76118831963662,
75.2407278057428));
#67972=CARTESIAN_POINT('Ctrl Pts',(4.09872809405852,-7.92673324829183,75.5055637552494));
#67973=CARTESIAN_POINT('Ctrl Pts',(8.88326754126994,-0.838407728998665,
75.8233668946569));
#67974=CARTESIAN_POINT('Ctrl Pts',(5.51619802321942,7.00799436149701,76.1411700340646));
#67975=CARTESIAN_POINT('Ctrl Pts',(-2.90287476372161,8.43601988074216,76.4589731734724));
#67976=CARTESIAN_POINT('Ctrl Pts',(-8.66435079961945,2.12653204614075,76.77677631288));
#67977=CARTESIAN_POINT('Ctrl Pts',(-6.47933415350991,-6.12851160799295,
77.0945794522877));
#67978=CARTESIAN_POINT('Ctrl Pts',(1.63988578694652,-8.77075506074561,77.4123825916953));
#67979=CARTESIAN_POINT('Ctrl Pts',(8.26551738858123,-3.36361327706695,77.7301857311031));
#67980=CARTESIAN_POINT('Ctrl Pts',(7.45684676779562,3.69728324689203,77.9950216806093));
#67981=CARTESIAN_POINT('Ctrl Pts',(3.48460647847746,7.02662036791392,78.2068904402145));
#67982=CARTESIAN_POINT('Ctrl Pts',(-1.56971333319493,8.17355834568325,78.4187591998196));
#67983=CARTESIAN_POINT('Ctrl Pts',(-7.68005149993975,4.54465089995841,78.683595149326));
#67984=CARTESIAN_POINT('Ctrl Pts',(-7.97461028152683,-4.00365538448797,
79.0013982887337));
#67985=CARTESIAN_POINT('Ctrl Pts',(-0.957114982245634,-8.86536592560338,
79.3192014281413));
#67986=CARTESIAN_POINT('Ctrl Pts',(6.9363636744491,-5.61345996202913,79.6370045675491));
#67987=CARTESIAN_POINT('Ctrl Pts',(8.4730346335444,2.800791198554,79.9548077069567));
#67988=CARTESIAN_POINT('Ctrl Pts',(3.27809593601825,7.65012919672485,80.2196436564631));
#67989=CARTESIAN_POINT('Ctrl Pts',(-1.90466288199341,7.60852657288711,80.4315124160682));
#67990=CARTESIAN_POINT('Ctrl Pts',(-6.49575484723515,5.20341514208813,80.6433811756733));
#67991=CARTESIAN_POINT('Ctrl Pts',(-8.79327968646819,-1.52152827671527,
80.9082171251798));
#67992=CARTESIAN_POINT('Ctrl Pts',(-3.47354142326441,-8.21940168690237,
81.2260202645873));
#67993=CARTESIAN_POINT('Ctrl Pts',(5.02105235293711,-7.36882987433891,81.5438234039952));
#67994=CARTESIAN_POINT('Ctrl Pts',(8.92037652050399,0.225699237984256,81.8616265434027));
#67995=CARTESIAN_POINT('Ctrl Pts',(4.6330392710093,7.62704121462448,82.1794296828104));
#67996=CARTESIAN_POINT('Ctrl Pts',(-2.46623939907536,7.94908956504783,82.4442656323168));
#67997=CARTESIAN_POINT('Ctrl Pts',(-6.38425326485288,4.55617529140441,82.656134391922));
#67998=CARTESIAN_POINT('Ctrl Pts',(-8.31906383227824,-0.252068432127678,
82.8680031515269));
#67999=CARTESIAN_POINT('Ctrl Pts',(-5.70646083775828,-6.86098504659725,
83.1328391010336));
#68000=CARTESIAN_POINT('Ctrl Pts',(2.68666917777219,-8.50916361916542,83.4506422404409));
#68001=CARTESIAN_POINT('Ctrl Pts',(8.60092246953097,-2.35260555303574,83.7684453798489));
#68002=CARTESIAN_POINT('Ctrl Pts',(6.64360685990785,5.95705839106529,84.0862485192562));
#68003=CARTESIAN_POINT('Ctrl Pts',(-1.41991428712019,8.81025847953791,84.4040516586642));
#68004=CARTESIAN_POINT('Ctrl Pts',(-7.03258258710037,4.45119576593135,84.6688876081705));
#68005=CARTESIAN_POINT('Ctrl Pts',(-7.81442749145392,-0.672418024438525,
84.8807563677757));
#68006=CARTESIAN_POINT('Ctrl Pts',(-6.16880005396275,-5.58715200125982,
85.0926251273807));
#68007=CARTESIAN_POINT('Ctrl Pts',(0.106029250967578,-8.92331602372033,
85.3574610768872));
#68008=CARTESIAN_POINT('Ctrl Pts',(7.5636015661477,-4.73455257929366,85.6752642162948));
#68009=CARTESIAN_POINT('Ctrl Pts',(8.07259136044653,3.78733269572646,85.9930673557024));
#68010=CARTESIAN_POINT('Ctrl Pts',(1.19354116897602,8.84304903613462,86.3108704951103));
#68011=CARTESIAN_POINT('Ctrl Pts',(-6.79465066921202,5.78528593454319,86.6286736345177));
#68012=CARTESIAN_POINT('Ctrl Pts',(-8.23983677665961,-1.17279643819476,
86.8935095840243));
#68013=CARTESIAN_POINT('Ctrl Pts',(-5.51206719219005,-5.57983317735208,
87.1053783436294));
#68014=CARTESIAN_POINT('Ctrl Pts',(-1.07203005270189,-8.25355154812431,
87.3172471032343));
#68015=CARTESIAN_POINT('Ctrl Pts',(5.86787482937588,-6.72345566266486,87.582083052741));
#68016=CARTESIAN_POINT('Ctrl Pts',(8.82780556978323,1.30150128681965,87.8998861921484));
#68017=CARTESIAN_POINT('Ctrl Pts',(3.6884146331611,8.11826445213714,88.2176893315562));
#68018=CARTESIAN_POINT('Ctrl Pts',(-4.82661537364263,7.50518759341862,88.5354924709639));
#68019=CARTESIAN_POINT('Ctrl Pts',(-8.923945428409,-0.00300862480821861,
88.8532956103715));
#68020=CARTESIAN_POINT('Ctrl Pts',(-5.51136114809949,-6.23660643993697,
89.1181315598778));
#68021=CARTESIAN_POINT('Ctrl Pts',(-0.576886875348588,-7.82206012194633,
89.3300003194832));
#68022=CARTESIAN_POINT('Ctrl Pts',(4.53679143195664,-6.9776704632971,89.5418690790879));
#68023=CARTESIAN_POINT('Ctrl Pts',(8.82695009077069,-1.31215972963913,89.8067050285948));
#68024=CARTESIAN_POINT('Ctrl Pts',(5.87543847491016,6.71589752043862,90.1245081680019));
#68025=CARTESIAN_POINT('Ctrl Pts',(-2.45752071223338,8.57153499496415,90.4423113074101));
#68026=CARTESIAN_POINT('Ctrl Pts',(-8.54135561236971,2.58249899913411,90.7601144468174));
#68027=CARTESIAN_POINT('Ctrl Pts',(-6.79074821486224,-5.78986612482438,
91.0779175862253));
#68028=CARTESIAN_POINT('Ctrl Pts',(-0.150402741474938,-8.32152273365876,
91.3427535357315));
#68029=CARTESIAN_POINT('Ctrl Pts',(4.63384148188355,-6.32810683688797,91.5546222953368));
#68030=CARTESIAN_POINT('Ctrl Pts',(7.97863002593425,-2.36892897755592,91.7664910549419));
#68031=CARTESIAN_POINT('Ctrl Pts',(7.56986287027127,4.72588480459817,92.0313270044481));
#68032=CARTESIAN_POINT('Ctrl Pts',(0.11668831364906,8.92246830282663,92.349130143856));
#68033=CARTESIAN_POINT('Ctrl Pts',(-7.42962970550756,4.93064120170904,92.6669332832636));
#68034=CARTESIAN_POINT('Ctrl Pts',(-8.1763465937579,-3.57371139800513,92.9847364226712));
#68035=CARTESIAN_POINT('Ctrl Pts',(-1.41397337222863,-8.81121389841784,
93.3025395620791));
#68036=CARTESIAN_POINT('Ctrl Pts',(5.28239501954281,-6.43169219171388,93.5673755115852));
#68037=CARTESIAN_POINT('Ctrl Pts',(7.63123132444705,-1.81155499256043,93.7792442711905));
#68038=CARTESIAN_POINT('Ctrl Pts',(7.60950331181201,3.37132332162994,93.9911130307955));
#68039=CARTESIAN_POINT('Ctrl Pts',(2.69705657370164,8.5066266462856,94.2559489803021));
#68040=CARTESIAN_POINT('Ctrl Pts',(-5.69779762101329,6.86725265644592,94.5737521197095));
#68041=CARTESIAN_POINT('Ctrl Pts',(-8.85300151361534,-1.06535647596267,
94.8915552591175));
#68042=CARTESIAN_POINT('Ctrl Pts',(-3.90593362552959,-8.02295078449604,
95.2093583985248));
#68043=CARTESIAN_POINT('Ctrl Pts',(4.63818100932635,-7.62391552850421,95.5271615379327));
#68044=CARTESIAN_POINT('Ctrl Pts',(8.19207488967919,-1.46978590050783,95.791997487439));
#68045=CARTESIAN_POINT('Ctrl Pts',(6.98358965896691,3.57027989007352,96.0038662470443));
#68046=CARTESIAN_POINT('Ctrl Pts',(3.60572340047096,7.50127458174534,96.2157350066492));
#68047=CARTESIAN_POINT('Ctrl Pts',(-3.46398955889884,8.2242074023509,96.4805709561558));
#68048=CARTESIAN_POINT('Ctrl Pts',(-8.79075003479858,1.53191729645467,96.7983740955633));
#68049=CARTESIAN_POINT('Ctrl Pts',(-6.0477674669237,-6.55249028133353,97.1161772349711));
#68050=CARTESIAN_POINT('Ctrl Pts',(2.23013516258891,-8.64005520434183,97.4339803743786));
#68051=CARTESIAN_POINT('Ctrl Pts',(8.47492411579095,-2.79508001542504,97.7517835137864));
#68052=CARTESIAN_POINT('Ctrl Pts',(7.1888382435156,4.19415859261561,98.0166194632927));
#68053=CARTESIAN_POINT('Ctrl Pts',(3.00026030903199,7.24678281007098,98.2284882228979));
#68054=CARTESIAN_POINT('Ctrl Pts',(-2.12031794486745,8.04826772691589,98.440356982503));
#68055=CARTESIAN_POINT('Ctrl Pts',(-7.97047294154431,4.01352365748019,98.7051929320094));
#68056=CARTESIAN_POINT('Ctrl Pts',(-7.68483079945345,-4.53513311395154,
99.022996071417));
#68057=CARTESIAN_POINT('Ctrl Pts',(-0.353838000969954,-8.90984954362422,
99.3407992108247));
#68058=CARTESIAN_POINT('Ctrl Pts',(7.3009875276655,-5.13026684475196,99.6586023502325));
#68059=CARTESIAN_POINT('Ctrl Pts',(8.26364874175473,3.36881589493082,99.97640548964));
#68060=CARTESIAN_POINT('Ctrl Pts',(2.75187762938652,7.85477759738149,100.241241439146));
#68061=CARTESIAN_POINT('Ctrl Pts',(-2.41613310275605,7.46188473832575,100.453110198751));
#68062=CARTESIAN_POINT('Ctrl Pts',(-6.83359668512604,4.75103335459544,100.664978958356));
#68063=CARTESIAN_POINT('Ctrl Pts',(-8.66988721951361,-2.11420591758654,
100.929814907864));
#68064=CARTESIAN_POINT('Ctrl Pts',(-2.90827845038575,-8.43599272359275,
101.247618047271));
#68065=CARTESIAN_POINT('Ctrl Pts',(5.50910097438566,-7.0114496842646,101.565421186678));
#68066=CARTESIAN_POINT('Ctrl Pts',(8.88454820327112,0.829975904011698,101.883224326085));
#68067=CARTESIAN_POINT('Ctrl Pts',(4.10526984608823,7.92360842999213,102.201027465493));
#68068=CARTESIAN_POINT('Ctrl Pts',(-2.99950791027979,7.76358898239801,102.465863415));
#68069=CARTESIAN_POINT('Ctrl Pts',(-6.67846881235397,4.11284297544998,102.677732174605));
#68070=CARTESIAN_POINT('Ctrl Pts',(-8.28283137121611,-0.815515829056787,
102.88960093421));
#68071=CARTESIAN_POINT('Ctrl Pts',(-5.22815955816402,-7.23209227647307,
103.154436883716));
#68072=CARTESIAN_POINT('Ctrl Pts',(3.25740314075584,-8.30742929889158,103.472240023124));
#68073=CARTESIAN_POINT('Ctrl Pts',(8.74063673591143,-1.76405489477698,103.790043162533));
#68074=CARTESIAN_POINT('Ctrl Pts',(6.22443485579875,6.39378350457737,104.107846301939));
#68075=CARTESIAN_POINT('Ctrl Pts',(-2.01397713256718,8.69371653382717,104.425649441348));
#68076=CARTESIAN_POINT('Ctrl Pts',(-7.31818876878027,3.9641486773256,104.690485390853));
#68077=CARTESIAN_POINT('Ctrl Pts',(-7.75085676495864,-1.20068414971929,
104.902354150459));
#68078=CARTESIAN_POINT('Ctrl Pts',(-5.77580001840686,-5.99253666979313,
105.114222910065));
#68079=CARTESIAN_POINT('Ctrl Pts',(0.710780611675296,-8.89559452668069,
105.37905885957));
#68080=CARTESIAN_POINT('Ctrl Pts',(7.86719727708827,-4.21085071937526,105.696861998978));
#68081=CARTESIAN_POINT('Ctrl Pts',(7.79723729390108,4.32593467398078,106.014665138385));
#68082=CARTESIAN_POINT('Ctrl Pts',(0.591241515787013,8.90362231046995,106.332468277793));
#68083=CARTESIAN_POINT('Ctrl Pts',(-7.17125483096129,5.31130070796763,106.650271417201));
#68084=CARTESIAN_POINT('Ctrl Pts',(-8.141361823899,-1.728753667763,106.915107366707));
#68085=CARTESIAN_POINT('Ctrl Pts',(-5.12107452753105,-5.94070860266393,
107.126976126312));
#68086=CARTESIAN_POINT('Ctrl Pts',(-0.509977566734008,-8.3072428923724,
107.338844885917));
#68087=CARTESIAN_POINT('Ctrl Pts',(6.31021885650242,-6.31014651526292,107.603680835425));
#68088=CARTESIAN_POINT('Ctrl Pts',(8.71925157619185,1.89702628568087,107.921483974831));
#68089=CARTESIAN_POINT('Ctrl Pts',(3.12951416104503,8.3496563604001,108.239287114239));
#68090=CARTESIAN_POINT('Ctrl Pts',(-5.32435630946186,7.16067641130234,108.557090253647));
#68091=CARTESIAN_POINT('Ctrl Pts',(-8.90320721817968,-0.608039711858129,
108.874893393056));
#68092=CARTESIAN_POINT('Ctrl Pts',(-5.07584128491461,-6.59592274377136,
109.139729342561));
#68093=CARTESIAN_POINT('Ctrl Pts',(-0.0452285797699074,-7.84317393622409,
109.351598102166));
#68094=CARTESIAN_POINT('Ctrl Pts',(4.99943392320907,-6.65402299657202,109.563466861771));
#68095=CARTESIAN_POINT('Ctrl Pts',(8.89560267463199,-0.710678630693007,
109.828302811278));
#68096=CARTESIAN_POINT('Ctrl Pts',(5.40658522006346,7.09879518197837,110.146105950685));
#68097=CARTESIAN_POINT('Ctrl Pts',(-3.0330106934329,8.38519328068666,110.463909090093));
#68098=CARTESIAN_POINT('Ctrl Pts',(-8.6967935774011,1.99745794688234,110.7817122295));
#68099=CARTESIAN_POINT('Ctrl Pts',(-6.38257316774903,-6.23695204562081,
111.099515368908));
#68100=CARTESIAN_POINT('Ctrl Pts',(0.414137460974179,-8.31257190975582,
111.364351318415));
#68101=CARTESIAN_POINT('Ctrl Pts',(5.05222064422742,-5.99937409904855,111.57622007802));
#68102=CARTESIAN_POINT('Ctrl Pts',(8.1208829209,-1.8225318039691,111.788088837625));
#68103=CARTESIAN_POINT('Ctrl Pts',(7.23203233929537,5.22824246802203,112.052924787131));
#68104=CARTESIAN_POINT('Ctrl Pts',(-0.488518050920525,8.90984887029028,
112.370727926539));
#68105=CARTESIAN_POINT('Ctrl Pts',(-7.74682837710603,4.41557134656612,112.688531065946));
#68106=CARTESIAN_POINT('Ctrl Pts',(-7.91523717632062,-4.11983946532877,
113.006334205354));
#68107=CARTESIAN_POINT('Ctrl Pts',(-0.813324901639997,-8.88680559399253,
113.324137344762));
#68108=CARTESIAN_POINT('Ctrl Pts',(5.7063048668929,-6.05874957045746,113.588973294268));
#68109=CARTESIAN_POINT('Ctrl Pts',(7.7364939794529,-1.28999376904755,113.800842053873));
#68110=CARTESIAN_POINT('Ctrl Pts',(7.36342000237286,3.87948546331845,114.012710813478));
#68111=CARTESIAN_POINT('Ctrl Pts',(2.11410652406723,8.66991145663782,114.277546762985));
#68112=CARTESIAN_POINT('Ctrl Pts',(-6.15028234787188,6.46514375856746,114.595349902392));
#68113=CARTESIAN_POINT('Ctrl Pts',(-8.76040001640918,-1.66313311958161,
114.9131530418));
#68114=CARTESIAN_POINT('Ctrl Pts',(-3.35299484466143,-8.26930966581624,
115.230956181208));
#68115=CARTESIAN_POINT('Ctrl Pts',(5.14440521840749,-7.29190688433863,115.548759320616));
#68116=CARTESIAN_POINT('Ctrl Pts',(8.27287529507401,-0.910986247753953,
115.813595270122));
#68117=CARTESIAN_POINT('Ctrl Pts',(6.72545745995588,4.03554766699847,116.025464029727));
#68118=CARTESIAN_POINT('Ctrl Pts',(3.08884473663849,7.72847978482084,116.237332789332));
#68119=CARTESIAN_POINT('Ctrl Pts',(-4.01361503236695,7.97042692915515,116.50216873884));
#68120=CARTESIAN_POINT('Ctrl Pts',(-8.87438534375087,0.932384871234997,
116.819971878246));
#68121=CARTESIAN_POINT('Ctrl Pts',(-5.58959658892818,-6.94744774676236,
117.137775017654));
#68122=CARTESIAN_POINT('Ctrl Pts',(2.81079399181202,-8.46897242368175,117.455578157061));
#68123=CARTESIAN_POINT('Ctrl Pts',(8.64492780352305,-2.21405382340118,117.773381296471));
#68124=CARTESIAN_POINT('Ctrl Pts',(6.88793517002941,4.6719065364063,118.038217245975));
#68125=CARTESIAN_POINT('Ctrl Pts',(2.50202921685677,7.43352358012588,118.250086005581));
#68126=CARTESIAN_POINT('Ctrl Pts',(-2.66110663942737,7.88599220422133,118.461954765186));
#68127=CARTESIAN_POINT('Ctrl Pts',(-8.22424711370316,3.46389527465665,118.726790714692));
#68128=CARTESIAN_POINT('Ctrl Pts',(-7.35966857159775,-5.04572445677769,
119.0445938541));
#68129=CARTESIAN_POINT('Ctrl Pts',(0.251058507001858,-8.91333775008066,
119.362396993508));
#68130=CARTESIAN_POINT('Ctrl Pts',(7.63201670400195,-4.62345950640031,119.680200132915));
#68131=CARTESIAN_POINT('Ctrl Pts',(8.01623022889107,3.92133446398752,119.998003272323));
#68132=CARTESIAN_POINT('Ctrl Pts',(2.21299639959071,8.02327916296338,120.262839221829));
#68133=CARTESIAN_POINT('Ctrl Pts',(-2.91648471317105,7.28090241221048,120.474707981436));
#68134=CARTESIAN_POINT('Ctrl Pts',(-7.13998954245359,4.27678745381348,120.686576741039));
#68135=CARTESIAN_POINT('Ctrl Pts',(-8.50659572611224,-2.6971540952516,120.951412690547));
#68136=CARTESIAN_POINT('Ctrl Pts',(-2.32963131029981,-8.61376077770682,
121.269215829955));
#68137=CARTESIAN_POINT('Ctrl Pts',(5.97179636684307,-6.62180250188054,121.587018969362));
#68138=CARTESIAN_POINT('Ctrl Pts',(8.80783277429343,1.43043301051482,121.904822108769));
#68139=CARTESIAN_POINT('Ctrl Pts',(3.55860773798312,8.1837107737389,122.222625248177));
#68140=CARTESIAN_POINT('Ctrl Pts',(-3.51897252243771,7.54235997402486,122.487461197683));
#68141=CARTESIAN_POINT('Ctrl Pts',(-6.94194970780889,3.65058314143714,122.699329957288));
#68142=CARTESIAN_POINT('Ctrl Pts',(-8.20848089228814,-1.37521017753044,
122.911198716893));
#68143=CARTESIAN_POINT('Ctrl Pts',(-4.72579802181384,-7.56991704829477,
123.1760346664));
#68144=CARTESIAN_POINT('Ctrl Pts',(3.81314636825754,-8.06746376203405,123.493837805807));
#68145=CARTESIAN_POINT('Ctrl Pts',(8.84012614320339,-1.16738596582406,123.811640945215));
#68146=CARTESIAN_POINT('Ctrl Pts',(5.77661768343671,6.80108409864888,124.129444084624));
#68147=CARTESIAN_POINT('Ctrl Pts',(-2.59877155208799,8.53716565852516,124.44724722403));
#68148=CARTESIAN_POINT('Ctrl Pts',(-7.57011627027233,3.45885837322116,124.712083173537));
#68149=CARTESIAN_POINT('Ctrl Pts',(-7.65161619806151,-1.72342466497812,
124.923951933143));
#68150=CARTESIAN_POINT('Ctrl Pts',(-5.35621945486108,-6.37034337715102,
125.135820692747));
#68151=CARTESIAN_POINT('Ctrl Pts',(1.31226092353452,-8.82693504732008,125.400656642255));
#68152=CARTESIAN_POINT('Ctrl Pts',(8.13458774259943,-3.66777030843524,125.718459781661));
#68153=CARTESIAN_POINT('Ctrl Pts',(7.48599994134832,4.84462847895318,126.036262921069));
#68154=CARTESIAN_POINT('Ctrl Pts',(-0.0137790611847593,8.92322065820189,
126.354066060476));
#68155=CARTESIAN_POINT('Ctrl Pts',(-7.51485651011302,4.81287260307762,126.671869199884));
#68156=CARTESIAN_POINT('Ctrl Pts',(-8.00541990639399,-2.27675508427092,
126.93670514939));
#68157=CARTESIAN_POINT('Ctrl Pts',(-4.70651441519925,-6.27424458224373,
127.148573908996));
#68158=CARTESIAN_POINT('Ctrl Pts',(0.0544218621563285,-8.32270387869009,
127.360442668602));
#68159=CARTESIAN_POINT('Ctrl Pts',(6.72352293275359,-5.86779774990415,127.625278618107));
#68160=CARTESIAN_POINT('Ctrl Pts',(8.57057113957244,2.4838210722627,127.943081757516));
#68161=CARTESIAN_POINT('Ctrl Pts',(2.55621150422421,8.54262272177712,128.260884896923));
#68162=CARTESIAN_POINT('Ctrl Pts',(-5.79759428441931,6.78321142901773,128.578688036331));
#68163=CARTESIAN_POINT('Ctrl Pts',(-8.84149599162147,-1.21027256896321,
128.896491175739));
#68164=CARTESIAN_POINT('Ctrl Pts',(-4.61696213975944,-6.9248842727855,129.161327125244));
#68165=CARTESIAN_POINT('Ctrl Pts',(0.486637860052813,-7.82819306171326,
129.373195884849));
#68166=CARTESIAN_POINT('Ctrl Pts',(5.43906876308912,-6.29975337468319,129.585064644454));
#68167=CARTESIAN_POINT('Ctrl Pts',(8.92331723866387,-0.105926952232459,
129.849900593961));
#68168=CARTESIAN_POINT('Ctrl Pts',(4.9128505826903,7.44902382394148,130.167703733368));
#68169=CARTESIAN_POINT('Ctrl Pts',(-3.59454260383601,8.16026247679319,130.485506872776));
#68170=CARTESIAN_POINT('Ctrl Pts',(-8.81220845226687,1.40322449069441,130.803310012184));
#68171=CARTESIAN_POINT('Ctrl Pts',(-5.94502519150861,-6.6553351931643,131.121113151591));
#68172=CARTESIAN_POINT('Ctrl Pts',(0.976771781583879,-8.26536620351122,
131.385949101099));
#68173=CARTESIAN_POINT('Ctrl Pts',(5.44734922800118,-5.64303193385323,131.597817860703));
#68174=CARTESIAN_POINT('Ctrl Pts',(8.22576309608399,-1.26774724552918,131.809686620308));
#68175=CARTESIAN_POINT('Ctrl Pts',(6.86091962450978,5.70653949141333,132.074522569815));
#68176=CARTESIAN_POINT('Ctrl Pts',(-1.0914762303603,8.8562258562012,132.392325709222));
#68177=CARTESIAN_POINT('Ctrl Pts',(-8.02837574712145,3.88018080557894,132.71012884863));
#68178=CARTESIAN_POINT('Ctrl Pts',(-7.6177014313671,-4.64700782009627,133.027931988037));
#68179=CARTESIAN_POINT('Ctrl Pts',(-0.208933468132588,-8.92149975435394,
133.345735127445));
#68180=CARTESIAN_POINT('Ctrl Pts',(6.10395400652709,-5.65792427288009,133.610571076951));
#68181=CARTESIAN_POINT('Ctrl Pts',(7.80615289230366,-0.762495928036403,
133.822439836557));
#68182=CARTESIAN_POINT('Ctrl Pts',(7.08344985635885,4.36979401389729,134.034308596162));
#68183=CARTESIAN_POINT('Ctrl Pts',(1.52142724776122,8.79329688972305,134.299144545668));
#68184=CARTESIAN_POINT('Ctrl Pts',(-6.57446315987215,6.03328193746754,134.616947685076));
#68185=CARTESIAN_POINT('Ctrl Pts',(-8.62748270894221,-2.25325593926971,
134.934750824484));
#68186=CARTESIAN_POINT('Ctrl Pts',(-2.78462540951867,-8.4776127598606,135.252553963892));
#68187=CARTESIAN_POINT('Ctrl Pts',(5.62695461077901,-6.92634051063592,135.5703571033));
#68188=CARTESIAN_POINT('Ctrl Pts',(8.31560350398447,-0.347994189556737,
135.835193052805));
#68189=CARTESIAN_POINT('Ctrl Pts',(6.43637436071595,4.48224364654699,136.047061812411));
#68190=CARTESIAN_POINT('Ctrl Pts',(2.55775105087846,7.92011812747601,136.258930572016));
#68191=CARTESIAN_POINT('Ctrl Pts',(-4.54476964356802,7.67996614236977,136.523766521522));
#68192=CARTESIAN_POINT('Ctrl Pts',(-8.91718027611874,0.328561563009237,
136.84156966093));
#68193=CARTESIAN_POINT('Ctrl Pts',(-5.10570210069917,-7.31043270127474,
137.159372800337));
#68194=CARTESIAN_POINT('Ctrl Pts',(3.37851740289849,-8.25891499749212,137.477175939745));
#68195=CARTESIAN_POINT('Ctrl Pts',(8.77514709004157,-1.62283844210692,137.794979079154));
#68196=CARTESIAN_POINT('Ctrl Pts',(6.55533346555773,5.12815412666026,138.05981502866));
#68197=CARTESIAN_POINT('Ctrl Pts',(1.99228365787784,7.58605489334511,138.271683788265));
#68198=CARTESIAN_POINT('Ctrl Pts',(-3.18964878472523,7.68742494087226,138.483552547869));
#68199=CARTESIAN_POINT('Ctrl Pts',(-8.44017287876276,2.89832586809018,138.748388497376));
#68200=CARTESIAN_POINT('Ctrl Pts',(-7.00063677144394,-5.5330951168216,139.066191636784));
#68201=CARTESIAN_POINT('Ctrl Pts',(0.854799630846115,-8.87580631898063,
139.383994776191));
#68202=CARTESIAN_POINT('Ctrl Pts',(7.92792294796447,-4.09537477022881,139.7017979156));
#68203=CARTESIAN_POINT('Ctrl Pts',(7.73192061330253,4.45580685068717,140.019601055006));
#68204=CARTESIAN_POINT('Ctrl Pts',(1.66393084684311,8.15485718626432,140.284437004514));
#68205=CARTESIAN_POINT('Ctrl Pts',(-3.40341451132808,7.06641299970321,140.496305764118));
#68206=CARTESIAN_POINT('Ctrl Pts',(-7.41352380164428,3.78285955778124,140.708174523723));
#68207=CARTESIAN_POINT('Ctrl Pts',(-8.30415644281345,-3.26768983141359,
140.973010473231));
#68208=CARTESIAN_POINT('Ctrl Pts',(-1.74026308741985,-8.75188786285867,
141.290813612637));
#68209=CARTESIAN_POINT('Ctrl Pts',(6.40700924608265,-6.20168144470193,141.608616752046));
#68210=CARTESIAN_POINT('Ctrl Pts',(8.69058324707021,2.02430719092564,141.926419891452));
#68211=CARTESIAN_POINT('Ctrl Pts',(2.99556873452046,8.40615126070251,142.24422303086));
#68212=CARTESIAN_POINT('Ctrl Pts',(-4.02224264253235,7.28642063814767,142.509058980366));
#68213=CARTESIAN_POINT('Ctrl Pts',(-7.17348339460544,3.17152313654336,142.720927739972));
#68214=CARTESIAN_POINT('Ctrl Pts',(-8.09635456321866,-1.92857573822395,
142.932796499578));
#68215=CARTESIAN_POINT('Ctrl Pts',(-4.20168812055101,-7.87290467353922,
143.197632449083));
#68216=CARTESIAN_POINT('Ctrl Pts',(4.35134130057544,-7.79037134311117,143.515435588491));
#68217=CARTESIAN_POINT('Ctrl Pts',(8.89893283649567,-0.565344666760167,
143.8332387279));
#68218=CARTESIAN_POINT('Ctrl Pts',(5.30221622019615,7.17708575479655,144.151041867307));
#68219=CARTESIAN_POINT('Ctrl Pts',(-3.17160629166672,8.3413263089766,144.468845006715));
#68220=CARTESIAN_POINT('Ctrl Pts',(-7.78720570827248,2.93765022536944,144.73368095622));
#68221=CARTESIAN_POINT('Ctrl Pts',(-7.51716250103231,-2.23823389140988,
144.945549715825));
#68222=CARTESIAN_POINT('Ctrl Pts',(-4.91198929433456,-6.71883343777705,
145.15741847543));
#68223=CARTESIAN_POINT('Ctrl Pts',(1.90770214269294,-8.71765355949647,145.422254424937));
#68224=CARTESIAN_POINT('Ctrl Pts',(8.36454241906866,-3.10781063135707,145.740057564344));
#68225=CARTESIAN_POINT('Ctrl Pts',(7.14031163116602,5.34102705691939,146.057860703752));
#68226=CARTESIAN_POINT('Ctrl Pts',(-0.618736222637683,8.90175388337603,
146.37566384316));
#68227=CARTESIAN_POINT('Ctrl Pts',(-7.82387444120206,4.29229541822987,146.693466982568));
#68228=CARTESIAN_POINT('Ctrl Pts',(-7.83263662343708,-2.81427876870812,
146.958302932074));
#68229=CARTESIAN_POINT('Ctrl Pts',(-4.27029469863186,-6.57890615089385,
147.170171691679));
#68230=CARTESIAN_POINT('Ctrl Pts',(0.618570879103147,-8.2998633925873,147.382040451284));
#68231=CARTESIAN_POINT('Ctrl Pts',(7.10588492607867,-5.39844499810615,147.646876400792));
#68232=CARTESIAN_POINT('Ctrl Pts',(8.3824486383776,3.05918505229256,147.964679540198));
#68233=CARTESIAN_POINT('Ctrl Pts',(1.97114476862672,8.69627574122246,148.282482679606));
#68234=CARTESIAN_POINT('Ctrl Pts',(-6.24415093653934,6.37452929401478,148.600285819015));
#68235=CARTESIAN_POINT('Ctrl Pts',(-8.73909673220554,-1.80693476545242,
148.918088958421));
#68236=CARTESIAN_POINT('Ctrl Pts',(-4.13683377657115,-7.22197874387156,
149.182924907929));
#68237=CARTESIAN_POINT('Ctrl Pts',(1.01626246935375,-7.77718428549169,149.394793667533));
#68238=CARTESIAN_POINT('Ctrl Pts',(5.85367832461859,-5.91649721289159,149.606662427138));
#68239=CARTESIAN_POINT('Ctrl Pts',(8.909954357225,0.499323352786752,149.871498376644));
#68240=CARTESIAN_POINT('Ctrl Pts',(4.39652669300149,7.76495297395151,150.189301516052));
#68241=CARTESIAN_POINT('Ctrl Pts',(-4.13956870112755,7.8978119229406,150.50710465546));
#68242=CARTESIAN_POINT('Ctrl Pts',(-8.88700008103003,0.802468590361602,
150.824907794867));
#68243=CARTESIAN_POINT('Ctrl Pts',(-5.4802548365995,-7.04296170243578,151.142710934275));
#68244=CARTESIAN_POINT('Ctrl Pts',(1.53515019871226,-8.18034727796208,151.407546883781));
#68245=CARTESIAN_POINT('Ctrl Pts',(5.817089426409,-5.26042064170382,151.619415643387));
#68246=CARTESIAN_POINT('Ctrl Pts',(8.29356557029805,-0.707857898752759,
151.831284402991));
#68247=CARTESIAN_POINT('Ctrl Pts',(6.45658054965811,6.16012403831793,152.096120352499));
#68248=CARTESIAN_POINT('Ctrl Pts',(-1.68663607804514,8.75924487711618,152.413923491905));
#68249=CARTESIAN_POINT('Ctrl Pts',(-8.27807529560295,3.33170044403166,152.731726631313));
#68250=CARTESIAN_POINT('Ctrl Pts',(-7.27525669696981,-5.1619012277632,153.049529770721));
#68251=CARTESIAN_POINT('Ctrl Pts',(-0.899851274104358,-8.27397708193549,
153.314365720227));
#68252=CARTESIAN_POINT('Ctrl Pts',(4.06460834341926,-6.71766665604379,153.526237920521));
#68253=CARTESIAN_POINT('Ctrl Pts',(5.88183385080656,-4.89010705830048,153.632175741013));
#68254=CARTESIAN_POINT('Ctrl Pts',(6.51518125436024,-3.80590017975039,153.685146371603));
#68255=CARTESIAN_POINT('Ctrl Pts',(4.14970254892029,-5.82589768344819,-0.222854153409353));
#68256=CARTESIAN_POINT('Ctrl Pts',(5.12020403053176,-5.13464909858868,-0.169830221776262));
#68257=CARTESIAN_POINT('Ctrl Pts',(6.69075495720071,-3.26142663595671,-0.0638391002418928));
#68258=CARTESIAN_POINT('Ctrl Pts',(7.73384029383181,1.56021684963465,0.148086401095035));
#68259=CARTESIAN_POINT('Ctrl Pts',(4.24822985914703,7.31166922656103,0.412922350601427));
#68260=CARTESIAN_POINT('Ctrl Pts',(-3.85638135699804,7.5288227374144,0.730725490009101));
#68261=CARTESIAN_POINT('Ctrl Pts',(-8.41413174439718,0.839900777573334,
1.04852862941677));
#68262=CARTESIAN_POINT('Ctrl Pts',(-5.26093362085182,-6.62453301130198,
1.36633176882444));
#68263=CARTESIAN_POINT('Ctrl Pts',(1.38064608400363,-7.76882450453534,1.63116771833084));
#68264=CARTESIAN_POINT('Ctrl Pts',(5.46582045917633,-5.03983377869041,1.84303647793595));
#68265=CARTESIAN_POINT('Ctrl Pts',(7.85460539252143,-0.74661404229422,2.05490523754107));
#68266=CARTESIAN_POINT('Ctrl Pts',(6.17824832881788,5.77865494324373,2.31974118704746));
#68267=CARTESIAN_POINT('Ctrl Pts',(-1.52093803950862,8.32093582721797,2.63754432645514));
#68268=CARTESIAN_POINT('Ctrl Pts',(-7.81158451531416,3.22961110439484,2.9553474658628));
#68269=CARTESIAN_POINT('Ctrl Pts',(-6.95293978484151,-4.81756640596561,
3.27315060527048));
#68270=CARTESIAN_POINT('Ctrl Pts',(0.293939508506351,-8.4544249858399,3.59095374467815));
#68271=CARTESIAN_POINT('Ctrl Pts',(6.08833921177905,-5.01802144693415,3.85578969418455));
#68272=CARTESIAN_POINT('Ctrl Pts',(7.42942471280202,-0.291382842792715,
4.06765845378966));
#68273=CARTESIAN_POINT('Ctrl Pts',(6.46264594464048,4.52576120477877,4.27952721339478));
#68274=CARTESIAN_POINT('Ctrl Pts',(0.955200652235128,8.40544387467254,4.54436316290117));
#68275=CARTESIAN_POINT('Ctrl Pts',(-6.55428925885352,5.34730797572404,4.86216630230884));
#68276=CARTESIAN_POINT('Ctrl Pts',(-8.04049572987898,-2.60785644394081,
5.17996944171652));
#68277=CARTESIAN_POINT('Ctrl Pts',(-2.16803525546429,-8.17631003184262,
5.49777258112419));
#68278=CARTESIAN_POINT('Ctrl Pts',(5.70682637845079,-6.24467880353645,5.81557572053187));
#68279=CARTESIAN_POINT('Ctrl Pts',(7.88870517433334,0.128958167596947,6.08041167003825));
#68280=CARTESIAN_POINT('Ctrl Pts',(5.84408279748823,4.59651890592599,6.29228042964337));
#68281=CARTESIAN_POINT('Ctrl Pts',(1.98405567635904,7.6362177736106,6.50414918924849));
#68282=CARTESIAN_POINT('Ctrl Pts',(-4.7242269156689,7.01751827523279,6.76898513875488));
#68283=CARTESIAN_POINT('Ctrl Pts',(-8.45694035083907,-0.180502158241452,
7.08678827816255));
#68284=CARTESIAN_POINT('Ctrl Pts',(-4.42892672371275,-7.19965915629606,
7.40459141757022));
#68285=CARTESIAN_POINT('Ctrl Pts',(3.65244304644529,-7.62968420039558,7.7223945569779));
#68286=CARTESIAN_POINT('Ctrl Pts',(8.39385575585232,-1.05217302843921,8.04019769638557));
#68287=CARTESIAN_POINT('Ctrl Pts',(5.92106350224164,5.21433657636706,8.30503364589196));
#68288=CARTESIAN_POINT('Ctrl Pts',(1.46733253957555,7.28891110333928,8.51690240549708));
#68289=CARTESIAN_POINT('Ctrl Pts',(-3.44221033706579,7.09925960380392,8.72877116510219));
#68290=CARTESIAN_POINT('Ctrl Pts',(-8.14714462265909,2.27769994544157,8.9936071146086));
#68291=CARTESIAN_POINT('Ctrl Pts',(-6.3201623689668,-5.62209647855652,9.31141025401626));
#68292=CARTESIAN_POINT('Ctrl Pts',(1.29810371260021,-8.35256910472367,9.62921339342394));
#68293=CARTESIAN_POINT('Ctrl Pts',(7.72834457329497,-3.43876596193245,9.9470165328316));
#68294=CARTESIAN_POINT('Ctrl Pts',(7.07158859510588,4.64289966341321,10.2648196722393));
#68295=CARTESIAN_POINT('Ctrl Pts',(1.1252461643865,7.80910494218149,10.5296556217457));
#68296=CARTESIAN_POINT('Ctrl Pts',(-3.61028409669472,6.49977988812623,10.7415243813508));
#68297=CARTESIAN_POINT('Ctrl Pts',(-7.22431635935756,3.17136438593861,10.9533931409559));
#68298=CARTESIAN_POINT('Ctrl Pts',(-7.67860660833376,-3.55005395697526,
11.2182290904623));
#68299=CARTESIAN_POINT('Ctrl Pts',(-1.16458047228838,-8.37831567249255,
11.53603222987));
#68300=CARTESIAN_POINT('Ctrl Pts',(6.40509935429006,-5.51590302305541,11.8538353692777));
#68301=CARTESIAN_POINT('Ctrl Pts',(8.1128287823567,2.39466706089449,12.1716385086853));
#68302=CARTESIAN_POINT('Ctrl Pts',(2.37160135883004,8.12030723173545,12.489441648093));
#68303=CARTESIAN_POINT('Ctrl Pts',(-4.2080411500674,6.67388107534385,12.7542775975994));
#68304=CARTESIAN_POINT('Ctrl Pts',(-6.96346089814949,2.60605106873689,12.9661463572045));
#68305=CARTESIAN_POINT('Ctrl Pts',(-7.55575241306533,-2.27132217022394,
13.1780151168096));
#68306=CARTESIAN_POINT('Ctrl Pts',(-3.5424084439077,-7.68213674439024,13.442851066316));
#68307=CARTESIAN_POINT('Ctrl Pts',(4.54725929875602,-7.13266107804405,13.7606542057237));
#68308=CARTESIAN_POINT('Ctrl Pts',(8.45272122443086,-0.044584752292944,
14.0784573451314));
#68309=CARTESIAN_POINT('Ctrl Pts',(4.62224810690034,7.08429556290701,14.3962604845391));
#68310=CARTESIAN_POINT('Ctrl Pts',(-3.46117314465833,7.71907785980134,14.7140636239467));
#68311=CARTESIAN_POINT('Ctrl Pts',(-7.53137202013759,2.35090076838269,14.9788995734532));
#68312=CARTESIAN_POINT('Ctrl Pts',(-6.99056444882148,-2.53244911889549,
15.1907683330582));
#68313=CARTESIAN_POINT('Ctrl Pts',(-4.2782092022636,-6.62911947019817,15.4026370926634));
#68314=CARTESIAN_POINT('Ctrl Pts',(2.28580898234256,-8.14487322425717,15.6674730421697));
#68315=CARTESIAN_POINT('Ctrl Pts',(8.08711623839152,-2.48011534633209,15.9852761815774));
#68316=CARTESIAN_POINT('Ctrl Pts',(6.46292974909255,5.44802927271645,16.3030793209851));
#68317=CARTESIAN_POINT('Ctrl Pts',(-1.07613354736694,8.3901345503275,16.6208824603928));
#68318=CARTESIAN_POINT('Ctrl Pts',(-7.64073014880849,3.63085738305271,16.9386855998004));
#68319=CARTESIAN_POINT('Ctrl Pts',(-7.25736883688716,-3.09497923965129,
17.2035215493068));
#68320=CARTESIAN_POINT('Ctrl Pts',(-3.67864883055087,-6.461333657567,17.415390308912));
#68321=CARTESIAN_POINT('Ctrl Pts',(1.04280598275233,-7.82054055745697,17.6272590685171));
#68322=CARTESIAN_POINT('Ctrl Pts',(7.02221757620737,-4.7172389016652,17.8920950180235));
#68323=CARTESIAN_POINT('Ctrl Pts',(7.76418980207104,3.35704898709919,18.2098981574311));
#68324=CARTESIAN_POINT('Ctrl Pts',(1.38614201218807,8.3384107730507,18.5277012968388));
#68325=CARTESIAN_POINT('Ctrl Pts',(-6.26050369808442,5.68845450281879,18.8455044362465));
#68326=CARTESIAN_POINT('Ctrl Pts',(-8.17071856398859,-2.19162968839898,
19.1633075756542));
#68327=CARTESIAN_POINT('Ctrl Pts',(-3.51690828243854,-7.06255301299811,
19.4281435251605));
#68328=CARTESIAN_POINT('Ctrl Pts',(1.39036080365274,-7.30398430232345,19.6400122847657));
#68329=CARTESIAN_POINT('Ctrl Pts',(5.86572846132239,-5.27650722983735,19.8518810443708));
#68330=CARTESIAN_POINT('Ctrl Pts',(8.40448799323367,0.96356842754967,20.1167169938771));
#68331=CARTESIAN_POINT('Ctrl Pts',(3.73272469620222,7.59073036846454,20.4345201332849));
#68332=CARTESIAN_POINT('Ctrl Pts',(-4.35273170982645,7.24597892353766,20.7523232726925));
#68333=CARTESIAN_POINT('Ctrl Pts',(-8.45456569726709,0.269703642841959,
21.0701264121002));
#68334=CARTESIAN_POINT('Ctrl Pts',(-4.7979912386976,-6.96729234468889,21.3879295515078));
#68335=CARTESIAN_POINT('Ctrl Pts',(1.90339146903726,-7.65672252625688,21.6527655010143));
#68336=CARTESIAN_POINT('Ctrl Pts',(5.79526936145095,-4.65791185845644,21.8646342606193));
#68337=CARTESIAN_POINT('Ctrl Pts',(7.88690582824129,-0.212168293925783,
22.0765030202245));
#68338=CARTESIAN_POINT('Ctrl Pts',(5.7723835024817,6.18413059720254,22.3413389697309));
#68339=CARTESIAN_POINT('Ctrl Pts',(-2.08166357763857,8.19872538471076,22.6591421091385));
#68340=CARTESIAN_POINT('Ctrl Pts',(-8.0125380371007,2.69253005593165,22.9769452485462));
#68341=CARTESIAN_POINT('Ctrl Pts',(-6.61033334483714,-5.27787023850547,
23.2947483879539));
#68342=CARTESIAN_POINT('Ctrl Pts',(0.866480170453653,-8.415051672877,23.6125515273616));
#68343=CARTESIAN_POINT('Ctrl Pts',(6.41454280372272,-4.59368474622524,23.8773874768679));
#68344=CARTESIAN_POINT('Ctrl Pts',(7.43208735535594,0.212996233017501,24.0892562364731));
#68345=CARTESIAN_POINT('Ctrl Pts',(6.14092963596756,4.95351210098338,24.3011249960782));
#68346=CARTESIAN_POINT('Ctrl Pts',(0.383119799997728,8.45086396540785,24.5659609455846));
#68347=CARTESIAN_POINT('Ctrl Pts',(-6.90175237252995,4.89062729848073,24.8837640849922));
#68348=CARTESIAN_POINT('Ctrl Pts',(-7.84518301086339,-3.14699657199386,
25.2015672244));
#68349=CARTESIAN_POINT('Ctrl Pts',(-1.60869790813515,-8.30448747513831,
25.5193703638076));
#68350=CARTESIAN_POINT('Ctrl Pts',(6.11708029355421,-5.84339038788187,25.8371735032153));
#68351=CARTESIAN_POINT('Ctrl Pts',(7.86180973559087,0.663510821209555,26.1020094527216));
#68352=CARTESIAN_POINT('Ctrl Pts',(5.5189942760609,4.98216740322208,26.3138782123268));
#68353=CARTESIAN_POINT('Ctrl Pts',(1.46175943343325,7.7531644047616,26.5257469719319));
#68354=CARTESIAN_POINT('Ctrl Pts',(-5.18913976291492,6.68107110154611,26.7905829214383));
#68355=CARTESIAN_POINT('Ctrl Pts',(-8.42524278257166,-0.753462168321561,
27.108386060846));
#68356=CARTESIAN_POINT('Ctrl Pts',(-3.93060318626917,-7.48337106457854,
27.4261892002536));
#68357=CARTESIAN_POINT('Ctrl Pts',(4.16132657520632,-7.36449470899731,27.7439923396613));
#68358=CARTESIAN_POINT('Ctrl Pts',(8.44587796312302,-0.480653695514949,
28.061795479069));
#68359=CARTESIAN_POINT('Ctrl Pts',(5.55391017097628,5.60378271716701,28.3266314285754));
#68360=CARTESIAN_POINT('Ctrl Pts',(0.96977248127154,7.37162337531496,28.5385001881804));
#68361=CARTESIAN_POINT('Ctrl Pts',(-3.91561515650766,6.84954428225856,28.7503689477857));
#68362=CARTESIAN_POINT('Ctrl Pts',(-8.28282448891055,1.72008750617031,29.015204897292));
#68363=CARTESIAN_POINT('Ctrl Pts',(-5.92444483078517,-6.03766301074766,
29.3330080366997));
#68364=CARTESIAN_POINT('Ctrl Pts',(1.86141578941846,-8.2453389958803,29.6508111761073));
#68365=CARTESIAN_POINT('Ctrl Pts',(7.9437076708687,-2.90687626571029,29.968614315515));
#68366=CARTESIAN_POINT('Ctrl Pts',(6.74053094754093,5.11166558845771,30.2864174549227));
#68367=CARTESIAN_POINT('Ctrl Pts',(0.593204433234717,7.86742698910412,30.5512534044291));
#68368=CARTESIAN_POINT('Ctrl Pts',(-4.04265781809357,6.24004868720817,30.7631221640342));
#68369=CARTESIAN_POINT('Ctrl Pts',(-7.42270957644242,2.67426279043094,30.9749909236393));
#68370=CARTESIAN_POINT('Ctrl Pts',(-7.42024646331645,-4.06248999587925,
31.2398268731457));
#68371=CARTESIAN_POINT('Ctrl Pts',(-0.593856094554934,-8.43799479280045,
31.5576300125534));
#68372=CARTESIAN_POINT('Ctrl Pts',(6.76433588793489,-5.0689489929646,31.875433151961));
#68373=CARTESIAN_POINT('Ctrl Pts',(7.93180400173229,2.93920167094248,32.1932362913687));
#68374=CARTESIAN_POINT('Ctrl Pts',(1.81559240863278,8.2624153096231,32.5110394307764));
#68375=CARTESIAN_POINT('Ctrl Pts',(-4.6508433705407,6.37322170265487,32.7758753802828));
#68376=CARTESIAN_POINT('Ctrl Pts',(-7.1241264552189,2.12793611346102,32.9877441398879));
#68377=CARTESIAN_POINT('Ctrl Pts',(-7.38437218715985,-2.77837116490822,
33.199612899493));
#68378=CARTESIAN_POINT('Ctrl Pts',(-3.01341312605451,-7.90463306388738,
33.4644488489995));
#68379=CARTESIAN_POINT('Ctrl Pts',(5.02038597150706,-6.80794725901008,33.7822519884071));
#68380=CARTESIAN_POINT('Ctrl Pts',(8.43629411486896,0.528607137209164,34.1000551278148));
#68381=CARTESIAN_POINT('Ctrl Pts',(4.1313013145946,7.38137999512265,34.4178582672224));
#68382=CARTESIAN_POINT('Ctrl Pts',(-3.97655762654219,7.46665065379174,34.7356614066301));
#68383=CARTESIAN_POINT('Ctrl Pts',(-7.67343176575536,1.83486889580421,35.0004973561365));
#68384=CARTESIAN_POINT('Ctrl Pts',(-6.80278048844522,-3.0005778575052,35.2123661157416));
#68385=CARTESIAN_POINT('Ctrl Pts',(-3.81891471135974,-6.90392564819853,
35.4242348753467));
#68386=CARTESIAN_POINT('Ctrl Pts',(2.83276667106822,-7.9711552193057,35.6890708248531));
#68387=CARTESIAN_POINT('Ctrl Pts',(8.23665787120028,-1.92610703159567,36.0068739642608));
#68388=CARTESIAN_POINT('Ctrl Pts',(6.07868534894961,5.87367587857433,36.3246771036684));
#68389=CARTESIAN_POINT('Ctrl Pts',(-1.64250329731608,8.29786744306471,36.6424802430762));
#68390=CARTESIAN_POINT('Ctrl Pts',(-7.86931852960366,3.10446588362884,36.9602833824838));
#68391=CARTESIAN_POINT('Ctrl Pts',(-7.03083175665605,-3.57990275539581,
37.2251193319902));
#68392=CARTESIAN_POINT('Ctrl Pts',(-3.23210971831374,-6.69587609067724,
37.4369880915954));
#68393=CARTESIAN_POINT('Ctrl Pts',(1.57063429798398,-7.73184368895865,37.6488568512004));
#68394=CARTESIAN_POINT('Ctrl Pts',(7.32588516890857,-4.23028238241191,37.9136928007069));
#68395=CARTESIAN_POINT('Ctrl Pts',(7.51871834614993,3.87573162327282,38.2314959401145));
#68396=CARTESIAN_POINT('Ctrl Pts',(0.817613343300754,8.4132034516549,38.5492990795222));
#68397=CARTESIAN_POINT('Ctrl Pts',(-6.63177183421585,5.25090692388172,38.8671022189298));
#68398=CARTESIAN_POINT('Ctrl Pts',(-8.00332638643711,-2.74055638422911,
39.1849053583376));
#68399=CARTESIAN_POINT('Ctrl Pts',(-3.02997903692706,-7.28474611529298,
39.4497413078438));
#68400=CARTESIAN_POINT('Ctrl Pts',(1.88236719001822,-7.19291203997827,39.6616100674491));
#68401=CARTESIAN_POINT('Ctrl Pts',(6.20997521372375,-4.86667307032534,39.8734788270541));
#68402=CARTESIAN_POINT('Ctrl Pts',(8.31981970420338,1.53117034732538,40.1383147765605));
#68403=CARTESIAN_POINT('Ctrl Pts',(3.20948875182505,7.82634034119881,40.4561179159682));
#68404=CARTESIAN_POINT('Ctrl Pts',(-4.83398887575954,6.93419320808945,40.7739210553758));
#68405=CARTESIAN_POINT('Ctrl Pts',(-8.4533972658104,-0.304131305124825,
41.0917241947836));
#68406=CARTESIAN_POINT('Ctrl Pts',(-4.31457280315205,-7.27656128052804,
41.4095273341912));
#68407=CARTESIAN_POINT('Ctrl Pts',(2.41813279325872,-7.51005544071813,41.6743632836976));
#68408=CARTESIAN_POINT('Ctrl Pts',(6.09773785643282,-4.25427818638455,41.8862320433027));
#68409=CARTESIAN_POINT('Ctrl Pts',(7.88314273544256,0.323047273835714,42.0981008029079));
#68410=CARTESIAN_POINT('Ctrl Pts',(5.33982085001841,6.56126480434131,42.3629367524142));
#68411=CARTESIAN_POINT('Ctrl Pts',(-2.63274215352489,8.03872439740416,42.6807398918219));
#68412=CARTESIAN_POINT('Ctrl Pts',(-8.17665286289524,2.14308932566695,42.9985430312296));
#68413=CARTESIAN_POINT('Ctrl Pts',(-6.23728644307629,-5.71390225777308,
43.3163461706372));
#68414=CARTESIAN_POINT('Ctrl Pts',(1.43502170377997,-8.33694160065068,43.634149310045));
#68415=CARTESIAN_POINT('Ctrl Pts',(6.71123177593405,-4.14821250398127,43.8989852595513));
#68416=CARTESIAN_POINT('Ctrl Pts',(7.40054491816626,0.716397073643458,44.1108540191565));
#68417=CARTESIAN_POINT('Ctrl Pts',(5.79095412635695,5.35846519396396,44.3227227787615));
#68418=CARTESIAN_POINT('Ctrl Pts',(-0.190725146312963,8.4573935974119,44.587558728268));
#68419=CARTESIAN_POINT('Ctrl Pts',(-7.21745278538906,4.41143927477727,44.9053618676755));
#68420=CARTESIAN_POINT('Ctrl Pts',(-7.61376661200979,-3.67165383389088,
45.2231650070833));
#68421=CARTESIAN_POINT('Ctrl Pts',(-1.04195711115155,-8.39444736494835,
45.540968146491));
#68422=CARTESIAN_POINT('Ctrl Pts',(6.49918300830777,-5.41521031609143,45.8587712858986));
#68423=CARTESIAN_POINT('Ctrl Pts',(7.79873388426272,1.19500992922489,46.123607235405));
#68424=CARTESIAN_POINT('Ctrl Pts',(5.16850704380232,5.34488772483455,46.3354759950102));
#68425=CARTESIAN_POINT('Ctrl Pts',(0.932736110642546,7.83443056491003,46.5473447546152));
#68426=CARTESIAN_POINT('Ctrl Pts',(-5.6301719296693,6.31387730205009,46.8121807041218));
#68427=CARTESIAN_POINT('Ctrl Pts',(-8.35477181135561,-1.32295470993732,
47.1299838435293));
#68428=CARTESIAN_POINT('Ctrl Pts',(-3.41419081316633,-7.732644113715,47.447786982937));
#68429=CARTESIAN_POINT('Ctrl Pts',(4.65105946660589,-7.06541343606045,47.7655901223447));
#68430=CARTESIAN_POINT('Ctrl Pts',(8.4590318061587,0.0930776309034,48.0833932617524));
#68431=CARTESIAN_POINT('Ctrl Pts',(5.16119746048464,5.96743996219319,48.3482292112587));
#68432=CARTESIAN_POINT('Ctrl Pts',(0.467749480146434,7.4204110584754,48.5600979708639));
#68433=CARTESIAN_POINT('Ctrl Pts',(-4.37100011405199,6.56830700648585,48.7719667304689));
#68434=CARTESIAN_POINT('Ctrl Pts',(-8.38038637202662,1.15455913600378,49.0368026799754));
#68435=CARTESIAN_POINT('Ctrl Pts',(-5.50146269355898,-6.42544390806941,
49.354605819383));
#68436=CARTESIAN_POINT('Ctrl Pts',(2.41616153527492,-8.10016341400214,49.6724089587907));
#68437=CARTESIAN_POINT('Ctrl Pts',(8.12251341825707,-2.36160897580472,49.9902120981984));
#68438=CARTESIAN_POINT('Ctrl Pts',(6.37845303077979,5.55690736625286,50.3080152376061));
#68439=CARTESIAN_POINT('Ctrl Pts',(0.0584327448535862,7.88954273344295,
50.5728511871124));
#68440=CARTESIAN_POINT('Ctrl Pts',(-4.45642702083661,5.95160046213443,50.7847199467176));
#68441=CARTESIAN_POINT('Ctrl Pts',(-7.58694310329044,2.16485410037873,50.9965887063226));
#68442=CARTESIAN_POINT('Ctrl Pts',(-7.12773796343645,-4.55623024742675,
51.2614246558292));
#68443=CARTESIAN_POINT('Ctrl Pts',(-0.0203987606110949,-8.45884182822524,
51.5792277952367));
#68444=CARTESIAN_POINT('Ctrl Pts',(7.09244260083074,-4.59866739958459,51.8970309346444));
#68445=CARTESIAN_POINT('Ctrl Pts',(7.71427665221152,3.47020992412735,52.2148340740521));
#68446=CARTESIAN_POINT('Ctrl Pts',(1.25122800903597,8.3664993284159,52.5326372134597));
#68447=CARTESIAN_POINT('Ctrl Pts',(-5.07224217124685,6.0432324367609,52.7974731629662));
#68448=CARTESIAN_POINT('Ctrl Pts',(-7.25200641689262,1.64002828703338,53.0093419225713));
#68449=CARTESIAN_POINT('Ctrl Pts',(-7.17900870165025,-3.27263395296864,
53.2212106821764));
#68450=CARTESIAN_POINT('Ctrl Pts',(-2.470549926415,-8.09075185653782,53.4860466316827));
#68451=CARTESIAN_POINT('Ctrl Pts',(5.47040857048482,-6.45190291746039,53.8038497710905));
#68452=CARTESIAN_POINT('Ctrl Pts',(8.38104274703086,1.09936634954972,54.1216529104981));
#68453=CARTESIAN_POINT('Ctrl Pts',(3.62134206171429,7.64449493795545,54.4394560499058));
#68454=CARTESIAN_POINT('Ctrl Pts',(-4.47364178624171,7.17986153845404,54.7572591893135));
#68455=CARTESIAN_POINT('Ctrl Pts',(-7.7801779847604,1.31039286244344,55.0220951388199));
#68456=CARTESIAN_POINT('Ctrl Pts',(-6.58368978329653,-3.45489778289289,
55.233963898425));
#68457=CARTESIAN_POINT('Ctrl Pts',(-3.34204537905406,-7.14695960621277,
55.4458326580302));
#68458=CARTESIAN_POINT('Ctrl Pts',(3.36668782226014,-7.76075354913583,55.7106686075364));
#68459=CARTESIAN_POINT('Ctrl Pts',(8.34829398196702,-1.36323467349575,56.0284717469442));
#68460=CARTESIAN_POINT('Ctrl Pts',(5.66646652701038,6.272291526735,56.3462748863518));
#68461=CARTESIAN_POINT('Ctrl Pts',(-2.20131416283494,8.16741312417033,56.6640780257595));
#68462=CARTESIAN_POINT('Ctrl Pts',(-8.06169190285053,2.5637874729575,56.9818811651672));
#68463=CARTESIAN_POINT('Ctrl Pts',(-6.77193842801764,-4.04835137502064,
57.2467171146735));
#68464=CARTESIAN_POINT('Ctrl Pts',(-2.77069627135412,-6.89960375853757,
57.4585858742787));
#68465=CARTESIAN_POINT('Ctrl Pts',(2.09123447360709,-7.60756447918061,57.6704546338838));
#68466=CARTESIAN_POINT('Ctrl Pts',(7.5958386622641,-3.72385788663226,57.9352905833903));
#68467=CARTESIAN_POINT('Ctrl Pts',(7.23864536270936,4.37657794370142,58.2530937227978));
#68468=CARTESIAN_POINT('Ctrl Pts',(0.245321975866281,8.44927813639946,58.5708968622056));
#68469=CARTESIAN_POINT('Ctrl Pts',(-6.97252021617379,4.78919440192351,58.8887000016132));
#68470=CARTESIAN_POINT('Ctrl Pts',(-7.79910249030586,-3.27687089899559,
59.2065031410209));
#68471=CARTESIAN_POINT('Ctrl Pts',(-2.52910567245795,-7.473414442277,59.4713390905273));
#68472=CARTESIAN_POINT('Ctrl Pts',(2.36571082601458,-7.04873762744781,59.6832078501324));
#68473=CARTESIAN_POINT('Ctrl Pts',(6.52564334163617,-4.43444223169647,59.8950766097376));
#68474=CARTESIAN_POINT('Ctrl Pts',(8.19686317810968,2.09172574261759,60.1599125592438));
#68475=CARTESIAN_POINT('Ctrl Pts',(2.67148257557379,8.0259330942124,60.4777156986516));
#68476=CARTESIAN_POINT('Ctrl Pts',(-5.29299977691561,6.59049597979186,60.7955188380592));
#68477=CARTESIAN_POINT('Ctrl Pts',(-8.41332586649955,-0.876566625224416,
61.113321977467));
#68478=CARTESIAN_POINT('Ctrl Pts',(-3.81129848224015,-7.55234310808594,
61.4311251168746));
#68479=CARTESIAN_POINT('Ctrl Pts',(2.92174574632196,-7.32882669479521,61.6959610663809));
#68480=CARTESIAN_POINT('Ctrl Pts',(6.37214424900164,-3.83106610786561,61.9078298259862));
#68481=CARTESIAN_POINT('Ctrl Pts',(7.84310101539102,0.856776161471738,62.1196985855912));
#68482=CARTESIAN_POINT('Ctrl Pts',(4.8826840680845,6.90820373427514,62.3845345350977));
#68483=CARTESIAN_POINT('Ctrl Pts',(-3.17170471496819,7.84172878805536,62.7023376745052));
#68484=CARTESIAN_POINT('Ctrl Pts',(-8.3031383127742,1.58378598839051,63.020140813913));
#68485=CARTESIAN_POINT('Ctrl Pts',(-5.83553522914796,-6.12363860574255,
63.3379439533206));
#68486=CARTESIAN_POINT('Ctrl Pts',(1.99695919361291,-8.2204644955151,63.6557470927283));
#68487=CARTESIAN_POINT('Ctrl Pts',(6.97703531524421,-3.68364997500153,63.9205830422348));
#68488=CARTESIAN_POINT('Ctrl Pts',(7.3349447936348,1.21650101818743,64.1324518018397));
#68489=CARTESIAN_POINT('Ctrl Pts',(5.41432834879617,5.73875835524684,64.344320561445));
#68490=CARTESIAN_POINT('Ctrl Pts',(-0.763692365716531,8.42500187023871,
64.6091565109513));
#68491=CARTESIAN_POINT('Ctrl Pts',(-7.49993811029349,3.91194958123631,64.926959650359));
#68492=CARTESIAN_POINT('Ctrl Pts',(-7.34731126864177,-4.17941395649796,
65.2447627897667));
#68493=CARTESIAN_POINT('Ctrl Pts',(-0.470421174093057,-8.44577557737201,
65.5625659291743));
#68494=CARTESIAN_POINT('Ctrl Pts',(6.85137614946615,-4.96210916864047,65.8803690685821));
#68495=CARTESIAN_POINT('Ctrl Pts',(7.69976785954471,1.72100954024463,66.1452050180884));
#68496=CARTESIAN_POINT('Ctrl Pts',(4.79423407699781,5.68301059895882,66.3570737776935));
#68497=CARTESIAN_POINT('Ctrl Pts',(0.399420288423597,7.87964227371272,66.5689425372987));
#68498=CARTESIAN_POINT('Ctrl Pts',(-6.04529375638949,5.91762671532605,66.833778486805));
#68499=CARTESIAN_POINT('Ctrl Pts',(-8.24585175168749,-1.8863589461156,67.1515816262127));
#68500=CARTESIAN_POINT('Ctrl Pts',(-2.88206615879987,-7.94633113797258,
67.4693847656204));
#68501=CARTESIAN_POINT('Ctrl Pts',(5.11938794374809,-6.73381676806031,67.787187905028));
#68502=CARTESIAN_POINT('Ctrl Pts',(8.43325675090628,0.666380609302265,68.1049910444358));
#68503=CARTESIAN_POINT('Ctrl Pts',(4.74473265450711,6.30363474237736,68.3698269939421));
#68504=CARTESIAN_POINT('Ctrl Pts',(-0.0364261280579175,7.4350496293269,
68.5816957535472));
#68505=CARTESIAN_POINT('Ctrl Pts',(-4.80626950490606,6.25684204486051,68.7935645131524));
#68506=CARTESIAN_POINT('Ctrl Pts',(-8.43938128704969,0.583717425620363,
69.0584004626587));
#68507=CARTESIAN_POINT('Ctrl Pts',(-5.05316254300341,-6.7836545831746,69.3762036020665));
#68508=CARTESIAN_POINT('Ctrl Pts',(2.95978798216355,-7.91771046410669,69.694006741474));
#68509=CARTESIAN_POINT('Ctrl Pts',(8.26393894154964,-1.80547344113602,70.0118098808819));
#68510=CARTESIAN_POINT('Ctrl Pts',(5.98702114732562,5.97657597305592,70.3296130202893));
#68511=CARTESIAN_POINT('Ctrl Pts',(-0.476607856380058,7.87535039433149,
70.5944489697959));
#68512=CARTESIAN_POINT('Ctrl Pts',(-4.84968751467229,5.63576267054211,70.8063177294009));
#68513=CARTESIAN_POINT('Ctrl Pts',(-7.71626113646769,1.64548263069972,71.0181864890061));
#68514=CARTESIAN_POINT('Ctrl Pts',(-6.80242723150402,-5.02900247240576,
71.2830224385124));
#68515=CARTESIAN_POINT('Ctrl Pts',(0.553152422106158,-8.44076087529441,
71.6008255779202));
#68516=CARTESIAN_POINT('Ctrl Pts',(7.38790957909878,-4.10722243773945,71.9186287173277));
#68517=CARTESIAN_POINT('Ctrl Pts',(7.46124771108228,3.98524796982142,72.2364318567355));
#68518=CARTESIAN_POINT('Ctrl Pts',(0.681105581927244,8.43208053298718,72.5542349961431));
#68519=CARTESIAN_POINT('Ctrl Pts',(-5.4702985817129,5.68543147735568,72.8190709456496));
#68520=CARTESIAN_POINT('Ctrl Pts',(-7.34651183457599,1.14457353746562,73.0309397052545));
#68521=CARTESIAN_POINT('Ctrl Pts',(-6.94060811730116,-3.75183730228112,
73.2428084648599));
#68522=CARTESIAN_POINT('Ctrl Pts',(-1.91631486239838,-8.23963364106499,
73.507644414366));
#68523=CARTESIAN_POINT('Ctrl Pts',(5.89525226469161,-6.06617154303566,73.8254475537739));
#68524=CARTESIAN_POINT('Ctrl Pts',(8.28722834591438,1.66507528224125,74.1432506931814));
#68525=CARTESIAN_POINT('Ctrl Pts',(3.09470404059807,7.8724123713359,74.4610538325893));
#68526=CARTESIAN_POINT('Ctrl Pts',(-4.95011189218524,6.86006436447352,74.7788569719968));
#68527=CARTESIAN_POINT('Ctrl Pts',(-7.85116507114007,0.779826871913311,
75.0436929215033));
#68528=CARTESIAN_POINT('Ctrl Pts',(-6.33423966281534,-3.89323870918931,
75.2555616811083));
#68529=CARTESIAN_POINT('Ctrl Pts',(-2.84994413976273,-7.35729615265609,
75.4674304407135));
#68530=CARTESIAN_POINT('Ctrl Pts',(3.88543032268657,-7.5142261247853,75.7322663902198));
#68531=CARTESIAN_POINT('Ctrl Pts',(8.42098238217486,-0.794776998686755,
76.0500695296276));
#68532=CARTESIAN_POINT('Ctrl Pts',(5.22913513009899,6.64329840099667,76.3678726690352));
#68533=CARTESIAN_POINT('Ctrl Pts',(-2.7518091883857,7.99700948568447,76.6856758084429));
#68534=CARTESIAN_POINT('Ctrl Pts',(-8.21345806569579,2.01586733850936,77.0034789478505));
#68535=CARTESIAN_POINT('Ctrl Pts',(-6.14214966524969,-5.80958392169303,
77.3212820872583));
#68536=CARTESIAN_POINT('Ctrl Pts',(1.55454614605433,-8.31432505007639,77.6390852266658));
#68537=CARTESIAN_POINT('Ctrl Pts',(7.83537994160767,-3.18857087384152,77.9568883660737));
#68538=CARTESIAN_POINT('Ctrl Pts',(7.06879253230392,3.50487666158179,78.2217243155799));
#68539=CARTESIAN_POINT('Ctrl Pts',(3.30326759019129,6.66095511021538,78.4335930751852));
#68540=CARTESIAN_POINT('Ctrl Pts',(-1.48802546613442,7.74820644643544,78.6454618347901));
#68541=CARTESIAN_POINT('Ctrl Pts',(-7.28038169229118,4.30814730997263,78.9102977842966));
#68542=CARTESIAN_POINT('Ctrl Pts',(-7.55961163766212,-3.79530519602571,
79.2281009237043));
#68543=CARTESIAN_POINT('Ctrl Pts',(-0.90730672759395,-8.4040123664188,79.5459040631119));
#68544=CARTESIAN_POINT('Ctrl Pts',(6.57539537422739,-5.32133555853004,79.8637072025197));
#68545=CARTESIAN_POINT('Ctrl Pts',(8.03209799109985,2.65503805098697,80.1815103419273));
#68546=CARTESIAN_POINT('Ctrl Pts',(3.10750385441467,7.25201654545354,80.4463462914337));
#68547=CARTESIAN_POINT('Ctrl Pts',(-1.80554424357141,7.21257892176842,80.6582150510388));
#68548=CARTESIAN_POINT('Ctrl Pts',(-6.15771582622757,4.93262946715277,80.8700838106439));
#68549=CARTESIAN_POINT('Ctrl Pts',(-8.33567749448872,-1.44234795953961,
81.1349197601503));
#68550=CARTESIAN_POINT('Ctrl Pts',(-3.29277836034727,-7.79166410060939,
81.4527228995579));
#68551=CARTESIAN_POINT('Ctrl Pts',(4.75975683582896,-6.98535603715296,81.7705260389657));
#68552=CARTESIAN_POINT('Ctrl Pts',(8.45616021047951,0.213953851766904,82.0883291783733));
#68553=CARTESIAN_POINT('Ctrl Pts',(4.39193595102736,7.23013006172392,82.406132317781));
#68554=CARTESIAN_POINT('Ctrl Pts',(-2.337896323999,7.53541901902798,82.6709682672874));
#68555=CARTESIAN_POINT('Ctrl Pts',(-6.05201678514127,4.31907197219638,82.8828370268925));
#68556=CARTESIAN_POINT('Ctrl Pts',(-7.88613982887975,-0.238950793295768,
83.0947057864976));
#68557=CARTESIAN_POINT('Ctrl Pts',(-5.40949666956307,-6.50393944945827,
83.359541736004));
#68558=CARTESIAN_POINT('Ctrl Pts',(2.54685493909067,-8.06634682464978,83.6773448754118));
#68559=CARTESIAN_POINT('Ctrl Pts',(8.15333054530708,-2.230175982237,83.9951480148192));
#68560=CARTESIAN_POINT('Ctrl Pts',(6.29787362155546,5.6470531285578,84.3129511542271));
#68561=CARTESIAN_POINT('Ctrl Pts',(-1.34602196100505,8.35177271132716,84.6307542936346));
#68562=CARTESIAN_POINT('Ctrl Pts',(-6.66660705557152,4.21955558023922,84.8955902431412));
#68563=CARTESIAN_POINT('Ctrl Pts',(-7.40776475847419,-0.637425396785901,
85.1074590027462));
#68564=CARTESIAN_POINT('Ctrl Pts',(-5.84777575731517,-5.29639666379029,
85.3193277623513));
#68565=CARTESIAN_POINT('Ctrl Pts',(0.100511489746323,-8.45894674197618,
85.5841637118577));
#68566=CARTESIAN_POINT('Ctrl Pts',(7.16999181195573,-4.4881665077057,85.9019668512654));
#68567=CARTESIAN_POINT('Ctrl Pts',(7.65249378215863,3.59023993794783,86.219769990673));
#68568=CARTESIAN_POINT('Ctrl Pts',(1.13142929779594,8.38285684766757,86.5375731300808));
#68569=CARTESIAN_POINT('Ctrl Pts',(-6.44105711244674,5.48421970905446,86.8553762694884));
#68570=CARTESIAN_POINT('Ctrl Pts',(-7.81103574848863,-1.11176412260787,
87.1202122189948));
#68571=CARTESIAN_POINT('Ctrl Pts',(-5.22521926747735,-5.28945871140975,
87.3320809786));
#68572=CARTESIAN_POINT('Ctrl Pts',(-1.01624161886705,-7.82403680337547,
87.543949738205));
#68573=CARTESIAN_POINT('Ctrl Pts',(5.56251067857787,-6.37356709336982,87.8087856877114));
#68574=CARTESIAN_POINT('Ctrl Pts',(8.36840665116155,1.23377117212372,88.1265888271191));
#68575=CARTESIAN_POINT('Ctrl Pts',(3.49646957042679,7.69579004658781,88.4443919665267));
#68576=CARTESIAN_POINT('Ctrl Pts',(-4.57543835510379,7.11461770181735,88.7621951059345));
#68577=CARTESIAN_POINT('Ctrl Pts',(-8.45954339245076,-0.002852056000995,
89.0799982453421));
#68578=CARTESIAN_POINT('Ctrl Pts',(-5.22454996591466,-5.91205349960188,
89.3448341948485));
#68579=CARTESIAN_POINT('Ctrl Pts',(-0.54686568779491,-7.41500018694766,
89.5567029544537));
#68580=CARTESIAN_POINT('Ctrl Pts',(4.30069684861065,-6.61455255817383,89.7685717140586));
#68581=CARTESIAN_POINT('Ctrl Pts',(8.36759569126859,-1.24387494968049,90.0334076635652));
#68582=CARTESIAN_POINT('Ctrl Pts',(5.56968071207069,6.36640227679301,90.3512108029727));
#68583=CARTESIAN_POINT('Ctrl Pts',(-2.32963135753805,8.12547239463998,90.6690139423806));
#68584=CARTESIAN_POINT('Ctrl Pts',(-8.09686354683089,2.44810577556786,90.9868170817879));
#68585=CARTESIAN_POINT('Ctrl Pts',(-6.43735774178527,-5.48856154627573,
91.3046202211961));
#68586=CARTESIAN_POINT('Ctrl Pts',(-0.142575784227132,-7.88847076905561,
91.5694561707021));
#68587=CARTESIAN_POINT('Ctrl Pts',(4.39269641485442,-5.99879221675887,91.7813249303074));
#68588=CARTESIAN_POINT('Ctrl Pts',(7.5634221946081,-2.24564993589899,91.9931936899123));
#68589=CARTESIAN_POINT('Ctrl Pts',(7.17592727787235,4.47994980392269,92.258029639419));
#68590=CARTESIAN_POINT('Ctrl Pts',(0.11061585490748,8.45814313646977,92.5758327788264));
#68591=CARTESIAN_POINT('Ctrl Pts',(-7.04299184568019,4.67405068005932,92.8936359182344));
#68592=CARTESIAN_POINT('Ctrl Pts',(-7.75084959410668,-3.38773549054587,
93.2114390576417));
#68593=CARTESIAN_POINT('Ctrl Pts',(-1.34039021126954,-8.35267841021741,
93.5292421970496));
#68594=CARTESIAN_POINT('Ctrl Pts',(5.00749923252853,-6.0969869906963,93.7940781465558));
#68595=CARTESIAN_POINT('Ctrl Pts',(7.234102118271,-1.71728168782766,94.0059469061612));
#68596=CARTESIAN_POINT('Ctrl Pts',(7.21350483120897,3.19587968775712,94.217815665766));
#68597=CARTESIAN_POINT('Ctrl Pts',(2.55670177503496,8.06394187581435,94.4826516152727));
#68598=CARTESIAN_POINT('Ctrl Pts',(-5.40128428653493,6.50988089295023,94.8004547546802));
#68599=CARTESIAN_POINT('Ctrl Pts',(-8.39229139831418,-1.00991533499733,
95.1182578940879));
#68600=CARTESIAN_POINT('Ctrl Pts',(-3.70266887648321,-7.60543650131208,
95.4360610334955));
#68601=CARTESIAN_POINT('Ctrl Pts',(4.39681011332992,-7.22716703628046,95.7538641729033));
#68602=CARTESIAN_POINT('Ctrl Pts',(7.76575938965619,-1.39329825610326,96.0187001224095));
#68603=CARTESIAN_POINT('Ctrl Pts',(6.62016371895673,3.38448255825473,96.2305688820149));
#68604=CARTESIAN_POINT('Ctrl Pts',(3.41808158870619,7.11090832323413,96.4424376416197));
#68605=CARTESIAN_POINT('Ctrl Pts',(-3.28372357491219,7.79621972667172,96.7072735911263));
#68606=CARTESIAN_POINT('Ctrl Pts',(-8.33327948586795,1.45219633479086,97.0250767305339));
#68607=CARTESIAN_POINT('Ctrl Pts',(-5.73304170496459,-6.21149874887032,
97.3428798699416));
#68608=CARTESIAN_POINT('Ctrl Pts',(2.11407894975325,-8.19042681296763,97.6606830093493));
#68609=CARTESIAN_POINT('Ctrl Pts',(8.03388914470774,-2.64962407777525,97.978486148757));
#68610=CARTESIAN_POINT('Ctrl Pts',(6.81473116910066,3.97589461899854,98.2433220982633));
#68611=CARTESIAN_POINT('Ctrl Pts',(2.84412679083728,6.86966030095835,98.4551908578685));
#68612=CARTESIAN_POINT('Ctrl Pts',(-2.00997661900668,7.62943595028749,98.6670596174735));
#68613=CARTESIAN_POINT('Ctrl Pts',(-7.55568960481281,3.80465992418547,98.93189556698));
#68614=CARTESIAN_POINT('Ctrl Pts',(-7.28491227710381,-4.29912482945887,
99.2496987063876));
#68615=CARTESIAN_POINT('Ctrl Pts',(-0.335424274736072,-8.44618105737727,
99.5675018457952));
#68616=CARTESIAN_POINT('Ctrl Pts',(6.92104420556015,-4.86328780652038,99.8853049852031));
#68617=CARTESIAN_POINT('Ctrl Pts',(7.83360853914484,3.19350274751976,100.20310812461));
#68618=CARTESIAN_POINT('Ctrl Pts',(2.60866994349881,7.44601504526949,100.467944074117));
#68619=CARTESIAN_POINT('Ctrl Pts',(-2.29039755886778,7.0735683268951,100.679812833722));
#68620=CARTESIAN_POINT('Ctrl Pts',(-6.47797637805987,4.50378962361612,100.891681593327));
#68621=CARTESIAN_POINT('Ctrl Pts',(-8.21870637035112,-2.00418266156781,
101.156517542833));
#68622=CARTESIAN_POINT('Ctrl Pts',(-2.75693166724786,-7.9969837417925,101.474320682241));
#68623=CARTESIAN_POINT('Ctrl Pts',(5.22240741161874,-6.64657390880071,101.792123821649));
#68624=CARTESIAN_POINT('Ctrl Pts',(8.42219639853767,0.786783965791493,102.109926961056));
#68625=CARTESIAN_POINT('Ctrl Pts',(3.89163164200336,7.51126392199993,102.427730100465));
#68626=CARTESIAN_POINT('Ctrl Pts',(-2.8434135469081,7.35957188495038,102.69256604997));
#68627=CARTESIAN_POINT('Ctrl Pts',(-6.33092135832433,3.89881066578444,102.904434809576));
#68628=CARTESIAN_POINT('Ctrl Pts',(-7.85179290474972,-0.773076393000939,
103.116303569181));
#68629=CARTESIAN_POINT('Ctrl Pts',(-4.95608618404943,-6.85573426259024,
103.381139518688));
#68630=CARTESIAN_POINT('Ctrl Pts',(3.08788791202162,-7.87511075650104,103.698942658095));
#68631=CARTESIAN_POINT('Ctrl Pts',(8.28577408258241,-1.6722534946851,104.016745797503));
#68632=CARTESIAN_POINT('Ctrl Pts',(5.90051532458819,6.06105107128024,104.33454893691));
#68633=CARTESIAN_POINT('Ctrl Pts',(-1.90916978157587,8.24129560737247,104.652352076318));
#68634=CARTESIAN_POINT('Ctrl Pts',(-6.93735029424958,3.75785441753258,104.917188025824));
#68635=CARTESIAN_POINT('Ctrl Pts',(-7.3475022519864,-1.13820055788763,105.12905678543));
#68636=CARTESIAN_POINT('Ctrl Pts',(-5.47522743990438,-5.68068511799518,
105.340925545035));
#68637=CARTESIAN_POINT('Ctrl Pts',(0.673791595344492,-8.43266787138114,
105.605761494541));
#68638=CARTESIAN_POINT('Ctrl Pts',(7.45778840496133,-3.99171808763995,105.923564633949));
#68639=CARTESIAN_POINT('Ctrl Pts',(7.39146913864016,4.10081307433183,106.241367773356));
#68640=CARTESIAN_POINT('Ctrl Pts',(0.560473312880324,8.44027788937762,106.559170912764));
#68641=CARTESIAN_POINT('Ctrl Pts',(-6.79806279716929,5.03490066920113,106.876974052172));
#68642=CARTESIAN_POINT('Ctrl Pts',(-7.71768543134127,-1.63878934319104,
107.141810001678));
#68643=CARTESIAN_POINT('Ctrl Pts',(-4.8545738574009,-5.63155418299077,107.353678761283));
#68644=CARTESIAN_POINT('Ctrl Pts',(-0.483438338969841,-7.87493405057514,
107.565547520888));
#68645=CARTESIAN_POINT('Ctrl Pts',(5.98183512670323,-5.98176655010195,107.830383470395));
#68646=CARTESIAN_POINT('Ctrl Pts',(8.26550180637324,1.79830505565891,108.148186609802));
#68647=CARTESIAN_POINT('Ctrl Pts',(2.96665427361026,7.91514032212636,108.46598974921));
#68648=CARTESIAN_POINT('Ctrl Pts',(-5.04727685731576,6.78803487837035,108.783792888618));
#68649=CARTESIAN_POINT('Ctrl Pts',(-8.43988439848631,-0.576397330985157,
109.101596028025));
#68650=CARTESIAN_POINT('Ctrl Pts',(-4.81169455230378,-6.25267098637243,
109.366431977532));
#68651=CARTESIAN_POINT('Ctrl Pts',(-0.0428748849056034,-7.4350152385295,
109.578300737137));
#68652=CARTESIAN_POINT('Ctrl Pts',(4.73926342898019,-6.30774770256575,109.790169496742));
#68653=CARTESIAN_POINT('Ctrl Pts',(8.43267559531305,-0.673694921452692,
110.055005446249));
#68654=CARTESIAN_POINT('Ctrl Pts',(5.12522657618584,6.72937394763629,110.372808585656));
#68655=CARTESIAN_POINT('Ctrl Pts',(-2.87517284554175,7.94882790141666,110.690611725064));
#68656=CARTESIAN_POINT('Ctrl Pts',(-8.24421252162756,1.89351025415944,111.008414864471));
#68657=CARTESIAN_POINT('Ctrl Pts',(-6.05042412027553,-5.91238111996912,
111.326218003879));
#68658=CARTESIAN_POINT('Ctrl Pts',(0.392585751409091,-7.87998574594424,
111.591053953385));
#68659=CARTESIAN_POINT('Ctrl Pts',(4.78930312953449,-5.68716672749729,111.802922712991));
#68660=CARTESIAN_POINT('Ctrl Pts',(7.69827225026102,-1.72768726607415,112.014791472596));
#68661=CARTESIAN_POINT('Ctrl Pts',(6.85567744454336,4.9561647792783,112.279627422102));
#68662=CARTESIAN_POINT('Ctrl Pts',(-0.463095576155875,8.44618041908367,
112.59743056151));
#68663=CARTESIAN_POINT('Ctrl Pts',(-7.34368350139931,4.18578505532193,112.915233700918));
#68664=CARTESIAN_POINT('Ctrl Pts',(-7.50332830829109,-3.90544305839496,
113.233036840325));
#68665=CARTESIAN_POINT('Ctrl Pts',(-0.770999481427355,-8.42433631466713,
113.550839979733));
#68666=CARTESIAN_POINT('Ctrl Pts',(5.40934881541923,-5.74345229993392,113.815675929239));
#68667=CARTESIAN_POINT('Ctrl Pts',(7.3338869057028,-1.22286250546905,114.027544688844));
#68668=CARTESIAN_POINT('Ctrl Pts',(6.98022769487296,3.67759707638322,114.239413448449));
#68669=CARTESIAN_POINT('Ctrl Pts',(2.00408844048741,8.21872934617535,114.504249397956));
#68670=CARTESIAN_POINT('Ctrl Pts',(-5.83022171247392,6.12869773832626,114.822052537364));
#68671=CARTESIAN_POINT('Ctrl Pts',(-8.3045088821496,-1.57658368771828,115.139855676771));
#68672=CARTESIAN_POINT('Ctrl Pts',(-3.17850502455827,-7.83897486877112,
115.457658816179));
#68673=CARTESIAN_POINT('Ctrl Pts',(4.87669041934326,-6.91243611882708,115.775461955587));
#68674=CARTESIAN_POINT('Ctrl Pts',(7.8423549427161,-0.863578532010263,116.040297905093));
#68675=CARTESIAN_POINT('Ctrl Pts',(6.37546471714856,3.82553780445514,116.252166664698));
#68676=CARTESIAN_POINT('Ctrl Pts',(2.92810128566636,7.32628976968374,116.464035424303));
#68677=CARTESIAN_POINT('Ctrl Pts',(-3.80474654392298,7.55564598690843,116.728871373809));
#68678=CARTESIAN_POINT('Ctrl Pts',(-8.41256241413094,0.883863571327154,
117.046674513217));
#68679=CARTESIAN_POINT('Ctrl Pts',(-5.29871403514028,-6.58590263152199,
117.364477652625));
#68680=CARTESIAN_POINT('Ctrl Pts',(2.66452029897814,-8.02824717860013,117.682280792032));
#68681=CARTESIAN_POINT('Ctrl Pts',(8.19504584213313,-2.09883448330634,118.00008393144));
#68682=CARTESIAN_POINT('Ctrl Pts',(6.52948708872176,4.42878056429865,118.264919880946));
#68683=CARTESIAN_POINT('Ctrl Pts',(2.37182364000149,7.04668308310025,118.476788640552));
#68684=CARTESIAN_POINT('Ctrl Pts',(-2.52262267500035,7.47560524426402,118.688657400157));
#68685=CARTESIAN_POINT('Ctrl Pts',(-7.79625737144515,3.28363419722211,118.953493349663));
#68686=CARTESIAN_POINT('Ctrl Pts',(-6.97667148852008,-4.78314500361829,
119.271296489071));
#68687=CARTESIAN_POINT('Ctrl Pts',(0.237993424663934,-8.44948773760265,
119.589099628479));
#68688=CARTESIAN_POINT('Ctrl Pts',(7.23484662668109,-4.38285471727832,119.906902767886));
#68689=CARTESIAN_POINT('Ctrl Pts',(7.59906568335794,3.71726825545198,120.224705907294));
#68690=CARTESIAN_POINT('Ctrl Pts',(2.09783208782094,7.6057477909672,120.4895418568));
#68691=CARTESIAN_POINT('Ctrl Pts',(-2.76471087619419,6.90200431932459,120.701410616405));
#68692=CARTESIAN_POINT('Ctrl Pts',(-6.76842455398081,4.0542234750396,120.913279376011));
#68693=CARTESIAN_POINT('Ctrl Pts',(-8.06391256472688,-2.55679422156329,
121.178115325517));
#68694=CARTESIAN_POINT('Ctrl Pts',(-2.20839731887642,-8.16550074804653,
121.495918464925));
#68695=CARTESIAN_POINT('Ctrl Pts',(5.66102414021502,-6.2772039621143,121.813721604332));
#68696=CARTESIAN_POINT('Ctrl Pts',(8.34947323976075,1.35599329013339,122.13152474374));
#68697=CARTESIAN_POINT('Ctrl Pts',(3.37341782485002,7.75783054223044,122.449327883148));
#68698=CARTESIAN_POINT('Ctrl Pts',(-3.33584522554693,7.14985563208721,122.714163832654));
#68699=CARTESIAN_POINT('Ctrl Pts',(-6.58069071046394,3.46060682917539,122.926032592259));
#68700=CARTESIAN_POINT('Ctrl Pts',(-7.78131162404423,-1.30364425285691,
123.137901351864));
#68701=CARTESIAN_POINT('Ctrl Pts',(-4.47986753731459,-7.17597863647143,
123.402737301371));
#68702=CARTESIAN_POINT('Ctrl Pts',(3.61471026720376,-7.64763302391918,123.720540440778));
#68703=CARTESIAN_POINT('Ctrl Pts',(8.38008606205693,-1.1066352111694,124.038343580186));
#68704=CARTESIAN_POINT('Ctrl Pts',(5.47600255365382,6.44715574627637,124.356146719594));
#68705=CARTESIAN_POINT('Ctrl Pts',(-2.46353150501837,8.09289163814524,124.673949859001));
#68706=CARTESIAN_POINT('Ctrl Pts',(-7.17616749093923,3.27885941608981,124.938785808508));
#68707=CARTESIAN_POINT('Ctrl Pts',(-7.25342616325499,-1.63373766166086,
125.150654568113));
#68708=CARTESIAN_POINT('Ctrl Pts',(-5.07748184492967,-6.0388307678642,125.362523327718));
#68709=CARTESIAN_POINT('Ctrl Pts',(1.24397087744539,-8.36758143067917,125.627359277224));
#68710=CARTESIAN_POINT('Ctrl Pts',(7.71126387316832,-3.47689957616502,125.945162416632));
#68711=CARTESIAN_POINT('Ctrl Pts',(7.0964285749799,4.59251405858379,126.26296555604));
#68712=CARTESIAN_POINT('Ctrl Pts',(-0.01306199897006,8.45885633927841,126.580768695447));
#68713=CARTESIAN_POINT('Ctrl Pts',(-7.12378344817752,4.56241075819036,126.898571834855));
#68714=CARTESIAN_POINT('Ctrl Pts',(-7.58881792994159,-2.15827277115052,
127.163407784361));
#68715=CARTESIAN_POINT('Ctrl Pts',(-4.46158744940634,-5.94773295333789,
127.375276543967));
#68716=CARTESIAN_POINT('Ctrl Pts',(0.0515897489622841,-7.88959044731065,
127.587145303571));
#68717=CARTESIAN_POINT('Ctrl Pts',(6.373630862723,-5.56243761032195,127.851981253078));
#68718=CARTESIAN_POINT('Ctrl Pts',(8.12455869827376,2.35456304707941,128.169784392486));
#68719=CARTESIAN_POINT('Ctrl Pts',(2.42318628164524,8.09806471587669,128.487587531893));
#68720=CARTESIAN_POINT('Ctrl Pts',(-5.49588753251821,6.43021317020505,128.805390671301));
#68721=CARTESIAN_POINT('Ctrl Pts',(-8.38138462357639,-1.14728999588441,
129.123193810709));
#68722=CARTESIAN_POINT('Ctrl Pts',(-4.37669547353614,-6.56451336051821,
129.388029760215));
#68723=CARTESIAN_POINT('Ctrl Pts',(0.461313230403254,-7.420813968587,129.59989851982));
#68724=CARTESIAN_POINT('Ctrl Pts',(5.15601967593785,-5.97191426845995,129.811767279426));
#68725=CARTESIAN_POINT('Ctrl Pts',(8.45894789369403,-0.100414514637539,
130.076603228932));
#68726=CARTESIAN_POINT('Ctrl Pts',(4.65718588468659,7.06137669437366,130.39440636834));
#68727=CARTESIAN_POINT('Ctrl Pts',(-3.40748264062172,7.73560249443716,130.712209507747));
#68728=CARTESIAN_POINT('Ctrl Pts',(-8.35362120749351,1.33020070142903,131.030012647155));
#68729=CARTESIAN_POINT('Ctrl Pts',(-5.63564613659342,-6.30899161245907,
131.347815786563));
#68730=CARTESIAN_POINT('Ctrl Pts',(0.925940587278862,-7.83523662420755,
131.612651736069));
#68731=CARTESIAN_POINT('Ctrl Pts',(5.16386922553399,-5.34936860521914,131.824520495674));
#68732=CARTESIAN_POINT('Ctrl Pts',(7.7976944621173,-1.20177369082486,132.036389255279));
#68733=CARTESIAN_POINT('Ctrl Pts',(6.50387743193635,5.40957123008177,132.301225204786));
#68734=CARTESIAN_POINT('Ctrl Pts',(-1.03467581762238,8.39534794614227,132.619028344193));
#68735=CARTESIAN_POINT('Ctrl Pts',(-7.61057914893361,3.67825623303999,132.936831483601));
#68736=CARTESIAN_POINT('Ctrl Pts',(-7.22127632069979,-4.4051775769506,133.254634623009));
#68737=CARTESIAN_POINT('Ctrl Pts',(-0.198060572421381,-8.45722499125046,
133.572437762416));
#68738=CARTESIAN_POINT('Ctrl Pts',(5.78630429757597,-5.36348594706348,133.837273711923));
#68739=CARTESIAN_POINT('Ctrl Pts',(7.3999207693856,-0.722815647130796,134.049142471528));
#68740=CARTESIAN_POINT('Ctrl Pts',(6.71482719261795,4.14238997461265,134.261011231133));
#68741=CARTESIAN_POINT('Ctrl Pts',(1.4422521881325,8.33569380248617,134.525847180639));
#68742=CARTESIAN_POINT('Ctrl Pts',(-6.23232815901695,5.71931000232475,134.843650320047));
#68743=CARTESIAN_POINT('Ctrl Pts',(-8.17850859011008,-2.13599652143357,
135.161453459455));
#68744=CARTESIAN_POINT('Ctrl Pts',(-2.63971352946167,-8.03643787176537,
135.479256598862));
#68745=CARTESIAN_POINT('Ctrl Pts',(5.33412794588531,-6.56589381576526,135.79705973827));
#68746=CARTESIAN_POINT('Ctrl Pts',(7.88285957603773,-0.329884575213671,
136.061895687776));
#68747=CARTESIAN_POINT('Ctrl Pts',(6.10142549966758,4.24898772943948,136.273764447381));
#68748=CARTESIAN_POINT('Ctrl Pts',(2.42464571030607,7.50795525479395,136.485633206987));
#68749=CARTESIAN_POINT('Ctrl Pts',(-4.30825987416497,7.2803007767289,136.750469156493));
#68750=CARTESIAN_POINT('Ctrl Pts',(-8.45313029862189,0.311463222368526,
137.068272295901));
#68751=CARTESIAN_POINT('Ctrl Pts',(-4.84000141151651,-6.92999785242384,
137.386075435308));
#68752=CARTESIAN_POINT('Ctrl Pts',(3.20269938910426,-7.82912113888902,137.703878574716));
#68753=CARTESIAN_POINT('Ctrl Pts',(8.31848851820898,-1.53838594488056,138.021681714124));
#68754=CARTESIAN_POINT('Ctrl Pts',(6.21419397381502,4.86128503425738,138.28651766363));
#68755=CARTESIAN_POINT('Ctrl Pts',(1.88860523510587,7.19127666821767,138.498386423235));
#68756=CARTESIAN_POINT('Ctrl Pts',(-3.02365949204008,7.28737141942756,138.71025518284));
#68757=CARTESIAN_POINT('Ctrl Pts',(-8.00094636172687,2.74749701724112,138.975091132347));
#68758=CARTESIAN_POINT('Ctrl Pts',(-6.63632369986131,-5.24515289910853,
139.292894271754));
#68759=CARTESIAN_POINT('Ctrl Pts',(0.810315866115488,-8.41390944182324,
139.610697411162));
#68760=CARTESIAN_POINT('Ctrl Pts',(7.51535391249767,-3.88225150579835,139.928500550569));
#68761=CARTESIAN_POINT('Ctrl Pts',(7.32955153748415,4.22392670418686,140.246303689978));
#68762=CARTESIAN_POINT('Ctrl Pts',(1.57733990126167,7.73047849517612,140.511139639483));
#68763=CARTESIAN_POINT('Ctrl Pts',(-3.22630085224598,6.69867693382198,140.723008399089));
#68764=CARTESIAN_POINT('Ctrl Pts',(-7.0277240929022,3.58599958206011,140.934877158694));
#68765=CARTESIAN_POINT('Ctrl Pts',(-7.87200821982235,-3.09763928339454,
141.1997131082));
#68766=CARTESIAN_POINT('Ctrl Pts',(-1.64969981275852,-8.29643970098937,
141.517516247608));
#68767=CARTESIAN_POINT('Ctrl Pts',(6.07358854532228,-5.87894600079035,141.835319387016));
#68768=CARTESIAN_POINT('Ctrl Pts',(8.23832537682881,1.91896226379478,142.153122526423));
#68769=CARTESIAN_POINT('Ctrl Pts',(2.83967936581918,7.96869522834969,142.470925665831));
#68770=CARTESIAN_POINT('Ctrl Pts',(-3.81292517333676,6.9072353768361,142.735761615337));
#68771=CARTESIAN_POINT('Ctrl Pts',(-6.80017538638254,3.00647710241965,142.947630374943));
#68772=CARTESIAN_POINT('Ctrl Pts',(-7.67502034808243,-1.82821267498914,
143.159499134547));
#68773=CARTESIAN_POINT('Ctrl Pts',(-3.98303231037213,-7.46319878855479,
143.424335084054));
#68774=CARTESIAN_POINT('Ctrl Pts',(4.12489754031804,-7.38496049186462,143.742138223462));
#68775=CARTESIAN_POINT('Ctrl Pts',(8.43583245558475,-0.535924135632676,
144.059941362869));
#68776=CARTESIAN_POINT('Ctrl Pts',(5.02628893808761,6.80359027978314,144.377744502277));
#68777=CARTESIAN_POINT('Ctrl Pts',(-3.00655593015018,7.90724376650081,144.695547641685));
#68778=CARTESIAN_POINT('Ctrl Pts',(-7.38195959663264,2.78477493533829,144.960383591191));
#68779=CARTESIAN_POINT('Ctrl Pts',(-7.12596943535156,-2.12175622080281,
145.172252350796));
#68780=CARTESIAN_POINT('Ctrl Pts',(-4.65636941776872,-6.36918540902089,
145.384121110401));
#68781=CARTESIAN_POINT('Ctrl Pts',(1.80842534117273,-8.26398695045161,145.648957059908));
#68782=CARTESIAN_POINT('Ctrl Pts',(7.92925171044218,-2.94608019540264,145.966760199315));
#68783=CARTESIAN_POINT('Ctrl Pts',(6.76872988120031,5.06308005923279,146.284563338723));
#68784=CARTESIAN_POINT('Ctrl Pts',(-0.586537195444585,8.43850669521212,
146.602366478131));
#68785=CARTESIAN_POINT('Ctrl Pts',(-7.41672008904618,4.06892440513404,146.920169617539));
#68786=CARTESIAN_POINT('Ctrl Pts',(-7.42502628740076,-2.66782372811747,
147.185005567045));
#68787=CARTESIAN_POINT('Ctrl Pts',(-4.04806860277639,-6.23653993682789,
147.39687432665));
#68788=CARTESIAN_POINT('Ctrl Pts',(0.586380456386066,-7.86793857988935,
147.608743086255));
#68789=CARTESIAN_POINT('Ctrl Pts',(6.73609474152045,-5.11750997130243,147.873579035761));
#68790=CARTESIAN_POINT('Ctrl Pts',(7.9462260902675,2.89998509101313,148.191382175169));
#68791=CARTESIAN_POINT('Ctrl Pts',(1.86856641345216,8.2437216336388,148.509185314577));
#68792=CARTESIAN_POINT('Ctrl Pts',(-5.91920538067212,6.04279884965457,148.826988453984));
#68793=CARTESIAN_POINT('Ctrl Pts',(-8.28431422065509,-1.71290189729374,
149.144791593392));
#68794=CARTESIAN_POINT('Ctrl Pts',(-3.92155298584147,-6.84614703813004,
149.409627542898));
#68795=CARTESIAN_POINT('Ctrl Pts',(0.963376180029544,-7.3724596885991,149.621496302504));
#68796=CARTESIAN_POINT('Ctrl Pts',(5.54905295979434,-5.60860275371463,149.833365062109));
#68797=CARTESIAN_POINT('Ctrl Pts',(8.44628041647932,0.473338570214859,150.098201011615));
#68798=CARTESIAN_POINT('Ctrl Pts',(4.16773148534924,7.36086489439583,150.416004151023));
#68799=CARTESIAN_POINT('Ctrl Pts',(-3.92414558494879,7.48680986493268,150.733807290431));
#68800=CARTESIAN_POINT('Ctrl Pts',(-8.42452068060102,0.760708132485531,
151.051610429838));
#68801=CARTESIAN_POINT('Ctrl Pts',(-5.1950624265719,-6.67644604184268,151.369413569246));
#68802=CARTESIAN_POINT('Ctrl Pts',(1.45526099684437,-7.75464208274247,151.634249518752));
#68803=CARTESIAN_POINT('Ctrl Pts',(5.51436814750265,-4.98666840110588,151.846118278357));
#68804=CARTESIAN_POINT('Ctrl Pts',(7.86196849621255,-0.671020980375969,
152.057987037962));
#68805=CARTESIAN_POINT('Ctrl Pts',(6.12058015872781,5.83955124144195,152.322822987469));
#68806=CARTESIAN_POINT('Ctrl Pts',(-1.59886355244496,8.30341385629451,152.640626126877));
#68807=CARTESIAN_POINT('Ctrl Pts',(-7.84728433526637,3.1583187843365,152.958429266284));
#68808=CARTESIAN_POINT('Ctrl Pts',(-6.89665240705195,-4.89327593653704,
153.276232405692));
#68809=CARTESIAN_POINT('Ctrl Pts',(-0.853023022284405,-7.84339939259971,
153.541068355198));
#68810=CARTESIAN_POINT('Ctrl Pts',(3.85308616354897,-6.36807934659861,153.752940555492));
#68811=CARTESIAN_POINT('Ctrl Pts',(5.575743272665,-4.63562593309149,153.858878375984));
#68812=CARTESIAN_POINT('Ctrl Pts',(6.17613128330911,-3.60784117027914,153.911849006574));
#68813=CARTESIAN_POINT('Ctrl Pts',(3.92189707255582,-5.50607442349664,0.00384848156121544));
#68814=CARTESIAN_POINT('Ctrl Pts',(4.83912110844101,-4.85277318818901,0.0568724131943062));
#68815=CARTESIAN_POINT('Ctrl Pts',(6.32345378264837,-3.08238468302881,0.162863534728675));
#68816=CARTESIAN_POINT('Ctrl Pts',(7.30927705068616,1.47456590514539,0.374789036065603));
#68817=CARTESIAN_POINT('Ctrl Pts',(4.01501554670995,6.91028183275668,0.639624985571995));
#68818=CARTESIAN_POINT('Ctrl Pts',(-3.64467828148407,7.11551430628303,0.95742812497967));
#68819=CARTESIAN_POINT('Ctrl Pts',(-7.95222266353516,0.793792895267176,
1.27523126438734));
#68820=CARTESIAN_POINT('Ctrl Pts',(-4.97212509168922,-6.26086721103317,
1.59303440379501));
#68821=CARTESIAN_POINT('Ctrl Pts',(1.30485300361989,-7.34234073945092,1.85787035330141));
#68822=CARTESIAN_POINT('Ctrl Pts',(5.16576429400649,-4.76316292789717,2.06973911290652));
#68823=CARTESIAN_POINT('Ctrl Pts',(7.42341252941831,-0.705627305158844,
2.28160787251164));
#68824=CARTESIAN_POINT('Ctrl Pts',(5.83908213869992,5.46142515952503,2.54644382201803));
#68825=CARTESIAN_POINT('Ctrl Pts',(-1.43744337681211,7.86414290590199,2.8642469614257));
#68826=CARTESIAN_POINT('Ctrl Pts',(-7.38275336158889,3.05231572299541,3.18205010083337));
#68827=CARTESIAN_POINT('Ctrl Pts',(-6.57124549684319,-4.5530973272568,3.49985324024105));
#68828=CARTESIAN_POINT('Ctrl Pts',(0.277803164040553,-7.99030393413117,
3.81765637964872));
#68829=CARTESIAN_POINT('Ctrl Pts',(5.75410874632856,-4.74254802380421,4.08249232915512));
#68830=CARTESIAN_POINT('Ctrl Pts',(7.02157291719532,-0.275386851147049,
4.29436108876022));
#68831=CARTESIAN_POINT('Ctrl Pts',(6.10786722962805,4.27731130384919,4.50622984836535));
#68832=CARTESIAN_POINT('Ctrl Pts',(0.90276317339467,7.94401173023616,4.77106579787173));
#68833=CARTESIAN_POINT('Ctrl Pts',(-6.19447961726102,5.05375776909775,5.08886893727942));
#68834=CARTESIAN_POINT('Ctrl Pts',(-7.59909807827523,-2.46469341659131,
5.40667207668708));
#68835=CARTESIAN_POINT('Ctrl Pts',(-2.04901701299504,-7.72745660686897,
5.72447521609476));
#68836=CARTESIAN_POINT('Ctrl Pts',(5.39353975456735,-5.9018657915656,6.04227835550243));
#68837=CARTESIAN_POINT('Ctrl Pts',(7.45564034162571,0.121878774205148,6.30711430500882));
#68838=CARTESIAN_POINT('Ctrl Pts',(5.5232612325937,4.34418463217063,6.51898306461393));
#68839=CARTESIAN_POINT('Ctrl Pts',(1.87513732783761,7.2170136964436,6.73085182421905));
#68840=CARTESIAN_POINT('Ctrl Pts',(-4.46488187821364,6.63227883343294,6.99568777372545));
#68841=CARTESIAN_POINT('Ctrl Pts',(-7.99268121358921,-0.170593163642286,
7.31349091313311));
#68842=CARTESIAN_POINT('Ctrl Pts',(-4.18579272791893,-6.80442075922423,
7.6312940525408));
#68843=CARTESIAN_POINT('Ctrl Pts',(3.45193553577881,-7.21083879562565,7.94909719194845));
#68844=CARTESIAN_POINT('Ctrl Pts',(7.93305976229589,-0.994412074459289,
8.26690033135614));
#68845=CARTESIAN_POINT('Ctrl Pts',(5.59601594140876,4.92808607679508,8.53173628086252));
#68846=CARTESIAN_POINT('Ctrl Pts',(1.38678064839306,6.88877305814278,8.74360504046765));
#68847=CARTESIAN_POINT('Ctrl Pts',(-3.25324393373007,6.70953282295394,8.95547380007275));
#68848=CARTESIAN_POINT('Ctrl Pts',(-7.69989228592105,2.15266146016066,9.22030974957918));
#68849=CARTESIAN_POINT('Ctrl Pts',(-5.9732055492464,-5.31346125678687,9.53811288898681));
#68850=CARTESIAN_POINT('Ctrl Pts',(1.22684194597112,-7.89403961704749,9.85591602839451));
#68851=CARTESIAN_POINT('Ctrl Pts',(7.30408302773333,-3.24998864384153,10.1737191678022));
#68852=CARTESIAN_POINT('Ctrl Pts',(6.68338086465625,4.38801923353478,10.4915223072099));
#68853=CARTESIAN_POINT('Ctrl Pts',(1.06347372757189,7.3804099091378,10.7563582567163));
#68854=CARTESIAN_POINT('Ctrl Pts',(-3.41209097832941,6.14296263768009,10.9682270163214));
#68855=CARTESIAN_POINT('Ctrl Pts',(-6.82772436023289,2.99726656419267,11.1800957759264));
#68856=CARTESIAN_POINT('Ctrl Pts',(-7.25707551891202,-3.35516728178466,
11.4449317254329));
#68857=CARTESIAN_POINT('Ctrl Pts',(-1.10064870702956,-7.91837278010439,
11.7627348648406));
#68858=CARTESIAN_POINT('Ctrl Pts',(6.05347976412343,-5.21309748436201,12.0805380042483));
#68859=CARTESIAN_POINT('Ctrl Pts',(7.66746027614776,2.26320745285952,12.3983411436559));
#68860=CARTESIAN_POINT('Ctrl Pts',(2.24140798450443,7.67452818243227,12.7161442830636));
#68861=CARTESIAN_POINT('Ctrl Pts',(-3.97703306998174,6.30750622325713,12.9809802325699));
#68862=CARTESIAN_POINT('Ctrl Pts',(-6.58118903448087,2.46298715074713,13.1928489921751));
#68863=CARTESIAN_POINT('Ctrl Pts',(-7.14096562836087,-2.14663380452386,
13.4047177517802));
#68864=CARTESIAN_POINT('Ctrl Pts',(-3.34794148307743,-7.26041186172221,
13.6695537012866));
#68865=CARTESIAN_POINT('Ctrl Pts',(4.29762922081813,-6.74110066245508,13.9873568406943));
#68866=CARTESIAN_POINT('Ctrl Pts',(7.98869370380649,-0.0421371911454969,
14.3051599801019));
#68867=CARTESIAN_POINT('Ctrl Pts',(4.36850138181588,6.695390260325,14.6229631195097));
#68868=CARTESIAN_POINT('Ctrl Pts',(-3.27116574347611,7.29532502734838,14.9407662589173));
#68869=CARTESIAN_POINT('Ctrl Pts',(-7.11792364148947,2.22184379065709,15.2056022084237));
#68870=CARTESIAN_POINT('Ctrl Pts',(-6.6068046863944,-2.39342571394088,15.4174709680288));
#68871=CARTESIAN_POINT('Ctrl Pts',(-4.04334911920576,-6.26520188791823,
15.6293397276339));
#68872=CARTESIAN_POINT('Ctrl Pts',(2.16032533671653,-7.69774558007002,15.8941756771403));
#68873=CARTESIAN_POINT('Ctrl Pts',(7.64315926909541,-2.34396489910217,16.211978816548));
#68874=CARTESIAN_POINT('Ctrl Pts',(6.10813545411811,5.14894978711782,16.5297819559557));
#68875=CARTESIAN_POINT('Ctrl Pts',(-1.01705723707682,7.92954283912332,16.8475850953633));
#68876=CARTESIAN_POINT('Ctrl Pts',(-7.22127835658967,3.43153485667809,17.165388234771));
#68877=CARTESIAN_POINT('Ctrl Pts',(-6.85896236183368,-2.92507471957642,
17.4302241842774));
#68878=CARTESIAN_POINT('Ctrl Pts',(-3.4767027056567,-6.10662698294204,17.6420929438824));
#68879=CARTESIAN_POINT('Ctrl Pts',(0.985559249797878,-7.39121774549323,
17.8539617034876));
#68880=CARTESIAN_POINT('Ctrl Pts',(6.63672015772432,-4.45827748396203,18.118797652994));
#68881=CARTESIAN_POINT('Ctrl Pts',(7.33796046741645,3.17275767111442,18.4366007924016));
#68882=CARTESIAN_POINT('Ctrl Pts',(1.3100472228219,7.88065853276818,18.7544039318094));
#68883=CARTESIAN_POINT('Ctrl Pts',(-5.91682194971578,5.37617643649685,19.072207071217));
#68884=CARTESIAN_POINT('Ctrl Pts',(-7.72217209282292,-2.07131618657662,
19.3900102106246));
#68885=CARTESIAN_POINT('Ctrl Pts',(-3.32384119939761,-6.6748413072779,19.6548461601311));
#68886=CARTESIAN_POINT('Ctrl Pts',(1.31403441604731,-6.90301878642667,19.8667149197362));
#68887=CARTESIAN_POINT('Ctrl Pts',(5.54371861830293,-4.98684375905617,20.0785836793414));
#68888=CARTESIAN_POINT('Ctrl Pts',(7.94310832364928,0.910671584447784,20.3434196288477));
#68889=CARTESIAN_POINT('Ctrl Pts',(3.52780997821278,7.1740234052172,20.6612227682555));
#68890=CARTESIAN_POINT('Ctrl Pts',(-4.11378057803941,6.84819771851404,20.9790259076631));
#68891=CARTESIAN_POINT('Ctrl Pts',(-7.99043692094834,0.254897770346762,
21.2968290470708));
#68892=CARTESIAN_POINT('Ctrl Pts',(-4.53459677443546,-6.5848101467868,21.6146321864784));
#68893=CARTESIAN_POINT('Ctrl Pts',(1.79890132903279,-7.23639280336275,21.8794681359848));
#68894=CARTESIAN_POINT('Ctrl Pts',(5.4771274989967,-4.40220730680084,22.0913368955899));
#68895=CARTESIAN_POINT('Ctrl Pts',(7.45393977391325,-0.200520929158071,
22.3032056551951));
#68896=CARTESIAN_POINT('Ctrl Pts',(5.45549800092228,5.84464148925155,22.5680416047014));
#68897=CARTESIAN_POINT('Ctrl Pts',(-1.96738686567052,7.74864142813236,22.8858447441091));
#68898=CARTESIAN_POINT('Ctrl Pts',(-7.57267517394138,2.54471871649641,23.2036478835168));
#68899=CARTESIAN_POINT('Ctrl Pts',(-6.24744706111155,-4.98813194288109,
23.5214510229244));
#68900=CARTESIAN_POINT('Ctrl Pts',(0.818913163983748,-7.95309209086637,
23.8392541623321));
#68901=CARTESIAN_POINT('Ctrl Pts',(6.06240479820683,-4.34150605882739,24.1040901118385));
#68902=CARTESIAN_POINT('Ctrl Pts',(7.02408938913868,0.20130341702492,24.3159588714437));
#68903=CARTESIAN_POINT('Ctrl Pts',(5.80381212343591,4.68158003584414,24.5278276310488));
#68904=CARTESIAN_POINT('Ctrl Pts',(0.362087741070216,7.98693840239888,24.7926635805551));
#68905=CARTESIAN_POINT('Ctrl Pts',(-6.52286811072147,4.62214740906376,25.1104667199629));
#68906=CARTESIAN_POINT('Ctrl Pts',(-7.41450740655606,-2.97423646575735,
25.4282698593705));
#68907=CARTESIAN_POINT('Ctrl Pts',(-1.5203855076761,-7.84859751605537,25.7460729987782));
#68908=CARTESIAN_POINT('Ctrl Pts',(5.78127203409363,-5.52260683407338,26.0638761381858));
#68909=CARTESIAN_POINT('Ctrl Pts',(7.43022137695885,0.627086186692075,26.3287120876923));
#68910=CARTESIAN_POINT('Ctrl Pts',(5.21601903740572,4.70866225309671,26.5405808472972));
#68911=CARTESIAN_POINT('Ctrl Pts',(1.38151348805886,7.32754032936478,26.7524496069024));
#68912=CARTESIAN_POINT('Ctrl Pts',(-4.90427248829062,6.31430153988095,27.0172855564088));
#68913=CARTESIAN_POINT('Ctrl Pts',(-7.96272374104042,-0.712099490839074,
27.3350886958166));
#68914=CARTESIAN_POINT('Ctrl Pts',(-3.7148255683103,-7.07255778577618,27.6528918352242));
#68915=CARTESIAN_POINT('Ctrl Pts',(3.93288297675611,-6.96020736416123,27.9706949746319));
#68916=CARTESIAN_POINT('Ctrl Pts',(7.98222611578696,-0.454267335822995,
28.2884981140396));
#68917=CARTESIAN_POINT('Ctrl Pts',(5.24901816070196,5.29615286267089,28.553334063546));
#68918=CARTESIAN_POINT('Ctrl Pts',(0.916535055346602,6.96694468936257,28.7652028231511));
#68919=CARTESIAN_POINT('Ctrl Pts',(-3.70066033372871,6.47352607861612,28.9770715827562));
#68920=CARTESIAN_POINT('Ctrl Pts',(-7.82812375889614,1.62566017093144,29.2419075322626));
#68921=CARTESIAN_POINT('Ctrl Pts',(-5.59921164576593,-5.70621450761371,
29.5597106716702));
#68922=CARTESIAN_POINT('Ctrl Pts',(1.75922998076748,-7.79269610025208,29.877513811078));
#68923=CARTESIAN_POINT('Ctrl Pts',(7.50762337597611,-2.74729800085093,30.1953169504856));
#68924=CARTESIAN_POINT('Ctrl Pts',(6.37049722937737,4.83105139968957,30.5131200898933));
#68925=CARTESIAN_POINT('Ctrl Pts',(0.560639395885922,7.43553026111364,30.7779560393996));
#68926=CARTESIAN_POINT('Ctrl Pts',(-3.82072875711326,5.89748985390262,30.9898247990048));
#68927=CARTESIAN_POINT('Ctrl Pts',(-7.01522642047157,2.52745426579268,31.2016935586098));
#68928=CARTESIAN_POINT('Ctrl Pts',(-7.01289852442548,-3.83947221139287,
31.4665295081164));
#68929=CARTESIAN_POINT('Ctrl Pts',(-0.561255283071585,-7.97477570645133,
31.7843326475239));
#68930=CARTESIAN_POINT('Ctrl Pts',(6.39299535422847,-4.79067980947678,32.1021357869317));
#68931=CARTESIAN_POINT('Ctrl Pts',(7.49637318042916,2.77784884411021,32.4199389263393));
#68932=CARTESIAN_POINT('Ctrl Pts',(1.71592215789716,7.80883497866261,32.7377420657469));
#68933=CARTESIAN_POINT('Ctrl Pts',(-4.39552685639725,6.02335209421187,33.0025780152534));
#68934=CARTESIAN_POINT('Ctrl Pts',(-6.73303456328756,2.01111918639638,33.2144467748584));
#68935=CARTESIAN_POINT('Ctrl Pts',(-6.97899363197104,-2.62584742151247,
33.4263155344636));
#68936=CARTESIAN_POINT('Ctrl Pts',(-2.84798632628573,-7.47069384068419,
33.6911514839699));
#68937=CARTESIAN_POINT('Ctrl Pts',(4.74478274349493,-6.43421259969041,34.0089546233777));
#68938=CARTESIAN_POINT('Ctrl Pts',(7.97316839033122,0.499588286030254,34.3267577627853));
#68939=CARTESIAN_POINT('Ctrl Pts',(3.90450600749062,6.97616570176283,34.6445609021931));
#68940=CARTESIAN_POINT('Ctrl Pts',(-3.75825725591887,7.05675527238122,34.9623640416006));
#68941=CARTESIAN_POINT('Ctrl Pts',(-7.25218475873788,1.73414042721053,35.2271999911071));
#68942=CARTESIAN_POINT('Ctrl Pts',(-6.42932946840217,-2.83585567317026,
35.4390687507122));
#68943=CARTESIAN_POINT('Ctrl Pts',(-3.60926843557079,-6.52492208046566,
35.6509375103173));
#68944=CARTESIAN_POINT('Ctrl Pts',(2.67725678732941,-7.5335641412711,35.9157734598237));
#68945=CARTESIAN_POINT('Ctrl Pts',(7.78449154171594,-1.82036987942978,36.2335765992314));
#68946=CARTESIAN_POINT('Ctrl Pts',(5.74498484987571,5.55122974761572,36.551379738639));
#68947=CARTESIAN_POINT('Ctrl Pts',(-1.55233508847075,7.8423409026951,36.8691828780467));
#68948=CARTESIAN_POINT('Ctrl Pts',(-7.43731796205355,2.93404057696251,37.1869860174544));
#68949=CARTESIAN_POINT('Ctrl Pts',(-6.64486144705489,-3.38337747607327,
37.4518219669608));
#68950=CARTESIAN_POINT('Ctrl Pts',(-3.05467717095417,-6.3282937821792,37.6636907265659));
#68951=CARTESIAN_POINT('Ctrl Pts',(1.48441146870158,-7.3073900530725,37.875559486171));
#68952=CARTESIAN_POINT('Ctrl Pts',(6.92371736506755,-3.99805332938537,38.1403954356774));
#68953=CARTESIAN_POINT('Ctrl Pts',(7.10596461397305,3.66296627966264,38.4581985750851));
#68954=CARTESIAN_POINT('Ctrl Pts',(0.772728970275458,7.95134533111302,38.7760017144927));
#68955=CARTESIAN_POINT('Ctrl Pts',(-6.2677086455842,4.96264882850391,39.0938048539005));
#68956=CARTESIAN_POINT('Ctrl Pts',(-7.56396921361207,-2.59010855206421,
39.4116079933081));
#68957=CARTESIAN_POINT('Ctrl Pts',(-2.86364282132101,-6.88483671469794,
39.6764439428145));
#68958=CARTESIAN_POINT('Ctrl Pts',(1.77903121608731,-6.79804403814093,39.8883127024196));
#68959=CARTESIAN_POINT('Ctrl Pts',(5.86906731849622,-4.59950819187393,40.1001814620248));
#68960=CARTESIAN_POINT('Ctrl Pts',(7.86308805449229,1.44711396346235,40.3650174115311));
#68961=CARTESIAN_POINT('Ctrl Pts',(3.03329802360466,7.3966991395472,40.6828205509388));
#68962=CARTESIAN_POINT('Ctrl Pts',(-4.56861825567268,6.55352804755189,41.0006236903464));
#68963=CARTESIAN_POINT('Ctrl Pts',(-7.98933263266374,-0.287435463428486,
41.3184268297541));
#68964=CARTESIAN_POINT('Ctrl Pts',(-4.07771647401996,-6.87710120133864,
41.6362299691616));
#68965=CARTESIAN_POINT('Ctrl Pts',(2.28538499112399,-7.0977772745065,41.9010659186683));
#68966=CARTESIAN_POINT('Ctrl Pts',(5.76299143527295,-4.02073184001211,42.1129346782732));
#68967=CARTESIAN_POINT('Ctrl Pts',(7.45038326294484,0.305313005598657,42.3248034378785));
#68968=CARTESIAN_POINT('Ctrl Pts',(5.04668166278878,6.2010722274796,42.5896393873848));
#68969=CARTESIAN_POINT('Ctrl Pts',(-2.48821297984089,7.59742398632151,42.9074425267925));
#68970=CARTESIAN_POINT('Ctrl Pts',(-7.7277806175868,2.02544053543043,43.2252456662));
#68971=CARTESIAN_POINT('Ctrl Pts',(-5.89487924819143,-5.40022719061191,
43.5430488056078));
#68972=CARTESIAN_POINT('Ctrl Pts',(1.35624357475243,-7.87927001326201,43.8608519450155));
#68973=CARTESIAN_POINT('Ctrl Pts',(6.34280648913723,-3.9204888263474,44.1256878945219));
#68974=CARTESIAN_POINT('Ctrl Pts',(6.99427853146466,0.677069152014045,44.337556654127));
#68975=CARTESIAN_POINT('Ctrl Pts',(5.47304915659019,5.0643024915287,44.5494254137322));
#68976=CARTESIAN_POINT('Ctrl Pts',(-0.180254942171659,7.99310957836625,
44.8142613632384));
#68977=CARTESIAN_POINT('Ctrl Pts',(-6.82123757465311,4.16926528433038,45.1320645026462));
#68978=CARTESIAN_POINT('Ctrl Pts',(-7.19579503223384,-3.47009171207247,
45.4498676420539));
#68979=CARTESIAN_POINT('Ctrl Pts',(-0.98475697855021,-7.9336188939335,45.7676707814614));
#68980=CARTESIAN_POINT('Ctrl Pts',(6.14239852466531,-5.11793248686778,46.0854739208693));
#68981=CARTESIAN_POINT('Ctrl Pts',(7.37060818932517,1.12940768352659,46.3503098703756));
#68982=CARTESIAN_POINT('Ctrl Pts',(4.88477243985844,5.05147038228633,46.5621786299808));
#68983=CARTESIAN_POINT('Ctrl Pts',(0.881531863711674,7.40434523569889,46.7740473895858));
#68984=CARTESIAN_POINT('Ctrl Pts',(-5.32109339130866,5.96726551252067,47.0388833390923));
#68985=CARTESIAN_POINT('Ctrl Pts',(-7.89612140208864,-1.25032870256573,
47.3566864784998));
#68986=CARTESIAN_POINT('Ctrl Pts',(-3.2267625926084,-7.30814653705427,47.6744896179076));
#68987=CARTESIAN_POINT('Ctrl Pts',(4.39573108947547,-6.67754470220911,47.9922927573153));
#68988=CARTESIAN_POINT('Ctrl Pts',(7.99465785466138,0.0879679648973956,
48.310095896723));
#68989=CARTESIAN_POINT('Ctrl Pts',(4.87786412942484,5.63984648115765,48.5749318462293));
#68990=CARTESIAN_POINT('Ctrl Pts',(0.442071520850445,7.01305408383319,48.7868006058345));
#68991=CARTESIAN_POINT('Ctrl Pts',(-4.13104610495561,6.20772783511707,48.9986693654394));
#68992=CARTESIAN_POINT('Ctrl Pts',(-7.92032980481764,1.09117751024513,49.2635053149461));
#68993=CARTESIAN_POINT('Ctrl Pts',(-5.19944988304332,-6.07270746658381,
49.5813084543535));
#68994=CARTESIAN_POINT('Ctrl Pts',(2.28352194893603,-7.65549019624757,49.8991115937613));
#68995=CARTESIAN_POINT('Ctrl Pts',(7.67661325632821,-2.23196415153741,50.216914733169));
#68996=CARTESIAN_POINT('Ctrl Pts',(6.02829623905529,5.2518508194863,50.5347178725766));
#68997=CARTESIAN_POINT('Ctrl Pts',(0.055224972942848,7.45643192140313,50.799553822083));
#68998=CARTESIAN_POINT('Ctrl Pts',(-4.21178334616425,5.62487651929266,51.0114225816882));
#68999=CARTESIAN_POINT('Ctrl Pts',(-7.17044404886006,2.04601049320944,51.2232913412932));
#69000=CARTESIAN_POINT('Ctrl Pts',(-6.73644781118686,-4.30610769292906,
51.4881272907997));
#69001=CARTESIAN_POINT('Ctrl Pts',(-0.019278933510005,-7.99447830591245,
51.8059304302074));
#69002=CARTESIAN_POINT('Ctrl Pts',(6.70309005176943,-4.3462151803592,52.123733569615));
#69003=CARTESIAN_POINT('Ctrl Pts',(7.29078739079027,3.27970643248381,52.4415367090227));
#69004=CARTESIAN_POINT('Ctrl Pts',(1.18253956949703,7.90720511574864,52.7593398484304));
#69005=CARTESIAN_POINT('Ctrl Pts',(-4.79379220274076,5.71147818984704,53.0241757979367));
#69006=CARTESIAN_POINT('Ctrl Pts',(-6.85389432164721,1.54999594838462,53.2360445575419));
#69007=CARTESIAN_POINT('Ctrl Pts',(-6.78490394888292,-3.09297675396837,
53.4479133171469));
#69008=CARTESIAN_POINT('Ctrl Pts',(-2.33492459032621,-7.64659530336457,
53.7127492666534));
#69009=CARTESIAN_POINT('Ctrl Pts',(5.17010053259149,-6.09771396048381,54.030552406061));
#69010=CARTESIAN_POINT('Ctrl Pts',(7.92095014692118,1.03901463228617,54.3483555454688));
#69011=CARTESIAN_POINT('Ctrl Pts',(3.42254189622809,7.22483647078226,54.6661586848763));
#69012=CARTESIAN_POINT('Ctrl Pts',(-4.22805307568117,6.78570996765777,54.9839618242842));
#69013=CARTESIAN_POINT('Ctrl Pts',(-7.35307094970871,1.23845646056125,55.2487977737904));
#69014=CARTESIAN_POINT('Ctrl Pts',(-6.2222661463888,-3.26523487911977,55.4606665333956));
#69015=CARTESIAN_POINT('Ctrl Pts',(-3.15857771344953,-6.75461424688753,
55.6725352930006));
#69016=CARTESIAN_POINT('Ctrl Pts',(3.18186736487078,-7.33471285384217,55.9373712425071));
#69017=CARTESIAN_POINT('Ctrl Pts',(7.88999918493768,-1.28839742419215,56.2551743819147));
#69018=CARTESIAN_POINT('Ctrl Pts',(5.35539553065171,5.92796266405168,56.5729775213225));
#69019=CARTESIAN_POINT('Ctrl Pts',(-2.08046901415689,7.71904811114137,56.89078066073));
#69020=CARTESIAN_POINT('Ctrl Pts',(-7.61913064874144,2.42304369200314,57.2085838001378));
#69021=CARTESIAN_POINT('Ctrl Pts',(-6.40018053903285,-3.82610975586708,
57.4734197496441));
#69022=CARTESIAN_POINT('Ctrl Pts',(-2.61859385521392,-6.52083744880613,
57.6852885092493));
#69023=CARTESIAN_POINT('Ctrl Pts',(1.97643234988012,-7.18993337677778,57.8971572688543));
#69024=CARTESIAN_POINT('Ctrl Pts',(7.1788512699285,-3.51942992829707,58.1619932183609));
#69025=CARTESIAN_POINT('Ctrl Pts',(6.84126674685888,4.13631772949141,58.4797963577683));
#69026=CARTESIAN_POINT('Ctrl Pts',(0.231854579368945,7.98543963036104,58.7975994971761));
#69027=CARTESIAN_POINT('Ctrl Pts',(-6.5897510247487,4.52628285603161,59.1154026365838));
#69028=CARTESIAN_POINT('Ctrl Pts',(-7.37095656006863,-3.09698110512935,
59.4332057759915));
#69029=CARTESIAN_POINT('Ctrl Pts',(-2.39026581208361,-7.06314775038297,
59.6980417254979));
#69030=CARTESIAN_POINT('Ctrl Pts',(2.2358408232111,-6.66178434247006,59.9099104851029));
#69031=CARTESIAN_POINT('Ctrl Pts',(6.16740626982208,-4.19100545205031,60.1217792447082));
#69032=CARTESIAN_POINT('Ctrl Pts',(7.74688145075298,1.97689664978385,60.3866151942145));
#69033=CARTESIAN_POINT('Ctrl Pts',(2.52482667589181,7.58533488500591,60.704418333622));
#69034=CARTESIAN_POINT('Ctrl Pts',(-5.0024309177354,6.22869870433632,61.0222214730299));
#69035=CARTESIAN_POINT('Ctrl Pts',(-7.95146102577201,-0.828445904456495,
61.3400246124374));
#69036=CARTESIAN_POINT('Ctrl Pts',(-3.60207031321488,-7.13774348338487,
61.6578277518453));
#69037=CARTESIAN_POINT('Ctrl Pts',(2.76135119425199,-6.92649741053579,61.9226637013515));
#69038=CARTESIAN_POINT('Ctrl Pts',(6.02233378933796,-3.62075275904264,62.1345324609568));
#69039=CARTESIAN_POINT('Ctrl Pts',(7.4125397060154,0.809741874242037,62.3464012205618));
#69040=CARTESIAN_POINT('Ctrl Pts',(4.61464023676158,6.52896531321834,62.6112371700682));
#69041=CARTESIAN_POINT('Ctrl Pts',(-2.99758821023952,7.4112428095978,62.9290403094758));
#69042=CARTESIAN_POINT('Ctrl Pts',(-7.84732241841548,1.49684117312045,63.2468434488836));
#69043=CARTESIAN_POINT('Ctrl Pts',(-5.51518289857927,-5.78747031579437,
63.5646465882912));
#69044=CARTESIAN_POINT('Ctrl Pts',(1.8873324830186,-7.7691871308709,63.8824497276989));
#69045=CARTESIAN_POINT('Ctrl Pts',(6.59401825923553,-3.48142930317772,64.1472856772053));
#69046=CARTESIAN_POINT('Ctrl Pts',(6.93227964520087,1.14971898003392,64.3591544368104));
#69047=CARTESIAN_POINT('Ctrl Pts',(5.11709893677285,5.42371876736192,64.5710231964155));
#69048=CARTESIAN_POINT('Ctrl Pts',(-0.721768082922962,7.96249605402861,
64.8358591459219));
#69049=CARTESIAN_POINT('Ctrl Pts',(-7.08821535335468,3.69719598688643,65.1536622853295));
#69050=CARTESIAN_POINT('Ctrl Pts',(-6.94396724004815,-3.94997741832189,
65.4714654247371));
#69051=CARTESIAN_POINT('Ctrl Pts',(-0.444596547293857,-7.98212935068814,
65.7892685641449));
#69052=CARTESIAN_POINT('Ctrl Pts',(6.47525738213762,-4.68970515182132,66.1070717035525));
#69053=CARTESIAN_POINT('Ctrl Pts',(7.27707508471146,1.62653158826546,66.371907653059));
#69054=CARTESIAN_POINT('Ctrl Pts',(4.53104586896739,5.37103138564965,66.5837764126641));
#69055=CARTESIAN_POINT('Ctrl Pts',(0.377493384507276,7.44707496543455,66.7956451722693));
#69056=CARTESIAN_POINT('Ctrl Pts',(-5.71342634958102,5.59276782316797,67.0604811217756));
#69057=CARTESIAN_POINT('Ctrl Pts',(-7.79318070739572,-1.78280383746625,
67.3782842611832));
#69058=CARTESIAN_POINT('Ctrl Pts',(-2.72384988992859,-7.51010282307705,
67.696087400591));
#69059=CARTESIAN_POINT('Ctrl Pts',(4.83834982222698,-6.36415163700317,68.0138905399985));
#69060=CARTESIAN_POINT('Ctrl Pts',(7.97029776799309,0.62979843254267,68.3316936794063));
#69061=CARTESIAN_POINT('Ctrl Pts',(4.48426191718657,5.95758523680802,68.5965296289128));
#69062=CARTESIAN_POINT('Ctrl Pts',(-0.0344264494403155,7.02688904368688,
68.8083983885178));
#69063=CARTESIAN_POINT('Ctrl Pts',(-4.54242059014808,5.91336130961274,69.0202671481229));
#69064=CARTESIAN_POINT('Ctrl Pts',(-7.97608608657452,0.551673194826624,
69.2851030976293));
#69065=CARTESIAN_POINT('Ctrl Pts',(-4.77575998542697,-6.41125351452142,
69.6029062370369));
#69066=CARTESIAN_POINT('Ctrl Pts',(2.79730503229739,-7.48305333321018,69.9207093764445));
#69067=CARTESIAN_POINT('Ctrl Pts',(7.81027496804063,-1.70635868954371,70.2385125158524));
#69068=CARTESIAN_POINT('Ctrl Pts',(5.65835272148355,5.64848095407101,70.5563156552599));
#69069=CARTESIAN_POINT('Ctrl Pts',(-0.450443600392101,7.44301869658579,
70.8211516047665));
#69070=CARTESIAN_POINT('Ctrl Pts',(-4.58345508922149,5.32637721828354,71.0330203643715));
#69071=CARTESIAN_POINT('Ctrl Pts',(-7.29266293316989,1.55515086592525,71.2448891239765));
#69072=CARTESIAN_POINT('Ctrl Pts',(-6.42899560414404,-4.75292622588962,
71.5097250734831));
#69073=CARTESIAN_POINT('Ctrl Pts',(0.522786112825735,-7.97738993981093,
71.8275282128906));
#69074=CARTESIAN_POINT('Ctrl Pts',(6.98233683233883,-3.8817489844184,72.1453313522984));
#69075=CARTESIAN_POINT('Ctrl Pts',(7.0516489340484,3.76647052698219,72.4631344917059));
#69076=CARTESIAN_POINT('Ctrl Pts',(0.643715050988336,7.96918612069798,72.7809376311138));
#69077=CARTESIAN_POINT('Ctrl Pts',(-5.16999658185351,5.37331936552019,73.04577358062));
#69078=CARTESIAN_POINT('Ctrl Pts',(-6.94321169237049,1.08174008931842,73.2576423402253));
#69079=CARTESIAN_POINT('Ctrl Pts',(-6.5595907986434,-3.54587336298357,73.4695110998303));
#69080=CARTESIAN_POINT('Ctrl Pts',(-1.81111526918817,-7.78730395127627,
73.7343470493367));
#69081=CARTESIAN_POINT('Ctrl Pts',(5.57162165873517,-5.73315801212,74.0521501887443));
#69082=CARTESIAN_POINT('Ctrl Pts',(7.83228585815234,1.57366794318893,74.3699533281521));
#69083=CARTESIAN_POINT('Ctrl Pts',(2.92481462807732,7.44024196171124,74.6877564675598));
#69084=CARTESIAN_POINT('Ctrl Pts',(-4.67836648769833,6.48346864176512,75.0055596069673));
#69085=CARTESIAN_POINT('Ctrl Pts',(-7.42016107074263,0.737016856028769,
75.2703955564739));
#69086=CARTESIAN_POINT('Ctrl Pts',(-5.98651004441989,-3.67951228222445,
75.4822643160789));
#69087=CARTESIAN_POINT('Ctrl Pts',(-2.69349126760775,-6.95340398567554,
75.6941330756841));
#69088=CARTESIAN_POINT('Ctrl Pts',(3.67213255131463,-7.10171900127879,75.9589690251904));
#69089=CARTESIAN_POINT('Ctrl Pts',(7.95869722307977,-0.751146268374845,
76.2767721645981));
#69090=CARTESIAN_POINT('Ctrl Pts',(4.94207223697856,6.27860244049634,76.5945753040058));
#69091=CARTESIAN_POINT('Ctrl Pts',(-2.60074361304978,7.55799909062679,76.9123784434135));
#69092=CARTESIAN_POINT('Ctrl Pts',(-7.76256533177215,1.90520263087797,77.230181582821));
#69093=CARTESIAN_POINT('Ctrl Pts',(-5.80496517698946,-5.49065623539311,
77.5479847222288));
#69094=CARTESIAN_POINT('Ctrl Pts',(1.46920650516214,-7.85789503940717,77.8657878616364));
#69095=CARTESIAN_POINT('Ctrl Pts',(7.40524249463413,-3.01352847061608,78.1835910010441));
#69096=CARTESIAN_POINT('Ctrl Pts',(6.68073829681224,3.31247007627155,78.4484269505505));
#69097=CARTESIAN_POINT('Ctrl Pts',(3.12192870190511,6.29528985251686,78.6602957101557));
#69098=CARTESIAN_POINT('Ctrl Pts',(-1.40633759907391,7.3228545471876,78.8721644697607));
#69099=CARTESIAN_POINT('Ctrl Pts',(-6.88071188464259,4.07164371998688,79.1370004192671));
#69100=CARTESIAN_POINT('Ctrl Pts',(-7.14461299379745,-3.58695500756345,
79.454803558675));
#69101=CARTESIAN_POINT('Ctrl Pts',(-0.857498472942246,-7.94265880723423,
79.7726066980824));
#69102=CARTESIAN_POINT('Ctrl Pts',(6.21442707400568,-5.02921115503095,80.0904098374902));
#69103=CARTESIAN_POINT('Ctrl Pts',(7.59116134865531,2.50928490341992,80.4082129768979));
#69104=CARTESIAN_POINT('Ctrl Pts',(2.9369117728111,6.85390389418223,80.6730489264042));
#69105=CARTESIAN_POINT('Ctrl Pts',(-1.70642560514941,6.81663127064972,80.8849176860094));
#69106=CARTESIAN_POINT('Ctrl Pts',(-5.81967680521998,4.66184379221742,81.0967864456144));
#69107=CARTESIAN_POINT('Ctrl Pts',(-7.87807530250925,-1.36316764236396,
81.361622395121));
#69108=CARTESIAN_POINT('Ctrl Pts',(-3.11201529743014,-7.36392651431642,
81.6794255345284));
#69109=CARTESIAN_POINT('Ctrl Pts',(4.49846131872081,-6.601882199967,81.9972286739362));
#69110=CARTESIAN_POINT('Ctrl Pts',(7.99194390045502,0.202208465549562,82.3150318133438));
#69111=CARTESIAN_POINT('Ctrl Pts',(4.15083263104545,6.83321890882335,82.6328349527516));
#69112=CARTESIAN_POINT('Ctrl Pts',(-2.20955324892266,7.12174847300815,82.8976709022579));
#69113=CARTESIAN_POINT('Ctrl Pts',(-5.71978030542964,4.08196865298834,83.1095396618632));
#69114=CARTESIAN_POINT('Ctrl Pts',(-7.45321582548128,-0.225833154463851,
83.321408421468));
#69115=CARTESIAN_POINT('Ctrl Pts',(-5.11253250136785,-6.14689385231929,
83.5862443709747));
#69116=CARTESIAN_POINT('Ctrl Pts',(2.40704070040914,-7.62353003013413,83.9040475103822));
#69117=CARTESIAN_POINT('Ctrl Pts',(7.70573862108322,-2.10774641143824,84.22185064979));
#69118=CARTESIAN_POINT('Ctrl Pts',(5.95214038320305,5.3370478660503,84.5396537891976));
#69119=CARTESIAN_POINT('Ctrl Pts',(-1.27212963488989,7.89328694311642,84.8574569286053));
#69120=CARTESIAN_POINT('Ctrl Pts',(-6.30063152404268,3.98791539454707,85.1222928781117));
#69121=CARTESIAN_POINT('Ctrl Pts',(-7.00110202549445,-0.602432769133268,
85.3341616377169));
#69122=CARTESIAN_POINT('Ctrl Pts',(-5.52675146066759,-5.00564132632078,
85.5460303973217));
#69123=CARTESIAN_POINT('Ctrl Pts',(0.0949937285250582,-7.99457746023201,
85.8108663468282));
#69124=CARTESIAN_POINT('Ctrl Pts',(6.77638205776378,-4.24178043611775,86.128669486236));
#69125=CARTESIAN_POINT('Ctrl Pts',(7.23239620387072,3.3931471801692,86.4464726256435));
#69126=CARTESIAN_POINT('Ctrl Pts',(1.06931742661586,7.92266465920051,86.7642757650515));
#69127=CARTESIAN_POINT('Ctrl Pts',(-6.08746355568148,5.18315348356572,87.0820789044588));
#69128=CARTESIAN_POINT('Ctrl Pts',(-7.38223472031762,-1.05073180702098,
87.3469148539655));
#69129=CARTESIAN_POINT('Ctrl Pts',(-4.93837134276466,-4.99908424546743,
87.5587836135705));
#69130=CARTESIAN_POINT('Ctrl Pts',(-0.960453185032206,-7.39452205862662,
87.7706523731756));
#69131=CARTESIAN_POINT('Ctrl Pts',(5.25714652777984,-6.02367852407476,88.0354883226819));
#69132=CARTESIAN_POINT('Ctrl Pts',(7.90900773253987,1.16604105742781,88.3532914620898));
#69133=CARTESIAN_POINT('Ctrl Pts',(3.30452450769246,7.27331564103845,88.6710946014972));
#69134=CARTESIAN_POINT('Ctrl Pts',(-4.32426133656494,6.72404781021609,88.9888977409051));
#69135=CARTESIAN_POINT('Ctrl Pts',(-7.99514135649253,-0.00269548719377464,
89.3067008803125));
#69136=CARTESIAN_POINT('Ctrl Pts',(-4.93773878372982,-5.58750055926678,
89.5715368298191));
#69137=CARTESIAN_POINT('Ctrl Pts',(-0.516844500241237,-7.00794025194897,
89.7834055894242));
#69138=CARTESIAN_POINT('Ctrl Pts',(4.06460226526468,-6.25143465305058,89.9952743490292));
#69139=CARTESIAN_POINT('Ctrl Pts',(7.90824129176649,-1.17559016972185,90.2601102985357));
#69140=CARTESIAN_POINT('Ctrl Pts',(5.26392294923123,6.0169070331474,90.5779134379432));
#69141=CARTESIAN_POINT('Ctrl Pts',(-2.20174200284272,7.6794097943158,90.8957165773511));
#69142=CARTESIAN_POINT('Ctrl Pts',(-7.65237148129207,2.31371255200161,91.2135197167587));
#69143=CARTESIAN_POINT('Ctrl Pts',(-6.0839672687083,-5.18725696772707,91.5313228561664));
#69144=CARTESIAN_POINT('Ctrl Pts',(-0.134748826979324,-7.45541880445244,
91.7961588056728));
#69145=CARTESIAN_POINT('Ctrl Pts',(4.15155134782528,-5.66947759662977,92.0080275652779));
#69146=CARTESIAN_POINT('Ctrl Pts',(7.14821436328194,-2.12237089424207,92.219896324883));
#69147=CARTESIAN_POINT('Ctrl Pts',(6.78199168547343,4.23401480324719,92.4847322743895));
#69148=CARTESIAN_POINT('Ctrl Pts',(0.1045433961659,7.99381797011292,92.8025354137969));
#69149=CARTESIAN_POINT('Ctrl Pts',(-6.65635398585283,4.41746015840961,93.1203385532049));
#69150=CARTESIAN_POINT('Ctrl Pts',(-7.32535259445545,-3.2017595830866,93.4381416926121));
#69151=CARTESIAN_POINT('Ctrl Pts',(-1.26680705031046,-7.89414292201699,
93.7559448320203));
#69152=CARTESIAN_POINT('Ctrl Pts',(4.73260344551426,-5.76228178967871,94.0207807815264));
#69153=CARTESIAN_POINT('Ctrl Pts',(6.83697291209494,-1.62300838309489,94.2326495411316));
#69154=CARTESIAN_POINT('Ctrl Pts',(6.81750635060592,3.02043605388431,94.4445183007367));
#69155=CARTESIAN_POINT('Ctrl Pts',(2.41634697636828,7.62125710534312,94.7093542502432));
#69156=CARTESIAN_POINT('Ctrl Pts',(-5.10477095205658,6.15250912945454,95.0271573896507));
#69157=CARTESIAN_POINT('Ctrl Pts',(-7.931581283013,-0.954474194032004,95.3449605290586));
#69158=CARTESIAN_POINT('Ctrl Pts',(-3.49940412743684,-7.18792221812814,
95.662763668466));
#69159=CARTESIAN_POINT('Ctrl Pts',(4.15543921733351,-6.83041854405671,95.9805668078738));
#69160=CARTESIAN_POINT('Ctrl Pts',(7.33944388963318,-1.31681061169869,96.2454027573801));
#69161=CARTESIAN_POINT('Ctrl Pts',(6.25673777894657,3.19868522643596,96.4572715169854));
#69162=CARTESIAN_POINT('Ctrl Pts',(3.23043977694139,6.72054206472292,96.6691402765903));
#69163=CARTESIAN_POINT('Ctrl Pts',(-3.10345759092554,7.36823205099255,96.933976226097));
#69164=CARTESIAN_POINT('Ctrl Pts',(-7.87580893693733,1.37247537312704,97.2517793655042));
#69165=CARTESIAN_POINT('Ctrl Pts',(-5.41831594300546,-5.87050721640711,
97.5695825049123));
#69166=CARTESIAN_POINT('Ctrl Pts',(1.9980227369176,-7.74079842159345,97.8873856443198));
#69167=CARTESIAN_POINT('Ctrl Pts',(7.59285417362454,-2.50416814012545,98.2051887837274));
#69168=CARTESIAN_POINT('Ctrl Pts',(6.44062409468572,3.75763064538146,98.4700247332341));
#69169=CARTESIAN_POINT('Ctrl Pts',(2.68799327264257,6.49253779184573,98.6818934928389));
#69170=CARTESIAN_POINT('Ctrl Pts',(-1.89963529314591,7.21060417365909,98.8937622524443));
#69171=CARTESIAN_POINT('Ctrl Pts',(-7.14090626808129,3.59579619089075,99.1585982019505));
#69172=CARTESIAN_POINT('Ctrl Pts',(-6.88499375475416,-4.06311654496619,
99.4764013413583));
#69173=CARTESIAN_POINT('Ctrl Pts',(-0.317010548502199,-7.98251257113032,
99.7942044807658));
#69174=CARTESIAN_POINT('Ctrl Pts',(6.54110088345483,-4.59630876828881,100.112007620174));
#69175=CARTESIAN_POINT('Ctrl Pts',(7.40356833653495,3.01818960010868,100.429810759582));
#69176=CARTESIAN_POINT('Ctrl Pts',(2.46546225761111,7.03725249315749,100.694646709088));
#69177=CARTESIAN_POINT('Ctrl Pts',(-2.16466201497952,6.68525191546445,100.906515468693));
#69178=CARTESIAN_POINT('Ctrl Pts',(-6.12235607099368,4.25654589263679,101.118384228298));
#69179=CARTESIAN_POINT('Ctrl Pts',(-7.76752552118866,-1.89415940554908,
101.383220177805));
#69180=CARTESIAN_POINT('Ctrl Pts',(-2.60558488410996,-7.55797475999223,
101.701023317212));
#69181=CARTESIAN_POINT('Ctrl Pts',(4.93571384885182,-6.28169813333685,102.01882645662));
#69182=CARTESIAN_POINT('Ctrl Pts',(7.95984459380424,0.743592027571294,102.336629596027));
#69183=CARTESIAN_POINT('Ctrl Pts',(3.67799343791845,7.09891941400772,102.654432735435));
#69184=CARTESIAN_POINT('Ctrl Pts',(-2.68731918353641,6.95555478750277,102.919268684942));
#69185=CARTESIAN_POINT('Ctrl Pts',(-5.98337390429468,3.68477835611888,103.131137444547));
#69186=CARTESIAN_POINT('Ctrl Pts',(-7.42075443828335,-0.730636956945093,
103.343006204152));
#69187=CARTESIAN_POINT('Ctrl Pts',(-4.68401280993483,-6.4793762487074,103.607842153658));
#69188=CARTESIAN_POINT('Ctrl Pts',(2.9183726832874,-7.44279221411051,103.925645293066));
#69189=CARTESIAN_POINT('Ctrl Pts',(7.83091142925338,-1.5804520945932,104.243448432474));
#69190=CARTESIAN_POINT('Ctrl Pts',(5.57659579337766,5.72831863798309,104.561251571881));
#69191=CARTESIAN_POINT('Ctrl Pts',(-1.80436243058459,7.78887468091779,104.879054711289));
#69192=CARTESIAN_POINT('Ctrl Pts',(-6.55651181971887,3.55156015773956,105.143890660795));
#69193=CARTESIAN_POINT('Ctrl Pts',(-6.94414773901417,-1.07571696605596,
105.3557594204));
#69194=CARTESIAN_POINT('Ctrl Pts',(-5.1746548614019,-5.36883356619723,105.567628180006));
#69195=CARTESIAN_POINT('Ctrl Pts',(0.636802579013681,-7.96974121608161,
105.832464129512));
#69196=CARTESIAN_POINT('Ctrl Pts',(7.0483795328344,-3.77258545590462,106.15026726892));
#69197=CARTESIAN_POINT('Ctrl Pts',(6.98570098337924,3.87569147468288,106.468070408327));
#69198=CARTESIAN_POINT('Ctrl Pts',(0.529705109973643,7.97693346828529,106.785873547735));
#69199=CARTESIAN_POINT('Ctrl Pts',(-6.4248707633773,4.75850063043461,107.103676687143));
#69200=CARTESIAN_POINT('Ctrl Pts',(-7.29400903878353,-1.54882501861905,
107.368512636649));
#69201=CARTESIAN_POINT('Ctrl Pts',(-4.58807318727075,-5.32239976331763,
107.580381396254));
#69202=CARTESIAN_POINT('Ctrl Pts',(-0.456899111205659,-7.44262520877786,
107.792250155859));
#69203=CARTESIAN_POINT('Ctrl Pts',(5.65345139690404,-5.65338658494099,108.057086105366));
#69204=CARTESIAN_POINT('Ctrl Pts',(7.81175203655464,1.69958382563695,108.374889244773));
#69205=CARTESIAN_POINT('Ctrl Pts',(2.80379438617548,7.48062428385264,108.692692384181));
#69206=CARTESIAN_POINT('Ctrl Pts',(-4.77019740516966,6.41539334543834,109.010495523589));
#69207=CARTESIAN_POINT('Ctrl Pts',(-7.97656157879294,-0.544754950112174,
109.328298662996));
#69208=CARTESIAN_POINT('Ctrl Pts',(-4.54754781969298,-5.9094192289735,109.593134612503));
#69209=CARTESIAN_POINT('Ctrl Pts',(-0.0405211900412987,-7.02685654083492,
109.805003372108));
#69210=CARTESIAN_POINT('Ctrl Pts',(4.47909293475132,-5.9614724085595,110.016872131713));
#69211=CARTESIAN_POINT('Ctrl Pts',(7.96974851599409,-0.636711212212364,
110.281708081219));
#69212=CARTESIAN_POINT('Ctrl Pts',(4.84386793230822,6.3599527132942,110.599511220627));
#69213=CARTESIAN_POINT('Ctrl Pts',(-2.71733499765062,7.51246252214666,110.917314360035));
#69214=CARTESIAN_POINT('Ctrl Pts',(-7.79163146585404,1.78956256143654,111.235117499442));
#69215=CARTESIAN_POINT('Ctrl Pts',(-5.71827507280204,-5.58781019431744,
111.55292063885));
#69216=CARTESIAN_POINT('Ctrl Pts',(0.37103404184402,-7.44739958213263,111.817756588356));
#69217=CARTESIAN_POINT('Ctrl Pts',(4.52638561484153,-5.37495935594604,112.029625347962));
#69218=CARTESIAN_POINT('Ctrl Pts',(7.27566157962207,-1.63284272817919,112.241494107567));
#69219=CARTESIAN_POINT('Ctrl Pts',(6.47932254979134,4.68408709053455,112.506330057073));
#69220=CARTESIAN_POINT('Ctrl Pts',(-0.437673101391219,7.98251196787706,
112.824133196481));
#69221=CARTESIAN_POINT('Ctrl Pts',(-6.94053862569258,3.95599876407772,113.141936335888));
#69222=CARTESIAN_POINT('Ctrl Pts',(-7.09141944026156,-3.69104665146115,
113.459739475296));
#69223=CARTESIAN_POINT('Ctrl Pts',(-0.728674061214709,-7.96186703534172,
113.777542614704));
#69224=CARTESIAN_POINT('Ctrl Pts',(5.11239276394556,-5.42815502941039,114.04237856421));
#69225=CARTESIAN_POINT('Ctrl Pts',(6.93127983195271,-1.15573124189053,114.254247323815));
#69226=CARTESIAN_POINT('Ctrl Pts',(6.59703538737303,3.47570868944796,114.46611608342));
#69227=CARTESIAN_POINT('Ctrl Pts',(1.89407035690759,7.7675472357129,114.730952032927));
#69228=CARTESIAN_POINT('Ctrl Pts',(-5.51016107707595,5.79225171808505,115.048755172334));
#69229=CARTESIAN_POINT('Ctrl Pts',(-7.84861774789,-1.49003425585493,115.366558311742));
#69230=CARTESIAN_POINT('Ctrl Pts',(-3.00401520445511,-7.40864007172603,
115.68436145115));
#69231=CARTESIAN_POINT('Ctrl Pts',(4.60897562027904,-6.53296535331549,116.002164590558));
#69232=CARTESIAN_POINT('Ctrl Pts',(7.41183459035819,-0.816170816266582,
116.267000540064));
#69233=CARTESIAN_POINT('Ctrl Pts',(6.02547197434124,3.61552794191181,116.478869299669));
#69234=CARTESIAN_POINT('Ctrl Pts',(2.76735783469423,6.92409975454661,116.690738059274));
#69235=CARTESIAN_POINT('Ctrl Pts',(-3.595878055479,7.14086504466174,116.95557400878));
#69236=CARTESIAN_POINT('Ctrl Pts',(-7.95073948451101,0.835342271419291,
117.273377148188));
#69237=CARTESIAN_POINT('Ctrl Pts',(-5.00783148135237,-6.2243575162816,117.591180287596));
#69238=CARTESIAN_POINT('Ctrl Pts',(2.51824660614424,-7.58752193351855,117.908983427003));
#69239=CARTESIAN_POINT('Ctrl Pts',(7.74516388074322,-1.98361514321149,118.226786566411));
#69240=CARTESIAN_POINT('Ctrl Pts',(6.17103900741412,4.185654592191,118.491622515917));
#69241=CARTESIAN_POINT('Ctrl Pts',(2.24161806314621,6.65984258607461,118.703491275523));
#69242=CARTESIAN_POINT('Ctrl Pts',(-2.38413871057332,7.06521828430672,118.915360035128));
#69243=CARTESIAN_POINT('Ctrl Pts',(-7.36826762918714,3.10337311978758,119.180195984634));
#69244=CARTESIAN_POINT('Ctrl Pts',(-6.59367440544241,-4.52056555045889,
119.497999124042));
#69245=CARTESIAN_POINT('Ctrl Pts',(0.224928342326,-7.98563772512462,119.81580226345));
#69246=CARTESIAN_POINT('Ctrl Pts',(6.83767654936024,-4.14224992815635,120.133605402857));
#69247=CARTESIAN_POINT('Ctrl Pts',(7.1819011378248,3.51320204691645,120.451408542265));
#69248=CARTESIAN_POINT('Ctrl Pts',(1.98266777605119,7.188216418971,120.716244491771));
#69249=CARTESIAN_POINT('Ctrl Pts',(-2.61293703921732,6.52310622643868,120.928113251376));
#69250=CARTESIAN_POINT('Ctrl Pts',(-6.39685956550806,3.83165949626573,121.139982010982));
#69251=CARTESIAN_POINT('Ctrl Pts',(-7.62122940334152,-2.41643434787499,
121.404817960488));
#69252=CARTESIAN_POINT('Ctrl Pts',(-2.08716332745305,-7.71724071838623,
121.722621099896));
#69253=CARTESIAN_POINT('Ctrl Pts',(5.35025191358701,-5.93260542234808,122.040424239303));
#69254=CARTESIAN_POINT('Ctrl Pts',(7.89111370522805,1.28155356975195,122.358227378711));
#69255=CARTESIAN_POINT('Ctrl Pts',(3.18822791171694,7.33195031072198,122.676030518119));
#69256=CARTESIAN_POINT('Ctrl Pts',(-3.15271792865614,6.75735129014959,122.940866467625));
#69257=CARTESIAN_POINT('Ctrl Pts',(-6.21943171311898,3.27063051691363,123.15273522723));
#69258=CARTESIAN_POINT('Ctrl Pts',(-7.35414235580032,-1.23207832818336,
123.364603986835));
#69259=CARTESIAN_POINT('Ctrl Pts',(-4.23393705281535,-6.78204022464807,
123.629439936342));
#69260=CARTESIAN_POINT('Ctrl Pts',(3.41627416614999,-7.22780228580432,123.947243075749));
#69261=CARTESIAN_POINT('Ctrl Pts',(7.92004598091047,-1.04588445651475,124.265046215157));
#69262=CARTESIAN_POINT('Ctrl Pts',(5.17538742387095,6.09322739390386,124.582849354565));
#69263=CARTESIAN_POINT('Ctrl Pts',(-2.32829145794874,7.64861761776532,124.900652493972));
#69264=CARTESIAN_POINT('Ctrl Pts',(-6.78221871160612,3.09886045895844,125.165488443479));
#69265=CARTESIAN_POINT('Ctrl Pts',(-6.85523612844846,-1.5440506583436,125.377357203084));
#69266=CARTESIAN_POINT('Ctrl Pts',(-4.79874423499827,-5.70731815857739,
125.589225962689));
#69267=CARTESIAN_POINT('Ctrl Pts',(1.17568083135626,-7.90822781403826,125.854061912195));
#69268=CARTESIAN_POINT('Ctrl Pts',(7.28794000373724,-3.28602884389481,126.171865051603));
#69269=CARTESIAN_POINT('Ctrl Pts',(6.70685720861144,4.34039963821441,126.489668191011));
#69270=CARTESIAN_POINT('Ctrl Pts',(-0.0123449367553314,7.99449202035492,
126.807471330418));
#69271=CARTESIAN_POINT('Ctrl Pts',(-6.73271038624204,4.3119489133031,127.125274469826));
#69272=CARTESIAN_POINT('Ctrl Pts',(-7.17221595348917,-2.03979045803012,
127.390110419332));
#69273=CARTESIAN_POINT('Ctrl Pts',(-4.21666048361343,-5.62122132443205,
127.601979178938));
#69274=CARTESIAN_POINT('Ctrl Pts',(0.0487576357682374,-7.45647701593123,
127.813847938542));
#69275=CARTESIAN_POINT('Ctrl Pts',(6.02373879269242,-5.25707747073975,128.078683888049));
#69276=CARTESIAN_POINT('Ctrl Pts',(7.67854625697508,2.2253050218961,128.396487027457));
#69277=CARTESIAN_POINT('Ctrl Pts',(2.29016105906626,7.65350670997627,128.714290166864));
#69278=CARTESIAN_POINT('Ctrl Pts',(-5.19418078061711,6.07721491139238,129.032093306272));
#69279=CARTESIAN_POINT('Ctrl Pts',(-7.92127325553131,-1.08430742280561,
129.34989644568));
#69280=CARTESIAN_POINT('Ctrl Pts',(-4.13642880731286,-6.2041424482509,129.614732395186));
#69281=CARTESIAN_POINT('Ctrl Pts',(0.4359886007537,-7.01343487546074,129.826601154791));
#69282=CARTESIAN_POINT('Ctrl Pts',(4.87297058878657,-5.64407516223672,130.038469914396));
#69283=CARTESIAN_POINT('Ctrl Pts',(7.99457854872422,-0.0949020770426225,
130.303305863903));
#69284=CARTESIAN_POINT('Ctrl Pts',(4.40152118668289,6.67372956480586,130.62110900331));
#69285=CARTESIAN_POINT('Ctrl Pts',(-3.2204226774074,7.31094251208114,130.938912142718));
#69286=CARTESIAN_POINT('Ctrl Pts',(-7.89503396272016,1.25717691216364,131.256715282126));
#69287=CARTESIAN_POINT('Ctrl Pts',(-5.32626708167825,-5.96264803175383,
131.574518421534));
#69288=CARTESIAN_POINT('Ctrl Pts',(0.875109392973854,-7.40510704490388,
131.83935437104));
#69289=CARTESIAN_POINT('Ctrl Pts',(4.8803892230668,-5.05570527658503,132.051223130645));
#69290=CARTESIAN_POINT('Ctrl Pts',(7.36962582815063,-1.13580013612054,132.26309189025));
#69291=CARTESIAN_POINT('Ctrl Pts',(6.1468352393629,5.11260296875023,132.527927839757));
#69292=CARTESIAN_POINT('Ctrl Pts',(-0.977875404884448,7.93447003608332,
132.845730979164));
#69293=CARTESIAN_POINT('Ctrl Pts',(-7.19278255074581,3.47633166050105,133.163534118572));
#69294=CARTESIAN_POINT('Ctrl Pts',(-6.82485121003244,-4.16334733380493,
133.481337257979));
#69295=CARTESIAN_POINT('Ctrl Pts',(-0.187187676710187,-7.99295022814698,
133.799140397387));
#69296=CARTESIAN_POINT('Ctrl Pts',(5.46865458862486,-5.06904762124686,134.063976346893));
#69297=CARTESIAN_POINT('Ctrl Pts',(6.99368864646755,-0.68313536622519,134.275845106499));
#69298=CARTESIAN_POINT('Ctrl Pts',(6.34620452887703,3.91498593532799,134.487713866104));
#69299=CARTESIAN_POINT('Ctrl Pts',(1.36307712850379,7.87809071524929,134.75254981561));
#69300=CARTESIAN_POINT('Ctrl Pts',(-5.89019315816176,5.40533806718196,135.070352955018));
#69301=CARTESIAN_POINT('Ctrl Pts',(-7.72953447127796,-2.01873710359743,
135.388156094426));
#69302=CARTESIAN_POINT('Ctrl Pts',(-2.4948016494047,-7.59526298367014,135.705959233833));
#69303=CARTESIAN_POINT('Ctrl Pts',(5.04130128099164,-6.20544712089461,136.023762373241));
#69304=CARTESIAN_POINT('Ctrl Pts',(7.450115648091,-0.311774960870602,136.288598322747));
#69305=CARTESIAN_POINT('Ctrl Pts',(5.76647663861923,4.01573181233197,136.500467082352));
#69306=CARTESIAN_POINT('Ctrl Pts',(2.29154036973368,7.09579238211189,136.712335841958));
#69307=CARTESIAN_POINT('Ctrl Pts',(-4.0717501047619,6.88063541108804,136.977171791464));
#69308=CARTESIAN_POINT('Ctrl Pts',(-7.98908032112504,0.294364881727811,
137.294974930872));
#69309=CARTESIAN_POINT('Ctrl Pts',(-4.57430072233384,-6.54956300357293,
137.612778070279));
#69310=CARTESIAN_POINT('Ctrl Pts',(3.02688137531002,-7.39932728028593,137.930581209687));
#69311=CARTESIAN_POINT('Ctrl Pts',(7.8618299463764,-1.45393344765422,138.248384349095));
#69312=CARTESIAN_POINT('Ctrl Pts',(5.87305448207229,4.59441594185449,138.513220298601));
#69313=CARTESIAN_POINT('Ctrl Pts',(1.78492681233391,6.79649844309022,138.725089058206));
#69314=CARTESIAN_POINT('Ctrl Pts',(-2.85767019935493,6.88731789798286,138.936957817811));
#69315=CARTESIAN_POINT('Ctrl Pts',(-7.56171984469098,2.59666816639205,139.201793767318));
#69316=CARTESIAN_POINT('Ctrl Pts',(-6.27201062827867,-4.95721068139547,
139.519596906725));
#69317=CARTESIAN_POINT('Ctrl Pts',(0.765832101384861,-7.95201256466585,
139.837400046133));
#69318=CARTESIAN_POINT('Ctrl Pts',(7.10278487703089,-3.66912824136791,140.155203185541));
#69319=CARTESIAN_POINT('Ctrl Pts',(6.92718246166577,3.99204655768657,140.473006324948));
#69320=CARTESIAN_POINT('Ctrl Pts',(1.49074895568024,7.30609980408792,140.737842274455));
#69321=CARTESIAN_POINT('Ctrl Pts',(-3.04918719316388,6.33094086794075,140.94971103406));
#69322=CARTESIAN_POINT('Ctrl Pts',(-6.64192438416009,3.38913960633895,141.161579793665));
#69323=CARTESIAN_POINT('Ctrl Pts',(-7.43985999683126,-2.92758873537547,
141.426415743171));
#69324=CARTESIAN_POINT('Ctrl Pts',(-1.55913653809718,-7.8409915391201,141.744218882579));
#69325=CARTESIAN_POINT('Ctrl Pts',(5.74016784456189,-5.55621055687876,142.062022021987));
#69326=CARTESIAN_POINT('Ctrl Pts',(7.78606750658739,1.8136173366639,142.379825161394));
#69327=CARTESIAN_POINT('Ctrl Pts',(2.68378999711791,7.53123919599689,142.697628300802));
#69328=CARTESIAN_POINT('Ctrl Pts',(-3.60360770414117,6.52805011552451,142.962464250308));
#69329=CARTESIAN_POINT('Ctrl Pts',(-6.42686737815966,2.84143106829594,143.174333009914));
#69330=CARTESIAN_POINT('Ctrl Pts',(-7.25368613294617,-1.72784961175433,
143.386201769518));
#69331=CARTESIAN_POINT('Ctrl Pts',(-3.76437650019324,-7.05349290357036,
143.651037719025));
#69332=CARTESIAN_POINT('Ctrl Pts',(3.89845378006065,-6.97954964061808,143.968840858433));
#69333=CARTESIAN_POINT('Ctrl Pts',(7.97273207467384,-0.506503604505183,
144.28664399784));
#69334=CARTESIAN_POINT('Ctrl Pts',(4.75036165597909,6.43009480476973,144.604447137248));
#69335=CARTESIAN_POINT('Ctrl Pts',(-2.84150556863367,7.47316122402503,144.922250276656));
#69336=CARTESIAN_POINT('Ctrl Pts',(-6.97671348499278,2.63189964530712,145.187086226162));
#69337=CARTESIAN_POINT('Ctrl Pts',(-6.73477636967082,-2.00527855019573,
145.398954985767));
#69338=CARTESIAN_POINT('Ctrl Pts',(-4.40074954120288,-6.01953738026474,
145.610823745372));
#69339=CARTESIAN_POINT('Ctrl Pts',(1.70914853965251,-7.81032034140677,145.875659694879));
#69340=CARTESIAN_POINT('Ctrl Pts',(7.49396100181569,-2.78434975944821,146.193462834286));
#69341=CARTESIAN_POINT('Ctrl Pts',(6.3971481312346,4.78513306154618,146.511265973694));
#69342=CARTESIAN_POINT('Ctrl Pts',(-0.554338168251488,7.97525950704822,
146.829069113102));
#69343=CARTESIAN_POINT('Ctrl Pts',(-7.00956573689031,3.8455533920382,147.146872252509));
#69344=CARTESIAN_POINT('Ctrl Pts',(-7.01741595136444,-2.52136868752679,
147.411708202016));
#69345=CARTESIAN_POINT('Ctrl Pts',(-3.82584250692092,-5.89417372276192,
147.623576961621));
#69346=CARTESIAN_POINT('Ctrl Pts',(0.55419003366898,-7.43601376719139,147.835445721226));
#69347=CARTESIAN_POINT('Ctrl Pts',(6.36630455696223,-4.83657494449871,148.100281670732));
#69348=CARTESIAN_POINT('Ctrl Pts',(7.51000354215738,2.74078512973372,148.41808481014));
#69349=CARTESIAN_POINT('Ctrl Pts',(1.7659880582776,7.79116752605513,148.735887949548));
#69350=CARTESIAN_POINT('Ctrl Pts',(-5.59425982480493,5.71106840529436,149.053691088956));
#69351=CARTESIAN_POINT('Ctrl Pts',(-7.8295317091046,-1.61886902913507,149.371494228363));
#69352=CARTESIAN_POINT('Ctrl Pts',(-3.7062721951118,-6.47031533238849,149.63633017787));
#69353=CARTESIAN_POINT('Ctrl Pts',(0.910489890705346,-6.96773509170653,
149.848198937475));
#69354=CARTESIAN_POINT('Ctrl Pts',(5.24442759497008,-5.30070829453768,150.06006769708));
#69355=CARTESIAN_POINT('Ctrl Pts',(7.98260647573363,0.447353787642963,150.324903646586));
#69356=CARTESIAN_POINT('Ctrl Pts',(3.93893627769698,6.95677681484015,150.642706785994));
#69357=CARTESIAN_POINT('Ctrl Pts',(-3.70872246877002,7.07580780692477,150.960509925402));
#69358=CARTESIAN_POINT('Ctrl Pts',(-7.96204128017202,0.718947674609458,
151.278313064809));
#69359=CARTESIAN_POINT('Ctrl Pts',(-4.9098700165443,-6.30993038124958,151.596116204217));
#69360=CARTESIAN_POINT('Ctrl Pts',(1.37537179497646,-7.32893688752285,151.860952153723));
#69361=CARTESIAN_POINT('Ctrl Pts',(5.21164686859631,-4.71291616050793,152.072820913328));
#69362=CARTESIAN_POINT('Ctrl Pts',(7.43037142212706,-0.634184061999188,
152.284689672933));
#69363=CARTESIAN_POINT('Ctrl Pts',(5.78457976779752,5.51897844456597,152.54952562244));
#69364=CARTESIAN_POINT('Ctrl Pts',(-1.51109102684477,7.84758283547285,152.867328761848));
#69365=CARTESIAN_POINT('Ctrl Pts',(-7.41649337492981,2.98493712464134,153.185131901255));
#69366=CARTESIAN_POINT('Ctrl Pts',(-6.51804811713408,-4.62465064531089,
153.502935040663));
#69367=CARTESIAN_POINT('Ctrl Pts',(-0.806194770464466,-7.41282170326391,
153.767770990169));
#69368=CARTESIAN_POINT('Ctrl Pts',(3.64156398367868,-6.01849203715341,153.979643190462));
#69369=CARTESIAN_POINT('Ctrl Pts',(5.26965269452346,-4.3811448078825,154.085581010954));
#69370=CARTESIAN_POINT('Ctrl Pts',(5.83708131225798,-3.40978216080788,154.138551641544));
#69371=CARTESIAN_POINT('Ctrl Pts',(3.43101696651027,7.14016450787011,1.65822217068623E-14));
#69372=CARTESIAN_POINT('Ctrl Pts',(3.61003597782292,7.03974453288905,1.31692278925585E-14));
#69373=CARTESIAN_POINT('Ctrl Pts',(3.78453304467846,6.93211991481877,1.59736015986178E-14));
#69374=CARTESIAN_POINT('Ctrl Pts',(3.95400783053005,6.81726961947616,1.53627111032506E-14));
#69375=CARTESIAN_POINT('Ctrl Pts',(4.12383106727608,6.70218318465156,1.45970944988586E-14));
#69376=CARTESIAN_POINT('Ctrl Pts',(4.28861172272689,6.57984074250072,1.20659957845407E-14));
#69377=CARTESIAN_POINT('Ctrl Pts',(4.44814243011172,6.45071609426073,1.22124532708767E-14));
#69378=CARTESIAN_POINT('Ctrl Pts',(4.60928369061434,6.32028785934319,1.23603893287374E-14));
#69379=CARTESIAN_POINT('Ctrl Pts',(4.76506884842713,6.18293913020302,1.03995638427172E-14));
#69380=CARTESIAN_POINT('Ctrl Pts',(4.91524218627338,6.03912581706056,1.29757316003065E-14));
#69381=CARTESIAN_POINT('Ctrl Pts',(4.96008620607599,5.99618099639577,1.37450140814249E-14));
#69382=CARTESIAN_POINT('Ctrl Pts',(5.00442975271524,5.95265929902808,1.55276531095038E-14));
#69383=CARTESIAN_POINT('Ctrl Pts',(5.04826448447757,5.90857319066696,1.45022882591661E-14));
#69384=CARTESIAN_POINT('Ctrl Pts',(5.07244303315987,5.88425598660599,1.39367131329073E-14));
#69385=CARTESIAN_POINT('Ctrl Pts',(5.09646351320685,5.85977024716788,1.48017877861931E-14));
#69386=CARTESIAN_POINT('Ctrl Pts',(5.1203146633298,5.83512874369868,1.43218770176645E-14));
#69387=CARTESIAN_POINT('Ctrl Pts',(5.26273479984385,5.6879892443495,1.14562308406016E-14));
#69388=CARTESIAN_POINT('Ctrl Pts',(5.39923071701932,5.53518844907465,1.30927522722923E-14));
#69389=CARTESIAN_POINT('Ctrl Pts',(5.52960032490143,5.37719968636751,1.25732757538799E-14));
#69390=CARTESIAN_POINT('Ctrl Pts',(5.66063860884131,5.21840058676716,1.20511347992075E-14));
#69391=CARTESIAN_POINT('Ctrl Pts',(5.78548791527577,5.05435946905415,8.76473059902014E-15));
#69392=CARTESIAN_POINT('Ctrl Pts',(5.90389832912926,4.88552923085758,7.13318293321663E-15));
#69393=CARTESIAN_POINT('Ctrl Pts',(6.02173466768101,4.71751751247513,5.50954530832999E-15));
#69394=CARTESIAN_POINT('Ctrl Pts',(6.13319465726933,4.54476228664395,7.19754582327447E-15));
#69395=CARTESIAN_POINT('Ctrl Pts',(6.23798347774738,4.36769307789513,6.16173778666962E-15));
#69396=CARTESIAN_POINT('Ctrl Pts',(6.25387388903657,4.34084190674124,6.00466553751931E-15));
#69397=CARTESIAN_POINT('Ctrl Pts',(6.26961079874451,4.31389151400701,5.35714192551716E-15));
#69398=CARTESIAN_POINT('Ctrl Pts',(6.28519307487105,4.28684337930822,5.57887069874141E-15));
#69399=CARTESIAN_POINT('Ctrl Pts',(6.29843934789536,4.26385014172799,5.0289415732972E-15));
#69400=CARTESIAN_POINT('Ctrl Pts',(6.31156974583608,4.24079340614484,7.2115050195674E-15));
#69401=CARTESIAN_POINT('Ctrl Pts',(6.3245813935981,4.21767852568033,7.16093850883226E-15));
#69402=CARTESIAN_POINT('Ctrl Pts',(6.42415862933386,4.04078195246255,6.90070714083338E-15));
#69403=CARTESIAN_POINT('Ctrl Pts',(6.51683135396108,3.860401258507,4.02818541900997E-15));
#69404=CARTESIAN_POINT('Ctrl Pts',(6.60240201838025,3.67698384153671,4.10782519111308E-15));
#69405=CARTESIAN_POINT('Ctrl Pts',(6.68774671377467,3.4940507804507,3.96951696376866E-15));
#69406=CARTESIAN_POINT('Ctrl Pts',(6.76602705909268,3.30809630596838,2.71533609189988E-15));
#69407=CARTESIAN_POINT('Ctrl Pts',(6.83699907130241,3.11954532599916,1.58206781009085E-15));
#69408=CARTESIAN_POINT('Ctrl Pts',(6.90718750333259,2.93307607946455,8.69852090214781E-16));
#69409=CARTESIAN_POINT('Ctrl Pts',(6.97022825956894,2.7440666764262,-1.05615630689871E-15));
#69410=CARTESIAN_POINT('Ctrl Pts',(7.025835331104,2.55291979031694,-2.1094237467878E-15));
#69411=CARTESIAN_POINT('Ctrl Pts',(7.07793698356765,2.37382262956653,-3.46212101854286E-15));
#69412=CARTESIAN_POINT('Ctrl Pts',(7.12351236716729,2.19284848651913,-2.88434274368081E-15));
#69413=CARTESIAN_POINT('Ctrl Pts',(7.16228352934668,2.01032949625264,-4.38538094726937E-15));
#69414=CARTESIAN_POINT('Ctrl Pts',(7.19136190098122,1.87344025355278,-5.55485411509882E-15));
#69415=CARTESIAN_POINT('Ctrl Pts',(7.21661206831502,1.73568201351242,-6.23233312377065E-15));
#69416=CARTESIAN_POINT('Ctrl Pts',(7.23790051720632,1.597197609874,-5.99520433297585E-15));
#69417=CARTESIAN_POINT('Ctrl Pts',(7.24390133298475,1.55816144530123,-6.56938230126875E-15));
#69418=CARTESIAN_POINT('Ctrl Pts',(7.24958816967185,1.51906011540194,-6.87988353579413E-15));
#69419=CARTESIAN_POINT('Ctrl Pts',(7.25495188924773,1.47994306170205,-6.32827124036339E-15));
#69420=CARTESIAN_POINT('Ctrl Pts',(7.28130928311069,1.28772130652989,-3.61764061834054E-15));
#69421=CARTESIAN_POINT('Ctrl Pts',(7.29990057069104,1.09492930404099,-4.9161174975687E-15));
#69422=CARTESIAN_POINT('Ctrl Pts',(7.31049892499678,0.901945400796462,-5.38458166943201E-15));
#69423=CARTESIAN_POINT('Ctrl Pts',(7.32069773744585,0.716236697529725,-5.83538545369078E-15));
#69424=CARTESIAN_POINT('Ctrl Pts',(7.32349479503547,0.530349761762813,-8.49735146053655E-15));
#69425=CARTESIAN_POINT('Ctrl Pts',(7.3186423718122,0.34462194553665,-8.49320613838245E-15));
#69426=CARTESIAN_POINT('Ctrl Pts',(7.31355073209503,0.14973805306282,-8.40735269849132E-15));
#69427=CARTESIAN_POINT('Ctrl Pts',(7.30003679274451,-0.04497140859214,-8.72424650198269E-15));
#69428=CARTESIAN_POINT('Ctrl Pts',(7.27832783927718,-0.239012460972904,
-7.88258347483861E-15));
#69429=CARTESIAN_POINT('Ctrl Pts',(7.25659221464526,-0.433291908118023,
-7.33792831234507E-15));
#69430=CARTESIAN_POINT('Ctrl Pts',(7.22664105273108,-0.626902029575905,
-8.15483405442268E-15));
#69431=CARTESIAN_POINT('Ctrl Pts',(7.18865483465271,-0.81932603837647,-7.66053886991358E-15));
#69432=CARTESIAN_POINT('Ctrl Pts',(7.16907168253685,-0.918526980868588,
-7.92704640417113E-15));
#69433=CARTESIAN_POINT('Ctrl Pts',(7.14735227907707,-1.01741227644876,-6.68596638540915E-15));
#69434=CARTESIAN_POINT('Ctrl Pts',(7.12351690973822,-1.11590797526994,-8.38218383591993E-15));
#69435=CARTESIAN_POINT('Ctrl Pts',(7.11427622357686,-1.15409357365995,-8.33885810172723E-15));
#69436=CARTESIAN_POINT('Ctrl Pts',(7.10471747311699,-1.19222058884854,-8.36988889943339E-15));
#69437=CARTESIAN_POINT('Ctrl Pts',(7.09484172726625,-1.23028460780204,-8.10462807976364E-15));
#69438=CARTESIAN_POINT('Ctrl Pts',(7.08652641365314,-1.26233426357057,-7.88128019919228E-15));
#69439=CARTESIAN_POINT('Ctrl Pts',(7.0779855309813,-1.29434187629915,-5.88751111059832E-15));
#69440=CARTESIAN_POINT('Ctrl Pts',(7.06922855023602,-1.32627370263882,-5.55111512312578E-15));
#69441=CARTESIAN_POINT('Ctrl Pts',(7.01841803332525,-1.51155132850308,-3.59924900541043E-15));
#69442=CARTESIAN_POINT('Ctrl Pts',(6.96027727489818,-1.6945131914679,-6.19570876562944E-15));
#69443=CARTESIAN_POINT('Ctrl Pts',(6.89506241820436,-1.87470313308216,-4.6074255521944E-15));
#69444=CARTESIAN_POINT('Ctrl Pts',(6.82965550073751,-2.05542374241897,-3.01446477114324E-15));
#69445=CARTESIAN_POINT('Ctrl Pts',(6.75713237389037,-2.23335678785184,-2.31960625851253E-15));
#69446=CARTESIAN_POINT('Ctrl Pts',(6.6777034145667,-2.40802117644964,-2.22044604925031E-15));
#69447=CARTESIAN_POINT('Ctrl Pts',(6.5989855489093,-2.58112186911696,-2.12217357913706E-15));
#69448=CARTESIAN_POINT('Ctrl Pts',(6.51348450654554,-2.75101279163696,-4.30431460656709E-15));
#69449=CARTESIAN_POINT('Ctrl Pts',(6.42136423171764,-2.91719531413377,-2.33146835171283E-15));
#69450=CARTESIAN_POINT('Ctrl Pts',(6.39153541170114,-2.97100571106004,-1.69265484441239E-15));
#69451=CARTESIAN_POINT('Ctrl Pts',(6.36101228159959,-3.02442701025753,-1.86620021322499E-15));
#69452=CARTESIAN_POINT('Ctrl Pts',(6.32979959358533,-3.07744142707614,-1.4432899320127E-15));
#69453=CARTESIAN_POINT('Ctrl Pts',(6.25665722612945,-3.2016729560503,-9.6487752581363E-16));
#69454=CARTESIAN_POINT('Ctrl Pts',(6.17972892780882,-3.32367110683975,-8.91121715210751E-16));
#69455=CARTESIAN_POINT('Ctrl Pts',(6.09910488142111,-3.44327304576849,-3.33066907387547E-16));
#69456=CARTESIAN_POINT('Ctrl Pts',(6.06259861362104,-3.49742835807996,-9.66891900049288E-16));
#69457=CARTESIAN_POINT('Ctrl Pts',(6.02533449549714,-3.55109219988174,1.72414040061109E-15));
#69458=CARTESIAN_POINT('Ctrl Pts',(5.98732028987866,-3.60424847320198,0.));
#69459=CARTESIAN_POINT('Ctrl Pts',(5.96420424303597,-3.63657225543186,-1.89149828765009E-16));
#69460=CARTESIAN_POINT('Ctrl Pts',(5.94081130726099,-3.66870769301961,-2.08278402782922E-15));
#69461=CARTESIAN_POINT('Ctrl Pts',(5.91714166721159,-3.70065306896213,-7.7715611723761E-16));
#69462=CARTESIAN_POINT('Ctrl Pts',(5.89678246694326,-3.72813055932968,3.45866457342017E-16));
#69463=CARTESIAN_POINT('Ctrl Pts',(5.87621810525247,-3.75546774264844,2.65112159864947E-15));
#69464=CARTESIAN_POINT('Ctrl Pts',(5.85547020257177,-3.7826359155115,2.22044604925031E-15));
#69465=CARTESIAN_POINT('Ctrl Pts',(5.74169178169016,-3.93162214579068,-1.41314783979673E-16));
#69466=CARTESIAN_POINT('Ctrl Pts',(5.62227441123033,-4.07569710199864,-3.93788939876355E-16));
#69467=CARTESIAN_POINT('Ctrl Pts',(5.49748908512713,-4.21457279958388,3.33066907387547E-16));
#69468=CARTESIAN_POINT('Ctrl Pts',(5.37305505713184,-4.35305753156988,1.05787649575351E-15));
#69469=CARTESIAN_POINT('Ctrl Pts',(5.24328275729723,-4.48637266644393,6.27024174355871E-16));
#69470=CARTESIAN_POINT('Ctrl Pts',(5.10840575685314,-4.61419509848205,2.22044604925031E-16));
#69471=CARTESIAN_POINT('Ctrl Pts',(4.97464552680793,-4.74095917136371,-1.79581767194132E-16));
#69472=CARTESIAN_POINT('Ctrl Pts',(4.83586429127236,-4.8623214916972,1.92427926616426E-15));
#69473=CARTESIAN_POINT('Ctrl Pts',(4.69226263119319,-4.97792406018082,-3.33066907387547E-16));
#69474=CARTESIAN_POINT('Ctrl Pts',(4.55148028125308,-5.09125702054677,-2.54609493760483E-15));
#69475=CARTESIAN_POINT('Ctrl Pts',(4.40606445652634,-5.19905441201978,1.48420063567409E-15));
#69476=CARTESIAN_POINT('Ctrl Pts',(4.25618497479233,-5.30093319600521,-3.33066907387547E-16));
#69477=CARTESIAN_POINT('Ctrl Pts',(4.14933403573732,-5.37356384306032,-1.62861944896186E-15));
#69478=CARTESIAN_POINT('Ctrl Pts',(4.04021406211686,-5.4431854630145,2.9443224414169E-15));
#69479=CARTESIAN_POINT('Ctrl Pts',(3.92888236737297,-5.50964357679762,-1.11022302462516E-16));
#69480=CARTESIAN_POINT('Ctrl Pts',(-2.92283340683968,6.09544329646178,-0.664547330701837));
#69481=CARTESIAN_POINT('Ctrl Pts',(-3.93854213988516,5.60840058998238,-0.611506103854861));
#69482=CARTESIAN_POINT('Ctrl Pts',(-5.7050272011839,4.11645562634411,-0.505426300633415));
#69483=CARTESIAN_POINT('Ctrl Pts',(-7.45550178091418,-0.210827257858674,
-0.293269344663029));
#69484=CARTESIAN_POINT('Ctrl Pts',(-5.12620949291362,-6.13604307561665,
-0.0280764627906812));
#69485=CARTESIAN_POINT('Ctrl Pts',(2.40255415416736,-7.62885674758421,0.290154995456135));
#69486=CARTESIAN_POINT('Ctrl Pts',(7.71325449472373,-2.10499323613276,0.608386453702953));
#69487=CARTESIAN_POINT('Ctrl Pts',(5.93871117578135,5.35810720449711,0.926617911949768));
#69488=CARTESIAN_POINT('Ctrl Pts',(-0.0856345739722672,7.4588348660275,
1.19181079382212));
#69489=CARTESIAN_POINT('Ctrl Pts',(-4.32158964384802,5.5412541473786,1.40396509932));
#69490=CARTESIAN_POINT('Ctrl Pts',(-7.21288526193602,1.89948635041438,1.61611940481787));
#69491=CARTESIAN_POINT('Ctrl Pts',(-6.64449808808741,-4.45309590180648,
1.88131228669022));
#69492=CARTESIAN_POINT('Ctrl Pts',(0.164673416110273,-7.99633117084599,
2.19954374493704));
#69493=CARTESIAN_POINT('Ctrl Pts',(6.80998385256597,-4.18360353937514,2.51777520318386));
#69494=CARTESIAN_POINT('Ctrl Pts',(7.20734006215933,3.46751732933175,2.83600666143067));
#69495=CARTESIAN_POINT('Ctrl Pts',(0.968699846707641,7.93984220175686,3.15423811967749));
#69496=CARTESIAN_POINT('Ctrl Pts',(-4.95436512982973,5.57535620991625,3.41943100154983));
#69497=CARTESIAN_POINT('Ctrl Pts',(-6.89665372451194,1.35030356582765,3.63158530704772));
#69498=CARTESIAN_POINT('Ctrl Pts',(-6.69115139650215,-3.29525832728733,
3.84373961254559));
#69499=CARTESIAN_POINT('Ctrl Pts',(-2.09715951672875,-7.71891001831387,
4.10893249441794));
#69500=CARTESIAN_POINT('Ctrl Pts',(5.36749476028327,-5.92954507333267,4.42716395266475));
#69501=CARTESIAN_POINT('Ctrl Pts',(7.88485451519108,1.30645067348062,4.74539541091158));
#69502=CARTESIAN_POINT('Ctrl Pts',(3.1682124011442,7.34383728681522,5.06362686915839));
#69503=CARTESIAN_POINT('Ctrl Pts',(-4.47465103507491,6.63001770779555,5.38185832740521));
#69504=CARTESIAN_POINT('Ctrl Pts',(-7.39638799231719,0.961079031362873,
5.64705120927755));
#69505=CARTESIAN_POINT('Ctrl Pts',(-6.09258682522784,-3.50250887814472,
5.85920551477544));
#69506=CARTESIAN_POINT('Ctrl Pts',(-2.89139378365477,-6.87532323477221,
6.0713598202733));
#69507=CARTESIAN_POINT('Ctrl Pts',(3.4777477733007,-7.20311800115464,6.33655270214567));
#69508=CARTESIAN_POINT('Ctrl Pts',(7.94055883120079,-0.957622040899968,
6.65478416039247));
#69509=CARTESIAN_POINT('Ctrl Pts',(5.09671433411442,6.15639866781965,6.97301561863929));
#69510=CARTESIAN_POINT('Ctrl Pts',(-2.42313748367644,7.62219911374143,7.2912470768861));
#69511=CARTESIAN_POINT('Ctrl Pts',(-7.72572038657178,2.07192733349136,7.60947853513293));
#69512=CARTESIAN_POINT('Ctrl Pts',(-6.21469165940851,-4.12405568382962,
7.87467141700526));
#69513=CARTESIAN_POINT('Ctrl Pts',(-2.30356798303852,-6.63933409733441,
8.08682572250317));
#69514=CARTESIAN_POINT('Ctrl Pts',(2.32494740867123,-7.08694907910043,8.29898002800102));
#69515=CARTESIAN_POINT('Ctrl Pts',(7.34879763468661,-3.15829252949285,8.56417290987339));
#69516=CARTESIAN_POINT('Ctrl Pts',(6.62329263599618,4.4834706682624,8.88240436812019));
#69517=CARTESIAN_POINT('Ctrl Pts',(-0.188466539193348,7.99013278561538,
9.20063582636702));
#69518=CARTESIAN_POINT('Ctrl Pts',(-6.82731609888302,4.16620564318667,9.51886728461381));
#69519=CARTESIAN_POINT('Ctrl Pts',(-7.19171590592274,-3.50126558618686,
9.83709874286067));
#69520=CARTESIAN_POINT('Ctrl Pts',(-1.98822215884615,-7.18868557884129,
10.102291624733));
#69521=CARTESIAN_POINT('Ctrl Pts',(2.61404138588895,-6.52334042805334,10.3144459302309));
#69522=CARTESIAN_POINT('Ctrl Pts',(6.40222362337669,-3.82645532845434,10.5266002357288));
#69523=CARTESIAN_POINT('Ctrl Pts',(7.61944006308874,2.43387992751043,10.7917931176011));
#69524=CARTESIAN_POINT('Ctrl Pts',(2.06106675097439,7.72796987722388,11.1100245758479));
#69525=CARTESIAN_POINT('Ctrl Pts',(-5.3813117170739,5.9092491716001,11.4282560340947));
#69526=CARTESIAN_POINT('Ctrl Pts',(-7.88657750684671,-1.33094320079776,
11.7464874923416));
#69527=CARTESIAN_POINT('Ctrl Pts',(-3.13426327320923,-7.35907821066942,
12.0647189505884));
#69528=CARTESIAN_POINT('Ctrl Pts',(3.21234000341252,-6.73135197466789,12.3299118324607));
#69529=CARTESIAN_POINT('Ctrl Pts',(6.25094954120617,-3.21135680681792,12.5420661379586));
#69530=CARTESIAN_POINT('Ctrl Pts',(7.34284882357209,1.30873941583336,12.7542204434565));
#69531=CARTESIAN_POINT('Ctrl Pts',(4.15707880260768,6.83361794406501,13.0194133253288));
#69532=CARTESIAN_POINT('Ctrl Pts',(-3.51094065617307,7.18629322280136,13.3376447835757));
#69533=CARTESIAN_POINT('Ctrl Pts',(-7.93768278073829,0.933238255080724,
13.6558762418225));
#69534=CARTESIAN_POINT('Ctrl Pts',(-5.08195617773027,-6.17602104780083,
13.9741077000693));
#69535=CARTESIAN_POINT('Ctrl Pts',(2.45876366208963,-7.61144661877917,14.2923391583161));
#69536=CARTESIAN_POINT('Ctrl Pts',(6.83907561365005,-2.97611700965661,14.5575320401884));
#69537=CARTESIAN_POINT('Ctrl Pts',(6.8253206198653,1.67397166745522,14.7696863456863));
#69538=CARTESIAN_POINT('Ctrl Pts',(4.68598109533263,5.80274149679056,14.9818406511842));
#69539=CARTESIAN_POINT('Ctrl Pts',(-1.34196630560764,7.88535128013655,15.2470335330566));
#69540=CARTESIAN_POINT('Ctrl Pts',(-7.36282764599865,3.12382516005102,15.5652649913034));
#69541=CARTESIAN_POINT('Ctrl Pts',(-6.60513302389061,-4.49999547834049,
15.8834964495502));
#69542=CARTESIAN_POINT('Ctrl Pts',(0.212475557574551,-7.9952716472102,16.201727907797));
#69543=CARTESIAN_POINT('Ctrl Pts',(6.84716483161442,-4.13472757811682,16.5199593660438));
#69544=CARTESIAN_POINT('Ctrl Pts',(7.11513265916595,2.23721142202968,16.7851522479161));
#69545=CARTESIAN_POINT('Ctrl Pts',(4.05575213852165,5.73916869400773,16.9973065534141));
#69546=CARTESIAN_POINT('Ctrl Pts',(-0.266696373551286,7.453797739993,17.2094608589119));
#69547=CARTESIAN_POINT('Ctrl Pts',(-6.1835398505895,5.07380264621208,17.4746537407843));
#69548=CARTESIAN_POINT('Ctrl Pts',(-7.60743345297728,-2.46910324485873,
17.7928851990311));
#69549=CARTESIAN_POINT('Ctrl Pts',(-2.03652054591839,-7.7285396831761,18.1111166572779));
#69550=CARTESIAN_POINT('Ctrl Pts',(5.40280882453206,-5.89738682645189,18.4293481155248));
#69551=CARTESIAN_POINT('Ctrl Pts',(7.8809242737375,1.36772474136872,18.7475795737715));
#69552=CARTESIAN_POINT('Ctrl Pts',(3.90526209794003,6.35445950894199,19.0127724556439));
#69553=CARTESIAN_POINT('Ctrl Pts',(-0.70085706616846,6.99256620134576,19.2249267611418));
#69554=CARTESIAN_POINT('Ctrl Pts',(-5.08871088845878,5.45300368586626,19.4370810666396));
#69555=CARTESIAN_POINT('Ctrl Pts',(-7.99560244965949,-0.223561721984852,
19.702273948512));
#69556=CARTESIAN_POINT('Ctrl Pts',(-4.12491798751938,-6.85234019671303,
20.0205054067588));
#69557=CARTESIAN_POINT('Ctrl Pts',(3.52984749513087,-7.17062885871895,20.3387368650056));
#69558=CARTESIAN_POINT('Ctrl Pts',(7.94613586721033,-0.910186439738384,
20.6569683232524));
#69559=CARTESIAN_POINT('Ctrl Pts',(5.05357067574419,6.20008562858578,20.9751997814993));
#69560=CARTESIAN_POINT('Ctrl Pts',(-1.21791937551955,7.35845772557836,21.2403926633716));
#69561=CARTESIAN_POINT('Ctrl Pts',(-5.11409431809678,4.82008527030502,21.4525469688695));
#69562=CARTESIAN_POINT('Ctrl Pts',(-7.41760565162783,0.780611363822664,
21.6647012743673));
#69563=CARTESIAN_POINT('Ctrl Pts',(-5.89036755802206,-5.41139616069077,
21.9298941562398));
#69564=CARTESIAN_POINT('Ctrl Pts',(1.37852472933923,-7.87839984678675,22.2481256144865));
#69565=CARTESIAN_POINT('Ctrl Pts',(7.36683206291293,-3.09960109130408,22.5663570727334));
#69566=CARTESIAN_POINT('Ctrl Pts',(6.59640065605321,4.52294295343979,22.8845885309801));
#69567=CARTESIAN_POINT('Ctrl Pts',(-0.24968637690976,7.99482927208096,23.202819989227));
#69568=CARTESIAN_POINT('Ctrl Pts',(-5.74440378410562,4.75731572102831,23.4680128710993));
#69569=CARTESIAN_POINT('Ctrl Pts',(-7.02177567656341,0.286092739201462,
23.6801671765972));
#69570=CARTESIAN_POINT('Ctrl Pts',(-6.11238176155939,-4.27422705355557,
23.8923214820951));
#69571=CARTESIAN_POINT('Ctrl Pts',(-0.899256061130584,-7.94801716864386,
24.1575143639675));
#69572=CARTESIAN_POINT('Ctrl Pts',(6.20658475963767,-5.04458325302331,24.4757458222142));
#69573=CARTESIAN_POINT('Ctrl Pts',(7.59457355786801,2.4900188839659,24.7939772804611));
#69574=CARTESIAN_POINT('Ctrl Pts',(2.0148809858328,7.74014012716691,25.1122087387078));
#69575=CARTESIAN_POINT('Ctrl Pts',(-5.4306142087339,5.87265422891856,25.4304401969547));
#69576=CARTESIAN_POINT('Ctrl Pts',(-7.45652383794003,-0.174585104238434,
25.695633078827));
#69577=CARTESIAN_POINT('Ctrl Pts',(-5.48926795468329,-4.38806563636966,
25.9077873843249));
#69578=CARTESIAN_POINT('Ctrl Pts',(-1.81250951477807,-7.23498700504909,
26.1199416898228));
#69579=CARTESIAN_POINT('Ctrl Pts',(4.53242930545347,-6.59065421393082,26.3851345716951));
#69580=CARTESIAN_POINT('Ctrl Pts',(7.99384341719809,0.260733573918202,26.703366029942));
#69581=CARTESIAN_POINT('Ctrl Pts',(4.1014942480699,6.85970017576753,27.0215974881888));
#69582=CARTESIAN_POINT('Ctrl Pts',(-3.55379234536194,7.16519884869196,27.3398289464356));
#69583=CARTESIAN_POINT('Ctrl Pts',(-7.95091308272635,0.873280898375759,
27.6580604046824));
#69584=CARTESIAN_POINT('Ctrl Pts',(-5.51545799319263,-5.02095118774497,
27.9232532865547));
#69585=CARTESIAN_POINT('Ctrl Pts',(-1.26739495731764,-6.91237243857469,
28.1354075920526));
#69586=CARTESIAN_POINT('Ctrl Pts',(3.37536823488139,-6.65109893050344,28.3475618975505));
#69587=CARTESIAN_POINT('Ctrl Pts',(7.7435347899277,-2.00432216315541,28.6127547794229));
#69588=CARTESIAN_POINT('Ctrl Pts',(5.8646663894612,5.4383088102437,28.9309862376697));
#69589=CARTESIAN_POINT('Ctrl Pts',(-1.40103628535671,7.86859828022052,29.2492176959165));
#69590=CARTESIAN_POINT('Ctrl Pts',(-7.38135086693103,3.07980096020935,29.5674491541633));
#69591=CARTESIAN_POINT('Ctrl Pts',(-6.57580919452638,-4.5539402514438,29.8856806124101));
#69592=CARTESIAN_POINT('Ctrl Pts',(-0.872195548143221,-7.40739513123128,
30.1508734942825));
#69593=CARTESIAN_POINT('Ctrl Pts',(3.57541475085797,-6.0500902527771,30.3630277997804));
#69594=CARTESIAN_POINT('Ctrl Pts',(6.90954676675677,-2.80862798931996,30.5751821052782));
#69595=CARTESIAN_POINT('Ctrl Pts',(7.1608386699862,3.56399044877616,30.8403749871506));
#69596=CARTESIAN_POINT('Ctrl Pts',(0.862204568500049,7.95148526108846,31.1586064453974));
#69597=CARTESIAN_POINT('Ctrl Pts',(-6.2171550118467,5.02242223703313,31.4768379036442));
#69598=CARTESIAN_POINT('Ctrl Pts',(-7.59255309626208,-2.51448842822771,
31.795069361891));
#69599=CARTESIAN_POINT('Ctrl Pts',(-1.97900925286816,-7.75004262914722,
32.1133008201379));
#69600=CARTESIAN_POINT('Ctrl Pts',(4.19838296891676,-6.16472287703994,32.3784937020102));
#69601=CARTESIAN_POINT('Ctrl Pts',(6.666516151879,-2.223678282517,32.5906480075081));
#69602=CARTESIAN_POINT('Ctrl Pts',(7.05852069625791,2.40987827179894,32.802802313006));
#69603=CARTESIAN_POINT('Ctrl Pts',(3.06982212892467,7.38619187899295,33.0679951948783));
#69604=CARTESIAN_POINT('Ctrl Pts',(-4.56267842884224,6.56897862153834,33.3862266531251));
#69605=CARTESIAN_POINT('Ctrl Pts',(-7.98729366609293,-0.284396659556839,
33.7044581113719));
#69606=CARTESIAN_POINT('Ctrl Pts',(-4.08392440862244,-6.87685073270514,
34.0226895696187));
#69607=CARTESIAN_POINT('Ctrl Pts',(3.58736965787411,-7.14915500701318,34.3409210278655));
#69608=CARTESIAN_POINT('Ctrl Pts',(7.21204142614238,-1.90175870498772,34.606113909738));
#69609=CARTESIAN_POINT('Ctrl Pts',(6.49148130388875,2.69218372119435,34.8182682152357));
#69610=CARTESIAN_POINT('Ctrl Pts',(3.74930300284587,6.44770925967051,35.0304225207337));
#69611=CARTESIAN_POINT('Ctrl Pts',(-2.52519696832531,7.58966525267737,35.295615402606));
#69612=CARTESIAN_POINT('Ctrl Pts',(-7.7521615457203,1.9681224413906,35.6138468608529));
#69613=CARTESIAN_POINT('Ctrl Pts',(-5.84420556441641,-5.45188067452137,
35.9320783190996));
#69614=CARTESIAN_POINT('Ctrl Pts',(1.42554748487432,-7.87002725177103,36.2503097773465));
#69615=CARTESIAN_POINT('Ctrl Pts',(7.39618317595128,-3.04567115826906,36.5685412355932));
#69616=CARTESIAN_POINT('Ctrl Pts',(6.69229361918976,3.29293695945461,36.8337341174657));
#69617=CARTESIAN_POINT('Ctrl Pts',(3.13606529227772,6.28906011976134,37.0458884229635));
#69618=CARTESIAN_POINT('Ctrl Pts',(-1.39681632961355,7.32660438714381,37.2580427284614));
#69619=CARTESIAN_POINT('Ctrl Pts',(-6.88304253051742,4.07472255492631,37.5232356103338));
#69620=CARTESIAN_POINT('Ctrl Pts',(-7.14361653878869,-3.59697891597865,
37.8414670685805));
#69621=CARTESIAN_POINT('Ctrl Pts',(-0.837857072193403,-7.94831662020021,
38.1596985268274));
#69622=CARTESIAN_POINT('Ctrl Pts',(6.23659876272117,-5.00742952502321,38.4779299850742));
#69623=CARTESIAN_POINT('Ctrl Pts',(7.58137358640385,2.54998292541648,38.796161443321));
#69624=CARTESIAN_POINT('Ctrl Pts',(2.89378037003512,6.87431908441773,39.0613543251934));
#69625=CARTESIAN_POINT('Ctrl Pts',(-1.75580788781819,6.8047278688039,39.2735086306912));
#69626=CARTESIAN_POINT('Ctrl Pts',(-5.85859134437765,4.61596524726659,39.4856629361891));
#69627=CARTESIAN_POINT('Ctrl Pts',(-7.86866875051649,-1.43655507071012,
39.7508558180615));
#69628=CARTESIAN_POINT('Ctrl Pts',(-3.03518877528446,-7.39980700245872,
40.0690872763082));
#69629=CARTESIAN_POINT('Ctrl Pts',(4.57898399105715,-6.55062189246316,40.3873187345551));
#69630=CARTESIAN_POINT('Ctrl Pts',(7.99214386231922,0.308465653263491,40.7055501928019));
#69631=CARTESIAN_POINT('Ctrl Pts',(4.05221027390455,6.89632005294123,41.0237816510487));
#69632=CARTESIAN_POINT('Ctrl Pts',(-2.32248703255162,7.08775575820863,41.2889745329211));
#69633=CARTESIAN_POINT('Ctrl Pts',(-5.78745547810781,3.98654509523236,41.5011288384189));
#69634=CARTESIAN_POINT('Ctrl Pts',(-7.45005792185978,-0.35618066388343,
41.7132831439168));
#69635=CARTESIAN_POINT('Ctrl Pts',(-4.99918629725736,-6.24401911767182,
41.9784760257892));
#69636=CARTESIAN_POINT('Ctrl Pts',(2.5602735735563,-7.57723655456257,42.296707484036));
#69637=CARTESIAN_POINT('Ctrl Pts',(7.75243656531128,-1.9435711639145,42.6149389422828));
#69638=CARTESIAN_POINT('Ctrl Pts',(5.83208594208859,5.47323379176722,42.9331704005297));
#69639=CARTESIAN_POINT('Ctrl Pts',(-1.46225849090136,7.86393276181355,43.2514018587764));
#69640=CARTESIAN_POINT('Ctrl Pts',(-6.40089488270372,3.82867763137183,43.5165947406488));
#69641=CARTESIAN_POINT('Ctrl Pts',(-6.98364633268417,-0.784771691250313,
43.7287490461467));
#69642=CARTESIAN_POINT('Ctrl Pts',(-5.39150645671536,-5.15382244858969,
43.9409033516445));
#69643=CARTESIAN_POINT('Ctrl Pts',(0.31955499060767,-7.9923415207632,44.2060962335169));
#69644=CARTESIAN_POINT('Ctrl Pts',(6.90137725357106,-4.04233924592448,44.5243276917637));
#69645=CARTESIAN_POINT('Ctrl Pts',(7.12772627499534,3.61569629768823,44.8425591500105));
#69646=CARTESIAN_POINT('Ctrl Pts',(0.814705416041519,7.95649229625233,45.1607906082574));
#69647=CARTESIAN_POINT('Ctrl Pts',(-6.2603207618579,4.97875710747049,45.4790220665041));
#69648=CARTESIAN_POINT('Ctrl Pts',(-7.34330271032281,-1.30619026522004,
45.7442149483766));
#69649=CARTESIAN_POINT('Ctrl Pts',(-4.75832887350283,-5.17160410694695,
45.9563692538743));
#69650=CARTESIAN_POINT('Ctrl Pts',(-0.691486153294226,-7.42644427732359,
46.1685235593723));
#69651=CARTESIAN_POINT('Ctrl Pts',(5.48173622302567,-5.82496406492823,46.4337164412445));
#69652=CARTESIAN_POINT('Ctrl Pts',(7.86127883304989,1.47302738748871,46.7519478994915));
#69653=CARTESIAN_POINT('Ctrl Pts',(3.0109183688609,7.40352025353016,47.0701793577382));
#69654=CARTESIAN_POINT('Ctrl Pts',(-4.60182495543848,6.54161460610092,47.3884108159851));
#69655=CARTESIAN_POINT('Ctrl Pts',(-7.99125469997778,-0.345668477910065,
47.7066422742318));
#69656=CARTESIAN_POINT('Ctrl Pts',(-4.6879952360915,-5.80111440766116,47.9718351561042));
#69657=CARTESIAN_POINT('Ctrl Pts',(-0.201756218294636,-7.02470477214385,
48.1839894616021));
#69658=CARTESIAN_POINT('Ctrl Pts',(4.34731499750045,-6.06061713168695,48.3961437670999));
#69659=CARTESIAN_POINT('Ctrl Pts',(7.95824221253658,-0.803753235227211,
48.6613366489724));
#69660=CARTESIAN_POINT('Ctrl Pts',(4.96969229260987,6.26671150540889,48.9795681072191));
#69661=CARTESIAN_POINT('Ctrl Pts',(-2.58103328601835,7.5641264363336,49.297799565466));
#69662=CARTESIAN_POINT('Ctrl Pts',(-7.7637763300124,1.92179386844403,49.6160310237127));
#69663=CARTESIAN_POINT('Ctrl Pts',(-5.80702124690748,-5.50074018787491,
49.9342624819596));
#69664=CARTESIAN_POINT('Ctrl Pts',(0.26410876978471,-7.453889874563,50.1994553638319));
#69665=CARTESIAN_POINT('Ctrl Pts',(4.45366316330294,-5.43618130080664,50.4116096693298));
#69666=CARTESIAN_POINT('Ctrl Pts',(7.25622959650091,-1.72550275202747,50.6237639748277));
#69667=CARTESIAN_POINT('Ctrl Pts',(6.53575466830331,4.61124162154712,50.8889568567));
#69668=CARTESIAN_POINT('Ctrl Pts',(-0.356703040538174,7.99013626392697,
51.2071883149469));
#69669=CARTESIAN_POINT('Ctrl Pts',(-6.90845543503368,4.01882881826647,51.5254197731937));
#69670=CARTESIAN_POINT('Ctrl Pts',(-7.1220091321019,-3.63957421926061,51.8436512314404));
#69671=CARTESIAN_POINT('Ctrl Pts',(-0.777745171693893,-7.96082601395384,
52.1618826896873));
#69672=CARTESIAN_POINT('Ctrl Pts',(5.0868175702758,-5.45476990450777,52.4270755715598));
#69673=CARTESIAN_POINT('Ctrl Pts',(6.92709267685679,-1.18430137787557,52.6392298770574));
#69674=CARTESIAN_POINT('Ctrl Pts',(6.61008875479717,3.45498977684364,52.8513841825556));
#69675=CARTESIAN_POINT('Ctrl Pts',(1.91119504467174,7.76704396007644,53.1165770644276));
#69676=CARTESIAN_POINT('Ctrl Pts',(-5.50833831846516,5.79894158830544,53.4348085226747));
#69677=CARTESIAN_POINT('Ctrl Pts',(-7.85120765946141,-1.49541962551961,
53.7530399809213));
#69678=CARTESIAN_POINT('Ctrl Pts',(-2.99094532675873,-7.41780025530413,
54.0712714391683));
#69679=CARTESIAN_POINT('Ctrl Pts',(4.63257276104932,-6.5206524205881,54.389502897415));
#69680=CARTESIAN_POINT('Ctrl Pts',(7.41733421524318,-0.78318634038966,54.6546957792874));
#69681=CARTESIAN_POINT('Ctrl Pts',(6.00672129400615,3.64780509396192,54.8668500847852));
#69682=CARTESIAN_POINT('Ctrl Pts',(2.72545722329887,6.94277398655306,55.0790043902831));
#69683=CARTESIAN_POINT('Ctrl Pts',(-3.64971923139309,7.11752681122709,55.3441972721555));
#69684=CARTESIAN_POINT('Ctrl Pts',(-7.96126514899932,0.766662769787909,
55.6624287304023));
#69685=CARTESIAN_POINT('Ctrl Pts',(-4.94740594913963,-6.27701489107626,
55.9806601886491));
#69686=CARTESIAN_POINT('Ctrl Pts',(2.60547680487975,-7.5618122956394,56.2988916468959));
#69687=CARTESIAN_POINT('Ctrl Pts',(7.7732473784035,-1.88580581467994,56.6171231051428));
#69688=CARTESIAN_POINT('Ctrl Pts',(6.11386519220779,4.27210488119153,56.8823159870151));
#69689=CARTESIAN_POINT('Ctrl Pts',(2.14346794565811,6.69273694936065,57.094470292513));
#69690=CARTESIAN_POINT('Ctrl Pts',(-2.49446165009483,7.02907453229768,57.3066245980108));
#69691=CARTESIAN_POINT('Ctrl Pts',(-7.42252109479894,2.98090908512862,57.5718174798833));
#69692=CARTESIAN_POINT('Ctrl Pts',(-6.51371741399781,-4.64122828848479,
57.8900489381299));
#69693=CARTESIAN_POINT('Ctrl Pts',(0.380285772234508,-7.98330284404963,
58.2082803963769));
#69694=CARTESIAN_POINT('Ctrl Pts',(6.92539378082645,-4.00105430552253,58.5265118546236));
#69695=CARTESIAN_POINT('Ctrl Pts',(7.10556325834136,3.67295646016214,58.8447433128705));
#69696=CARTESIAN_POINT('Ctrl Pts',(1.81502103305887,7.23435735597458,59.1099361947428));
#69697=CARTESIAN_POINT('Ctrl Pts',(-2.76993786559711,6.45868616114241,59.3220905002406));
#69698=CARTESIAN_POINT('Ctrl Pts',(-6.49226518895258,3.67161005836745,59.5342448057386));
#69699=CARTESIAN_POINT('Ctrl Pts',(-7.55879607452801,-2.6161498963625,59.7994376876108));
#69700=CARTESIAN_POINT('Ctrl Pts',(-1.87489434462579,-7.7752354158405,60.1176691458578));
#69701=CARTESIAN_POINT('Ctrl Pts',(5.52166351530564,-5.77831927052477,60.4359006041045));
#69702=CARTESIAN_POINT('Ctrl Pts',(7.85234220304677,1.51994621664714,60.7541320623515));
#69703=CARTESIAN_POINT('Ctrl Pts',(2.95663988242443,7.43222167203017,61.0723635205981));
#69704=CARTESIAN_POINT('Ctrl Pts',(-3.37305910088342,6.65227028963328,61.3375564024706));
#69705=CARTESIAN_POINT('Ctrl Pts',(-6.3262638672153,3.06032158273721,61.5497107079684));
#69706=CARTESIAN_POINT('Ctrl Pts',(-7.30930351420548,-1.48469183388794,
61.7618650134663));
#69707=CARTESIAN_POINT('Ctrl Pts',(-3.99177876553422,-6.93147463845664,
62.0270578953387));
#69708=CARTESIAN_POINT('Ctrl Pts',(3.68249852080414,-7.09990980361901,62.3452893535855));
#69709=CARTESIAN_POINT('Ctrl Pts',(7.95780437732607,-0.742355077159724,
62.6635208118322));
#69710=CARTESIAN_POINT('Ctrl Pts',(4.93218084187855,6.29627721103956,62.9817522700792));
#69711=CARTESIAN_POINT('Ctrl Pts',(-2.64083450203343,7.5502073818808,63.2999837283258));
#69712=CARTESIAN_POINT('Ctrl Pts',(-6.90857133452179,2.81102647092016,63.5651766101983));
#69713=CARTESIAN_POINT('Ctrl Pts',(-6.78315393156382,-1.83739093502485,
63.7773309156961));
#69714=CARTESIAN_POINT('Ctrl Pts',(-4.54528381471436,-5.91359643094503,
63.989485221194));
#69715=CARTESIAN_POINT('Ctrl Pts',(1.53093669630508,-7.85085162313262,64.2546781030663));
#69716=CARTESIAN_POINT('Ctrl Pts',(7.4357193671895,-2.94611474108738,64.5729095613132));
#69717=CARTESIAN_POINT('Ctrl Pts',(6.49516621486331,4.65731225168266,64.8911410195599));
#69718=CARTESIAN_POINT('Ctrl Pts',(-0.404411270724643,7.98786367556194,
65.2093724778069));
#69719=CARTESIAN_POINT('Ctrl Pts',(-6.94448088124453,3.96910867406852,65.5276039360535));
#69720=CARTESIAN_POINT('Ctrl Pts',(-7.05935686076257,-2.40742775941292,
65.7927968179261));
#69721=CARTESIAN_POINT('Ctrl Pts',(-3.91676322470201,-5.83490775839923,
66.0049511234238));
#69722=CARTESIAN_POINT('Ctrl Pts',(0.445613595873354,-7.44524386622448,
66.2171054289218));
#69723=CARTESIAN_POINT('Ctrl Pts',(6.30359804819689,-4.9238491064726,66.482298310794));
#69724=CARTESIAN_POINT('Ctrl Pts',(7.54594708052756,2.65107473171896,66.800529769041));
#69725=CARTESIAN_POINT('Ctrl Pts',(1.85034153482128,7.77521560940999,67.1187612272876));
#69726=CARTESIAN_POINT('Ctrl Pts',(-5.54286956338981,5.76594411857648,67.4369926855345));
#69727=CARTESIAN_POINT('Ctrl Pts',(-7.84580733502515,-1.55658139471971,
67.7552241437814));
#69728=CARTESIAN_POINT('Ctrl Pts',(-3.75154110074661,-6.44640729967567,
68.0204170256537));
#69729=CARTESIAN_POINT('Ctrl Pts',(0.868573158644488,-6.97371947930176,
68.2325713311516));
#69730=CARTESIAN_POINT('Ctrl Pts',(5.21819086966696,-5.32923181627554,68.4447256366494));
#69731=CARTESIAN_POINT('Ctrl Pts',(7.98792816139811,0.415502181809365,68.7099185185218));
#69732=CARTESIAN_POINT('Ctrl Pts',(3.95917763219824,6.94941918853656,69.0281499767686));
#69733=CARTESIAN_POINT('Ctrl Pts',(-3.70102374668385,7.08379593074294,69.3463814350154));
#69734=CARTESIAN_POINT('Ctrl Pts',(-7.96570146350195,0.719106919648195,
69.6646128932623));
#69735=CARTESIAN_POINT('Ctrl Pts',(-4.90322564425964,-6.31965321033109,
69.9828443515091));
#69736=CARTESIAN_POINT('Ctrl Pts',(1.39427281500069,-7.32708884673901,70.2480372333814));
#69737=CARTESIAN_POINT('Ctrl Pts',(5.22836818999202,-4.69588636995774,70.4601915388793));
#69738=CARTESIAN_POINT('Ctrl Pts',(7.43421207706811,-0.602261222926253,
70.6723458443772));
#69739=CARTESIAN_POINT('Ctrl Pts',(5.75872064546006,5.55128583577292,70.9375387262495));
#69740=CARTESIAN_POINT('Ctrl Pts',(-1.56731762340354,7.84302433409703,71.2557701844964));
#69741=CARTESIAN_POINT('Ctrl Pts',(-7.4391409603632,2.92180141067608,71.5740016427431));
#69742=CARTESIAN_POINT('Ctrl Pts',(-6.48588522666362,-4.6800432492488,71.89223310099));
#69743=CARTESIAN_POINT('Ctrl Pts',(0.441600573455518,-7.98652817688489,
72.2104645592367));
#69744=CARTESIAN_POINT('Ctrl Pts',(5.85698884249447,-4.61799821676437,72.4756574411092));
#69745=CARTESIAN_POINT('Ctrl Pts',(7.02662058273795,-0.117391358426442,
72.687811746607));
#69746=CARTESIAN_POINT('Ctrl Pts',(6.00797953533027,4.41977792653008,72.8999660521049));
#69747=CARTESIAN_POINT('Ctrl Pts',(0.708132550329375,7.96731585161226,73.1651589339772));
#69748=CARTESIAN_POINT('Ctrl Pts',(-6.32593134632851,4.89409127288728,73.4833903922241));
#69749=CARTESIAN_POINT('Ctrl Pts',(-7.53259465664785,-2.67168746361502,
73.8016218504708));
#69750=CARTESIAN_POINT('Ctrl Pts',(-1.82841823496171,-7.78627045868244,
74.1198533087177));
#69751=CARTESIAN_POINT('Ctrl Pts',(5.5700503670788,-5.74059578517867,74.4380847669645));
#69752=CARTESIAN_POINT('Ctrl Pts',(7.45022067480577,0.353672707356798,74.7032776488368));
#69753=CARTESIAN_POINT('Ctrl Pts',(5.38225798952639,4.51851390470657,74.9154319543348));
#69754=CARTESIAN_POINT('Ctrl Pts',(1.63837574292985,7.27668056502784,75.1275862598326));
#69755=CARTESIAN_POINT('Ctrl Pts',(-4.68966200686914,6.47937198055273,75.3927791417049));
#69756=CARTESIAN_POINT('Ctrl Pts',(-7.98481911427963,-0.451714078618975,
75.7110105999518));
#69757=CARTESIAN_POINT('Ctrl Pts',(-3.93641975399691,-6.95786990334269,
76.0292420581986));
#69758=CARTESIAN_POINT('Ctrl Pts',(3.72640233843597,-7.07468376429424,76.3474735164454));
#69759=CARTESIAN_POINT('Ctrl Pts',(7.96656438966708,-0.688066392457169,
76.6657049746923));
#69760=CARTESIAN_POINT('Ctrl Pts',(4.88424055995273,6.3309887778437,76.983936432939));
#69761=CARTESIAN_POINT('Ctrl Pts',(-2.68513291585741,7.52976860837553,77.3021678911859));
#69762=CARTESIAN_POINT('Ctrl Pts',(-7.78912256814826,1.81409798934657,77.6203993494327));
#69763=CARTESIAN_POINT('Ctrl Pts',(-5.73116360124679,-5.57933282541807,
77.9386308076794));
#69764=CARTESIAN_POINT('Ctrl Pts',(0.366457134883102,-7.44983652765403,
78.2038236895519));
#69765=CARTESIAN_POINT('Ctrl Pts',(4.52781078590357,-5.37443936238026,78.4159779950496));
#69766=CARTESIAN_POINT('Ctrl Pts',(7.27925103524264,-1.62584650356412,78.6281323005476));
#69767=CARTESIAN_POINT('Ctrl Pts',(6.47184422235408,4.70054607701997,78.8933251824199));
#69768=CARTESIAN_POINT('Ctrl Pts',(-0.466311279410581,7.98446458370159,
79.2115566406668));
#69769=CARTESIAN_POINT('Ctrl Pts',(-6.96295945194999,3.92365796612018,79.5297880989135));
#69770=CARTESIAN_POINT('Ctrl Pts',(-7.07139022597889,-3.73697431858228,
79.8480195571604));
#69771=CARTESIAN_POINT('Ctrl Pts',(-0.668426236305269,-7.9707452571768,
80.1662510154071));
#69772=CARTESIAN_POINT('Ctrl Pts',(5.16119534842955,-5.38445146622561,80.4314438972796));
#69773=CARTESIAN_POINT('Ctrl Pts',(6.94269238652436,-1.08912807827487,80.6435982027774));
#69774=CARTESIAN_POINT('Ctrl Pts',(6.56205343067632,3.54537453650439,80.8557525082755));
#69775=CARTESIAN_POINT('Ctrl Pts',(1.80442728846643,7.7925403782906,81.1209453901475));
#69776=CARTESIAN_POINT('Ctrl Pts',(-5.58739884552956,5.72280404428344,81.4391768483945));
#69777=CARTESIAN_POINT('Ctrl Pts',(-7.82994662556973,-1.60302138236276,
81.7574083066413));
#69778=CARTESIAN_POINT('Ctrl Pts',(-2.88886868043504,-7.4581467527175,82.0756397648882));
#69779=CARTESIAN_POINT('Ctrl Pts',(4.72161988681341,-6.45646525177274,82.3938712231348));
#69780=CARTESIAN_POINT('Ctrl Pts',(7.42738348108055,-0.681324014282815,
82.6590641050074));
#69781=CARTESIAN_POINT('Ctrl Pts',(5.95609658300921,3.72989225361022,82.8712184105051));
#69782=CARTESIAN_POINT('Ctrl Pts',(2.62992441186326,6.97952184884766,83.0833727160031));
#69783=CARTESIAN_POINT('Ctrl Pts',(-3.74704986675743,7.06677123681013,83.3485655978754));
#69784=CARTESIAN_POINT('Ctrl Pts',(-7.97103643639252,0.657337582393124,
83.6667970561222));
#69785=CARTESIAN_POINT('Ctrl Pts',(-4.86080016327485,-6.34431740494078,
83.9850285143689));
#69786=CARTESIAN_POINT('Ctrl Pts',(2.70900273192573,-7.52534509372946,84.3032599726158));
#69787=CARTESIAN_POINT('Ctrl Pts',(7.79839444842538,-1.77895542426286,84.6214914308625));
#69788=CARTESIAN_POINT('Ctrl Pts',(6.05466308452315,4.35560359040991,84.886684312735));
#69789=CARTESIAN_POINT('Ctrl Pts',(2.05142121191431,6.7215216818231,85.0988386182328));
#69790=CARTESIAN_POINT('Ctrl Pts',(-2.59068723364047,6.99418096429851,85.3109929237309));
#69791=CARTESIAN_POINT('Ctrl Pts',(-7.46272936928494,2.87876861479598,85.576185805603));
#69792=CARTESIAN_POINT('Ctrl Pts',(-6.44941214782463,-4.73017943875191,
85.89441726385));
#69793=CARTESIAN_POINT('Ctrl Pts',(0.489805379921119,-7.97733240238224,
86.2126487220966));
#69794=CARTESIAN_POINT('Ctrl Pts',(6.97964839115342,-3.90563988498063,86.5308801803437));
#69795=CARTESIAN_POINT('Ctrl Pts',(7.05448992189358,3.77012072995617,86.8491116385901));
#69796=CARTESIAN_POINT('Ctrl Pts',(1.71557253344269,7.25858378658518,87.1143045204627));
#69797=CARTESIAN_POINT('Ctrl Pts',(-2.85831002962552,6.42006592504683,87.3264588259607));
#69798=CARTESIAN_POINT('Ctrl Pts',(-6.54203959894669,3.58217051383667,87.5386131314584));
#69799=CARTESIAN_POINT('Ctrl Pts',(-7.52218268870725,-2.71963342644761,
87.8038060133308));
#69800=CARTESIAN_POINT('Ctrl Pts',(-1.76801769993584,-7.80023255986408,
88.1220374715777));
#69801=CARTESIAN_POINT('Ctrl Pts',(5.6004398390903,-5.70200098010378,88.4402689298243));
#69802=CARTESIAN_POINT('Ctrl Pts',(7.83074445421797,1.62756132541459,88.7585003880712));
#69803=CARTESIAN_POINT('Ctrl Pts',(2.85436857570851,7.47209598509982,89.0767318463181));
#69804=CARTESIAN_POINT('Ctrl Pts',(-3.46403103994571,6.60535515007955,89.3419247281905));
#69805=CARTESIAN_POINT('Ctrl Pts',(-6.36766515477992,2.97321764827318,89.5540790336882));
#69806=CARTESIAN_POINT('Ctrl Pts',(-7.28824069935606,-1.58485810489139,
89.7662333391863));
#69807=CARTESIAN_POINT('Ctrl Pts',(-3.89628177039754,-6.98560138729692,
90.0314262210585));
#69808=CARTESIAN_POINT('Ctrl Pts',(3.7795843093107,-7.0487060531747,90.3496576793053));
#69809=CARTESIAN_POINT('Ctrl Pts',(7.96724241483808,-0.633079672380178,
90.6678891375522));
#69810=CARTESIAN_POINT('Ctrl Pts',(4.84531215134557,6.36336897651491,90.9861205957989));
#69811=CARTESIAN_POINT('Ctrl Pts',(-2.74419784445042,7.51325605626818,91.3043520540459));
#69812=CARTESIAN_POINT('Ctrl Pts',(-6.94649669459085,2.71595496583219,91.569544935918));
#69813=CARTESIAN_POINT('Ctrl Pts',(-6.75730054780259,-1.93030360670755,
91.7816992414161));
#69814=CARTESIAN_POINT('Ctrl Pts',(-4.46370311146622,-5.97541481715509,
91.9938535469138));
#69815=CARTESIAN_POINT('Ctrl Pts',(1.6385303148144,-7.82910319155211,92.2590464287863));
#69816=CARTESIAN_POINT('Ctrl Pts',(7.47544891365297,-2.84379642636655,92.577277887033));
#69817=CARTESIAN_POINT('Ctrl Pts',(6.43064197423995,4.74600730799249,92.8955093452797));
#69818=CARTESIAN_POINT('Ctrl Pts',(-0.513991195223748,7.98156172853921,
93.2137408035268));
#69819=CARTESIAN_POINT('Ctrl Pts',(-6.99829530210772,3.87343532810802,93.5319722617734));
#69820=CARTESIAN_POINT('Ctrl Pts',(-7.02565481334343,-2.50407710506977,
93.797165143646));
#69821=CARTESIAN_POINT('Ctrl Pts',(-3.83632155666589,-5.88810832281994,
94.0093194491437));
#69822=CARTESIAN_POINT('Ctrl Pts',(0.547743231317241,-7.43842759304252,
94.2214737546418));
#69823=CARTESIAN_POINT('Ctrl Pts',(6.37057478731908,-4.83688073614729,94.4866666365138));
#69824=CARTESIAN_POINT('Ctrl Pts',(7.50885562870737,2.75437864544419,94.8048980947609));
#69825=CARTESIAN_POINT('Ctrl Pts',(1.74346747397237,7.79987581539445,95.1231295530076));
#69826=CARTESIAN_POINT('Ctrl Pts',(-5.62147406522839,5.68933598139671,95.4413610112545));
#69827=CARTESIAN_POINT('Ctrl Pts',(-7.82370745446396,-1.66410337524508,
95.7595924695011));
#69828=CARTESIAN_POINT('Ctrl Pts',(-3.66272334045319,-6.49728292716958,
96.0247853513737));
#69829=CARTESIAN_POINT('Ctrl Pts',(0.964192204000728,-6.96114330416675,
96.2369396568714));
#69830=CARTESIAN_POINT('Ctrl Pts',(5.29083291191058,-5.25712039073047,96.4490939623694));
#69831=CARTESIAN_POINT('Ctrl Pts',(7.98147400706142,0.525081947070879,96.7142868442416));
#69832=CARTESIAN_POINT('Ctrl Pts',(3.86343745250282,7.00309685966486,97.0325183024886));
#69833=CARTESIAN_POINT('Ctrl Pts',(-3.79788665865216,7.03233947533876,97.3507497607354));
#69834=CARTESIAN_POINT('Ctrl Pts',(-7.97481972187845,0.609725330610525,
97.668981218982));
#69835=CARTESIAN_POINT('Ctrl Pts',(-4.81603888871812,-6.38634541806905,
97.9872126772292));
#69836=CARTESIAN_POINT('Ctrl Pts',(1.49469166773618,-7.30726518766016,98.2524055591011));
#69837=CARTESIAN_POINT('Ctrl Pts',(5.29231783318236,-4.62369491424136,98.4645598645992));
#69838=CARTESIAN_POINT('Ctrl Pts',(7.44177689490699,-0.500184316846411,
98.676714170097));
#69839=CARTESIAN_POINT('Ctrl Pts',(5.68199770515192,5.6297904450508,98.9419070519693));
#69840=CARTESIAN_POINT('Ctrl Pts',(-1.67480042471626,7.82077733429483,99.2601385102162));
#69841=CARTESIAN_POINT('Ctrl Pts',(-7.47853648893081,2.81943851717081,99.578369968463));
#69842=CARTESIAN_POINT('Ctrl Pts',(-6.42105000078872,-4.7686089651617,99.8966014267099));
#69843=CARTESIAN_POINT('Ctrl Pts',(0.551158827295702,-7.97971567937298,
100.214832884957));
#69844=CARTESIAN_POINT('Ctrl Pts',(5.91981014714418,-4.53718806378571,100.480025766829));
#69845=CARTESIAN_POINT('Ctrl Pts',(7.02757025506314,-0.020952745718006,
100.692180072327));
#69846=CARTESIAN_POINT('Ctrl Pts',(5.94675997122199,4.50180780898751,100.904334377825));
#69847=CARTESIAN_POINT('Ctrl Pts',(0.598731752276945,7.9762872732464,101.169527259698));
#69848=CARTESIAN_POINT('Ctrl Pts',(-6.39250081992776,4.80681264898825,101.487758717944));
#69849=CARTESIAN_POINT('Ctrl Pts',(-7.49521572953847,-2.77479417904354,
101.805990176191));
#69850=CARTESIAN_POINT('Ctrl Pts',(-1.72140562995735,-7.81065152419441,
102.124221634438));
#69851=CARTESIAN_POINT('Ctrl Pts',(5.64832647306271,-5.66357187914456,102.442453092685));
#69852=CARTESIAN_POINT('Ctrl Pts',(7.44462716948537,0.455800407799888,102.707645974557));
#69853=CARTESIAN_POINT('Ctrl Pts',(5.31979465006875,4.59205483291529,102.919800280055));
#69854=CARTESIAN_POINT('Ctrl Pts',(1.53823802277218,7.29822248836579,103.131954585553));
#69855=CARTESIAN_POINT('Ctrl Pts',(-4.77787174527572,6.4149497240613,103.397147467425));
#69856=CARTESIAN_POINT('Ctrl Pts',(-7.97831370836171,-0.562160961128552,
103.715378925672));
#69857=CARTESIAN_POINT('Ctrl Pts',(-3.83975269512832,-7.00956780469594,
104.033610383919));
#69858=CARTESIAN_POINT('Ctrl Pts',(3.82160958092987,-7.02600987660817,104.351841842166));
#69859=CARTESIAN_POINT('Ctrl Pts',(7.97820106506273,-0.57266582050002,104.670073300412));
#69860=CARTESIAN_POINT('Ctrl Pts',(5.32208684584968,5.22547790251025,104.935266182285));
#69861=CARTESIAN_POINT('Ctrl Pts',(1.00568407969865,6.9552701054123,105.147420487783));
#69862=CARTESIAN_POINT('Ctrl Pts',(-3.62391518544271,6.51900808659635,105.359574793281));
#69863=CARTESIAN_POINT('Ctrl Pts',(-7.81364537834605,1.71072624285364,105.624767675153));
#69864=CARTESIAN_POINT('Ctrl Pts',(-5.65529940502205,-5.65571420908154,
105.9429991334));
#69865=CARTESIAN_POINT('Ctrl Pts',(1.69692613162078,-7.810133370961,106.261230591646));
#69866=CARTESIAN_POINT('Ctrl Pts',(7.49229788260741,-2.79910468070165,106.579462049893));
#69867=CARTESIAN_POINT('Ctrl Pts',(6.39930365278937,4.79880726180303,106.89769350814));
#69868=CARTESIAN_POINT('Ctrl Pts',(0.592088537923887,7.43502917732339,107.162886390013));
#69869=CARTESIAN_POINT('Ctrl Pts',(-3.80114279899899,5.91087947170466,107.37504069551));
#69870=CARTESIAN_POINT('Ctrl Pts',(-7.01059819590207,2.5459262833012,107.587195001008));
#69871=CARTESIAN_POINT('Ctrl Pts',(-7.02126802134622,-3.83163591028142,
107.852387882881));
#69872=CARTESIAN_POINT('Ctrl Pts',(-0.561575788910652,-7.97835491868844,
108.170619341127));
#69873=CARTESIAN_POINT('Ctrl Pts',(6.40222739562009,-4.78426859019708,108.488850799374));
#69874=CARTESIAN_POINT('Ctrl Pts',(7.49227345438683,2.79917006627677,108.807082257621));
#69875=CARTESIAN_POINT('Ctrl Pts',(1.68518581163966,7.81919351063693,109.125313715868));
#69876=CARTESIAN_POINT('Ctrl Pts',(-4.42799259471567,6.0019254648432,109.39050659774));
#69877=CARTESIAN_POINT('Ctrl Pts',(-6.74567008963042,1.97056280013258,109.602660903238));
#69878=CARTESIAN_POINT('Ctrl Pts',(-6.96256832586624,-2.67448499940349,
109.814815208736));
#69879=CARTESIAN_POINT('Ctrl Pts',(-2.78895030028104,-7.49675893964188,
110.080008090608));
#69880=CARTESIAN_POINT('Ctrl Pts',(4.80728149506295,-6.39214824628434,110.398239548855));
#69881=CARTESIAN_POINT('Ctrl Pts',(7.97087579703635,0.585560070868035,110.716471007102));
#69882=CARTESIAN_POINT('Ctrl Pts',(3.82154826442267,7.02604322773049,111.034702465349));
#69883=CARTESIAN_POINT('Ctrl Pts',(-3.85455763969707,7.00871056463248,111.352933923595));
#69884=CARTESIAN_POINT('Ctrl Pts',(-7.2786606794505,1.62828941463469,111.618126805468));
#69885=CARTESIAN_POINT('Ctrl Pts',(-6.38528112390476,-2.9351946572768,111.830281110966));
#69886=CARTESIAN_POINT('Ctrl Pts',(-3.50335692154129,-6.5845818382551,112.042435416464));
#69887=CARTESIAN_POINT('Ctrl Pts',(2.8097620210391,-7.48898362674566,112.307628298336));
#69888=CARTESIAN_POINT('Ctrl Pts',(7.82090015176617,-1.67422680403625,112.625859756583));
#69889=CARTESIAN_POINT('Ctrl Pts',(5.63434107372123,5.66850440886771,112.94409121483));
#69890=CARTESIAN_POINT('Ctrl Pts',(-1.72147379386281,7.81063650109863,113.262322673076));
#69891=CARTESIAN_POINT('Ctrl Pts',(-7.50583189001486,2.76443954814953,113.580554131323));
#69892=CARTESIAN_POINT('Ctrl Pts',(-6.56328362939538,-3.5430969087086,113.845747013196));
#69893=CARTESIAN_POINT('Ctrl Pts',(-2.89654180789393,-6.40290779744046,
114.057901318693));
#69894=CARTESIAN_POINT('Ctrl Pts',(1.67225938963234,-7.26868462915931,114.270055624191));
#69895=CARTESIAN_POINT('Ctrl Pts',(7.03188342456394,-3.81211934229238,114.535248506064));
#69896=CARTESIAN_POINT('Ctrl Pts',(7.00281347638515,3.86395108537982,114.853479964311));
#69897=CARTESIAN_POINT('Ctrl Pts',(0.537365184297669,7.97426988677213,115.171711422557));
#69898=CARTESIAN_POINT('Ctrl Pts',(-6.42109161644814,4.76855292813543,115.489942880804));
#69899=CARTESIAN_POINT('Ctrl Pts',(-7.4797626739027,-2.83421747906345,115.808174339051));
#69900=CARTESIAN_POINT('Ctrl Pts',(-2.63234719477822,-6.97860845373441,
116.073367220923));
#69901=CARTESIAN_POINT('Ctrl Pts',(2.01130457693764,-6.73363472473754,116.285521526421));
#69902=CARTESIAN_POINT('Ctrl Pts',(6.02858315192499,-4.3916298665434,116.497675831919));
#69903=CARTESIAN_POINT('Ctrl Pts',(7.80886364361634,1.73242228453224,116.762868713792));
#69904=CARTESIAN_POINT('Ctrl Pts',(2.75382789980835,7.50905762885649,117.081100172038));
#69905=CARTESIAN_POINT('Ctrl Pts',(-4.82288283518692,6.37318936847433,117.399331630285));
#69906=CARTESIAN_POINT('Ctrl Pts',(-7.97481440046939,-0.609794927262758,
117.717563088532));
#69907=CARTESIAN_POINT('Ctrl Pts',(-3.78912212147895,-7.04430208928159,
118.035794546779));
#69908=CARTESIAN_POINT('Ctrl Pts',(2.58825904592296,-6.99507990058644,118.300987428651));
#69909=CARTESIAN_POINT('Ctrl Pts',(5.93374949616459,-3.76534190003606,118.513141734149));
#69910=CARTESIAN_POINT('Ctrl Pts',(7.43131413590726,0.637022698069072,118.725296039647));
#69911=CARTESIAN_POINT('Ctrl Pts',(4.76003559506075,6.42819566521531,118.990488921519));
#69912=CARTESIAN_POINT('Ctrl Pts',(-2.84434470672376,7.47524031483816,119.308720379766));
#69913=CARTESIAN_POINT('Ctrl Pts',(-7.82024863945352,1.64968263175073,119.626951838013));
#69914=CARTESIAN_POINT('Ctrl Pts',(-5.62142441387692,-5.68938504008292,
119.94518329626));
#69915=CARTESIAN_POINT('Ctrl Pts',(1.75792871045866,-7.8031612200109,120.263414754506));
#69916=CARTESIAN_POINT('Ctrl Pts',(6.54079565338119,-3.58444136862353,120.528607636379));
#69917=CARTESIAN_POINT('Ctrl Pts',(6.94906363216944,1.04771052464956,120.740761941877));
#69918=CARTESIAN_POINT('Ctrl Pts',(5.19321024840485,5.35357777754774,120.952916247375));
#69919=CARTESIAN_POINT('Ctrl Pts',(-0.620883826172455,7.97459351007532,
121.218109129247));
#69920=CARTESIAN_POINT('Ctrl Pts',(-7.04898324843627,3.77906731066201,121.536340587494));
#69921=CARTESIAN_POINT('Ctrl Pts',(-6.98622830803955,-3.88205558903035,
121.854572045741));
#69922=CARTESIAN_POINT('Ctrl Pts',(-0.513921539690748,-7.98156621386383,
122.172803503987));
#69923=CARTESIAN_POINT('Ctrl Pts',(6.44371489477547,-4.73900588007502,122.491034962234));
#69924=CARTESIAN_POINT('Ctrl Pts',(7.28879044406725,1.58232789486348,122.756227844106));
#69925=CARTESIAN_POINT('Ctrl Pts',(4.55981260870684,5.34745656185066,122.968382149604));
#69926=CARTESIAN_POINT('Ctrl Pts',(0.410789081138449,7.44724647337578,123.180536455102));
#69927=CARTESIAN_POINT('Ctrl Pts',(-5.69761270396623,5.6139868054832,123.445729336975));
#69928=CARTESIAN_POINT('Ctrl Pts',(-7.80010286333989,-1.76858980449572,
123.763960795221));
#69929=CARTESIAN_POINT('Ctrl Pts',(-2.72943467181251,-7.51185249726616,
124.082192253468));
#69930=CARTESIAN_POINT('Ctrl Pts',(4.84536768462038,-6.36332669097587,124.400423711715));
#69931=CARTESIAN_POINT('Ctrl Pts',(7.97252218387298,0.646937712759203,124.718655169962));
#69932=CARTESIAN_POINT('Ctrl Pts',(4.46577720920391,5.97386488147713,124.983848051834));
#69933=CARTESIAN_POINT('Ctrl Pts',(-0.0634342396665083,7.02731519178123,
125.196002357332));
#69934=CARTESIAN_POINT('Ctrl Pts',(-4.57289059627595,5.89227454374625,125.40815666283));
#69935=CARTESIAN_POINT('Ctrl Pts',(-7.98290165102412,0.50291113192436,125.673349544702));
#69936=CARTESIAN_POINT('Ctrl Pts',(-4.72970639284564,-6.44975906625399,
125.991581002949));
#69937=CARTESIAN_POINT('Ctrl Pts',(2.8645949836211,-7.46135625393853,126.309812461196));
#69938=CARTESIAN_POINT('Ctrl Pts',(7.83075865773387,-1.62749298602955,126.628043919442));
#69939=CARTESIAN_POINT('Ctrl Pts',(5.59533973146904,5.71592614245338,126.94627537769));
#69940=CARTESIAN_POINT('Ctrl Pts',(-0.545160946366092,7.43861729402364,
127.211468259562));
#69941=CARTESIAN_POINT('Ctrl Pts',(-4.65560265593447,5.26427075837259,127.42362256506));
#69942=CARTESIAN_POINT('Ctrl Pts',(-7.31616713073084,1.45049171648925,127.635776870558));
#69943=CARTESIAN_POINT('Ctrl Pts',(-6.35711562868407,-4.85455654618202,
127.90096975243));
#69944=CARTESIAN_POINT('Ctrl Pts',(0.657922218832197,-7.97098820280248,
128.219201210677));
#69945=CARTESIAN_POINT('Ctrl Pts',(7.05516932572682,-3.755306559217,128.537432668924));
#69946=CARTESIAN_POINT('Ctrl Pts',(6.97961430616004,3.90570079659165,128.855664127171));
#69947=CARTESIAN_POINT('Ctrl Pts',(0.476824099015226,7.98450231104828,129.173895585417));
#69948=CARTESIAN_POINT('Ctrl Pts',(-5.28900758248167,5.2589567878849,129.43908846729));
#69949=CARTESIAN_POINT('Ctrl Pts',(-6.96684468589892,0.922094263057371,
129.651242772787));
#69950=CARTESIAN_POINT('Ctrl Pts',(-6.47502293851151,-3.70193269119533,
129.863397078285));
#69951=CARTESIAN_POINT('Ctrl Pts',(-1.61677841934224,-7.833624060375,130.128589960158));
#69952=CARTESIAN_POINT('Ctrl Pts',(5.72321401184765,-5.58697914349428,130.446821418405));
#69953=CARTESIAN_POINT('Ctrl Pts',(7.78919398690618,1.7905861059219,130.765052876651));
#69954=CARTESIAN_POINT('Ctrl Pts',(2.70893705762593,7.52536873469137,131.083284334898));
#69955=CARTESIAN_POINT('Ctrl Pts',(-4.87530267885765,6.34121929648078,131.401515793145));
#69956=CARTESIAN_POINT('Ctrl Pts',(-7.44160280738336,0.502767701364091,
131.666708675017));
#69957=CARTESIAN_POINT('Ctrl Pts',(-5.86481005809476,-3.87184525644711,
131.878862980515));
#69958=CARTESIAN_POINT('Ctrl Pts',(-2.46156105428565,-7.0406636676107,132.091017286013));
#69959=CARTESIAN_POINT('Ctrl Pts',(3.91566946395988,-6.97475239887046,132.356210167885));
#69960=CARTESIAN_POINT('Ctrl Pts',(7.98452298698976,-0.465733019532299,
132.674441626132));
#69961=CARTESIAN_POINT('Ctrl Pts',(4.70704716486712,6.45921423673906,132.992673084379));
#69962=CARTESIAN_POINT('Ctrl Pts',(-2.88893378327778,7.45812149077002,133.310904542626));
#69963=CARTESIAN_POINT('Ctrl Pts',(-7.83886510894448,1.59117320877073,133.629136000873));
#69964=CARTESIAN_POINT('Ctrl Pts',(-5.94832241656495,-4.49974311855476,
133.894328882745));
#69965=CARTESIAN_POINT('Ctrl Pts',(-1.8894202492775,-6.76884582695023,134.106483188243));
#69966=CARTESIAN_POINT('Ctrl Pts',(2.75789712626501,-6.9299517419192,134.318637493741));
#69967=CARTESIAN_POINT('Ctrl Pts',(7.52970753859752,-2.69872984193025,134.583830375613));
#69968=CARTESIAN_POINT('Ctrl Pts',(6.33396264917428,4.88369038065638,134.90206183386));
#69969=CARTESIAN_POINT('Ctrl Pts',(-0.681230328833862,7.96326985650064,
135.220293292107));
#69970=CARTESIAN_POINT('Ctrl Pts',(-7.07142496626254,3.73690560782156,135.538524750354));
#69971=CARTESIAN_POINT('Ctrl Pts',(-6.96192060855357,-3.93843875371134,
135.8567562086));
#69972=CARTESIAN_POINT('Ctrl Pts',(-1.54077150979294,-7.29768804889607,
136.121949090473));
#69973=CARTESIAN_POINT('Ctrl Pts',(3.01165605383282,-6.34957561737892,136.334103395971));
#69974=CARTESIAN_POINT('Ctrl Pts',(6.62617463464419,-3.42403817379246,136.546257701469));
#69975=CARTESIAN_POINT('Ctrl Pts',(7.45470471451398,2.89948547089672,136.811450583341));
#69976=CARTESIAN_POINT('Ctrl Pts',(1.58019449830633,7.8404400337463,137.129682041588));
#69977=CARTESIAN_POINT('Ctrl Pts',(-5.73575162660879,5.56586874137625,137.447913499834));
#69978=CARTESIAN_POINT('Ctrl Pts',(-7.78940231799192,-1.81513803985067,
137.766144958081));
#69979=CARTESIAN_POINT('Ctrl Pts',(-2.67411191098722,-7.53848551527781,
138.084376416328));
#69980=CARTESIAN_POINT('Ctrl Pts',(3.62165189183669,-6.52026573681974,138.349569298201));
#69981=CARTESIAN_POINT('Ctrl Pts',(6.4372271930946,-2.81944830984448,138.561723603698));
#69982=CARTESIAN_POINT('Ctrl Pts',(7.24808047400849,1.75941954822804,138.773877909196));
#69983=CARTESIAN_POINT('Ctrl Pts',(3.72740723771489,7.07715152167648,139.039070791069));
#69984=CARTESIAN_POINT('Ctrl Pts',(-3.9477607112626,6.95591115109018,139.357302249315));
#69985=CARTESIAN_POINT('Ctrl Pts',(-7.98014753412108,0.441573212544696,
139.675533707562));
#69986=CARTESIAN_POINT('Ctrl Pts',(-4.69110611854187,-6.47788838741673,
139.993765165809));
#69987=CARTESIAN_POINT('Ctrl Pts',(2.92382844266543,-7.44519077085319,140.311996624056));
#69988=CARTESIAN_POINT('Ctrl Pts',(7.00971395453912,-2.54835986075936,140.577189505928));
#69989=CARTESIAN_POINT('Ctrl Pts',(6.70899796654445,2.09201553347577,140.789343811426));
#69990=CARTESIAN_POINT('Ctrl Pts',(4.31892338446397,6.08088221424489,141.001498116924));
#69991=CARTESIAN_POINT('Ctrl Pts',(-1.82606445310679,7.78749812132479,141.266690998797));
#69992=CARTESIAN_POINT('Ctrl Pts',(-7.54158359928277,2.6634622937598,141.584922457043));
#69993=CARTESIAN_POINT('Ctrl Pts',(-6.31481780085691,-4.89906294206899,
141.90315391529));
#69994=CARTESIAN_POINT('Ctrl Pts',(0.705510731853791,-7.96691716930022,
142.221385373537));
#69995=CARTESIAN_POINT('Ctrl Pts',(7.08929314563132,-3.70426255438861,142.539616831784));
#69996=CARTESIAN_POINT('Ctrl Pts',(6.96349635444189,2.67206778096168,142.804809713656));
#69997=CARTESIAN_POINT('Ctrl Pts',(3.69381931185978,5.97853507129855,143.016964019154));
#69998=CARTESIAN_POINT('Ctrl Pts',(-0.726210311352885,7.4231291439697,143.229118324652));
#69999=CARTESIAN_POINT('Ctrl Pts',(-6.48488964979702,4.68250409572428,143.494311206524));
#70000=CARTESIAN_POINT('Ctrl Pts',(-7.44054713237905,-2.93390063673488,
143.812542664771));
#70001=CARTESIAN_POINT('Ctrl Pts',(-1.55565991875539,-7.83949384752223,
144.130774123018));
#70002=CARTESIAN_POINT('Ctrl Pts',(5.7564756520609,-5.55270228289268,144.449005581264));
#70003=CARTESIAN_POINT('Ctrl Pts',(7.78148983349211,1.8515005667527,144.767237039512));
#70004=CARTESIAN_POINT('Ctrl Pts',(3.50564254954319,6.5833652502107,145.032429921384));
#70005=CARTESIAN_POINT('Ctrl Pts',(-1.13107777388849,6.93598196205286,145.244584226882));
#70006=CARTESIAN_POINT('Ctrl Pts',(-5.41555070126417,5.12855128734094,145.456738532379));
#70007=CARTESIAN_POINT('Ctrl Pts',(-7.96656314127199,-0.716596178392399,
145.721931414252));
#70008=CARTESIAN_POINT('Ctrl Pts',(-3.69415225913557,-7.09385323224563,
146.040162872499));
#70009=CARTESIAN_POINT('Ctrl Pts',(3.96566476044414,-6.93910978213129,146.358394330745));
#70010=CARTESIAN_POINT('Ctrl Pts',(7.98716182589273,-0.418043648415986,
146.676625788992));
#70011=CARTESIAN_POINT('Ctrl Pts',(4.66128955204064,6.50015524624547,146.994857247239));
#70012=CARTESIAN_POINT('Ctrl Pts',(-1.66973597467493,7.26926470625684,147.260050129111));
#70013=CARTESIAN_POINT('Ctrl Pts',(-5.40182421568405,4.49527282901404,147.472204434609));
#70014=CARTESIAN_POINT('Ctrl Pts',(-7.45164225692231,0.321334579947432,
147.684358740107));
#70015=CARTESIAN_POINT('Ctrl Pts',(-5.54516633579186,-5.76461334347584,
147.949551621979));
#70016=CARTESIAN_POINT('Ctrl Pts',(1.86212403554058,-7.77830379904534,148.267783080226));
#70017=CARTESIAN_POINT('Ctrl Pts',(7.54408560015588,-2.6390370489041,148.586014538473));
#70018=CARTESIAN_POINT('Ctrl Pts',(6.30468538270765,4.92142733395752,148.90424599672));
#70019=CARTESIAN_POINT('Ctrl Pts',(-0.742622404887226,7.96417992471234,
149.222477454967));
#70020=CARTESIAN_POINT('Ctrl Pts',(-6.02705982360509,4.39372101266743,149.487670336839));
#70021=CARTESIAN_POINT('Ctrl Pts',(-7.02604472395381,-0.14781019150323,
149.699824642337));
#70022=CARTESIAN_POINT('Ctrl Pts',(-5.83694466737079,-4.643318603884,149.911978947835));
#70023=CARTESIAN_POINT('Ctrl Pts',(-0.407007019060977,-7.988355204186,150.177171829707));
#70024=CARTESIAN_POINT('Ctrl Pts',(6.50606889048119,-4.65193452158739,150.495403287954));
#70025=CARTESIAN_POINT('Ctrl Pts',(7.42645459139895,2.95401266902674,150.813634746201));
#70026=CARTESIAN_POINT('Ctrl Pts',(1.53328191626781,7.84967999940523,151.131866204448));
#70027=CARTESIAN_POINT('Ctrl Pts',(-5.78257511906035,5.52641320801365,151.450097662695));
#70028=CARTESIAN_POINT('Ctrl Pts',(-7.43175585864685,-0.634639310737093,
151.715290544567));
#70029=CARTESIAN_POINT('Ctrl Pts',(-5.20769272559132,-4.71821693561009,
151.927444850065));
#70030=CARTESIAN_POINT('Ctrl Pts',(-1.3632546876904,-7.33369535060035,152.139599155562));
#70031=CARTESIAN_POINT('Ctrl Pts',(4.93206728293985,-6.29700846122896,152.404792037435));
#70032=CARTESIAN_POINT('Ctrl Pts',(7.95995131862168,0.751309809408091,152.723023495682));
#70033=CARTESIAN_POINT('Ctrl Pts',(3.67501525946745,7.10394148213151,153.041254953929));
#70034=CARTESIAN_POINT('Ctrl Pts',(-3.99821329042567,6.92411285836137,153.359486412175));
#70035=CARTESIAN_POINT('Ctrl Pts',(-7.30894614683688,1.48602192463945,153.624679294048));
#70036=CARTESIAN_POINT('Ctrl Pts',(-6.32629632928619,-3.07755403250854,
153.836847387308));
#70037=CARTESIAN_POINT('Ctrl Pts',(-4.84151887665322,-4.85041839127279,
153.94293832782));
#70038=CARTESIAN_POINT('Ctrl Pts',(-3.92409368265873,-5.50444119324983,
153.995990691956));
#70039=CARTESIAN_POINT('Ctrl Pts',(-3.08954740555787,6.44311816685693,-0.44193303580599));
#70040=CARTESIAN_POINT('Ctrl Pts',(-4.16319062916384,5.92829528072251,-0.388891808959014));
#70041=CARTESIAN_POINT('Ctrl Pts',(-6.03043332774519,4.35125203191573,-0.282812005737566));
#70042=CARTESIAN_POINT('Ctrl Pts',(-7.88075233109425,-0.222852525913893,
-0.0706550497671821));
#70043=CARTESIAN_POINT('Ctrl Pts',(-5.41860073246465,-6.48603369603572,
0.194537832105166));
#70044=CARTESIAN_POINT('Ctrl Pts',(2.5395922108837,-8.06399520298082,0.512769290351983));
#70045=CARTESIAN_POINT('Ctrl Pts',(8.15320687002302,-2.22505886794282,0.831000748598799));
#70046=CARTESIAN_POINT('Ctrl Pts',(6.27744628296401,5.66372553892937,1.14923220684562));
#70047=CARTESIAN_POINT('Ctrl Pts',(-0.0905190406078649,7.88427553034339,
1.41442508871796));
#70048=CARTESIAN_POINT('Ctrl Pts',(-4.56808658365247,5.85731890654616,1.62657939421585));
#70049=CARTESIAN_POINT('Ctrl Pts',(-7.6242973326671,2.00783018015323,1.83873369971372));
#70050=CARTESIAN_POINT('Ctrl Pts',(-7.0234902137228,-4.70709375975071,2.10392658158607));
#70051=CARTESIAN_POINT('Ctrl Pts',(0.174066138808668,-8.45242981178917,
2.42215803983288));
#70052=CARTESIAN_POINT('Ctrl Pts',(7.19841503602263,-4.42222996039016,2.74038949807971));
#70053=CARTESIAN_POINT('Ctrl Pts',(7.6184358430781,3.66529927552298,3.05862095632652));
#70054=CARTESIAN_POINT('Ctrl Pts',(1.02395302145998,8.39271879730463,3.37685241457334));
#70055=CARTESIAN_POINT('Ctrl Pts',(-5.23695462670971,5.89336609917461,3.64204529644568));
#70056=CARTESIAN_POINT('Ctrl Pts',(-7.2900284264346,1.42732283980118,3.85419960194356));
#70057=CARTESIAN_POINT('Ctrl Pts',(-7.07280455631803,-3.48321488042714,
4.06635390744144));
#70058=CARTESIAN_POINT('Ctrl Pts',(-2.2167783250272,-8.1591849761286,4.33154678931379));
#70059=CARTESIAN_POINT('Ctrl Pts',(5.67364854670524,-6.26775735988919,4.6497782475606));
#70060=CARTESIAN_POINT('Ctrl Pts',(8.33459469622863,1.38096864477367,4.96800970580742));
#70061=CARTESIAN_POINT('Ctrl Pts',(3.34892244672672,7.76271866306914,5.28624116405423));
#70062=CARTESIAN_POINT('Ctrl Pts',(-4.72987836523322,7.00818389443088,5.60447262230106));
#70063=CARTESIAN_POINT('Ctrl Pts',(-7.81826678136539,1.0158975263293,5.8696655041734));
#70064=CARTESIAN_POINT('Ctrl Pts',(-6.44009876682224,-3.7022866893791,6.08181980967128));
#70065=CARTESIAN_POINT('Ctrl Pts',(-3.05631451379665,-7.26748127780818,
6.29397411516916));
#70066=CARTESIAN_POINT('Ctrl Pts',(3.67611324854931,-7.61397296209672,6.55916699704151));
#70067=CARTESIAN_POINT('Ctrl Pts',(8.39347630220861,-1.01224335435673,6.87739845528832));
#70068=CARTESIAN_POINT('Ctrl Pts',(5.38742321439901,6.50755034044391,7.19562991353514));
#70069=CARTESIAN_POINT('Ctrl Pts',(-2.56134958238959,8.05695782776883,7.51386137178195));
#70070=CARTESIAN_POINT('Ctrl Pts',(-8.16638379749588,2.19010693620455,7.83209283002878));
#70071=CARTESIAN_POINT('Ctrl Pts',(-6.56916827614357,-4.35928558519119,
8.09728571190112));
#70072=CARTESIAN_POINT('Ctrl Pts',(-2.43496001820217,-7.01803167674481,
8.309440017399));
#70073=CARTESIAN_POINT('Ctrl Pts',(2.4575588939521,-7.49117794035554,8.52159432289688));
#70074=CARTESIAN_POINT('Ctrl Pts',(7.76796194168394,-3.33843676059349,8.78678720476922));
#70075=CARTESIAN_POINT('Ctrl Pts',(7.00107523470319,4.73920105696399,9.10501866301604));
#70076=CARTESIAN_POINT('Ctrl Pts',(-0.199216385661401,8.44587788003586,
9.42325012126286));
#70077=CARTESIAN_POINT('Ctrl Pts',(-7.21673588746628,4.40383971450563,9.74148157950967));
#70078=CARTESIAN_POINT('Ctrl Pts',(-7.60192050859073,-3.7009724819277,10.0597130377566));
#70079=CARTESIAN_POINT('Ctrl Pts',(-2.10162734494506,-7.5987173362343,10.3249059196288));
#70080=CARTESIAN_POINT('Ctrl Pts',(2.7631423545712,-6.89542190392953,10.5370602251268));
#70081=CARTESIAN_POINT('Ctrl Pts',(6.76739677982186,-4.04471055546355,10.7492145306247));
#70082=CARTESIAN_POINT('Ctrl Pts',(8.05404140503811,2.5727047589792,11.0144074124969));
#70083=CARTESIAN_POINT('Ctrl Pts',(2.17862688248009,8.16876159569394,11.3326388707437));
#70084=CARTESIAN_POINT('Ctrl Pts',(-5.6882536018224,6.24630381060562,11.6508703289905));
#70085=CARTESIAN_POINT('Ctrl Pts',(-8.33641596472343,-1.40685818882059,
11.9691017872373));
#70086=CARTESIAN_POINT('Ctrl Pts',(-3.31303691185947,-7.7788289061784,12.2873332454843));
#70087=CARTESIAN_POINT('Ctrl Pts',(3.3955670207164,-7.11529811468617,12.5525261273565));
#70088=CARTESIAN_POINT('Ctrl Pts',(6.607494252704,-3.39452774407344,12.7646804328544));
#70089=CARTESIAN_POINT('Ctrl Pts',(7.76167381937667,1.38338793352998,12.9768347383524));
#70090=CARTESIAN_POINT('Ctrl Pts',(4.3941922927382,7.22339718037018,13.2420276202246));
#70091=CARTESIAN_POINT('Ctrl Pts',(-3.71119940327893,7.59618852382226,13.5602590784714));
#70092=CARTESIAN_POINT('Ctrl Pts',(-8.3904362061758,0.986468754258332,13.8784905367182));
#70093=CARTESIAN_POINT('Ctrl Pts',(-5.37182327508643,-6.52829195131364,
14.1967219949651));
#70094=CARTESIAN_POINT('Ctrl Pts',(2.59900782415898,-8.04559202674982,14.5149534532119));
#70095=CARTESIAN_POINT('Ctrl Pts',(7.22916614717721,-3.14587022452307,14.7801463350843));
#70096=CARTESIAN_POINT('Ctrl Pts',(7.21462658934175,1.76945248061757,14.9923006405821));
#70097=CARTESIAN_POINT('Ctrl Pts',(4.95326237263331,6.13372109904654,15.20445494608));
#70098=CARTESIAN_POINT('Ctrl Pts',(-1.41851003486382,8.33511979589558,15.4696478279523));
#70099=CARTESIAN_POINT('Ctrl Pts',(-7.78279220363034,3.30200342450728,15.7878792861993));
#70100=CARTESIAN_POINT('Ctrl Pts',(-6.98187982577724,-4.75666841722636,
16.1061107444459));
#70101=CARTESIAN_POINT('Ctrl Pts',(0.224594842153657,-8.45130985452697,
16.4243422026929));
#70102=CARTESIAN_POINT('Ctrl Pts',(7.23771676190491,-4.37056618819351,16.7425736609397));
#70103=CARTESIAN_POINT('Ctrl Pts',(7.52096906921939,2.36481857927387,17.0077665428119));
#70104=CARTESIAN_POINT('Ctrl Pts',(4.28708610892083,6.06652219970378,17.2199208483098));
#70105=CARTESIAN_POINT('Ctrl Pts',(-0.281908331501364,7.87895109425512,
17.4320751538077));
#70106=CARTESIAN_POINT('Ctrl Pts',(-6.53623961524628,5.36320467845715,17.6972680356801));
#70107=CARTESIAN_POINT('Ctrl Pts',(-8.04134995603776,-2.6099371610976,18.015499493927));
#70108=CARTESIAN_POINT('Ctrl Pts',(-2.15268059899722,-8.16936390251621,
18.3337309521738));
#70109=CARTESIAN_POINT('Ctrl Pts',(5.71097687179014,-6.23376485522393,18.6519624104205));
#70110=CARTESIAN_POINT('Ctrl Pts',(8.33044027974437,1.44573769285852,18.9701938686673));
#70111=CARTESIAN_POINT('Ctrl Pts',(4.12801234393877,6.71690827251071,19.2353867505397));
#70112=CARTESIAN_POINT('Ctrl Pts',(-0.740832893651014,7.39141160594412,
19.4475410560375));
#70113=CARTESIAN_POINT('Ctrl Pts',(-5.37896326430388,5.76403477212821,19.6596953615354));
#70114=CARTESIAN_POINT('Ctrl Pts',(-8.45165952544785,-0.236313344621609,
19.9248882434079));
#70115=CARTESIAN_POINT('Ctrl Pts',(-4.36019707337875,-7.24318732200448,
20.2431197016547));
#70116=CARTESIAN_POINT('Ctrl Pts',(3.73118465974708,-7.57963068809433,20.5613511599015));
#70117=CARTESIAN_POINT('Ctrl Pts',(8.39937144392063,-0.962102098219144,
20.8795826181483));
#70118=CARTESIAN_POINT('Ctrl Pts',(5.34181870698094,6.55372913940518,21.197814076395));
#70119=CARTESIAN_POINT('Ctrl Pts',(-1.28738765542055,7.77817302955547,21.4630069582675));
#70120=CARTESIAN_POINT('Ctrl Pts',(-5.40579452639309,5.09501564700433,21.6751612637654));
#70121=CARTESIAN_POINT('Ctrl Pts',(-7.84069466388574,0.825136255867873,
21.8873155692632));
#70122=CARTESIAN_POINT('Ctrl Pts',(-6.22634521833476,-5.7200540166208,22.1525084511356));
#70123=CARTESIAN_POINT('Ctrl Pts',(1.45715369581518,-8.32777186329684,22.4707399093824));
#70124=CARTESIAN_POINT('Ctrl Pts',(7.78702502643142,-3.27639765150152,22.7889713676291));
#70125=CARTESIAN_POINT('Ctrl Pts',(6.97264937688021,4.78092478161278,23.107202825876));
#70126=CARTESIAN_POINT('Ctrl Pts',(-0.263928110367578,8.45084224698918,
23.4254342841228));
#70127=CARTESIAN_POINT('Ctrl Pts',(-6.07205589142636,5.02866581753332,23.6906271659952));
#70128=CARTESIAN_POINT('Ctrl Pts',(-7.42228714546869,0.302411036523226,
23.902781471493));
#70129=CARTESIAN_POINT('Ctrl Pts',(-6.46102277639563,-4.51802250281368,
24.1149357769908));
#70130=CARTESIAN_POINT('Ctrl Pts',(-0.950548267340358,-8.40136005194374,
24.3801286588633));
#70131=CARTESIAN_POINT('Ctrl Pts',(6.56059897106672,-5.33231865525546,24.6983601171101));
#70132=CARTESIAN_POINT('Ctrl Pts',(8.02775655195335,2.63204579663869,25.0165915753568));
#70133=CARTESIAN_POINT('Ctrl Pts',(2.12980675111955,8.18162601829445,25.3348230336038));
#70134=CARTESIAN_POINT('Ctrl Pts',(-5.74036823307002,6.20762154771861,25.6530544918505));
#70135=CARTESIAN_POINT('Ctrl Pts',(-7.88183268470767,-0.184543174642897,
25.9182473737229));
#70136=CARTESIAN_POINT('Ctrl Pts',(-5.80236750001345,-4.63835426628759,
26.1304016792208));
#70137=CARTESIAN_POINT('Ctrl Pts',(-1.91589231730585,-7.6476597257934,26.3425559847187));
#70138=CARTESIAN_POINT('Ctrl Pts',(4.79095222080362,-6.96657516638674,26.607748866591));
#70139=CARTESIAN_POINT('Ctrl Pts',(8.44980016043421,0.275605422791958,26.9259803248378));
#70140=CARTESIAN_POINT('Ctrl Pts',(4.33543727924364,7.25096710313725,27.2442117830847));
#70141=CARTESIAN_POINT('Ctrl Pts',(-3.75649528803494,7.57389095850464,27.5624432413314));
#70142=CARTESIAN_POINT('Ctrl Pts',(-8.40442114458738,0.923091520571846,
27.8806746995783));
#70143=CARTESIAN_POINT('Ctrl Pts',(-5.83005137872459,-5.30733865270204,
28.1458675814506));
#70144=CARTESIAN_POINT('Ctrl Pts',(-1.33968524960494,-7.30664371218358,
28.3580218869484));
#70145=CARTESIAN_POINT('Ctrl Pts',(3.56789413603829,-7.030467558211,28.5701761924464));
#70146=CARTESIAN_POINT('Ctrl Pts',(8.18521430748699,-2.11864566915973,28.8353690743186));
#70147=CARTESIAN_POINT('Ctrl Pts',(6.19917809397479,5.74850172301705,29.1536005325656));
#70148=CARTESIAN_POINT('Ctrl Pts',(-1.48094927695439,8.31741123019191,29.4718319908123));
#70149=CARTESIAN_POINT('Ctrl Pts',(-7.80237196108085,3.25546815086346,29.7900634490592));
#70150=CARTESIAN_POINT('Ctrl Pts',(-6.95088340951852,-4.81369011863248,
30.108294907306));
#70151=CARTESIAN_POINT('Ctrl Pts',(-0.92194426360296,-7.82990175084229,
30.3734877891782));
#70152=CARTESIAN_POINT('Ctrl Pts',(3.77935100285112,-6.39517825412621,30.5856420946763));
#70153=CARTESIAN_POINT('Ctrl Pts',(7.30365686831716,-2.96882788368026,30.797796400174));
#70154=CARTESIAN_POINT('Ctrl Pts',(7.56928208179731,3.76727507585018,31.0629892820465));
#70155=CARTESIAN_POINT('Ctrl Pts',(0.911383413585489,8.40502595913824,31.3812207402932));
#70156=CARTESIAN_POINT('Ctrl Pts',(-6.57177213448138,5.30889360841674,31.6994521985401));
#70157=CARTESIAN_POINT('Ctrl Pts',(-8.02562084627201,-2.65791104671155,
32.0176836567869));
#70158=CARTESIAN_POINT('Ctrl Pts',(-2.09188894873834,-8.19209334401688,
32.3359151150337));
#70159=CARTESIAN_POINT('Ctrl Pts',(4.43785238624996,-6.51634934997266,32.6011079969061));
#70160=CARTESIAN_POINT('Ctrl Pts',(7.04676415458615,-2.35051352994202,32.8132623024038));
#70161=CARTESIAN_POINT('Ctrl Pts',(7.46112804553437,2.54733408511215,33.0254166079019));
#70162=CARTESIAN_POINT('Ctrl Pts',(3.24492014212853,7.80748909715203,33.2906094897741));
#70163=CARTESIAN_POINT('Ctrl Pts',(-4.82292670845914,6.94366323097387,33.6088409480209));
#70164=CARTESIAN_POINT('Ctrl Pts',(-8.44287682142809,-0.30061821506101,
33.9270724062678));
#70165=CARTESIAN_POINT('Ctrl Pts',(-4.31686528271657,-7.26909590191398,
34.2453038645147));
#70166=CARTESIAN_POINT('Ctrl Pts',(3.79198779968982,-7.55693200035196,34.5635353227614));
#70167=CARTESIAN_POINT('Ctrl Pts',(7.62340536575552,-2.01023214639604,34.8287282046339));
#70168=CARTESIAN_POINT('Ctrl Pts',(6.86174558348796,2.845741810545,35.0408825101316));
#70169=CARTESIAN_POINT('Ctrl Pts',(3.96315757784307,6.81547684804362,35.2530368156296));
#70170=CARTESIAN_POINT('Ctrl Pts',(-2.66923038574688,8.02256828445513,35.5182296975018));
#70171=CARTESIAN_POINT('Ctrl Pts',(-8.19433312038786,2.08038116999304,35.8364611557488));
#70172=CARTESIAN_POINT('Ctrl Pts',(-6.17755021440263,-5.76284770591486,
36.1546926139953));
#70173=CARTESIAN_POINT('Ctrl Pts',(1.50685855823589,-8.31892170811928,36.4729240722423));
#70174=CARTESIAN_POINT('Ctrl Pts',(7.81805028258378,-3.21939163661875,36.791155530489));
#70175=CARTESIAN_POINT('Ctrl Pts',(7.07401192966089,3.48076110528274,37.0563484123616));
#70176=CARTESIAN_POINT('Ctrl Pts',(3.31494171537135,6.64777860104349,37.2685027178592));
#70177=CARTESIAN_POINT('Ctrl Pts',(-1.47648862131544,7.74450282485324,37.4806570233573));
#70178=CARTESIAN_POINT('Ctrl Pts',(-7.27564087051258,4.30713856919719,37.7458499052295));
#70179=CARTESIAN_POINT('Ctrl Pts',(-7.55107762627309,-3.80214515534913,
38.0640813634764));
#70180=CARTESIAN_POINT('Ctrl Pts',(-0.88564717289864,-8.40167658376415,
38.3823128217233));
#70181=CARTESIAN_POINT('Ctrl Pts',(6.59232492751021,-5.29304573478011,38.70054427997));
#70182=CARTESIAN_POINT('Ctrl Pts',(8.0138036740729,2.69543009635854,39.0187757382169));
#70183=CARTESIAN_POINT('Ctrl Pts',(3.05883722745604,7.26641985223558,39.2839686200891));
#70184=CARTESIAN_POINT('Ctrl Pts',(-1.85595651526812,7.19285925889241,39.4961229255871));
#70185=CARTESIAN_POINT('Ctrl Pts',(-6.19275653750488,4.87925292644519,39.7082772310848));
#70186=CARTESIAN_POINT('Ctrl Pts',(-8.317485720007,-1.51849400012624,39.9734701129573));
#70187=CARTESIAN_POINT('Ctrl Pts',(-3.20831135435621,-7.82188080667661,
40.2917015712041));
#70188=CARTESIAN_POINT('Ctrl Pts',(4.84016231529167,-6.92425946182438,40.6099330294509));
#70189=CARTESIAN_POINT('Ctrl Pts',(8.44800366551446,0.326060067780617,40.9281644876977));
#70190=CARTESIAN_POINT('Ctrl Pts',(4.28334222170055,7.28967572274216,41.2463959459445));
#70191=CARTESIAN_POINT('Ctrl Pts',(-2.45495818169829,7.4920306312205,41.5115888278169));
#70192=CARTESIAN_POINT('Ctrl Pts',(-6.11756318896782,4.21393160051117,41.7237431333147));
#70193=CARTESIAN_POINT('Ctrl Pts',(-7.87499796254952,-0.376496670469604,
41.9358974388127));
#70194=CARTESIAN_POINT('Ctrl Pts',(-5.28433232576479,-6.60016852828897,
42.2010903206851));
#70195=CARTESIAN_POINT('Ctrl Pts',(2.70630770751061,-8.00943067218986,42.5193217789319));
#70196=CARTESIAN_POINT('Ctrl Pts',(8.19462382668053,-2.05442952476689,42.8375532371787));
#70197=CARTESIAN_POINT('Ctrl Pts',(6.16473930713995,5.78541877268626,43.1557846954255));
#70198=CARTESIAN_POINT('Ctrl Pts',(-1.54566350454616,8.31247959766842,43.4740161536723));
#70199=CARTESIAN_POINT('Ctrl Pts',(-6.76599224978972,4.04705961517972,43.7392090355446));
#70200=CARTESIAN_POINT('Ctrl Pts',(-7.38198296145935,-0.829533882083435,
43.9513633410425));
#70201=CARTESIAN_POINT('Ctrl Pts',(-5.6990298339995,-5.44778868938746,44.1635176465404));
#70202=CARTESIAN_POINT('Ctrl Pts',(0.337781924161787,-8.44821259809727,
44.4287105284128));
#70203=CARTESIAN_POINT('Ctrl Pts',(7.29502137845032,-4.27290816520776,44.7469419866596));
#70204=CARTESIAN_POINT('Ctrl Pts',(7.53428100585627,3.82193014821406,45.0651734449063));
#70205=CARTESIAN_POINT('Ctrl Pts',(0.861174981281068,8.41031858801809,45.3834049031532));
#70206=CARTESIAN_POINT('Ctrl Pts',(-6.61739999361422,5.26273788587781,45.7016363613999));
#70207=CARTESIAN_POINT('Ctrl Pts',(-7.76215359514146,-1.38069338321955,
45.9668292432723));
#70208=CARTESIAN_POINT('Ctrl Pts',(-5.02973675869332,-5.46658458665463,
46.1789835487703));
#70209=CARTESIAN_POINT('Ctrl Pts',(-0.730927478072492,-7.85003743142875,
46.3911378542681));
#70210=CARTESIAN_POINT('Ctrl Pts',(5.79440616976952,-6.15721120887338,46.6563307361405));
#70211=CARTESIAN_POINT('Ctrl Pts',(8.30967429282036,1.55704664271416,46.9745621943871));
#70212=CARTESIAN_POINT('Ctrl Pts',(3.18265660064284,7.82580585597539,47.2927936526342));
#70213=CARTESIAN_POINT('Ctrl Pts',(-4.86430609374981,6.91473841346546,47.6110251108809));
#70214=CARTESIAN_POINT('Ctrl Pts',(-8.44706378669732,-0.365384885300918,
47.9292565691279));
#70215=CARTESIAN_POINT('Ctrl Pts',(-4.95539139693606,-6.13200120321307,
48.194449451));
#70216=CARTESIAN_POINT('Ctrl Pts',(-0.213264087965808,-7.42538331223274,
48.406603756498));
#70217=CARTESIAN_POINT('Ctrl Pts',(4.59527927258509,-6.40630557029426,48.6187580619957));
#70218=CARTESIAN_POINT('Ctrl Pts',(8.41216831688165,-0.849598104630865,
48.8839509438682));
#70219=CARTESIAN_POINT('Ctrl Pts',(5.25315602768194,6.62415525551567,49.202182402115));
#70220=CARTESIAN_POINT('Ctrl Pts',(-2.72825152258647,7.99557277263729,49.5204138603617));
#70221=CARTESIAN_POINT('Ctrl Pts',(-8.20661039441647,2.03141008528623,49.8386453186087));
#70222=CARTESIAN_POINT('Ctrl Pts',(-6.13824495963909,-5.81449409204312,
50.1568767768553));
#70223=CARTESIAN_POINT('Ctrl Pts',(0.279173134727941,-7.87904848404171,
50.4220696587278));
#70224=CARTESIAN_POINT('Ctrl Pts',(4.70769337698525,-5.74625286365732,50.6342239642257));
#70225=CARTESIAN_POINT('Ctrl Pts',(7.67011396254657,-1.82392282034684,50.8463782697236));
#70226=CARTESIAN_POINT('Ctrl Pts',(6.90854423367506,4.87425987225694,51.1115711515959));
#70227=CARTESIAN_POINT('Ctrl Pts',(-0.377048842699031,8.44588155674506,
51.4298026098427));
#70228=CARTESIAN_POINT('Ctrl Pts',(-7.3025032886826,4.24805673829975,51.7480340680896));
#70229=CARTESIAN_POINT('Ctrl Pts',(-7.52823776577549,-3.84717003033372,
52.0662655263364));
#70230=CARTESIAN_POINT('Ctrl Pts',(-0.822106580473215,-8.41489949442549,
52.3844969845832));
#70231=CARTESIAN_POINT('Ctrl Pts',(5.37696195411409,-5.76590173321082,52.6496898664556));
#70232=CARTESIAN_POINT('Ctrl Pts',(7.32220357060287,-1.25185213801433,52.8618441719534));
#70233=CARTESIAN_POINT('Ctrl Pts',(6.9871182240826,3.65205717038036,53.0739984774512));
#70234=CARTESIAN_POINT('Ctrl Pts',(2.02020672062951,8.21006440515927,53.3391913593236));
#70235=CARTESIAN_POINT('Ctrl Pts',(-5.82252560851519,6.12970444952542,53.6574228175704));
#70236=CARTESIAN_POINT('Ctrl Pts',(-8.29902867471625,-1.58071610014923,
53.9756542758171));
#70237=CARTESIAN_POINT('Ctrl Pts',(-3.16154432641485,-7.8409003674617,54.2938857340642));
#70238=CARTESIAN_POINT('Ctrl Pts',(4.89680770770741,-6.89258057658212,54.6121171923107));
#70239=CARTESIAN_POINT('Ctrl Pts',(7.84040774518007,-0.827858105205332,
54.8773100741832));
#70240=CARTESIAN_POINT('Ctrl Pts',(6.34933559551319,3.85587038168426,55.0894643796811));
#70241=CARTESIAN_POINT('Ctrl Pts',(2.88091318290485,7.33877931849697,55.3016186851791));
#70242=CARTESIAN_POINT('Ctrl Pts',(-3.85789369862079,7.52349978009444,55.5668115670513));
#70243=CARTESIAN_POINT('Ctrl Pts',(-8.41536367707005,0.810392055117173,
55.8850430252982));
#70244=CARTESIAN_POINT('Ctrl Pts',(-5.22959850487317,-6.63504633072462,
56.203274483545));
#70245=CARTESIAN_POINT('Ctrl Pts',(2.75408926280945,-7.99312663685644,56.5215059417917));
#70246=CARTESIAN_POINT('Ctrl Pts',(8.21662165708924,-1.99336932734302,56.8397374000387));
#70247=CARTESIAN_POINT('Ctrl Pts',(6.46259081968553,4.51577928494635,57.1049302819109));
#70248=CARTESIAN_POINT('Ctrl Pts',(2.2657281167326,7.07448054671492,57.3170845874089));
#70249=CARTESIAN_POINT('Ctrl Pts',(-2.63674197143089,7.43000231689924,57.5292388929067));
#70250=CARTESIAN_POINT('Ctrl Pts',(-7.8458904765042,3.1509356327352,57.794431774779));
#70251=CARTESIAN_POINT('Ctrl Pts',(-6.88525000770043,-4.90595693334218,
58.1126632330257));
#70252=CARTESIAN_POINT('Ctrl Pts',(0.401976697758393,-8.43865836892884,
58.4308946912727));
#70253=CARTESIAN_POINT('Ctrl Pts',(7.3204077721116,-4.22926839422082,58.7491261495195));
#70254=CARTESIAN_POINT('Ctrl Pts',(7.5108538442389,3.88245634378822,59.0673576077664));
#70255=CARTESIAN_POINT('Ctrl Pts',(1.91854708879243,7.64699416248759,59.3325504896385));
#70256=CARTESIAN_POINT('Ctrl Pts',(-2.92793093379394,6.82707985537983,59.5447047951366));
#70257=CARTESIAN_POINT('Ctrl Pts',(-6.86257418017123,3.88103314526963,59.7568591006344));
#70258=CARTESIAN_POINT('Ctrl Pts',(-7.98993837505287,-2.76537113129454,
60.0220519825068));
#70259=CARTESIAN_POINT('Ctrl Pts',(-1.98183548353321,-8.21872308917607,
60.3402834407536));
#70260=CARTESIAN_POINT('Ctrl Pts',(5.83661085443811,-6.10790586591585,60.6585148990004));
#70261=CARTESIAN_POINT('Ctrl Pts',(8.30022793095247,1.6066416509548,60.9767463572473));
#70262=CARTESIAN_POINT('Ctrl Pts',(3.1252821513995,7.85614435999515,61.294977815494));
#70263=CARTESIAN_POINT('Ctrl Pts',(-3.5654532925281,7.03170572989474,61.5601706973665));
#70264=CARTESIAN_POINT('Ctrl Pts',(-6.68710439400672,3.23487769914977,61.7723250028642));
#70265=CARTESIAN_POINT('Ctrl Pts',(-7.72621513627836,-1.56937641150137,
61.9844793083622));
#70266=CARTESIAN_POINT('Ctrl Pts',(-4.21946379145455,-7.32683547266784,
62.2496721902343));
#70267=CARTESIAN_POINT('Ctrl Pts',(3.89254266914332,-7.5048779250062,62.5679036484814));
#70268=CARTESIAN_POINT('Ctrl Pts',(8.41170550821265,-0.784697888450407,
62.886135106728));
#70269=CARTESIAN_POINT('Ctrl Pts',(5.2135049805116,6.6554073442974,63.2043665649751));
#70270=CARTESIAN_POINT('Ctrl Pts',(-2.79146370955416,7.98085979636165,63.5225980232217));
#70271=CARTESIAN_POINT('Ctrl Pts',(-7.30262579890221,2.97136317104487,63.7877909050942));
#70272=CARTESIAN_POINT('Ctrl Pts',(-7.17005477688813,-1.94219293614828,
63.999945210592));
#70273=CARTESIAN_POINT('Ctrl Pts',(-4.80453993183803,-6.25089903105207,
64.2120995160899));
#70274=CARTESIAN_POINT('Ctrl Pts',(1.61825901095675,-8.29865233061352,64.4772923979622));
#70275=CARTESIAN_POINT('Ctrl Pts',(7.85984155839847,-3.11415667191275,64.7955238562089));
#70276=CARTESIAN_POINT('Ctrl Pts',(6.86564067621341,4.92295830148474,65.1137553144559));
#70277=CARTESIAN_POINT('Ctrl Pts',(-0.427478278208905,8.44347934337543,
65.4319867727027));
#70278=CARTESIAN_POINT('Ctrl Pts',(-7.34058357188119,4.19550063224483,65.7502182309494));
#70279=CARTESIAN_POINT('Ctrl Pts',(-7.46201190359825,-2.54474379920436,
66.0154111128219));
#70280=CARTESIAN_POINT('Ctrl Pts',(-4.14016947758362,-6.1677220755876,66.2275654183197));
#70281=CARTESIAN_POINT('Ctrl Pts',(0.471030721693415,-7.86990932045876,
66.4397197238176));
#70282=CARTESIAN_POINT('Ctrl Pts',(6.66314575093835,-5.20469801551421,66.7049126056898));
#70283=CARTESIAN_POINT('Ctrl Pts',(7.97635649386006,2.80228802645955,67.0231440639369));
#70284=CARTESIAN_POINT('Ctrl Pts',(1.95588221857694,8.21870215301671,67.3413755221834));
#70285=CARTESIAN_POINT('Ctrl Pts',(-5.8590264634452,6.09482485400949,67.6596069804306));
#70286=CARTESIAN_POINT('Ctrl Pts',(-8.29332032393845,-1.6453664441987,67.9778384386769));
#70287=CARTESIAN_POINT('Ctrl Pts',(-3.96552333346447,-6.814100626219,68.2430313205496));
#70288=CARTESIAN_POINT('Ctrl Pts',(0.918115258484746,-7.37148989536762,
68.4551856260474));
#70289=CARTESIAN_POINT('Ctrl Pts',(5.51582858788926,-5.63320314221727,68.6673399315454));
#70290=CARTESIAN_POINT('Ctrl Pts',(8.44354750738623,0.439201798094404,68.9325328134176));
#70291=CARTESIAN_POINT('Ctrl Pts',(4.18500313876025,7.34580355275531,69.2507642716645));
#70292=CARTESIAN_POINT('Ctrl Pts',(-3.91212454590034,7.48784494118263,69.5689957299112));
#70293=CARTESIAN_POINT('Ctrl Pts',(-8.42005303224499,0.760123691181521,
69.8872271881581));
#70294=CARTESIAN_POINT('Ctrl Pts',(-5.18289822219567,-6.68011667524811,
70.2054586464048));
#70295=CARTESIAN_POINT('Ctrl Pts',(1.47380002847441,-7.74501491729134,70.4706515282772));
#70296=CARTESIAN_POINT('Ctrl Pts',(5.5265864071793,-4.96373262914806,70.682805833775));
#70297=CARTESIAN_POINT('Ctrl Pts',(7.85824829472714,-0.636613292568681,
70.8949601392731));
#70298=CARTESIAN_POINT('Ctrl Pts',(6.08718936490711,5.86792278728112,71.1601530211452));
#70299=CARTESIAN_POINT('Ctrl Pts',(-1.65671505113536,8.29037858484482,71.4783844793922));
#70300=CARTESIAN_POINT('Ctrl Pts',(-7.86345831407396,3.08845654589225,71.7966159376389));
#70301=CARTESIAN_POINT('Ctrl Pts',(-6.85583031447803,-4.94698584078679,
72.1148473958858));
#70302=CARTESIAN_POINT('Ctrl Pts',(0.46678880254388,-8.4420676698729,72.4330788541326));
#70303=CARTESIAN_POINT('Ctrl Pts',(6.19106263133698,-4.88140185344963,72.698271736005));
#70304=CARTESIAN_POINT('Ctrl Pts',(7.42740839776675,-0.124087184035522,
72.9104260415028));
#70305=CARTESIAN_POINT('Ctrl Pts',(6.35066560502015,4.67187537753541,73.1225803470006));
#70306=CARTESIAN_POINT('Ctrl Pts',(0.748523360428059,8.42175950261246,73.3877732288731));
#70307=CARTESIAN_POINT('Ctrl Pts',(-6.6867529066314,5.17324284008979,73.7060046871199));
#70308=CARTESIAN_POINT('Ctrl Pts',(-7.96224246790876,-2.82407647742015,
74.0242361453667));
#70309=CARTESIAN_POINT('Ctrl Pts',(-1.93270844683755,-8.23038755417868,
74.3424676036136));
#70310=CARTESIAN_POINT('Ctrl Pts',(5.88775761908401,-6.06803068999685,74.6606990618602));
#70311=CARTESIAN_POINT('Ctrl Pts',(7.8751699986775,0.373845663894274,74.9258919437329));
#70312=CARTESIAN_POINT('Ctrl Pts',(5.68925384822416,4.77624310663567,75.1380462492305));
#70313=CARTESIAN_POINT('Ctrl Pts',(1.73182621837097,7.69173142340001,75.3502005547285));
#70314=CARTESIAN_POINT('Ctrl Pts',(-4.95715323779993,6.84894556265586,75.6153934366008));
#70315=CARTESIAN_POINT('Ctrl Pts',(-8.44026112492043,-0.477479166752036,
75.9336248948477));
#70316=CARTESIAN_POINT('Ctrl Pts',(-4.16094718559222,-7.354736283558,76.2518563530945));
#70317=CARTESIAN_POINT('Ctrl Pts',(3.93895069415804,-7.47821303053569,76.5700878113412));
#70318=CARTESIAN_POINT('Ctrl Pts',(8.42096517841398,-0.727312659247321,
76.8883192695882));
#70319=CARTESIAN_POINT('Ctrl Pts',(5.16283025738198,6.69209880639428,77.2065507278348));
#70320=CARTESIAN_POINT('Ctrl Pts',(-2.83828883793128,7.95925522611546,77.5247821860818));
#70321=CARTESIAN_POINT('Ctrl Pts',(-8.23340234365653,1.91757139606222,77.8430136443285));
#70322=CARTESIAN_POINT('Ctrl Pts',(-6.05806050855332,-5.89756953481354,
78.1612451025754));
#70323=CARTESIAN_POINT('Ctrl Pts',(0.387359295838887,-7.87476394035296,
78.4264379844476));
#70324=CARTESIAN_POINT('Ctrl Pts',(4.78607026788089,-5.68098925840602,78.6385922899456));
#70325=CARTESIAN_POINT('Ctrl Pts',(7.69444850934977,-1.71858233013379,78.8507465954435));
#70326=CARTESIAN_POINT('Ctrl Pts',(6.8409884325102,4.96865811885738,79.1159394773158));
#70327=CARTESIAN_POINT('Ctrl Pts',(-0.492908969808402,8.43988637245421,
79.4341709355625));
#70328=CARTESIAN_POINT('Ctrl Pts',(-7.36011613232335,4.14745748462858,79.7524023938093));
#70329=CARTESIAN_POINT('Ctrl Pts',(-7.47473163377407,-3.95012568406894,
80.0706338520563));
#70330=CARTESIAN_POINT('Ctrl Pts',(-0.706552258280965,-8.4253845162857,
80.3888653103029));
#70331=CARTESIAN_POINT('Ctrl Pts',(5.45558212828763,-5.69157243751812,80.6540581921753));
#70332=CARTESIAN_POINT('Ctrl Pts',(7.33869306412585,-1.15125029728964,80.8662124976733));
#70333=CARTESIAN_POINT('Ctrl Pts',(6.93634303769482,3.74759734008634,81.0783668031711));
#70334=CARTESIAN_POINT('Ctrl Pts',(1.90734909302426,8.23701510052229,81.3435596850435));
#70335=CARTESIAN_POINT('Ctrl Pts',(-5.90609562851779,6.04922413509894,81.6617911432904));
#70336=CARTESIAN_POINT('Ctrl Pts',(-8.2765549435943,-1.69445529852785,81.9800226015371));
#70337=CARTESIAN_POINT('Ctrl Pts',(-3.05364538250673,-7.88354816809072,
82.298254059784));
#70338=CARTESIAN_POINT('Ctrl Pts',(4.99093394690154,-6.8247322686972,82.6164855180308));
#70339=CARTESIAN_POINT('Ctrl Pts',(7.85103020594809,-0.720185706015227,
82.8816783999031));
#70340=CARTESIAN_POINT('Ctrl Pts',(6.29582332753661,3.94263966881761,83.0938327054011));
#70341=CARTESIAN_POINT('Ctrl Pts',(2.77993132433371,7.37762322330055,83.3059870108988));
#70342=CARTESIAN_POINT('Ctrl Pts',(-3.96077592627955,7.46984918444621,83.5711798927711));
#70343=CARTESIAN_POINT('Ctrl Pts',(-8.42569230392369,0.694831124313766,
83.8894113510182));
#70344=CARTESIAN_POINT('Ctrl Pts',(-5.13805285591533,-6.70618767823044,
84.2076428092648));
#70345=CARTESIAN_POINT('Ctrl Pts',(2.8635201522212,-7.95457940088155,84.5258742675119));
#70346=CARTESIAN_POINT('Ctrl Pts',(8.24320307796721,-1.88042435219548,84.8441057257583));
#70347=CARTESIAN_POINT('Ctrl Pts',(6.4000119132817,4.60404063430321,85.1092986076311));
#70348=CARTESIAN_POINT('Ctrl Pts',(2.16843117645446,7.1049071167996,85.3214529131286));
#70349=CARTESIAN_POINT('Ctrl Pts',(-2.73845611678586,7.39311847253433,85.5336072186269));
#70350=CARTESIAN_POINT('Ctrl Pts',(-7.88839217017907,3.04296922439314,85.7988001004986));
#70351=CARTESIAN_POINT('Ctrl Pts',(-6.81727686636293,-4.99998172274208,
86.1170315587459));
#70352=CARTESIAN_POINT('Ctrl Pts',(0.517743138293131,-8.432347382295,86.4352630169924));
#70353=CARTESIAN_POINT('Ctrl Pts',(7.3777569833882,-4.12841167938097,86.7534944752395));
#70354=CARTESIAN_POINT('Ctrl Pts',(7.45686736189402,3.98516271663605,87.071725933486));
#70355=CARTESIAN_POINT('Ctrl Pts',(1.8134261971067,7.67260243207413,87.3369188153587));
#70356=CARTESIAN_POINT('Ctrl Pts',(-3.0213437124554,6.78625677940435,87.5490731208563));
#70357=CARTESIAN_POINT('Ctrl Pts',(-6.9151876472613,3.78649210433562,87.7612274263544));
#70358=CARTESIAN_POINT('Ctrl Pts',(-7.95123661705785,-2.87475720548686,
88.0264203082266));
#70359=CARTESIAN_POINT('Ctrl Pts',(-1.86886275660877,-8.2451460325035,88.3446517664734));
#70360=CARTESIAN_POINT('Ctrl Pts',(5.91988046063556,-6.02723449558902,88.6628832247204));
#70361=CARTESIAN_POINT('Ctrl Pts',(8.27739827918244,1.72039496283128,88.981114682967));
#70362=CARTESIAN_POINT('Ctrl Pts',(3.01717744396469,7.89829304359937,89.2993461412138));
#70363=CARTESIAN_POINT('Ctrl Pts',(-3.66161413346099,6.98211462170826,89.5645390230864));
#70364=CARTESIAN_POINT('Ctrl Pts',(-6.73086714842256,3.14280548794969,89.776693328584));
#70365=CARTESIAN_POINT('Ctrl Pts',(-7.7039509303132,-1.67525601516913,89.9888476340821));
#70366=CARTESIAN_POINT('Ctrl Pts',(-4.11851979208988,-7.38404952943188,
90.2540405159544));
#70367=CARTESIAN_POINT('Ctrl Pts',(3.9951660842497,-7.45075359004759,90.5722719742013));
#70368=CARTESIAN_POINT('Ctrl Pts',(8.42168187711568,-0.669189579787365,
90.890503432448));
#70369=CARTESIAN_POINT('Ctrl Pts',(5.12168143120076,6.72632592264454,91.2087348906947));
#70370=CARTESIAN_POINT('Ctrl Pts',(-2.9007227407555,7.94180082299996,91.5269663489418));
#70371=CARTESIAN_POINT('Ctrl Pts',(-7.34271436417314,2.870868931038,91.7921592308139));
#70372=CARTESIAN_POINT('Ctrl Pts',(-7.14272675520292,-2.04040520615619,
92.004313536312));
#70373=CARTESIAN_POINT('Ctrl Pts',(-4.71830598861224,-6.31624344455306,
92.2164678418096));
#70374=CARTESIAN_POINT('Ctrl Pts',(1.73198960680328,-8.27566340137542,92.4816607236824));
#70375=CARTESIAN_POINT('Ctrl Pts',(7.90183721812814,-3.00600227520748,92.7998921819287));
#70376=CARTESIAN_POINT('Ctrl Pts',(6.79743607045418,5.01671238971521,93.118123640176));
#70377=CARTESIAN_POINT('Ctrl Pts',(-0.543308475935934,8.43681794282195,
93.4363550984225));
#70378=CARTESIAN_POINT('Ctrl Pts',(-7.3974674859525,4.09437022327196,93.7545865566693));
#70379=CARTESIAN_POINT('Ctrl Pts',(-7.42638754234585,-2.64690587742072,
94.0197794385418));
#70380=CARTESIAN_POINT('Ctrl Pts',(-4.05513953841633,-6.22395711977298,
94.2319337440395));
#70381=CARTESIAN_POINT('Ctrl Pts',(0.578985677141032,-7.86270425735951,
94.4440880495374));
#70382=CARTESIAN_POINT('Ctrl Pts',(6.73394274200306,-5.11276910082636,94.70928093141));
#70383=CARTESIAN_POINT('Ctrl Pts',(7.93714940170376,2.91148423924637,95.0275123896566));
#70384=CARTESIAN_POINT('Ctrl Pts',(1.84291222287195,8.24476893986864,95.3457438479035));
#70385=CARTESIAN_POINT('Ctrl Pts',(-5.94211444723251,6.01384710450294,95.6639753061503));
#70386=CARTESIAN_POINT('Ctrl Pts',(-8.26995989960118,-1.75902131593898,
95.982206764397));
#70387=CARTESIAN_POINT('Ctrl Pts',(-3.87163954240068,-6.86787812259019,
96.2473996462695));
#70388=CARTESIAN_POINT('Ctrl Pts',(1.01918826962898,-7.35819639421587,96.4595539517673));
#70389=CARTESIAN_POINT('Ctrl Pts',(5.5926140224005,-5.55697858997884,96.6717082572652));
#70390=CARTESIAN_POINT('Ctrl Pts',(8.43672521784369,0.555031827501162,96.9369011391376));
#70391=CARTESIAN_POINT('Ctrl Pts',(4.08380208395726,7.40254291709361,97.2551325973842));
#70392=CARTESIAN_POINT('Ctrl Pts',(-4.01451237192768,7.43345348735528,97.5733640556311));
#70393=CARTESIAN_POINT('Ctrl Pts',(-8.42969138229406,0.644503141670811,
97.8915955138779));
#70394=CARTESIAN_POINT('Ctrl Pts',(-5.09073846592904,-6.7506129056886,98.2098269721248));
#70395=CARTESIAN_POINT('Ctrl Pts',(1.57994662075434,-7.72406054666849,98.475019853997));
#70396=CARTESIAN_POINT('Ctrl Pts',(5.59418364133663,-4.88742348193836,98.6871741594951));
#70397=CARTESIAN_POINT('Ctrl Pts',(7.86624459833887,-0.528714074088318,
98.8993284649929));
#70398=CARTESIAN_POINT('Ctrl Pts',(6.00609026407533,5.95090518078709,99.1645213468653));
#70399=CARTESIAN_POINT('Ctrl Pts',(-1.77032850893993,8.26686264980742,99.4827528051121));
#70400=CARTESIAN_POINT('Ctrl Pts',(-7.90510090403196,2.98025502769608,99.8009842633589));
#70401=CARTESIAN_POINT('Ctrl Pts',(-6.78729698533865,-5.04060321123964,
100.119215721606));
#70402=CARTESIAN_POINT('Ctrl Pts',(0.582596093550364,-8.43486659780217,
100.437447179853));
#70403=CARTESIAN_POINT('Ctrl Pts',(6.25746716822917,-4.79598241151577,100.702640061725));
#70404=CARTESIAN_POINT('Ctrl Pts',(7.42841223796564,-0.0221478586563569,
100.914794367223));
#70405=CARTESIAN_POINT('Ctrl Pts',(6.28595416952829,4.75858412047349,101.126948672721));
#70406=CARTESIAN_POINT('Ctrl Pts',(0.632882506249434,8.43124264057339,101.392141554594));
#70407=CARTESIAN_POINT('Ctrl Pts',(-6.75711940236345,5.08098597543341,101.71037301284));
#70408=CARTESIAN_POINT('Ctrl Pts',(-7.92273150330738,-2.93306424401754,
102.028604471087));
#70409=CARTESIAN_POINT('Ctrl Pts',(-1.81959200462792,-8.25615927880757,
102.346835929334));
#70410=CARTESIAN_POINT('Ctrl Pts',(5.9704984758136,-5.98661345680911,102.665067387581));
#70411=CARTESIAN_POINT('Ctrl Pts',(7.86925744826999,0.481798573971578,102.930260269453));
#70412=CARTESIAN_POINT('Ctrl Pts',(5.62322769431742,4.8539786982085,103.142414574951));
#70413=CARTESIAN_POINT('Ctrl Pts',(1.62597679404605,7.71450206547757,103.354568880449));
#70414=CARTESIAN_POINT('Ctrl Pts',(-5.05039432632765,6.78084875804923,103.619761762321));
#70415=CARTESIAN_POINT('Ctrl Pts',(-8.43338466048396,-0.594225772463747,
103.937993220568));
#70416=CARTESIAN_POINT('Ctrl Pts',(-4.05876638382929,-7.40938295504631,
104.256224678815));
#70417=CARTESIAN_POINT('Ctrl Pts',(4.03958841382724,-7.42676285788232,104.574456137062));
#70418=CARTESIAN_POINT('Ctrl Pts',(8.43326559218159,-0.605329813131043,
104.892687595308));
#70419=CARTESIAN_POINT('Ctrl Pts',(5.62565063348024,5.52353126206922,105.157880477181));
#70420=CARTESIAN_POINT('Ctrl Pts',(1.06304677918724,7.35198819708387,105.370034782679));
#70421=CARTESIAN_POINT('Ctrl Pts',(-3.83061782890051,6.89084245226548,105.582189088177));
#70422=CARTESIAN_POINT('Ctrl Pts',(-8.25932389787385,1.80830348142917,105.847381970049));
#70423=CARTESIAN_POINT('Ctrl Pts',(-5.97786913326917,-5.97830759712599,
106.165613428296));
#70424=CARTESIAN_POINT('Ctrl Pts',(1.79371623271613,-8.25561157089681,106.483844886542));
#70425=CARTESIAN_POINT('Ctrl Pts',(7.91964722679908,-2.95876137993589,106.802076344789));
#70426=CARTESIAN_POINT('Ctrl Pts',(6.76431025852604,5.07252397306689,107.120307803036));
#70427=CARTESIAN_POINT('Ctrl Pts',(0.625860372993087,7.85911200114565,107.385500684908));
#70428=CARTESIAN_POINT('Ctrl Pts',(-4.01795423759709,6.24802710056353,107.597654990406));
#70429=CARTESIAN_POINT('Ctrl Pts',(-7.41047211820897,2.6911420695088,107.809809295904));
#70430=CARTESIAN_POINT('Ctrl Pts',(-7.42175053436507,-4.05018662984695,
108.075002177777));
#70431=CARTESIAN_POINT('Ctrl Pts',(-0.593607222905992,-8.4334282213855,
108.393233636023));
#70432=CARTESIAN_POINT('Ctrl Pts',(6.7674007672284,-5.05715603761144,108.71146509427));
#70433=CARTESIAN_POINT('Ctrl Pts',(7.91962140522928,2.95883049500652,109.029696552517));
#70434=CARTESIAN_POINT('Ctrl Pts',(1.78130626263137,8.26518848724278,109.347928010764));
#70435=CARTESIAN_POINT('Ctrl Pts',(-4.68055859797518,6.34426621950518,109.613120892636));
#70436=CARTESIAN_POINT('Ctrl Pts',(-7.13043291328011,2.08296072310835,109.825275198134));
#70437=CARTESIAN_POINT('Ctrl Pts',(-7.35970269699859,-2.82703358042056,
110.037429503632));
#70438=CARTESIAN_POINT('Ctrl Pts',(-2.94802780900771,-7.92436273578246,
110.302622385504));
#70439=CARTESIAN_POINT('Ctrl Pts',(5.0814815637804,-6.75674671845169,110.620853843751));
#70440=CARTESIAN_POINT('Ctrl Pts',(8.42552250194139,0.618959532047456,110.939085301998));
#70441=CARTESIAN_POINT('Ctrl Pts',(4.03952359991809,7.42679811130282,111.257316760245));
#70442=CARTESIAN_POINT('Ctrl Pts',(-4.07441578005489,7.40847681930506,111.575548218491));
#70443=CARTESIAN_POINT('Ctrl Pts',(-7.69382448055576,1.72116458115858,111.840741100364));
#70444=CARTESIAN_POINT('Ctrl Pts',(-6.74948790579361,-3.10261372303192,
112.052895405862));
#70445=CARTESIAN_POINT('Ctrl Pts',(-3.70318310388795,-6.96015643158348,
112.26504971136));
#70446=CARTESIAN_POINT('Ctrl Pts',(2.97002659885532,-7.91614393079309,112.530242593232));
#70447=CARTESIAN_POINT('Ctrl Pts',(8.26699247260189,-1.76972216980235,112.848474051479));
#70448=CARTESIAN_POINT('Ctrl Pts',(5.95571537043626,5.99182733057143,113.166705509726));
#70449=CARTESIAN_POINT('Ctrl Pts',(-1.81966405650071,8.25614339881686,113.484936967973));
#70450=CARTESIAN_POINT('Ctrl Pts',(-7.93395319352799,2.92211900063055,113.803168426219));
#70451=CARTESIAN_POINT('Ctrl Pts',(-6.93764340508899,-3.74518979984444,
114.068361308092));
#70452=CARTESIAN_POINT('Ctrl Pts',(-3.06175617355554,-6.76811997813982,
114.280515613589));
#70453=CARTESIAN_POINT('Ctrl Pts',(1.76764253705638,-7.68327941143772,114.492669919087));
#70454=CARTESIAN_POINT('Ctrl Pts',(7.43297142413431,-4.02955686632436,114.75786280096));
#70455=CARTESIAN_POINT('Ctrl Pts',(7.40224337005944,4.08434501367814,115.076094259207));
#70456=CARTESIAN_POINT('Ctrl Pts',(0.568015682008036,8.42911018542453,115.394325717453));
#70457=CARTESIAN_POINT('Ctrl Pts',(-6.78734097469309,5.04054397794511,115.7125571757));
#70458=CARTESIAN_POINT('Ctrl Pts',(-7.90639702874043,-2.99587695923303,
116.030788633947));
#70459=CARTESIAN_POINT('Ctrl Pts',(-2.78249229912331,-7.37665772951092,
116.295981515819));
#70460=CARTESIAN_POINT('Ctrl Pts',(2.12602634926904,-7.11771106936877,116.508135821317));
#70461=CARTESIAN_POINT('Ctrl Pts',(6.37244442075708,-4.64212179476106,116.720290126815));
#70462=CARTESIAN_POINT('Ctrl Pts',(8.25426942022403,1.83123703252574,116.985483008687));
#70463=CARTESIAN_POINT('Ctrl Pts',(2.91090207991093,7.93736292363641,117.303714466934));
#70464=CARTESIAN_POINT('Ctrl Pts',(-5.09797278075856,6.73670645491388,117.621945925181));
#70465=CARTESIAN_POINT('Ctrl Pts',(-8.42968575735979,-0.6445767080121,117.940177383428));
#70466=CARTESIAN_POINT('Ctrl Pts',(-4.00524791880345,-7.44609843071264,
118.258408841675));
#70467=CARTESIAN_POINT('Ctrl Pts',(2.73588942891193,-7.39406868278906,118.523601723547));
#70468=CARTESIAN_POINT('Ctrl Pts',(6.27220159664381,-3.98011130948106,118.735756029045));
#70469=CARTESIAN_POINT('Ctrl Pts',(7.85518505938354,0.673357509701594,118.947910334543));
#70470=CARTESIAN_POINT('Ctrl Pts',(5.03154082906854,6.79485022766188,119.213103216415));
#70471=CARTESIAN_POINT('Ctrl Pts',(-3.00658182864851,7.90161672115188,119.531334674662));
#70472=CARTESIAN_POINT('Ctrl Pts',(-8.26630379901193,1.74377803503611,119.849566132909));
#70473=CARTESIAN_POINT('Ctrl Pts',(-5.94206196384213,-6.01389896142331,
120.167797591156));
#70474=CARTESIAN_POINT('Ctrl Pts',(1.85819830642578,-8.24824173899719,120.486029049402));
#70475=CARTESIAN_POINT('Ctrl Pts',(6.91387274892134,-3.78889248524638,120.751221931275));
#70476=CARTESIAN_POINT('Ctrl Pts',(7.34542771599016,1.10747034902265,120.963376236773));
#70477=CARTESIAN_POINT('Ctrl Pts',(5.48942310975583,5.65893776031443,121.17553054227));
#70478=CARTESIAN_POINT('Ctrl Pts',(-0.656298100951151,8.4294522677116,121.440723424143));
#70479=CARTESIAN_POINT('Ctrl Pts',(-7.45104659610839,3.99461959677861,121.758954882389));
#70480=CARTESIAN_POINT('Ctrl Pts',(-7.38471220878525,-4.10348217084607,
122.077186340637));
#70481=CARTESIAN_POINT('Ctrl Pts',(-0.543234847355393,-8.43682268398279,
122.395417798883));
#70482=CARTESIAN_POINT('Ctrl Pts',(6.81125465061382,-5.00931161093324,122.71364925713));
#70483=CARTESIAN_POINT('Ctrl Pts',(7.70453203163159,1.67258148578646,122.978842139003));
#70484=CARTESIAN_POINT('Ctrl Pts',(4.81989742627491,5.65246739972814,123.1909964445));
#70485=CARTESIAN_POINT('Ctrl Pts',(0.434219869285401,7.87202615329449,123.403150749998));
#70486=CARTESIAN_POINT('Ctrl Pts',(-6.02259591881576,5.93420012550998,123.66834363187));
#70487=CARTESIAN_POINT('Ctrl Pts',(-8.24500893828536,-1.86946749314901,
123.986575090117));
#70488=CARTESIAN_POINT('Ctrl Pts',(-2.88511749906848,-7.94031720711482,
124.304806548364));
#70489=CARTESIAN_POINT('Ctrl Pts',(5.12174013201059,-6.72628122520153,124.623038006611));
#70490=CARTESIAN_POINT('Ctrl Pts',(8.42726279619414,0.683838061839922,124.941269464858));
#70491=CARTESIAN_POINT('Ctrl Pts',(4.72049838974924,6.31460510288725,125.20646234673));
#70492=CARTESIAN_POINT('Ctrl Pts',(-0.0670524327962581,7.42814262625973,
125.418616652228));
#70493=CARTESIAN_POINT('Ctrl Pts',(-4.83372136248423,6.2283609756417,125.630770957726));
#70494=CARTESIAN_POINT('Ctrl Pts',(-8.43823429245977,0.531596422575805,
125.895963839598));
#70495=CARTESIAN_POINT('Ctrl Pts',(-4.99948169501149,-6.81764357249575,
126.214195297845));
#70496=CARTESIAN_POINT('Ctrl Pts',(3.02798715072524,-7.88694073440878,126.532426756092));
#70497=CARTESIAN_POINT('Ctrl Pts',(8.27741329284568,-1.72032272546982,126.850658214339));
#70498=CARTESIAN_POINT('Ctrl Pts',(5.91448945058515,6.04195392814753,127.168889672586));
#70499=CARTESIAN_POINT('Ctrl Pts',(-0.57625610256022,7.86290477859779,127.434082554458));
#70500=CARTESIAN_POINT('Ctrl Pts',(-4.92115119297959,5.56453680378123,127.646236859956));
#70501=CARTESIAN_POINT('Ctrl Pts',(-7.73347024311397,1.53322557110968,127.858391165454));
#70502=CARTESIAN_POINT('Ctrl Pts',(-6.71971589330665,-5.13145311234377,
128.123584047326));
#70503=CARTESIAN_POINT('Ctrl Pts',(0.695449107532702,-8.42564131916249,
128.441815505573));
#70504=CARTESIAN_POINT('Ctrl Pts',(7.45758551789534,-3.96950356799327,128.76004696382));
#70505=CARTESIAN_POINT('Ctrl Pts',(7.37772095423774,4.12847606529929,129.078278422067));
#70506=CARTESIAN_POINT('Ctrl Pts',(0.504021424748521,8.43992625171176,129.396509880313));
#70507=CARTESIAN_POINT('Ctrl Pts',(-5.59068457894054,5.55891973245065,129.661702762186));
#70508=CARTESIAN_POINT('Ctrl Pts',(-7.36422297414272,0.974689125777787,
129.873857067684));
#70509=CARTESIAN_POINT('Ctrl Pts',(-6.84434845783166,-3.91308533523255,
130.086011373181));
#70510=CARTESIAN_POINT('Ctrl Pts',(-1.70899701609721,-8.28044213372148,
130.351204255054));
#70511=CARTESIAN_POINT('Ctrl Pts',(6.04965748659407,-5.90565198731203,130.669435713301));
#70512=CARTESIAN_POINT('Ctrl Pts',(8.23347783603216,1.89271843035402,130.987667171547));
#70513=CARTESIAN_POINT('Ctrl Pts',(2.86345073195746,7.95460439028861,131.305898629794));
#70514=CARTESIAN_POINT('Ctrl Pts',(-5.15338257306271,6.70291285834692,131.624130088041));
#70515=CARTESIAN_POINT('Ctrl Pts',(-7.86606058112608,0.531444810953261,
131.889322969913));
#70516=CARTESIAN_POINT('Ctrl Pts',(-6.19932995725014,-4.09268945632841,
132.101477275411));
#70517=CARTESIAN_POINT('Ctrl Pts',(-2.60196477537556,-7.44225247897018,
132.313631580909));
#70518=CARTESIAN_POINT('Ctrl Pts',(4.13901333038334,-7.37258173110669,132.578824462781));
#70519=CARTESIAN_POINT('Ctrl Pts',(8.4399481069777,-0.492297726859653,132.897055921028));
#70520=CARTESIAN_POINT('Ctrl Pts',(4.97553001892583,6.82763805161073,133.215287379275));
#70521=CARTESIAN_POINT('Ctrl Pts',(-3.05371419871836,7.88352146523951,133.533518837522));
#70522=CARTESIAN_POINT('Ctrl Pts',(-8.28598212377782,1.68193132302526,133.851750295769));
#70523=CARTESIAN_POINT('Ctrl Pts',(-6.28760573439148,-4.75640166321992,
134.116943177641));
#70524=CARTESIAN_POINT('Ctrl Pts',(-1.99718992382571,-7.15493055961901,
134.329097483139));
#70525=CARTESIAN_POINT('Ctrl Pts',(2.91520340889385,-7.32522571241372,134.541251788637));
#70526=CARTESIAN_POINT('Ctrl Pts',(7.95919067301005,-2.85266131211001,134.806444670509));
#70527=CARTESIAN_POINT('Ctrl Pts',(6.69524230284883,5.16224869669132,135.124676128756));
#70528=CARTESIAN_POINT('Ctrl Pts',(-0.720086676891106,8.41748273005637,
135.442907587003));
#70529=CARTESIAN_POINT('Ctrl Pts',(-7.47476835559155,3.95005305414921,135.76113904525));
#70530=CARTESIAN_POINT('Ctrl Pts',(-7.35901803486954,-4.16308134599907,
136.079370503496));
#70531=CARTESIAN_POINT('Ctrl Pts',(-1.6286547873363,-7.71393714238848,136.344563385369));
#70532=CARTESIAN_POINT('Ctrl Pts',(3.18343636205135,-6.71174581115595,136.556717690867));
#70533=CARTESIAN_POINT('Ctrl Pts',(7.00412161819763,-3.61934013468348,136.768871996364));
#70534=CARTESIAN_POINT('Ctrl Pts',(7.87990980123138,3.0648677386468,137.034064878237));
#70535=CARTESIAN_POINT('Ctrl Pts',(1.67032640351384,8.28764687990933,137.352296336484));
#70536=CARTESIAN_POINT('Ctrl Pts',(-6.06291022794655,5.8833374797724,137.670527794731));
#70537=CARTESIAN_POINT('Ctrl Pts',(-8.23369805000805,-1.9186707694759,137.988759252977));
#70538=CARTESIAN_POINT('Ctrl Pts',(-2.82663921160395,-7.96846933220942,
138.306990711224));
#70539=CARTESIAN_POINT('Ctrl Pts',(3.82822544044891,-6.89217183695629,138.572183593096));
#70540=CARTESIAN_POINT('Ctrl Pts',(6.80439690023717,-2.98026537892912,138.784337898594));
#70541=CARTESIAN_POINT('Ctrl Pts',(7.66150002642696,1.85977417932761,138.996492204092));
#70542=CARTESIAN_POINT('Ctrl Pts',(3.94001291137149,7.48082154506875,139.261685085965));
#70543=CARTESIAN_POINT('Ctrl Pts',(-4.17293501391588,7.3526658070377,139.579916544211));
#70544=CARTESIAN_POINT('Ctrl Pts',(-8.43532308489233,0.466759881006833,
139.898148002458));
#70545=CARTESIAN_POINT('Ctrl Pts',(-4.95867971941822,-6.84737734761105,
140.216379460705));
#70546=CARTESIAN_POINT('Ctrl Pts',(3.0905991967229,-7.86985319660759,140.534610918952));
#70547=CARTESIAN_POINT('Ctrl Pts',(7.40953744105551,-2.69371445454605,140.799803800824));
#70548=CARTESIAN_POINT('Ctrl Pts',(7.09166906773478,2.21134093674737,141.011958106322));
#70549=CARTESIAN_POINT('Ctrl Pts',(4.56526824486317,6.42772654252474,141.22411241182));
#70550=CARTESIAN_POINT('Ctrl Pts',(-1.93022040882533,8.23168524084186,141.489305293693));
#70551=CARTESIAN_POINT('Ctrl Pts',(-7.97174412624228,2.81538215631022,141.807536751939));
#70552=CARTESIAN_POINT('Ctrl Pts',(-6.67500546132707,-5.17849808576631,
142.125768210186));
#70553=CARTESIAN_POINT('Ctrl Pts',(0.745751997391611,-8.42133808006394,
142.443999668433));
#70554=CARTESIAN_POINT('Ctrl Pts',(7.49365570889798,-3.91554809029897,142.76223112668));
#70555=CARTESIAN_POINT('Ctrl Pts',(7.3606836589212,2.82447848749324,143.027424008552));
#70556=CARTESIAN_POINT('Ctrl Pts',(3.90450918100473,6.31954167327552,143.23957831405));
#70557=CARTESIAN_POINT('Ctrl Pts',(-0.76763224961116,7.84653320788012,143.451732619548));
#70558=CARTESIAN_POINT('Ctrl Pts',(-6.85477795141283,4.94958705022387,143.71692550142));
#70559=CARTESIAN_POINT('Ctrl Pts',(-7.86494469201523,-3.10124589351471,
144.035156959667));
#70560=CARTESIAN_POINT('Ctrl Pts',(-1.64439240863728,-8.2866467246535,144.353388417914));
#70561=CARTESIAN_POINT('Ctrl Pts',(6.08481632047936,-5.86942002640229,144.67161987616));
#70562=CARTESIAN_POINT('Ctrl Pts',(8.22533424935467,1.95710735993869,144.989851334407));
#70563=CARTESIAN_POINT('Ctrl Pts',(3.70559910065562,6.95887045119629,145.25504421628));
#70564=CARTESIAN_POINT('Ctrl Pts',(-1.1955927401216,7.3315998871873,145.467198521778));
#70565=CARTESIAN_POINT('Ctrl Pts',(-5.72444552590752,5.42107609930576,145.679352827275));
#70566=CARTESIAN_POINT('Ctrl Pts',(-8.42096385881222,-0.757469741041528,
145.944545709148));
#70567=CARTESIAN_POINT('Ctrl Pts',(-3.90486111908968,-7.49847589595874,
146.262777167394));
#70568=CARTESIAN_POINT('Ctrl Pts',(4.19186028299498,-7.33490611339408,146.581008625642));
#70569=CARTESIAN_POINT('Ctrl Pts',(8.44273746126223,-0.441888226112777,
146.899240083888));
#70570=CARTESIAN_POINT('Ctrl Pts',(4.92716246104114,6.87091427440382,147.217471542135));
#70571=CARTESIAN_POINT('Ctrl Pts',(-1.76497519032476,7.68389257525593,147.482664424007));
#70572=CARTESIAN_POINT('Ctrl Pts',(-5.70993610234189,4.7516763951212,147.694818729505));
#70573=CARTESIAN_POINT('Ctrl Pts',(-7.87667266568883,0.339663018585871,
147.906973035003));
#70574=CARTESIAN_POINT('Ctrl Pts',(-5.86145424027185,-6.09341817350986,
148.172165916875));
#70575=CARTESIAN_POINT('Ctrl Pts',(1.96833677532543,-8.22196648831977,148.490397375122));
#70576=CARTESIAN_POINT('Ctrl Pts',(7.97438883746259,-2.78956373241462,148.808628833369));
#70577=CARTESIAN_POINT('Ctrl Pts',(6.664295105365,5.20213810875714,149.126860291616));
#70578=CARTESIAN_POINT('Ctrl Pts',(-0.784980464148565,8.41844470718301,
149.445091749863));
#70579=CARTESIAN_POINT('Ctrl Pts',(-6.37083420409281,4.64433221669856,149.710284631735));
#70580=CARTESIAN_POINT('Ctrl Pts',(-7.42679969286816,-0.156241061364189,
149.922438937233));
#70581=CARTESIAN_POINT('Ctrl Pts',(-6.16987516676678,-4.90816647717152,
150.134593242731));
#70582=CARTESIAN_POINT('Ctrl Pts',(-0.430222084104789,-8.44399890804918,
150.399786124603));
#70583=CARTESIAN_POINT('Ctrl Pts',(6.87716522396635,-4.917273833794,150.71801758285));
#70584=CARTESIAN_POINT('Ctrl Pts',(7.85004833380309,3.12250508572264,151.036249041097));
#70585=CARTESIAN_POINT('Ctrl Pts',(1.62073799871939,8.29741387924024,151.354480499344));
#70586=CARTESIAN_POINT('Ctrl Pts',(-6.11240446161866,5.8416314624366,151.67271195759));
#70587=CARTESIAN_POINT('Ctrl Pts',(-7.85565197732039,-0.670838177559451,
151.937904839463));
#70588=CARTESIAN_POINT('Ctrl Pts',(-5.50473164554611,-4.98733689650615,
152.150059144961));
#70589=CARTESIAN_POINT('Ctrl Pts',(-1.44101267407513,-7.75199824614526,
152.362213450459));
#70590=CARTESIAN_POINT('Ctrl Pts',(5.21338494434369,-6.65618030389132,152.627406332331));
#70591=CARTESIAN_POINT('Ctrl Pts',(8.41397490779385,0.79416338508947,152.945637790578));
#70592=CARTESIAN_POINT('Ctrl Pts',(3.88463257389226,7.50913956436645,153.263869248825));
#70593=CARTESIAN_POINT('Ctrl Pts',(-4.22626533191902,7.31905378776502,153.582100707071));
#70594=CARTESIAN_POINT('Ctrl Pts',(-7.72583738521557,1.57078236861736,153.847293588944));
#70595=CARTESIAN_POINT('Ctrl Pts',(-6.68713870766457,-3.25309306180461,
154.059461682204));
#70596=CARTESIAN_POINT('Ctrl Pts',(-5.11767179385483,-5.12707892333455,
154.165552622715));
#70597=CARTESIAN_POINT('Ctrl Pts',(-4.14791805377987,-5.81840619716922,
154.218604986852));
#70598=CARTESIAN_POINT('Ctrl Pts',(-3.25626140427607,6.79079303725207,-0.219318740910142));
#70599=CARTESIAN_POINT('Ctrl Pts',(-4.38783911844251,6.24818997146264,-0.166277514063165));
#70600=CARTESIAN_POINT('Ctrl Pts',(-6.35583945430648,4.58604843748734,-0.0601977108417193));
#70601=CARTESIAN_POINT('Ctrl Pts',(-8.30600288127432,-0.23487779396911,
0.151959245128665));
#70602=CARTESIAN_POINT('Ctrl Pts',(-5.71099197201566,-6.83602431645478,
0.417152127001014));
#70603=CARTESIAN_POINT('Ctrl Pts',(2.67663026760001,-8.49913365837745,0.73538358524783));
#70604=CARTESIAN_POINT('Ctrl Pts',(8.59315924532233,-2.34512449975285,1.05361504349465));
#70605=CARTESIAN_POINT('Ctrl Pts',(6.61618139014667,5.96934387336162,1.37184650174147));
#70606=CARTESIAN_POINT('Ctrl Pts',(-0.0954035072434517,8.3097161946593,
1.63703938361381));
#70607=CARTESIAN_POINT('Ctrl Pts',(-4.81458352345695,6.17338366571372,1.84919368911169));
#70608=CARTESIAN_POINT('Ctrl Pts',(-8.03570940339818,2.11617400989208,2.06134799460957));
#70609=CARTESIAN_POINT('Ctrl Pts',(-7.40248233935818,-4.96109161769496,
2.32654087648192));
#70610=CARTESIAN_POINT('Ctrl Pts',(0.18345886150707,-8.90852845273233,2.64477233472873));
#70611=CARTESIAN_POINT('Ctrl Pts',(7.58684621947925,-4.66085638140519,2.96300379297555));
#70612=CARTESIAN_POINT('Ctrl Pts',(8.02953162399686,3.86308122171422,3.28123525122236));
#70613=CARTESIAN_POINT('Ctrl Pts',(1.07920619621232,8.84559539285239,3.59946670946919));
#70614=CARTESIAN_POINT('Ctrl Pts',(-5.51954412358968,6.21137598843296,3.86465959134152));
#70615=CARTESIAN_POINT('Ctrl Pts',(-7.68340312835726,1.50434211377469,4.07681389683941));
#70616=CARTESIAN_POINT('Ctrl Pts',(-7.45445771613391,-3.67117143356693,
4.28896820233728));
#70617=CARTESIAN_POINT('Ctrl Pts',(-2.33639713332563,-8.59945993394335,
4.55416108420963));
#70618=CARTESIAN_POINT('Ctrl Pts',(5.9798023331272,-6.60596964644571,4.87239254245645));
#70619=CARTESIAN_POINT('Ctrl Pts',(8.78433487726616,1.4554866160667,5.19062400070327));
#70620=CARTESIAN_POINT('Ctrl Pts',(3.52963249230927,8.18160003932308,5.50885545895009));
#70621=CARTESIAN_POINT('Ctrl Pts',(-4.98510569539155,7.38635008106619,5.8270869171969));
#70622=CARTESIAN_POINT('Ctrl Pts',(-8.24014557041358,1.07071602129575,6.09227979906925));
#70623=CARTESIAN_POINT('Ctrl Pts',(-6.78761070841664,-3.90206450061349,
6.30443410456712));
#70624=CARTESIAN_POINT('Ctrl Pts',(-3.22123524393854,-7.65963932084413,
6.51658841006501));
#70625=CARTESIAN_POINT('Ctrl Pts',(3.87447872379791,-8.02482792303879,6.78178129193735));
#70626=CARTESIAN_POINT('Ctrl Pts',(8.84639377321643,-1.06686466781347,7.10001275018417));
#70627=CARTESIAN_POINT('Ctrl Pts',(5.6781320946836,6.85870201306817,7.41824420843098));
#70628=CARTESIAN_POINT('Ctrl Pts',(-2.69956168110274,8.49171654179624,7.73647566667781));
#70629=CARTESIAN_POINT('Ctrl Pts',(-8.60704720841996,2.30828653891773,8.05470712492461));
#70630=CARTESIAN_POINT('Ctrl Pts',(-6.92364489287862,-4.59451548655276,
8.31990000679697));
#70631=CARTESIAN_POINT('Ctrl Pts',(-2.56635205336581,-7.39672925615521,
8.53205431229485));
#70632=CARTESIAN_POINT('Ctrl Pts',(2.59017037923298,-7.89540680161064,8.74420861779272));
#70633=CARTESIAN_POINT('Ctrl Pts',(8.18712624868128,-3.51858099169413,9.00940149966508));
#70634=CARTESIAN_POINT('Ctrl Pts',(7.37885783341021,4.9949314456656,9.32763295791187));
#70635=CARTESIAN_POINT('Ctrl Pts',(-0.209966232129463,8.90162297445633,
9.64586441615873));
#70636=CARTESIAN_POINT('Ctrl Pts',(-7.60615567604954,4.6414737858246,9.9640958744055));
#70637=CARTESIAN_POINT('Ctrl Pts',(-8.01212511125873,-3.90067937766853,
10.2823273326523));
#70638=CARTESIAN_POINT('Ctrl Pts',(-2.21503253104398,-8.00874909362732,
10.5475202145246));
#70639=CARTESIAN_POINT('Ctrl Pts',(2.91224332325345,-7.26750337980572,10.7596745200225));
#70640=CARTESIAN_POINT('Ctrl Pts',(7.13256993626704,-4.26296578247275,10.9718288255204));
#70641=CARTESIAN_POINT('Ctrl Pts',(8.48864274698747,2.71152959044796,11.2370217073928));
#70642=CARTESIAN_POINT('Ctrl Pts',(2.29618701398579,8.60955331416399,11.5552531656396));
#70643=CARTESIAN_POINT('Ctrl Pts',(-5.99519548657091,6.58335844961113,11.8734846238864));
#70644=CARTESIAN_POINT('Ctrl Pts',(-8.78625442260016,-1.48277317684341,
12.1917160821332));
#70645=CARTESIAN_POINT('Ctrl Pts',(-3.49181055050968,-8.19857960168739,
12.5099475403801));
#70646=CARTESIAN_POINT('Ctrl Pts',(3.57879403802026,-7.49924425470446,12.7751404222524));
#70647=CARTESIAN_POINT('Ctrl Pts',(6.96403896420184,-3.57769868132897,12.9872947277503));
#70648=CARTESIAN_POINT('Ctrl Pts',(8.18049881518126,1.45803645122659,13.1994490332481));
#70649=CARTESIAN_POINT('Ctrl Pts',(4.63130578286872,7.61317641667533,13.4646419151205));
#70650=CARTESIAN_POINT('Ctrl Pts',(-3.91145815038478,8.00608382484316,13.7828733733673));
#70651=CARTESIAN_POINT('Ctrl Pts',(-8.84318963161335,1.03969925343594,14.1011048316142));
#70652=CARTESIAN_POINT('Ctrl Pts',(-5.66169037244258,-6.88056285482645,
14.4193362898609));
#70653=CARTESIAN_POINT('Ctrl Pts',(2.73925198622831,-8.47973743472043,14.7375677481078));
#70654=CARTESIAN_POINT('Ctrl Pts',(7.61925668070438,-3.31562343938954,15.0027606299801));
#70655=CARTESIAN_POINT('Ctrl Pts',(7.60393255881819,1.86493329377995,15.214914935478));
#70656=CARTESIAN_POINT('Ctrl Pts',(5.22054364993401,6.4647007013025,15.4270692409758));
#70657=CARTESIAN_POINT('Ctrl Pts',(-1.49505376412002,8.78488831165459,15.6922621228482));
#70658=CARTESIAN_POINT('Ctrl Pts',(-8.202756761262,3.48018168896353,16.010493581095));
#70659=CARTESIAN_POINT('Ctrl Pts',(-7.35862662766388,-5.01334135611222,
16.3287250393419));
#70660=CARTESIAN_POINT('Ctrl Pts',(0.236714126732794,-8.90734806184376,
16.6469564975886));
#70661=CARTESIAN_POINT('Ctrl Pts',(7.62826869219535,-4.60640479827018,16.9651879558355));
#70662=CARTESIAN_POINT('Ctrl Pts',(7.92680547927285,2.49242573651805,17.2303808377078));
#70663=CARTESIAN_POINT('Ctrl Pts',(4.51842007932001,6.39387570539983,17.4425351432057));
#70664=CARTESIAN_POINT('Ctrl Pts',(-0.297120289451444,8.30410444851726,
17.6546894487036));
#70665=CARTESIAN_POINT('Ctrl Pts',(-6.88893937990305,5.6526067107022,17.9198823305759));
#70666=CARTESIAN_POINT('Ctrl Pts',(-8.47526645909824,-2.75077107733645,
18.2381137888227));
#70667=CARTESIAN_POINT('Ctrl Pts',(-2.26884065207606,-8.61018812185635,
18.5563452470696));
#70668=CARTESIAN_POINT('Ctrl Pts',(6.01914491904821,-6.57014288399595,18.8745767053164));
#70669=CARTESIAN_POINT('Ctrl Pts',(8.77995628575123,1.52375064434829,19.1928081635632));
#70670=CARTESIAN_POINT('Ctrl Pts',(4.35076258993752,7.07935703607947,19.4580010454356));
#70671=CARTESIAN_POINT('Ctrl Pts',(-0.780808721133584,7.79025701054246,
19.6701553509334));
#70672=CARTESIAN_POINT('Ctrl Pts',(-5.66921564014895,6.07506585839019,19.8823096564313));
#70673=CARTESIAN_POINT('Ctrl Pts',(-8.90771660123625,-0.249064967258383,
20.1475025383036));
#70674=CARTESIAN_POINT('Ctrl Pts',(-4.59547615923811,-7.63403444729592,
20.4657339965505));
#70675=CARTESIAN_POINT('Ctrl Pts',(3.93252182436328,-7.98863251746972,20.7839654547973));
#70676=CARTESIAN_POINT('Ctrl Pts',(8.85260702063095,-1.01401775669988,21.1021969130441));
#70677=CARTESIAN_POINT('Ctrl Pts',(5.63006673821769,6.90737265022453,21.420428371291));
#70678=CARTESIAN_POINT('Ctrl Pts',(-1.35685593532154,8.1978883335326,21.6856212531632));
#70679=CARTESIAN_POINT('Ctrl Pts',(-5.69749473468943,5.36994602370365,21.8977755586612));
#70680=CARTESIAN_POINT('Ctrl Pts',(-8.26378367614365,0.869661147913093,
22.109929864159));
#70681=CARTESIAN_POINT('Ctrl Pts',(-6.56232287864745,-6.02871187255083,
22.3751227460314));
#70682=CARTESIAN_POINT('Ctrl Pts',(1.53578266229113,-8.77714387980692,22.6933542042781));
#70683=CARTESIAN_POINT('Ctrl Pts',(8.20721798994993,-3.45319421169897,23.011585662525));
#70684=CARTESIAN_POINT('Ctrl Pts',(7.34889809770717,5.03890660978577,23.3298171207718));
#70685=CARTESIAN_POINT('Ctrl Pts',(-0.27816984382537,8.90685522189735,23.6480485790186));
#70686=CARTESIAN_POINT('Ctrl Pts',(-6.39970799874712,5.30001591403834,23.913241460891));
#70687=CARTESIAN_POINT('Ctrl Pts',(-7.82279861437396,0.318729333844981,
24.1253957663889));
#70688=CARTESIAN_POINT('Ctrl Pts',(-6.80966379123187,-4.76181795207178,
24.3375500718868));
#70689=CARTESIAN_POINT('Ctrl Pts',(-1.00184047355013,-8.85470293524363,
24.6027429537591));
#70690=CARTESIAN_POINT('Ctrl Pts',(6.91461318249575,-5.62005405748759,24.9209744120059));
#70691=CARTESIAN_POINT('Ctrl Pts',(8.4609395460387,2.77407270931146,25.2392058702527));
#70692=CARTESIAN_POINT('Ctrl Pts',(2.2447325164063,8.62311190942198,25.5574373284995));
#70693=CARTESIAN_POINT('Ctrl Pts',(-6.05012225740613,6.54258886651866,25.8756687867463));
#70694=CARTESIAN_POINT('Ctrl Pts',(-8.30714153147531,-0.194501245047355,
26.1408616686187));
#70695=CARTESIAN_POINT('Ctrl Pts',(-6.11546704534361,-4.88864289620552,
26.3530159741166));
#70696=CARTESIAN_POINT('Ctrl Pts',(-2.01927511983364,-8.0603324465377,26.5651702796144));
#70697=CARTESIAN_POINT('Ctrl Pts',(5.04947513615378,-7.34249611884268,26.8303631614868));
#70698=CARTESIAN_POINT('Ctrl Pts',(8.90575690367034,0.29047727166572,27.1485946197336));
#70699=CARTESIAN_POINT('Ctrl Pts',(4.56938031041736,7.64223403050698,27.4668260779804));
#70700=CARTESIAN_POINT('Ctrl Pts',(-3.95919823070793,7.9825830683173,27.7850575362273));
#70701=CARTESIAN_POINT('Ctrl Pts',(-8.85792920644842,0.972902142767944,
28.103288994474));
#70702=CARTESIAN_POINT('Ctrl Pts',(-6.14464476425655,-5.59372611765914,
28.3684818763464));
#70703=CARTESIAN_POINT('Ctrl Pts',(-1.41197554189225,-7.70091498579245,
28.5806361818443));
#70704=CARTESIAN_POINT('Ctrl Pts',(3.76042003719523,-7.40983618591857,28.7927904873422));
#70705=CARTESIAN_POINT('Ctrl Pts',(8.62689382504626,-2.23296917516404,29.0579833692145));
#70706=CARTESIAN_POINT('Ctrl Pts',(6.53368979848841,6.0586946357904,29.3762148274614));
#70707=CARTESIAN_POINT('Ctrl Pts',(-1.56086226855208,8.76622418016329,29.6944462857081));
#70708=CARTESIAN_POINT('Ctrl Pts',(-8.22339305523067,3.43113534151757,30.012677743955));
#70709=CARTESIAN_POINT('Ctrl Pts',(-7.32595762451067,-5.07343998582116,
30.3309092022018));
#70710=CARTESIAN_POINT('Ctrl Pts',(-0.971692979062693,-8.25240837045328,
30.5961020840741));
#70711=CARTESIAN_POINT('Ctrl Pts',(3.98328725484426,-6.74026625547534,30.808256389572));
#70712=CARTESIAN_POINT('Ctrl Pts',(7.69776696987758,-3.12902777804056,31.0204106950699));
#70713=CARTESIAN_POINT('Ctrl Pts',(7.97772549360841,3.97055970292418,31.2856035769423));
#70714=CARTESIAN_POINT('Ctrl Pts',(0.960562258670931,8.85856665718801,31.603835035189));
#70715=CARTESIAN_POINT('Ctrl Pts',(-6.92638925711606,5.59536497980034,31.9220664934359));
#70716=CARTESIAN_POINT('Ctrl Pts',(-8.45868859628192,-2.80133366519539,
32.2402979516827));
#70717=CARTESIAN_POINT('Ctrl Pts',(-2.20476864460852,-8.63414405888652,
32.5585294099295));
#70718=CARTESIAN_POINT('Ctrl Pts',(4.67732180358315,-6.86797582290539,32.8237222918018));
#70719=CARTESIAN_POINT('Ctrl Pts',(7.42701215729331,-2.47734877736705,33.0358765972997));
#70720=CARTESIAN_POINT('Ctrl Pts',(7.86373539481082,2.68478989842535,33.2480309027976));
#70721=CARTESIAN_POINT('Ctrl Pts',(3.4200181553324,8.22878631531108,33.5132237846699));
#70722=CARTESIAN_POINT('Ctrl Pts',(-5.08317498807606,7.3183478404094,33.8314552429168));
#70723=CARTESIAN_POINT('Ctrl Pts',(-8.89845997676324,-0.316839770565183,
34.1496867011636));
#70724=CARTESIAN_POINT('Ctrl Pts',(-4.54980615681072,-7.66134107112282,
34.4679181594104));
#70725=CARTESIAN_POINT('Ctrl Pts',(3.99660594150553,-7.96470899369072,34.7861496176572));
#70726=CARTESIAN_POINT('Ctrl Pts',(8.03476930536867,-2.11870558780435,35.0513424995296));
#70727=CARTESIAN_POINT('Ctrl Pts',(7.23200986308717,2.99929989989564,35.2634968050274));
#70728=CARTESIAN_POINT('Ctrl Pts',(4.17701215284028,7.18324443641673,35.4756511105253));
#70729=CARTESIAN_POINT('Ctrl Pts',(-2.81326380316848,8.4554713162329,35.7408439923976));
#70730=CARTESIAN_POINT('Ctrl Pts',(-8.6365046950554,2.19263989859547,36.0590754506445));
#70731=CARTESIAN_POINT('Ctrl Pts',(-6.51089486438885,-6.07381473730833,
36.3773069088913));
#70732=CARTESIAN_POINT('Ctrl Pts',(1.58816963159744,-8.76781616446756,36.6955383671382));
#70733=CARTESIAN_POINT('Ctrl Pts',(8.23991738921627,-3.39311211496841,37.0137698253849));
#70734=CARTESIAN_POINT('Ctrl Pts',(7.45573024013204,3.66858525111086,37.2789627072573));
#70735=CARTESIAN_POINT('Ctrl Pts',(3.49381813846497,7.00649708232563,37.4911170127552));
#70736=CARTESIAN_POINT('Ctrl Pts',(-1.55616091301732,8.16240126256267,37.7032713182531));
#70737=CARTESIAN_POINT('Ctrl Pts',(-7.66823921050773,4.53955458346809,37.9684642001254));
#70738=CARTESIAN_POINT('Ctrl Pts',(-7.95853871375751,-4.00731139471962,
38.2866956583722));
#70739=CARTESIAN_POINT('Ctrl Pts',(-0.933437273603877,-8.85503654732807,
38.604927116619));
#70740=CARTESIAN_POINT('Ctrl Pts',(6.94805109229926,-5.578661944537,38.9231585748658));
#70741=CARTESIAN_POINT('Ctrl Pts',(8.44623376174194,2.84087726730062,39.2413900331127));
#70742=CARTESIAN_POINT('Ctrl Pts',(3.22389408487697,7.65852062005342,39.506582914985));
#70743=CARTESIAN_POINT('Ctrl Pts',(-1.95610514271807,7.58099064898092,39.7187372204829));
#70744=CARTESIAN_POINT('Ctrl Pts',(-6.52692173063208,5.1425406056238,39.9308915259807));
#70745=CARTESIAN_POINT('Ctrl Pts',(-8.76630268949753,-1.60043292954236,
40.1960844078531));
#70746=CARTESIAN_POINT('Ctrl Pts',(-3.38143393342795,-8.2439546108945,40.5143158660999));
#70747=CARTESIAN_POINT('Ctrl Pts',(5.10134063952619,-7.2978970311856,40.8325473243467));
#70748=CARTESIAN_POINT('Ctrl Pts',(8.90386346870972,0.343654482297748,41.1507787825936));
#70749=CARTESIAN_POINT('Ctrl Pts',(4.51447416949656,7.68303139254309,41.4690102408403));
#70750=CARTESIAN_POINT('Ctrl Pts',(-2.58742933084496,7.89630550423239,41.7342031227127));
#70751=CARTESIAN_POINT('Ctrl Pts',(-6.44767089982784,4.44131810578996,41.9463574282106));
#70752=CARTESIAN_POINT('Ctrl Pts',(-8.29993800323926,-0.396812677055769,
42.1585117337085));
#70753=CARTESIAN_POINT('Ctrl Pts',(-5.56947835427224,-6.95631793890613,
42.4237046155808));
#70754=CARTESIAN_POINT('Ctrl Pts',(2.85234184146494,-8.44162478981714,42.7419360738277));
#70755=CARTESIAN_POINT('Ctrl Pts',(8.63681108804976,-2.16528788561929,43.0601675320744));
#70756=CARTESIAN_POINT('Ctrl Pts',(6.49739267219132,6.0976037536053,43.3783989903213));
#70757=CARTESIAN_POINT('Ctrl Pts',(-1.62906851819094,8.76102643352332,43.6966304485681));
#70758=CARTESIAN_POINT('Ctrl Pts',(-7.13108961687574,4.26544159898762,43.9618233304404));
#70759=CARTESIAN_POINT('Ctrl Pts',(-7.78031959023451,-0.874296072916558,
44.1739776359383));
#70760=CARTESIAN_POINT('Ctrl Pts',(-6.00655321128364,-5.74175493018522,
44.3861319414362));
#70761=CARTESIAN_POINT('Ctrl Pts',(0.356008857715901,-8.90408367543134,
44.6513248233086));
#70762=CARTESIAN_POINT('Ctrl Pts',(7.68866550332958,-4.50347708449103,44.9695562815553));
#70763=CARTESIAN_POINT('Ctrl Pts',(7.94083573671719,4.02816399873989,45.2877877398022));
#70764=CARTESIAN_POINT('Ctrl Pts',(0.907644546520611,8.86414487978386,45.606019198049));
#70765=CARTESIAN_POINT('Ctrl Pts',(-6.97447922537052,5.54671866428513,45.9242506562958));
#70766=CARTESIAN_POINT('Ctrl Pts',(-8.18100447996011,-1.45519650121904,
46.1894435381681));
#70767=CARTESIAN_POINT('Ctrl Pts',(-5.30114464388381,-5.76156506636232,
46.401597843666));
#70768=CARTESIAN_POINT('Ctrl Pts',(-0.770368802850766,-8.27363058553387,
46.6137521491639));
#70769=CARTESIAN_POINT('Ctrl Pts',(6.10707611651337,-6.48945835281855,46.8789450310363));
#70770=CARTESIAN_POINT('Ctrl Pts',(8.75806975259084,1.64106589793963,47.197176489283));
#70771=CARTESIAN_POINT('Ctrl Pts',(3.35439483242474,8.24809145842061,47.51540794753));
#70772=CARTESIAN_POINT('Ctrl Pts',(-5.12678723206113,7.28786222083,47.8336394057766));
#70773=CARTESIAN_POINT('Ctrl Pts',(-8.90287287341688,-0.385101292691789,
48.1518708640236));
#70774=CARTESIAN_POINT('Ctrl Pts',(-5.2227875577806,-6.46288799876496,48.4170637458958));
#70775=CARTESIAN_POINT('Ctrl Pts',(-0.224771957636989,-7.82606185232166,
48.6292180513938));
#70776=CARTESIAN_POINT('Ctrl Pts',(4.84324354766974,-6.75199400890155,48.8413723568916));
#70777=CARTESIAN_POINT('Ctrl Pts',(8.86609442122669,-0.895442974034532,
49.106565238764));
#70778=CARTESIAN_POINT('Ctrl Pts',(5.53661976275402,6.98159900562246,49.4247966970108));
#70779=CARTESIAN_POINT('Ctrl Pts',(-2.87546975915461,8.42701910894097,49.7430281552576));
#70780=CARTESIAN_POINT('Ctrl Pts',(-8.64944445882054,2.14102630212842,50.0612596135045));
#70781=CARTESIAN_POINT('Ctrl Pts',(-6.46946867237072,-6.12824799621133,
50.3794910717512));
#70782=CARTESIAN_POINT('Ctrl Pts',(0.294237499671178,-8.30420709352041,
50.6446839536236));
#70783=CARTESIAN_POINT('Ctrl Pts',(4.96172359066756,-6.05632442650801,50.8568382591214));
#70784=CARTESIAN_POINT('Ctrl Pts',(8.08399832859222,-1.9223428886662,51.0689925646194));
#70785=CARTESIAN_POINT('Ctrl Pts',(7.28133379904682,5.13727812296675,51.3341854464917));
#70786=CARTESIAN_POINT('Ctrl Pts',(-0.397394644859894,8.90162684956315,
51.6524169047385));
#70787=CARTESIAN_POINT('Ctrl Pts',(-7.69655114233151,4.47728465833303,51.9706483629853));
#70788=CARTESIAN_POINT('Ctrl Pts',(-7.93446639944908,-4.05476584140684,
52.2888798212321));
#70789=CARTESIAN_POINT('Ctrl Pts',(-0.866467989252532,-8.86897297489713,
52.607111279479));
#70790=CARTESIAN_POINT('Ctrl Pts',(5.66710633795237,-6.07703356191387,52.8723041613512));
#70791=CARTESIAN_POINT('Ctrl Pts',(7.71731446434895,-1.31940289815309,53.0844584668492));
#70792=CARTESIAN_POINT('Ctrl Pts',(7.36414769336802,3.84912456391707,53.296612772347));
#70793=CARTESIAN_POINT('Ctrl Pts',(2.12921839658729,8.65308485024211,53.5618056542195));
#70794=CARTESIAN_POINT('Ctrl Pts',(-6.13671289856523,6.46046731074539,53.8800371124662));
#70795=CARTESIAN_POINT('Ctrl Pts',(-8.74684968997108,-1.66601257477884,
54.1982685707131));
#70796=CARTESIAN_POINT('Ctrl Pts',(-3.33214332607097,-8.26400047961927,
54.5165000289599));
#70797=CARTESIAN_POINT('Ctrl Pts',(5.16104265436551,-7.26450873257612,54.8347314872066));
#70798=CARTESIAN_POINT('Ctrl Pts',(8.26348127511696,-0.872529870021032,
55.0999243690791));
#70799=CARTESIAN_POINT('Ctrl Pts',(6.69194989702022,4.06393566940663,55.3120786745769));
#70800=CARTESIAN_POINT('Ctrl Pts',(3.03636914251083,7.73478465044085,55.5242329800748));
#70801=CARTESIAN_POINT('Ctrl Pts',(-4.06606816584847,7.92947274896181,55.7894258619471));
#70802=CARTESIAN_POINT('Ctrl Pts',(-8.86946220514079,0.854121340446415,
56.1076573201939));
#70803=CARTESIAN_POINT('Ctrl Pts',(-5.51179106060672,-6.99307777037299,
56.4258887784408));
#70804=CARTESIAN_POINT('Ctrl Pts',(2.90270172073915,-8.42444097807349,56.7441202366875));
#70805=CARTESIAN_POINT('Ctrl Pts',(8.65999593577497,-2.10093284000611,57.0623516949345));
#70806=CARTESIAN_POINT('Ctrl Pts',(6.81131644716327,4.75945368870117,57.3275445768066));
#70807=CARTESIAN_POINT('Ctrl Pts',(2.38798828780706,7.4562241440692,57.5396988823047));
#70808=CARTESIAN_POINT('Ctrl Pts',(-2.77902229276694,7.8309301015008,57.7518531878024));
#70809=CARTESIAN_POINT('Ctrl Pts',(-8.26925985820949,3.32096218034177,58.0170460696748));
#70810=CARTESIAN_POINT('Ctrl Pts',(-7.25678260140303,-5.17068557819958,
58.3352775279216));
#70811=CARTESIAN_POINT('Ctrl Pts',(0.423667623282275,-8.89401389380803,
58.6535089861685));
#70812=CARTESIAN_POINT('Ctrl Pts',(7.71542176339676,-4.45748248291911,58.9717404444153));
#70813=CARTESIAN_POINT('Ctrl Pts',(7.91614443013644,4.0919562274143,59.2899719026621));
#70814=CARTESIAN_POINT('Ctrl Pts',(2.02207314452598,8.05963096900062,59.5551647845345));
#70815=CARTESIAN_POINT('Ctrl Pts',(-3.08592400199076,7.19547354961726,59.7673190900323));
#70816=CARTESIAN_POINT('Ctrl Pts',(-7.23288317138988,4.0904562321718,59.9794733955303));
#70817=CARTESIAN_POINT('Ctrl Pts',(-8.42108067557773,-2.91459236622659,
60.2446662774025));
#70818=CARTESIAN_POINT('Ctrl Pts',(-2.08877662244061,-8.66221076251164,
60.5628977356495));
#70819=CARTESIAN_POINT('Ctrl Pts',(6.15155819357058,-6.43749246130692,60.8811291938961));
#70820=CARTESIAN_POINT('Ctrl Pts',(8.74811365885818,1.69333708526246,61.1993606521431));
#70821=CARTESIAN_POINT('Ctrl Pts',(3.29392442037457,8.28006704796012,61.5175921103899));
#70822=CARTESIAN_POINT('Ctrl Pts',(-3.75784748417278,7.41114117015618,61.7827849922621));
#70823=CARTESIAN_POINT('Ctrl Pts',(-7.04794492079813,3.40943381556233,61.9949392977601));
#70824=CARTESIAN_POINT('Ctrl Pts',(-8.14312675835125,-1.65406098911481,
62.2070936032579));
#70825=CARTESIAN_POINT('Ctrl Pts',(-4.44714881737489,-7.72219630687904,
62.4722864851303));
#70826=CARTESIAN_POINT('Ctrl Pts',(4.10258681748251,-7.90984604639341,62.7905179433771));
#70827=CARTESIAN_POINT('Ctrl Pts',(8.86560663909921,-0.82704069974108,63.1087494016239));
#70828=CARTESIAN_POINT('Ctrl Pts',(5.49482911914465,7.01453747755524,63.4269808598707));
#70829=CARTESIAN_POINT('Ctrl Pts',(-2.94209291707492,8.4115122108425,63.7452123181176));
#70830=CARTESIAN_POINT('Ctrl Pts',(-7.69668026328262,3.13169987116955,64.0104051999898));
#70831=CARTESIAN_POINT('Ctrl Pts',(-7.55695562221244,-2.04699493727171,
64.2225595054878));
#70832=CARTESIAN_POINT('Ctrl Pts',(-5.06379604896171,-6.58820163115909,
64.4347138109856));
#70833=CARTESIAN_POINT('Ctrl Pts',(1.70558132560844,-8.74645303809441,64.699906692858));
#70834=CARTESIAN_POINT('Ctrl Pts',(8.28396374960744,-3.28219860273811,65.0181381511048));
#70835=CARTESIAN_POINT('Ctrl Pts',(7.23611513756351,5.18860435128682,65.3363696093517));
#70836=CARTESIAN_POINT('Ctrl Pts',(-0.450545285693165,8.89909501118893,
65.6546010675985));
#70837=CARTESIAN_POINT('Ctrl Pts',(-7.73668626251787,4.42189259042114,65.9728325258452));
#70838=CARTESIAN_POINT('Ctrl Pts',(-7.86466694643391,-2.68205983899581,
66.2380254077176));
#70839=CARTESIAN_POINT('Ctrl Pts',(-4.36357573046525,-6.50053639277595,
66.4501797132155));
#70840=CARTESIAN_POINT('Ctrl Pts',(0.496447847513485,-8.29457477469306,
66.6623340187134));
#70841=CARTESIAN_POINT('Ctrl Pts',(7.02269345367981,-5.48554692455582,66.9275269005857));
#70842=CARTESIAN_POINT('Ctrl Pts',(8.40676590719256,2.95350132120013,67.2457583588326));
#70843=CARTESIAN_POINT('Ctrl Pts',(2.06142290233261,8.66218869662343,67.5639898170793));
#70844=CARTESIAN_POINT('Ctrl Pts',(-6.17518336350058,6.42370558944248,67.8822212753262));
#70845=CARTESIAN_POINT('Ctrl Pts',(-8.74083331285178,-1.73415149367768,
68.200452733573));
#70846=CARTESIAN_POINT('Ctrl Pts',(-4.17950556618231,-7.18179395276235,
68.4656456154453));
#70847=CARTESIAN_POINT('Ctrl Pts',(0.967657358324997,-7.7692603114335,68.6777999209432));
#70848=CARTESIAN_POINT('Ctrl Pts',(5.81346630611157,-5.93717446815899,68.8899542264411));
#70849=CARTESIAN_POINT('Ctrl Pts',(8.89916685337432,0.462901414379444,69.1551471083135));
#70850=CARTESIAN_POINT('Ctrl Pts',(4.41082864532226,7.74218791697406,69.4733785665602));
#70851=CARTESIAN_POINT('Ctrl Pts',(-4.12322534511683,7.89189395162231,69.7916100248071));
#70852=CARTESIAN_POINT('Ctrl Pts',(-8.87440460098803,0.801140462714857,
70.1098414830539));
#70853=CARTESIAN_POINT('Ctrl Pts',(-5.46257080013168,-7.04058014016515,
70.4280729413007));
#70854=CARTESIAN_POINT('Ctrl Pts',(1.55332724194812,-8.16294098784365,70.6932658231731));
#70855=CARTESIAN_POINT('Ctrl Pts',(5.82480462436658,-5.23157888833839,70.9054201286709));
#70856=CARTESIAN_POINT('Ctrl Pts',(8.28228451238616,-0.670965362211112,
71.1175744341688));
#70857=CARTESIAN_POINT('Ctrl Pts',(6.41565808435416,6.18455973878933,71.3827673160413));
#70858=CARTESIAN_POINT('Ctrl Pts',(-1.7461124788672,8.73773283559258,71.7009987742879));
#70859=CARTESIAN_POINT('Ctrl Pts',(-8.28777566778471,3.25511168110842,72.0192302325349));
#70860=CARTESIAN_POINT('Ctrl Pts',(-7.22577540229245,-5.21392843232479,
72.3374616907816));
#70861=CARTESIAN_POINT('Ctrl Pts',(0.491977031632255,-8.89760716286088,
72.6556931490285));
#70862=CARTESIAN_POINT('Ctrl Pts',(6.52513642017948,-5.1448054901349,72.9208860309008));
#70863=CARTESIAN_POINT('Ctrl Pts',(7.82819621279558,-0.130783009644597,
73.1330403363986));
#70864=CARTESIAN_POINT('Ctrl Pts',(6.69335167471002,4.92397282854073,73.3451946418965));
#70865=CARTESIAN_POINT('Ctrl Pts',(0.788914170526756,8.87620315361264,73.6103875237689));
#70866=CARTESIAN_POINT('Ctrl Pts',(-7.04757446693429,5.45239440729228,73.9286189820157));
#70867=CARTESIAN_POINT('Ctrl Pts',(-8.39189027916964,-2.97646549122528,
74.2468504402625));
#70868=CARTESIAN_POINT('Ctrl Pts',(-2.0369986587134,-8.67450464967492,74.5650818985094));
#70869=CARTESIAN_POINT('Ctrl Pts',(6.20546487108924,-6.39546559481504,74.8833133567561));
#70870=CARTESIAN_POINT('Ctrl Pts',(8.30011932254924,0.394018620431757,75.1485062386285));
#70871=CARTESIAN_POINT('Ctrl Pts',(5.99624970692194,5.03397230856475,75.3606605441264));
#70872=CARTESIAN_POINT('Ctrl Pts',(1.82527669381207,8.10678228177219,75.5728148496243));
#70873=CARTESIAN_POINT('Ctrl Pts',(-5.22464446873074,7.21851914475899,75.8380077314966));
#70874=CARTESIAN_POINT('Ctrl Pts',(-8.89570313556121,-0.503244254885089,
76.1562391897434));
#70875=CARTESIAN_POINT('Ctrl Pts',(-4.38547461718753,-7.75160266377331,
76.4744706479903));
#70876=CARTESIAN_POINT('Ctrl Pts',(4.15149904988012,-7.88174229677711,76.792702106237));
#70877=CARTESIAN_POINT('Ctrl Pts',(8.87536596716089,-0.766558926037482,
77.1109335644839));
#70878=CARTESIAN_POINT('Ctrl Pts',(5.44141995481121,7.05320883494485,77.4291650227306));
#70879=CARTESIAN_POINT('Ctrl Pts',(-2.99144476000515,8.38874184385539,77.7473964809775));
#70880=CARTESIAN_POINT('Ctrl Pts',(-8.67768211916483,2.02104480277786,78.0656279392244));
#70881=CARTESIAN_POINT('Ctrl Pts',(-6.38495741585981,-6.215806244209,78.3838593974711));
#70882=CARTESIAN_POINT('Ctrl Pts',(0.408261456794656,-8.29969135305192,
78.6490522793435));
#70883=CARTESIAN_POINT('Ctrl Pts',(5.04432974985822,-5.98753915443177,78.8612065848413));
#70884=CARTESIAN_POINT('Ctrl Pts',(8.1096459834569,-1.81131815670348,79.0733608903393));
#70885=CARTESIAN_POINT('Ctrl Pts',(7.21013264266632,5.23677016069477,79.3385537722116));
#70886=CARTESIAN_POINT('Ctrl Pts',(-0.519506660206221,8.89530816120681,
79.6567852304584));
#70887=CARTESIAN_POINT('Ctrl Pts',(-7.75727281269671,4.37125700313697,79.9750166887053));
#70888=CARTESIAN_POINT('Ctrl Pts',(-7.87807304156925,-4.16327704955559,
80.2932481469521));
#70889=CARTESIAN_POINT('Ctrl Pts',(-0.744678280256665,-8.88002377539462,
80.6114796051989));
#70890=CARTESIAN_POINT('Ctrl Pts',(5.74996890814574,-5.99869340881063,80.8766724870712));
#70891=CARTESIAN_POINT('Ctrl Pts',(7.73469374172735,-1.2133725163044,81.0888267925691));
#70892=CARTESIAN_POINT('Ctrl Pts',(7.31063264471332,3.94982014366829,81.300981098067));
#70893=CARTESIAN_POINT('Ctrl Pts',(2.01027089758208,8.68148982275397,81.5661739799393));
#70894=CARTESIAN_POINT('Ctrl Pts',(-6.22479241150601,6.37564422591442,81.8844054381861));
#70895=CARTESIAN_POINT('Ctrl Pts',(-8.72316326161886,-1.78588921469291,
82.202636896433));
#70896=CARTESIAN_POINT('Ctrl Pts',(-3.21842208457843,-8.30894958346396,
82.5208683546798));
#70897=CARTESIAN_POINT('Ctrl Pts',(5.26024800698969,-7.19299928562165,82.8390998129265));
#70898=CARTESIAN_POINT('Ctrl Pts',(8.27467693081562,-0.759047397747646,
83.1042926947989));
#70899=CARTESIAN_POINT('Ctrl Pts',(6.635550072064,4.155387084025,83.3164470002968));
#70900=CARTESIAN_POINT('Ctrl Pts',(2.92993823680416,7.77572459775343,83.5286013057947));
#70901=CARTESIAN_POINT('Ctrl Pts',(-4.17450198580167,7.87292713208229,83.7937941876671));
#70902=CARTESIAN_POINT('Ctrl Pts',(-8.88034817145485,0.73232466623441,84.1120256459139));
#70903=CARTESIAN_POINT('Ctrl Pts',(-5.41530554855583,-7.06805795152009,
84.4302571041607));
#70904=CARTESIAN_POINT('Ctrl Pts',(3.01803757251667,-8.38381370803362,84.7484885624074));
#70905=CARTESIAN_POINT('Ctrl Pts',(8.68801170750906,-1.9818932801281,85.0667200206544));
#70906=CARTESIAN_POINT('Ctrl Pts',(6.74536074204024,4.85247767819652,85.3319129025265));
#70907=CARTESIAN_POINT('Ctrl Pts',(2.28544114099461,7.48829255177608,85.5440672080246));
#70908=CARTESIAN_POINT('Ctrl Pts',(-2.88622499993125,7.79205598077012,85.7562215135223));
#70909=CARTESIAN_POINT('Ctrl Pts',(-8.31405497107321,3.2071698339903,86.0214143953948));
#70910=CARTESIAN_POINT('Ctrl Pts',(-7.18514158490123,-5.26978400673226,
86.3396458536415));
#70911=CARTESIAN_POINT('Ctrl Pts',(0.545680896665126,-8.88736236220775,
86.6578773118885));
#70912=CARTESIAN_POINT('Ctrl Pts',(7.77586557562302,-4.35118347378131,86.9761087701351));
#70913=CARTESIAN_POINT('Ctrl Pts',(7.85924480189443,4.20020470331594,87.294340228382));
#70914=CARTESIAN_POINT('Ctrl Pts',(1.91127986077075,8.08662107756309,87.5595331102544));
#70915=CARTESIAN_POINT('Ctrl Pts',(-3.18437739528528,7.15244763376184,87.7716874157523));
#70916=CARTESIAN_POINT('Ctrl Pts',(-7.28833569557586,3.99081369483458,87.9838417212501));
#70917=CARTESIAN_POINT('Ctrl Pts',(-8.38029054540848,-3.02988098452613,
88.2490346031225));
#70918=CARTESIAN_POINT('Ctrl Pts',(-1.96970781328168,-8.69005950514289,
88.5672660613693));
#70919=CARTESIAN_POINT('Ctrl Pts',(6.23932108218079,-6.35246801107428,88.8854975196161));
#70920=CARTESIAN_POINT('Ctrl Pts',(8.72405210414693,1.81322860024798,89.2037289778631));
#70921=CARTESIAN_POINT('Ctrl Pts',(3.17998631222084,8.32449010209889,89.5219604361096));
#70922=CARTESIAN_POINT('Ctrl Pts',(-3.85919722697625,7.35887409333698,89.7871533179823));
#70923=CARTESIAN_POINT('Ctrl Pts',(-7.09406914206523,3.3123933276262,89.9993076234798));
#70924=CARTESIAN_POINT('Ctrl Pts',(-8.11966116127032,-1.76565392544688,
90.2114619289779));
#70925=CARTESIAN_POINT('Ctrl Pts',(-4.34075781378223,-7.7824976715668,90.4766548108502));
#70926=CARTESIAN_POINT('Ctrl Pts',(4.21074785918872,-7.85280112692049,90.7948862690971));
#70927=CARTESIAN_POINT('Ctrl Pts',(8.87612133939328,-0.705299487194537,
91.1131177273438));
#70928=CARTESIAN_POINT('Ctrl Pts',(5.39805071105593,7.08928286877416,91.4313491855907));
#70929=CARTESIAN_POINT('Ctrl Pts',(-3.05724763706058,8.37034558973175,91.7495806438375));
#70930=CARTESIAN_POINT('Ctrl Pts',(-7.73893203375542,3.02578289624382,92.0147735257097));
#70931=CARTESIAN_POINT('Ctrl Pts',(-7.52815296260325,-2.15050680560483,
92.2269278312078));
#70932=CARTESIAN_POINT('Ctrl Pts',(-4.97290886575827,-6.65707207195101,
92.4390821367053));
#70933=CARTESIAN_POINT('Ctrl Pts',(1.82544889879216,-8.72222361119875,92.7042750185781));
#70934=CARTESIAN_POINT('Ctrl Pts',(8.32822552260333,-3.1682081240484,93.0225064768246));
#70935=CARTESIAN_POINT('Ctrl Pts',(7.16423016666839,5.28741747143791,93.3407379350716));
#70936=CARTESIAN_POINT('Ctrl Pts',(-0.572625756648104,8.89207415710469,
93.6589693933183));
#70937=CARTESIAN_POINT('Ctrl Pts',(-7.79663966979729,4.31530511843589,93.9772008515652));
#70938=CARTESIAN_POINT('Ctrl Pts',(-7.82712027134826,-2.78973464977167,
94.2423937334375));
#70939=CARTESIAN_POINT('Ctrl Pts',(-4.27395752016678,-6.55980591672602,
94.4545480389354));
#70940=CARTESIAN_POINT('Ctrl Pts',(0.610228122964827,-8.28698092167651,
94.6667023444334));
#70941=CARTESIAN_POINT('Ctrl Pts',(7.09731069668704,-5.38865746550544,94.9318952263055));
#70942=CARTESIAN_POINT('Ctrl Pts',(8.36544317470014,3.06858983304855,95.2501266845525));
#70943=CARTESIAN_POINT('Ctrl Pts',(1.94235697177152,8.68966206434282,95.5683581427993));
#70944=CARTESIAN_POINT('Ctrl Pts',(-6.26275482923662,6.33835822760918,95.886589601046));
#70945=CARTESIAN_POINT('Ctrl Pts',(-8.71621234473839,-1.85393925663286,
96.2048210592929));
#70946=CARTESIAN_POINT('Ctrl Pts',(-4.08055574434818,-7.23847331801081,
96.4700139411653));
#70947=CARTESIAN_POINT('Ctrl Pts',(1.07418433525722,-7.755249484265,96.6821682466631));
#70948=CARTESIAN_POINT('Ctrl Pts',(5.89439513289042,-5.85683678922722,96.8943225521609));
#70949=CARTESIAN_POINT('Ctrl Pts',(8.89197642862596,0.584981707931448,97.1595154340334));
#70950=CARTESIAN_POINT('Ctrl Pts',(4.30416671541171,7.80198897452233,97.47774689228));
#70951=CARTESIAN_POINT('Ctrl Pts',(-4.23113808520321,7.83456749937178,97.7959783505271));
#70952=CARTESIAN_POINT('Ctrl Pts',(-8.88456304270969,0.679280952731093,
98.1142098087737));
#70953=CARTESIAN_POINT('Ctrl Pts',(-5.36543804313997,-7.11488039330814,
98.4324412670207));
#70954=CARTESIAN_POINT('Ctrl Pts',(1.6652015737725,-8.14085590567682,98.6976341488928));
#70955=CARTESIAN_POINT('Ctrl Pts',(5.8960494494909,-5.15115204963536,98.9097884543909));
#70956=CARTESIAN_POINT('Ctrl Pts',(8.29071230177075,-0.557243831330223,
99.1219427598887));
#70957=CARTESIAN_POINT('Ctrl Pts',(6.33018282299873,6.27201991652337,99.3871356417611));
#70958=CARTESIAN_POINT('Ctrl Pts',(-1.86585659316359,8.71294796532002,99.7053671000079));
#70959=CARTESIAN_POINT('Ctrl Pts',(-8.33166531913313,3.14107153822133,100.023598558254));
#70960=CARTESIAN_POINT('Ctrl Pts',(-7.15354396988856,-5.31259745731755,
100.341830016501));
#70961=CARTESIAN_POINT('Ctrl Pts',(0.614033359805018,-8.89001751623139,
100.660061474748));
#70962=CARTESIAN_POINT('Ctrl Pts',(6.59512418931417,-5.05477675924581,100.92525435662));
#70963=CARTESIAN_POINT('Ctrl Pts',(7.82925422086814,-0.0233429715947194,
101.137408662118));
#70964=CARTESIAN_POINT('Ctrl Pts',(6.62514836783461,5.01536043195949,101.349562967616));
#70965=CARTESIAN_POINT('Ctrl Pts',(0.667033260221919,8.88619800790035,101.614755849489));
#70966=CARTESIAN_POINT('Ctrl Pts',(-7.12173798479913,5.35515930187859,101.932987307735));
#70967=CARTESIAN_POINT('Ctrl Pts',(-8.3502472770763,-3.09133430899154,102.251218765982));
#70968=CARTESIAN_POINT('Ctrl Pts',(-1.91777837929849,-8.70166703342075,
102.569450224229));
#70969=CARTESIAN_POINT('Ctrl Pts',(6.29267047856448,-6.30965503447365,102.887681682476));
#70970=CARTESIAN_POINT('Ctrl Pts',(8.29388772705463,0.507796740143256,103.152874564348));
#70971=CARTESIAN_POINT('Ctrl Pts',(5.92666073856608,5.1159025635017,103.365028869846));
#70972=CARTESIAN_POINT('Ctrl Pts',(1.71371556531993,8.13078164258935,103.577183175344));
#70973=CARTESIAN_POINT('Ctrl Pts',(-5.32291690737959,7.14674779203716,103.842376057216));
#70974=CARTESIAN_POINT('Ctrl Pts',(-8.88845561260621,-0.626290583798954,
104.160607515463));
#70975=CARTESIAN_POINT('Ctrl Pts',(-4.27778007253026,-7.8091981053967,104.47883897371));
#70976=CARTESIAN_POINT('Ctrl Pts',(4.25756724672461,-7.82751583915647,104.797070431957));
#70977=CARTESIAN_POINT('Ctrl Pts',(8.88833011930044,-0.637993805762063,
105.115301890203));
#70978=CARTESIAN_POINT('Ctrl Pts',(5.92921442111081,5.8215846216282,105.380494772076));
#70979=CARTESIAN_POINT('Ctrl Pts',(1.12040947867581,7.74870628875543,105.592649077574));
#70980=CARTESIAN_POINT('Ctrl Pts',(-4.03732047235829,7.26267681793464,105.804803383071));
#70981=CARTESIAN_POINT('Ctrl Pts',(-8.70500241740163,1.90588072000468,106.069996264944));
#70982=CARTESIAN_POINT('Ctrl Pts',(-6.30043886151629,-6.30090098517042,
106.388227723191));
#70983=CARTESIAN_POINT('Ctrl Pts',(1.89050633381148,-8.70108977083264,106.706459181437));
#70984=CARTESIAN_POINT('Ctrl Pts',(8.34699657099074,-3.11841807917011,107.024690639684));
#70985=CARTESIAN_POINT('Ctrl Pts',(7.12931686426273,5.34624068433073,107.342922097931));
#70986=CARTESIAN_POINT('Ctrl Pts',(0.659632208062281,8.28319482496793,107.608114979804));
#70987=CARTESIAN_POINT('Ctrl Pts',(-4.2347656761952,6.58517472942241,107.820269285301));
#70988=CARTESIAN_POINT('Ctrl Pts',(-7.81034604051588,2.83635785571642,108.032423590799));
#70989=CARTESIAN_POINT('Ctrl Pts',(-7.82223304738392,-4.2687373494125,108.297616472671));
#70990=CARTESIAN_POINT('Ctrl Pts',(-0.625638656901327,-8.88850152408258,
108.615847930918));
#70991=CARTESIAN_POINT('Ctrl Pts',(7.13257413883672,-5.3300434850258,108.934079389165));
#70992=CARTESIAN_POINT('Ctrl Pts',(8.34696935607174,3.11849092373627,109.252310847412));
#70993=CARTESIAN_POINT('Ctrl Pts',(1.87742671362308,8.71118346384865,109.570542305659));
#70994=CARTESIAN_POINT('Ctrl Pts',(-4.93312460123469,6.68660697416714,109.835735187531));
#70995=CARTESIAN_POINT('Ctrl Pts',(-7.51519573692979,2.19535864608411,110.047889493029));
#70996=CARTESIAN_POINT('Ctrl Pts',(-7.75683706813093,-2.97958216143764,
110.260043798527));
#70997=CARTESIAN_POINT('Ctrl Pts',(-3.10710531773438,-8.35196653192304,
110.525236680399));
#70998=CARTESIAN_POINT('Ctrl Pts',(5.35568163249784,-7.12134519061905,110.843468138646));
#70999=CARTESIAN_POINT('Ctrl Pts',(8.88016920684646,0.652358993226878,111.161699596893));
#71000=CARTESIAN_POINT('Ctrl Pts',(4.25749893541349,7.82755299487516,111.47993105514));
#71001=CARTESIAN_POINT('Ctrl Pts',(-4.29427392041267,7.80824307397762,111.798162513386));
#71002=CARTESIAN_POINT('Ctrl Pts',(-8.10898828166102,1.81403974768247,112.063355395259));
#71003=CARTESIAN_POINT('Ctrl Pts',(-7.11369468768244,-3.27003278878704,
112.275509700757));
#71004=CARTESIAN_POINT('Ctrl Pts',(-3.90300928623461,-7.33573102491184,
112.487664006255));
#71005=CARTESIAN_POINT('Ctrl Pts',(3.13029117667154,-8.34330423484054,112.752856888127));
#71006=CARTESIAN_POINT('Ctrl Pts',(8.71308479343764,-1.86521753556844,113.071088346374));
#71007=CARTESIAN_POINT('Ctrl Pts',(6.27708966715128,6.31515025227515,113.389319804621));
#71008=CARTESIAN_POINT('Ctrl Pts',(-1.9178543191386,8.70165029653508,113.707551262868));
#71009=CARTESIAN_POINT('Ctrl Pts',(-8.36207449704115,3.07979845311157,114.025782721114));
#71010=CARTESIAN_POINT('Ctrl Pts',(-7.31200318078258,-3.9472826909803,114.290975602987));
#71011=CARTESIAN_POINT('Ctrl Pts',(-3.22697053921716,-7.13333215883917,
114.503129908485));
#71012=CARTESIAN_POINT('Ctrl Pts',(1.86302568448042,-8.09787419371614,114.715284213982));
#71013=CARTESIAN_POINT('Ctrl Pts',(7.83405942370468,-4.24699439035632,114.980477095855));
#71014=CARTESIAN_POINT('Ctrl Pts',(7.80167326373373,4.30473894197645,115.298708554102));
#71015=CARTESIAN_POINT('Ctrl Pts',(0.598666179718408,8.88395048407695,115.616940012348));
#71016=CARTESIAN_POINT('Ctrl Pts',(-7.15359033293806,5.31253502775477,115.935171470595));
#71017=CARTESIAN_POINT('Ctrl Pts',(-8.33303138357817,-3.15753643940262,
116.253402928842));
#71018=CARTESIAN_POINT('Ctrl Pts',(-2.9326374034684,-7.77470700528744,116.518595810714));
#71019=CARTESIAN_POINT('Ctrl Pts',(2.24074812160043,-7.501787414,116.730750116212));
#71020=CARTESIAN_POINT('Ctrl Pts',(6.71630568958916,-4.89261372297871,116.94290442171));
#71021=CARTESIAN_POINT('Ctrl Pts',(8.69967519683171,1.93005178051923,117.208097303583));
#71022=CARTESIAN_POINT('Ctrl Pts',(3.06797626001352,8.36566821841633,117.526328761829));
#71023=CARTESIAN_POINT('Ctrl Pts',(-5.3730627263302,7.10022354135342,117.844560220076));
#71024=CARTESIAN_POINT('Ctrl Pts',(-8.88455711425019,-0.679358488761448,
118.162791678323));
#71025=CARTESIAN_POINT('Ctrl Pts',(-4.22137371612796,-7.84789477214366,
118.48102313657));
#71026=CARTESIAN_POINT('Ctrl Pts',(2.8835198119009,-7.79305746499169,118.746216018442));
#71027=CARTESIAN_POINT('Ctrl Pts',(6.61065369712302,-4.19488071892606,118.95837032394));
#71028=CARTESIAN_POINT('Ctrl Pts',(8.27905598285984,0.709692321334109,119.170524629438));
#71029=CARTESIAN_POINT('Ctrl Pts',(5.30304606307633,7.16150479010844,119.43571751131));
#71030=CARTESIAN_POINT('Ctrl Pts',(-3.16881895057326,8.32799312746558,119.753948969557));
#71031=CARTESIAN_POINT('Ctrl Pts',(-8.71235895857032,1.83787343832149,120.072180427804));
#71032=CARTESIAN_POINT('Ctrl Pts',(-6.26269951380734,-6.3384128827637,120.390411886051));
#71033=CARTESIAN_POINT('Ctrl Pts',(1.9584679023929,-8.69332225798348,120.708643344297));
#71034=CARTESIAN_POINT('Ctrl Pts',(7.28694984446149,-3.99334360186924,120.97383622617));
#71035=CARTESIAN_POINT('Ctrl Pts',(7.74179179981089,1.16723017339574,121.185990531668));
#71036=CARTESIAN_POINT('Ctrl Pts',(5.7856359711068,5.96429774308113,121.398144837166));
#71037=CARTESIAN_POINT('Ctrl Pts',(-0.691712375729838,8.88431102534787,
121.663337719038));
#71038=CARTESIAN_POINT('Ctrl Pts',(-7.85310994378053,4.21017188289523,121.981569177285));
#71039=CARTESIAN_POINT('Ctrl Pts',(-7.78319610953094,-4.3249087526618,122.299800635532));
#71040=CARTESIAN_POINT('Ctrl Pts',(-0.572548155020054,-8.89207915410175,
122.618032093778));
#71041=CARTESIAN_POINT('Ctrl Pts',(7.17879440645219,-5.27961734179148,122.936263552025));
#71042=CARTESIAN_POINT('Ctrl Pts',(8.12027361919589,1.76283507670944,123.201456433897));
#71043=CARTESIAN_POINT('Ctrl Pts',(5.079982243843,5.95747823760563,123.413610739396));
#71044=CARTESIAN_POINT('Ctrl Pts',(0.457650657432336,8.29680583321317,123.625765044893));
#71045=CARTESIAN_POINT('Ctrl Pts',(-6.34757913366529,6.25441344553678,123.890957926766));
#71046=CARTESIAN_POINT('Ctrl Pts',(-8.68991501323083,-1.97034518180233,
124.209189385012));
#71047=CARTESIAN_POINT('Ctrl Pts',(-3.04080032632442,-8.36878191696348,
124.527420843259));
#71048=CARTESIAN_POINT('Ctrl Pts',(5.39811257940079,-7.08923575942719,124.845652301506));
#71049=CARTESIAN_POINT('Ctrl Pts',(8.88200340851531,0.720738410920663,125.163883759753));
#71050=CARTESIAN_POINT('Ctrl Pts',(4.97521957029455,6.65534532429735,125.429076641625));
#71051=CARTESIAN_POINT('Ctrl Pts',(-0.0706706259259978,7.82897006073825,
125.641230947123));
#71052=CARTESIAN_POINT('Ctrl Pts',(-5.09455212869252,6.56444740753711,125.853385252621));
#71053=CARTESIAN_POINT('Ctrl Pts',(-8.8935669338954,0.560281713227264,126.118578134493));
#71054=CARTESIAN_POINT('Ctrl Pts',(-5.26925699717732,-7.18552807873753,
126.43680959274));
#71055=CARTESIAN_POINT('Ctrl Pts',(3.19137931782936,-8.312525214879,126.755041050987));
#71056=CARTESIAN_POINT('Ctrl Pts',(8.72406792795749,-1.8131524649101,127.073272509233));
#71057=CARTESIAN_POINT('Ctrl Pts',(6.23363916970125,6.36798171384168,127.391503967481));
#71058=CARTESIAN_POINT('Ctrl Pts',(-0.607351258754355,8.28719226317197,
127.656696849353));
#71059=CARTESIAN_POINT('Ctrl Pts',(-5.18669973002471,5.86480284918986,127.868851154851));
#71060=CARTESIAN_POINT('Ctrl Pts',(-8.15077335549712,1.61595942573011,128.081005460349));
#71061=CARTESIAN_POINT('Ctrl Pts',(-7.08231615792921,-5.40834967850552,
128.346198342221));
#71062=CARTESIAN_POINT('Ctrl Pts',(0.732975996233196,-8.88029443552249,
128.664429800468));
#71063=CARTESIAN_POINT('Ctrl Pts',(7.86000171006385,-4.18370057676953,128.982661258715));
#71064=CARTESIAN_POINT('Ctrl Pts',(7.77582760231544,4.35125133400693,129.300892716962));
#71065=CARTESIAN_POINT('Ctrl Pts',(0.53121875048182,8.89535019237527,129.619124175208));
#71066=CARTESIAN_POINT('Ctrl Pts',(-5.89236157539941,5.8588826770164,129.884317057081));
#71067=CARTESIAN_POINT('Ctrl Pts',(-7.76160126238651,1.02728398849821,130.096471362578));
#71068=CARTESIAN_POINT('Ctrl Pts',(-7.21367397715182,-4.12423797926977,
130.308625668076));
#71069=CARTESIAN_POINT('Ctrl Pts',(-1.80121561285219,-8.72726020706794,
130.573818549949));
#71070=CARTESIAN_POINT('Ctrl Pts',(6.37610096134052,-6.2243248311298,130.892050008196));
#71071=CARTESIAN_POINT('Ctrl Pts',(8.67776168515813,1.99485075478615,131.210281466442));
#71072=CARTESIAN_POINT('Ctrl Pts',(3.01796440628899,8.38384004588583,131.528512924689));
#71073=CARTESIAN_POINT('Ctrl Pts',(-5.43146246726779,7.06460642021306,131.846744382936));
#71074=CARTESIAN_POINT('Ctrl Pts',(-8.29051835486879,0.560121920542435,
132.111937264808));
#71075=CARTESIAN_POINT('Ctrl Pts',(-6.53384985640553,-4.31353365620972,
132.324091570306));
#71076=CARTESIAN_POINT('Ctrl Pts',(-2.74236849646545,-7.84384129032964,
132.536245875804));
#71077=CARTESIAN_POINT('Ctrl Pts',(4.3623571968068,-7.77041106334294,132.801438757677));
#71078=CARTESIAN_POINT('Ctrl Pts',(8.89537322696565,-0.518862434187001,
133.119670215923));
#71079=CARTESIAN_POINT('Ctrl Pts',(5.24401287298454,7.19606186648241,133.43790167417));
#71080=CARTESIAN_POINT('Ctrl Pts',(-3.21849461415895,8.308921439709,133.756133132417));
#71081=CARTESIAN_POINT('Ctrl Pts',(-8.73309913861114,1.77268943727978,134.074364590664));
#71082=CARTESIAN_POINT('Ctrl Pts',(-6.62688905221802,-5.01306020788507,
134.339557472536));
#71083=CARTESIAN_POINT('Ctrl Pts',(-2.10495959837391,-7.54101529228778,
134.551711778034));
#71084=CARTESIAN_POINT('Ctrl Pts',(3.07250969152268,-7.72049968290824,134.763866083532));
#71085=CARTESIAN_POINT('Ctrl Pts',(8.38867380742258,-3.00659278228975,135.029058965404));
#71086=CARTESIAN_POINT('Ctrl Pts',(7.05652195652337,5.44080701272625,135.347290423651));
#71087=CARTESIAN_POINT('Ctrl Pts',(-0.758943024948333,8.87169560361212,
135.665521881898));
#71088=CARTESIAN_POINT('Ctrl Pts',(-7.87811174492057,4.16320050047685,135.983753340144));
#71089=CARTESIAN_POINT('Ctrl Pts',(-7.7561154611855,-4.38772393828678,136.301984798392));
#71090=CARTESIAN_POINT('Ctrl Pts',(-1.71653806487965,-8.13018623588088,
136.567177680264));
#71091=CARTESIAN_POINT('Ctrl Pts',(3.35521667026988,-7.07391600493298,136.779331985762));
#71092=CARTESIAN_POINT('Ctrl Pts',(7.38206860175106,-3.81464209557449,136.99148629126));
#71093=CARTESIAN_POINT('Ctrl Pts',(8.3051148879488,3.23025000639687,137.256679173132));
#71094=CARTESIAN_POINT('Ctrl Pts',(1.76045830872135,8.73485372607235,137.574910631379));
#71095=CARTESIAN_POINT('Ctrl Pts',(-6.39006882928428,6.20080621816854,137.893142089625));
#71096=CARTESIAN_POINT('Ctrl Pts',(-8.67799378202421,-2.02220349910113,
138.211373547872));
#71097=CARTESIAN_POINT('Ctrl Pts',(-2.97916651222067,-8.39845314914106,
138.529605006119));
#71098=CARTESIAN_POINT('Ctrl Pts',(4.03479898906111,-7.26407793709282,138.794797887992));
#71099=CARTESIAN_POINT('Ctrl Pts',(7.17156660737976,-3.14108244801377,139.006952193489));
#71100=CARTESIAN_POINT('Ctrl Pts',(8.07491957884542,1.96012881042716,139.219106498987));
#71101=CARTESIAN_POINT('Ctrl Pts',(4.15261858502811,7.88449156846104,139.48429938086));
#71102=CARTESIAN_POINT('Ctrl Pts',(-4.39810931656918,7.74942046298518,139.802530839106));
#71103=CARTESIAN_POINT('Ctrl Pts',(-8.89049863566354,0.491946549468975,
140.120762297353));
#71104=CARTESIAN_POINT('Ctrl Pts',(-5.22625332029457,-7.21686630780536,
140.4389937556));
#71105=CARTESIAN_POINT('Ctrl Pts',(3.25736995078038,-8.29451562236199,140.757225213847));
#71106=CARTESIAN_POINT('Ctrl Pts',(7.80936092757189,-2.83906904833273,141.022418095719));
#71107=CARTESIAN_POINT('Ctrl Pts',(7.4743401689251,2.33066634001897,141.234572401217));
#71108=CARTESIAN_POINT('Ctrl Pts',(4.8116131052624,6.7745708708046,141.446726706715));
#71109=CARTESIAN_POINT('Ctrl Pts',(-2.03437636454388,8.67587236035892,141.711919588587));
#71110=CARTESIAN_POINT('Ctrl Pts',(-8.40190465320179,2.96730201886063,142.030151046834));
#71111=CARTESIAN_POINT('Ctrl Pts',(-7.03519312179721,-5.4579332294636,142.348382505081));
#71112=CARTESIAN_POINT('Ctrl Pts',(0.785993262929414,-8.87575899082768,
142.666613963328));
#71113=CARTESIAN_POINT('Ctrl Pts',(7.89801827216467,-4.12683362620934,142.984845421574));
#71114=CARTESIAN_POINT('Ctrl Pts',(7.75787096340047,2.97688919402482,143.250038303447));
#71115=CARTESIAN_POINT('Ctrl Pts',(4.11519905014968,6.66054827525247,143.462192608945));
#71116=CARTESIAN_POINT('Ctrl Pts',(-0.809054187869451,8.26993727179055,
143.674346914443));
#71117=CARTESIAN_POINT('Ctrl Pts',(-7.22466625302864,5.21667000472345,143.939539796315));
#71118=CARTESIAN_POINT('Ctrl Pts',(-8.28934225165142,-3.26859115029452,
144.257771254562));
#71119=CARTESIAN_POINT('Ctrl Pts',(-1.73312489851915,-8.73379960178476,
144.576002712809));
#71120=CARTESIAN_POINT('Ctrl Pts',(6.41315698889781,-6.18613776991189,144.894234171056));
#71121=CARTESIAN_POINT('Ctrl Pts',(8.66917866521723,2.06271415312468,145.212465629302));
#71122=CARTESIAN_POINT('Ctrl Pts',(3.90555565176804,7.33437565218188,145.477658511175));
#71123=CARTESIAN_POINT('Ctrl Pts',(-1.26010770635471,7.72721781232174,145.689812816672));
#71124=CARTESIAN_POINT('Ctrl Pts',(-6.03334035055086,5.71360091127059,145.90196712217));
#71125=CARTESIAN_POINT('Ctrl Pts',(-8.87536457635244,-0.798343303690664,
146.167160004043));
#71126=CARTESIAN_POINT('Ctrl Pts',(-4.11556997904378,-7.90309855967184,
146.48539146229));
#71127=CARTESIAN_POINT('Ctrl Pts',(4.41805580554583,-7.73070244465686,146.803622920536));
#71128=CARTESIAN_POINT('Ctrl Pts',(8.89831309663174,-0.465732803809564,
147.121854378783));
#71129=CARTESIAN_POINT('Ctrl Pts',(5.19303537004166,7.24167330256215,147.44008583703));
#71130=CARTESIAN_POINT('Ctrl Pts',(-1.86021440597459,8.09852044425502,147.705278718902));
#71131=CARTESIAN_POINT('Ctrl Pts',(-6.01804798899972,5.00807996122836,147.9174330244));
#71132=CARTESIAN_POINT('Ctrl Pts',(-8.30170307445535,0.357991457224306,
148.129587329898));
#71133=CARTESIAN_POINT('Ctrl Pts',(-6.17774214475184,-6.42222300354386,
148.39478021177));
#71134=CARTESIAN_POINT('Ctrl Pts',(2.07454951511027,-8.66562917759421,148.713011670017));
#71135=CARTESIAN_POINT('Ctrl Pts',(8.40469207476932,-2.94009041592513,149.031243128264));
#71136=CARTESIAN_POINT('Ctrl Pts',(7.02390482802235,5.48284888355675,149.349474586511));
#71137=CARTESIAN_POINT('Ctrl Pts',(-0.827338523409895,8.87270948965367,
149.667706044757));
#71138=CARTESIAN_POINT('Ctrl Pts',(-6.71460858458054,4.89494342072968,149.93289892663));
#71139=CARTESIAN_POINT('Ctrl Pts',(-7.8275546617825,-0.164671931225144,
150.145053232128));
#71140=CARTESIAN_POINT('Ctrl Pts',(-6.50280566616276,-5.17301435045905,
150.357207537626));
#71141=CARTESIAN_POINT('Ctrl Pts',(-0.453437149148608,-8.89964261191235,
150.622400419498));
#71142=CARTESIAN_POINT('Ctrl Pts',(7.2482615574515,-5.18261314600062,150.940631877745));
#71143=CARTESIAN_POINT('Ctrl Pts',(8.27364207620721,3.29099750241855,151.258863335992));
#71144=CARTESIAN_POINT('Ctrl Pts',(1.70819408117098,8.74514775907524,151.577094794239));
#71145=CARTESIAN_POINT('Ctrl Pts',(-6.44223380417698,6.15684971685954,151.895326252485));
#71146=CARTESIAN_POINT('Ctrl Pts',(-8.27954809599393,-0.707037044381812,
152.160519134358));
#71147=CARTESIAN_POINT('Ctrl Pts',(-5.8017705655009,-5.25645685740221,152.372673439856));
#71148=CARTESIAN_POINT('Ctrl Pts',(-1.51877066045986,-8.17030114169019,
152.584827745354));
#71149=CARTESIAN_POINT('Ctrl Pts',(5.49470260574753,-7.01535214655366,152.850020627226));
#71150=CARTESIAN_POINT('Ctrl Pts',(8.86799849696601,0.837016960770842,153.168252085473));
#71151=CARTESIAN_POINT('Ctrl Pts',(4.09424988831707,7.91433764660141,153.48648354372));
#71152=CARTESIAN_POINT('Ctrl Pts',(-4.45431737341237,7.71399471716865,153.804715001966));
#71153=CARTESIAN_POINT('Ctrl Pts',(-8.14272862359425,1.65554281259527,154.069907883839));
#71154=CARTESIAN_POINT('Ctrl Pts',(-7.04798108604295,-3.4286320911007,154.2820759771));
#71155=CARTESIAN_POINT('Ctrl Pts',(-5.39382471105643,-5.40373945539631,
154.388166917611));
#71156=CARTESIAN_POINT('Ctrl Pts',(-4.37174242490101,-6.13237120108859,
154.441219281748));
#71157=CARTESIAN_POINT('Ctrl Pts',(-3.42297540299426,7.13846790764723,0.00329555398570502));
#71158=CARTESIAN_POINT('Ctrl Pts',(-4.61248760772119,6.56808466220277,0.0563367808326817));
#71159=CARTESIAN_POINT('Ctrl Pts',(-6.68124558086778,4.82084484305895,0.162416584054128));
#71160=CARTESIAN_POINT('Ctrl Pts',(-8.73125343145438,-0.246903062024332,
0.374573540024513));
#71161=CARTESIAN_POINT('Ctrl Pts',(-6.00338321156667,-7.18601493687386,
0.63976642189686));
#71162=CARTESIAN_POINT('Ctrl Pts',(2.81366832431631,-8.93427211377407,0.957997880143678));
#71163=CARTESIAN_POINT('Ctrl Pts',(9.03311162062166,-2.46519013156289,1.2762293383905));
#71164=CARTESIAN_POINT('Ctrl Pts',(6.95491649732933,6.27496220779387,1.59446079663731));
#71165=CARTESIAN_POINT('Ctrl Pts',(-0.100287973879036,8.7351568589752,1.85965367850966));
#71166=CARTESIAN_POINT('Ctrl Pts',(-5.06108046326141,6.48944842488126,2.07180798400754));
#71167=CARTESIAN_POINT('Ctrl Pts',(-8.44712147412926,2.22451783963094,2.28396228950542));
#71168=CARTESIAN_POINT('Ctrl Pts',(-7.78147446499357,-5.2150894756392,2.54915517137776));
#71169=CARTESIAN_POINT('Ctrl Pts',(0.192851584205466,-9.36462709367549,
2.86738662962458));
#71170=CARTESIAN_POINT('Ctrl Pts',(7.97527740293589,-4.89948280242022,3.1856180878714));
#71171=CARTESIAN_POINT('Ctrl Pts',(8.44062740491563,4.06086316790547,3.50384954611821));
#71172=CARTESIAN_POINT('Ctrl Pts',(1.13445937096465,9.29847198840014,3.82208100436503));
#71173=CARTESIAN_POINT('Ctrl Pts',(-5.80213362046967,6.5293858776913,4.08727388623738));
#71174=CARTESIAN_POINT('Ctrl Pts',(-8.07677783027992,1.58136138774822,4.29942819173525));
#71175=CARTESIAN_POINT('Ctrl Pts',(-7.83611087594979,-3.85912798670673,
4.51158249723313));
#71176=CARTESIAN_POINT('Ctrl Pts',(-2.45601594162407,-9.03973489175808,
4.77677537910549));
#71177=CARTESIAN_POINT('Ctrl Pts',(6.28595611954916,-6.94418193300223,5.09500683735229));
#71178=CARTESIAN_POINT('Ctrl Pts',(9.23407505830372,1.53000458735974,5.41323829559912));
#71179=CARTESIAN_POINT('Ctrl Pts',(3.7103425378918,8.600481415577,5.73146975384593));
#71180=CARTESIAN_POINT('Ctrl Pts',(-5.24033302554986,7.76451626770152,6.04970121209275));
#71181=CARTESIAN_POINT('Ctrl Pts',(-8.66202435946179,1.12553451626218,6.3148940939651));
#71182=CARTESIAN_POINT('Ctrl Pts',(-7.13512265001104,-4.10184231184789,
6.52704839946297));
#71183=CARTESIAN_POINT('Ctrl Pts',(-3.38615597408042,-8.05179736388011,
6.73920270496085));
#71184=CARTESIAN_POINT('Ctrl Pts',(4.07284419904651,-8.43568288398085,7.0043955868332));
#71185=CARTESIAN_POINT('Ctrl Pts',(9.29931124422426,-1.12148598127022,7.32262704508001));
#71186=CARTESIAN_POINT('Ctrl Pts',(5.96884097496818,7.20985368569242,7.64085850332684));
#71187=CARTESIAN_POINT('Ctrl Pts',(-2.83777377981589,8.92647525582364,7.95908996157364));
#71188=CARTESIAN_POINT('Ctrl Pts',(-9.04771061934406,2.42646614163091,8.27732141982047));
#71189=CARTESIAN_POINT('Ctrl Pts',(-7.27812150961367,-4.82974538791432,
8.54251430169281));
#71190=CARTESIAN_POINT('Ctrl Pts',(-2.69774408852947,-7.77542683556561,
8.7546686071907));
#71191=CARTESIAN_POINT('Ctrl Pts',(2.72278186451387,-8.29963566286574,8.96682291268856));
#71192=CARTESIAN_POINT('Ctrl Pts',(8.60629055567863,-3.69872522279475,9.23201579456092));
#71193=CARTESIAN_POINT('Ctrl Pts',(7.75664043211721,5.25066183436719,9.55024725280773));
#71194=CARTESIAN_POINT('Ctrl Pts',(-0.220716078597512,9.3573680688768,9.86847871105456));
#71195=CARTESIAN_POINT('Ctrl Pts',(-7.9955754646328,4.87910785714359,10.1867101693014));
#71196=CARTESIAN_POINT('Ctrl Pts',(-8.42232971392672,-4.10038627340938,
10.5049416275482));
#71197=CARTESIAN_POINT('Ctrl Pts',(-2.3284377171429,-8.41878085102033,10.7701345094205));
#71198=CARTESIAN_POINT('Ctrl Pts',(3.06134429193571,-7.63958485568192,10.9822888149184));
#71199=CARTESIAN_POINT('Ctrl Pts',(7.4977430927122,-4.48122100948196,11.1944431204163));
#71200=CARTESIAN_POINT('Ctrl Pts',(8.92324408893685,2.85035442191671,11.4596360022886));
#71201=CARTESIAN_POINT('Ctrl Pts',(2.41374714549149,9.05034503263406,11.7778674605355));
#71202=CARTESIAN_POINT('Ctrl Pts',(-6.30213737131939,6.92041308861664,12.0960989187823));
#71203=CARTESIAN_POINT('Ctrl Pts',(-9.23609288047689,-1.55868816486623,
12.4143303770291));
#71204=CARTESIAN_POINT('Ctrl Pts',(-3.67058418915988,-8.61833029719639,
12.7325618352759));
#71205=CARTESIAN_POINT('Ctrl Pts',(3.76202105532412,-7.88319039472274,12.9977547171482));
#71206=CARTESIAN_POINT('Ctrl Pts',(7.32058367569969,-3.76086961858448,13.2099090226462));
#71207=CARTESIAN_POINT('Ctrl Pts',(8.59932381098584,1.53268496892321,13.422063328144));
#71208=CARTESIAN_POINT('Ctrl Pts',(4.86841927299924,8.00295565298049,13.6872562100164));
#71209=CARTESIAN_POINT('Ctrl Pts',(-4.11171689749063,8.41597912586406,14.0054876682632));
#71210=CARTESIAN_POINT('Ctrl Pts',(-9.29594305705086,1.09292975261354,14.32371912651));
#71211=CARTESIAN_POINT('Ctrl Pts',(-5.95155746979874,-7.23283375833925,
14.6419505847568));
#71212=CARTESIAN_POINT('Ctrl Pts',(2.87949614829766,-8.91388284269106,14.9601820430037));
#71213=CARTESIAN_POINT('Ctrl Pts',(8.00934721423155,-3.485376654256,15.225374924876));
#71214=CARTESIAN_POINT('Ctrl Pts',(7.99323852829464,1.9604141069423,15.4375292303739));
#71215=CARTESIAN_POINT('Ctrl Pts',(5.48782492723469,6.79568030355847,15.6496835358718));
#71216=CARTESIAN_POINT('Ctrl Pts',(-1.57159749337621,9.2346568274136,15.9148764177441));
#71217=CARTESIAN_POINT('Ctrl Pts',(-8.62272131889369,3.65835995341979,16.2331078759909));
#71218=CARTESIAN_POINT('Ctrl Pts',(-7.7353734295505,-5.27001429499806,16.5513393342377));
#71219=CARTESIAN_POINT('Ctrl Pts',(0.248833411311902,-9.36338626916054,
16.8695707924846));
#71220=CARTESIAN_POINT('Ctrl Pts',(8.01882062248585,-4.84224340834686,17.1878022507313));
#71221=CARTESIAN_POINT('Ctrl Pts',(8.33264188932629,2.62003289376223,17.4529951326037));
#71222=CARTESIAN_POINT('Ctrl Pts',(4.74975404971919,6.72122921109588,17.6651494381016));
#71223=CARTESIAN_POINT('Ctrl Pts',(-0.312332247401522,8.72925780277937,
17.8773037435995));
#71224=CARTESIAN_POINT('Ctrl Pts',(-7.24163914455982,5.94200874294728,18.1424966254718));
#71225=CARTESIAN_POINT('Ctrl Pts',(-8.90918296215872,-2.89160499357533,
18.4607280837186));
#71226=CARTESIAN_POINT('Ctrl Pts',(-2.3850007051549,-9.05101234119646,18.7789595419654));
#71227=CARTESIAN_POINT('Ctrl Pts',(6.32731296630629,-6.906520912768,19.0971910002123));
#71228=CARTESIAN_POINT('Ctrl Pts',(9.22947229175811,1.6017635958381,19.4154224584591));
#71229=CARTESIAN_POINT('Ctrl Pts',(4.57351283593627,7.4418057996482,19.6806153403314));
#71230=CARTESIAN_POINT('Ctrl Pts',(-0.820784548616145,8.18910241514082,
19.8927696458293));
#71231=CARTESIAN_POINT('Ctrl Pts',(-5.95946801599405,6.38609694465212,20.1049239513272));
#71232=CARTESIAN_POINT('Ctrl Pts',(-9.36377367702461,-0.26181658989513,
20.3701168331995));
#71233=CARTESIAN_POINT('Ctrl Pts',(-4.83075524509748,-8.02488157258739,
20.6883482914463));
#71234=CARTESIAN_POINT('Ctrl Pts',(4.13385898897949,-8.3976343468451,21.0065797496932));
#71235=CARTESIAN_POINT('Ctrl Pts',(9.30584259734126,-1.06593341518065,21.32481120794));
#71236=CARTESIAN_POINT('Ctrl Pts',(5.91831476945442,7.26101616104393,21.6430426661868));
#71237=CARTESIAN_POINT('Ctrl Pts',(-1.42632421522254,8.61760363750972,21.9082355480591));
#71238=CARTESIAN_POINT('Ctrl Pts',(-5.98919494298574,5.64487640040296,22.120389853557));
#71239=CARTESIAN_POINT('Ctrl Pts',(-8.68687268840156,0.914186039958304,
22.3325441590549));
#71240=CARTESIAN_POINT('Ctrl Pts',(-6.89830053896013,-6.33736972848087,
22.5977370409273));
#71241=CARTESIAN_POINT('Ctrl Pts',(1.61441162876708,-9.226515896317,22.915968499174));
#71242=CARTESIAN_POINT('Ctrl Pts',(8.62741095346841,-3.62999077189642,23.2341999574209));
#71243=CARTESIAN_POINT('Ctrl Pts',(7.72514681853416,5.29688843795875,23.5524314156677));
#71244=CARTESIAN_POINT('Ctrl Pts',(-0.292411577283184,9.36286819680556,
23.8706628739145));
#71245=CARTESIAN_POINT('Ctrl Pts',(-6.72736010606789,5.57136601054333,24.1358557557869));
#71246=CARTESIAN_POINT('Ctrl Pts',(-8.22331008327924,0.335047631166753,
24.3480100612847));
#71247=CARTESIAN_POINT('Ctrl Pts',(-7.15830480606812,-5.00561340132991,
24.5601643667826));
#71248=CARTESIAN_POINT('Ctrl Pts',(-1.05313267975989,-9.30804581854349,
24.825357248655));
#71249=CARTESIAN_POINT('Ctrl Pts',(7.26862739392478,-5.90778945971974,25.1435887069018));
#71250=CARTESIAN_POINT('Ctrl Pts',(8.89412254012404,2.91609962198425,25.4618201651486));
#71251=CARTESIAN_POINT('Ctrl Pts',(2.35965828169305,9.06459780054951,25.7800516233954));
#71252=CARTESIAN_POINT('Ctrl Pts',(-6.35987628174224,6.87755618531872,26.0982830816422));
#71253=CARTESIAN_POINT('Ctrl Pts',(-8.73245037824297,-0.20445931545182,
26.3634759635146));
#71254=CARTESIAN_POINT('Ctrl Pts',(-6.42856659067376,-5.13893152612344,
26.5756302690125));
#71255=CARTESIAN_POINT('Ctrl Pts',(-2.12265792236143,-8.47300516728202,
26.7877845745103));
#71256=CARTESIAN_POINT('Ctrl Pts',(5.30799805150393,-7.71841707129861,27.0529774563827));
#71257=CARTESIAN_POINT('Ctrl Pts',(9.36171364690645,0.30534912053947,27.3712089146295));
#71258=CARTESIAN_POINT('Ctrl Pts',(4.80332334159109,8.03350095787672,27.6894403728763));
#71259=CARTESIAN_POINT('Ctrl Pts',(-4.16190117338093,8.39127517812996,28.0076718311231));
#71260=CARTESIAN_POINT('Ctrl Pts',(-9.31143726830945,1.02271276496403,28.3259032893699));
#71261=CARTESIAN_POINT('Ctrl Pts',(-6.45923814978851,-5.88011358261622,
28.5910961712423));
#71262=CARTESIAN_POINT('Ctrl Pts',(-1.48426583417955,-8.09518625940132,
28.8032504767402));
#71263=CARTESIAN_POINT('Ctrl Pts',(3.95294593835214,-7.78920481362613,29.0154047822381));
#71264=CARTESIAN_POINT('Ctrl Pts',(9.06857334260554,-2.34729268116836,29.2805976641104));
#71265=CARTESIAN_POINT('Ctrl Pts',(6.86820150300202,6.36888754856376,29.5988291223572));
#71266=CARTESIAN_POINT('Ctrl Pts',(-1.64077526014977,9.21503713013466,29.917060580604));
#71267=CARTESIAN_POINT('Ctrl Pts',(-8.64441414938049,3.60680253217169,30.2352920388509));
#71268=CARTESIAN_POINT('Ctrl Pts',(-7.70103183950281,-5.33318985300987,
30.5535234970977));
#71269=CARTESIAN_POINT('Ctrl Pts',(-1.02144169452243,-8.67491499006428,
30.81871637897));
#71270=CARTESIAN_POINT('Ctrl Pts',(4.18722350683741,-7.08535425682446,31.0308706844679));
#71271=CARTESIAN_POINT('Ctrl Pts',(8.09187707143799,-3.28922767240087,31.2430249899657));
#71272=CARTESIAN_POINT('Ctrl Pts',(8.38616890541952,4.17384432999819,31.5082178718381));
#71273=CARTESIAN_POINT('Ctrl Pts',(1.00974110375637,9.31210735523779,31.8264493300849));
#71274=CARTESIAN_POINT('Ctrl Pts',(-7.28100637975073,5.88183635118395,32.1446807883317));
#71275=CARTESIAN_POINT('Ctrl Pts',(-8.89175634629185,-2.94475628367924,
32.4629122465786));
#71276=CARTESIAN_POINT('Ctrl Pts',(-2.31764834047869,-9.07619477375616,
32.7811437048254));
#71277=CARTESIAN_POINT('Ctrl Pts',(4.91679122091634,-7.21960229583813,33.0463365866977));
#71278=CARTESIAN_POINT('Ctrl Pts',(7.80726016000046,-2.60418402479207,33.2584908921956));
#71279=CARTESIAN_POINT('Ctrl Pts',(8.26634274408729,2.82224571173855,33.4706451976935));
#71280=CARTESIAN_POINT('Ctrl Pts',(3.59511616853625,8.65008353347016,33.7358380795658));
#71281=CARTESIAN_POINT('Ctrl Pts',(-5.34342326769297,7.69303244984494,34.0540695378126));
#71282=CARTESIAN_POINT('Ctrl Pts',(-9.35404313209839,-0.333061326069361,
34.3723009960595));
#71283=CARTESIAN_POINT('Ctrl Pts',(-4.78274703090486,-8.05358624033165,
34.6905324543063));
#71284=CARTESIAN_POINT('Ctrl Pts',(4.20122408332126,-8.37248598702948,35.008763912553));
#71285=CARTESIAN_POINT('Ctrl Pts',(8.4461332449818,-2.22717902921267,35.2739567944255));
#71286=CARTESIAN_POINT('Ctrl Pts',(7.60227414268639,3.15285798924627,35.4861110999233));
#71287=CARTESIAN_POINT('Ctrl Pts',(4.39086672783747,7.55101202478985,35.6982654054212));
#71288=CARTESIAN_POINT('Ctrl Pts',(-2.95729722059006,8.88837434801064,35.9634582872935));
#71289=CARTESIAN_POINT('Ctrl Pts',(-9.07867626972295,2.30489862719791,36.2816897455404));
#71290=CARTESIAN_POINT('Ctrl Pts',(-6.84423951437506,-6.38478176870181,
36.5999212037871));
#71291=CARTESIAN_POINT('Ctrl Pts',(1.66948070495901,-9.21671062081584,36.9181526620341));
#71292=CARTESIAN_POINT('Ctrl Pts',(8.66178449584876,-3.56683259331808,37.2363841202807));
#71293=CARTESIAN_POINT('Ctrl Pts',(7.83744855060318,3.85640939693899,37.5015770021533));
#71294=CARTESIAN_POINT('Ctrl Pts',(3.6726945615586,7.36521556360778,37.713731307651));
#71295=CARTESIAN_POINT('Ctrl Pts',(-1.6358332047192,8.5802997002721,37.925885613149));
#71296=CARTESIAN_POINT('Ctrl Pts',(-8.06083755050287,4.77197059773897,38.1910784950212));
#71297=CARTESIAN_POINT('Ctrl Pts',(-8.36599980124193,-4.21247763409013,
38.5093099532681));
#71298=CARTESIAN_POINT('Ctrl Pts',(-0.981227374309102,-9.30839651089201,
38.8275414115149));
#71299=CARTESIAN_POINT('Ctrl Pts',(7.30377725708829,-5.86427815429389,39.1457728697617));
#71300=CARTESIAN_POINT('Ctrl Pts',(8.87866384941099,2.98632443824268,39.4640043280085));
#71301=CARTESIAN_POINT('Ctrl Pts',(3.38895094229788,8.05062138787126,39.7291972098809));
#71302=CARTESIAN_POINT('Ctrl Pts',(-2.05625377016801,7.96912203906943,39.9413515153788));
#71303=CARTESIAN_POINT('Ctrl Pts',(-6.86108692375931,5.4058282848024,40.1535058208766));
#71304=CARTESIAN_POINT('Ctrl Pts',(-9.21511965898805,-1.68237185895847,
40.418698702749));
#71305=CARTESIAN_POINT('Ctrl Pts',(-3.5545565124997,-8.66602841511239,40.7369301609958));
#71306=CARTESIAN_POINT('Ctrl Pts',(5.36251896376071,-7.67153460054681,41.0551616192426));
#71307=CARTESIAN_POINT('Ctrl Pts',(9.35972327190498,0.361248896814873,41.3733930774894));
#71308=CARTESIAN_POINT('Ctrl Pts',(4.74560611729256,8.07638706234402,41.6916245357363));
#71309=CARTESIAN_POINT('Ctrl Pts',(-2.71990047999163,8.30058037724426,41.9568174176086));
#71310=CARTESIAN_POINT('Ctrl Pts',(-6.77777861068786,4.66870461106876,42.1689717231065));
#71311=CARTESIAN_POINT('Ctrl Pts',(-8.724878043929,-0.417128683641938,42.3811260286043));
#71312=CARTESIAN_POINT('Ctrl Pts',(-5.85462438277968,-7.31246734952329,
42.6463189104767));
#71313=CARTESIAN_POINT('Ctrl Pts',(2.99837597541927,-8.87381890744443,42.9645503687235));
#71314=CARTESIAN_POINT('Ctrl Pts',(9.07899834941898,-2.27614624647169,43.2827818269704));
#71315=CARTESIAN_POINT('Ctrl Pts',(6.83004603724268,6.40978873452435,43.6010132852171));
#71316=CARTESIAN_POINT('Ctrl Pts',(-1.71247353183573,9.2095732693782,43.919244743464));
#71317=CARTESIAN_POINT('Ctrl Pts',(-7.49618698396174,4.48382358279551,44.1844376253363));
#71318=CARTESIAN_POINT('Ctrl Pts',(-8.17865621900968,-0.919058263749683,
44.3965919308342));
#71319=CARTESIAN_POINT('Ctrl Pts',(-6.31407658856778,-6.03572117098297,
44.6087462363321));
#71320=CARTESIAN_POINT('Ctrl Pts',(0.374235791270018,-9.35995475276541,
44.8739391182044));
#71321=CARTESIAN_POINT('Ctrl Pts',(8.08230962820882,-4.73404600377431,45.1921705764512));
#71322=CARTESIAN_POINT('Ctrl Pts',(8.34739046757811,4.23439784926572,45.510402034698));
#71323=CARTESIAN_POINT('Ctrl Pts',(0.954114111760157,9.31797117154962,45.8286334929449));
#71324=CARTESIAN_POINT('Ctrl Pts',(-7.33155845712685,5.83069944269244,46.1468649511917));
#71325=CARTESIAN_POINT('Ctrl Pts',(-8.59985536477875,-1.52969961921854,
46.412057833064));
#71326=CARTESIAN_POINT('Ctrl Pts',(-5.5725525290743,-6.05654554606999,46.624212138562));
#71327=CARTESIAN_POINT('Ctrl Pts',(-0.809810127629026,-8.69722373963903,
46.8363664440597));
#71328=CARTESIAN_POINT('Ctrl Pts',(6.41974606325721,-6.8217054967637,47.1015593259322));
#71329=CARTESIAN_POINT('Ctrl Pts',(9.20646521236131,1.72508515316507,47.4197907841789));
#71330=CARTESIAN_POINT('Ctrl Pts',(3.52613306420666,8.67037706086584,47.7380222424258));
#71331=CARTESIAN_POINT('Ctrl Pts',(-5.38926837037244,7.66098602819454,48.0562537006726));
#71332=CARTESIAN_POINT('Ctrl Pts',(-9.35868196013644,-0.404817700082644,
48.3744851589195));
#71333=CARTESIAN_POINT('Ctrl Pts',(-5.49018371862514,-6.79377479431687,
48.6396780407917));
#71334=CARTESIAN_POINT('Ctrl Pts',(-0.236279827308163,-8.22674039241056,
48.8518323462897));
#71335=CARTESIAN_POINT('Ctrl Pts',(5.09120782275439,-7.09768244750886,49.0639866517874));
#71336=CARTESIAN_POINT('Ctrl Pts',(9.32002052557175,-0.941287843438186,
49.3291795336599));
#71337=CARTESIAN_POINT('Ctrl Pts',(5.82008349782607,7.33904275572924,49.6474109919066));
#71338=CARTESIAN_POINT('Ctrl Pts',(-3.02268799572273,8.85846544524466,49.9656424501536));
#71339=CARTESIAN_POINT('Ctrl Pts',(-9.09227852322461,2.25064251897061,50.2838739084002));
#71340=CARTESIAN_POINT('Ctrl Pts',(-6.80069238510234,-6.44200190037953,
50.6021053666473));
#71341=CARTESIAN_POINT('Ctrl Pts',(0.309301864614412,-8.72936570299912,
50.8672982485194));
#71342=CARTESIAN_POINT('Ctrl Pts',(5.21575380434986,-6.36639598935869,51.0794525540174));
#71343=CARTESIAN_POINT('Ctrl Pts',(8.49788269463788,-2.02076295698556,51.2916068595152));
#71344=CARTESIAN_POINT('Ctrl Pts',(7.65412336441857,5.40029637367655,51.5567997413876));
#71345=CARTESIAN_POINT('Ctrl Pts',(-0.417740447020749,9.35737214238125,
51.8750311996344));
#71346=CARTESIAN_POINT('Ctrl Pts',(-8.09059899598044,4.7065125783663,52.1932626578812));
#71347=CARTESIAN_POINT('Ctrl Pts',(-8.34069503312267,-4.26236165247995,
52.511494116128));
#71348=CARTESIAN_POINT('Ctrl Pts',(-0.910829398031864,-9.32304645536878,
52.8297255743748));
#71349=CARTESIAN_POINT('Ctrl Pts',(5.95725072179067,-6.38816539061693,53.0949184562473));
#71350=CARTESIAN_POINT('Ctrl Pts',(8.11242535809501,-1.38695365829185,53.307072761745));
#71351=CARTESIAN_POINT('Ctrl Pts',(7.74117716265346,4.0461919574538,53.5192270672431));
#71352=CARTESIAN_POINT('Ctrl Pts',(2.23823007254506,9.09610529532493,53.7844199491152));
#71353=CARTESIAN_POINT('Ctrl Pts',(-6.45090018861527,6.79123017196538,54.1026514073622));
#71354=CARTESIAN_POINT('Ctrl Pts',(-9.1946707052259,-1.75130904940847,54.4208828656089));
#71355=CARTESIAN_POINT('Ctrl Pts',(-3.50274232572709,-8.68710059177684,
54.7391143238558));
#71356=CARTESIAN_POINT('Ctrl Pts',(5.42527760102361,-7.63643688857014,55.0573457821025));
#71357=CARTESIAN_POINT('Ctrl Pts',(8.68655480505386,-0.917201634836717,
55.322538663975));
#71358=CARTESIAN_POINT('Ctrl Pts',(7.03456419852726,4.27200095712899,55.5346929694727));
#71359=CARTESIAN_POINT('Ctrl Pts',(3.19182510211682,8.13078998238474,55.7468472749707));
#71360=CARTESIAN_POINT('Ctrl Pts',(-4.27424263307616,8.33544571782919,56.0120401568429));
#71361=CARTESIAN_POINT('Ctrl Pts',(-9.32356073321153,0.897850625775644,
56.3302716150898));
#71362=CARTESIAN_POINT('Ctrl Pts',(-5.79398361634028,-7.35110921002132,
56.6485030733367));
#71363=CARTESIAN_POINT('Ctrl Pts',(3.05131417866885,-8.85575531929058,56.9667345315834));
#71364=CARTESIAN_POINT('Ctrl Pts',(9.1033702144607,-2.20849635266917,57.2849659898303));
#71365=CARTESIAN_POINT('Ctrl Pts',(7.16004207464101,5.00312809245597,57.5501588717026));
#71366=CARTESIAN_POINT('Ctrl Pts',(2.51024845888154,7.83796774142348,57.7623131772005));
#71367=CARTESIAN_POINT('Ctrl Pts',(-2.92130261410299,8.23185788610236,57.9744674826984));
#71368=CARTESIAN_POINT('Ctrl Pts',(-8.69262923991475,3.49098872794833,58.2396603645707));
#71369=CARTESIAN_POINT('Ctrl Pts',(-7.62831519510564,-5.43541422305696,
58.5578918228176));
#71370=CARTESIAN_POINT('Ctrl Pts',(0.44535854880617,-9.34936941868726,58.8761232810643));
#71371=CARTESIAN_POINT('Ctrl Pts',(8.11043575468189,-4.68569657161741,59.1943547393112));
#71372=CARTESIAN_POINT('Ctrl Pts',(8.321435016034,4.30145611104038,59.5125861975579));
#71373=CARTESIAN_POINT('Ctrl Pts',(2.12559920025952,8.47226777551363,59.7777790794304));
#71374=CARTESIAN_POINT('Ctrl Pts',(-3.24391707018758,7.56386724385468,59.9899333849281));
#71375=CARTESIAN_POINT('Ctrl Pts',(-7.60319216260854,4.29987931907398,60.2020876904262));
#71376=CARTESIAN_POINT('Ctrl Pts',(-8.85222297610258,-3.06381360115863,
60.4672805722983));
#71377=CARTESIAN_POINT('Ctrl Pts',(-2.19571776134802,-9.10569843584722,
60.7855120305454));
#71378=CARTESIAN_POINT('Ctrl Pts',(6.46650553270306,-6.76707905669801,61.103743488792));
#71379=CARTESIAN_POINT('Ctrl Pts',(9.19599938676387,1.78003251957012,61.421974947039));
#71380=CARTESIAN_POINT('Ctrl Pts',(3.46256668934964,8.7039897359251,61.7402064052856));
#71381=CARTESIAN_POINT('Ctrl Pts',(-3.95024167581746,7.79057661041764,62.0053992871582));
#71382=CARTESIAN_POINT('Ctrl Pts',(-7.40878544758956,3.58398993197489,62.2175535926559));
#71383=CARTESIAN_POINT('Ctrl Pts',(-8.56003838042413,-1.73874556672825,
62.4297078981539));
#71384=CARTESIAN_POINT('Ctrl Pts',(-4.67483384329524,-8.11755714109021,
62.6949007800261));
#71385=CARTESIAN_POINT('Ctrl Pts',(4.3126309658217,-8.31481416778063,63.0131322382731));
#71386=CARTESIAN_POINT('Ctrl Pts',(9.31950776998579,-0.869383511031748,
63.3313636965197));
#71387=CARTESIAN_POINT('Ctrl Pts',(5.7761532577777,7.37366761081306,63.6495951547667));
#71388=CARTESIAN_POINT('Ctrl Pts',(-3.09272212459566,8.84216462532336,63.9678266130134));
#71389=CARTESIAN_POINT('Ctrl Pts',(-8.09073472766302,3.29203657129424,64.2330194948858));
#71390=CARTESIAN_POINT('Ctrl Pts',(-7.94385646753675,-2.15179693839514,
64.4451738003837));
#71391=CARTESIAN_POINT('Ctrl Pts',(-5.32305216608538,-6.92550423126613,
64.6573281058815));
#71392=CARTESIAN_POINT('Ctrl Pts',(1.79290364026012,-9.19425374557529,64.9225209877539));
#71393=CARTESIAN_POINT('Ctrl Pts',(8.70808594081639,-3.45024053356348,65.2407524460007));
#71394=CARTESIAN_POINT('Ctrl Pts',(7.60658959891365,5.4542504010889,65.5589839042475));
#71395=CARTESIAN_POINT('Ctrl Pts',(-0.473612293177449,9.35471067900242,
65.8772153624943));
#71396=CARTESIAN_POINT('Ctrl Pts',(-8.13278895315451,4.64828454859746,66.1954468207411));
#71397=CARTESIAN_POINT('Ctrl Pts',(-8.2673219892696,-2.81937587878726,66.4606397026135));
#71398=CARTESIAN_POINT('Ctrl Pts',(-4.58698198334685,-6.83335070996431,
66.6727940081113));
#71399=CARTESIAN_POINT('Ctrl Pts',(0.521864973333528,-8.71924022892736,
66.8849483136093));
#71400=CARTESIAN_POINT('Ctrl Pts',(7.38224115642129,-5.76639583359743,67.1501411954815));
#71401=CARTESIAN_POINT('Ctrl Pts',(8.83717532052503,3.10471461594072,67.4683726537285));
#71402=CARTESIAN_POINT('Ctrl Pts',(2.16696358608828,9.10567524023015,67.7866041119752));
#71403=CARTESIAN_POINT('Ctrl Pts',(-6.49134026355597,6.75258632487546,68.1048355702222));
#71404=CARTESIAN_POINT('Ctrl Pts',(-9.18834630176509,-1.82293654315669,
68.4230670284687));
#71405=CARTESIAN_POINT('Ctrl Pts',(-4.39348779890017,-7.54948727930569,
68.6882599103413));
#71406=CARTESIAN_POINT('Ctrl Pts',(1.01719945816525,-8.16703072749937,68.9004142158391));
#71407=CARTESIAN_POINT('Ctrl Pts',(6.11110402433387,-6.24114579410071,69.112568521337));
#71408=CARTESIAN_POINT('Ctrl Pts',(9.35478619936243,0.486601030664479,69.3777614032093));
#71409=CARTESIAN_POINT('Ctrl Pts',(4.63665415188428,8.13857228119282,69.6959928614562));
#71410=CARTESIAN_POINT('Ctrl Pts',(-4.33432614433332,8.29594296206201,70.0142243197029));
#71411=CARTESIAN_POINT('Ctrl Pts',(-9.32875616973107,0.842157234248181,
70.3324557779499));
#71412=CARTESIAN_POINT('Ctrl Pts',(-5.74224337806769,-7.40104360508217,
70.6506872361965));
#71413=CARTESIAN_POINT('Ctrl Pts',(1.63285445542184,-8.58086705839598,70.915880118069));
#71414=CARTESIAN_POINT('Ctrl Pts',(6.12302284155387,-5.49942514752871,71.1280344235668));
#71415=CARTESIAN_POINT('Ctrl Pts',(8.70632073004518,-0.70531743185354,71.3401887290648));
#71416=CARTESIAN_POINT('Ctrl Pts',(6.7441268038012,6.50119669029752,71.605381610937));
#71417=CARTESIAN_POINT('Ctrl Pts',(-1.83550990659903,9.18508708634037,71.9236130691839));
#71418=CARTESIAN_POINT('Ctrl Pts',(-8.71209302149546,3.42176681632458,72.2418445274307));
#71419=CARTESIAN_POINT('Ctrl Pts',(-7.59572049010687,-5.48087102386278,
72.5600759856775));
#71420=CARTESIAN_POINT('Ctrl Pts',(0.517165260720624,-9.35314665584888,
72.8783074439244));
#71421=CARTESIAN_POINT('Ctrl Pts',(6.85921020902198,-5.40820912682017,73.1435003257966));
#71422=CARTESIAN_POINT('Ctrl Pts',(8.22898402782439,-0.137478835253676,
73.3556546312946));
#71423=CARTESIAN_POINT('Ctrl Pts',(7.03603774439987,5.17607027954607,73.5678089367924));
#71424=CARTESIAN_POINT('Ctrl Pts',(0.829304980625463,9.3306468046128,73.8330018186647));
#71425=CARTESIAN_POINT('Ctrl Pts',(-7.4083960272372,5.73154597449478,74.1512332769116));
#71426=CARTESIAN_POINT('Ctrl Pts',(-8.82153809043052,-3.1288545050304,74.4694647351584));
#71427=CARTESIAN_POINT('Ctrl Pts',(-2.14128887058924,-9.11862174517115,
74.7876961934052));
#71428=CARTESIAN_POINT('Ctrl Pts',(6.52317212309447,-6.72290049963323,75.105927651652));
#71429=CARTESIAN_POINT('Ctrl Pts',(8.72506864642096,0.41419157696923,75.3711205335244));
#71430=CARTESIAN_POINT('Ctrl Pts',(6.30324556561973,5.29170151049384,75.5832748390223));
#71431=CARTESIAN_POINT('Ctrl Pts',(1.91872716925317,8.52183314014436,75.7954291445202));
#71432=CARTESIAN_POINT('Ctrl Pts',(-5.49213569966153,7.58809272686213,76.0606220263924));
#71433=CARTESIAN_POINT('Ctrl Pts',(-9.351145146202,-0.529009343018155,76.3788534846394));
#71434=CARTESIAN_POINT('Ctrl Pts',(-4.61000204878283,-8.1484690439886,76.6970849428861));
#71435=CARTESIAN_POINT('Ctrl Pts',(4.36404740560219,-8.28527156301856,77.0153164011329));
#71436=CARTESIAN_POINT('Ctrl Pts',(9.32976675590779,-0.805805192827627,
77.3335478593798));
#71437=CARTESIAN_POINT('Ctrl Pts',(5.72000965224047,7.41431886349542,77.6517793176265));
#71438=CARTESIAN_POINT('Ctrl Pts',(-3.14460068207903,8.81822846159531,77.9700107758735));
#71439=CARTESIAN_POINT('Ctrl Pts',(-9.12196189467311,2.12451820949349,78.2882422341201));
#71440=CARTESIAN_POINT('Ctrl Pts',(-6.71185432316634,-6.53404295360445,
78.6064736923671));
#71441=CARTESIAN_POINT('Ctrl Pts',(0.429163617750448,-8.72461876575088,
78.8716665742392));
#71442=CARTESIAN_POINT('Ctrl Pts',(5.30258923183553,-6.29408905045752,79.0838208797373));
#71443=CARTESIAN_POINT('Ctrl Pts',(8.52484345756404,-1.90405398327316,79.2959751852351));
#71444=CARTESIAN_POINT('Ctrl Pts',(7.57927685282243,5.50488220253219,79.5611680671074));
#71445=CARTESIAN_POINT('Ctrl Pts',(-0.546104350604037,9.35072994995942,
79.8793995253544));
#71446=CARTESIAN_POINT('Ctrl Pts',(-8.15442949307008,4.59505652164535,80.197630983601));
#71447=CARTESIAN_POINT('Ctrl Pts',(-8.28141444936442,-4.37642841504223,
80.515862441848));
#71448=CARTESIAN_POINT('Ctrl Pts',(-0.782804302232367,-9.33466303450356,
80.8340939000947));
#71449=CARTESIAN_POINT('Ctrl Pts',(6.04435568800383,-6.30581438010313,81.0992867819672));
#71450=CARTESIAN_POINT('Ctrl Pts',(8.13069441932884,-1.27549473531918,81.3114410874649));
#71451=CARTESIAN_POINT('Ctrl Pts',(7.68492225173183,4.15204294725026,81.5235953929629));
#71452=CARTESIAN_POINT('Ctrl Pts',(2.11319270213992,9.12596454498564,81.7887882748351));
#71453=CARTESIAN_POINT('Ctrl Pts',(-6.54348919449422,6.70206431672992,82.1070197330821));
#71454=CARTESIAN_POINT('Ctrl Pts',(-9.16977157964343,-1.877323130858,82.4252511913288));
#71455=CARTESIAN_POINT('Ctrl Pts',(-3.38319878665011,-8.73435099883718,
82.7434826495756));
#71456=CARTESIAN_POINT('Ctrl Pts',(5.52956206707782,-7.56126630254611,83.0617141078225));
#71457=CARTESIAN_POINT('Ctrl Pts',(8.69832365568315,-0.797909089480057,
83.3269069896948));
#71458=CARTESIAN_POINT('Ctrl Pts',(6.9752768165914,4.36813449923239,83.5390612951928));
#71459=CARTESIAN_POINT('Ctrl Pts',(3.0799451492746,8.17382597220634,83.7512156006905));
#71460=CARTESIAN_POINT('Ctrl Pts',(-4.38822804532377,8.27600507971838,84.0164084825631));
#71461=CARTESIAN_POINT('Ctrl Pts',(-9.33500403898603,0.769818208155055,
84.3346399408096));
#71462=CARTESIAN_POINT('Ctrl Pts',(-5.69255824119631,-7.42992822480975,
84.6528713990567));
#71463=CARTESIAN_POINT('Ctrl Pts',(3.17255499281213,-8.81304801518571,84.9711028573032));
#71464=CARTESIAN_POINT('Ctrl Pts',(9.1328203370509,-2.08336220806071,85.2893343155504));
#71465=CARTESIAN_POINT('Ctrl Pts',(7.09070957079878,5.10091472208982,85.5545271974224));
#71466=CARTESIAN_POINT('Ctrl Pts',(2.40245110553475,7.87167798675258,85.7666815029205));
#71467=CARTESIAN_POINT('Ctrl Pts',(-3.03399388307664,8.19099348900591,85.9788358084183));
#71468=CARTESIAN_POINT('Ctrl Pts',(-8.73971777196734,3.37137044358746,86.2440286902905));
#71469=CARTESIAN_POINT('Ctrl Pts',(-7.55300630343952,-5.53958629072243,
86.5622601485375));
#71470=CARTESIAN_POINT('Ctrl Pts',(0.573618655037129,-9.3423773421205,86.8804916067843));
#71471=CARTESIAN_POINT('Ctrl Pts',(8.17397416785781,-4.57395526818167,87.1987230650311));
#71472=CARTESIAN_POINT('Ctrl Pts',(8.26162224189486,4.41524668999585,87.5169545232779));
#71473=CARTESIAN_POINT('Ctrl Pts',(2.00913352443477,8.50063972305202,87.7821474051502));
#71474=CARTESIAN_POINT('Ctrl Pts',(-3.34741107811517,7.51863848811937,87.9943017106483));
#71475=CARTESIAN_POINT('Ctrl Pts',(-7.66148374389044,4.19513528533351,88.2064560161458));
#71476=CARTESIAN_POINT('Ctrl Pts',(-8.80934447375909,-3.18500476356538,
88.4716488980186));
#71477=CARTESIAN_POINT('Ctrl Pts',(-2.07055286995459,-9.1349729777823,88.789880356265));
#71478=CARTESIAN_POINT('Ctrl Pts',(6.55876170372602,-6.67770152655952,89.1081118145122));
#71479=CARTESIAN_POINT('Ctrl Pts',(9.17070592911142,1.90606223766466,89.4263432727587));
#71480=CARTESIAN_POINT('Ctrl Pts',(3.342795180477,8.75068716059845,89.7445747310057));
#71481=CARTESIAN_POINT('Ctrl Pts',(-4.05678032049151,7.73563356496568,90.0097676128779));
#71482=CARTESIAN_POINT('Ctrl Pts',(-7.45727113570789,3.48198116730271,90.2219219183759));
#71483=CARTESIAN_POINT('Ctrl Pts',(-8.53537139222743,-1.85605183572463,
90.4340762238736));
#71484=CARTESIAN_POINT('Ctrl Pts',(-4.56299583547458,-8.18094581370174,
90.6992691057461));
#71485=CARTESIAN_POINT('Ctrl Pts',(4.42632963412773,-8.25484866379338,91.0175005639929));
#71486=CARTESIAN_POINT('Ctrl Pts',(9.33056080167088,-0.741409394601718,
91.3357320222397));
#71487=CARTESIAN_POINT('Ctrl Pts',(5.67441999091111,7.45223981490379,91.6539634804866));
#71488=CARTESIAN_POINT('Ctrl Pts',(-3.21377253336565,8.79889035646353,91.9721949387333));
#71489=CARTESIAN_POINT('Ctrl Pts',(-8.13514970333771,3.18069686144963,92.2373878206056));
#71490=CARTESIAN_POINT('Ctrl Pts',(-7.91357917000356,-2.26060840505348,
92.4495421261036));
#71491=CARTESIAN_POINT('Ctrl Pts',(-5.22751174290429,-6.99790069934896,
92.6616964316014));
#71492=CARTESIAN_POINT('Ctrl Pts',(1.91890819078105,-9.16878382102207,92.9268893134739));
#71493=CARTESIAN_POINT('Ctrl Pts',(8.7546138270785,-3.33041397288932,93.2451207717205));
#71494=CARTESIAN_POINT('Ctrl Pts',(7.5310242628826,5.55812255316062,93.5633522299674));
#71495=CARTESIAN_POINT('Ctrl Pts',(-0.60194303736029,9.34733037138744,93.8815836882144));
#71496=CARTESIAN_POINT('Ctrl Pts',(-8.19581185364207,4.53624001359984,94.199815146461));
#71497=CARTESIAN_POINT('Ctrl Pts',(-8.2278530003507,-2.93256342212263,94.4650080283335));
#71498=CARTESIAN_POINT('Ctrl Pts',(-4.49277550191721,-6.89565471367907,
94.6771623338312));
#71499=CARTESIAN_POINT('Ctrl Pts',(0.641470568788609,-8.7112575859935,94.8893166393294));
#71500=CARTESIAN_POINT('Ctrl Pts',(7.46067865137102,-5.66454583018452,95.1545095212014));
#71501=CARTESIAN_POINT('Ctrl Pts',(8.79373694769651,3.22569542685074,95.4727409794484));
#71502=CARTESIAN_POINT('Ctrl Pts',(2.04180172067109,9.13455518881701,95.7909724376951));
#71503=CARTESIAN_POINT('Ctrl Pts',(-6.58339521124076,6.66286935071541,96.109203895942));
#71504=CARTESIAN_POINT('Ctrl Pts',(-9.1624647898756,-1.94885719732676,96.4274353541887));
#71505=CARTESIAN_POINT('Ctrl Pts',(-4.28947194629567,-7.60906851343142,
96.6926282360612));
#71506=CARTESIAN_POINT('Ctrl Pts',(1.12918040088547,-8.15230257431412,96.904782541559));
#71507=CARTESIAN_POINT('Ctrl Pts',(6.19617624338033,-6.15669498847559,97.1169368470568));
#71508=CARTESIAN_POINT('Ctrl Pts',(9.34722763940825,0.614931588361719,97.3821297289294));
#71509=CARTESIAN_POINT('Ctrl Pts',(4.52453134686614,8.20143503195108,97.700361187176));
#71510=CARTESIAN_POINT('Ctrl Pts',(-4.44776379847873,8.23568151138829,98.0185926454229));
#71511=CARTESIAN_POINT('Ctrl Pts',(-9.33943470312532,0.714058763791374,
98.3368241036697));
#71512=CARTESIAN_POINT('Ctrl Pts',(-5.64013762035087,-7.47914788092769,
98.6550555619165));
#71513=CARTESIAN_POINT('Ctrl Pts',(1.75045652679066,-8.55765126468515,98.9202484437888));
#71514=CARTESIAN_POINT('Ctrl Pts',(6.19791525764518,-5.41488061733235,99.1324027492867));
#71515=CARTESIAN_POINT('Ctrl Pts',(8.71518000520262,-0.585773588572133,
99.3445570547845));
#71516=CARTESIAN_POINT('Ctrl Pts',(6.65427538192215,6.59313465225967,99.6097499366571));
#71517=CARTESIAN_POINT('Ctrl Pts',(-1.96138467738728,9.1590332808326,99.9279813949035));
#71518=CARTESIAN_POINT('Ctrl Pts',(-8.75822973423427,3.30188804874659,100.24621285315));
#71519=CARTESIAN_POINT('Ctrl Pts',(-7.5197909544385,-5.58459170339549,100.564444311397));
#71520=CARTESIAN_POINT('Ctrl Pts',(0.645470626059692,-9.34516843466058,
100.882675769644));
#71521=CARTESIAN_POINT('Ctrl Pts',(6.93278121039915,-5.31357110697587,101.147868651516));
#71522=CARTESIAN_POINT('Ctrl Pts',(8.23009620377064,-0.0245380845330745,
101.360022957014));
#71523=CARTESIAN_POINT('Ctrl Pts',(6.96434256614091,5.27213674344548,101.572177262512));
#71524=CARTESIAN_POINT('Ctrl Pts',(0.70118401419441,9.34115337522732,101.837370144385));
#71525=CARTESIAN_POINT('Ctrl Pts',(-7.48635656723482,5.62933262832376,102.155601602631));
#71526=CARTESIAN_POINT('Ctrl Pts',(-8.77776305084519,-3.24960437396555,
102.473833060878));
#71527=CARTESIAN_POINT('Ctrl Pts',(-2.01596475396907,-9.14717478803391,
102.792064519125));
#71528=CARTESIAN_POINT('Ctrl Pts',(6.61484248131537,-6.63269661213821,103.110295977372));
#71529=CARTESIAN_POINT('Ctrl Pts',(8.71851800583927,0.533794906314948,103.375488859244));
#71530=CARTESIAN_POINT('Ctrl Pts',(6.23009378281474,5.37782642879489,103.587643164742));
#71531=CARTESIAN_POINT('Ctrl Pts',(1.80145433659379,8.54706121970112,103.79979747024));
#71532=CARTESIAN_POINT('Ctrl Pts',(-5.59543948843153,7.5126468260251,104.064990352112));
#71533=CARTESIAN_POINT('Ctrl Pts',(-9.34352656472846,-0.658355395134159,
104.383221810359));
#71534=CARTESIAN_POINT('Ctrl Pts',(-4.49679376123124,-8.20901325574707,
104.701453268606));
#71535=CARTESIAN_POINT('Ctrl Pts',(4.47554607962198,-8.22826882043062,105.019684726852));
#71536=CARTESIAN_POINT('Ctrl Pts',(9.34339464641931,-0.670657798393084,
105.3379161851));
#71537=CARTESIAN_POINT('Ctrl Pts',(6.23277820874136,6.11963798118718,105.603109066971));
#71538=CARTESIAN_POINT('Ctrl Pts',(1.17777217816441,8.14542438042699,105.81526337247));
#71539=CARTESIAN_POINT('Ctrl Pts',(-4.24402311581608,7.63451118360377,106.027417677967));
#71540=CARTESIAN_POINT('Ctrl Pts',(-9.15068093692945,2.0034579585802,106.29261055984));
#71541=CARTESIAN_POINT('Ctrl Pts',(-6.62300858976339,-6.62349437321487,
106.610842018087));
#71542=CARTESIAN_POINT('Ctrl Pts',(1.98729643490681,-9.14656797076846,106.929073476333));
#71543=CARTESIAN_POINT('Ctrl Pts',(8.77434591518241,-3.27807477840434,107.24730493458));
#71544=CARTESIAN_POINT('Ctrl Pts',(7.49432346999941,5.61995739559459,107.565536392827));
#71545=CARTESIAN_POINT('Ctrl Pts',(0.693404043131489,8.70727764879019,107.830729274699));
#71546=CARTESIAN_POINT('Ctrl Pts',(-4.45157711479331,6.92232235828129,108.042883580197));
#71547=CARTESIAN_POINT('Ctrl Pts',(-8.21021996282278,2.98157364192402,108.255037885695));
#71548=CARTESIAN_POINT('Ctrl Pts',(-8.22271556040278,-4.48728806897804,
108.520230767568));
#71549=CARTESIAN_POINT('Ctrl Pts',(-0.657670090896665,-9.34357482677965,
108.838462225814));
#71550=CARTESIAN_POINT('Ctrl Pts',(7.49774751044503,-5.60293093244015,109.156693684061));
#71551=CARTESIAN_POINT('Ctrl Pts',(8.77431730691419,3.278151352466,109.474925142308));
#71552=CARTESIAN_POINT('Ctrl Pts',(1.97354716461479,9.15717844045453,109.793156600555));
#71553=CARTESIAN_POINT('Ctrl Pts',(-5.1856906044942,7.02894772882912,110.058349482427));
#71554=CARTESIAN_POINT('Ctrl Pts',(-7.89995856057946,2.30775656905988,110.270503787925));
#71555=CARTESIAN_POINT('Ctrl Pts',(-8.1539714392633,-3.13213074245472,110.482658093423));
#71556=CARTESIAN_POINT('Ctrl Pts',(-3.26618282646103,-8.77957032806362,
110.747850975295));
#71557=CARTESIAN_POINT('Ctrl Pts',(5.62988170121529,-7.4859436627864,111.066082433542));
#71558=CARTESIAN_POINT('Ctrl Pts',(9.33481591175152,0.685758454406295,111.384313891789));
#71559=CARTESIAN_POINT('Ctrl Pts',(4.4754742709089,8.22830787844749,111.702545350036));
#71560=CARTESIAN_POINT('Ctrl Pts',(-4.51413206077047,8.20800932865017,112.020776808283));
#71561=CARTESIAN_POINT('Ctrl Pts',(-8.5241520827663,1.90691491420638,112.285969690155));
#71562=CARTESIAN_POINT('Ctrl Pts',(-7.47790146957128,-3.43745185454216,
112.498123995653));
#71563=CARTESIAN_POINT('Ctrl Pts',(-4.10283546858128,-7.71130561824021,
112.71027830115));
#71564=CARTESIAN_POINT('Ctrl Pts',(3.29055575448777,-8.77046453888797,112.975471183023));
#71565=CARTESIAN_POINT('Ctrl Pts',(9.15917711427336,-1.96071290133453,113.29370264127));
#71566=CARTESIAN_POINT('Ctrl Pts',(6.59846396386631,6.63847317397886,113.611934099517));
#71567=CARTESIAN_POINT('Ctrl Pts',(-2.0160445817765,9.1471571942533,113.930165557764));
#71568=CARTESIAN_POINT('Ctrl Pts',(-8.79019580055429,3.23747790559259,114.24839701601));
#71569=CARTESIAN_POINT('Ctrl Pts',(-7.68636295647619,-4.14937558211616,
114.513589897883));
#71570=CARTESIAN_POINT('Ctrl Pts',(-3.39218490487877,-7.49854433953852,
114.72574420338));
#71571=CARTESIAN_POINT('Ctrl Pts',(1.95840883190445,-8.51246897599455,114.937898508878));
#71572=CARTESIAN_POINT('Ctrl Pts',(8.23514742327505,-4.46443191438829,115.203091390751));
#71573=CARTESIAN_POINT('Ctrl Pts',(8.20110315740802,4.52513287027477,115.521322848998));
#71574=CARTESIAN_POINT('Ctrl Pts',(0.629316677428787,9.33879078272935,115.839554307244));
#71575=CARTESIAN_POINT('Ctrl Pts',(-7.51983969118302,5.58452607756445,116.157785765491));
#71576=CARTESIAN_POINT('Ctrl Pts',(-8.75966573841591,-3.31919591957222,
116.476017223738));
#71577=CARTESIAN_POINT('Ctrl Pts',(-3.08278250781349,-8.17275628106395,
116.74121010561));
#71578=CARTESIAN_POINT('Ctrl Pts',(2.35546989393181,-7.88586375863123,116.953364411108));
#71579=CARTESIAN_POINT('Ctrl Pts',(7.06016695842124,-5.14310565119636,117.165518716606));
#71580=CARTESIAN_POINT('Ctrl Pts',(9.1450809734394,2.02886652851272,117.430711598479));
#71581=CARTESIAN_POINT('Ctrl Pts',(3.2250504401161,8.79397351319627,117.748943056725));
#71582=CARTESIAN_POINT('Ctrl Pts',(-5.64815267190185,7.46374062779295,118.067174514972));
#71583=CARTESIAN_POINT('Ctrl Pts',(-9.3394284711406,-0.714140269510792,
118.385405973219));
#71584=CARTESIAN_POINT('Ctrl Pts',(-4.43749951345246,-8.2496911135747,118.703637431466));
#71585=CARTESIAN_POINT('Ctrl Pts',(3.03115019488987,-8.19204624719432,118.968830313338));
#71586=CARTESIAN_POINT('Ctrl Pts',(6.94910579760224,-4.40965012837104,119.180984618836));
#71587=CARTESIAN_POINT('Ctrl Pts',(8.70292690633611,0.746027132966607,119.393138924334));
#71588=CARTESIAN_POINT('Ctrl Pts',(5.57455129708413,7.52815935255504,119.658331806206));
#71589=CARTESIAN_POINT('Ctrl Pts',(-3.33105607249802,8.75436953377928,119.976563264453));
#71590=CARTESIAN_POINT('Ctrl Pts',(-9.15841411812871,1.93196884160687,120.2947947227));
#71591=CARTESIAN_POINT('Ctrl Pts',(-6.58333706377255,-6.66292680410411,
120.613026180947));
#71592=CARTESIAN_POINT('Ctrl Pts',(2.05873749836002,-9.13840277696978,120.931257639193));
#71593=CARTESIAN_POINT('Ctrl Pts',(7.66002694000164,-4.19779471849209,121.196450521066));
#71594=CARTESIAN_POINT('Ctrl Pts',(8.1381558836316,1.22698999776883,121.408604826563));
#71595=CARTESIAN_POINT('Ctrl Pts',(6.08184883245779,6.26965772584783,121.620759132062));
#71596=CARTESIAN_POINT('Ctrl Pts',(-0.727126650508542,9.33916978298414,
121.885952013934));
#71597=CARTESIAN_POINT('Ctrl Pts',(-8.25517329145266,4.42572416901183,122.204183472181));
#71598=CARTESIAN_POINT('Ctrl Pts',(-8.18168001027664,-4.54633533447753,
122.522414930428));
#71599=CARTESIAN_POINT('Ctrl Pts',(-0.601861462684696,-9.3473356242207,
122.840646388674));
#71600=CARTESIAN_POINT('Ctrl Pts',(7.54633416229053,-5.54992307264971,123.158877846921));
#71601=CARTESIAN_POINT('Ctrl Pts',(8.53601520676025,1.85308866763243,123.424070728793));
#71602=CARTESIAN_POINT('Ctrl Pts',(5.34006706141108,6.2624890754831,123.636225034291));
#71603=CARTESIAN_POINT('Ctrl Pts',(0.481081445579293,8.72158551313186,123.848379339789));
#71604=CARTESIAN_POINT('Ctrl Pts',(-6.67256234851482,6.57462676556356,124.113572221662));
#71605=CARTESIAN_POINT('Ctrl Pts',(-9.13482108817629,-2.07122287045563,
124.431803679908));
#71606=CARTESIAN_POINT('Ctrl Pts',(-3.19648315358039,-8.79724662681214,
124.750035138155));
#71607=CARTESIAN_POINT('Ctrl Pts',(5.674485026791,-7.45219029365284,125.068266596402));
#71608=CARTESIAN_POINT('Ctrl Pts',(9.33674402083647,0.757638760001384,125.386498054649));
#71609=CARTESIAN_POINT('Ctrl Pts',(5.22994075083988,6.99608554570746,125.651690936521));
#71610=CARTESIAN_POINT('Ctrl Pts',(-0.074288819055751,8.22979749521674,
125.863845242019));
#71611=CARTESIAN_POINT('Ctrl Pts',(-5.35538289490079,6.90053383943257,126.075999547517));
#71612=CARTESIAN_POINT('Ctrl Pts',(-9.34889957533105,0.588967003878703,
126.341192429389));
#71613=CARTESIAN_POINT('Ctrl Pts',(-5.53903229934317,-7.55341258497928,
126.659423887636));
#71614=CARTESIAN_POINT('Ctrl Pts',(3.35477148493349,-8.73810969534923,126.977655345883));
#71615=CARTESIAN_POINT('Ctrl Pts',(9.17072256306931,-1.90598220435038,127.29588680413));
#71616=CARTESIAN_POINT('Ctrl Pts',(6.55278888881734,6.69400949953583,127.614118262377));
#71617=CARTESIAN_POINT('Ctrl Pts',(-0.638446414948493,8.71147974774613,
127.879311144249));
#71618=CARTESIAN_POINT('Ctrl Pts',(-5.45224826706981,6.1650688945985,128.091465449747));
#71619=CARTESIAN_POINT('Ctrl Pts',(-8.56807646788026,1.69869328035053,128.303619755244));
#71620=CARTESIAN_POINT('Ctrl Pts',(-7.44491642255176,-5.68524624466725,
128.568812637117));
#71621=CARTESIAN_POINT('Ctrl Pts',(0.770502884933684,-9.33494755188252,
128.887044095364));
#71622=CARTESIAN_POINT('Ctrl Pts',(8.26241790223238,-4.39789758554576,129.205275553611));
#71623=CARTESIAN_POINT('Ctrl Pts',(8.17393425039314,4.57402660271456,129.523507011857));
#71624=CARTESIAN_POINT('Ctrl Pts',(0.558416076215122,9.35077413303877,129.841738470104));
#71625=CARTESIAN_POINT('Ctrl Pts',(-6.19403857185828,6.15884562158216,130.106931351977));
#71626=CARTESIAN_POINT('Ctrl Pts',(-8.1589795506303,1.07987885121863,130.319085657474));
#71627=CARTESIAN_POINT('Ctrl Pts',(-7.58299949647197,-4.33539062330698,
130.531239962973));
#71628=CARTESIAN_POINT('Ctrl Pts',(-1.89343420960715,-9.17407828041441,
130.796432844844));
#71629=CARTESIAN_POINT('Ctrl Pts',(6.70254443608692,-6.54299767494756,131.114664303092));
#71630=CARTESIAN_POINT('Ctrl Pts',(9.12204553428414,2.09698307921827,131.432895761338));
#71631=CARTESIAN_POINT('Ctrl Pts',(3.1724780806205,8.81307570148307,131.751127219585));
#71632=CARTESIAN_POINT('Ctrl Pts',(-5.70954236147284,7.42629998207919,132.069358677832));
#71633=CARTESIAN_POINT('Ctrl Pts',(-8.71497612861151,0.588799030131614,
132.334551559705));
#71634=CARTESIAN_POINT('Ctrl Pts',(-6.86836975556092,-4.53437785609103,
132.546705865202));
#71635=CARTESIAN_POINT('Ctrl Pts',(-2.88277221755536,-8.2454301016891,132.7588601707));
#71636=CARTESIAN_POINT('Ctrl Pts',(4.58570106323024,-8.16824039557919,133.024053052572));
#71637=CARTESIAN_POINT('Ctrl Pts',(9.3507983469536,-0.545427141514346,133.342284510819));
#71638=CARTESIAN_POINT('Ctrl Pts',(5.51249572704322,7.56448568135409,133.660515969066));
#71639=CARTESIAN_POINT('Ctrl Pts',(-3.38327502959951,8.7343214141785,133.978747427313));
#71640=CARTESIAN_POINT('Ctrl Pts',(-9.18021615344449,1.8634475515343,134.29697888556));
#71641=CARTESIAN_POINT('Ctrl Pts',(-6.96617237004453,-5.26971875255023,
134.562171767432));
#71642=CARTESIAN_POINT('Ctrl Pts',(-2.21272927292213,-7.92710002495654,
134.77432607293));
#71643=CARTESIAN_POINT('Ctrl Pts',(3.22981597415152,-8.11577365340277,134.986480378428));
#71644=CARTESIAN_POINT('Ctrl Pts',(8.8181569418351,-3.16052425246951,135.2516732603));
#71645=CARTESIAN_POINT('Ctrl Pts',(7.41780161019791,5.7193653287612,135.569904718547));
#71646=CARTESIAN_POINT('Ctrl Pts',(-0.797799373005577,9.32590847716784,
135.888136176794));
#71647=CARTESIAN_POINT('Ctrl Pts',(-8.28145513424959,4.3763479468045,136.206367635041));
#71648=CARTESIAN_POINT('Ctrl Pts',(-8.15321288750148,-4.61236653057451,
136.524599093288));
#71649=CARTESIAN_POINT('Ctrl Pts',(-1.80442134242299,-8.54643532937329,
136.78979197516));
#71650=CARTESIAN_POINT('Ctrl Pts',(3.52699697848842,-7.43608619871,137.001946280658));
#71651=CARTESIAN_POINT('Ctrl Pts',(7.76001558530448,-4.00994405646551,137.214100586155));
#71652=CARTESIAN_POINT('Ctrl Pts',(8.73031997466621,3.39563227414694,137.479293468028));
#71653=CARTESIAN_POINT('Ctrl Pts',(1.85059021392886,9.18206057223537,137.797524926275));
#71654=CARTESIAN_POINT('Ctrl Pts',(-6.71722743062202,6.51827495656469,138.115756384522));
#71655=CARTESIAN_POINT('Ctrl Pts',(-9.12228951404036,-2.12573622872636,
138.433987842768));
#71656=CARTESIAN_POINT('Ctrl Pts',(-3.1316938128374,-8.82843696607267,138.752219301015));
#71657=CARTESIAN_POINT('Ctrl Pts',(4.24137253767331,-7.63598403722936,139.017412182888));
#71658=CARTESIAN_POINT('Ctrl Pts',(7.53873631452235,-3.30189951709841,139.229566488385));
#71659=CARTESIAN_POINT('Ctrl Pts',(8.48833913126387,2.06048344152671,139.441720793883));
#71660=CARTESIAN_POINT('Ctrl Pts',(4.36522425868474,8.28816159185334,139.706913675756));
#71661=CARTESIAN_POINT('Ctrl Pts',(-4.62328361922247,8.14617511893268,140.025145134002));
#71662=CARTESIAN_POINT('Ctrl Pts',(-9.34567418643476,0.517133217931129,
140.343376592249));
#71663=CARTESIAN_POINT('Ctrl Pts',(-5.49382692117094,-7.58635526799968,
140.661608050496));
#71664=CARTESIAN_POINT('Ctrl Pts',(3.42414070483787,-8.71917804811639,140.979839508743));
#71665=CARTESIAN_POINT('Ctrl Pts',(8.20918441408827,-2.98442364211942,141.245032390615));
#71666=CARTESIAN_POINT('Ctrl Pts',(7.85701127011543,2.44999174329057,141.457186696113));
#71667=CARTESIAN_POINT('Ctrl Pts',(5.0579579656616,7.12141519908443,141.669341001611));
#71668=CARTESIAN_POINT('Ctrl Pts',(-2.13853232026243,9.12005947987599,141.934533883483));
#71669=CARTESIAN_POINT('Ctrl Pts',(-8.8320651801613,3.11922188141106,142.25276534173));
#71670=CARTESIAN_POINT('Ctrl Pts',(-7.39538078226736,-5.73736837316092,
142.570996799977));
#71671=CARTESIAN_POINT('Ctrl Pts',(0.82623452846722,-9.3301799015914,142.889228258224));
#71672=CARTESIAN_POINT('Ctrl Pts',(8.30238083543134,-4.3381191621197,143.20745971647));
#71673=CARTESIAN_POINT('Ctrl Pts',(8.15505826787976,3.12929990055637,143.472652598343));
#71674=CARTESIAN_POINT('Ctrl Pts',(4.32588891929462,7.00155487722944,143.684806903841));
#71675=CARTESIAN_POINT('Ctrl Pts',(-0.850476126127729,8.69334133570097,
143.896961209339));
#71676=CARTESIAN_POINT('Ctrl Pts',(-7.59455455464446,5.48375295922304,144.162154091211));
#71677=CARTESIAN_POINT('Ctrl Pts',(-8.71373981128762,-3.43593640707434,
144.480385549458));
#71678=CARTESIAN_POINT('Ctrl Pts',(-1.82185738840104,-9.18095247891603,
144.798617007704));
#71679=CARTESIAN_POINT('Ctrl Pts',(6.74149765731627,-6.5028555134215,145.116848465952));
#71680=CARTESIAN_POINT('Ctrl Pts',(9.11302308107979,2.16832094631068,145.435079924198));
#71681=CARTESIAN_POINT('Ctrl Pts',(4.10551220288046,7.70988085316744,145.700272806071));
#71682=CARTESIAN_POINT('Ctrl Pts',(-1.32462267258781,8.1228357374562,145.912427111569));
#71683=CARTESIAN_POINT('Ctrl Pts',(-6.34223517519423,6.00612572323542,146.124581417066));
#71684=CARTESIAN_POINT('Ctrl Pts',(-9.32976529389266,-0.839216866339801,
146.389774298939));
#71685=CARTESIAN_POINT('Ctrl Pts',(-4.32627883899791,-8.30772122338493,
146.708005757186));
#71686=CARTESIAN_POINT('Ctrl Pts',(4.64425132809667,-8.12649877591966,147.026237215432));
#71687=CARTESIAN_POINT('Ctrl Pts',(9.35388873200124,-0.489577381506351,
147.344468673679));
#71688=CARTESIAN_POINT('Ctrl Pts',(5.45890827904218,7.6124323307205,147.662700131926));
#71689=CARTESIAN_POINT('Ctrl Pts',(-1.95545362162443,8.51314831325412,147.927893013798));
#71690=CARTESIAN_POINT('Ctrl Pts',(-6.32615987565755,5.26448352733551,148.140047319296));
#71691=CARTESIAN_POINT('Ctrl Pts',(-8.72673348322189,0.376319895862742,
148.352201624794));
#71692=CARTESIAN_POINT('Ctrl Pts',(-6.49403004923184,-6.75102783357787,
148.617394506666));
#71693=CARTESIAN_POINT('Ctrl Pts',(2.18076225489512,-9.10929186686864,148.935625964913));
#71694=CARTESIAN_POINT('Ctrl Pts',(8.83499531207604,-3.09061709943564,149.25385742316));
#71695=CARTESIAN_POINT('Ctrl Pts',(7.3835145506797,5.76355965835638,149.572088881407));
#71696=CARTESIAN_POINT('Ctrl Pts',(-0.869696582671238,9.32697427212434,
149.890320339654));
#71697=CARTESIAN_POINT('Ctrl Pts',(-7.05838296506824,5.14555462476081,150.155513221526));
#71698=CARTESIAN_POINT('Ctrl Pts',(-8.22830963069686,-0.173102801086107,
150.367667527024));
#71699=CARTESIAN_POINT('Ctrl Pts',(-6.83573616555874,-5.43786222374656,
150.579821832522));
#71700=CARTESIAN_POINT('Ctrl Pts',(-0.476652214192424,-9.35528631577552,
150.845014714394));
#71701=CARTESIAN_POINT('Ctrl Pts',(7.61935789093666,-5.44795245820723,151.163246172641));
#71702=CARTESIAN_POINT('Ctrl Pts',(8.69723581861135,3.45948991911445,151.481477630888));
#71703=CARTESIAN_POINT('Ctrl Pts',(1.79565016362255,9.19288163891025,151.799709089134));
#71704=CARTESIAN_POINT('Ctrl Pts',(-6.77206314673528,6.47206797128248,152.117940547382));
#71705=CARTESIAN_POINT('Ctrl Pts',(-8.70344421466748,-0.743235911204164,
152.383133429254));
#71706=CARTESIAN_POINT('Ctrl Pts',(-6.09880948545569,-5.52557681829827,
152.595287734752));
#71707=CARTESIAN_POINT('Ctrl Pts',(-1.5965286468446,-8.58860403723511,152.807442040249));
#71708=CARTESIAN_POINT('Ctrl Pts',(5.77602026715138,-7.37452398921601,153.072634922122));
#71709=CARTESIAN_POINT('Ctrl Pts',(9.32202208613815,0.879870536452235,153.390866380369));
#71710=CARTESIAN_POINT('Ctrl Pts',(4.30386720274188,8.31953572883633,153.709097838616));
#71711=CARTESIAN_POINT('Ctrl Pts',(-4.68236941490573,8.10893564657233,154.027329296862));
#71712=CARTESIAN_POINT('Ctrl Pts',(-8.55961986197294,1.74030325657316,154.292522178735));
#71713=CARTESIAN_POINT('Ctrl Pts',(-7.40882346442135,-3.60417112039676,
154.504690271996));
#71714=CARTESIAN_POINT('Ctrl Pts',(-5.66997762825804,-5.68039998745807,
154.610781212507));
#71715=CARTESIAN_POINT('Ctrl Pts',(-4.59556679602214,-6.44633620500796,
154.663833576644));
#71716=CARTESIAN_POINT('Ctrl Pts',(-3.93864885562957,-5.51416611762882,
-4.5102810375397E-17));
#71717=CARTESIAN_POINT('Ctrl Pts',(-4.08585763522341,-5.42754158645561,
-9.48998345292704E-15));
#71718=CARTESIAN_POINT('Ctrl Pts',(-4.22926307194498,-5.33519815285744,
-8.48289216403754E-15));
#71719=CARTESIAN_POINT('Ctrl Pts',(-4.36847541855169,-5.23720844074822,
-7.17481629664007E-15));
#71720=CARTESIAN_POINT('Ctrl Pts',(-4.5153143814705,-5.13385045524223,-6.2635930340045E-15));
#71721=CARTESIAN_POINT('Ctrl Pts',(-4.65748939328674,-5.02421136591519,
-8.76666634847064E-15));
#71722=CARTESIAN_POINT('Ctrl Pts',(-4.79490097280245,-4.90875376760295,
-7.57727214306669E-15));
#71723=CARTESIAN_POINT('Ctrl Pts',(-4.9348947149667,-4.79112655375393,-6.36552749745673E-15));
#71724=CARTESIAN_POINT('Ctrl Pts',(-5.06994473026214,-4.66745971743739,
-3.71552428771349E-15));
#71725=CARTESIAN_POINT('Ctrl Pts',(-5.19991919475653,-4.53819530501257,
-3.6498581934552E-15));
#71726=CARTESIAN_POINT('Ctrl Pts',(-5.23498113790099,-4.50332490568703,
-3.6321440919018E-15));
#71727=CARTESIAN_POINT('Ctrl Pts',(-5.26967356318341,-4.46804692542487,
-2.38309310078048E-15));
#71728=CARTESIAN_POINT('Ctrl Pts',(-5.30399349825367,-4.43236952795225,
-3.17801340798951E-15));
#71729=CARTESIAN_POINT('Ctrl Pts',(-5.33072700462355,-4.40457862652305,
-3.79721641792535E-15));
#71730=CARTESIAN_POINT('Ctrl Pts',(-5.35723606352971,-4.37654348380284,
-3.20335373337224E-15));
#71731=CARTESIAN_POINT('Ctrl Pts',(-5.38349836887505,-4.34829087335799,
-2.5951463200613E-15));
#71732=CARTESIAN_POINT('Ctrl Pts',(-5.51182776783945,-4.21023595129815,
3.76827799100414E-16));
#71733=CARTESIAN_POINT('Ctrl Pts',(-5.63438296049573,-4.06687452090324,
1.5979460223273E-16));
#71734=CARTESIAN_POINT('Ctrl Pts',(-5.75105261248448,-3.91872155205454,
7.7715611723761E-16));
#71735=CARTESIAN_POINT('Ctrl Pts',(-5.86802410885443,-3.77018528608921,
1.39611485226759E-15));
#71736=CARTESIAN_POINT('Ctrl Pts',(-5.97907994344739,-3.61683206879924,
2.92190851021412E-15));
#71737=CARTESIAN_POINT('Ctrl Pts',(-6.08407689566617,-3.45913508104809,
2.33146835171283E-15));
#71738=CARTESIAN_POINT('Ctrl Pts',(-6.16258753371837,-3.3412184095103,1.889971407316E-15));
#71739=CARTESIAN_POINT('Ctrl Pts',(-6.23770993659032,-3.22087206005872,
2.51853654700645E-15));
#71740=CARTESIAN_POINT('Ctrl Pts',(-6.3093710339331,-3.09828019800675,2.4980018054066E-15));
#71741=CARTESIAN_POINT('Ctrl Pts',(-6.3341774208916,-3.05584348853973,2.49089344724426E-15));
#71742=CARTESIAN_POINT('Ctrl Pts',(-6.35856893839169,-3.01313761181226,
1.25464931670994E-15));
#71743=CARTESIAN_POINT('Ctrl Pts',(-6.38254220714328,-2.9701699351918,2.13717932240343E-15));
#71744=CARTESIAN_POINT('Ctrl Pts',(-6.4036413320246,-2.9323536330317,2.9139032224517E-15));
#71745=CARTESIAN_POINT('Ctrl Pts',(-6.42441971552428,-2.89432817575107,
3.01420564380196E-15));
#71746=CARTESIAN_POINT('Ctrl Pts',(-6.44485308977601,-2.85614028785739,
2.44249065417534E-15));
#71747=CARTESIAN_POINT('Ctrl Pts',(-6.47726144497496,-2.79557238458748,
1.53572203984232E-15));
#71748=CARTESIAN_POINT('Ctrl Pts',(-6.50881123945918,-2.73458002559567,
4.5774480660375E-15));
#71749=CARTESIAN_POINT('Ctrl Pts',(-6.53949852066889,-2.67318520039554,
4.35762537165374E-15));
#71750=CARTESIAN_POINT('Ctrl Pts',(-6.62571770655248,-2.50068989818723,
3.74001009257501E-15));
#71751=CARTESIAN_POINT('Ctrl Pts',(-6.70512878428164,-2.32502421973284,
2.90696192907388E-15));
#71752=CARTESIAN_POINT('Ctrl Pts',(-6.77760467320117,-2.1466793262714,4.57966997657877E-15));
#71753=CARTESIAN_POINT('Ctrl Pts',(-6.85107121035924,-1.96589669720997,
6.2752417006187E-15));
#71754=CARTESIAN_POINT('Ctrl Pts',(-6.91741213237192,-1.78236052985066,
6.40827725235636E-15));
#71755=CARTESIAN_POINT('Ctrl Pts',(-6.97645624116144,-1.59654609617019,
6.41153796721028E-15));
#71756=CARTESIAN_POINT('Ctrl Pts',(-7.03541281540019,-1.41100713761017,
6.41479384796279E-15));
#71757=CARTESIAN_POINT('Ctrl Pts',(-7.08709457358015,-1.22319598087583,
8.11353623083457E-15));
#71758=CARTESIAN_POINT('Ctrl Pts',(-7.13128646726196,-1.03355947757627,
5.93969318174459E-15));
#71759=CARTESIAN_POINT('Ctrl Pts',(-7.1748356573002,-0.84668094777523,3.79746536186948E-15));
#71760=CARTESIAN_POINT('Ctrl Pts',(-7.21111152210714,-0.658029091154123,
4.52783243078309E-15));
#71761=CARTESIAN_POINT('Ctrl Pts',(-7.23986029137286,-0.468016202745084,
4.27435864480685E-15));
#71762=CARTESIAN_POINT('Ctrl Pts',(-7.24843435095544,-0.411346582852196,
4.19876238802472E-15));
#71763=CARTESIAN_POINT('Ctrl Pts',(-7.25633855027266,-0.354555835328044,
3.81851370664238E-15));
#71764=CARTESIAN_POINT('Ctrl Pts',(-7.26356525899322,-0.297654766670134,
2.33146835171283E-15));
#71765=CARTESIAN_POINT('Ctrl Pts',(-7.26643816125284,-0.275034343591875,
2.05066034735898E-15));
#71766=CARTESIAN_POINT('Ctrl Pts',(-7.26920381458604,-0.25239753682228,
6.88911783367723E-15));
#71767=CARTESIAN_POINT('Ctrl Pts',(-7.27186036178065,-0.229757926941342,
6.82787160144471E-15));
#71768=CARTESIAN_POINT('Ctrl Pts',(-7.29508985368643,-0.0317916963596518,
2.89494710093888E-15));
#71769=CARTESIAN_POINT('Ctrl Pts',(-7.31001436370851,0.166647965845849,
3.28825056680269E-15));
#71770=CARTESIAN_POINT('Ctrl Pts',(-7.31647360189607,0.365072157842635,
3.10862446895044E-15));
#71771=CARTESIAN_POINT('Ctrl Pts',(-7.32239953343523,0.547113467257426,
2.84891488009813E-15));
#71772=CARTESIAN_POINT('Ctrl Pts',(-7.32120010776079,0.729142519857608,
3.27746221103623E-15));
#71773=CARTESIAN_POINT('Ctrl Pts',(-7.31271643791274,0.910797816932271,
3.88578058618805E-15));
#71774=CARTESIAN_POINT('Ctrl Pts',(-7.30374392664761,1.10292035689018,4.19327191292733E-15));
#71775=CARTESIAN_POINT('Ctrl Pts',(-7.28662463969137,1.29462530195052,4.84441888438171E-15));
#71776=CARTESIAN_POINT('Ctrl Pts',(-7.26166737560021,1.48549791199764,3.33066907387547E-15));
#71777=CARTESIAN_POINT('Ctrl Pts',(-7.23635360931169,1.67909704305478,1.8476684640108E-15));
#71778=CARTESIAN_POINT('Ctrl Pts',(-7.20297622264173,1.87184053501143,2.85422380346747E-15));
#71779=CARTESIAN_POINT('Ctrl Pts',(-7.16180345191425,2.06329674672944,3.1641356201817E-15));
#71780=CARTESIAN_POINT('Ctrl Pts',(-7.13907515744559,2.16898487703731,4.63215597939171E-15));
#71781=CARTESIAN_POINT('Ctrl Pts',(-7.11397044673297,2.2742806998604,2.85116288317276E-15));
#71782=CARTESIAN_POINT('Ctrl Pts',(-7.08652776855258,2.3791106285664,1.49880108324396E-15));
#71783=CARTESIAN_POINT('Ctrl Pts',(-7.07123960516252,2.43751079883005,-4.23777917910264E-16));
#71784=CARTESIAN_POINT('Ctrl Pts',(-7.05522576098077,2.49576635929609,6.98375336362743E-16));
#71785=CARTESIAN_POINT('Ctrl Pts',(-7.03849227337608,2.55386441534103,9.43689570931383E-16));
#71786=CARTESIAN_POINT('Ctrl Pts',(-7.02101618737152,2.6145407458302,1.00858386228158E-15));
#71787=CARTESIAN_POINT('Ctrl Pts',(-7.00277560991787,2.67497411182156,3.28000556455198E-16));
#71788=CARTESIAN_POINT('Ctrl Pts',(-6.98378477400738,2.73514402802049,5.55111512312578E-16));
#71789=CARTESIAN_POINT('Ctrl Pts',(-6.92410274331356,2.92423853667474,1.26884750067373E-15));
#71790=CARTESIAN_POINT('Ctrl Pts',(-6.85700877086983,3.11075193737884,2.68086629815529E-15));
#71791=CARTESIAN_POINT('Ctrl Pts',(-6.78285079805515,3.29425396444948,1.66533453693773E-15));
#71792=CARTESIAN_POINT('Ctrl Pts',(-6.70769973559542,3.48021336671545,6.36203238974364E-16));
#71793=CARTESIAN_POINT('Ctrl Pts',(-6.62529404332015,3.6630808733105,-9.33836692105665E-17));
#71794=CARTESIAN_POINT('Ctrl Pts',(-6.53594209786488,3.84240790796595,-2.77555756156289E-16));
#71795=CARTESIAN_POINT('Ctrl Pts',(-6.44578821461818,4.0233444109478,-4.63380795994014E-16));
#71796=CARTESIAN_POINT('Ctrl Pts',(-6.34856261409735,4.20067733546166,1.67798683334567E-15));
#71797=CARTESIAN_POINT('Ctrl Pts',(-6.24453069856692,4.37393447487679,-7.7715611723761E-16));
#71798=CARTESIAN_POINT('Ctrl Pts',(-6.22727537286666,4.40267189026762,-1.18438010265586E-15));
#71799=CARTESIAN_POINT('Ctrl Pts',(-6.2098326865377,4.43129713518358,-1.42691211972322E-15));
#71800=CARTESIAN_POINT('Ctrl Pts',(-6.19220372232323,4.45980800258806,-1.22124532708767E-15));
#71801=CARTESIAN_POINT('Ctrl Pts',(-6.08596170519876,4.63163046624324,-1.41530437407216E-15));
#71802=CARTESIAN_POINT('Ctrl Pts',(-5.97295776163549,4.79930104647229,-1.50003702229236E-15));
#71803=CARTESIAN_POINT('Ctrl Pts',(-5.85345634600849,4.96251156798406,1.88737914186277E-15));
#71804=CARTESIAN_POINT('Ctrl Pts',(-5.81488241610479,5.01519438503113,2.98080513171597E-15));
#71805=CARTESIAN_POINT('Ctrl Pts',(-5.77563115178433,5.06741226883694,-1.31746641749658E-15));
#71806=CARTESIAN_POINT('Ctrl Pts',(-5.73571051010428,5.11915416998263,-2.66453525910038E-15));
#71807=CARTESIAN_POINT('Ctrl Pts',(-5.72137816578353,5.13773059340222,-2.96003365710495E-15));
#71808=CARTESIAN_POINT('Ctrl Pts',(-5.70695815007714,5.15624742332188,1.25829997975076E-15));
#71809=CARTESIAN_POINT('Ctrl Pts',(-5.69245532260261,5.17469841337795,9.99200722162641E-16));
#71810=CARTESIAN_POINT('Ctrl Pts',(-5.56612038982047,5.33542600891682,-5.38442201744225E-16));
#71811=CARTESIAN_POINT('Ctrl Pts',(-5.43376647828372,5.4908295940974,6.83770205204893E-17));
#71812=CARTESIAN_POINT('Ctrl Pts',(-5.2957647648533,5.64065053822135,-7.7715611723761E-16));
#71813=CARTESIAN_POINT('Ctrl Pts',(-5.15609478068988,5.79228263301915,3.30164136699358E-16));
#71814=CARTESIAN_POINT('Ctrl Pts',(-5.01063933152216,5.93819685285966,-2.71421503180125E-15));
#71815=CARTESIAN_POINT('Ctrl Pts',(-4.85973389667245,6.07810484637022,-1.22124532708767E-15));
#71816=CARTESIAN_POINT('Ctrl Pts',(-4.7089054661251,6.21794144737296,5.73169886049089E-16));
#71817=CARTESIAN_POINT('Ctrl Pts',(-4.55263221916868,6.35177848028246,-5.16154924826819E-16));
#71818=CARTESIAN_POINT('Ctrl Pts',(-4.39120541678212,6.47929982942619,1.55431223447522E-15));
#71819=CARTESIAN_POINT('Ctrl Pts',(-4.23176612557716,6.60525111645157,2.78351566838913E-15));
#71820=CARTESIAN_POINT('Ctrl Pts',(-4.06729895549648,6.72504173207748,-1.21935944349465E-15));
#71821=CARTESIAN_POINT('Ctrl Pts',(-3.89804823092294,6.83833238416448,-5.55111512312578E-16));
#71822=CARTESIAN_POINT('Ctrl Pts',(-3.74289087714262,6.94218941538343,-1.70801214086168E-15));
#71823=CARTESIAN_POINT('Ctrl Pts',(-3.58371283294784,7.04058382880945,1.8720578375122E-15));
#71824=CARTESIAN_POINT('Ctrl Pts',(-3.42067962509758,7.13322310757502,-1.77635683940025E-15));
#71825=CARTESIAN_POINT('Origin',(-2.30940107675851,-4.,-10.));
#71826=CARTESIAN_POINT('',(-2.30940107675851,-4.,-10.));
#71827=CARTESIAN_POINT('',(2.3094010767585,-4.,-10.));
#71828=CARTESIAN_POINT('',(-1.15470053837925,-4.,-10.));
#71829=CARTESIAN_POINT('',(-2.30940107675851,-4.,-6.));
#71830=CARTESIAN_POINT('',(-2.30940107675851,-4.,-10.));
#71831=CARTESIAN_POINT('',(2.3094010767585,-4.,-6.));
#71832=CARTESIAN_POINT('',(-2.30940107675851,-4.,-6.));
#71833=CARTESIAN_POINT('',(2.3094010767585,-4.,-10.));
#71834=CARTESIAN_POINT('Origin',(-4.61880215351701,5.6564012731995E-16,
-10.));
#71835=CARTESIAN_POINT('',(-4.61880215351701,5.6564012731995E-16,-10.));
#71836=CARTESIAN_POINT('',(-4.04145188432738,-0.999999999999999,-10.));
#71837=CARTESIAN_POINT('',(-4.61880215351701,5.55111512312578E-16,-6.));
#71838=CARTESIAN_POINT('',(-4.61880215351701,5.6564012731995E-16,-10.));
#71839=CARTESIAN_POINT('',(-4.61880215351701,5.6564012731995E-16,-6.));
#71840=CARTESIAN_POINT('Origin',(-2.3094010767585,4.,-10.));
#71841=CARTESIAN_POINT('',(-2.3094010767585,4.,-10.));
#71842=CARTESIAN_POINT('',(-2.88675134594813,3.,-10.));
#71843=CARTESIAN_POINT('',(-2.3094010767585,4.,-6.));
#71844=CARTESIAN_POINT('',(-2.3094010767585,4.,-10.));
#71845=CARTESIAN_POINT('',(-2.3094010767585,4.,-6.));
#71846=CARTESIAN_POINT('Origin',(2.3094010767585,4.,-10.));
#71847=CARTESIAN_POINT('',(2.3094010767585,4.,-10.));
#71848=CARTESIAN_POINT('',(1.15470053837925,4.,-10.));
#71849=CARTESIAN_POINT('',(2.3094010767585,4.,-6.));
#71850=CARTESIAN_POINT('',(2.3094010767585,4.,-10.));
#71851=CARTESIAN_POINT('',(2.3094010767585,4.,-6.));
#71852=CARTESIAN_POINT('Origin',(4.61880215351701,0.,-10.));
#71853=CARTESIAN_POINT('',(4.61880215351701,0.,-10.));
#71854=CARTESIAN_POINT('',(4.04145188432738,1.,-10.));
#71855=CARTESIAN_POINT('',(4.61880215351701,0.,-6.));
#71856=CARTESIAN_POINT('',(4.61880215351701,0.,-10.));
#71857=CARTESIAN_POINT('',(4.61880215351701,0.,-6.));
#71858=CARTESIAN_POINT('Origin',(2.3094010767585,-4.,-10.));
#71859=CARTESIAN_POINT('',(2.88675134594813,-3.,-10.));
#71860=CARTESIAN_POINT('',(2.3094010767585,-4.,-6.));
#71861=CARTESIAN_POINT('Origin',(0.,0.,-6.));
#71862=CARTESIAN_POINT('Origin',(0.,0.,0.));
#71863=CARTESIAN_POINT('',(-45.,5.51091059616309E-15,0.));
#71864=CARTESIAN_POINT('Origin',(0.,0.,0.));
#71865=CARTESIAN_POINT('Origin',(0.,0.,-10.));
#71866=CARTESIAN_POINT('',(-45.,5.51091059616309E-15,-10.));
#71867=CARTESIAN_POINT('',(-45.,-5.51091059616309E-15,-10.));
#71868=CARTESIAN_POINT('Origin',(0.,0.,-10.));
#71869=CARTESIAN_POINT('Origin',(0.,0.,-10.));
#105783=UNCERTAINTY_MEASURE_WITH_UNIT(LENGTH_MEASURE(0.01),#105807,
'DISTANCE_ACCURACY_VALUE',
'Maximum model space distance between geometric entities at asserted c
onnectivities');
#105792=UNCERTAINTY_MEASURE_WITH_UNIT(LENGTH_MEASURE(0.01),#105807,
'DISTANCE_ACCURACY_VALUE',
'Maximum model space distance between geometric entities at asserted c
onnectivities');
#105797=(
GEOMETRIC_REPRESENTATION_CONTEXT(3)
GLOBAL_UNCERTAINTY_ASSIGNED_CONTEXT((#105783))
GLOBAL_UNIT_ASSIGNED_CONTEXT((#105807,#105809,#105810))
REPRESENTATION_CONTEXT('','3D')
);
#105806=(
GEOMETRIC_REPRESENTATION_CONTEXT(3)
GLOBAL_UNCERTAINTY_ASSIGNED_CONTEXT((#105792))
GLOBAL_UNIT_ASSIGNED_CONTEXT((#105807,#105809,#105810))
REPRESENTATION_CONTEXT('','3D')
);
#105807=(
LENGTH_UNIT()
NAMED_UNIT(*)
SI_UNIT(.MILLI.,.METRE.)
);
#105809=(
NAMED_UNIT(*)
PLANE_ANGLE_UNIT()
SI_UNIT($,.RADIAN.)
);
#105810=(
NAMED_UNIT(*)
SI_UNIT($,.STERADIAN.)
SOLID_ANGLE_UNIT()
);
#105815=SHAPE_DEFINITION_REPRESENTATION(#105828,#105862);
#105828=PRODUCT_DEFINITION_SHAPE('',$,#105876);
#105862=SHAPE_REPRESENTATION('',(#7398),#105797);
#105871=PRODUCT_DEFINITION_CONTEXT('part definition',#105912,'design');
#105876=PRODUCT_DEFINITION('Clamping spindle','Clamping spindle',#105889,
#105871);
#105889=PRODUCT_DEFINITION_FORMATION('',$,#105918);
#105912=APPLICATION_CONTEXT(
'Core Data for Automotive Mechanical Design Process');
#105913=PRODUCT_CONTEXT('part definition',#105912,'mechanical');
#105918=PRODUCT('Clamping spindle','Clamping spindle',$,(#105913));
#105931=PRESENTATION_STYLE_ASSIGNMENT((#105937));
#105937=SURFACE_STYLE_USAGE(.BOTH.,#105943);
#105943=SURFACE_SIDE_STYLE('',(#105949));
#105949=SURFACE_STYLE_FILL_AREA(#105955);
#105955=FILL_AREA_STYLE('Opaque(23,69,131)',(#105961));
#105961=FILL_AREA_STYLE_COLOUR('Opaque(23,69,131)',#105967);
#105967=COLOUR_RGB('Opaque(23,69,131)',0.0901960784313725,0.270588235294118,
0.513725490196078);
ENDSEC;
END-ISO-10303-21;
